#94780=CARTESIAN_POINT('Ctrl Pts',(-36.0397189421617,60.4806895737643,0.));
#94781=CARTESIAN_POINT('Ctrl Pts',(-36.0397189421617,60.4806895737643,12.));
#94782=CARTESIAN_POINT('Ctrl Pts',(-36.0547232187681,60.4947416988396,0.));
#94783=CARTESIAN_POINT('Ctrl Pts',(-36.0547232187681,60.4947416988396,12.));
#94784=CARTESIAN_POINT('Ctrl Pts',(-36.0697797118377,60.5088129911357,0.));
#94785=CARTESIAN_POINT('Ctrl Pts',(-36.0697797118377,60.5088129911357,12.));
#94786=CARTESIAN_POINT('Ctrl Pts',(-36.0848883531968,60.5229032759001,0.));
#94787=CARTESIAN_POINT('Ctrl Pts',(-36.0848883531968,60.5229032759001,12.));
#94788=CARTESIAN_POINT('Ctrl Pts',(-36.1000490738532,60.5370123768841,0.));
#94789=CARTESIAN_POINT('Ctrl Pts',(-36.1000490738532,60.5370123768841,12.));
#94790=CARTESIAN_POINT('Ctrl Pts',(-36.1152618043756,60.5511401172014,0.));
#94791=CARTESIAN_POINT('Ctrl Pts',(-36.1152618043756,60.5511401172014,12.));
#94792=CARTESIAN_POINT('Ctrl Pts',(-36.1305264752195,60.5652863200732,0.));
#94793=CARTESIAN_POINT('Ctrl Pts',(-36.1305264752195,60.5652863200732,12.));
#94794=CARTESIAN_POINT('Ctrl Pts',(-36.1458430170425,60.5794508095555,0.));
#94795=CARTESIAN_POINT('Ctrl Pts',(-36.1458430170425,60.5794508095555,12.));
#94796=CARTESIAN_POINT('Ctrl Pts',(-36.1612113610758,60.5936334114083,0.));
#94797=CARTESIAN_POINT('Ctrl Pts',(-36.1612113610758,60.5936334114083,12.));
#94798=CARTESIAN_POINT('Ctrl Pts',(-36.1766314392624,60.6078339534151,0.));
#94799=CARTESIAN_POINT('Ctrl Pts',(-36.1766314392624,60.6078339534151,12.));
#94800=CARTESIAN_POINT('Ctrl Pts',(-36.1921031840617,60.6220522649129,0.));
#94801=CARTESIAN_POINT('Ctrl Pts',(-36.1921031840617,60.6220522649129,12.));
#94802=CARTESIAN_POINT('Ctrl Pts',(-36.2076265283261,60.6362881765014,0.));
#94803=CARTESIAN_POINT('Ctrl Pts',(-36.2076265283261,60.6362881765014,12.));
#94804=CARTESIAN_POINT('Ctrl Pts',(-36.2232014051549,60.6505415197055,0.));
#94805=CARTESIAN_POINT('Ctrl Pts',(-36.2232014051549,60.6505415197055,12.));
#94806=CARTESIAN_POINT('Ctrl Pts',(-36.2388277477225,60.6648121265908,0.));
#94807=CARTESIAN_POINT('Ctrl Pts',(-36.2388277477225,60.6648121265908,12.));
#94808=CARTESIAN_POINT('Ctrl Pts',(-36.2545054892911,60.6790998297823,0.));
#94809=CARTESIAN_POINT('Ctrl Pts',(-36.2545054892911,60.6790998297823,12.));
#94810=CARTESIAN_POINT('Ctrl Pts',(-36.2702345632882,60.6934044626304,0.));
#94811=CARTESIAN_POINT('Ctrl Pts',(-36.2702345632882,60.6934044626304,12.));
#94812=CARTESIAN_POINT('Ctrl Pts',(-36.2860149033586,60.7077258593268,0.));
#94813=CARTESIAN_POINT('Ctrl Pts',(-36.2860149033586,60.7077258593268,12.));
#94814=CARTESIAN_POINT('Ctrl Pts',(-36.3018464434204,60.7220638550396,0.));
#94815=CARTESIAN_POINT('Ctrl Pts',(-36.3018464434204,60.7220638550396,12.));
#94816=CARTESIAN_POINT('Ctrl Pts',(-36.3177291177148,60.7364182860388,0.));
#94817=CARTESIAN_POINT('Ctrl Pts',(-36.3177291177148,60.7364182860388,12.));
#94818=CARTESIAN_POINT('Ctrl Pts',(-36.3336628607844,60.7507889896283,0.));
#94819=CARTESIAN_POINT('Ctrl Pts',(-36.3336628607844,60.7507889896283,12.));
#94820=CARTESIAN_POINT('Ctrl Pts',(-36.349647607448,60.7651758040791,0.));
#94821=CARTESIAN_POINT('Ctrl Pts',(-36.349647607448,60.7651758040791,12.));
#94822=CARTESIAN_POINT('Ctrl Pts',(-36.3656832927733,60.7795785685631,0.));
#94823=CARTESIAN_POINT('Ctrl Pts',(-36.3656832927733,60.7795785685631,12.));
#94824=CARTESIAN_POINT('Ctrl Pts',(-36.38176985204,60.7939971230781,0.));
#94825=CARTESIAN_POINT('Ctrl Pts',(-36.38176985204,60.7939971230781,12.));
#94826=CARTESIAN_POINT('Ctrl Pts',(-36.3979072207174,60.8084313084009,0.));
#94827=CARTESIAN_POINT('Ctrl Pts',(-36.3979072207174,60.8084313084009,12.));
#94828=CARTESIAN_POINT('Ctrl Pts',(-36.4140953344869,60.8228809661179,0.));
#94829=CARTESIAN_POINT('Ctrl Pts',(-36.4140953344869,60.8228809661179,12.));
#94830=CARTESIAN_POINT('Ctrl Pts',(-36.4303341292497,60.8373459386397,0.));
#94831=CARTESIAN_POINT('Ctrl Pts',(-36.4303341292497,60.8373459386397,12.));
#94832=CARTESIAN_POINT('Ctrl Pts',(-36.4466235411353,60.851826069218,0.));
#94833=CARTESIAN_POINT('Ctrl Pts',(-36.4466235411353,60.851826069218,12.));
#94834=CARTESIAN_POINT('Ctrl Pts',(-36.4629635065037,60.8663212019646,0.));
#94835=CARTESIAN_POINT('Ctrl Pts',(-36.4629635065037,60.8663212019646,12.));
#94836=CARTESIAN_POINT('Ctrl Pts',(-36.4793539619459,60.8808311818489,0.));
#94837=CARTESIAN_POINT('Ctrl Pts',(-36.4793539619459,60.8808311818489,12.));
#94838=CARTESIAN_POINT('Ctrl Pts',(-36.4957948442832,60.8953558546791,0.));
#94839=CARTESIAN_POINT('Ctrl Pts',(-36.4957948442832,60.8953558546791,12.));
#94840=CARTESIAN_POINT('Ctrl Pts',(-36.5122860905611,60.9098950670847,0.));
#94841=CARTESIAN_POINT('Ctrl Pts',(-36.5122860905611,60.9098950670847,12.));
#94842=CARTESIAN_POINT('Ctrl Pts',(-36.5288276380417,60.924448666499,0.));
#94843=CARTESIAN_POINT('Ctrl Pts',(-36.5288276380417,60.924448666499,12.));
#94844=CARTESIAN_POINT('Ctrl Pts',(-36.5454194241866,60.9390165011357,0.));
#94845=CARTESIAN_POINT('Ctrl Pts',(-36.5454194241866,60.9390165011357,12.));
#94846=CARTESIAN_POINT('Ctrl Pts',(-36.5620613866615,60.9535984199874,0.));
#94847=CARTESIAN_POINT('Ctrl Pts',(-36.5620613866615,60.9535984199874,12.));
#94848=CARTESIAN_POINT('Ctrl Pts',(-36.5787534633416,60.9681942728237,0.));
#94849=CARTESIAN_POINT('Ctrl Pts',(-36.5787534633416,60.9681942728237,12.));
#94850=CARTESIAN_POINT('Ctrl Pts',(-36.5954955923109,60.9828039101887,0.));
#94851=CARTESIAN_POINT('Ctrl Pts',(-36.5954955923109,60.9828039101887,12.));
#94852=CARTESIAN_POINT('Ctrl Pts',(-36.6122877118599,60.9974271833982,0.));
#94853=CARTESIAN_POINT('Ctrl Pts',(-36.6122877118599,60.9974271833982,12.));
#94854=CARTESIAN_POINT('Ctrl Pts',(-36.6291297604775,61.012063944535,0.));
#94855=CARTESIAN_POINT('Ctrl Pts',(-36.6291297604775,61.012063944535,12.));
#94856=CARTESIAN_POINT('Ctrl Pts',(-36.6460216768553,61.0267140464434,0.));
#94857=CARTESIAN_POINT('Ctrl Pts',(-36.6460216768553,61.0267140464434,12.));
#94858=CARTESIAN_POINT('Ctrl Pts',(-36.6629633998885,61.0413773427204,0.));
#94859=CARTESIAN_POINT('Ctrl Pts',(-36.6629633998885,61.0413773427204,12.));
#94860=CARTESIAN_POINT('Ctrl Pts',(-36.6799548686741,61.0560536877084,0.));
#94861=CARTESIAN_POINT('Ctrl Pts',(-36.6799548686741,61.0560536877084,12.));
#94862=CARTESIAN_POINT('Ctrl Pts',(-36.6969960225019,61.0707429364841,0.));
#94863=CARTESIAN_POINT('Ctrl Pts',(-36.6969960225019,61.0707429364841,12.));
#94864=CARTESIAN_POINT('Ctrl Pts',(-36.7140868008479,61.085444944851,0.));
#94865=CARTESIAN_POINT('Ctrl Pts',(-36.7140868008479,61.085444944851,12.));
#94866=CARTESIAN_POINT('Ctrl Pts',(-36.7312271433799,61.1001595693357,0.));
#94867=CARTESIAN_POINT('Ctrl Pts',(-36.7312271433799,61.1001595693357,12.));
#94868=CARTESIAN_POINT('Ctrl Pts',(-36.7484169899591,61.1148866671821,0.));
#94869=CARTESIAN_POINT('Ctrl Pts',(-36.7484169899591,61.1148866671821,12.));
#94870=CARTESIAN_POINT('Ctrl Pts',(-36.7656562806381,61.1296260963468,0.));
#94871=CARTESIAN_POINT('Ctrl Pts',(-36.7656562806381,61.1296260963468,12.));
#94872=CARTESIAN_POINT('Ctrl Pts',(-36.782944955654,61.1443777154926,0.));
#94873=CARTESIAN_POINT('Ctrl Pts',(-36.782944955654,61.1443777154926,12.));
#94874=CARTESIAN_POINT('Ctrl Pts',(-36.8002829554221,61.1591413839809,0.));
#94875=CARTESIAN_POINT('Ctrl Pts',(-36.8002829554221,61.1591413839809,12.));
#94876=CARTESIAN_POINT('Ctrl Pts',(-36.8176702205436,61.1739169618688,0.));
#94877=CARTESIAN_POINT('Ctrl Pts',(-36.8176702205436,61.1739169618688,12.));
#94878=CARTESIAN_POINT('Ctrl Pts',(-36.8351066918043,61.1887043099026,0.));
#94879=CARTESIAN_POINT('Ctrl Pts',(-36.8351066918043,61.1887043099026,12.));
#94880=CARTESIAN_POINT('Ctrl Pts',(-36.8525923101736,61.2035032895121,0.));
#94881=CARTESIAN_POINT('Ctrl Pts',(-36.8525923101736,61.2035032895121,12.));
#94882=CARTESIAN_POINT('Ctrl Pts',(-36.8701270167954,61.2183137628031,0.));
#94883=CARTESIAN_POINT('Ctrl Pts',(-36.8701270167954,61.2183137628031,12.));
#94884=CARTESIAN_POINT('Ctrl Pts',(-36.8877107529844,61.2331355925513,0.));
#94885=CARTESIAN_POINT('Ctrl Pts',(-36.8877107529844,61.2331355925513,12.));
#94886=CARTESIAN_POINT('Ctrl Pts',(-36.9053434602324,61.2479686421979,0.));
#94887=CARTESIAN_POINT('Ctrl Pts',(-36.9053434602324,61.2479686421979,12.));
#94888=CARTESIAN_POINT('Ctrl Pts',(-36.9230250802078,61.2628127758443,0.));
#94889=CARTESIAN_POINT('Ctrl Pts',(-36.9230250802078,61.2628127758443,12.));
#94890=CARTESIAN_POINT('Ctrl Pts',(-36.9407555547542,61.2776678582474,0.));
#94891=CARTESIAN_POINT('Ctrl Pts',(-36.9407555547542,61.2776678582474,12.));
#94892=CARTESIAN_POINT('Ctrl Pts',(-36.9585348258798,61.2925337548113,0.));
#94893=CARTESIAN_POINT('Ctrl Pts',(-36.9585348258798,61.2925337548113,12.));
#94894=CARTESIAN_POINT('Ctrl Pts',(-36.976362835757,61.3074103315834,0.));
#94895=CARTESIAN_POINT('Ctrl Pts',(-36.976362835757,61.3074103315834,12.));
#94896=CARTESIAN_POINT('Ctrl Pts',(-36.994239526729,61.3222974552519,0.));
#94897=CARTESIAN_POINT('Ctrl Pts',(-36.994239526729,61.3222974552519,12.));
#94898=CARTESIAN_POINT('Ctrl Pts',(-37.0121648413088,61.3371949931396,0.));
#94899=CARTESIAN_POINT('Ctrl Pts',(-37.0121648413088,61.3371949931396,12.));
#94900=CARTESIAN_POINT('Ctrl Pts',(-37.0301387221766,61.352102813199,0.));
#94901=CARTESIAN_POINT('Ctrl Pts',(-37.0301387221766,61.352102813199,12.));
#94902=CARTESIAN_POINT('Ctrl Pts',(-37.0481611121698,61.3670207840041,0.));
#94903=CARTESIAN_POINT('Ctrl Pts',(-37.0481611121698,61.3670207840041,12.));
#94904=CARTESIAN_POINT('Ctrl Pts',(-37.0662319542827,61.3819487747458,0.));
#94905=CARTESIAN_POINT('Ctrl Pts',(-37.0662319542827,61.3819487747458,12.));
#94906=CARTESIAN_POINT('Ctrl Pts',(-37.0843511916728,61.3968866552294,0.));
#94907=CARTESIAN_POINT('Ctrl Pts',(-37.0843511916728,61.3968866552294,12.));
#94908=CARTESIAN_POINT('Ctrl Pts',(-37.1025187676597,61.411834295869,0.));
#94909=CARTESIAN_POINT('Ctrl Pts',(-37.1025187676597,61.411834295869,12.));
#94910=CARTESIAN_POINT('Ctrl Pts',(-37.1207346257228,61.4267915676834,0.));
#94911=CARTESIAN_POINT('Ctrl Pts',(-37.1207346257228,61.4267915676834,12.));
#94912=CARTESIAN_POINT('Ctrl Pts',(-37.138998709492,61.4417583422888,0.));
#94913=CARTESIAN_POINT('Ctrl Pts',(-37.138998709492,61.4417583422888,12.));
#94914=CARTESIAN_POINT('Ctrl Pts',(-37.157310962747,61.4567344918946,0.));
#94915=CARTESIAN_POINT('Ctrl Pts',(-37.157310962747,61.4567344918946,12.));
#94916=CARTESIAN_POINT('Ctrl Pts',(-37.1756713294249,61.471719889301,0.));
#94917=CARTESIAN_POINT('Ctrl Pts',(-37.1756713294249,61.471719889301,12.));
#94918=CARTESIAN_POINT('Ctrl Pts',(-37.1940797536182,61.4867144078939,0.));
#94919=CARTESIAN_POINT('Ctrl Pts',(-37.1940797536182,61.4867144078939,12.));
#94920=CARTESIAN_POINT('Ctrl Pts',(-37.2125361795727,61.5017179216404,0.));
#94921=CARTESIAN_POINT('Ctrl Pts',(-37.2125361795727,61.5017179216404,12.));
#94922=CARTESIAN_POINT('Ctrl Pts',(-37.2310405516775,61.5167303050823,0.));
#94923=CARTESIAN_POINT('Ctrl Pts',(-37.2310405516775,61.5167303050823,12.));
#94924=CARTESIAN_POINT('Ctrl Pts',(-37.2495928144661,61.5317514333319,0.));
#94925=CARTESIAN_POINT('Ctrl Pts',(-37.2495928144661,61.5317514333319,12.));
#94926=CARTESIAN_POINT('Ctrl Pts',(-37.2681929126218,61.5467811820686,0.));
#94927=CARTESIAN_POINT('Ctrl Pts',(-37.2681929126218,61.5467811820686,12.));
#94928=CARTESIAN_POINT('Ctrl Pts',(-37.286840790977,61.5618194275349,0.));
#94929=CARTESIAN_POINT('Ctrl Pts',(-37.286840790977,61.5618194275349,12.));
#94930=CARTESIAN_POINT('Ctrl Pts',(-37.3055363945108,61.5768660465313,0.));
#94931=CARTESIAN_POINT('Ctrl Pts',(-37.3055363945108,61.5768660465313,12.));
#94932=CARTESIAN_POINT('Ctrl Pts',(-37.3242796683395,61.591920916412,0.));
#94933=CARTESIAN_POINT('Ctrl Pts',(-37.3242796683395,61.591920916412,12.));
#94934=CARTESIAN_POINT('Ctrl Pts',(-37.3430705577178,61.6069839150804,0.));
#94935=CARTESIAN_POINT('Ctrl Pts',(-37.3430705577178,61.6069839150804,12.));
#94936=CARTESIAN_POINT('Ctrl Pts',(-37.3619090080447,61.6220549209862,0.));
#94937=CARTESIAN_POINT('Ctrl Pts',(-37.3619090080447,61.6220549209862,12.));
#94938=CARTESIAN_POINT('Ctrl Pts',(-37.3807949648622,61.6371338131208,0.));
#94939=CARTESIAN_POINT('Ctrl Pts',(-37.3807949648622,61.6371338131208,12.));
#94940=CARTESIAN_POINT('Ctrl Pts',(-37.3997283738534,61.6522204710133,0.));
#94941=CARTESIAN_POINT('Ctrl Pts',(-37.3997283738534,61.6522204710133,12.));
#94942=CARTESIAN_POINT('Ctrl Pts',(-37.4187091808324,61.667314774725,0.));
#94943=CARTESIAN_POINT('Ctrl Pts',(-37.4187091808324,61.667314774725,12.));
#94944=CARTESIAN_POINT('Ctrl Pts',(-37.4377373317456,61.6824166048453,0.));
#94945=CARTESIAN_POINT('Ctrl Pts',(-37.4377373317456,61.6824166048453,12.));
#94946=CARTESIAN_POINT('Ctrl Pts',(-37.4568127726776,61.69752584249,0.));
#94947=CARTESIAN_POINT('Ctrl Pts',(-37.4568127726776,61.69752584249,12.));
#94948=CARTESIAN_POINT('Ctrl Pts',(-37.4759354498509,61.7126423692965,0.));
#94949=CARTESIAN_POINT('Ctrl Pts',(-37.4759354498509,61.7126423692965,12.));
#94950=CARTESIAN_POINT('Ctrl Pts',(-37.4951053096235,61.7277660674203,0.));
#94951=CARTESIAN_POINT('Ctrl Pts',(-37.4951053096235,61.7277660674203,12.));
#94952=CARTESIAN_POINT('Ctrl Pts',(-37.5143222984794,61.7428968195296,0.));
#94953=CARTESIAN_POINT('Ctrl Pts',(-37.5143222984794,61.7428968195296,12.));
#94954=CARTESIAN_POINT('Ctrl Pts',(-37.5335863630286,61.7580345088014,0.));
#94955=CARTESIAN_POINT('Ctrl Pts',(-37.5335863630286,61.7580345088014,12.));
#94956=CARTESIAN_POINT('Ctrl Pts',(-37.5528974500142,61.7731790189191,0.));
#94957=CARTESIAN_POINT('Ctrl Pts',(-37.5528974500142,61.7731790189191,12.));
#94958=CARTESIAN_POINT('Ctrl Pts',(-37.5722555063112,61.7883302340689,0.));
#94959=CARTESIAN_POINT('Ctrl Pts',(-37.5722555063112,61.7883302340689,12.));
#94960=CARTESIAN_POINT('Ctrl Pts',(-37.5916604789252,61.8034880389362,0.));
#94961=CARTESIAN_POINT('Ctrl Pts',(-37.5916604789252,61.8034880389362,12.));
#94962=CARTESIAN_POINT('Ctrl Pts',(-37.6111123149836,61.8186523187011,0.));
#94963=CARTESIAN_POINT('Ctrl Pts',(-37.6111123149836,61.8186523187011,12.));
#94964=CARTESIAN_POINT('Ctrl Pts',(-37.6306109617341,61.8338229590345,0.));
#94965=CARTESIAN_POINT('Ctrl Pts',(-37.6306109617341,61.8338229590345,12.));
#94966=CARTESIAN_POINT('Ctrl Pts',(-37.6501563665518,61.848999846095,0.));
#94967=CARTESIAN_POINT('Ctrl Pts',(-37.6501563665518,61.848999846095,12.));
#94968=CARTESIAN_POINT('Ctrl Pts',(-37.6697484769389,61.8641828665257,0.));
#94969=CARTESIAN_POINT('Ctrl Pts',(-37.6697484769389,61.8641828665257,12.));
#94970=CARTESIAN_POINT('Ctrl Pts',(-37.6893872405229,61.879371907451,0.));
#94971=CARTESIAN_POINT('Ctrl Pts',(-37.6893872405229,61.879371907451,12.));
#94972=CARTESIAN_POINT('Ctrl Pts',(-37.7090726050488,61.8945668564714,0.));
#94973=CARTESIAN_POINT('Ctrl Pts',(-37.7090726050488,61.8945668564714,12.));
#94974=CARTESIAN_POINT('Ctrl Pts',(-37.7288045183765,61.9097676016616,0.));
#94975=CARTESIAN_POINT('Ctrl Pts',(-37.7288045183765,61.9097676016616,12.));
#94976=CARTESIAN_POINT('Ctrl Pts',(-37.748582928488,61.9249740315664,0.));
#94977=CARTESIAN_POINT('Ctrl Pts',(-37.748582928488,61.9249740315664,12.));
#94978=CARTESIAN_POINT('Ctrl Pts',(-37.7684077834877,61.940186035198,0.));
#94979=CARTESIAN_POINT('Ctrl Pts',(-37.7684077834877,61.940186035198,12.));
#94980=CARTESIAN_POINT('Ctrl Pts',(-37.7882790316012,61.9554035020335,0.));
#94981=CARTESIAN_POINT('Ctrl Pts',(-37.7882790316012,61.9554035020335,12.));
#94982=CARTESIAN_POINT('Ctrl Pts',(-37.808196621168,61.9706263220101,0.));
#94983=CARTESIAN_POINT('Ctrl Pts',(-37.808196621168,61.9706263220101,12.));
#94984=CARTESIAN_POINT('Ctrl Pts',(-37.8281605006371,61.9858543855221,0.));
#94985=CARTESIAN_POINT('Ctrl Pts',(-37.8281605006371,61.9858543855221,12.));
#94986=CARTESIAN_POINT('Ctrl Pts',(-37.8481706185742,62.0010875834176,0.));
#94987=CARTESIAN_POINT('Ctrl Pts',(-37.8481706185742,62.0010875834176,12.));
#94988=CARTESIAN_POINT('Ctrl Pts',(-37.8682269236628,62.0163258069954,0.));
#94989=CARTESIAN_POINT('Ctrl Pts',(-37.8682269236628,62.0163258069954,12.));
#94990=CARTESIAN_POINT('Ctrl Pts',(-37.888329364703,62.0315689480022,0.));
#94991=CARTESIAN_POINT('Ctrl Pts',(-37.888329364703,62.0315689480022,12.));
#94992=CARTESIAN_POINT('Ctrl Pts',(-37.9084778906053,62.0468168986289,0.));
#94993=CARTESIAN_POINT('Ctrl Pts',(-37.9084778906053,62.0468168986289,12.));
#94994=CARTESIAN_POINT('Ctrl Pts',(-37.9286724503849,62.0620695515072,0.));
#94995=CARTESIAN_POINT('Ctrl Pts',(-37.9286724503849,62.0620695515072,12.));
#94996=CARTESIAN_POINT('Ctrl Pts',(-37.9489129931685,62.0773267997072,0.));
#94997=CARTESIAN_POINT('Ctrl Pts',(-37.9489129931685,62.0773267997072,12.));
#94998=CARTESIAN_POINT('Ctrl Pts',(-37.9691994681962,62.0925885367346,0.));
#94999=CARTESIAN_POINT('Ctrl Pts',(-37.9691994681962,62.0925885367346,12.));
#95000=CARTESIAN_POINT('Ctrl Pts',(-37.9895318248212,62.107854656528,0.));
#95001=CARTESIAN_POINT('Ctrl Pts',(-37.9895318248212,62.107854656528,12.));
#95002=CARTESIAN_POINT('Ctrl Pts',(-38.0099100125041,62.1231250534558,0.));
#95003=CARTESIAN_POINT('Ctrl Pts',(-38.0099100125041,62.1231250534558,12.));
#95004=CARTESIAN_POINT('Ctrl Pts',(-38.0303339808059,62.1383996223136,0.));
#95005=CARTESIAN_POINT('Ctrl Pts',(-38.0303339808059,62.1383996223136,12.));
#95006=CARTESIAN_POINT('Ctrl Pts',(-38.0508036793944,62.153678258321,0.));
#95007=CARTESIAN_POINT('Ctrl Pts',(-38.0508036793944,62.153678258321,12.));
#95008=CARTESIAN_POINT('Ctrl Pts',(-38.0713190580466,62.1689608571182,0.));
#95009=CARTESIAN_POINT('Ctrl Pts',(-38.0713190580466,62.1689608571182,12.));
#95010=CARTESIAN_POINT('Ctrl Pts',(-38.0918800666479,62.1842473147627,0.));
#95011=CARTESIAN_POINT('Ctrl Pts',(-38.0918800666479,62.1842473147627,12.));
#95012=CARTESIAN_POINT('Ctrl Pts',(-38.1124866551883,62.1995375277253,0.));
#95013=CARTESIAN_POINT('Ctrl Pts',(-38.1124866551883,62.1995375277253,12.));
#95014=CARTESIAN_POINT('Ctrl Pts',(-38.1331387737528,62.2148313928859,0.));
#95015=CARTESIAN_POINT('Ctrl Pts',(-38.1331387737528,62.2148313928859,12.));
#95016=CARTESIAN_POINT('Ctrl Pts',(-38.1538363725263,62.2301288075319,0.));
#95017=CARTESIAN_POINT('Ctrl Pts',(-38.1538363725263,62.2301288075319,12.));
#95018=CARTESIAN_POINT('Ctrl Pts',(-38.1745794017997,62.2454296693581,0.));
#95019=CARTESIAN_POINT('Ctrl Pts',(-38.1745794017997,62.2454296693581,12.));
#95020=CARTESIAN_POINT('Ctrl Pts',(-38.1953678119692,62.2607338764655,0.));
#95021=CARTESIAN_POINT('Ctrl Pts',(-38.1953678119692,62.2607338764655,12.));
#95022=CARTESIAN_POINT('Ctrl Pts',(-38.2162015535351,62.2760413273601,0.));
#95023=CARTESIAN_POINT('Ctrl Pts',(-38.2162015535351,62.2760413273601,12.));
#95024=CARTESIAN_POINT('Ctrl Pts',(-38.2370805770931,62.2913519209517,0.));
#95025=CARTESIAN_POINT('Ctrl Pts',(-38.2370805770931,62.2913519209517,12.));
#95026=CARTESIAN_POINT('Ctrl Pts',(-38.2580048333356,62.3066655565497,0.));
#95027=CARTESIAN_POINT('Ctrl Pts',(-38.2580048333356,62.3066655565497,12.));
#95028=CARTESIAN_POINT('Ctrl Pts',(-38.2789742730559,62.3219821338564,0.));
#95029=CARTESIAN_POINT('Ctrl Pts',(-38.2789742730559,62.3219821338564,12.));
#95030=CARTESIAN_POINT('Ctrl Pts',(-38.2999888471474,62.337301552961,0.));
#95031=CARTESIAN_POINT('Ctrl Pts',(-38.2999888471474,62.337301552961,12.));
#95032=CARTESIAN_POINT('Ctrl Pts',(-38.3210485066003,62.3526237143338,0.));
#95033=CARTESIAN_POINT('Ctrl Pts',(-38.3210485066003,62.3526237143338,12.));
#95034=CARTESIAN_POINT('Ctrl Pts',(-38.3421532024915,62.3679485188178,0.));
#95035=CARTESIAN_POINT('Ctrl Pts',(-38.3421532024915,62.3679485188178,12.));
#95036=CARTESIAN_POINT('Ctrl Pts',(-38.3633028859835,62.3832758676281,0.));
#95037=CARTESIAN_POINT('Ctrl Pts',(-38.3633028859835,62.3832758676281,12.));
#95038=CARTESIAN_POINT('Ctrl Pts',(-38.384497508335,62.3986056623587,0.));
#95039=CARTESIAN_POINT('Ctrl Pts',(-38.384497508335,62.3986056623587,12.));
#95040=CARTESIAN_POINT('Ctrl Pts',(-38.4057370209054,62.4139378049891,0.));
#95041=CARTESIAN_POINT('Ctrl Pts',(-38.4057370209054,62.4139378049891,12.));
#95042=CARTESIAN_POINT('Ctrl Pts',(-38.4270213751567,62.42927219789,0.));
#95043=CARTESIAN_POINT('Ctrl Pts',(-38.4270213751567,62.42927219789,12.));
#95044=CARTESIAN_POINT('Ctrl Pts',(-38.4483505226511,62.4446087438304,0.));
#95045=CARTESIAN_POINT('Ctrl Pts',(-38.4483505226511,62.4446087438304,12.));
#95046=CARTESIAN_POINT('Ctrl Pts',(-38.4697244150473,62.4599473459799,0.));
#95047=CARTESIAN_POINT('Ctrl Pts',(-38.4697244150473,62.4599473459799,12.));
#95048=CARTESIAN_POINT('Ctrl Pts',(-38.4911430040988,62.4752879078842,0.));
#95049=CARTESIAN_POINT('Ctrl Pts',(-38.4911430040988,62.4752879078842,12.));
#95050=CARTESIAN_POINT('Ctrl Pts',(-38.5126062416496,62.4906303334435,0.));
#95051=CARTESIAN_POINT('Ctrl Pts',(-38.5126062416496,62.4906303334435,12.));
#95052=CARTESIAN_POINT('Ctrl Pts',(-38.5341140796247,62.50597452689,0.));
#95053=CARTESIAN_POINT('Ctrl Pts',(-38.5341140796247,62.50597452689,12.));
#95054=CARTESIAN_POINT('Ctrl Pts',(-38.5556664700201,62.5213203927672,0.));
#95055=CARTESIAN_POINT('Ctrl Pts',(-38.5556664700201,62.5213203927672,12.));
#95056=CARTESIAN_POINT('Ctrl Pts',(-38.5772633648841,62.5366678359036,0.));
#95057=CARTESIAN_POINT('Ctrl Pts',(-38.5772633648841,62.5366678359036,12.));
#95058=CARTESIAN_POINT('Ctrl Pts',(-38.5989047163401,62.5520167614529,0.));
#95059=CARTESIAN_POINT('Ctrl Pts',(-38.5989047163401,62.5520167614529,12.));
#95060=CARTESIAN_POINT('Ctrl Pts',(-38.6205904766078,62.567367074937,0.));
#95061=CARTESIAN_POINT('Ctrl Pts',(-38.6205904766078,62.567367074937,12.));
#95062=CARTESIAN_POINT('Ctrl Pts',(-38.6423205980214,62.5827186822923,0.));
#95063=CARTESIAN_POINT('Ctrl Pts',(-38.6423205980214,62.5827186822923,12.));
#95064=CARTESIAN_POINT('Ctrl Pts',(-38.6640950330418,62.5980714899048,0.));
#95065=CARTESIAN_POINT('Ctrl Pts',(-38.6640950330418,62.5980714899048,12.));
#95066=CARTESIAN_POINT('Ctrl Pts',(-38.6859137342726,62.6134254046732,0.));
#95067=CARTESIAN_POINT('Ctrl Pts',(-38.6859137342726,62.6134254046732,12.));
#95068=CARTESIAN_POINT('Ctrl Pts',(-38.7077766544411,62.6287803339534,0.));
#95069=CARTESIAN_POINT('Ctrl Pts',(-38.7077766544411,62.6287803339534,12.));
#95070=CARTESIAN_POINT('Ctrl Pts',(-38.7296837463605,62.6441361854406,0.));
#95071=CARTESIAN_POINT('Ctrl Pts',(-38.7296837463605,62.6441361854406,12.));
#95072=CARTESIAN_POINT('Ctrl Pts',(-38.7516349628902,62.6594928670626,0.));
#95073=CARTESIAN_POINT('Ctrl Pts',(-38.7516349628902,62.6594928670626,12.));
#95074=CARTESIAN_POINT('Ctrl Pts',(-38.7736302568982,62.6748502868836,0.));
#95075=CARTESIAN_POINT('Ctrl Pts',(-38.7736302568982,62.6748502868836,12.));
#95076=CARTESIAN_POINT('Ctrl Pts',(-38.7956695812032,62.6902083529698,0.));
#95077=CARTESIAN_POINT('Ctrl Pts',(-38.7956695812032,62.6902083529698,12.));
#95078=CARTESIAN_POINT('Ctrl Pts',(-38.8177528885686,62.7055669733811,0.));
#95079=CARTESIAN_POINT('Ctrl Pts',(-38.8177528885686,62.7055669733811,12.));
#95080=CARTESIAN_POINT('Ctrl Pts',(-38.8398801318184,62.7209260564506,0.));
#95081=CARTESIAN_POINT('Ctrl Pts',(-38.8398801318184,62.7209260564506,12.));
#95082=CARTESIAN_POINT('Ctrl Pts',(-38.8620512639239,62.7362855110052,0.));
#95083=CARTESIAN_POINT('Ctrl Pts',(-38.8620512639239,62.7362855110052,12.));
#95084=CARTESIAN_POINT('Ctrl Pts',(-38.8842662380984,62.7516452466129,0.));
#95085=CARTESIAN_POINT('Ctrl Pts',(-38.8842662380984,62.7516452466129,12.));
#95086=CARTESIAN_POINT('Ctrl Pts',(-38.9065250078824,62.7670051738132,0.));
#95087=CARTESIAN_POINT('Ctrl Pts',(-38.9065250078824,62.7670051738132,12.));
#95088=CARTESIAN_POINT('Ctrl Pts',(-38.928827527232,62.7823652043677,0.));
#95089=CARTESIAN_POINT('Ctrl Pts',(-38.928827527232,62.7823652043677,12.));
#95090=CARTESIAN_POINT('Ctrl Pts',(-38.9511737503146,62.797725250709,0.));
#95091=CARTESIAN_POINT('Ctrl Pts',(-38.9511737503146,62.797725250709,12.));
#95092=CARTESIAN_POINT('Ctrl Pts',(-38.9735636313073,62.8130852254004,0.));
#95093=CARTESIAN_POINT('Ctrl Pts',(-38.9735636313073,62.8130852254004,12.));
#95094=CARTESIAN_POINT('Ctrl Pts',(-38.9959971241695,62.8284450405451,0.));
#95095=CARTESIAN_POINT('Ctrl Pts',(-38.9959971241695,62.8284450405451,12.));
#95096=CARTESIAN_POINT('Ctrl Pts',(-39.0184741824649,62.8438046073237,0.));
#95097=CARTESIAN_POINT('Ctrl Pts',(-39.0184741824649,62.8438046073237,12.));
#95098=CARTESIAN_POINT('Ctrl Pts',(-39.0409947590519,62.859163835209,0.));
#95099=CARTESIAN_POINT('Ctrl Pts',(-39.0409947590519,62.859163835209,12.));
#95100=CARTESIAN_POINT('Ctrl Pts',(-39.0635588063308,62.8745226326046,0.));
#95101=CARTESIAN_POINT('Ctrl Pts',(-39.0635588063308,62.8745226326046,12.));
#95102=CARTESIAN_POINT('Ctrl Pts',(-39.0861662767964,62.8898809082659,0.));
#95103=CARTESIAN_POINT('Ctrl Pts',(-39.0861662767964,62.8898809082659,12.));
#95104=CARTESIAN_POINT('Ctrl Pts',(-39.1088171235144,62.9052385725416,0.));
#95105=CARTESIAN_POINT('Ctrl Pts',(-39.1088171235144,62.9052385725416,12.));
#95106=CARTESIAN_POINT('Ctrl Pts',(-39.1315113005745,62.9205955385551,0.));
#95107=CARTESIAN_POINT('Ctrl Pts',(-39.1315113005745,62.9205955385551,12.));
#95108=CARTESIAN_POINT('Ctrl Pts',(-39.1542487636708,62.9359517237352,0.));
#95109=CARTESIAN_POINT('Ctrl Pts',(-39.1542487636708,62.9359517237352,12.));
#95110=CARTESIAN_POINT('Ctrl Pts',(-39.1770294702367,62.9513070501777,0.));
#95111=CARTESIAN_POINT('Ctrl Pts',(-39.1770294702367,62.9513070501777,12.));
#95112=CARTESIAN_POINT('Ctrl Pts',(-39.199853378159,62.9666614412627,0.));
#95113=CARTESIAN_POINT('Ctrl Pts',(-39.199853378159,62.9666614412627,12.));
#95114=CARTESIAN_POINT('Ctrl Pts',(-39.2227204447583,62.9820148189849,0.));
#95115=CARTESIAN_POINT('Ctrl Pts',(-39.2227204447583,62.9820148189849,12.));
#95116=CARTESIAN_POINT('Ctrl Pts',(-39.2456306256092,62.9973671008685,0.));
#95117=CARTESIAN_POINT('Ctrl Pts',(-39.2456306256092,62.9973671008685,12.));
#95118=CARTESIAN_POINT('Ctrl Pts',(-39.268583873541,63.0127181973702,0.));
#95119=CARTESIAN_POINT('Ctrl Pts',(-39.268583873541,63.0127181973702,12.));
#95120=CARTESIAN_POINT('Ctrl Pts',(-39.2915801372468,63.0280680082522,0.));
#95121=CARTESIAN_POINT('Ctrl Pts',(-39.2915801372468,63.0280680082522,12.));
#95122=CARTESIAN_POINT('Ctrl Pts',(-39.3146193632546,63.0434164278221,0.));
#95123=CARTESIAN_POINT('Ctrl Pts',(-39.3146193632546,63.0434164278221,12.));
#95124=CARTESIAN_POINT('Ctrl Pts',(-39.3377014983757,63.0587633513993,0.));
#95125=CARTESIAN_POINT('Ctrl Pts',(-39.3377014983757,63.0587633513993,12.));
#95126=CARTESIAN_POINT('Ctrl Pts',(-39.3608264920487,63.0741086815957,0.));
#95127=CARTESIAN_POINT('Ctrl Pts',(-39.3608264920487,63.0741086815957,12.));
#95128=CARTESIAN_POINT('Ctrl Pts',(-39.3839942985688,63.0894523341238,0.));
#95129=CARTESIAN_POINT('Ctrl Pts',(-39.3839942985688,63.0894523341238,12.));
#95130=CARTESIAN_POINT('Ctrl Pts',(-39.4072048797401,63.1047942451583,0.));
#95131=CARTESIAN_POINT('Ctrl Pts',(-39.4072048797401,63.1047942451583,12.));
#95132=CARTESIAN_POINT('Ctrl Pts',(-39.4304582059507,63.1201343730643,0.));
#95133=CARTESIAN_POINT('Ctrl Pts',(-39.4304582059507,63.1201343730643,12.));
#95134=CARTESIAN_POINT('Ctrl Pts',(-39.4537542551852,63.1354726927781,0.));
#95135=CARTESIAN_POINT('Ctrl Pts',(-39.4537542551852,63.1354726927781,12.));
#95136=CARTESIAN_POINT('Ctrl Pts',(-39.4724252610807,63.147741892189,0.));
#95137=CARTESIAN_POINT('Ctrl Pts',(-39.4724252610807,63.147741892189,12.));
#95138=CARTESIAN_POINT('Ctrl Pts',(-39.4864477303613,63.1569429707564,0.));
#95139=CARTESIAN_POINT('Ctrl Pts',(-39.4864477303613,63.1569429707564,12.));
#95140=CARTESIAN_POINT('Ctrl Pts',(-39.4958045828059,63.1630766582674,0.));
#95141=CARTESIAN_POINT('Ctrl Pts',(-39.4958045828059,63.1630766582674,12.));
#95142=CARTESIAN_POINT('Ctrl Pts',(-39.5004851439257,63.1661434108059,0.));
#95143=CARTESIAN_POINT('Ctrl Pts',(-39.5004851439257,63.1661434108059,12.));
#95144=CARTESIAN_POINT('',(-35.7368311217509,60.1903555511633,0.));
#95145=CARTESIAN_POINT('Ctrl Pts',(-35.7368311217509,60.1903555511633,0.));
#95146=CARTESIAN_POINT('Ctrl Pts',(-35.7396040203973,60.1930746580239,0.));
#95147=CARTESIAN_POINT('Ctrl Pts',(-35.7451551752456,60.1985151474406,0.));
#95148=CARTESIAN_POINT('Ctrl Pts',(-35.7534979801871,60.2066827086579,0.));
#95149=CARTESIAN_POINT('Ctrl Pts',(-35.7646538667299,60.2175864449678,0.));
#95150=CARTESIAN_POINT('Ctrl Pts',(-35.7786523045782,60.2312388621286,0.));
#95151=CARTESIAN_POINT('Ctrl Pts',(-35.7927043145164,60.2449139865206,0.));
#95152=CARTESIAN_POINT('Ctrl Pts',(-35.8068098723386,60.2586117365278,0.));
#95153=CARTESIAN_POINT('Ctrl Pts',(-35.8209689272574,60.2723319687507,0.));
#95154=CARTESIAN_POINT('Ctrl Pts',(-35.8351814020424,60.2860744798563,0.));
#95155=CARTESIAN_POINT('Ctrl Pts',(-35.8494472046783,60.2998390330173,0.));
#95156=CARTESIAN_POINT('Ctrl Pts',(-35.8637662371635,60.313625378281,0.));
#95157=CARTESIAN_POINT('Ctrl Pts',(-35.878138405151,60.3274332746782,0.));
#95158=CARTESIAN_POINT('Ctrl Pts',(-35.8925636280632,60.3412625135223,0.));
#95159=CARTESIAN_POINT('Ctrl Pts',(-35.9070418358501,60.3551129108794,0.));
#95160=CARTESIAN_POINT('Ctrl Pts',(-35.9215729642219,60.368984296546,0.));
#95161=CARTESIAN_POINT('Ctrl Pts',(-35.9361569506955,60.3828765049031,0.));
#95162=CARTESIAN_POINT('Ctrl Pts',(-35.9507937296726,60.3967893635487,0.));
#95163=CARTESIAN_POINT('Ctrl Pts',(-35.9654832299627,60.4107226875759,0.));
#95164=CARTESIAN_POINT('Ctrl Pts',(-35.9802253773534,60.4246762854961,0.));
#95165=CARTESIAN_POINT('Ctrl Pts',(-35.9950200962175,60.438649962949,0.));
#95166=CARTESIAN_POINT('Ctrl Pts',(-36.0098673113556,60.452643526964,0.));
#95167=CARTESIAN_POINT('Ctrl Pts',(-36.0247669500867,60.4666567908053,0.));
#95168=CARTESIAN_POINT('Ctrl Pts',(-36.0397189421617,60.4806895737643,0.));
#95169=CARTESIAN_POINT('Ctrl Pts',(-36.0547232187681,60.4947416988396,0.));
#95170=CARTESIAN_POINT('Ctrl Pts',(-36.0697797118377,60.5088129911357,0.));
#95171=CARTESIAN_POINT('Ctrl Pts',(-36.0848883531968,60.5229032759001,0.));
#95172=CARTESIAN_POINT('Ctrl Pts',(-36.1000490738532,60.5370123768841,0.));
#95173=CARTESIAN_POINT('Ctrl Pts',(-36.1152618043756,60.5511401172014,0.));
#95174=CARTESIAN_POINT('Ctrl Pts',(-36.1305264752195,60.5652863200732,0.));
#95175=CARTESIAN_POINT('Ctrl Pts',(-36.1458430170425,60.5794508095555,0.));
#95176=CARTESIAN_POINT('Ctrl Pts',(-36.1612113610758,60.5936334114083,0.));
#95177=CARTESIAN_POINT('Ctrl Pts',(-36.1766314392624,60.6078339534151,0.));
#95178=CARTESIAN_POINT('Ctrl Pts',(-36.1921031840617,60.6220522649129,0.));
#95179=CARTESIAN_POINT('Ctrl Pts',(-36.2076265283261,60.6362881765014,0.));
#95180=CARTESIAN_POINT('Ctrl Pts',(-36.2232014051549,60.6505415197055,0.));
#95181=CARTESIAN_POINT('Ctrl Pts',(-36.2388277477225,60.6648121265908,0.));
#95182=CARTESIAN_POINT('Ctrl Pts',(-36.2545054892911,60.6790998297823,0.));
#95183=CARTESIAN_POINT('Ctrl Pts',(-36.2702345632882,60.6934044626304,0.));
#95184=CARTESIAN_POINT('Ctrl Pts',(-36.2860149033586,60.7077258593268,0.));
#95185=CARTESIAN_POINT('Ctrl Pts',(-36.3018464434204,60.7220638550396,0.));
#95186=CARTESIAN_POINT('Ctrl Pts',(-36.3177291177148,60.7364182860388,0.));
#95187=CARTESIAN_POINT('Ctrl Pts',(-36.3336628607844,60.7507889896283,0.));
#95188=CARTESIAN_POINT('Ctrl Pts',(-36.349647607448,60.7651758040791,0.));
#95189=CARTESIAN_POINT('Ctrl Pts',(-36.3656832927733,60.7795785685631,0.));
#95190=CARTESIAN_POINT('Ctrl Pts',(-36.38176985204,60.7939971230781,0.));
#95191=CARTESIAN_POINT('Ctrl Pts',(-36.3979072207174,60.8084313084009,0.));
#95192=CARTESIAN_POINT('Ctrl Pts',(-36.4140953344869,60.8228809661179,0.));
#95193=CARTESIAN_POINT('Ctrl Pts',(-36.4303341292497,60.8373459386397,0.));
#95194=CARTESIAN_POINT('Ctrl Pts',(-36.4466235411353,60.851826069218,0.));
#95195=CARTESIAN_POINT('Ctrl Pts',(-36.4629635065037,60.8663212019646,0.));
#95196=CARTESIAN_POINT('Ctrl Pts',(-36.4793539619459,60.8808311818489,0.));
#95197=CARTESIAN_POINT('Ctrl Pts',(-36.4957948442832,60.8953558546791,0.));
#95198=CARTESIAN_POINT('Ctrl Pts',(-36.5122860905611,60.9098950670847,0.));
#95199=CARTESIAN_POINT('Ctrl Pts',(-36.5288276380417,60.924448666499,0.));
#95200=CARTESIAN_POINT('Ctrl Pts',(-36.5454194241866,60.9390165011357,0.));
#95201=CARTESIAN_POINT('Ctrl Pts',(-36.5620613866615,60.9535984199874,0.));
#95202=CARTESIAN_POINT('Ctrl Pts',(-36.5787534633416,60.9681942728237,0.));
#95203=CARTESIAN_POINT('Ctrl Pts',(-36.5954955923109,60.9828039101887,0.));
#95204=CARTESIAN_POINT('Ctrl Pts',(-36.6122877118599,60.9974271833982,0.));
#95205=CARTESIAN_POINT('Ctrl Pts',(-36.6291297604775,61.012063944535,0.));
#95206=CARTESIAN_POINT('Ctrl Pts',(-36.6460216768553,61.0267140464434,0.));
#95207=CARTESIAN_POINT('Ctrl Pts',(-36.6629633998885,61.0413773427204,0.));
#95208=CARTESIAN_POINT('Ctrl Pts',(-36.6799548686741,61.0560536877084,0.));
#95209=CARTESIAN_POINT('Ctrl Pts',(-36.6969960225019,61.0707429364841,0.));
#95210=CARTESIAN_POINT('Ctrl Pts',(-36.7140868008479,61.085444944851,0.));
#95211=CARTESIAN_POINT('Ctrl Pts',(-36.7312271433799,61.1001595693357,0.));
#95212=CARTESIAN_POINT('Ctrl Pts',(-36.7484169899591,61.1148866671821,0.));
#95213=CARTESIAN_POINT('Ctrl Pts',(-36.7656562806381,61.1296260963468,0.));
#95214=CARTESIAN_POINT('Ctrl Pts',(-36.782944955654,61.1443777154926,0.));
#95215=CARTESIAN_POINT('Ctrl Pts',(-36.8002829554221,61.1591413839809,0.));
#95216=CARTESIAN_POINT('Ctrl Pts',(-36.8176702205436,61.1739169618688,0.));
#95217=CARTESIAN_POINT('Ctrl Pts',(-36.8351066918043,61.1887043099026,0.));
#95218=CARTESIAN_POINT('Ctrl Pts',(-36.8525923101736,61.2035032895121,0.));
#95219=CARTESIAN_POINT('Ctrl Pts',(-36.8701270167954,61.2183137628031,0.));
#95220=CARTESIAN_POINT('Ctrl Pts',(-36.8877107529844,61.2331355925513,0.));
#95221=CARTESIAN_POINT('Ctrl Pts',(-36.9053434602324,61.2479686421979,0.));
#95222=CARTESIAN_POINT('Ctrl Pts',(-36.9230250802078,61.2628127758443,0.));
#95223=CARTESIAN_POINT('Ctrl Pts',(-36.9407555547542,61.2776678582474,0.));
#95224=CARTESIAN_POINT('Ctrl Pts',(-36.9585348258798,61.2925337548113,0.));
#95225=CARTESIAN_POINT('Ctrl Pts',(-36.976362835757,61.3074103315834,0.));
#95226=CARTESIAN_POINT('Ctrl Pts',(-36.994239526729,61.3222974552519,0.));
#95227=CARTESIAN_POINT('Ctrl Pts',(-37.0121648413088,61.3371949931396,0.));
#95228=CARTESIAN_POINT('Ctrl Pts',(-37.0301387221766,61.352102813199,0.));
#95229=CARTESIAN_POINT('Ctrl Pts',(-37.0481611121698,61.3670207840041,0.));
#95230=CARTESIAN_POINT('Ctrl Pts',(-37.0662319542827,61.3819487747458,0.));
#95231=CARTESIAN_POINT('Ctrl Pts',(-37.0843511916728,61.3968866552294,0.));
#95232=CARTESIAN_POINT('Ctrl Pts',(-37.1025187676597,61.411834295869,0.));
#95233=CARTESIAN_POINT('Ctrl Pts',(-37.1207346257228,61.4267915676834,0.));
#95234=CARTESIAN_POINT('Ctrl Pts',(-37.138998709492,61.4417583422888,0.));
#95235=CARTESIAN_POINT('Ctrl Pts',(-37.157310962747,61.4567344918946,0.));
#95236=CARTESIAN_POINT('Ctrl Pts',(-37.1756713294249,61.471719889301,0.));
#95237=CARTESIAN_POINT('Ctrl Pts',(-37.1940797536182,61.4867144078939,0.));
#95238=CARTESIAN_POINT('Ctrl Pts',(-37.2125361795727,61.5017179216404,0.));
#95239=CARTESIAN_POINT('Ctrl Pts',(-37.2310405516775,61.5167303050823,0.));
#95240=CARTESIAN_POINT('Ctrl Pts',(-37.2495928144661,61.5317514333319,0.));
#95241=CARTESIAN_POINT('Ctrl Pts',(-37.2681929126218,61.5467811820686,0.));
#95242=CARTESIAN_POINT('Ctrl Pts',(-37.286840790977,61.5618194275349,0.));
#95243=CARTESIAN_POINT('Ctrl Pts',(-37.3055363945108,61.5768660465313,0.));
#95244=CARTESIAN_POINT('Ctrl Pts',(-37.3242796683395,61.591920916412,0.));
#95245=CARTESIAN_POINT('Ctrl Pts',(-37.3430705577178,61.6069839150804,0.));
#95246=CARTESIAN_POINT('Ctrl Pts',(-37.3619090080447,61.6220549209862,0.));
#95247=CARTESIAN_POINT('Ctrl Pts',(-37.3807949648622,61.6371338131208,0.));
#95248=CARTESIAN_POINT('Ctrl Pts',(-37.3997283738534,61.6522204710133,0.));
#95249=CARTESIAN_POINT('Ctrl Pts',(-37.4187091808324,61.667314774725,0.));
#95250=CARTESIAN_POINT('Ctrl Pts',(-37.4377373317456,61.6824166048453,0.));
#95251=CARTESIAN_POINT('Ctrl Pts',(-37.4568127726776,61.69752584249,0.));
#95252=CARTESIAN_POINT('Ctrl Pts',(-37.4759354498509,61.7126423692965,0.));
#95253=CARTESIAN_POINT('Ctrl Pts',(-37.4951053096235,61.7277660674203,0.));
#95254=CARTESIAN_POINT('Ctrl Pts',(-37.5143222984794,61.7428968195296,0.));
#95255=CARTESIAN_POINT('Ctrl Pts',(-37.5335863630286,61.7580345088014,0.));
#95256=CARTESIAN_POINT('Ctrl Pts',(-37.5528974500142,61.7731790189191,0.));
#95257=CARTESIAN_POINT('Ctrl Pts',(-37.5722555063112,61.7883302340689,0.));
#95258=CARTESIAN_POINT('Ctrl Pts',(-37.5916604789252,61.8034880389362,0.));
#95259=CARTESIAN_POINT('Ctrl Pts',(-37.6111123149836,61.8186523187011,0.));
#95260=CARTESIAN_POINT('Ctrl Pts',(-37.6306109617341,61.8338229590345,0.));
#95261=CARTESIAN_POINT('Ctrl Pts',(-37.6501563665518,61.848999846095,0.));
#95262=CARTESIAN_POINT('Ctrl Pts',(-37.6697484769389,61.8641828665257,0.));
#95263=CARTESIAN_POINT('Ctrl Pts',(-37.6893872405229,61.879371907451,0.));
#95264=CARTESIAN_POINT('Ctrl Pts',(-37.7090726050488,61.8945668564714,0.));
#95265=CARTESIAN_POINT('Ctrl Pts',(-37.7288045183765,61.9097676016616,0.));
#95266=CARTESIAN_POINT('Ctrl Pts',(-37.748582928488,61.9249740315664,0.));
#95267=CARTESIAN_POINT('Ctrl Pts',(-37.7684077834877,61.940186035198,0.));
#95268=CARTESIAN_POINT('Ctrl Pts',(-37.7882790316012,61.9554035020335,0.));
#95269=CARTESIAN_POINT('Ctrl Pts',(-37.808196621168,61.9706263220101,0.));
#95270=CARTESIAN_POINT('Ctrl Pts',(-37.8281605006371,61.9858543855221,0.));
#95271=CARTESIAN_POINT('Ctrl Pts',(-37.8481706185742,62.0010875834176,0.));
#95272=CARTESIAN_POINT('Ctrl Pts',(-37.8682269236628,62.0163258069954,0.));
#95273=CARTESIAN_POINT('Ctrl Pts',(-37.888329364703,62.0315689480022,0.));
#95274=CARTESIAN_POINT('Ctrl Pts',(-37.9084778906053,62.0468168986289,0.));
#95275=CARTESIAN_POINT('Ctrl Pts',(-37.9286724503849,62.0620695515072,0.));
#95276=CARTESIAN_POINT('Ctrl Pts',(-37.9489129931685,62.0773267997072,0.));
#95277=CARTESIAN_POINT('Ctrl Pts',(-37.9691994681962,62.0925885367346,0.));
#95278=CARTESIAN_POINT('Ctrl Pts',(-37.9895318248212,62.107854656528,0.));
#95279=CARTESIAN_POINT('Ctrl Pts',(-38.0099100125041,62.1231250534558,0.));
#95280=CARTESIAN_POINT('Ctrl Pts',(-38.0303339808059,62.1383996223136,0.));
#95281=CARTESIAN_POINT('Ctrl Pts',(-38.0508036793944,62.153678258321,0.));
#95282=CARTESIAN_POINT('Ctrl Pts',(-38.0713190580466,62.1689608571182,0.));
#95283=CARTESIAN_POINT('Ctrl Pts',(-38.0918800666479,62.1842473147627,0.));
#95284=CARTESIAN_POINT('Ctrl Pts',(-38.1124866551883,62.1995375277253,0.));
#95285=CARTESIAN_POINT('Ctrl Pts',(-38.1331387737528,62.2148313928859,0.));
#95286=CARTESIAN_POINT('Ctrl Pts',(-38.1538363725263,62.2301288075319,0.));
#95287=CARTESIAN_POINT('Ctrl Pts',(-38.1745794017997,62.2454296693581,0.));
#95288=CARTESIAN_POINT('Ctrl Pts',(-38.1953678119692,62.2607338764655,0.));
#95289=CARTESIAN_POINT('Ctrl Pts',(-38.2162015535351,62.2760413273601,0.));
#95290=CARTESIAN_POINT('Ctrl Pts',(-38.2370805770931,62.2913519209517,0.));
#95291=CARTESIAN_POINT('Ctrl Pts',(-38.2580048333356,62.3066655565497,0.));
#95292=CARTESIAN_POINT('Ctrl Pts',(-38.2789742730559,62.3219821338564,0.));
#95293=CARTESIAN_POINT('Ctrl Pts',(-38.2999888471474,62.337301552961,0.));
#95294=CARTESIAN_POINT('Ctrl Pts',(-38.3210485066003,62.3526237143338,0.));
#95295=CARTESIAN_POINT('Ctrl Pts',(-38.3421532024915,62.3679485188178,0.));
#95296=CARTESIAN_POINT('Ctrl Pts',(-38.3633028859835,62.3832758676281,0.));
#95297=CARTESIAN_POINT('Ctrl Pts',(-38.384497508335,62.3986056623587,0.));
#95298=CARTESIAN_POINT('Ctrl Pts',(-38.4057370209054,62.4139378049891,0.));
#95299=CARTESIAN_POINT('Ctrl Pts',(-38.4270213751567,62.42927219789,0.));
#95300=CARTESIAN_POINT('Ctrl Pts',(-38.4483505226511,62.4446087438304,0.));
#95301=CARTESIAN_POINT('Ctrl Pts',(-38.4697244150473,62.4599473459799,0.));
#95302=CARTESIAN_POINT('Ctrl Pts',(-38.4911430040988,62.4752879078842,0.));
#95303=CARTESIAN_POINT('Ctrl Pts',(-38.5126062416496,62.4906303334435,0.));
#95304=CARTESIAN_POINT('Ctrl Pts',(-38.5341140796247,62.50597452689,0.));
#95305=CARTESIAN_POINT('Ctrl Pts',(-38.5556664700201,62.5213203927672,0.));
#95306=CARTESIAN_POINT('Ctrl Pts',(-38.5772633648841,62.5366678359036,0.));
#95307=CARTESIAN_POINT('Ctrl Pts',(-38.5989047163401,62.5520167614529,0.));
#95308=CARTESIAN_POINT('Ctrl Pts',(-38.6205904766078,62.567367074937,0.));
#95309=CARTESIAN_POINT('Ctrl Pts',(-38.6423205980214,62.5827186822923,0.));
#95310=CARTESIAN_POINT('Ctrl Pts',(-38.6640950330418,62.5980714899048,0.));
#95311=CARTESIAN_POINT('Ctrl Pts',(-38.6859137342726,62.6134254046732,0.));
#95312=CARTESIAN_POINT('Ctrl Pts',(-38.7077766544411,62.6287803339534,0.));
#95313=CARTESIAN_POINT('Ctrl Pts',(-38.7296837463605,62.6441361854406,0.));
#95314=CARTESIAN_POINT('Ctrl Pts',(-38.7516349628902,62.6594928670626,0.));
#95315=CARTESIAN_POINT('Ctrl Pts',(-38.7736302568982,62.6748502868836,0.));
#95316=CARTESIAN_POINT('Ctrl Pts',(-38.7956695812032,62.6902083529698,0.));
#95317=CARTESIAN_POINT('Ctrl Pts',(-38.8177528885686,62.7055669733811,0.));
#95318=CARTESIAN_POINT('Ctrl Pts',(-38.8398801318184,62.7209260564506,0.));
#95319=CARTESIAN_POINT('Ctrl Pts',(-38.8620512639239,62.7362855110052,0.));
#95320=CARTESIAN_POINT('Ctrl Pts',(-38.8842662380984,62.7516452466129,0.));
#95321=CARTESIAN_POINT('Ctrl Pts',(-38.9065250078824,62.7670051738132,0.));
#95322=CARTESIAN_POINT('Ctrl Pts',(-38.928827527232,62.7823652043677,0.));
#95323=CARTESIAN_POINT('Ctrl Pts',(-38.9511737503146,62.797725250709,0.));
#95324=CARTESIAN_POINT('Ctrl Pts',(-38.9735636313073,62.8130852254004,0.));
#95325=CARTESIAN_POINT('Ctrl Pts',(-38.9959971241695,62.8284450405451,0.));
#95326=CARTESIAN_POINT('Ctrl Pts',(-39.0184741824649,62.8438046073237,0.));
#95327=CARTESIAN_POINT('Ctrl Pts',(-39.0409947590519,62.859163835209,0.));
#95328=CARTESIAN_POINT('Ctrl Pts',(-39.0635588063308,62.8745226326046,0.));
#95329=CARTESIAN_POINT('Ctrl Pts',(-39.0861662767964,62.8898809082659,0.));
#95330=CARTESIAN_POINT('Ctrl Pts',(-39.1088171235144,62.9052385725416,0.));
#95331=CARTESIAN_POINT('Ctrl Pts',(-39.1315113005745,62.9205955385551,0.));
#95332=CARTESIAN_POINT('Ctrl Pts',(-39.1542487636708,62.9359517237352,0.));
#95333=CARTESIAN_POINT('Ctrl Pts',(-39.1770294702367,62.9513070501777,0.));
#95334=CARTESIAN_POINT('Ctrl Pts',(-39.1965939820804,62.9644687386694,0.));
#95335=CARTESIAN_POINT('Ctrl Pts',(-39.2116170128278,62.9745590018501,0.));
#95336=CARTESIAN_POINT('Ctrl Pts',(-39.2220794388575,62.9815782721131,0.));
#95337=CARTESIAN_POINT('Ctrl Pts',(-39.2279686274723,62.9855268615905,0.));
#95338=CARTESIAN_POINT('Ctrl Pts',(-39.2292784191471,62.9864049293634,0.));
#95339=CARTESIAN_POINT('',(-35.7368311217509,60.1903555511633,12.));
#95340=CARTESIAN_POINT('',(-35.7368311217509,60.1903555511633,0.));
#95341=CARTESIAN_POINT('Ctrl Pts',(-39.229278419147,62.9864049293633,12.));
#95342=CARTESIAN_POINT('Ctrl Pts',(-39.2279686274723,62.9855268615905,12.));
#95343=CARTESIAN_POINT('Ctrl Pts',(-39.2220794388575,62.9815782721131,12.));
#95344=CARTESIAN_POINT('Ctrl Pts',(-39.2116170128278,62.9745590018501,12.));
#95345=CARTESIAN_POINT('Ctrl Pts',(-39.1965939820804,62.9644687386693,12.));
#95346=CARTESIAN_POINT('Ctrl Pts',(-39.1770294702367,62.9513070501777,12.));
#95347=CARTESIAN_POINT('Ctrl Pts',(-39.1542487636708,62.9359517237352,12.));
#95348=CARTESIAN_POINT('Ctrl Pts',(-39.1315113005745,62.9205955385551,12.));
#95349=CARTESIAN_POINT('Ctrl Pts',(-39.1088171235144,62.9052385725416,12.));
#95350=CARTESIAN_POINT('Ctrl Pts',(-39.0861662767964,62.8898809082659,12.));
#95351=CARTESIAN_POINT('Ctrl Pts',(-39.0635588063308,62.8745226326046,12.));
#95352=CARTESIAN_POINT('Ctrl Pts',(-39.0409947590519,62.859163835209,12.));
#95353=CARTESIAN_POINT('Ctrl Pts',(-39.0184741824649,62.8438046073237,12.));
#95354=CARTESIAN_POINT('Ctrl Pts',(-38.9959971241695,62.8284450405451,12.));
#95355=CARTESIAN_POINT('Ctrl Pts',(-38.9735636313073,62.8130852254004,12.));
#95356=CARTESIAN_POINT('Ctrl Pts',(-38.9511737503146,62.797725250709,12.));
#95357=CARTESIAN_POINT('Ctrl Pts',(-38.928827527232,62.7823652043677,12.));
#95358=CARTESIAN_POINT('Ctrl Pts',(-38.9065250078824,62.7670051738132,12.));
#95359=CARTESIAN_POINT('Ctrl Pts',(-38.8842662380984,62.7516452466129,12.));
#95360=CARTESIAN_POINT('Ctrl Pts',(-38.8620512639239,62.7362855110052,12.));
#95361=CARTESIAN_POINT('Ctrl Pts',(-38.8398801318184,62.7209260564506,12.));
#95362=CARTESIAN_POINT('Ctrl Pts',(-38.8177528885686,62.7055669733811,12.));
#95363=CARTESIAN_POINT('Ctrl Pts',(-38.7956695812032,62.6902083529698,12.));
#95364=CARTESIAN_POINT('Ctrl Pts',(-38.7736302568982,62.6748502868836,12.));
#95365=CARTESIAN_POINT('Ctrl Pts',(-38.7516349628902,62.6594928670626,12.));
#95366=CARTESIAN_POINT('Ctrl Pts',(-38.7296837463605,62.6441361854406,12.));
#95367=CARTESIAN_POINT('Ctrl Pts',(-38.7077766544411,62.6287803339534,12.));
#95368=CARTESIAN_POINT('Ctrl Pts',(-38.6859137342726,62.6134254046732,12.));
#95369=CARTESIAN_POINT('Ctrl Pts',(-38.6640950330418,62.5980714899048,12.));
#95370=CARTESIAN_POINT('Ctrl Pts',(-38.6423205980214,62.5827186822923,12.));
#95371=CARTESIAN_POINT('Ctrl Pts',(-38.6205904766078,62.567367074937,12.));
#95372=CARTESIAN_POINT('Ctrl Pts',(-38.5989047163401,62.5520167614529,12.));
#95373=CARTESIAN_POINT('Ctrl Pts',(-38.5772633648841,62.5366678359036,12.));
#95374=CARTESIAN_POINT('Ctrl Pts',(-38.5556664700201,62.5213203927672,12.));
#95375=CARTESIAN_POINT('Ctrl Pts',(-38.5341140796247,62.50597452689,12.));
#95376=CARTESIAN_POINT('Ctrl Pts',(-38.5126062416496,62.4906303334435,12.));
#95377=CARTESIAN_POINT('Ctrl Pts',(-38.4911430040988,62.4752879078842,12.));
#95378=CARTESIAN_POINT('Ctrl Pts',(-38.4697244150473,62.4599473459799,12.));
#95379=CARTESIAN_POINT('Ctrl Pts',(-38.4483505226511,62.4446087438304,12.));
#95380=CARTESIAN_POINT('Ctrl Pts',(-38.4270213751567,62.42927219789,12.));
#95381=CARTESIAN_POINT('Ctrl Pts',(-38.4057370209054,62.4139378049891,12.));
#95382=CARTESIAN_POINT('Ctrl Pts',(-38.384497508335,62.3986056623587,12.));
#95383=CARTESIAN_POINT('Ctrl Pts',(-38.3633028859835,62.3832758676281,12.));
#95384=CARTESIAN_POINT('Ctrl Pts',(-38.3421532024915,62.3679485188178,12.));
#95385=CARTESIAN_POINT('Ctrl Pts',(-38.3210485066003,62.3526237143338,12.));
#95386=CARTESIAN_POINT('Ctrl Pts',(-38.2999888471474,62.337301552961,12.));
#95387=CARTESIAN_POINT('Ctrl Pts',(-38.2789742730559,62.3219821338564,12.));
#95388=CARTESIAN_POINT('Ctrl Pts',(-38.2580048333356,62.3066655565497,12.));
#95389=CARTESIAN_POINT('Ctrl Pts',(-38.2370805770931,62.2913519209517,12.));
#95390=CARTESIAN_POINT('Ctrl Pts',(-38.2162015535351,62.2760413273601,12.));
#95391=CARTESIAN_POINT('Ctrl Pts',(-38.1953678119692,62.2607338764655,12.));
#95392=CARTESIAN_POINT('Ctrl Pts',(-38.1745794017997,62.2454296693581,12.));
#95393=CARTESIAN_POINT('Ctrl Pts',(-38.1538363725263,62.2301288075319,12.));
#95394=CARTESIAN_POINT('Ctrl Pts',(-38.1331387737528,62.2148313928859,12.));
#95395=CARTESIAN_POINT('Ctrl Pts',(-38.1124866551883,62.1995375277253,12.));
#95396=CARTESIAN_POINT('Ctrl Pts',(-38.0918800666479,62.1842473147627,12.));
#95397=CARTESIAN_POINT('Ctrl Pts',(-38.0713190580466,62.1689608571182,12.));
#95398=CARTESIAN_POINT('Ctrl Pts',(-38.0508036793944,62.153678258321,12.));
#95399=CARTESIAN_POINT('Ctrl Pts',(-38.0303339808059,62.1383996223136,12.));
#95400=CARTESIAN_POINT('Ctrl Pts',(-38.0099100125041,62.1231250534558,12.));
#95401=CARTESIAN_POINT('Ctrl Pts',(-37.9895318248212,62.107854656528,12.));
#95402=CARTESIAN_POINT('Ctrl Pts',(-37.9691994681962,62.0925885367346,12.));
#95403=CARTESIAN_POINT('Ctrl Pts',(-37.9489129931685,62.0773267997072,12.));
#95404=CARTESIAN_POINT('Ctrl Pts',(-37.9286724503849,62.0620695515072,12.));
#95405=CARTESIAN_POINT('Ctrl Pts',(-37.9084778906053,62.0468168986289,12.));
#95406=CARTESIAN_POINT('Ctrl Pts',(-37.888329364703,62.0315689480022,12.));
#95407=CARTESIAN_POINT('Ctrl Pts',(-37.8682269236628,62.0163258069954,12.));
#95408=CARTESIAN_POINT('Ctrl Pts',(-37.8481706185742,62.0010875834176,12.));
#95409=CARTESIAN_POINT('Ctrl Pts',(-37.8281605006371,61.9858543855221,12.));
#95410=CARTESIAN_POINT('Ctrl Pts',(-37.808196621168,61.9706263220101,12.));
#95411=CARTESIAN_POINT('Ctrl Pts',(-37.7882790316012,61.9554035020335,12.));
#95412=CARTESIAN_POINT('Ctrl Pts',(-37.7684077834877,61.940186035198,12.));
#95413=CARTESIAN_POINT('Ctrl Pts',(-37.748582928488,61.9249740315664,12.));
#95414=CARTESIAN_POINT('Ctrl Pts',(-37.7288045183765,61.9097676016616,12.));
#95415=CARTESIAN_POINT('Ctrl Pts',(-37.7090726050488,61.8945668564714,12.));
#95416=CARTESIAN_POINT('Ctrl Pts',(-37.6893872405229,61.879371907451,12.));
#95417=CARTESIAN_POINT('Ctrl Pts',(-37.6697484769389,61.8641828665257,12.));
#95418=CARTESIAN_POINT('Ctrl Pts',(-37.6501563665518,61.848999846095,12.));
#95419=CARTESIAN_POINT('Ctrl Pts',(-37.6306109617341,61.8338229590345,12.));
#95420=CARTESIAN_POINT('Ctrl Pts',(-37.6111123149836,61.8186523187011,12.));
#95421=CARTESIAN_POINT('Ctrl Pts',(-37.5916604789252,61.8034880389362,12.));
#95422=CARTESIAN_POINT('Ctrl Pts',(-37.5722555063112,61.7883302340689,12.));
#95423=CARTESIAN_POINT('Ctrl Pts',(-37.5528974500142,61.7731790189191,12.));
#95424=CARTESIAN_POINT('Ctrl Pts',(-37.5335863630286,61.7580345088014,12.));
#95425=CARTESIAN_POINT('Ctrl Pts',(-37.5143222984794,61.7428968195296,12.));
#95426=CARTESIAN_POINT('Ctrl Pts',(-37.4951053096235,61.7277660674203,12.));
#95427=CARTESIAN_POINT('Ctrl Pts',(-37.4759354498509,61.7126423692965,12.));
#95428=CARTESIAN_POINT('Ctrl Pts',(-37.4568127726776,61.69752584249,12.));
#95429=CARTESIAN_POINT('Ctrl Pts',(-37.4377373317456,61.6824166048453,12.));
#95430=CARTESIAN_POINT('Ctrl Pts',(-37.4187091808324,61.667314774725,12.));
#95431=CARTESIAN_POINT('Ctrl Pts',(-37.3997283738534,61.6522204710133,12.));
#95432=CARTESIAN_POINT('Ctrl Pts',(-37.3807949648622,61.6371338131208,12.));
#95433=CARTESIAN_POINT('Ctrl Pts',(-37.3619090080447,61.6220549209862,12.));
#95434=CARTESIAN_POINT('Ctrl Pts',(-37.3430705577178,61.6069839150804,12.));
#95435=CARTESIAN_POINT('Ctrl Pts',(-37.3242796683395,61.591920916412,12.));
#95436=CARTESIAN_POINT('Ctrl Pts',(-37.3055363945108,61.5768660465313,12.));
#95437=CARTESIAN_POINT('Ctrl Pts',(-37.286840790977,61.5618194275349,12.));
#95438=CARTESIAN_POINT('Ctrl Pts',(-37.2681929126218,61.5467811820686,12.));
#95439=CARTESIAN_POINT('Ctrl Pts',(-37.2495928144661,61.5317514333319,12.));
#95440=CARTESIAN_POINT('Ctrl Pts',(-37.2310405516775,61.5167303050823,12.));
#95441=CARTESIAN_POINT('Ctrl Pts',(-37.2125361795727,61.5017179216404,12.));
#95442=CARTESIAN_POINT('Ctrl Pts',(-37.1940797536182,61.4867144078939,12.));
#95443=CARTESIAN_POINT('Ctrl Pts',(-37.1756713294249,61.471719889301,12.));
#95444=CARTESIAN_POINT('Ctrl Pts',(-37.157310962747,61.4567344918946,12.));
#95445=CARTESIAN_POINT('Ctrl Pts',(-37.138998709492,61.4417583422888,12.));
#95446=CARTESIAN_POINT('Ctrl Pts',(-37.1207346257228,61.4267915676834,12.));
#95447=CARTESIAN_POINT('Ctrl Pts',(-37.1025187676597,61.411834295869,12.));
#95448=CARTESIAN_POINT('Ctrl Pts',(-37.0843511916728,61.3968866552294,12.));
#95449=CARTESIAN_POINT('Ctrl Pts',(-37.0662319542827,61.3819487747458,12.));
#95450=CARTESIAN_POINT('Ctrl Pts',(-37.0481611121698,61.3670207840041,12.));
#95451=CARTESIAN_POINT('Ctrl Pts',(-37.0301387221766,61.352102813199,12.));
#95452=CARTESIAN_POINT('Ctrl Pts',(-37.0121648413088,61.3371949931396,12.));
#95453=CARTESIAN_POINT('Ctrl Pts',(-36.994239526729,61.3222974552519,12.));
#95454=CARTESIAN_POINT('Ctrl Pts',(-36.976362835757,61.3074103315834,12.));
#95455=CARTESIAN_POINT('Ctrl Pts',(-36.9585348258798,61.2925337548113,12.));
#95456=CARTESIAN_POINT('Ctrl Pts',(-36.9407555547542,61.2776678582474,12.));
#95457=CARTESIAN_POINT('Ctrl Pts',(-36.9230250802078,61.2628127758443,12.));
#95458=CARTESIAN_POINT('Ctrl Pts',(-36.9053434602324,61.2479686421979,12.));
#95459=CARTESIAN_POINT('Ctrl Pts',(-36.8877107529844,61.2331355925513,12.));
#95460=CARTESIAN_POINT('Ctrl Pts',(-36.8701270167954,61.2183137628031,12.));
#95461=CARTESIAN_POINT('Ctrl Pts',(-36.8525923101736,61.2035032895121,12.));
#95462=CARTESIAN_POINT('Ctrl Pts',(-36.8351066918043,61.1887043099026,12.));
#95463=CARTESIAN_POINT('Ctrl Pts',(-36.8176702205436,61.1739169618688,12.));
#95464=CARTESIAN_POINT('Ctrl Pts',(-36.8002829554221,61.1591413839809,12.));
#95465=CARTESIAN_POINT('Ctrl Pts',(-36.782944955654,61.1443777154926,12.));
#95466=CARTESIAN_POINT('Ctrl Pts',(-36.7656562806381,61.1296260963468,12.));
#95467=CARTESIAN_POINT('Ctrl Pts',(-36.7484169899591,61.1148866671821,12.));
#95468=CARTESIAN_POINT('Ctrl Pts',(-36.7312271433799,61.1001595693357,12.));
#95469=CARTESIAN_POINT('Ctrl Pts',(-36.7140868008479,61.085444944851,12.));
#95470=CARTESIAN_POINT('Ctrl Pts',(-36.6969960225019,61.0707429364841,12.));
#95471=CARTESIAN_POINT('Ctrl Pts',(-36.6799548686741,61.0560536877084,12.));
#95472=CARTESIAN_POINT('Ctrl Pts',(-36.6629633998885,61.0413773427204,12.));
#95473=CARTESIAN_POINT('Ctrl Pts',(-36.6460216768553,61.0267140464434,12.));
#95474=CARTESIAN_POINT('Ctrl Pts',(-36.6291297604775,61.012063944535,12.));
#95475=CARTESIAN_POINT('Ctrl Pts',(-36.6122877118599,60.9974271833982,12.));
#95476=CARTESIAN_POINT('Ctrl Pts',(-36.5954955923109,60.9828039101887,12.));
#95477=CARTESIAN_POINT('Ctrl Pts',(-36.5787534633416,60.9681942728237,12.));
#95478=CARTESIAN_POINT('Ctrl Pts',(-36.5620613866615,60.9535984199874,12.));
#95479=CARTESIAN_POINT('Ctrl Pts',(-36.5454194241866,60.9390165011357,12.));
#95480=CARTESIAN_POINT('Ctrl Pts',(-36.5288276380417,60.924448666499,12.));
#95481=CARTESIAN_POINT('Ctrl Pts',(-36.5122860905611,60.9098950670847,12.));
#95482=CARTESIAN_POINT('Ctrl Pts',(-36.4957948442832,60.8953558546791,12.));
#95483=CARTESIAN_POINT('Ctrl Pts',(-36.4793539619459,60.8808311818489,12.));
#95484=CARTESIAN_POINT('Ctrl Pts',(-36.4629635065037,60.8663212019646,12.));
#95485=CARTESIAN_POINT('Ctrl Pts',(-36.4466235411353,60.851826069218,12.));
#95486=CARTESIAN_POINT('Ctrl Pts',(-36.4303341292497,60.8373459386397,12.));
#95487=CARTESIAN_POINT('Ctrl Pts',(-36.4140953344869,60.8228809661179,12.));
#95488=CARTESIAN_POINT('Ctrl Pts',(-36.3979072207174,60.8084313084009,12.));
#95489=CARTESIAN_POINT('Ctrl Pts',(-36.38176985204,60.7939971230781,12.));
#95490=CARTESIAN_POINT('Ctrl Pts',(-36.3656832927733,60.7795785685631,12.));
#95491=CARTESIAN_POINT('Ctrl Pts',(-36.349647607448,60.7651758040791,12.));
#95492=CARTESIAN_POINT('Ctrl Pts',(-36.3336628607844,60.7507889896283,12.));
#95493=CARTESIAN_POINT('Ctrl Pts',(-36.3177291177148,60.7364182860388,12.));
#95494=CARTESIAN_POINT('Ctrl Pts',(-36.3018464434204,60.7220638550396,12.));
#95495=CARTESIAN_POINT('Ctrl Pts',(-36.2860149033586,60.7077258593268,12.));
#95496=CARTESIAN_POINT('Ctrl Pts',(-36.2702345632882,60.6934044626304,12.));
#95497=CARTESIAN_POINT('Ctrl Pts',(-36.2545054892911,60.6790998297823,12.));
#95498=CARTESIAN_POINT('Ctrl Pts',(-36.2388277477225,60.6648121265908,12.));
#95499=CARTESIAN_POINT('Ctrl Pts',(-36.2232014051549,60.6505415197055,12.));
#95500=CARTESIAN_POINT('Ctrl Pts',(-36.2076265283261,60.6362881765014,12.));
#95501=CARTESIAN_POINT('Ctrl Pts',(-36.1921031840617,60.6220522649129,12.));
#95502=CARTESIAN_POINT('Ctrl Pts',(-36.1766314392624,60.6078339534151,12.));
#95503=CARTESIAN_POINT('Ctrl Pts',(-36.1612113610758,60.5936334114083,12.));
#95504=CARTESIAN_POINT('Ctrl Pts',(-36.1458430170425,60.5794508095555,12.));
#95505=CARTESIAN_POINT('Ctrl Pts',(-36.1305264752195,60.5652863200732,12.));
#95506=CARTESIAN_POINT('Ctrl Pts',(-36.1152618043756,60.5511401172014,12.));
#95507=CARTESIAN_POINT('Ctrl Pts',(-36.1000490738532,60.5370123768841,12.));
#95508=CARTESIAN_POINT('Ctrl Pts',(-36.0848883531968,60.5229032759001,12.));
#95509=CARTESIAN_POINT('Ctrl Pts',(-36.0697797118377,60.5088129911357,12.));
#95510=CARTESIAN_POINT('Ctrl Pts',(-36.0547232187681,60.4947416988396,12.));
#95511=CARTESIAN_POINT('Ctrl Pts',(-36.0397189421617,60.4806895737643,12.));
#95512=CARTESIAN_POINT('Ctrl Pts',(-36.0247669500867,60.4666567908053,12.));
#95513=CARTESIAN_POINT('Ctrl Pts',(-36.0098673113556,60.452643526964,12.));
#95514=CARTESIAN_POINT('Ctrl Pts',(-35.9950200962175,60.438649962949,12.));
#95515=CARTESIAN_POINT('Ctrl Pts',(-35.9802253773534,60.4246762854961,12.));
#95516=CARTESIAN_POINT('Ctrl Pts',(-35.9654832299627,60.4107226875759,12.));
#95517=CARTESIAN_POINT('Ctrl Pts',(-35.9507937296726,60.3967893635487,12.));
#95518=CARTESIAN_POINT('Ctrl Pts',(-35.9361569506955,60.3828765049031,12.));
#95519=CARTESIAN_POINT('Ctrl Pts',(-35.9215729642219,60.368984296546,12.));
#95520=CARTESIAN_POINT('Ctrl Pts',(-35.9070418358501,60.3551129108794,12.));
#95521=CARTESIAN_POINT('Ctrl Pts',(-35.8925636280632,60.3412625135223,12.));
#95522=CARTESIAN_POINT('Ctrl Pts',(-35.878138405151,60.3274332746782,12.));
#95523=CARTESIAN_POINT('Ctrl Pts',(-35.8637662371635,60.313625378281,12.));
#95524=CARTESIAN_POINT('Ctrl Pts',(-35.8494472046783,60.2998390330173,12.));
#95525=CARTESIAN_POINT('Ctrl Pts',(-35.8351814020424,60.2860744798563,12.));
#95526=CARTESIAN_POINT('Ctrl Pts',(-35.8209689272574,60.2723319687507,12.));
#95527=CARTESIAN_POINT('Ctrl Pts',(-35.8068098723386,60.2586117365278,12.));
#95528=CARTESIAN_POINT('Ctrl Pts',(-35.7927043145164,60.2449139865206,12.));
#95529=CARTESIAN_POINT('Ctrl Pts',(-35.7786523045782,60.2312388621286,12.));
#95530=CARTESIAN_POINT('Ctrl Pts',(-35.7646538667299,60.2175864449678,12.));
#95531=CARTESIAN_POINT('Ctrl Pts',(-35.7534979801871,60.2066827086579,12.));
#95532=CARTESIAN_POINT('Ctrl Pts',(-35.7451551752456,60.1985151474406,12.));
#95533=CARTESIAN_POINT('Ctrl Pts',(-35.7396040203973,60.1930746580239,12.));
#95534=CARTESIAN_POINT('Ctrl Pts',(-35.7368311217509,60.1903555511633,12.));
#95535=CARTESIAN_POINT('Ctrl Pts',(-40.5060598100929,62.1730054756869,-5.55111512312578E-16));
#95536=CARTESIAN_POINT('Ctrl Pts',(-40.5060598100929,62.1730054756869,4.));
#95537=CARTESIAN_POINT('Ctrl Pts',(-40.5060598100929,62.1730054756869,8.));
#95538=CARTESIAN_POINT('Ctrl Pts',(-40.5060598100929,62.1730054756869,12.));
#95539=CARTESIAN_POINT('Ctrl Pts',(-40.5229411493977,62.2815834512352,-5.55111512312578E-16));
#95540=CARTESIAN_POINT('Ctrl Pts',(-40.5229411493977,62.2815834512352,4.));
#95541=CARTESIAN_POINT('Ctrl Pts',(-40.5229411493977,62.2815834512352,8.));
#95542=CARTESIAN_POINT('Ctrl Pts',(-40.5229411493977,62.2815834512352,12.));
#95543=CARTESIAN_POINT('Ctrl Pts',(-40.4873422218648,62.4810961163743,-5.55111512312578E-16));
#95544=CARTESIAN_POINT('Ctrl Pts',(-40.4873422218648,62.4810961163743,4.));
#95545=CARTESIAN_POINT('Ctrl Pts',(-40.4873422218648,62.4810961163743,7.99999999999999));
#95546=CARTESIAN_POINT('Ctrl Pts',(-40.4873422218648,62.4810961163743,12.));
#95547=CARTESIAN_POINT('Ctrl Pts',(-40.3516729626244,62.6258675056113,-5.55111512312578E-16));
#95548=CARTESIAN_POINT('Ctrl Pts',(-40.3516729626244,62.6258675056113,4.));
#95549=CARTESIAN_POINT('Ctrl Pts',(-40.3516729626244,62.6258675056113,8.00000000000001));
#95550=CARTESIAN_POINT('Ctrl Pts',(-40.3516729626244,62.6258675056113,12.));
#95551=CARTESIAN_POINT('Ctrl Pts',(-40.2823469776989,62.6704278106371,-5.55111512312578E-16));
#95552=CARTESIAN_POINT('Ctrl Pts',(-40.2823469776989,62.6704278106371,4.));
#95553=CARTESIAN_POINT('Ctrl Pts',(-40.2823469776989,62.6704278106371,8.));
#95554=CARTESIAN_POINT('Ctrl Pts',(-40.2823469776989,62.6704278106371,12.));
#95555=CARTESIAN_POINT('',(-40.5060598100929,62.1730054756869,2.77555756156289E-16));
#95556=CARTESIAN_POINT('',(-40.2823469776989,62.6704278106371,0.));
#95557=CARTESIAN_POINT('Ctrl Pts',(-40.5060598100929,62.1730054756869,-1.38777878078145E-16));
#95558=CARTESIAN_POINT('Ctrl Pts',(-40.5229411493977,62.2815834512352,-1.38777878078145E-16));
#95559=CARTESIAN_POINT('Ctrl Pts',(-40.5025989050932,62.3955906884575,-1.38777878078144E-16));
#95560=CARTESIAN_POINT('Ctrl Pts',(-40.4495806341086,62.4917232233445,-1.38777878078145E-16));
#95561=CARTESIAN_POINT('Ctrl Pts',(-40.4098169308703,62.5638226245097,-1.38777878078145E-16));
#95562=CARTESIAN_POINT('Ctrl Pts',(-40.3516729626244,62.6258675056113,-1.38777878078145E-16));
#95563=CARTESIAN_POINT('Ctrl Pts',(-40.2823469776989,62.6704278106371,-1.38777878078145E-16));
#95564=CARTESIAN_POINT('',(-40.2823469776989,62.6704278106371,12.));
#95565=CARTESIAN_POINT('Ctrl Pts',(-40.2823469776989,62.6704278106371,-5.55111512312578E-16));
#95566=CARTESIAN_POINT('Ctrl Pts',(-40.2823469776989,62.6704278106371,4.));
#95567=CARTESIAN_POINT('Ctrl Pts',(-40.2823469776989,62.6704278106371,8.));
#95568=CARTESIAN_POINT('Ctrl Pts',(-40.2823469776989,62.6704278106371,12.));
#95569=CARTESIAN_POINT('',(-40.5060598100929,62.1730054756869,12.));
#95570=CARTESIAN_POINT('Ctrl Pts',(-40.2823469776989,62.6704278106371,12.));
#95571=CARTESIAN_POINT('Ctrl Pts',(-40.3516729626244,62.6258675056113,12.));
#95572=CARTESIAN_POINT('Ctrl Pts',(-40.4098169308703,62.5638226245097,12.));
#95573=CARTESIAN_POINT('Ctrl Pts',(-40.4495806341086,62.4917232233445,12.));
#95574=CARTESIAN_POINT('Ctrl Pts',(-40.5025989050932,62.3955906884575,12.));
#95575=CARTESIAN_POINT('Ctrl Pts',(-40.5229411493977,62.2815834512352,12.));
#95576=CARTESIAN_POINT('Ctrl Pts',(-40.5060598100929,62.1730054756869,12.));
#95577=CARTESIAN_POINT('Ctrl Pts',(-40.5060598100929,62.1730054756869,12.));
#95578=CARTESIAN_POINT('Ctrl Pts',(-40.5060598100929,62.1730054756869,8.));
#95579=CARTESIAN_POINT('Ctrl Pts',(-40.5060598100929,62.1730054756869,4.));
#95580=CARTESIAN_POINT('Ctrl Pts',(-40.5060598100929,62.1730054756869,-5.55111512312578E-16));
#95581=CARTESIAN_POINT('Origin',(-2.01487121870483E-10,3.16086693261782E-10,
0.));
#95582=CARTESIAN_POINT('Origin',(-2.01487121870483E-10,3.16086693261782E-10,
12.));
#95583=CARTESIAN_POINT('Origin',(-2.01487121870483E-10,3.16086693261782E-10,
0.));
#95584=CARTESIAN_POINT('Ctrl Pts',(-34.1330090612035,66.2207497120638,0.));
#95585=CARTESIAN_POINT('Ctrl Pts',(-34.1330090612035,66.2207497120638,4.));
#95586=CARTESIAN_POINT('Ctrl Pts',(-34.1330090612036,66.2207497120638,8.));
#95587=CARTESIAN_POINT('Ctrl Pts',(-34.1330090612036,66.2207497120638,12.));
#95588=CARTESIAN_POINT('Ctrl Pts',(-34.0353379297088,66.2710935941676,0.));
#95589=CARTESIAN_POINT('Ctrl Pts',(-34.0353379297088,66.2710935941676,3.99999999999999));
#95590=CARTESIAN_POINT('Ctrl Pts',(-34.0353379297089,66.2710935941675,8.));
#95591=CARTESIAN_POINT('Ctrl Pts',(-34.0353379297089,66.2710935941675,12.));
#95592=CARTESIAN_POINT('Ctrl Pts',(-33.8348041971634,66.3003999311009,0.));
#95593=CARTESIAN_POINT('Ctrl Pts',(-33.8348041971634,66.3003999311009,4.00000000000001));
#95594=CARTESIAN_POINT('Ctrl Pts',(-33.8348041971635,66.3003999311009,7.99999999999999));
#95595=CARTESIAN_POINT('Ctrl Pts',(-33.8348041971635,66.3003999311009,12.));
#95596=CARTESIAN_POINT('Ctrl Pts',(-33.6545652280941,66.2174610329232,0.));
#95597=CARTESIAN_POINT('Ctrl Pts',(-33.6545652280941,66.2174610329232,3.99999999999999));
#95598=CARTESIAN_POINT('Ctrl Pts',(-33.6545652280943,66.2174610329232,8.00000000000001));
#95599=CARTESIAN_POINT('Ctrl Pts',(-33.6545652280943,66.2174610329232,12.));
#95600=CARTESIAN_POINT('Ctrl Pts',(-33.5903722664958,66.1657795405671,0.));
#95601=CARTESIAN_POINT('Ctrl Pts',(-33.5903722664958,66.1657795405671,4.));
#95602=CARTESIAN_POINT('Ctrl Pts',(-33.590372266496,66.1657795405672,8.));
#95603=CARTESIAN_POINT('Ctrl Pts',(-33.590372266496,66.1657795405672,12.));
#95604=CARTESIAN_POINT('',(-34.1330090612035,66.2207497120638,0.));
#95605=CARTESIAN_POINT('',(-33.5903722664959,66.1657795405671,0.));
#95606=CARTESIAN_POINT('Ctrl Pts',(-34.1330090612035,66.2207497120638,1.38777878078144E-16));
#95607=CARTESIAN_POINT('Ctrl Pts',(-34.0353379297088,66.2710935941676,1.38777878078144E-16));
#95608=CARTESIAN_POINT('Ctrl Pts',(-33.9207472253972,66.2878400724152,1.38777878078145E-16));
#95609=CARTESIAN_POINT('Ctrl Pts',(-33.8127833826287,66.2679350453204,1.38777878078144E-16));
#95610=CARTESIAN_POINT('Ctrl Pts',(-33.7318105005524,66.2530062749994,1.38777878078144E-16));
#95611=CARTESIAN_POINT('Ctrl Pts',(-33.6545652280941,66.2174610329232,1.38777878078144E-16));
#95612=CARTESIAN_POINT('Ctrl Pts',(-33.5903722664958,66.1657795405671,1.38777878078144E-16));
#95613=CARTESIAN_POINT('',(-33.590372266496,66.1657795405671,12.));
#95614=CARTESIAN_POINT('Ctrl Pts',(-33.5903722664958,66.1657795405671,0.));
#95615=CARTESIAN_POINT('Ctrl Pts',(-33.5903722664958,66.1657795405671,4.));
#95616=CARTESIAN_POINT('Ctrl Pts',(-33.590372266496,66.1657795405672,8.));
#95617=CARTESIAN_POINT('Ctrl Pts',(-33.590372266496,66.1657795405672,12.));
#95618=CARTESIAN_POINT('',(-34.1330090612036,66.2207497120638,12.));
#95619=CARTESIAN_POINT('Ctrl Pts',(-33.590372266496,66.1657795405672,12.));
#95620=CARTESIAN_POINT('Ctrl Pts',(-33.6545652280943,66.2174610329232,12.));
#95621=CARTESIAN_POINT('Ctrl Pts',(-33.7318105005525,66.2530062749993,12.));
#95622=CARTESIAN_POINT('Ctrl Pts',(-33.8127833826288,66.2679350453204,12.));
#95623=CARTESIAN_POINT('Ctrl Pts',(-33.9207472253972,66.2878400724152,12.));
#95624=CARTESIAN_POINT('Ctrl Pts',(-34.0353379297089,66.2710935941675,12.));
#95625=CARTESIAN_POINT('Ctrl Pts',(-34.1330090612036,66.2207497120638,12.));
#95626=CARTESIAN_POINT('Ctrl Pts',(-34.1330090612036,66.2207497120638,12.));
#95627=CARTESIAN_POINT('Ctrl Pts',(-34.1330090612036,66.2207497120638,8.));
#95628=CARTESIAN_POINT('Ctrl Pts',(-34.1330090612035,66.2207497120638,4.));
#95629=CARTESIAN_POINT('Ctrl Pts',(-34.1330090612035,66.2207497120638,0.));
#95630=CARTESIAN_POINT('Ctrl Pts',(-30.3549065457811,63.0759831361898,0.));
#95631=CARTESIAN_POINT('Ctrl Pts',(-30.3549065457811,63.0759831361898,12.));
#95632=CARTESIAN_POINT('Ctrl Pts',(-30.357431906933,63.078933570069,0.));
#95633=CARTESIAN_POINT('Ctrl Pts',(-30.357431906933,63.078933570069,12.));
#95634=CARTESIAN_POINT('Ctrl Pts',(-30.3624877680651,63.0848371718048,0.));
#95635=CARTESIAN_POINT('Ctrl Pts',(-30.3624877680651,63.0848371718048,12.));
#95636=CARTESIAN_POINT('Ctrl Pts',(-30.3700869762507,63.0937007763471,0.));
#95637=CARTESIAN_POINT('Ctrl Pts',(-30.3700869762507,63.0937007763471,12.));
#95638=CARTESIAN_POINT('Ctrl Pts',(-30.3802500880403,63.105535320226,0.));
#95639=CARTESIAN_POINT('Ctrl Pts',(-30.3802500880403,63.105535320226,12.));
#95640=CARTESIAN_POINT('Ctrl Pts',(-30.3930053710484,63.1203558300657,0.));
#95641=CARTESIAN_POINT('Ctrl Pts',(-30.3930053710484,63.1203558300657,12.));
#95642=CARTESIAN_POINT('Ctrl Pts',(-30.4058120432228,63.135203629844,0.));
#95643=CARTESIAN_POINT('Ctrl Pts',(-30.4058120432228,63.135203629844,12.));
#95644=CARTESIAN_POINT('Ctrl Pts',(-30.418670087563,63.1500786361459,0.));
#95645=CARTESIAN_POINT('Ctrl Pts',(-30.418670087563,63.1500786361459,12.));
#95646=CARTESIAN_POINT('Ctrl Pts',(-30.4315794659731,63.164980701691,0.));
#95647=CARTESIAN_POINT('Ctrl Pts',(-30.4315794659731,63.164980701691,12.));
#95648=CARTESIAN_POINT('Ctrl Pts',(-30.4445401192381,63.179909617189,0.));
#95649=CARTESIAN_POINT('Ctrl Pts',(-30.4445401192381,63.179909617189,12.));
#95650=CARTESIAN_POINT('Ctrl Pts',(-30.4575519763337,63.1948651386942,0.));
#95651=CARTESIAN_POINT('Ctrl Pts',(-30.4575519763337,63.1948651386942,12.));
#95652=CARTESIAN_POINT('Ctrl Pts',(-30.470614961416,63.2098470086636,0.));
#95653=CARTESIAN_POINT('Ctrl Pts',(-30.470614961416,63.2098470086636,12.));
#95654=CARTESIAN_POINT('Ctrl Pts',(-30.4837290014989,63.2248549788221,0.));
#95655=CARTESIAN_POINT('Ctrl Pts',(-30.4837290014989,63.2248549788221,12.));
#95656=CARTESIAN_POINT('Ctrl Pts',(-30.4968940344998,63.2398888342545,0.));
#95657=CARTESIAN_POINT('Ctrl Pts',(-30.4968940344998,63.2398888342545,12.));
#95658=CARTESIAN_POINT('Ctrl Pts',(-30.5101100066659,63.2549483856215,0.));
#95659=CARTESIAN_POINT('Ctrl Pts',(-30.5101100066659,63.2549483856215,12.));
#95660=CARTESIAN_POINT('Ctrl Pts',(-30.5233768687865,63.2700334577639,0.));
#95661=CARTESIAN_POINT('Ctrl Pts',(-30.5233768687865,63.2700334577639,12.));
#95662=CARTESIAN_POINT('Ctrl Pts',(-30.5366945730508,63.2851438802473,0.));
#95663=CARTESIAN_POINT('Ctrl Pts',(-30.5366945730508,63.2851438802473,12.));
#95664=CARTESIAN_POINT('Ctrl Pts',(-30.5500630691359,63.3002794756086,0.));
#95665=CARTESIAN_POINT('Ctrl Pts',(-30.5500630691359,63.3002794756086,12.));
#95666=CARTESIAN_POINT('Ctrl Pts',(-30.563482302238,63.3154400534397,0.));
#95667=CARTESIAN_POINT('Ctrl Pts',(-30.563482302238,63.3154400534397,12.));
#95668=CARTESIAN_POINT('Ctrl Pts',(-30.5769522151164,63.3306254165126,0.));
#95669=CARTESIAN_POINT('Ctrl Pts',(-30.5769522151164,63.3306254165126,12.));
#95670=CARTESIAN_POINT('Ctrl Pts',(-30.5904727493712,63.3458353646154,0.));
#95671=CARTESIAN_POINT('Ctrl Pts',(-30.5904727493712,63.3458353646154,12.));
#95672=CARTESIAN_POINT('Ctrl Pts',(-30.6040438469078,63.3610696989577,0.));
#95673=CARTESIAN_POINT('Ctrl Pts',(-30.6040438469078,63.3610696989577,12.));
#95674=CARTESIAN_POINT('Ctrl Pts',(-30.6176654515967,63.3763282271796,0.));
#95675=CARTESIAN_POINT('Ctrl Pts',(-30.6176654515967,63.3763282271796,12.));
#95676=CARTESIAN_POINT('Ctrl Pts',(-30.6313375092062,63.3916107631376,0.));
#95677=CARTESIAN_POINT('Ctrl Pts',(-30.6313375092062,63.3916107631376,12.));
#95678=CARTESIAN_POINT('Ctrl Pts',(-30.6450599666121,63.4069171245066,0.));
#95679=CARTESIAN_POINT('Ctrl Pts',(-30.6450599666121,63.4069171245066,12.));
#95680=CARTESIAN_POINT('Ctrl Pts',(-30.6588327712484,63.4222471311239,0.));
#95681=CARTESIAN_POINT('Ctrl Pts',(-30.6588327712484,63.4222471311239,12.));
#95682=CARTESIAN_POINT('Ctrl Pts',(-30.6726558704315,63.4376006029604,0.));
#95683=CARTESIAN_POINT('Ctrl Pts',(-30.6726558704315,63.4376006029604,12.));
#95684=CARTESIAN_POINT('Ctrl Pts',(-30.6865292107929,63.4529773584249,0.));
#95685=CARTESIAN_POINT('Ctrl Pts',(-30.6865292107929,63.4529773584249,12.));
#95686=CARTESIAN_POINT('Ctrl Pts',(-30.7004527385821,63.4683772152529,0.));
#95687=CARTESIAN_POINT('Ctrl Pts',(-30.7004527385821,63.4683772152529,12.));
#95688=CARTESIAN_POINT('Ctrl Pts',(-30.7144263999265,63.4837999912771,0.));
#95689=CARTESIAN_POINT('Ctrl Pts',(-30.7144263999265,63.4837999912771,12.));
#95690=CARTESIAN_POINT('Ctrl Pts',(-30.7284501410822,63.4992455051795,0.));
#95691=CARTESIAN_POINT('Ctrl Pts',(-30.7284501410822,63.4992455051795,12.));
#95692=CARTESIAN_POINT('Ctrl Pts',(-30.7425239087281,63.5147135773894,0.));
#95693=CARTESIAN_POINT('Ctrl Pts',(-30.7425239087281,63.5147135773894,12.));
#95694=CARTESIAN_POINT('Ctrl Pts',(-30.7566476500757,63.5302040304142,0.));
#95695=CARTESIAN_POINT('Ctrl Pts',(-30.7566476500757,63.5302040304142,12.));
#95696=CARTESIAN_POINT('Ctrl Pts',(-30.7708213127159,63.5457166883537,0.));
#95697=CARTESIAN_POINT('Ctrl Pts',(-30.7708213127159,63.5457166883537,12.));
#95698=CARTESIAN_POINT('Ctrl Pts',(-30.7850448445205,63.5612513766,0.));
#95699=CARTESIAN_POINT('Ctrl Pts',(-30.7850448445205,63.5612513766,12.));
#95700=CARTESIAN_POINT('Ctrl Pts',(-30.7993181935271,63.5768079214881,0.));
#95701=CARTESIAN_POINT('Ctrl Pts',(-30.7993181935271,63.5768079214881,12.));
#95702=CARTESIAN_POINT('Ctrl Pts',(-30.813641307801,63.5923861498987,0.));
#95703=CARTESIAN_POINT('Ctrl Pts',(-30.813641307801,63.5923861498987,12.));
#95704=CARTESIAN_POINT('Ctrl Pts',(-30.8280141354459,63.6079858892771,0.));
#95705=CARTESIAN_POINT('Ctrl Pts',(-30.8280141354459,63.6079858892771,12.));
#95706=CARTESIAN_POINT('Ctrl Pts',(-30.8424366246671,63.6236069678055,0.));
#95707=CARTESIAN_POINT('Ctrl Pts',(-30.8424366246671,63.6236069678055,12.));
#95708=CARTESIAN_POINT('Ctrl Pts',(-30.8569087238131,63.6392492145233,0.));
#95709=CARTESIAN_POINT('Ctrl Pts',(-30.8569087238131,63.6392492145233,12.));
#95710=CARTESIAN_POINT('Ctrl Pts',(-30.8714303814194,63.6549124594666,0.));
#95711=CARTESIAN_POINT('Ctrl Pts',(-30.8714303814194,63.6549124594666,12.));
#95712=CARTESIAN_POINT('Ctrl Pts',(-30.8860015462475,63.6705965337971,0.));
#95713=CARTESIAN_POINT('Ctrl Pts',(-30.8860015462475,63.6705965337971,12.));
#95714=CARTESIAN_POINT('Ctrl Pts',(-30.900622167269,63.6863012697328,0.));
#95715=CARTESIAN_POINT('Ctrl Pts',(-30.900622167269,63.6863012697328,12.));
#95716=CARTESIAN_POINT('Ctrl Pts',(-30.9152921936465,63.7020265004792,0.));
#95717=CARTESIAN_POINT('Ctrl Pts',(-30.9152921936465,63.7020265004792,12.));
#95718=CARTESIAN_POINT('Ctrl Pts',(-30.9300115747115,63.7177720601609,0.));
#95719=CARTESIAN_POINT('Ctrl Pts',(-30.9300115747115,63.7177720601609,12.));
#95720=CARTESIAN_POINT('Ctrl Pts',(-30.9447802599355,63.7335377837441,0.));
#95721=CARTESIAN_POINT('Ctrl Pts',(-30.9447802599355,63.7335377837441,12.));
#95722=CARTESIAN_POINT('Ctrl Pts',(-30.9595981989104,63.749323506987,0.));
#95723=CARTESIAN_POINT('Ctrl Pts',(-30.9595981989104,63.749323506987,12.));
#95724=CARTESIAN_POINT('Ctrl Pts',(-30.9744653413689,63.7651290664733,0.));
#95725=CARTESIAN_POINT('Ctrl Pts',(-30.9744653413689,63.7651290664733,12.));
#95726=CARTESIAN_POINT('Ctrl Pts',(-30.989381637191,63.7809542996264,0.));
#95727=CARTESIAN_POINT('Ctrl Pts',(-30.989381637191,63.7809542996264,12.));
#95728=CARTESIAN_POINT('Ctrl Pts',(-31.0043470364108,63.796799044728,0.));
#95729=CARTESIAN_POINT('Ctrl Pts',(-31.0043470364108,63.796799044728,12.));
#95730=CARTESIAN_POINT('Ctrl Pts',(-31.0193614892171,63.8126631409364,0.));
#95731=CARTESIAN_POINT('Ctrl Pts',(-31.0193614892171,63.8126631409364,12.));
#95732=CARTESIAN_POINT('Ctrl Pts',(-31.0344249459538,63.8285464282846,0.));
#95733=CARTESIAN_POINT('Ctrl Pts',(-31.0344249459538,63.8285464282846,12.));
#95734=CARTESIAN_POINT('Ctrl Pts',(-31.0495373571215,63.8444487476611,0.));
#95735=CARTESIAN_POINT('Ctrl Pts',(-31.0495373571215,63.8444487476611,12.));
#95736=CARTESIAN_POINT('Ctrl Pts',(-31.0646986733723,63.8603699407922,0.));
#95737=CARTESIAN_POINT('Ctrl Pts',(-31.0646986733723,63.8603699407922,12.));
#95738=CARTESIAN_POINT('Ctrl Pts',(-31.0799088455041,63.8763098502237,0.));
#95739=CARTESIAN_POINT('Ctrl Pts',(-31.0799088455041,63.8763098502237,12.));
#95740=CARTESIAN_POINT('Ctrl Pts',(-31.0951678244455,63.8922683192964,0.));
#95741=CARTESIAN_POINT('Ctrl Pts',(-31.0951678244455,63.8922683192964,12.));
#95742=CARTESIAN_POINT('Ctrl Pts',(-31.1104755612607,63.9082451921448,0.));
#95743=CARTESIAN_POINT('Ctrl Pts',(-31.1104755612607,63.9082451921448,12.));
#95744=CARTESIAN_POINT('Ctrl Pts',(-31.1258320071545,63.9242403136955,0.));
#95745=CARTESIAN_POINT('Ctrl Pts',(-31.1258320071545,63.9242403136955,12.));
#95746=CARTESIAN_POINT('Ctrl Pts',(-31.1412371134727,63.940253529665,0.));
#95747=CARTESIAN_POINT('Ctrl Pts',(-31.1412371134727,63.940253529665,12.));
#95748=CARTESIAN_POINT('Ctrl Pts',(-31.1566908316992,63.9562846865567,0.));
#95749=CARTESIAN_POINT('Ctrl Pts',(-31.1566908316992,63.9562846865567,12.));
#95750=CARTESIAN_POINT('Ctrl Pts',(-31.1721931134487,63.9723336316551,0.));
#95751=CARTESIAN_POINT('Ctrl Pts',(-31.1721931134487,63.9723336316551,12.));
#95752=CARTESIAN_POINT('Ctrl Pts',(-31.1877439104717,63.9884002130211,0.));
#95753=CARTESIAN_POINT('Ctrl Pts',(-31.1877439104717,63.9884002130211,12.));
#95754=CARTESIAN_POINT('Ctrl Pts',(-31.2033431746558,64.0044842794831,0.));
#95755=CARTESIAN_POINT('Ctrl Pts',(-31.2033431746558,64.0044842794831,12.));
#95756=CARTESIAN_POINT('Ctrl Pts',(-31.2189908580245,64.02058568063,0.));
#95757=CARTESIAN_POINT('Ctrl Pts',(-31.2189908580245,64.02058568063,12.));
#95758=CARTESIAN_POINT('Ctrl Pts',(-31.2346869127297,64.0367042667984,0.));
#95759=CARTESIAN_POINT('Ctrl Pts',(-31.2346869127297,64.0367042667984,12.));
#95760=CARTESIAN_POINT('Ctrl Pts',(-31.2504312910451,64.0528398890657,0.));
#95761=CARTESIAN_POINT('Ctrl Pts',(-31.2504312910451,64.0528398890657,12.));
#95762=CARTESIAN_POINT('Ctrl Pts',(-31.2662239453728,64.0689923992461,0.));
#95763=CARTESIAN_POINT('Ctrl Pts',(-31.2662239453728,64.0689923992461,12.));
#95764=CARTESIAN_POINT('Ctrl Pts',(-31.2820648282447,64.0851616498852,0.));
#95765=CARTESIAN_POINT('Ctrl Pts',(-31.2820648282447,64.0851616498852,12.));
#95766=CARTESIAN_POINT('Ctrl Pts',(-31.2979538923214,64.1013474942556,0.));
#95767=CARTESIAN_POINT('Ctrl Pts',(-31.2979538923214,64.1013474942556,12.));
#95768=CARTESIAN_POINT('Ctrl Pts',(-31.3138910903859,64.117549786349,0.));
#95769=CARTESIAN_POINT('Ctrl Pts',(-31.3138910903859,64.117549786349,12.));
#95770=CARTESIAN_POINT('Ctrl Pts',(-31.3298763753377,64.133768380869,0.));
#95771=CARTESIAN_POINT('Ctrl Pts',(-31.3298763753377,64.133768380869,12.));
#95772=CARTESIAN_POINT('Ctrl Pts',(-31.3459097002006,64.1500031332282,0.));
#95773=CARTESIAN_POINT('Ctrl Pts',(-31.3459097002006,64.1500031332282,12.));
#95774=CARTESIAN_POINT('Ctrl Pts',(-31.3619910181228,64.166253899542,0.));
#95775=CARTESIAN_POINT('Ctrl Pts',(-31.3619910181228,64.166253899542,12.));
#95776=CARTESIAN_POINT('Ctrl Pts',(-31.3781202823754,64.1825205366224,0.));
#95777=CARTESIAN_POINT('Ctrl Pts',(-31.3781202823754,64.1825205366224,12.));
#95778=CARTESIAN_POINT('Ctrl Pts',(-31.3942974463445,64.1988029019707,0.));
#95779=CARTESIAN_POINT('Ctrl Pts',(-31.3942974463445,64.1988029019707,12.));
#95780=CARTESIAN_POINT('Ctrl Pts',(-31.410522463528,64.2151008537697,0.));
#95781=CARTESIAN_POINT('Ctrl Pts',(-31.410522463528,64.2151008537697,12.));
#95782=CARTESIAN_POINT('Ctrl Pts',(-31.4267952875423,64.231414250881,0.));
#95783=CARTESIAN_POINT('Ctrl Pts',(-31.4267952875423,64.231414250881,12.));
#95784=CARTESIAN_POINT('Ctrl Pts',(-31.4431158721222,64.2477429528393,0.));
#95785=CARTESIAN_POINT('Ctrl Pts',(-31.4431158721222,64.2477429528393,12.));
#95786=CARTESIAN_POINT('Ctrl Pts',(-31.4594841711195,64.2640868198473,0.));
#95787=CARTESIAN_POINT('Ctrl Pts',(-31.4594841711195,64.2640868198473,12.));
#95788=CARTESIAN_POINT('Ctrl Pts',(-31.4759001384941,64.2804457127671,0.));
#95789=CARTESIAN_POINT('Ctrl Pts',(-31.4759001384941,64.2804457127671,12.));
#95790=CARTESIAN_POINT('Ctrl Pts',(-31.4923637283132,64.2968194931158,0.));
#95791=CARTESIAN_POINT('Ctrl Pts',(-31.4923637283132,64.2968194931158,12.));
#95792=CARTESIAN_POINT('Ctrl Pts',(-31.5088748947582,64.3132080230637,0.));
#95793=CARTESIAN_POINT('Ctrl Pts',(-31.5088748947582,64.3132080230637,12.));
#95794=CARTESIAN_POINT('Ctrl Pts',(-31.5254335921245,64.3296111654283,0.));
#95795=CARTESIAN_POINT('Ctrl Pts',(-31.5254335921245,64.3296111654283,12.));
#95796=CARTESIAN_POINT('Ctrl Pts',(-31.5420397748191,64.3460287836687,0.));
#95797=CARTESIAN_POINT('Ctrl Pts',(-31.5420397748191,64.3460287836687,12.));
#95798=CARTESIAN_POINT('Ctrl Pts',(-31.5586933973515,64.3624607418768,0.));
#95799=CARTESIAN_POINT('Ctrl Pts',(-31.5586933973515,64.3624607418768,12.));
#95800=CARTESIAN_POINT('Ctrl Pts',(-31.5753944143336,64.3789069047733,0.));
#95801=CARTESIAN_POINT('Ctrl Pts',(-31.5753944143336,64.3789069047733,12.));
#95802=CARTESIAN_POINT('Ctrl Pts',(-31.5921427804865,64.3953671377046,0.));
#95803=CARTESIAN_POINT('Ctrl Pts',(-31.5921427804865,64.3953671377046,12.));
#95804=CARTESIAN_POINT('Ctrl Pts',(-31.6089384506395,64.4118413066378,0.));
#95805=CARTESIAN_POINT('Ctrl Pts',(-31.6089384506395,64.4118413066378,12.));
#95806=CARTESIAN_POINT('Ctrl Pts',(-31.6257813797287,64.4283292781565,0.));
#95807=CARTESIAN_POINT('Ctrl Pts',(-31.6257813797287,64.4283292781565,12.));
#95808=CARTESIAN_POINT('Ctrl Pts',(-31.6426715227878,64.4448309194525,0.));
#95809=CARTESIAN_POINT('Ctrl Pts',(-31.6426715227878,64.4448309194525,12.));
#95810=CARTESIAN_POINT('Ctrl Pts',(-31.6596088349482,64.4613460983214,0.));
#95811=CARTESIAN_POINT('Ctrl Pts',(-31.6596088349482,64.4613460983214,12.));
#95812=CARTESIAN_POINT('Ctrl Pts',(-31.6765932714464,64.4778746831614,0.));
#95813=CARTESIAN_POINT('Ctrl Pts',(-31.6765932714464,64.4778746831614,12.));
#95814=CARTESIAN_POINT('Ctrl Pts',(-31.6936247876229,64.4944165429675,0.));
#95815=CARTESIAN_POINT('Ctrl Pts',(-31.6936247876229,64.4944165429675,12.));
#95816=CARTESIAN_POINT('Ctrl Pts',(-31.7107033389201,64.510971547327,0.));
#95817=CARTESIAN_POINT('Ctrl Pts',(-31.7107033389201,64.510971547327,12.));
#95818=CARTESIAN_POINT('Ctrl Pts',(-31.7278288808731,64.5275395664124,0.));
#95819=CARTESIAN_POINT('Ctrl Pts',(-31.7278288808731,64.5275395664124,12.));
#95820=CARTESIAN_POINT('Ctrl Pts',(-31.7450013691112,64.544120470977,0.));
#95821=CARTESIAN_POINT('Ctrl Pts',(-31.7450013691112,64.544120470977,12.));
#95822=CARTESIAN_POINT('Ctrl Pts',(-31.7622207593634,64.5607141323521,0.));
#95823=CARTESIAN_POINT('Ctrl Pts',(-31.7622207593634,64.5607141323521,12.));
#95824=CARTESIAN_POINT('Ctrl Pts',(-31.7794870074583,64.5773204224429,0.));
#95825=CARTESIAN_POINT('Ctrl Pts',(-31.7794870074583,64.5773204224429,12.));
#95826=CARTESIAN_POINT('Ctrl Pts',(-31.7968000693218,64.5939392137235,0.));
#95827=CARTESIAN_POINT('Ctrl Pts',(-31.7968000693218,64.5939392137235,12.));
#95828=CARTESIAN_POINT('Ctrl Pts',(-31.8141599009684,64.6105703792312,0.));
#95829=CARTESIAN_POINT('Ctrl Pts',(-31.8141599009684,64.6105703792312,12.));
#95830=CARTESIAN_POINT('Ctrl Pts',(-31.8315664585026,64.6272137925627,0.));
#95831=CARTESIAN_POINT('Ctrl Pts',(-31.8315664585026,64.6272137925627,12.));
#95832=CARTESIAN_POINT('Ctrl Pts',(-31.8490196981248,64.6438693278714,0.));
#95833=CARTESIAN_POINT('Ctrl Pts',(-31.8490196981248,64.6438693278714,12.));
#95834=CARTESIAN_POINT('Ctrl Pts',(-31.866519576131,64.6605368598629,0.));
#95835=CARTESIAN_POINT('Ctrl Pts',(-31.866519576131,64.6605368598629,12.));
#95836=CARTESIAN_POINT('Ctrl Pts',(-31.8840660489107,64.6772162637907,0.));
#95837=CARTESIAN_POINT('Ctrl Pts',(-31.8840660489107,64.6772162637907,12.));
#95838=CARTESIAN_POINT('Ctrl Pts',(-31.9016590729374,64.6939074154498,0.));
#95839=CARTESIAN_POINT('Ctrl Pts',(-31.9016590729374,64.6939074154498,12.));
#95840=CARTESIAN_POINT('Ctrl Pts',(-31.9192986047706,64.7106101911732,0.));
#95841=CARTESIAN_POINT('Ctrl Pts',(-31.9192986047706,64.7106101911732,12.));
#95842=CARTESIAN_POINT('Ctrl Pts',(-31.9369846010615,64.7273244678297,0.));
#95843=CARTESIAN_POINT('Ctrl Pts',(-31.9369846010615,64.7273244678297,12.));
#95844=CARTESIAN_POINT('Ctrl Pts',(-31.9547170185534,64.7440501228202,0.));
#95845=CARTESIAN_POINT('Ctrl Pts',(-31.9547170185534,64.7440501228202,12.));
#95846=CARTESIAN_POINT('Ctrl Pts',(-31.9724958140789,64.7607870340735,0.));
#95847=CARTESIAN_POINT('Ctrl Pts',(-31.9724958140789,64.7607870340735,12.));
#95848=CARTESIAN_POINT('Ctrl Pts',(-31.990320944552,64.77753508004,0.));
#95849=CARTESIAN_POINT('Ctrl Pts',(-31.990320944552,64.77753508004,12.));
#95850=CARTESIAN_POINT('Ctrl Pts',(-32.0081923669677,64.7942941396881,0.));
#95851=CARTESIAN_POINT('Ctrl Pts',(-32.0081923669677,64.7942941396881,12.));
#95852=CARTESIAN_POINT('Ctrl Pts',(-32.0261100384092,64.8110640925021,0.));
#95853=CARTESIAN_POINT('Ctrl Pts',(-32.0261100384092,64.8110640925021,12.));
#95854=CARTESIAN_POINT('Ctrl Pts',(-32.0440739160477,64.8278448184786,0.));
#95855=CARTESIAN_POINT('Ctrl Pts',(-32.0440739160477,64.8278448184786,12.));
#95856=CARTESIAN_POINT('Ctrl Pts',(-32.0620839571408,64.8446361981234,0.));
#95857=CARTESIAN_POINT('Ctrl Pts',(-32.0620839571408,64.8446361981234,12.));
#95858=CARTESIAN_POINT('Ctrl Pts',(-32.0801401190241,64.861438112445,0.));
#95859=CARTESIAN_POINT('Ctrl Pts',(-32.0801401190241,64.861438112445,12.));
#95860=CARTESIAN_POINT('Ctrl Pts',(-32.0982423591108,64.878250442952,0.));
#95861=CARTESIAN_POINT('Ctrl Pts',(-32.0982423591108,64.878250442952,12.));
#95862=CARTESIAN_POINT('Ctrl Pts',(-32.1163906348979,64.8950730716493,0.));
#95863=CARTESIAN_POINT('Ctrl Pts',(-32.1163906348979,64.8950730716493,12.));
#95864=CARTESIAN_POINT('Ctrl Pts',(-32.1345849039671,64.9119058810362,0.));
#95865=CARTESIAN_POINT('Ctrl Pts',(-32.1345849039671,64.9119058810362,12.));
#95866=CARTESIAN_POINT('Ctrl Pts',(-32.1528251239832,64.9287487541018,0.));
#95867=CARTESIAN_POINT('Ctrl Pts',(-32.1528251239832,64.9287487541018,12.));
#95868=CARTESIAN_POINT('Ctrl Pts',(-32.171111252686,64.9456015743203,0.));
#95869=CARTESIAN_POINT('Ctrl Pts',(-32.171111252686,64.9456015743203,12.));
#95870=CARTESIAN_POINT('Ctrl Pts',(-32.1894432478889,64.9624642256477,0.));
#95871=CARTESIAN_POINT('Ctrl Pts',(-32.1894432478889,64.9624642256477,12.));
#95872=CARTESIAN_POINT('Ctrl Pts',(-32.2078210674857,64.9793365925194,0.));
#95873=CARTESIAN_POINT('Ctrl Pts',(-32.2078210674857,64.9793365925194,12.));
#95874=CARTESIAN_POINT('Ctrl Pts',(-32.2262446694516,64.996218559847,0.));
#95875=CARTESIAN_POINT('Ctrl Pts',(-32.2262446694516,64.996218559847,12.));
#95876=CARTESIAN_POINT('Ctrl Pts',(-32.244714011842,65.0131100130155,0.));
#95877=CARTESIAN_POINT('Ctrl Pts',(-32.244714011842,65.0131100130155,12.));
#95878=CARTESIAN_POINT('Ctrl Pts',(-32.2632290527855,65.0300108378786,0.));
#95879=CARTESIAN_POINT('Ctrl Pts',(-32.2632290527855,65.0300108378786,12.));
#95880=CARTESIAN_POINT('Ctrl Pts',(-32.2817897504799,65.0469209207548,0.));
#95881=CARTESIAN_POINT('Ctrl Pts',(-32.2817897504799,65.0469209207548,12.));
#95882=CARTESIAN_POINT('Ctrl Pts',(-32.3003960632,65.0638401484245,0.));
#95883=CARTESIAN_POINT('Ctrl Pts',(-32.3003960632,65.0638401484245,12.));
#95884=CARTESIAN_POINT('Ctrl Pts',(-32.3190479492985,65.0807684081278,0.));
#95885=CARTESIAN_POINT('Ctrl Pts',(-32.3190479492985,65.0807684081278,12.));
#95886=CARTESIAN_POINT('Ctrl Pts',(-32.3377453672052,65.097705587561,0.));
#95887=CARTESIAN_POINT('Ctrl Pts',(-32.3377453672052,65.097705587561,12.));
#95888=CARTESIAN_POINT('Ctrl Pts',(-32.3564882754212,65.1146515748723,0.));
#95889=CARTESIAN_POINT('Ctrl Pts',(-32.3564882754212,65.1146515748723,12.));
#95890=CARTESIAN_POINT('Ctrl Pts',(-32.3752766325135,65.1316062586586,0.));
#95891=CARTESIAN_POINT('Ctrl Pts',(-32.3752766325135,65.1316062586586,12.));
#95892=CARTESIAN_POINT('Ctrl Pts',(-32.3941103971218,65.1485695279628,0.));
#95893=CARTESIAN_POINT('Ctrl Pts',(-32.3941103971218,65.1485695279628,12.));
#95894=CARTESIAN_POINT('Ctrl Pts',(-32.4129895279612,65.165541272272,0.));
#95895=CARTESIAN_POINT('Ctrl Pts',(-32.4129895279612,65.165541272272,12.));
#95896=CARTESIAN_POINT('Ctrl Pts',(-32.4319139838212,65.182521381514,0.));
#95897=CARTESIAN_POINT('Ctrl Pts',(-32.4319139838212,65.182521381514,12.));
#95898=CARTESIAN_POINT('Ctrl Pts',(-32.4508837235613,65.1995097460546,0.));
#95899=CARTESIAN_POINT('Ctrl Pts',(-32.4508837235613,65.1995097460546,12.));
#95900=CARTESIAN_POINT('Ctrl Pts',(-32.4698987061037,65.2165062566936,0.));
#95901=CARTESIAN_POINT('Ctrl Pts',(-32.4698987061037,65.2165062566936,12.));
#95902=CARTESIAN_POINT('Ctrl Pts',(-32.4889588904397,65.2335108046625,0.));
#95903=CARTESIAN_POINT('Ctrl Pts',(-32.4889588904397,65.2335108046625,12.));
#95904=CARTESIAN_POINT('Ctrl Pts',(-32.508064235633,65.2505232816215,0.));
#95905=CARTESIAN_POINT('Ctrl Pts',(-32.508064235633,65.2505232816215,12.));
#95906=CARTESIAN_POINT('Ctrl Pts',(-32.5272147008191,65.2675435796558,0.));
#95907=CARTESIAN_POINT('Ctrl Pts',(-32.5272147008191,65.2675435796558,12.));
#95908=CARTESIAN_POINT('Ctrl Pts',(-32.5464102452013,65.2845715912717,0.));
#95909=CARTESIAN_POINT('Ctrl Pts',(-32.5464102452013,65.2845715912717,12.));
#95910=CARTESIAN_POINT('Ctrl Pts',(-32.565650828042,65.3016072093907,0.));
#95911=CARTESIAN_POINT('Ctrl Pts',(-32.565650828042,65.3016072093907,12.));
#95912=CARTESIAN_POINT('Ctrl Pts',(-32.5849364086679,65.3186503273498,0.));
#95913=CARTESIAN_POINT('Ctrl Pts',(-32.5849364086679,65.3186503273498,12.));
#95914=CARTESIAN_POINT('Ctrl Pts',(-32.6042669464752,65.3357008389004,0.));
#95915=CARTESIAN_POINT('Ctrl Pts',(-32.6042669464752,65.3357008389004,12.));
#95916=CARTESIAN_POINT('Ctrl Pts',(-32.6236424009302,65.3527586382082,0.));
#95917=CARTESIAN_POINT('Ctrl Pts',(-32.6236424009302,65.3527586382082,12.));
#95918=CARTESIAN_POINT('Ctrl Pts',(-32.6430627315673,65.3698236198511,0.));
#95919=CARTESIAN_POINT('Ctrl Pts',(-32.6430627315673,65.3698236198511,12.));
#95920=CARTESIAN_POINT('Ctrl Pts',(-32.6625278979807,65.3868956788178,0.));
#95921=CARTESIAN_POINT('Ctrl Pts',(-32.6625278979807,65.3868956788178,12.));
#95922=CARTESIAN_POINT('Ctrl Pts',(-32.6820378598262,65.4039747105033,0.));
#95923=CARTESIAN_POINT('Ctrl Pts',(-32.6820378598262,65.4039747105033,12.));
#95924=CARTESIAN_POINT('Ctrl Pts',(-32.7015925768261,65.4210606107029,0.));
#95925=CARTESIAN_POINT('Ctrl Pts',(-32.7015925768261,65.4210606107029,12.));
#95926=CARTESIAN_POINT('Ctrl Pts',(-32.7211920087682,65.4381532756062,0.));
#95927=CARTESIAN_POINT('Ctrl Pts',(-32.7211920087682,65.4381532756062,12.));
#95928=CARTESIAN_POINT('Ctrl Pts',(-32.7408361155038,65.4552526017907,0.));
#95929=CARTESIAN_POINT('Ctrl Pts',(-32.7408361155038,65.4552526017907,12.));
#95930=CARTESIAN_POINT('Ctrl Pts',(-32.7605248569382,65.4723584862129,0.));
#95931=CARTESIAN_POINT('Ctrl Pts',(-32.7605248569382,65.4723584862129,12.));
#95932=CARTESIAN_POINT('Ctrl Pts',(-32.7802581930293,65.4894708262071,0.));
#95933=CARTESIAN_POINT('Ctrl Pts',(-32.7802581930293,65.4894708262071,12.));
#95934=CARTESIAN_POINT('Ctrl Pts',(-32.8000360837981,65.5065895194938,0.));
#95935=CARTESIAN_POINT('Ctrl Pts',(-32.8000360837981,65.5065895194938,12.));
#95936=CARTESIAN_POINT('Ctrl Pts',(-32.8198584893319,65.5237144641864,0.));
#95937=CARTESIAN_POINT('Ctrl Pts',(-32.8198584893319,65.5237144641864,12.));
#95938=CARTESIAN_POINT('Ctrl Pts',(-32.8397253697864,65.5408455587963,0.));
#95939=CARTESIAN_POINT('Ctrl Pts',(-32.8397253697864,65.5408455587963,12.));
#95940=CARTESIAN_POINT('Ctrl Pts',(-32.8596366853826,65.5579827022412,0.));
#95941=CARTESIAN_POINT('Ctrl Pts',(-32.8596366853826,65.5579827022412,12.));
#95942=CARTESIAN_POINT('Ctrl Pts',(-32.8795923964022,65.575125793846,0.));
#95943=CARTESIAN_POINT('Ctrl Pts',(-32.8795923964022,65.575125793846,12.));
#95944=CARTESIAN_POINT('Ctrl Pts',(-32.899592463189,65.5922747333181,0.));
#95945=CARTESIAN_POINT('Ctrl Pts',(-32.899592463189,65.5922747333181,12.));
#95946=CARTESIAN_POINT('Ctrl Pts',(-32.9196368461457,65.6094294207267,0.));
#95947=CARTESIAN_POINT('Ctrl Pts',(-32.9196368461457,65.6094294207267,12.));
#95948=CARTESIAN_POINT('Ctrl Pts',(-32.9397255057273,65.6265897564782,0.));
#95949=CARTESIAN_POINT('Ctrl Pts',(-32.9397255057273,65.6265897564782,12.));
#95950=CARTESIAN_POINT('Ctrl Pts',(-32.9598584024318,65.6437556412956,0.));
#95951=CARTESIAN_POINT('Ctrl Pts',(-32.9598584024318,65.6437556412956,12.));
#95952=CARTESIAN_POINT('Ctrl Pts',(-32.9800354967847,65.6609269761902,0.));
#95953=CARTESIAN_POINT('Ctrl Pts',(-32.9800354967847,65.6609269761902,12.));
#95954=CARTESIAN_POINT('Ctrl Pts',(-33.0002567493581,65.6781036625041,0.));
#95955=CARTESIAN_POINT('Ctrl Pts',(-33.0002567493581,65.6781036625041,12.));
#95956=CARTESIAN_POINT('Ctrl Pts',(-33.0205221207877,65.6952856019542,0.));
#95957=CARTESIAN_POINT('Ctrl Pts',(-33.0205221207877,65.6952856019542,12.));
#95958=CARTESIAN_POINT('Ctrl Pts',(-33.0408315717874,65.7124726966805,0.));
#95959=CARTESIAN_POINT('Ctrl Pts',(-33.0408315717874,65.7124726966805,12.));
#95960=CARTESIAN_POINT('Ctrl Pts',(-33.061185063158,65.729664849282,0.));
#95961=CARTESIAN_POINT('Ctrl Pts',(-33.061185063158,65.729664849282,12.));
#95962=CARTESIAN_POINT('Ctrl Pts',(-33.0815825557976,65.7468619628808,0.));
#95963=CARTESIAN_POINT('Ctrl Pts',(-33.0815825557976,65.7468619628808,12.));
#95964=CARTESIAN_POINT('Ctrl Pts',(-33.102024010688,65.7640639410653,0.));
#95965=CARTESIAN_POINT('Ctrl Pts',(-33.102024010688,65.7640639410653,12.));
#95966=CARTESIAN_POINT('Ctrl Pts',(-33.1225093888669,65.7812706877691,0.));
#95967=CARTESIAN_POINT('Ctrl Pts',(-33.1225093888669,65.7812706877691,12.));
#95968=CARTESIAN_POINT('Ctrl Pts',(-33.1430386513975,65.7984821071621,0.));
#95969=CARTESIAN_POINT('Ctrl Pts',(-33.1430386513975,65.7984821071621,12.));
#95970=CARTESIAN_POINT('Ctrl Pts',(-33.16361175934,65.8156981035504,0.));
#95971=CARTESIAN_POINT('Ctrl Pts',(-33.16361175934,65.8156981035504,12.));
#95972=CARTESIAN_POINT('Ctrl Pts',(-33.1842286737053,65.8329185812379,0.));
#95973=CARTESIAN_POINT('Ctrl Pts',(-33.1842286737053,65.8329185812379,12.));
#95974=CARTESIAN_POINT('Ctrl Pts',(-33.2048893554496,65.8501434445174,0.));
#95975=CARTESIAN_POINT('Ctrl Pts',(-33.2048893554496,65.8501434445174,12.));
#95976=CARTESIAN_POINT('Ctrl Pts',(-33.2255937655656,65.8673725979591,0.));
#95977=CARTESIAN_POINT('Ctrl Pts',(-33.2255937655656,65.8673725979591,12.));
#95978=CARTESIAN_POINT('Ctrl Pts',(-33.2463418651498,65.8846059466382,0.));
#95979=CARTESIAN_POINT('Ctrl Pts',(-33.2463418651498,65.8846059466382,12.));
#95980=CARTESIAN_POINT('Ctrl Pts',(-33.2671336154754,65.901843396389,0.));
#95981=CARTESIAN_POINT('Ctrl Pts',(-33.2671336154754,65.901843396389,12.));
#95982=CARTESIAN_POINT('Ctrl Pts',(-33.2879689780566,65.9190848540422,0.));
#95983=CARTESIAN_POINT('Ctrl Pts',(-33.2879689780566,65.9190848540422,12.));
#95984=CARTESIAN_POINT('Ctrl Pts',(-33.3088479147151,65.9363302276822,0.));
#95985=CARTESIAN_POINT('Ctrl Pts',(-33.3088479147151,65.9363302276822,12.));
#95986=CARTESIAN_POINT('Ctrl Pts',(-33.3297703874249,65.9535794260802,0.));
#95987=CARTESIAN_POINT('Ctrl Pts',(-33.3297703874249,65.9535794260802,12.));
#95988=CARTESIAN_POINT('Ctrl Pts',(-33.3507363581579,65.9708323581385,0.));
#95989=CARTESIAN_POINT('Ctrl Pts',(-33.3507363581579,65.9708323581385,12.));
#95990=CARTESIAN_POINT('Ctrl Pts',(-33.3717457887095,65.9880889322822,0.));
#95991=CARTESIAN_POINT('Ctrl Pts',(-33.3717457887095,65.9880889322822,12.));
#95992=CARTESIAN_POINT('Ctrl Pts',(-33.3927986405612,66.0053490559826,0.));
#95993=CARTESIAN_POINT('Ctrl Pts',(-33.3927986405612,66.0053490559826,12.));
#95994=CARTESIAN_POINT('Ctrl Pts',(-33.4138948746408,66.0226126349482,0.));
#95995=CARTESIAN_POINT('Ctrl Pts',(-33.4138948746408,66.0226126349482,12.));
#95996=CARTESIAN_POINT('Ctrl Pts',(-33.4350344515128,66.0398795737827,0.));
#95997=CARTESIAN_POINT('Ctrl Pts',(-33.4350344515128,66.0398795737827,12.));
#95998=CARTESIAN_POINT('Ctrl Pts',(-33.4562173318053,66.0571497774484,0.));
#95999=CARTESIAN_POINT('Ctrl Pts',(-33.4562173318053,66.0571497774484,12.));
#96000=CARTESIAN_POINT('Ctrl Pts',(-33.4774434765762,66.0744231525445,0.));
#96001=CARTESIAN_POINT('Ctrl Pts',(-33.4774434765762,66.0744231525445,12.));
#96002=CARTESIAN_POINT('Ctrl Pts',(-33.4987128476618,66.0916996085237,0.));
#96003=CARTESIAN_POINT('Ctrl Pts',(-33.4987128476618,66.0916996085237,12.));
#96004=CARTESIAN_POINT('Ctrl Pts',(-33.5200254081212,66.1089790592673,0.));
#96005=CARTESIAN_POINT('Ctrl Pts',(-33.5200254081212,66.1089790592673,12.));
#96006=CARTESIAN_POINT('Ctrl Pts',(-33.5413811223398,66.1262614234579,0.));
#96007=CARTESIAN_POINT('Ctrl Pts',(-33.5413811223398,66.1262614234579,12.));
#96008=CARTESIAN_POINT('Ctrl Pts',(-33.5627799550422,66.1435466210966,0.));
#96009=CARTESIAN_POINT('Ctrl Pts',(-33.5627799550422,66.1435466210966,12.));
#96010=CARTESIAN_POINT('Ctrl Pts',(-33.5842218705103,66.1608345707552,0.));
#96011=CARTESIAN_POINT('Ctrl Pts',(-33.5842218705103,66.1608345707552,12.));
#96012=CARTESIAN_POINT('Ctrl Pts',(-33.6057068316758,66.1781251863998,0.));
#96013=CARTESIAN_POINT('Ctrl Pts',(-33.6057068316758,66.1781251863998,12.));
#96014=CARTESIAN_POINT('Ctrl Pts',(-33.6272347993519,66.1954183747167,0.));
#96015=CARTESIAN_POINT('Ctrl Pts',(-33.6272347993519,66.1954183747167,12.));
#96016=CARTESIAN_POINT('Ctrl Pts',(-33.648805731163,66.2127140313777,0.));
#96017=CARTESIAN_POINT('Ctrl Pts',(-33.648805731163,66.2127140313777,12.));
#96018=CARTESIAN_POINT('Ctrl Pts',(-33.6704195830526,66.2300120464323,0.));
#96019=CARTESIAN_POINT('Ctrl Pts',(-33.6704195830526,66.2300120464323,12.));
#96020=CARTESIAN_POINT('Ctrl Pts',(-33.6920763111575,66.2473123109626,0.));
#96021=CARTESIAN_POINT('Ctrl Pts',(-33.6920763111575,66.2473123109626,12.));
#96022=CARTESIAN_POINT('Ctrl Pts',(-33.713775873597,66.2646147235444,0.));
#96023=CARTESIAN_POINT('Ctrl Pts',(-33.713775873597,66.2646147235444,12.));
#96024=CARTESIAN_POINT('Ctrl Pts',(-33.7355182321862,66.2819191962273,0.));
#96025=CARTESIAN_POINT('Ctrl Pts',(-33.7355182321862,66.2819191962273,12.));
#96026=CARTESIAN_POINT('Ctrl Pts',(-33.7573033544374,66.2992256621001,0.));
#96027=CARTESIAN_POINT('Ctrl Pts',(-33.7573033544374,66.2992256621001,12.));
#96028=CARTESIAN_POINT('Ctrl Pts',(-33.7791312144798,66.3165340771053,0.));
#96029=CARTESIAN_POINT('Ctrl Pts',(-33.7791312144798,66.3165340771053,12.));
#96030=CARTESIAN_POINT('Ctrl Pts',(-33.8010017925666,66.3338444143559,0.));
#96031=CARTESIAN_POINT('Ctrl Pts',(-33.8010017925666,66.3338444143559,12.));
#96032=CARTESIAN_POINT('Ctrl Pts',(-33.8185324184602,66.3476942111456,0.));
#96033=CARTESIAN_POINT('Ctrl Pts',(-33.8185324184602,66.3476942111456,12.));
#96034=CARTESIAN_POINT('Ctrl Pts',(-33.831699601175,66.3580824155565,0.));
#96035=CARTESIAN_POINT('Ctrl Pts',(-33.831699601175,66.3580824155565,12.));
#96036=CARTESIAN_POINT('Ctrl Pts',(-33.8404862618803,66.3650082659593,0.));
#96037=CARTESIAN_POINT('Ctrl Pts',(-33.8404862618803,66.3650082659593,12.));
#96038=CARTESIAN_POINT('Ctrl Pts',(-33.8448817269567,66.3684712863594,0.));
#96039=CARTESIAN_POINT('Ctrl Pts',(-33.8448817269567,66.3684712863594,12.));
#96040=CARTESIAN_POINT('',(-30.3549065457811,63.0759831361898,0.));
#96041=CARTESIAN_POINT('Ctrl Pts',(-30.3549065457811,63.0759831361898,0.));
#96042=CARTESIAN_POINT('Ctrl Pts',(-30.357431906933,63.078933570069,0.));
#96043=CARTESIAN_POINT('Ctrl Pts',(-30.3624877680651,63.0848371718048,0.));
#96044=CARTESIAN_POINT('Ctrl Pts',(-30.3700869762507,63.0937007763471,0.));
#96045=CARTESIAN_POINT('Ctrl Pts',(-30.3802500880403,63.105535320226,0.));
#96046=CARTESIAN_POINT('Ctrl Pts',(-30.3930053710484,63.1203558300657,0.));
#96047=CARTESIAN_POINT('Ctrl Pts',(-30.4058120432228,63.135203629844,0.));
#96048=CARTESIAN_POINT('Ctrl Pts',(-30.418670087563,63.1500786361459,0.));
#96049=CARTESIAN_POINT('Ctrl Pts',(-30.4315794659731,63.164980701691,0.));
#96050=CARTESIAN_POINT('Ctrl Pts',(-30.4445401192381,63.179909617189,0.));
#96051=CARTESIAN_POINT('Ctrl Pts',(-30.4575519763337,63.1948651386942,0.));
#96052=CARTESIAN_POINT('Ctrl Pts',(-30.470614961416,63.2098470086636,0.));
#96053=CARTESIAN_POINT('Ctrl Pts',(-30.4837290014989,63.2248549788221,0.));
#96054=CARTESIAN_POINT('Ctrl Pts',(-30.4968940344998,63.2398888342545,0.));
#96055=CARTESIAN_POINT('Ctrl Pts',(-30.5101100066659,63.2549483856215,0.));
#96056=CARTESIAN_POINT('Ctrl Pts',(-30.5233768687865,63.2700334577639,0.));
#96057=CARTESIAN_POINT('Ctrl Pts',(-30.5366945730508,63.2851438802473,0.));
#96058=CARTESIAN_POINT('Ctrl Pts',(-30.5500630691359,63.3002794756086,0.));
#96059=CARTESIAN_POINT('Ctrl Pts',(-30.563482302238,63.3154400534397,0.));
#96060=CARTESIAN_POINT('Ctrl Pts',(-30.5769522151164,63.3306254165126,0.));
#96061=CARTESIAN_POINT('Ctrl Pts',(-30.5904727493712,63.3458353646154,0.));
#96062=CARTESIAN_POINT('Ctrl Pts',(-30.6040438469078,63.3610696989577,0.));
#96063=CARTESIAN_POINT('Ctrl Pts',(-30.6176654515967,63.3763282271796,0.));
#96064=CARTESIAN_POINT('Ctrl Pts',(-30.6313375092062,63.3916107631376,0.));
#96065=CARTESIAN_POINT('Ctrl Pts',(-30.6450599666121,63.4069171245066,0.));
#96066=CARTESIAN_POINT('Ctrl Pts',(-30.6588327712484,63.4222471311239,0.));
#96067=CARTESIAN_POINT('Ctrl Pts',(-30.6726558704315,63.4376006029604,0.));
#96068=CARTESIAN_POINT('Ctrl Pts',(-30.6865292107929,63.4529773584249,0.));
#96069=CARTESIAN_POINT('Ctrl Pts',(-30.7004527385821,63.4683772152529,0.));
#96070=CARTESIAN_POINT('Ctrl Pts',(-30.7144263999265,63.4837999912771,0.));
#96071=CARTESIAN_POINT('Ctrl Pts',(-30.7284501410822,63.4992455051795,0.));
#96072=CARTESIAN_POINT('Ctrl Pts',(-30.7425239087281,63.5147135773894,0.));
#96073=CARTESIAN_POINT('Ctrl Pts',(-30.7566476500757,63.5302040304142,0.));
#96074=CARTESIAN_POINT('Ctrl Pts',(-30.7708213127159,63.5457166883537,0.));
#96075=CARTESIAN_POINT('Ctrl Pts',(-30.7850448445205,63.5612513766,0.));
#96076=CARTESIAN_POINT('Ctrl Pts',(-30.7993181935271,63.5768079214881,0.));
#96077=CARTESIAN_POINT('Ctrl Pts',(-30.813641307801,63.5923861498987,0.));
#96078=CARTESIAN_POINT('Ctrl Pts',(-30.8280141354459,63.6079858892771,0.));
#96079=CARTESIAN_POINT('Ctrl Pts',(-30.8424366246671,63.6236069678055,0.));
#96080=CARTESIAN_POINT('Ctrl Pts',(-30.8569087238131,63.6392492145233,0.));
#96081=CARTESIAN_POINT('Ctrl Pts',(-30.8714303814194,63.6549124594666,0.));
#96082=CARTESIAN_POINT('Ctrl Pts',(-30.8860015462475,63.6705965337971,0.));
#96083=CARTESIAN_POINT('Ctrl Pts',(-30.900622167269,63.6863012697328,0.));
#96084=CARTESIAN_POINT('Ctrl Pts',(-30.9152921936465,63.7020265004792,0.));
#96085=CARTESIAN_POINT('Ctrl Pts',(-30.9300115747115,63.7177720601609,0.));
#96086=CARTESIAN_POINT('Ctrl Pts',(-30.9447802599355,63.7335377837441,0.));
#96087=CARTESIAN_POINT('Ctrl Pts',(-30.9595981989104,63.749323506987,0.));
#96088=CARTESIAN_POINT('Ctrl Pts',(-30.9744653413689,63.7651290664733,0.));
#96089=CARTESIAN_POINT('Ctrl Pts',(-30.989381637191,63.7809542996264,0.));
#96090=CARTESIAN_POINT('Ctrl Pts',(-31.0043470364108,63.796799044728,0.));
#96091=CARTESIAN_POINT('Ctrl Pts',(-31.0193614892171,63.8126631409364,0.));
#96092=CARTESIAN_POINT('Ctrl Pts',(-31.0344249459538,63.8285464282846,0.));
#96093=CARTESIAN_POINT('Ctrl Pts',(-31.0495373571215,63.8444487476611,0.));
#96094=CARTESIAN_POINT('Ctrl Pts',(-31.0646986733723,63.8603699407922,0.));
#96095=CARTESIAN_POINT('Ctrl Pts',(-31.0799088455041,63.8763098502237,0.));
#96096=CARTESIAN_POINT('Ctrl Pts',(-31.0951678244455,63.8922683192964,0.));
#96097=CARTESIAN_POINT('Ctrl Pts',(-31.1104755612607,63.9082451921448,0.));
#96098=CARTESIAN_POINT('Ctrl Pts',(-31.1258320071545,63.9242403136955,0.));
#96099=CARTESIAN_POINT('Ctrl Pts',(-31.1412371134727,63.940253529665,0.));
#96100=CARTESIAN_POINT('Ctrl Pts',(-31.1566908316992,63.9562846865567,0.));
#96101=CARTESIAN_POINT('Ctrl Pts',(-31.1721931134487,63.9723336316551,0.));
#96102=CARTESIAN_POINT('Ctrl Pts',(-31.1877439104717,63.9884002130211,0.));
#96103=CARTESIAN_POINT('Ctrl Pts',(-31.2033431746558,64.0044842794831,0.));
#96104=CARTESIAN_POINT('Ctrl Pts',(-31.2189908580245,64.02058568063,0.));
#96105=CARTESIAN_POINT('Ctrl Pts',(-31.2346869127297,64.0367042667984,0.));
#96106=CARTESIAN_POINT('Ctrl Pts',(-31.2504312910451,64.0528398890657,0.));
#96107=CARTESIAN_POINT('Ctrl Pts',(-31.2662239453728,64.0689923992461,0.));
#96108=CARTESIAN_POINT('Ctrl Pts',(-31.2820648282447,64.0851616498852,0.));
#96109=CARTESIAN_POINT('Ctrl Pts',(-31.2979538923214,64.1013474942556,0.));
#96110=CARTESIAN_POINT('Ctrl Pts',(-31.3138910903859,64.117549786349,0.));
#96111=CARTESIAN_POINT('Ctrl Pts',(-31.3298763753377,64.133768380869,0.));
#96112=CARTESIAN_POINT('Ctrl Pts',(-31.3459097002006,64.1500031332282,0.));
#96113=CARTESIAN_POINT('Ctrl Pts',(-31.3619910181228,64.166253899542,0.));
#96114=CARTESIAN_POINT('Ctrl Pts',(-31.3781202823754,64.1825205366224,0.));
#96115=CARTESIAN_POINT('Ctrl Pts',(-31.3942974463445,64.1988029019707,0.));
#96116=CARTESIAN_POINT('Ctrl Pts',(-31.410522463528,64.2151008537697,0.));
#96117=CARTESIAN_POINT('Ctrl Pts',(-31.4267952875423,64.231414250881,0.));
#96118=CARTESIAN_POINT('Ctrl Pts',(-31.4431158721222,64.2477429528393,0.));
#96119=CARTESIAN_POINT('Ctrl Pts',(-31.4594841711195,64.2640868198473,0.));
#96120=CARTESIAN_POINT('Ctrl Pts',(-31.4759001384941,64.2804457127671,0.));
#96121=CARTESIAN_POINT('Ctrl Pts',(-31.4923637283132,64.2968194931158,0.));
#96122=CARTESIAN_POINT('Ctrl Pts',(-31.5088748947582,64.3132080230637,0.));
#96123=CARTESIAN_POINT('Ctrl Pts',(-31.5254335921245,64.3296111654283,0.));
#96124=CARTESIAN_POINT('Ctrl Pts',(-31.5420397748191,64.3460287836687,0.));
#96125=CARTESIAN_POINT('Ctrl Pts',(-31.5586933973515,64.3624607418768,0.));
#96126=CARTESIAN_POINT('Ctrl Pts',(-31.5753944143336,64.3789069047733,0.));
#96127=CARTESIAN_POINT('Ctrl Pts',(-31.5921427804865,64.3953671377046,0.));
#96128=CARTESIAN_POINT('Ctrl Pts',(-31.6089384506395,64.4118413066378,0.));
#96129=CARTESIAN_POINT('Ctrl Pts',(-31.6257813797287,64.4283292781565,0.));
#96130=CARTESIAN_POINT('Ctrl Pts',(-31.6426715227878,64.4448309194525,0.));
#96131=CARTESIAN_POINT('Ctrl Pts',(-31.6596088349482,64.4613460983214,0.));
#96132=CARTESIAN_POINT('Ctrl Pts',(-31.6765932714464,64.4778746831614,0.));
#96133=CARTESIAN_POINT('Ctrl Pts',(-31.6936247876229,64.4944165429675,0.));
#96134=CARTESIAN_POINT('Ctrl Pts',(-31.7107033389201,64.510971547327,0.));
#96135=CARTESIAN_POINT('Ctrl Pts',(-31.7278288808731,64.5275395664124,0.));
#96136=CARTESIAN_POINT('Ctrl Pts',(-31.7450013691112,64.544120470977,0.));
#96137=CARTESIAN_POINT('Ctrl Pts',(-31.7622207593634,64.5607141323521,0.));
#96138=CARTESIAN_POINT('Ctrl Pts',(-31.7794870074583,64.5773204224429,0.));
#96139=CARTESIAN_POINT('Ctrl Pts',(-31.7968000693218,64.5939392137235,0.));
#96140=CARTESIAN_POINT('Ctrl Pts',(-31.8141599009684,64.6105703792312,0.));
#96141=CARTESIAN_POINT('Ctrl Pts',(-31.8315664585026,64.6272137925627,0.));
#96142=CARTESIAN_POINT('Ctrl Pts',(-31.8490196981248,64.6438693278714,0.));
#96143=CARTESIAN_POINT('Ctrl Pts',(-31.866519576131,64.6605368598629,0.));
#96144=CARTESIAN_POINT('Ctrl Pts',(-31.8840660489107,64.6772162637907,0.));
#96145=CARTESIAN_POINT('Ctrl Pts',(-31.9016590729374,64.6939074154498,0.));
#96146=CARTESIAN_POINT('Ctrl Pts',(-31.9192986047706,64.7106101911732,0.));
#96147=CARTESIAN_POINT('Ctrl Pts',(-31.9369846010615,64.7273244678297,0.));
#96148=CARTESIAN_POINT('Ctrl Pts',(-31.9547170185534,64.7440501228202,0.));
#96149=CARTESIAN_POINT('Ctrl Pts',(-31.9724958140789,64.7607870340735,0.));
#96150=CARTESIAN_POINT('Ctrl Pts',(-31.990320944552,64.77753508004,0.));
#96151=CARTESIAN_POINT('Ctrl Pts',(-32.0081923669677,64.7942941396881,0.));
#96152=CARTESIAN_POINT('Ctrl Pts',(-32.0261100384092,64.8110640925021,0.));
#96153=CARTESIAN_POINT('Ctrl Pts',(-32.0440739160477,64.8278448184786,0.));
#96154=CARTESIAN_POINT('Ctrl Pts',(-32.0620839571408,64.8446361981234,0.));
#96155=CARTESIAN_POINT('Ctrl Pts',(-32.0801401190241,64.861438112445,0.));
#96156=CARTESIAN_POINT('Ctrl Pts',(-32.0982423591108,64.878250442952,0.));
#96157=CARTESIAN_POINT('Ctrl Pts',(-32.1163906348979,64.8950730716493,0.));
#96158=CARTESIAN_POINT('Ctrl Pts',(-32.1345849039671,64.9119058810362,0.));
#96159=CARTESIAN_POINT('Ctrl Pts',(-32.1528251239832,64.9287487541018,0.));
#96160=CARTESIAN_POINT('Ctrl Pts',(-32.171111252686,64.9456015743203,0.));
#96161=CARTESIAN_POINT('Ctrl Pts',(-32.1894432478889,64.9624642256477,0.));
#96162=CARTESIAN_POINT('Ctrl Pts',(-32.2078210674857,64.9793365925194,0.));
#96163=CARTESIAN_POINT('Ctrl Pts',(-32.2262446694516,64.996218559847,0.));
#96164=CARTESIAN_POINT('Ctrl Pts',(-32.244714011842,65.0131100130155,0.));
#96165=CARTESIAN_POINT('Ctrl Pts',(-32.2632290527855,65.0300108378786,0.));
#96166=CARTESIAN_POINT('Ctrl Pts',(-32.2817897504799,65.0469209207548,0.));
#96167=CARTESIAN_POINT('Ctrl Pts',(-32.3003960632,65.0638401484245,0.));
#96168=CARTESIAN_POINT('Ctrl Pts',(-32.3190479492985,65.0807684081278,0.));
#96169=CARTESIAN_POINT('Ctrl Pts',(-32.3377453672052,65.097705587561,0.));
#96170=CARTESIAN_POINT('Ctrl Pts',(-32.3564882754212,65.1146515748723,0.));
#96171=CARTESIAN_POINT('Ctrl Pts',(-32.3752766325135,65.1316062586586,0.));
#96172=CARTESIAN_POINT('Ctrl Pts',(-32.3941103971218,65.1485695279628,0.));
#96173=CARTESIAN_POINT('Ctrl Pts',(-32.4129895279612,65.165541272272,0.));
#96174=CARTESIAN_POINT('Ctrl Pts',(-32.4319139838212,65.182521381514,0.));
#96175=CARTESIAN_POINT('Ctrl Pts',(-32.4508837235613,65.1995097460546,0.));
#96176=CARTESIAN_POINT('Ctrl Pts',(-32.4698987061037,65.2165062566936,0.));
#96177=CARTESIAN_POINT('Ctrl Pts',(-32.4889588904397,65.2335108046625,0.));
#96178=CARTESIAN_POINT('Ctrl Pts',(-32.508064235633,65.2505232816215,0.));
#96179=CARTESIAN_POINT('Ctrl Pts',(-32.5272147008191,65.2675435796558,0.));
#96180=CARTESIAN_POINT('Ctrl Pts',(-32.5464102452013,65.2845715912717,0.));
#96181=CARTESIAN_POINT('Ctrl Pts',(-32.565650828042,65.3016072093907,0.));
#96182=CARTESIAN_POINT('Ctrl Pts',(-32.5849364086679,65.3186503273498,0.));
#96183=CARTESIAN_POINT('Ctrl Pts',(-32.6042669464752,65.3357008389004,0.));
#96184=CARTESIAN_POINT('Ctrl Pts',(-32.6236424009302,65.3527586382082,0.));
#96185=CARTESIAN_POINT('Ctrl Pts',(-32.6430627315673,65.3698236198511,0.));
#96186=CARTESIAN_POINT('Ctrl Pts',(-32.6625278979807,65.3868956788178,0.));
#96187=CARTESIAN_POINT('Ctrl Pts',(-32.6820378598262,65.4039747105033,0.));
#96188=CARTESIAN_POINT('Ctrl Pts',(-32.7015925768261,65.4210606107029,0.));
#96189=CARTESIAN_POINT('Ctrl Pts',(-32.7211920087682,65.4381532756062,0.));
#96190=CARTESIAN_POINT('Ctrl Pts',(-32.7408361155038,65.4552526017907,0.));
#96191=CARTESIAN_POINT('Ctrl Pts',(-32.7605248569382,65.4723584862129,0.));
#96192=CARTESIAN_POINT('Ctrl Pts',(-32.7802581930293,65.4894708262071,0.));
#96193=CARTESIAN_POINT('Ctrl Pts',(-32.8000360837981,65.5065895194938,0.));
#96194=CARTESIAN_POINT('Ctrl Pts',(-32.8198584893319,65.5237144641864,0.));
#96195=CARTESIAN_POINT('Ctrl Pts',(-32.8397253697864,65.5408455587963,0.));
#96196=CARTESIAN_POINT('Ctrl Pts',(-32.8596366853826,65.5579827022412,0.));
#96197=CARTESIAN_POINT('Ctrl Pts',(-32.8795923964022,65.575125793846,0.));
#96198=CARTESIAN_POINT('Ctrl Pts',(-32.899592463189,65.5922747333181,0.));
#96199=CARTESIAN_POINT('Ctrl Pts',(-32.9196368461457,65.6094294207267,0.));
#96200=CARTESIAN_POINT('Ctrl Pts',(-32.9397255057273,65.6265897564782,0.));
#96201=CARTESIAN_POINT('Ctrl Pts',(-32.9598584024318,65.6437556412956,0.));
#96202=CARTESIAN_POINT('Ctrl Pts',(-32.9800354967847,65.6609269761902,0.));
#96203=CARTESIAN_POINT('Ctrl Pts',(-33.0002567493581,65.6781036625041,0.));
#96204=CARTESIAN_POINT('Ctrl Pts',(-33.0205221207877,65.6952856019542,0.));
#96205=CARTESIAN_POINT('Ctrl Pts',(-33.0408315717874,65.7124726966805,0.));
#96206=CARTESIAN_POINT('Ctrl Pts',(-33.061185063158,65.729664849282,0.));
#96207=CARTESIAN_POINT('Ctrl Pts',(-33.0815825557976,65.7468619628808,0.));
#96208=CARTESIAN_POINT('Ctrl Pts',(-33.102024010688,65.7640639410653,0.));
#96209=CARTESIAN_POINT('Ctrl Pts',(-33.1225093888669,65.7812706877691,0.));
#96210=CARTESIAN_POINT('Ctrl Pts',(-33.1430386513975,65.7984821071621,0.));
#96211=CARTESIAN_POINT('Ctrl Pts',(-33.16361175934,65.8156981035504,0.));
#96212=CARTESIAN_POINT('Ctrl Pts',(-33.1842286737053,65.8329185812379,0.));
#96213=CARTESIAN_POINT('Ctrl Pts',(-33.2048893554496,65.8501434445174,0.));
#96214=CARTESIAN_POINT('Ctrl Pts',(-33.2255937655656,65.8673725979591,0.));
#96215=CARTESIAN_POINT('Ctrl Pts',(-33.2463418651498,65.8846059466382,0.));
#96216=CARTESIAN_POINT('Ctrl Pts',(-33.2671336154754,65.901843396389,0.));
#96217=CARTESIAN_POINT('Ctrl Pts',(-33.2879689780566,65.9190848540422,0.));
#96218=CARTESIAN_POINT('Ctrl Pts',(-33.3088479147151,65.9363302276822,0.));
#96219=CARTESIAN_POINT('Ctrl Pts',(-33.3297703874249,65.9535794260802,0.));
#96220=CARTESIAN_POINT('Ctrl Pts',(-33.3507363581579,65.9708323581385,0.));
#96221=CARTESIAN_POINT('Ctrl Pts',(-33.3717457887095,65.9880889322822,0.));
#96222=CARTESIAN_POINT('Ctrl Pts',(-33.3927986405612,66.0053490559826,0.));
#96223=CARTESIAN_POINT('Ctrl Pts',(-33.4138948746408,66.0226126349482,0.));
#96224=CARTESIAN_POINT('Ctrl Pts',(-33.4350344515128,66.0398795737827,0.));
#96225=CARTESIAN_POINT('Ctrl Pts',(-33.4562173318053,66.0571497774484,0.));
#96226=CARTESIAN_POINT('Ctrl Pts',(-33.4774434765762,66.0744231525445,0.));
#96227=CARTESIAN_POINT('Ctrl Pts',(-33.4987128476618,66.0916996085237,0.));
#96228=CARTESIAN_POINT('Ctrl Pts',(-33.5200254081212,66.1089790592673,0.));
#96229=CARTESIAN_POINT('Ctrl Pts',(-33.5413811223398,66.1262614234579,0.));
#96230=CARTESIAN_POINT('Ctrl Pts',(-33.5597240685729,66.1410781873125,0.));
#96231=CARTESIAN_POINT('Ctrl Pts',(-33.5738105077707,66.1524393973986,0.));
#96232=CARTESIAN_POINT('Ctrl Pts',(-33.5836213513974,66.1603438177306,0.));
#96233=CARTESIAN_POINT('Ctrl Pts',(-33.5891439876228,66.1647906582409,0.));
#96234=CARTESIAN_POINT('Ctrl Pts',(-33.5903722664959,66.165779540567,0.));
#96235=CARTESIAN_POINT('',(-30.3549065457811,63.0759831361898,12.));
#96236=CARTESIAN_POINT('',(-30.3549065457811,63.0759831361898,0.));
#96237=CARTESIAN_POINT('Ctrl Pts',(-33.590372266496,66.1657795405671,12.));
#96238=CARTESIAN_POINT('Ctrl Pts',(-33.5891439876229,66.164790658241,12.));
#96239=CARTESIAN_POINT('Ctrl Pts',(-33.5836213513975,66.1603438177307,12.));
#96240=CARTESIAN_POINT('Ctrl Pts',(-33.5738105077708,66.1524393973986,12.));
#96241=CARTESIAN_POINT('Ctrl Pts',(-33.5597240685729,66.1410781873125,12.));
#96242=CARTESIAN_POINT('Ctrl Pts',(-33.5413811223398,66.1262614234579,12.));
#96243=CARTESIAN_POINT('Ctrl Pts',(-33.5200254081212,66.1089790592673,12.));
#96244=CARTESIAN_POINT('Ctrl Pts',(-33.4987128476618,66.0916996085237,12.));
#96245=CARTESIAN_POINT('Ctrl Pts',(-33.4774434765762,66.0744231525445,12.));
#96246=CARTESIAN_POINT('Ctrl Pts',(-33.4562173318053,66.0571497774484,12.));
#96247=CARTESIAN_POINT('Ctrl Pts',(-33.4350344515128,66.0398795737827,12.));
#96248=CARTESIAN_POINT('Ctrl Pts',(-33.4138948746408,66.0226126349482,12.));
#96249=CARTESIAN_POINT('Ctrl Pts',(-33.3927986405612,66.0053490559826,12.));
#96250=CARTESIAN_POINT('Ctrl Pts',(-33.3717457887095,65.9880889322822,12.));
#96251=CARTESIAN_POINT('Ctrl Pts',(-33.3507363581579,65.9708323581385,12.));
#96252=CARTESIAN_POINT('Ctrl Pts',(-33.3297703874249,65.9535794260802,12.));
#96253=CARTESIAN_POINT('Ctrl Pts',(-33.3088479147151,65.9363302276822,12.));
#96254=CARTESIAN_POINT('Ctrl Pts',(-33.2879689780566,65.9190848540422,12.));
#96255=CARTESIAN_POINT('Ctrl Pts',(-33.2671336154754,65.901843396389,12.));
#96256=CARTESIAN_POINT('Ctrl Pts',(-33.2463418651498,65.8846059466382,12.));
#96257=CARTESIAN_POINT('Ctrl Pts',(-33.2255937655656,65.8673725979591,12.));
#96258=CARTESIAN_POINT('Ctrl Pts',(-33.2048893554496,65.8501434445174,12.));
#96259=CARTESIAN_POINT('Ctrl Pts',(-33.1842286737053,65.8329185812379,12.));
#96260=CARTESIAN_POINT('Ctrl Pts',(-33.16361175934,65.8156981035504,12.));
#96261=CARTESIAN_POINT('Ctrl Pts',(-33.1430386513975,65.7984821071621,12.));
#96262=CARTESIAN_POINT('Ctrl Pts',(-33.1225093888669,65.7812706877691,12.));
#96263=CARTESIAN_POINT('Ctrl Pts',(-33.102024010688,65.7640639410653,12.));
#96264=CARTESIAN_POINT('Ctrl Pts',(-33.0815825557976,65.7468619628808,12.));
#96265=CARTESIAN_POINT('Ctrl Pts',(-33.061185063158,65.729664849282,12.));
#96266=CARTESIAN_POINT('Ctrl Pts',(-33.0408315717874,65.7124726966805,12.));
#96267=CARTESIAN_POINT('Ctrl Pts',(-33.0205221207877,65.6952856019542,12.));
#96268=CARTESIAN_POINT('Ctrl Pts',(-33.0002567493581,65.6781036625041,12.));
#96269=CARTESIAN_POINT('Ctrl Pts',(-32.9800354967847,65.6609269761902,12.));
#96270=CARTESIAN_POINT('Ctrl Pts',(-32.9598584024318,65.6437556412956,12.));
#96271=CARTESIAN_POINT('Ctrl Pts',(-32.9397255057273,65.6265897564782,12.));
#96272=CARTESIAN_POINT('Ctrl Pts',(-32.9196368461457,65.6094294207267,12.));
#96273=CARTESIAN_POINT('Ctrl Pts',(-32.899592463189,65.5922747333181,12.));
#96274=CARTESIAN_POINT('Ctrl Pts',(-32.8795923964022,65.575125793846,12.));
#96275=CARTESIAN_POINT('Ctrl Pts',(-32.8596366853826,65.5579827022412,12.));
#96276=CARTESIAN_POINT('Ctrl Pts',(-32.8397253697864,65.5408455587963,12.));
#96277=CARTESIAN_POINT('Ctrl Pts',(-32.8198584893319,65.5237144641864,12.));
#96278=CARTESIAN_POINT('Ctrl Pts',(-32.8000360837981,65.5065895194938,12.));
#96279=CARTESIAN_POINT('Ctrl Pts',(-32.7802581930293,65.4894708262071,12.));
#96280=CARTESIAN_POINT('Ctrl Pts',(-32.7605248569382,65.4723584862129,12.));
#96281=CARTESIAN_POINT('Ctrl Pts',(-32.7408361155038,65.4552526017907,12.));
#96282=CARTESIAN_POINT('Ctrl Pts',(-32.7211920087682,65.4381532756062,12.));
#96283=CARTESIAN_POINT('Ctrl Pts',(-32.7015925768261,65.4210606107029,12.));
#96284=CARTESIAN_POINT('Ctrl Pts',(-32.6820378598262,65.4039747105033,12.));
#96285=CARTESIAN_POINT('Ctrl Pts',(-32.6625278979807,65.3868956788178,12.));
#96286=CARTESIAN_POINT('Ctrl Pts',(-32.6430627315673,65.3698236198511,12.));
#96287=CARTESIAN_POINT('Ctrl Pts',(-32.6236424009302,65.3527586382082,12.));
#96288=CARTESIAN_POINT('Ctrl Pts',(-32.6042669464752,65.3357008389004,12.));
#96289=CARTESIAN_POINT('Ctrl Pts',(-32.5849364086679,65.3186503273498,12.));
#96290=CARTESIAN_POINT('Ctrl Pts',(-32.565650828042,65.3016072093907,12.));
#96291=CARTESIAN_POINT('Ctrl Pts',(-32.5464102452013,65.2845715912717,12.));
#96292=CARTESIAN_POINT('Ctrl Pts',(-32.5272147008191,65.2675435796558,12.));
#96293=CARTESIAN_POINT('Ctrl Pts',(-32.508064235633,65.2505232816215,12.));
#96294=CARTESIAN_POINT('Ctrl Pts',(-32.4889588904397,65.2335108046625,12.));
#96295=CARTESIAN_POINT('Ctrl Pts',(-32.4698987061037,65.2165062566936,12.));
#96296=CARTESIAN_POINT('Ctrl Pts',(-32.4508837235613,65.1995097460546,12.));
#96297=CARTESIAN_POINT('Ctrl Pts',(-32.4319139838212,65.182521381514,12.));
#96298=CARTESIAN_POINT('Ctrl Pts',(-32.4129895279612,65.165541272272,12.));
#96299=CARTESIAN_POINT('Ctrl Pts',(-32.3941103971218,65.1485695279628,12.));
#96300=CARTESIAN_POINT('Ctrl Pts',(-32.3752766325135,65.1316062586586,12.));
#96301=CARTESIAN_POINT('Ctrl Pts',(-32.3564882754212,65.1146515748723,12.));
#96302=CARTESIAN_POINT('Ctrl Pts',(-32.3377453672052,65.097705587561,12.));
#96303=CARTESIAN_POINT('Ctrl Pts',(-32.3190479492985,65.0807684081278,12.));
#96304=CARTESIAN_POINT('Ctrl Pts',(-32.3003960632,65.0638401484245,12.));
#96305=CARTESIAN_POINT('Ctrl Pts',(-32.2817897504799,65.0469209207548,12.));
#96306=CARTESIAN_POINT('Ctrl Pts',(-32.2632290527855,65.0300108378786,12.));
#96307=CARTESIAN_POINT('Ctrl Pts',(-32.244714011842,65.0131100130155,12.));
#96308=CARTESIAN_POINT('Ctrl Pts',(-32.2262446694516,64.996218559847,12.));
#96309=CARTESIAN_POINT('Ctrl Pts',(-32.2078210674857,64.9793365925194,12.));
#96310=CARTESIAN_POINT('Ctrl Pts',(-32.1894432478889,64.9624642256477,12.));
#96311=CARTESIAN_POINT('Ctrl Pts',(-32.171111252686,64.9456015743203,12.));
#96312=CARTESIAN_POINT('Ctrl Pts',(-32.1528251239832,64.9287487541018,12.));
#96313=CARTESIAN_POINT('Ctrl Pts',(-32.1345849039671,64.9119058810362,12.));
#96314=CARTESIAN_POINT('Ctrl Pts',(-32.1163906348979,64.8950730716493,12.));
#96315=CARTESIAN_POINT('Ctrl Pts',(-32.0982423591108,64.878250442952,12.));
#96316=CARTESIAN_POINT('Ctrl Pts',(-32.0801401190241,64.861438112445,12.));
#96317=CARTESIAN_POINT('Ctrl Pts',(-32.0620839571408,64.8446361981234,12.));
#96318=CARTESIAN_POINT('Ctrl Pts',(-32.0440739160477,64.8278448184786,12.));
#96319=CARTESIAN_POINT('Ctrl Pts',(-32.0261100384092,64.8110640925021,12.));
#96320=CARTESIAN_POINT('Ctrl Pts',(-32.0081923669677,64.7942941396881,12.));
#96321=CARTESIAN_POINT('Ctrl Pts',(-31.990320944552,64.77753508004,12.));
#96322=CARTESIAN_POINT('Ctrl Pts',(-31.9724958140789,64.7607870340735,12.));
#96323=CARTESIAN_POINT('Ctrl Pts',(-31.9547170185534,64.7440501228202,12.));
#96324=CARTESIAN_POINT('Ctrl Pts',(-31.9369846010615,64.7273244678297,12.));
#96325=CARTESIAN_POINT('Ctrl Pts',(-31.9192986047706,64.7106101911732,12.));
#96326=CARTESIAN_POINT('Ctrl Pts',(-31.9016590729374,64.6939074154498,12.));
#96327=CARTESIAN_POINT('Ctrl Pts',(-31.8840660489107,64.6772162637907,12.));
#96328=CARTESIAN_POINT('Ctrl Pts',(-31.866519576131,64.6605368598629,12.));
#96329=CARTESIAN_POINT('Ctrl Pts',(-31.8490196981248,64.6438693278714,12.));
#96330=CARTESIAN_POINT('Ctrl Pts',(-31.8315664585026,64.6272137925627,12.));
#96331=CARTESIAN_POINT('Ctrl Pts',(-31.8141599009684,64.6105703792312,12.));
#96332=CARTESIAN_POINT('Ctrl Pts',(-31.7968000693218,64.5939392137235,12.));
#96333=CARTESIAN_POINT('Ctrl Pts',(-31.7794870074583,64.5773204224429,12.));
#96334=CARTESIAN_POINT('Ctrl Pts',(-31.7622207593634,64.5607141323521,12.));
#96335=CARTESIAN_POINT('Ctrl Pts',(-31.7450013691112,64.544120470977,12.));
#96336=CARTESIAN_POINT('Ctrl Pts',(-31.7278288808731,64.5275395664124,12.));
#96337=CARTESIAN_POINT('Ctrl Pts',(-31.7107033389201,64.510971547327,12.));
#96338=CARTESIAN_POINT('Ctrl Pts',(-31.6936247876229,64.4944165429675,12.));
#96339=CARTESIAN_POINT('Ctrl Pts',(-31.6765932714464,64.4778746831614,12.));
#96340=CARTESIAN_POINT('Ctrl Pts',(-31.6596088349482,64.4613460983214,12.));
#96341=CARTESIAN_POINT('Ctrl Pts',(-31.6426715227878,64.4448309194525,12.));
#96342=CARTESIAN_POINT('Ctrl Pts',(-31.6257813797287,64.4283292781565,12.));
#96343=CARTESIAN_POINT('Ctrl Pts',(-31.6089384506395,64.4118413066378,12.));
#96344=CARTESIAN_POINT('Ctrl Pts',(-31.5921427804865,64.3953671377046,12.));
#96345=CARTESIAN_POINT('Ctrl Pts',(-31.5753944143336,64.3789069047733,12.));
#96346=CARTESIAN_POINT('Ctrl Pts',(-31.5586933973515,64.3624607418768,12.));
#96347=CARTESIAN_POINT('Ctrl Pts',(-31.5420397748191,64.3460287836687,12.));
#96348=CARTESIAN_POINT('Ctrl Pts',(-31.5254335921245,64.3296111654283,12.));
#96349=CARTESIAN_POINT('Ctrl Pts',(-31.5088748947582,64.3132080230637,12.));
#96350=CARTESIAN_POINT('Ctrl Pts',(-31.4923637283132,64.2968194931158,12.));
#96351=CARTESIAN_POINT('Ctrl Pts',(-31.4759001384941,64.2804457127671,12.));
#96352=CARTESIAN_POINT('Ctrl Pts',(-31.4594841711195,64.2640868198473,12.));
#96353=CARTESIAN_POINT('Ctrl Pts',(-31.4431158721222,64.2477429528393,12.));
#96354=CARTESIAN_POINT('Ctrl Pts',(-31.4267952875423,64.231414250881,12.));
#96355=CARTESIAN_POINT('Ctrl Pts',(-31.410522463528,64.2151008537697,12.));
#96356=CARTESIAN_POINT('Ctrl Pts',(-31.3942974463445,64.1988029019707,12.));
#96357=CARTESIAN_POINT('Ctrl Pts',(-31.3781202823754,64.1825205366224,12.));
#96358=CARTESIAN_POINT('Ctrl Pts',(-31.3619910181228,64.166253899542,12.));
#96359=CARTESIAN_POINT('Ctrl Pts',(-31.3459097002006,64.1500031332282,12.));
#96360=CARTESIAN_POINT('Ctrl Pts',(-31.3298763753377,64.133768380869,12.));
#96361=CARTESIAN_POINT('Ctrl Pts',(-31.3138910903859,64.117549786349,12.));
#96362=CARTESIAN_POINT('Ctrl Pts',(-31.2979538923214,64.1013474942556,12.));
#96363=CARTESIAN_POINT('Ctrl Pts',(-31.2820648282447,64.0851616498852,12.));
#96364=CARTESIAN_POINT('Ctrl Pts',(-31.2662239453728,64.0689923992461,12.));
#96365=CARTESIAN_POINT('Ctrl Pts',(-31.2504312910451,64.0528398890657,12.));
#96366=CARTESIAN_POINT('Ctrl Pts',(-31.2346869127297,64.0367042667984,12.));
#96367=CARTESIAN_POINT('Ctrl Pts',(-31.2189908580245,64.02058568063,12.));
#96368=CARTESIAN_POINT('Ctrl Pts',(-31.2033431746558,64.0044842794831,12.));
#96369=CARTESIAN_POINT('Ctrl Pts',(-31.1877439104717,63.9884002130211,12.));
#96370=CARTESIAN_POINT('Ctrl Pts',(-31.1721931134487,63.9723336316551,12.));
#96371=CARTESIAN_POINT('Ctrl Pts',(-31.1566908316992,63.9562846865567,12.));
#96372=CARTESIAN_POINT('Ctrl Pts',(-31.1412371134727,63.940253529665,12.));
#96373=CARTESIAN_POINT('Ctrl Pts',(-31.1258320071545,63.9242403136955,12.));
#96374=CARTESIAN_POINT('Ctrl Pts',(-31.1104755612607,63.9082451921448,12.));
#96375=CARTESIAN_POINT('Ctrl Pts',(-31.0951678244455,63.8922683192964,12.));
#96376=CARTESIAN_POINT('Ctrl Pts',(-31.0799088455041,63.8763098502237,12.));
#96377=CARTESIAN_POINT('Ctrl Pts',(-31.0646986733723,63.8603699407922,12.));
#96378=CARTESIAN_POINT('Ctrl Pts',(-31.0495373571215,63.8444487476611,12.));
#96379=CARTESIAN_POINT('Ctrl Pts',(-31.0344249459538,63.8285464282846,12.));
#96380=CARTESIAN_POINT('Ctrl Pts',(-31.0193614892171,63.8126631409364,12.));
#96381=CARTESIAN_POINT('Ctrl Pts',(-31.0043470364108,63.796799044728,12.));
#96382=CARTESIAN_POINT('Ctrl Pts',(-30.989381637191,63.7809542996264,12.));
#96383=CARTESIAN_POINT('Ctrl Pts',(-30.9744653413689,63.7651290664733,12.));
#96384=CARTESIAN_POINT('Ctrl Pts',(-30.9595981989104,63.749323506987,12.));
#96385=CARTESIAN_POINT('Ctrl Pts',(-30.9447802599355,63.7335377837441,12.));
#96386=CARTESIAN_POINT('Ctrl Pts',(-30.9300115747115,63.7177720601609,12.));
#96387=CARTESIAN_POINT('Ctrl Pts',(-30.9152921936465,63.7020265004792,12.));
#96388=CARTESIAN_POINT('Ctrl Pts',(-30.900622167269,63.6863012697328,12.));
#96389=CARTESIAN_POINT('Ctrl Pts',(-30.8860015462475,63.6705965337971,12.));
#96390=CARTESIAN_POINT('Ctrl Pts',(-30.8714303814194,63.6549124594666,12.));
#96391=CARTESIAN_POINT('Ctrl Pts',(-30.8569087238131,63.6392492145233,12.));
#96392=CARTESIAN_POINT('Ctrl Pts',(-30.8424366246671,63.6236069678055,12.));
#96393=CARTESIAN_POINT('Ctrl Pts',(-30.8280141354459,63.6079858892771,12.));
#96394=CARTESIAN_POINT('Ctrl Pts',(-30.813641307801,63.5923861498987,12.));
#96395=CARTESIAN_POINT('Ctrl Pts',(-30.7993181935271,63.5768079214881,12.));
#96396=CARTESIAN_POINT('Ctrl Pts',(-30.7850448445205,63.5612513766,12.));
#96397=CARTESIAN_POINT('Ctrl Pts',(-30.7708213127159,63.5457166883537,12.));
#96398=CARTESIAN_POINT('Ctrl Pts',(-30.7566476500757,63.5302040304142,12.));
#96399=CARTESIAN_POINT('Ctrl Pts',(-30.7425239087281,63.5147135773894,12.));
#96400=CARTESIAN_POINT('Ctrl Pts',(-30.7284501410822,63.4992455051795,12.));
#96401=CARTESIAN_POINT('Ctrl Pts',(-30.7144263999265,63.4837999912771,12.));
#96402=CARTESIAN_POINT('Ctrl Pts',(-30.7004527385821,63.4683772152529,12.));
#96403=CARTESIAN_POINT('Ctrl Pts',(-30.6865292107929,63.4529773584249,12.));
#96404=CARTESIAN_POINT('Ctrl Pts',(-30.6726558704315,63.4376006029604,12.));
#96405=CARTESIAN_POINT('Ctrl Pts',(-30.6588327712484,63.4222471311239,12.));
#96406=CARTESIAN_POINT('Ctrl Pts',(-30.6450599666121,63.4069171245066,12.));
#96407=CARTESIAN_POINT('Ctrl Pts',(-30.6313375092062,63.3916107631376,12.));
#96408=CARTESIAN_POINT('Ctrl Pts',(-30.6176654515967,63.3763282271796,12.));
#96409=CARTESIAN_POINT('Ctrl Pts',(-30.6040438469078,63.3610696989577,12.));
#96410=CARTESIAN_POINT('Ctrl Pts',(-30.5904727493712,63.3458353646154,12.));
#96411=CARTESIAN_POINT('Ctrl Pts',(-30.5769522151164,63.3306254165126,12.));
#96412=CARTESIAN_POINT('Ctrl Pts',(-30.563482302238,63.3154400534397,12.));
#96413=CARTESIAN_POINT('Ctrl Pts',(-30.5500630691359,63.3002794756086,12.));
#96414=CARTESIAN_POINT('Ctrl Pts',(-30.5366945730508,63.2851438802473,12.));
#96415=CARTESIAN_POINT('Ctrl Pts',(-30.5233768687865,63.2700334577639,12.));
#96416=CARTESIAN_POINT('Ctrl Pts',(-30.5101100066659,63.2549483856215,12.));
#96417=CARTESIAN_POINT('Ctrl Pts',(-30.4968940344998,63.2398888342545,12.));
#96418=CARTESIAN_POINT('Ctrl Pts',(-30.4837290014989,63.2248549788221,12.));
#96419=CARTESIAN_POINT('Ctrl Pts',(-30.470614961416,63.2098470086636,12.));
#96420=CARTESIAN_POINT('Ctrl Pts',(-30.4575519763337,63.1948651386942,12.));
#96421=CARTESIAN_POINT('Ctrl Pts',(-30.4445401192381,63.179909617189,12.));
#96422=CARTESIAN_POINT('Ctrl Pts',(-30.4315794659731,63.164980701691,12.));
#96423=CARTESIAN_POINT('Ctrl Pts',(-30.418670087563,63.1500786361459,12.));
#96424=CARTESIAN_POINT('Ctrl Pts',(-30.4058120432228,63.135203629844,12.));
#96425=CARTESIAN_POINT('Ctrl Pts',(-30.3930053710484,63.1203558300657,12.));
#96426=CARTESIAN_POINT('Ctrl Pts',(-30.3802500880403,63.105535320226,12.));
#96427=CARTESIAN_POINT('Ctrl Pts',(-30.3700869762507,63.0937007763471,12.));
#96428=CARTESIAN_POINT('Ctrl Pts',(-30.3624877680651,63.0848371718048,12.));
#96429=CARTESIAN_POINT('Ctrl Pts',(-30.357431906933,63.078933570069,12.));
#96430=CARTESIAN_POINT('Ctrl Pts',(-30.3549065457811,63.0759831361898,12.));
#96431=CARTESIAN_POINT('Ctrl Pts',(-34.933187552314,65.4667541478384,-5.55111512312578E-16));
#96432=CARTESIAN_POINT('Ctrl Pts',(-34.933187552314,65.4667541478384,4.));
#96433=CARTESIAN_POINT('Ctrl Pts',(-34.933187552314,65.4667541478384,8.));
#96434=CARTESIAN_POINT('Ctrl Pts',(-34.933187552314,65.4667541478384,12.));
#96435=CARTESIAN_POINT('Ctrl Pts',(-34.940541458921,65.5763902570748,-5.55111512312578E-16));
#96436=CARTESIAN_POINT('Ctrl Pts',(-34.940541458921,65.5763902570748,4.));
#96437=CARTESIAN_POINT('Ctrl Pts',(-34.940541458921,65.5763902570748,8.));
#96438=CARTESIAN_POINT('Ctrl Pts',(-34.940541458921,65.5763902570748,12.));
#96439=CARTESIAN_POINT('Ctrl Pts',(-34.8876896346299,65.7720412680587,-5.55111512312578E-16));
#96440=CARTESIAN_POINT('Ctrl Pts',(-34.8876896346299,65.7720412680587,4.00000000000001));
#96441=CARTESIAN_POINT('Ctrl Pts',(-34.8876896346299,65.7720412680587,7.99999999999999));
#96442=CARTESIAN_POINT('Ctrl Pts',(-34.8876896346299,65.7720412680587,12.));
#96443=CARTESIAN_POINT('Ctrl Pts',(-34.7399186668304,65.9044372006541,-5.55111512312578E-16));
#96444=CARTESIAN_POINT('Ctrl Pts',(-34.7399186668304,65.9044372006541,4.));
#96445=CARTESIAN_POINT('Ctrl Pts',(-34.7399186668304,65.9044372006541,8.00000000000001));
#96446=CARTESIAN_POINT('Ctrl Pts',(-34.7399186668304,65.9044372006541,12.));
#96447=CARTESIAN_POINT('Ctrl Pts',(-34.6669728017261,65.9427857825583,-5.55111512312578E-16));
#96448=CARTESIAN_POINT('Ctrl Pts',(-34.6669728017261,65.9427857825583,4.));
#96449=CARTESIAN_POINT('Ctrl Pts',(-34.6669728017261,65.9427857825583,8.));
#96450=CARTESIAN_POINT('Ctrl Pts',(-34.6669728017261,65.9427857825583,12.));
#96451=CARTESIAN_POINT('',(-34.933187552314,65.4667541478384,0.));
#96452=CARTESIAN_POINT('',(-34.6669728017262,65.9427857825584,2.77555756156289E-16));
#96453=CARTESIAN_POINT('Ctrl Pts',(-34.933187552314,65.4667541478384,4.16333634234434E-16));
#96454=CARTESIAN_POINT('Ctrl Pts',(-34.940541458921,65.5763902570748,4.16333634234433E-16));
#96455=CARTESIAN_POINT('Ctrl Pts',(-34.910340416469,65.6881908347799,4.16333634234434E-16));
#96456=CARTESIAN_POINT('Ctrl Pts',(-34.8491453679733,65.7793366930112,4.16333634234434E-16));
#96457=CARTESIAN_POINT('Ctrl Pts',(-34.8032490816016,65.8476960866847,4.16333634234434E-16));
#96458=CARTESIAN_POINT('Ctrl Pts',(-34.7399186668304,65.9044372006541,4.16333634234433E-16));
#96459=CARTESIAN_POINT('Ctrl Pts',(-34.6669728017261,65.9427857825583,4.16333634234434E-16));
#96460=CARTESIAN_POINT('',(-34.6669728017262,65.9427857825584,12.));
#96461=CARTESIAN_POINT('Ctrl Pts',(-34.6669728017261,65.9427857825583,-5.55111512312578E-16));
#96462=CARTESIAN_POINT('Ctrl Pts',(-34.6669728017261,65.9427857825583,4.));
#96463=CARTESIAN_POINT('Ctrl Pts',(-34.6669728017261,65.9427857825583,8.));
#96464=CARTESIAN_POINT('Ctrl Pts',(-34.6669728017261,65.9427857825583,12.));
#96465=CARTESIAN_POINT('',(-34.933187552314,65.4667541478384,12.));
#96466=CARTESIAN_POINT('Ctrl Pts',(-34.6669728017261,65.9427857825583,12.));
#96467=CARTESIAN_POINT('Ctrl Pts',(-34.7399186668304,65.9044372006541,12.));
#96468=CARTESIAN_POINT('Ctrl Pts',(-34.8032490816016,65.8476960866846,12.));
#96469=CARTESIAN_POINT('Ctrl Pts',(-34.8491453679733,65.7793366930112,12.));
#96470=CARTESIAN_POINT('Ctrl Pts',(-34.910340416469,65.6881908347799,12.));
#96471=CARTESIAN_POINT('Ctrl Pts',(-34.940541458921,65.5763902570748,12.));
#96472=CARTESIAN_POINT('Ctrl Pts',(-34.933187552314,65.4667541478384,12.));
#96473=CARTESIAN_POINT('Ctrl Pts',(-34.933187552314,65.4667541478384,12.));
#96474=CARTESIAN_POINT('Ctrl Pts',(-34.933187552314,65.4667541478384,8.));
#96475=CARTESIAN_POINT('Ctrl Pts',(-34.933187552314,65.4667541478384,4.));
#96476=CARTESIAN_POINT('Ctrl Pts',(-34.933187552314,65.4667541478384,-5.55111512312578E-16));
#96477=CARTESIAN_POINT('Origin',(-1.73171632017259E-10,3.32444647725448E-10,
0.));
#96478=CARTESIAN_POINT('Origin',(-1.73171632017259E-10,3.32444647725448E-10,
12.));
#96479=CARTESIAN_POINT('Origin',(-1.73171632017259E-10,3.32444647725448E-10,
0.));
#96480=CARTESIAN_POINT('Ctrl Pts',(-28.2316040302268,68.9436475237602,-5.55111512312578E-16));
#96481=CARTESIAN_POINT('Ctrl Pts',(-28.2316040302268,68.9436475237602,4.));
#96482=CARTESIAN_POINT('Ctrl Pts',(-28.2316040302269,68.9436475237602,8.));
#96483=CARTESIAN_POINT('Ctrl Pts',(-28.2316040302269,68.9436475237602,12.));
#96484=CARTESIAN_POINT('Ctrl Pts',(-28.1299168084378,68.9852872321828,-5.55111512312578E-16));
#96485=CARTESIAN_POINT('Ctrl Pts',(-28.1299168084378,68.9852872321828,4.));
#96486=CARTESIAN_POINT('Ctrl Pts',(-28.1299168084378,68.9852872321828,8.00000000000001));
#96487=CARTESIAN_POINT('Ctrl Pts',(-28.1299168084378,68.9852872321828,12.));
#96488=CARTESIAN_POINT('Ctrl Pts',(-27.9275918177432,68.9970049015576,-5.55111512312578E-16));
#96489=CARTESIAN_POINT('Ctrl Pts',(-27.9275918177432,68.9970049015576,4.));
#96490=CARTESIAN_POINT('Ctrl Pts',(-27.9275918177433,68.9970049015576,7.99999999999999));
#96491=CARTESIAN_POINT('Ctrl Pts',(-27.9275918177433,68.9970049015576,12.));
#96492=CARTESIAN_POINT('Ctrl Pts',(-27.7552674476222,68.8986722313991,-5.55111512312578E-16));
#96493=CARTESIAN_POINT('Ctrl Pts',(-27.7552674476222,68.8986722313991,4.));
#96494=CARTESIAN_POINT('Ctrl Pts',(-27.7552674476223,68.8986722313991,8.00000000000001));
#96495=CARTESIAN_POINT('Ctrl Pts',(-27.7552674476223,68.8986722313991,12.));
#96496=CARTESIAN_POINT('Ctrl Pts',(-27.6958230984758,68.8415926174774,-5.55111512312578E-16));
#96497=CARTESIAN_POINT('Ctrl Pts',(-27.6958230984758,68.8415926174774,4.));
#96498=CARTESIAN_POINT('Ctrl Pts',(-27.6958230984758,68.8415926174774,8.));
#96499=CARTESIAN_POINT('Ctrl Pts',(-27.6958230984758,68.8415926174774,12.));
#96500=CARTESIAN_POINT('',(-28.2316040302268,68.9436475237602,0.));
#96501=CARTESIAN_POINT('',(-27.6958230984757,68.8415926174774,2.77555756156289E-16));
#96502=CARTESIAN_POINT('Ctrl Pts',(-28.2316040302268,68.9436475237602,-5.55111512312578E-16));
#96503=CARTESIAN_POINT('Ctrl Pts',(-28.1299168084378,68.9852872321828,-5.55111512312578E-16));
#96504=CARTESIAN_POINT('Ctrl Pts',(-28.0143025280409,68.9919830432541,-5.55111512312578E-16));
#96505=CARTESIAN_POINT('Ctrl Pts',(-27.9084843686476,68.9627440495799,-5.55111512312578E-16));
#96506=CARTESIAN_POINT('Ctrl Pts',(-27.8291207491026,68.9408148043242,-5.55111512312578E-16));
#96507=CARTESIAN_POINT('Ctrl Pts',(-27.7552674476222,68.8986722313991,-5.55111512312578E-16));
#96508=CARTESIAN_POINT('Ctrl Pts',(-27.6958230984758,68.8415926174774,-5.55111512312578E-16));
#96509=CARTESIAN_POINT('',(-27.6958230984758,68.8415926174774,12.));
#96510=CARTESIAN_POINT('Ctrl Pts',(-27.6958230984758,68.8415926174774,-5.55111512312578E-16));
#96511=CARTESIAN_POINT('Ctrl Pts',(-27.6958230984758,68.8415926174774,4.));
#96512=CARTESIAN_POINT('Ctrl Pts',(-27.6958230984758,68.8415926174774,8.));
#96513=CARTESIAN_POINT('Ctrl Pts',(-27.6958230984758,68.8415926174774,12.));
#96514=CARTESIAN_POINT('',(-28.2316040302269,68.9436475237602,12.));
#96515=CARTESIAN_POINT('Ctrl Pts',(-27.6958230984758,68.8415926174774,12.));
#96516=CARTESIAN_POINT('Ctrl Pts',(-27.7552674476223,68.8986722313991,12.));
#96517=CARTESIAN_POINT('Ctrl Pts',(-27.8291207491027,68.9408148043242,12.));
#96518=CARTESIAN_POINT('Ctrl Pts',(-27.9084843686477,68.9627440495799,12.));
#96519=CARTESIAN_POINT('Ctrl Pts',(-28.0143025280409,68.9919830432541,12.));
#96520=CARTESIAN_POINT('Ctrl Pts',(-28.1299168084378,68.9852872321828,12.));
#96521=CARTESIAN_POINT('Ctrl Pts',(-28.2316040302269,68.9436475237602,12.));
#96522=CARTESIAN_POINT('Ctrl Pts',(-28.2316040302269,68.9436475237602,12.));
#96523=CARTESIAN_POINT('Ctrl Pts',(-28.2316040302269,68.9436475237602,8.));
#96524=CARTESIAN_POINT('Ctrl Pts',(-28.2316040302268,68.9436475237602,4.));
#96525=CARTESIAN_POINT('Ctrl Pts',(-28.2316040302268,68.9436475237602,-5.55111512312578E-16));
#96526=CARTESIAN_POINT('Ctrl Pts',(-24.7419628022042,65.4815644032299,0.));
#96527=CARTESIAN_POINT('Ctrl Pts',(-24.7419628022042,65.4815644032299,12.));
#96528=CARTESIAN_POINT('Ctrl Pts',(-24.7442214063382,65.4847237095443,0.));
#96529=CARTESIAN_POINT('Ctrl Pts',(-24.7442214063382,65.4847237095443,12.));
#96530=CARTESIAN_POINT('Ctrl Pts',(-24.7487434955982,65.4910454936254,0.));
#96531=CARTESIAN_POINT('Ctrl Pts',(-24.7487434955982,65.4910454936254,12.));
#96532=CARTESIAN_POINT('Ctrl Pts',(-24.7555412724651,65.5005376841101,0.));
#96533=CARTESIAN_POINT('Ctrl Pts',(-24.7555412724651,65.5005376841101,12.));
#96534=CARTESIAN_POINT('Ctrl Pts',(-24.7646342620841,65.5132129675333,0.));
#96535=CARTESIAN_POINT('Ctrl Pts',(-24.7646342620841,65.5132129675333,12.));
#96536=CARTESIAN_POINT('Ctrl Pts',(-24.7760493148465,65.5290887770232,0.));
#96537=CARTESIAN_POINT('Ctrl Pts',(-24.7760493148465,65.5290887770232,12.));
#96538=CARTESIAN_POINT('Ctrl Pts',(-24.7875131827491,65.5449962514661,0.));
#96539=CARTESIAN_POINT('Ctrl Pts',(-24.7875131827491,65.5449962514661,12.));
#96540=CARTESIAN_POINT('Ctrl Pts',(-24.799025856126,65.5609353062829,0.));
#96541=CARTESIAN_POINT('Ctrl Pts',(-24.799025856126,65.5609353062829,12.));
#96542=CARTESIAN_POINT('Ctrl Pts',(-24.8105873098626,65.5769057914333,0.));
#96543=CARTESIAN_POINT('Ctrl Pts',(-24.8105873098626,65.5769057914333,12.));
#96544=CARTESIAN_POINT('Ctrl Pts',(-24.8221975032104,65.5929074932624,0.));
#96545=CARTESIAN_POINT('Ctrl Pts',(-24.8221975032104,65.5929074932624,12.));
#96546=CARTESIAN_POINT('Ctrl Pts',(-24.8338563866764,65.6089401625628,0.));
#96547=CARTESIAN_POINT('Ctrl Pts',(-24.8338563866764,65.6089401625628,12.));
#96548=CARTESIAN_POINT('Ctrl Pts',(-24.8455639071517,65.6250035361612,0.));
#96549=CARTESIAN_POINT('Ctrl Pts',(-24.8455639071517,65.6250035361612,12.));
#96550=CARTESIAN_POINT('Ctrl Pts',(-24.8573200135666,65.6410973603661,0.));
#96551=CARTESIAN_POINT('Ctrl Pts',(-24.8573200135666,65.6410973603661,12.));
#96552=CARTESIAN_POINT('Ctrl Pts',(-24.8691246628057,65.6572214156692,0.));
#96553=CARTESIAN_POINT('Ctrl Pts',(-24.8691246628057,65.6572214156692,12.));
#96554=CARTESIAN_POINT('Ctrl Pts',(-24.8809778178229,65.6733755087669,0.));
#96555=CARTESIAN_POINT('Ctrl Pts',(-24.8809778178229,65.6733755087669,12.));
#96556=CARTESIAN_POINT('Ctrl Pts',(-24.8928794448607,65.6895594608775,0.));
#96557=CARTESIAN_POINT('Ctrl Pts',(-24.8928794448607,65.6895594608775,12.));
#96558=CARTESIAN_POINT('Ctrl Pts',(-24.9048295111448,65.7057730980483,0.));
#96559=CARTESIAN_POINT('Ctrl Pts',(-24.9048295111448,65.7057730980483,12.));
#96560=CARTESIAN_POINT('Ctrl Pts',(-24.9168279820106,65.7220162391053,0.));
#96561=CARTESIAN_POINT('Ctrl Pts',(-24.9168279820106,65.7220162391053,12.));
#96562=CARTESIAN_POINT('Ctrl Pts',(-24.928874819458,65.7382886895888,0.));
#96563=CARTESIAN_POINT('Ctrl Pts',(-24.928874819458,65.7382886895888,12.));
#96564=CARTESIAN_POINT('Ctrl Pts',(-24.9409699836537,65.7545902480323,0.));
#96565=CARTESIAN_POINT('Ctrl Pts',(-24.9409699836537,65.7545902480323,12.));
#96566=CARTESIAN_POINT('Ctrl Pts',(-24.9531134338696,65.7709207098959,0.));
#96567=CARTESIAN_POINT('Ctrl Pts',(-24.9531134338696,65.7709207098959,12.));
#96568=CARTESIAN_POINT('Ctrl Pts',(-24.9653051295581,65.7872798720823,0.));
#96569=CARTESIAN_POINT('Ctrl Pts',(-24.9653051295581,65.7872798720823,12.));
#96570=CARTESIAN_POINT('Ctrl Pts',(-24.9775450315683,65.8036675380718,0.));
#96571=CARTESIAN_POINT('Ctrl Pts',(-24.9775450315683,65.8036675380718,12.));
#96572=CARTESIAN_POINT('Ctrl Pts',(-24.9898331020983,65.8200835177024,0.));
#96573=CARTESIAN_POINT('Ctrl Pts',(-24.9898331020983,65.8200835177024,12.));
#96574=CARTESIAN_POINT('Ctrl Pts',(-25.002169304117,65.8365276247128,0.));
#96575=CARTESIAN_POINT('Ctrl Pts',(-25.002169304117,65.8365276247128,12.));
#96576=CARTESIAN_POINT('Ctrl Pts',(-25.0145536009604,65.8529996750445,0.));
#96577=CARTESIAN_POINT('Ctrl Pts',(-25.0145536009604,65.8529996750445,12.));
#96578=CARTESIAN_POINT('Ctrl Pts',(-25.0269859558363,65.8694994847616,0.));
#96579=CARTESIAN_POINT('Ctrl Pts',(-25.0269859558363,65.8694994847616,12.));
#96580=CARTESIAN_POINT('Ctrl Pts',(-25.0394663314055,65.8860268683128,0.));
#96581=CARTESIAN_POINT('Ctrl Pts',(-25.0394663314055,65.8860268683128,12.));
#96582=CARTESIAN_POINT('Ctrl Pts',(-25.0519946900078,65.9025816394424,0.));
#96583=CARTESIAN_POINT('Ctrl Pts',(-25.0519946900078,65.9025816394424,12.));
#96584=CARTESIAN_POINT('Ctrl Pts',(-25.0645709938524,65.919163611981,0.));
#96585=CARTESIAN_POINT('Ctrl Pts',(-25.0645709938524,65.919163611981,12.));
#96586=CARTESIAN_POINT('Ctrl Pts',(-25.0771952052028,65.9357726006163,0.));
#96587=CARTESIAN_POINT('Ctrl Pts',(-25.0771952052028,65.9357726006163,12.));
#96588=CARTESIAN_POINT('Ctrl Pts',(-25.0898672865915,65.9524084218139,0.));
#96589=CARTESIAN_POINT('Ctrl Pts',(-25.0898672865915,65.9524084218139,12.));
#96590=CARTESIAN_POINT('Ctrl Pts',(-25.1025872009004,65.9690708941558,0.));
#96591=CARTESIAN_POINT('Ctrl Pts',(-25.1025872009004,65.9690708941558,12.));
#96592=CARTESIAN_POINT('Ctrl Pts',(-25.1153549112503,65.9857598378433,0.));
#96593=CARTESIAN_POINT('Ctrl Pts',(-25.1153549112503,65.9857598378433,12.));
#96594=CARTESIAN_POINT('Ctrl Pts',(-25.1281703809297,66.0024750743897,0.));
#96595=CARTESIAN_POINT('Ctrl Pts',(-25.1281703809297,66.0024750743897,12.));
#96596=CARTESIAN_POINT('Ctrl Pts',(-25.1410335733099,66.0192164262621,0.));
#96597=CARTESIAN_POINT('Ctrl Pts',(-25.1410335733099,66.0192164262621,12.));
#96598=CARTESIAN_POINT('Ctrl Pts',(-25.1539444517419,66.0359837164734,0.));
#96599=CARTESIAN_POINT('Ctrl Pts',(-25.1539444517419,66.0359837164734,12.));
#96600=CARTESIAN_POINT('Ctrl Pts',(-25.1669029795661,66.0527767686025,0.));
#96601=CARTESIAN_POINT('Ctrl Pts',(-25.1669029795661,66.0527767686025,12.));
#96602=CARTESIAN_POINT('Ctrl Pts',(-25.1799091201599,66.0695954069713,0.));
#96603=CARTESIAN_POINT('Ctrl Pts',(-25.1799091201599,66.0695954069713,12.));
#96604=CARTESIAN_POINT('Ctrl Pts',(-25.1929628369685,66.086439456768,0.));
#96605=CARTESIAN_POINT('Ctrl Pts',(-25.1929628369685,66.086439456768,12.));
#96606=CARTESIAN_POINT('Ctrl Pts',(-25.2060640935365,66.10330874419,0.));
#96607=CARTESIAN_POINT('Ctrl Pts',(-25.2060640935365,66.10330874419,12.));
#96608=CARTESIAN_POINT('Ctrl Pts',(-25.2192128535357,66.1202030965758,0.));
#96609=CARTESIAN_POINT('Ctrl Pts',(-25.2192128535357,66.1202030965758,12.));
#96610=CARTESIAN_POINT('Ctrl Pts',(-25.232409080755,66.1371223423345,0.));
#96611=CARTESIAN_POINT('Ctrl Pts',(-25.232409080755,66.1371223423345,12.));
#96612=CARTESIAN_POINT('Ctrl Pts',(-25.2456527390875,66.1540663108754,0.));
#96613=CARTESIAN_POINT('Ctrl Pts',(-25.2456527390875,66.1540663108754,12.));
#96614=CARTESIAN_POINT('Ctrl Pts',(-25.2589437925147,66.1710348325384,0.));
#96615=CARTESIAN_POINT('Ctrl Pts',(-25.2589437925147,66.1710348325384,12.));
#96616=CARTESIAN_POINT('Ctrl Pts',(-25.2722822050837,66.1880277385136,0.));
#96617=CARTESIAN_POINT('Ctrl Pts',(-25.2722822050837,66.1880277385136,12.));
#96618=CARTESIAN_POINT('Ctrl Pts',(-25.285667940893,66.2050448607911,0.));
#96619=CARTESIAN_POINT('Ctrl Pts',(-25.285667940893,66.2050448607911,12.));
#96620=CARTESIAN_POINT('Ctrl Pts',(-25.2991009641094,66.2220860321952,0.));
#96621=CARTESIAN_POINT('Ctrl Pts',(-25.2991009641094,66.2220860321952,12.));
#96622=CARTESIAN_POINT('Ctrl Pts',(-25.312581238973,66.2391510863998,0.));
#96623=CARTESIAN_POINT('Ctrl Pts',(-25.312581238973,66.2391510863998,12.));
#96624=CARTESIAN_POINT('Ctrl Pts',(-25.3261087298026,66.2562398579471,0.));
#96625=CARTESIAN_POINT('Ctrl Pts',(-25.3261087298026,66.2562398579471,12.));
#96626=CARTESIAN_POINT('Ctrl Pts',(-25.3396834009949,66.2733521822662,0.));
#96627=CARTESIAN_POINT('Ctrl Pts',(-25.3396834009949,66.2733521822662,12.));
#96628=CARTESIAN_POINT('Ctrl Pts',(-25.3533052170249,66.290487895671,0.));
#96629=CARTESIAN_POINT('Ctrl Pts',(-25.3533052170249,66.290487895671,12.));
#96630=CARTESIAN_POINT('Ctrl Pts',(-25.3669741424488,66.3076468353412,0.));
#96631=CARTESIAN_POINT('Ctrl Pts',(-25.3669741424488,66.3076468353412,12.));
#96632=CARTESIAN_POINT('Ctrl Pts',(-25.3806901419012,66.3248288393046,0.));
#96633=CARTESIAN_POINT('Ctrl Pts',(-25.3806901419012,66.3248288393046,12.));
#96634=CARTESIAN_POINT('Ctrl Pts',(-25.3944531800901,66.3420337464178,0.));
#96635=CARTESIAN_POINT('Ctrl Pts',(-25.3944531800901,66.3420337464178,12.));
#96636=CARTESIAN_POINT('Ctrl Pts',(-25.4082632217847,66.359261396341,0.));
#96637=CARTESIAN_POINT('Ctrl Pts',(-25.4082632217847,66.359261396341,12.));
#96638=CARTESIAN_POINT('Ctrl Pts',(-25.4221202318199,66.3765116295364,0.));
#96639=CARTESIAN_POINT('Ctrl Pts',(-25.4221202318199,66.3765116295364,12.));
#96640=CARTESIAN_POINT('Ctrl Pts',(-25.4360241751018,66.3937842872685,0.));
#96641=CARTESIAN_POINT('Ctrl Pts',(-25.4360241751018,66.3937842872685,12.));
#96642=CARTESIAN_POINT('Ctrl Pts',(-25.4499750166079,66.4110792116,0.));
#96643=CARTESIAN_POINT('Ctrl Pts',(-25.4499750166079,66.4110792116,12.));
#96644=CARTESIAN_POINT('Ctrl Pts',(-25.4639727213849,66.4283962453899,0.));
#96645=CARTESIAN_POINT('Ctrl Pts',(-25.4639727213849,66.4283962453899,12.));
#96646=CARTESIAN_POINT('Ctrl Pts',(-25.4780172545417,66.4457352322871,0.));
#96647=CARTESIAN_POINT('Ctrl Pts',(-25.4780172545417,66.4457352322871,12.));
#96648=CARTESIAN_POINT('Ctrl Pts',(-25.4921085812548,66.4630960167252,0.));
#96649=CARTESIAN_POINT('Ctrl Pts',(-25.4921085812548,66.4630960167252,12.));
#96650=CARTESIAN_POINT('Ctrl Pts',(-25.5062466667702,66.4804784439148,0.));
#96651=CARTESIAN_POINT('Ctrl Pts',(-25.5062466667702,66.4804784439148,12.));
#96652=CARTESIAN_POINT('Ctrl Pts',(-25.5204314764033,66.4978823598354,0.));
#96653=CARTESIAN_POINT('Ctrl Pts',(-25.5204314764033,66.4978823598354,12.));
#96654=CARTESIAN_POINT('Ctrl Pts',(-25.534662975532,66.5153076112231,0.));
#96655=CARTESIAN_POINT('Ctrl Pts',(-25.534662975532,66.5153076112231,12.));
#96656=CARTESIAN_POINT('Ctrl Pts',(-25.5489411295912,66.5327540455624,0.));
#96657=CARTESIAN_POINT('Ctrl Pts',(-25.5489411295912,66.5327540455624,12.));
#96658=CARTESIAN_POINT('Ctrl Pts',(-25.5632659040792,66.5502215110829,0.));
#96659=CARTESIAN_POINT('Ctrl Pts',(-25.5632659040792,66.5502215110829,12.));
#96660=CARTESIAN_POINT('Ctrl Pts',(-25.5776372645601,66.5677098567542,0.));
#96661=CARTESIAN_POINT('Ctrl Pts',(-25.5776372645601,66.5677098567542,12.));
#96662=CARTESIAN_POINT('Ctrl Pts',(-25.5920551766629,66.5852189322813,0.));
#96663=CARTESIAN_POINT('Ctrl Pts',(-25.5920551766629,66.5852189322813,12.));
#96664=CARTESIAN_POINT('Ctrl Pts',(-25.6065196060756,66.6027485880963,0.));
#96665=CARTESIAN_POINT('Ctrl Pts',(-25.6065196060756,66.6027485880963,12.));
#96666=CARTESIAN_POINT('Ctrl Pts',(-25.6210305185403,66.6202986753506,0.));
#96667=CARTESIAN_POINT('Ctrl Pts',(-25.6210305185403,66.6202986753506,12.));
#96668=CARTESIAN_POINT('Ctrl Pts',(-25.6355878798614,66.6378690459129,0.));
#96669=CARTESIAN_POINT('Ctrl Pts',(-25.6355878798614,66.6378690459129,12.));
#96670=CARTESIAN_POINT('Ctrl Pts',(-25.6501916559055,66.6554595523624,0.));
#96671=CARTESIAN_POINT('Ctrl Pts',(-25.6501916559055,66.6554595523624,12.));
#96672=CARTESIAN_POINT('Ctrl Pts',(-25.6648418126013,66.6730700479837,0.));
#96673=CARTESIAN_POINT('Ctrl Pts',(-25.6648418126013,66.6730700479837,12.));
#96674=CARTESIAN_POINT('Ctrl Pts',(-25.6795383159319,66.6907003867572,0.));
#96675=CARTESIAN_POINT('Ctrl Pts',(-25.6795383159319,66.6907003867572,12.));
#96676=CARTESIAN_POINT('Ctrl Pts',(-25.6942811319322,66.7083504233529,0.));
#96677=CARTESIAN_POINT('Ctrl Pts',(-25.6942811319322,66.7083504233529,12.));
#96678=CARTESIAN_POINT('Ctrl Pts',(-25.7090702266963,66.7260200131266,0.));
#96679=CARTESIAN_POINT('Ctrl Pts',(-25.7090702266963,66.7260200131266,12.));
#96680=CARTESIAN_POINT('Ctrl Pts',(-25.7239055663772,66.7437090121153,0.));
#96681=CARTESIAN_POINT('Ctrl Pts',(-25.7239055663772,66.7437090121153,12.));
#96682=CARTESIAN_POINT('Ctrl Pts',(-25.7387871171866,66.7614172770316,0.));
#96683=CARTESIAN_POINT('Ctrl Pts',(-25.7387871171866,66.7614172770316,12.));
#96684=CARTESIAN_POINT('Ctrl Pts',(-25.7537148453864,66.7791446652545,0.));
#96685=CARTESIAN_POINT('Ctrl Pts',(-25.7537148453864,66.7791446652545,12.));
#96686=CARTESIAN_POINT('Ctrl Pts',(-25.7686887172878,66.7968910348245,0.));
#96687=CARTESIAN_POINT('Ctrl Pts',(-25.7686887172878,66.7968910348245,12.));
#96688=CARTESIAN_POINT('Ctrl Pts',(-25.7837086992595,66.8146562444433,0.));
#96689=CARTESIAN_POINT('Ctrl Pts',(-25.7837086992595,66.8146562444433,12.));
#96690=CARTESIAN_POINT('Ctrl Pts',(-25.7987747577269,66.8324401534668,0.));
#96691=CARTESIAN_POINT('Ctrl Pts',(-25.7987747577269,66.8324401534668,12.));
#96692=CARTESIAN_POINT('Ctrl Pts',(-25.8138868591709,66.8502426219001,0.));
#96693=CARTESIAN_POINT('Ctrl Pts',(-25.8138868591709,66.8502426219001,12.));
#96694=CARTESIAN_POINT('Ctrl Pts',(-25.8290449701193,66.8680635103876,0.));
#96695=CARTESIAN_POINT('Ctrl Pts',(-25.8290449701193,66.8680635103876,12.));
#96696=CARTESIAN_POINT('Ctrl Pts',(-25.844249057147,66.8859026802088,0.));
#96697=CARTESIAN_POINT('Ctrl Pts',(-25.844249057147,66.8859026802088,12.));
#96698=CARTESIAN_POINT('Ctrl Pts',(-25.8594990868833,66.9037599932761,0.));
#96699=CARTESIAN_POINT('Ctrl Pts',(-25.8594990868833,66.9037599932761,12.));
#96700=CARTESIAN_POINT('Ctrl Pts',(-25.8747950260111,66.92163531213,0.));
#96701=CARTESIAN_POINT('Ctrl Pts',(-25.8747950260111,66.92163531213,12.));
#96702=CARTESIAN_POINT('Ctrl Pts',(-25.890136841266,66.939528499934,0.));
#96703=CARTESIAN_POINT('Ctrl Pts',(-25.890136841266,66.939528499934,12.));
#96704=CARTESIAN_POINT('Ctrl Pts',(-25.9055244994277,66.9574394204663,0.));
#96705=CARTESIAN_POINT('Ctrl Pts',(-25.9055244994277,66.9574394204663,12.));
#96706=CARTESIAN_POINT('Ctrl Pts',(-25.9209579673209,66.975367938115,0.));
#96707=CARTESIAN_POINT('Ctrl Pts',(-25.9209579673209,66.975367938115,12.));
#96708=CARTESIAN_POINT('Ctrl Pts',(-25.9364372118222,66.9933139178778,0.));
#96709=CARTESIAN_POINT('Ctrl Pts',(-25.9364372118222,66.9933139178778,12.));
#96710=CARTESIAN_POINT('Ctrl Pts',(-25.9519621998598,67.0112772253556,0.));
#96711=CARTESIAN_POINT('Ctrl Pts',(-25.9519621998598,67.0112772253556,12.));
#96712=CARTESIAN_POINT('Ctrl Pts',(-25.9675328984121,67.0292577267489,0.));
#96713=CARTESIAN_POINT('Ctrl Pts',(-25.9675328984121,67.0292577267489,12.));
#96714=CARTESIAN_POINT('Ctrl Pts',(-25.9831492744984,67.0472552888485,0.));
#96715=CARTESIAN_POINT('Ctrl Pts',(-25.9831492744984,67.0472552888485,12.));
#96716=CARTESIAN_POINT('Ctrl Pts',(-25.9988112951814,67.0652697790325,0.));
#96717=CARTESIAN_POINT('Ctrl Pts',(-25.9988112951814,67.0652697790325,12.));
#96718=CARTESIAN_POINT('Ctrl Pts',(-26.014518927573,67.0833010652634,0.));
#96719=CARTESIAN_POINT('Ctrl Pts',(-26.014518927573,67.0833010652634,12.));
#96720=CARTESIAN_POINT('Ctrl Pts',(-26.030272138834,67.101349016084,0.));
#96721=CARTESIAN_POINT('Ctrl Pts',(-26.030272138834,67.101349016084,12.));
#96722=CARTESIAN_POINT('Ctrl Pts',(-26.0460708961725,67.1194135006124,0.));
#96723=CARTESIAN_POINT('Ctrl Pts',(-26.0460708961725,67.1194135006124,12.));
#96724=CARTESIAN_POINT('Ctrl Pts',(-26.061915166836,67.1374943885354,0.));
#96725=CARTESIAN_POINT('Ctrl Pts',(-26.061915166836,67.1374943885354,12.));
#96726=CARTESIAN_POINT('Ctrl Pts',(-26.0778049181128,67.1555915501049,0.));
#96727=CARTESIAN_POINT('Ctrl Pts',(-26.0778049181128,67.1555915501049,12.));
#96728=CARTESIAN_POINT('Ctrl Pts',(-26.0937401173383,67.173704856136,0.));
#96729=CARTESIAN_POINT('Ctrl Pts',(-26.0937401173383,67.173704856136,12.));
#96730=CARTESIAN_POINT('Ctrl Pts',(-26.1097207318949,67.1918341780018,0.));
#96731=CARTESIAN_POINT('Ctrl Pts',(-26.1097207318949,67.1918341780018,12.));
#96732=CARTESIAN_POINT('Ctrl Pts',(-26.1257467292102,67.2099793876297,0.));
#96733=CARTESIAN_POINT('Ctrl Pts',(-26.1257467292102,67.2099793876297,12.));
#96734=CARTESIAN_POINT('Ctrl Pts',(-26.1418180767489,67.2281403574938,0.));
#96735=CARTESIAN_POINT('Ctrl Pts',(-26.1418180767489,67.2281403574938,12.));
#96736=CARTESIAN_POINT('Ctrl Pts',(-26.1579347420138,67.2463169606115,0.));
#96737=CARTESIAN_POINT('Ctrl Pts',(-26.1579347420138,67.2463169606115,12.));
#96738=CARTESIAN_POINT('Ctrl Pts',(-26.1740966925529,67.2645090705421,0.));
#96739=CARTESIAN_POINT('Ctrl Pts',(-26.1740966925529,67.2645090705421,12.));
#96740=CARTESIAN_POINT('Ctrl Pts',(-26.1903038959589,67.282716561383,0.));
#96741=CARTESIAN_POINT('Ctrl Pts',(-26.1903038959589,67.282716561383,12.));
#96742=CARTESIAN_POINT('Ctrl Pts',(-26.2065563198683,67.3009393077651,0.));
#96743=CARTESIAN_POINT('Ctrl Pts',(-26.2065563198683,67.3009393077651,12.));
#96744=CARTESIAN_POINT('Ctrl Pts',(-26.2228539319526,67.3191771848463,0.));
#96745=CARTESIAN_POINT('Ctrl Pts',(-26.2228539319526,67.3191771848463,12.));
#96746=CARTESIAN_POINT('Ctrl Pts',(-26.2391966999191,67.3374300683073,0.));
#96747=CARTESIAN_POINT('Ctrl Pts',(-26.2391966999191,67.3374300683073,12.));
#96748=CARTESIAN_POINT('Ctrl Pts',(-26.255584591518,67.3556978343507,0.));
#96749=CARTESIAN_POINT('Ctrl Pts',(-26.255584591518,67.3556978343507,12.));
#96750=CARTESIAN_POINT('Ctrl Pts',(-26.2720175745423,67.3739803596969,0.));
#96751=CARTESIAN_POINT('Ctrl Pts',(-26.2720175745423,67.3739803596969,12.));
#96752=CARTESIAN_POINT('Ctrl Pts',(-26.288495616827,67.392277521581,0.));
#96753=CARTESIAN_POINT('Ctrl Pts',(-26.288495616827,67.392277521581,12.));
#96754=CARTESIAN_POINT('Ctrl Pts',(-26.3050186862407,67.4105891977461,0.));
#96755=CARTESIAN_POINT('Ctrl Pts',(-26.3050186862407,67.4105891977461,12.));
#96756=CARTESIAN_POINT('Ctrl Pts',(-26.321586750686,67.4289152664398,0.));
#96757=CARTESIAN_POINT('Ctrl Pts',(-26.321586750686,67.4289152664398,12.));
#96758=CARTESIAN_POINT('Ctrl Pts',(-26.3381997781055,67.4472556064119,0.));
#96759=CARTESIAN_POINT('Ctrl Pts',(-26.3381997781055,67.4472556064119,12.));
#96760=CARTESIAN_POINT('Ctrl Pts',(-26.3548577364833,67.4656100969116,0.));
#96761=CARTESIAN_POINT('Ctrl Pts',(-26.3548577364833,67.4656100969116,12.));
#96762=CARTESIAN_POINT('Ctrl Pts',(-26.3715605938433,67.4839786176836,0.));
#96763=CARTESIAN_POINT('Ctrl Pts',(-26.3715605938433,67.4839786176836,12.));
#96764=CARTESIAN_POINT('Ctrl Pts',(-26.3883083182421,67.5023610489622,0.));
#96765=CARTESIAN_POINT('Ctrl Pts',(-26.3883083182421,67.5023610489622,12.));
#96766=CARTESIAN_POINT('Ctrl Pts',(-26.4051008777675,67.5207572714683,0.));
#96767=CARTESIAN_POINT('Ctrl Pts',(-26.4051008777675,67.5207572714683,12.));
#96768=CARTESIAN_POINT('Ctrl Pts',(-26.4219382405458,67.5391671664072,0.));
#96769=CARTESIAN_POINT('Ctrl Pts',(-26.4219382405458,67.5391671664072,12.));
#96770=CARTESIAN_POINT('Ctrl Pts',(-26.4388203747425,67.5575906154657,0.));
#96771=CARTESIAN_POINT('Ctrl Pts',(-26.4388203747425,67.5575906154657,12.));
#96772=CARTESIAN_POINT('Ctrl Pts',(-26.4557472485621,67.5760275008093,0.));
#96773=CARTESIAN_POINT('Ctrl Pts',(-26.4557472485621,67.5760275008093,12.));
#96774=CARTESIAN_POINT('Ctrl Pts',(-26.4727188302409,67.5944777050768,0.));
#96775=CARTESIAN_POINT('Ctrl Pts',(-26.4727188302409,67.5944777050768,12.));
#96776=CARTESIAN_POINT('Ctrl Pts',(-26.489735088044,67.6129411113757,0.));
#96777=CARTESIAN_POINT('Ctrl Pts',(-26.489735088044,67.6129411113757,12.));
#96778=CARTESIAN_POINT('Ctrl Pts',(-26.5067959902725,67.6314176032811,0.));
#96779=CARTESIAN_POINT('Ctrl Pts',(-26.5067959902725,67.6314176032811,12.));
#96780=CARTESIAN_POINT('Ctrl Pts',(-26.5239015052654,67.649907064832,0.));
#96781=CARTESIAN_POINT('Ctrl Pts',(-26.5239015052654,67.649907064832,12.));
#96782=CARTESIAN_POINT('Ctrl Pts',(-26.5410516013985,67.6684093805291,0.));
#96783=CARTESIAN_POINT('Ctrl Pts',(-26.5410516013985,67.6684093805291,12.));
#96784=CARTESIAN_POINT('Ctrl Pts',(-26.5582462470794,67.6869244353294,0.));
#96785=CARTESIAN_POINT('Ctrl Pts',(-26.5582462470794,67.6869244353294,12.));
#96786=CARTESIAN_POINT('Ctrl Pts',(-26.5754854107421,67.7054521146424,0.));
#96787=CARTESIAN_POINT('Ctrl Pts',(-26.5754854107421,67.7054521146424,12.));
#96788=CARTESIAN_POINT('Ctrl Pts',(-26.5927690608544,67.7239923043288,0.));
#96789=CARTESIAN_POINT('Ctrl Pts',(-26.5927690608544,67.7239923043288,12.));
#96790=CARTESIAN_POINT('Ctrl Pts',(-26.6100971659202,67.7425448906977,0.));
#96791=CARTESIAN_POINT('Ctrl Pts',(-26.6100971659202,67.7425448906977,12.));
#96792=CARTESIAN_POINT('Ctrl Pts',(-26.6274696944793,67.7611097605042,0.));
#96793=CARTESIAN_POINT('Ctrl Pts',(-26.6274696944793,67.7611097605042,12.));
#96794=CARTESIAN_POINT('Ctrl Pts',(-26.6448866151029,67.7796868009455,0.));
#96795=CARTESIAN_POINT('Ctrl Pts',(-26.6448866151029,67.7796868009455,12.));
#96796=CARTESIAN_POINT('Ctrl Pts',(-26.6623478963871,67.798275899657,0.));
#96797=CARTESIAN_POINT('Ctrl Pts',(-26.6623478963871,67.798275899657,12.));
#96798=CARTESIAN_POINT('Ctrl Pts',(-26.6798535069589,67.8168769447098,0.));
#96799=CARTESIAN_POINT('Ctrl Pts',(-26.6798535069589,67.8168769447098,12.));
#96800=CARTESIAN_POINT('Ctrl Pts',(-26.6974034154804,67.8354898246086,0.));
#96801=CARTESIAN_POINT('Ctrl Pts',(-26.6974034154804,67.8354898246086,12.));
#96802=CARTESIAN_POINT('Ctrl Pts',(-26.7149975906478,67.8541144282875,0.));
#96803=CARTESIAN_POINT('Ctrl Pts',(-26.7149975906478,67.8541144282875,12.));
#96804=CARTESIAN_POINT('Ctrl Pts',(-26.7326360011885,67.8727506451063,0.));
#96805=CARTESIAN_POINT('Ctrl Pts',(-26.7326360011885,67.8727506451063,12.));
#96806=CARTESIAN_POINT('Ctrl Pts',(-26.7503186158522,67.8913983648436,0.));
#96807=CARTESIAN_POINT('Ctrl Pts',(-26.7503186158522,67.8913983648436,12.));
#96808=CARTESIAN_POINT('Ctrl Pts',(-26.7680454034169,67.9100574776972,0.));
#96809=CARTESIAN_POINT('Ctrl Pts',(-26.7680454034169,67.9100574776972,12.));
#96810=CARTESIAN_POINT('Ctrl Pts',(-26.7858163326934,67.928727874284,0.));
#96811=CARTESIAN_POINT('Ctrl Pts',(-26.7858163326934,67.928727874284,12.));
#96812=CARTESIAN_POINT('Ctrl Pts',(-26.8036313725262,67.9474094456396,0.));
#96813=CARTESIAN_POINT('Ctrl Pts',(-26.8036313725262,67.9474094456396,12.));
#96814=CARTESIAN_POINT('Ctrl Pts',(-26.821490491792,67.9661020832164,0.));
#96815=CARTESIAN_POINT('Ctrl Pts',(-26.821490491792,67.9661020832164,12.));
#96816=CARTESIAN_POINT('Ctrl Pts',(-26.8393936593911,67.9848056788809,0.));
#96817=CARTESIAN_POINT('Ctrl Pts',(-26.8393936593911,67.9848056788809,12.));
#96818=CARTESIAN_POINT('Ctrl Pts',(-26.8573408442496,68.0035201249102,0.));
#96819=CARTESIAN_POINT('Ctrl Pts',(-26.8573408442496,68.0035201249102,12.));
#96820=CARTESIAN_POINT('Ctrl Pts',(-26.8753320153252,68.0222453139856,0.));
#96821=CARTESIAN_POINT('Ctrl Pts',(-26.8753320153252,68.0222453139856,12.));
#96822=CARTESIAN_POINT('Ctrl Pts',(-26.8933671416063,68.0409811391869,0.));
#96823=CARTESIAN_POINT('Ctrl Pts',(-26.8933671416063,68.0409811391869,12.));
#96824=CARTESIAN_POINT('Ctrl Pts',(-26.911446192111,68.0597274939859,0.));
#96825=CARTESIAN_POINT('Ctrl Pts',(-26.911446192111,68.0597274939859,12.));
#96826=CARTESIAN_POINT('Ctrl Pts',(-26.9295691358779,68.0784842722369,0.));
#96827=CARTESIAN_POINT('Ctrl Pts',(-26.9295691358779,68.0784842722369,12.));
#96828=CARTESIAN_POINT('Ctrl Pts',(-26.9477359419652,68.0972513681751,0.));
#96829=CARTESIAN_POINT('Ctrl Pts',(-26.9477359419652,68.0972513681751,12.));
#96830=CARTESIAN_POINT('Ctrl Pts',(-26.9659465794601,68.1160286764255,0.));
#96831=CARTESIAN_POINT('Ctrl Pts',(-26.9659465794601,68.1160286764255,12.));
#96832=CARTESIAN_POINT('Ctrl Pts',(-26.9842010174822,68.1348160920106,0.));
#96833=CARTESIAN_POINT('Ctrl Pts',(-26.9842010174822,68.1348160920106,12.));
#96834=CARTESIAN_POINT('Ctrl Pts',(-27.0024992251838,68.1536135103557,0.));
#96835=CARTESIAN_POINT('Ctrl Pts',(-27.0024992251838,68.1536135103557,12.));
#96836=CARTESIAN_POINT('Ctrl Pts',(-27.0208411717472,68.1724208272958,0.));
#96837=CARTESIAN_POINT('Ctrl Pts',(-27.0208411717472,68.1724208272958,12.));
#96838=CARTESIAN_POINT('Ctrl Pts',(-27.0392268263798,68.1912379390773,0.));
#96839=CARTESIAN_POINT('Ctrl Pts',(-27.0392268263798,68.1912379390773,12.));
#96840=CARTESIAN_POINT('Ctrl Pts',(-27.0576561583172,68.2100647423332,0.));
#96841=CARTESIAN_POINT('Ctrl Pts',(-27.0576561583172,68.2100647423332,12.));
#96842=CARTESIAN_POINT('Ctrl Pts',(-27.0761291368226,68.2289011340615,0.));
#96843=CARTESIAN_POINT('Ctrl Pts',(-27.0761291368226,68.2289011340615,12.));
#96844=CARTESIAN_POINT('Ctrl Pts',(-27.0946457311813,68.2477470116012,0.));
#96845=CARTESIAN_POINT('Ctrl Pts',(-27.0946457311813,68.2477470116012,12.));
#96846=CARTESIAN_POINT('Ctrl Pts',(-27.1132059106943,68.2666022726104,0.));
#96847=CARTESIAN_POINT('Ctrl Pts',(-27.1132059106943,68.2666022726104,12.));
#96848=CARTESIAN_POINT('Ctrl Pts',(-27.1318096446649,68.2854668150364,0.));
#96849=CARTESIAN_POINT('Ctrl Pts',(-27.1318096446649,68.2854668150364,12.));
#96850=CARTESIAN_POINT('Ctrl Pts',(-27.1504569024136,68.3043405371603,0.));
#96851=CARTESIAN_POINT('Ctrl Pts',(-27.1504569024136,68.3043405371603,12.));
#96852=CARTESIAN_POINT('Ctrl Pts',(-27.1691476532921,68.3232233376425,0.));
#96853=CARTESIAN_POINT('Ctrl Pts',(-27.1691476532921,68.3232233376425,12.));
#96854=CARTESIAN_POINT('Ctrl Pts',(-27.1878818666926,68.3421151155711,0.));
#96855=CARTESIAN_POINT('Ctrl Pts',(-27.1878818666926,68.3421151155711,12.));
#96856=CARTESIAN_POINT('Ctrl Pts',(-27.2066595120542,68.3610157704994,0.));
#96857=CARTESIAN_POINT('Ctrl Pts',(-27.2066595120542,68.3610157704994,12.));
#96858=CARTESIAN_POINT('Ctrl Pts',(-27.2254805588673,68.3799252025102,0.));
#96859=CARTESIAN_POINT('Ctrl Pts',(-27.2254805588673,68.3799252025102,12.));
#96860=CARTESIAN_POINT('Ctrl Pts',(-27.244344976665,68.3988433121581,0.));
#96861=CARTESIAN_POINT('Ctrl Pts',(-27.244344976665,68.3988433121581,12.));
#96862=CARTESIAN_POINT('Ctrl Pts',(-27.263252735006,68.4177700003465,0.));
#96863=CARTESIAN_POINT('Ctrl Pts',(-27.263252735006,68.4177700003465,12.));
#96864=CARTESIAN_POINT('Ctrl Pts',(-27.2822038034538,68.4367051682164,0.));
#96865=CARTESIAN_POINT('Ctrl Pts',(-27.2822038034538,68.4367051682164,12.));
#96866=CARTESIAN_POINT('Ctrl Pts',(-27.301198151557,68.4556487170441,0.));
#96867=CARTESIAN_POINT('Ctrl Pts',(-27.301198151557,68.4556487170441,12.));
#96868=CARTESIAN_POINT('Ctrl Pts',(-27.3202357488154,68.4746005480997,0.));
#96869=CARTESIAN_POINT('Ctrl Pts',(-27.3202357488154,68.4746005480997,12.));
#96870=CARTESIAN_POINT('Ctrl Pts',(-27.3393165646752,68.4935605626372,0.));
#96871=CARTESIAN_POINT('Ctrl Pts',(-27.3393165646752,68.4935605626372,12.));
#96872=CARTESIAN_POINT('Ctrl Pts',(-27.3584405685947,68.5125286621902,0.));
#96873=CARTESIAN_POINT('Ctrl Pts',(-27.3584405685947,68.5125286621902,12.));
#96874=CARTESIAN_POINT('Ctrl Pts',(-27.3776077300918,68.5315047488046,0.));
#96875=CARTESIAN_POINT('Ctrl Pts',(-27.3776077300918,68.5315047488046,12.));
#96876=CARTESIAN_POINT('Ctrl Pts',(-27.3968180187941,68.5504887252976,0.));
#96877=CARTESIAN_POINT('Ctrl Pts',(-27.3968180187941,68.5504887252976,12.));
#96878=CARTESIAN_POINT('Ctrl Pts',(-27.4160714044825,68.5694804955002,0.));
#96879=CARTESIAN_POINT('Ctrl Pts',(-27.4160714044825,68.5694804955002,12.));
#96880=CARTESIAN_POINT('Ctrl Pts',(-27.4353678571349,68.5884799645193,0.));
#96881=CARTESIAN_POINT('Ctrl Pts',(-27.4353678571349,68.5884799645193,12.));
#96882=CARTESIAN_POINT('Ctrl Pts',(-27.4547073468213,68.6074870381588,0.));
#96883=CARTESIAN_POINT('Ctrl Pts',(-27.4547073468213,68.6074870381588,12.));
#96884=CARTESIAN_POINT('Ctrl Pts',(-27.4740898435977,68.6265016223536,0.));
#96885=CARTESIAN_POINT('Ctrl Pts',(-27.4740898435977,68.6265016223536,12.));
#96886=CARTESIAN_POINT('Ctrl Pts',(-27.4935153173863,68.6455236225471,0.));
#96887=CARTESIAN_POINT('Ctrl Pts',(-27.4935153173863,68.6455236225471,12.));
#96888=CARTESIAN_POINT('Ctrl Pts',(-27.5129837378798,68.6645529432059,0.));
#96889=CARTESIAN_POINT('Ctrl Pts',(-27.5129837378798,68.6645529432059,12.));
#96890=CARTESIAN_POINT('Ctrl Pts',(-27.5324950743723,68.683589486992,0.));
#96891=CARTESIAN_POINT('Ctrl Pts',(-27.5324950743723,68.683589486992,12.));
#96892=CARTESIAN_POINT('Ctrl Pts',(-27.552049295893,68.7026331554348,0.));
#96893=CARTESIAN_POINT('Ctrl Pts',(-27.552049295893,68.7026331554348,12.));
#96894=CARTESIAN_POINT('Ctrl Pts',(-27.5716463715027,68.721683850427,0.));
#96895=CARTESIAN_POINT('Ctrl Pts',(-27.5716463715027,68.721683850427,12.));
#96896=CARTESIAN_POINT('Ctrl Pts',(-27.5912862705482,68.7407414755291,0.));
#96897=CARTESIAN_POINT('Ctrl Pts',(-27.5912862705482,68.7407414755291,12.));
#96898=CARTESIAN_POINT('Ctrl Pts',(-27.6109689629025,68.7598059372121,0.));
#96899=CARTESIAN_POINT('Ctrl Pts',(-27.6109689629025,68.7598059372121,12.));
#96900=CARTESIAN_POINT('Ctrl Pts',(-27.6306944192711,68.7788771464655,0.));
#96901=CARTESIAN_POINT('Ctrl Pts',(-27.6306944192711,68.7788771464655,12.));
#96902=CARTESIAN_POINT('Ctrl Pts',(-27.6504626112621,68.7979550191773,0.));
#96903=CARTESIAN_POINT('Ctrl Pts',(-27.6504626112621,68.7979550191773,12.));
#96904=CARTESIAN_POINT('Ctrl Pts',(-27.670273510707,68.8170394725786,0.));
#96905=CARTESIAN_POINT('Ctrl Pts',(-27.670273510707,68.8170394725786,12.));
#96906=CARTESIAN_POINT('Ctrl Pts',(-27.6901270891201,68.8361304224378,0.));
#96907=CARTESIAN_POINT('Ctrl Pts',(-27.6901270891201,68.8361304224378,12.));
#96908=CARTESIAN_POINT('Ctrl Pts',(-27.7100233170728,68.855227779818,0.));
#96909=CARTESIAN_POINT('Ctrl Pts',(-27.7100233170728,68.855227779818,12.));
#96910=CARTESIAN_POINT('Ctrl Pts',(-27.7299621636602,68.8743314483451,0.));
#96911=CARTESIAN_POINT('Ctrl Pts',(-27.7299621636602,68.8743314483451,12.));
#96912=CARTESIAN_POINT('Ctrl Pts',(-27.7499435957608,68.8934413203945,0.));
#96913=CARTESIAN_POINT('Ctrl Pts',(-27.7499435957608,68.8934413203945,12.));
#96914=CARTESIAN_POINT('Ctrl Pts',(-27.7699675790683,68.9125572825946,0.));
#96915=CARTESIAN_POINT('Ctrl Pts',(-27.7699675790683,68.9125572825946,12.));
#96916=CARTESIAN_POINT('Ctrl Pts',(-27.7900340793796,68.9316792226187,0.));
#96917=CARTESIAN_POINT('Ctrl Pts',(-27.7900340793796,68.9316792226187,12.));
#96918=CARTESIAN_POINT('Ctrl Pts',(-27.8101430638128,68.9508070357786,0.));
#96919=CARTESIAN_POINT('Ctrl Pts',(-27.8101430638128,68.9508070357786,12.));
#96920=CARTESIAN_POINT('Ctrl Pts',(-27.8302945019939,68.9699406311305,0.));
#96921=CARTESIAN_POINT('Ctrl Pts',(-27.8302945019939,68.9699406311305,12.));
#96922=CARTESIAN_POINT('Ctrl Pts',(-27.8504883673903,68.9890799391863,0.));
#96923=CARTESIAN_POINT('Ctrl Pts',(-27.8504883673903,68.9890799391863,12.));
#96924=CARTESIAN_POINT('Ctrl Pts',(-27.8707246380697,69.0082249138015,0.));
#96925=CARTESIAN_POINT('Ctrl Pts',(-27.8707246380697,69.0082249138015,12.));
#96926=CARTESIAN_POINT('Ctrl Pts',(-27.8910032967037,69.0273755264702,0.));
#96927=CARTESIAN_POINT('Ctrl Pts',(-27.8910032967037,69.0273755264702,12.));
#96928=CARTESIAN_POINT('Ctrl Pts',(-27.9072601239469,69.0427005153223,0.));
#96929=CARTESIAN_POINT('Ctrl Pts',(-27.9072601239469,69.0427005153223,12.));
#96930=CARTESIAN_POINT('Ctrl Pts',(-27.9194718098851,69.0541967850685,0.));
#96931=CARTESIAN_POINT('Ctrl Pts',(-27.9194718098851,69.0541967850685,12.));
#96932=CARTESIAN_POINT('Ctrl Pts',(-27.9276214070576,69.0618620884596,0.));
#96933=CARTESIAN_POINT('Ctrl Pts',(-27.9276214070576,69.0618620884596,12.));
#96934=CARTESIAN_POINT('Ctrl Pts',(-27.9316983239472,69.065695021045,0.));
#96935=CARTESIAN_POINT('Ctrl Pts',(-27.9316983239472,69.065695021045,12.));
#96936=CARTESIAN_POINT('',(-24.7419628022042,65.4815644032299,0.));
#96937=CARTESIAN_POINT('Ctrl Pts',(-24.7419628022042,65.4815644032299,0.));
#96938=CARTESIAN_POINT('Ctrl Pts',(-24.7442214063382,65.4847237095443,0.));
#96939=CARTESIAN_POINT('Ctrl Pts',(-24.7487434955982,65.4910454936254,0.));
#96940=CARTESIAN_POINT('Ctrl Pts',(-24.7555412724651,65.5005376841101,0.));
#96941=CARTESIAN_POINT('Ctrl Pts',(-24.7646342620841,65.5132129675333,0.));
#96942=CARTESIAN_POINT('Ctrl Pts',(-24.7760493148465,65.5290887770232,0.));
#96943=CARTESIAN_POINT('Ctrl Pts',(-24.7875131827491,65.5449962514661,0.));
#96944=CARTESIAN_POINT('Ctrl Pts',(-24.799025856126,65.5609353062829,0.));
#96945=CARTESIAN_POINT('Ctrl Pts',(-24.8105873098626,65.5769057914333,0.));
#96946=CARTESIAN_POINT('Ctrl Pts',(-24.8221975032104,65.5929074932624,0.));
#96947=CARTESIAN_POINT('Ctrl Pts',(-24.8338563866764,65.6089401625628,0.));
#96948=CARTESIAN_POINT('Ctrl Pts',(-24.8455639071517,65.6250035361612,0.));
#96949=CARTESIAN_POINT('Ctrl Pts',(-24.8573200135666,65.6410973603661,0.));
#96950=CARTESIAN_POINT('Ctrl Pts',(-24.8691246628057,65.6572214156692,0.));
#96951=CARTESIAN_POINT('Ctrl Pts',(-24.8809778178229,65.6733755087669,0.));
#96952=CARTESIAN_POINT('Ctrl Pts',(-24.8928794448607,65.6895594608775,0.));
#96953=CARTESIAN_POINT('Ctrl Pts',(-24.9048295111448,65.7057730980483,0.));
#96954=CARTESIAN_POINT('Ctrl Pts',(-24.9168279820106,65.7220162391053,0.));
#96955=CARTESIAN_POINT('Ctrl Pts',(-24.928874819458,65.7382886895888,0.));
#96956=CARTESIAN_POINT('Ctrl Pts',(-24.9409699836537,65.7545902480323,0.));
#96957=CARTESIAN_POINT('Ctrl Pts',(-24.9531134338696,65.7709207098959,0.));
#96958=CARTESIAN_POINT('Ctrl Pts',(-24.9653051295581,65.7872798720823,0.));
#96959=CARTESIAN_POINT('Ctrl Pts',(-24.9775450315683,65.8036675380718,0.));
#96960=CARTESIAN_POINT('Ctrl Pts',(-24.9898331020983,65.8200835177024,0.));
#96961=CARTESIAN_POINT('Ctrl Pts',(-25.002169304117,65.8365276247128,0.));
#96962=CARTESIAN_POINT('Ctrl Pts',(-25.0145536009604,65.8529996750445,0.));
#96963=CARTESIAN_POINT('Ctrl Pts',(-25.0269859558363,65.8694994847616,0.));
#96964=CARTESIAN_POINT('Ctrl Pts',(-25.0394663314055,65.8860268683128,0.));
#96965=CARTESIAN_POINT('Ctrl Pts',(-25.0519946900078,65.9025816394424,0.));
#96966=CARTESIAN_POINT('Ctrl Pts',(-25.0645709938524,65.919163611981,0.));
#96967=CARTESIAN_POINT('Ctrl Pts',(-25.0771952052028,65.9357726006163,0.));
#96968=CARTESIAN_POINT('Ctrl Pts',(-25.0898672865915,65.9524084218139,0.));
#96969=CARTESIAN_POINT('Ctrl Pts',(-25.1025872009004,65.9690708941558,0.));
#96970=CARTESIAN_POINT('Ctrl Pts',(-25.1153549112503,65.9857598378433,0.));
#96971=CARTESIAN_POINT('Ctrl Pts',(-25.1281703809297,66.0024750743897,0.));
#96972=CARTESIAN_POINT('Ctrl Pts',(-25.1410335733099,66.0192164262621,0.));
#96973=CARTESIAN_POINT('Ctrl Pts',(-25.1539444517419,66.0359837164734,0.));
#96974=CARTESIAN_POINT('Ctrl Pts',(-25.1669029795661,66.0527767686025,0.));
#96975=CARTESIAN_POINT('Ctrl Pts',(-25.1799091201599,66.0695954069713,0.));
#96976=CARTESIAN_POINT('Ctrl Pts',(-25.1929628369685,66.086439456768,0.));
#96977=CARTESIAN_POINT('Ctrl Pts',(-25.2060640935365,66.10330874419,0.));
#96978=CARTESIAN_POINT('Ctrl Pts',(-25.2192128535357,66.1202030965758,0.));
#96979=CARTESIAN_POINT('Ctrl Pts',(-25.232409080755,66.1371223423345,0.));
#96980=CARTESIAN_POINT('Ctrl Pts',(-25.2456527390875,66.1540663108754,0.));
#96981=CARTESIAN_POINT('Ctrl Pts',(-25.2589437925147,66.1710348325384,0.));
#96982=CARTESIAN_POINT('Ctrl Pts',(-25.2722822050837,66.1880277385136,0.));
#96983=CARTESIAN_POINT('Ctrl Pts',(-25.285667940893,66.2050448607911,0.));
#96984=CARTESIAN_POINT('Ctrl Pts',(-25.2991009641094,66.2220860321952,0.));
#96985=CARTESIAN_POINT('Ctrl Pts',(-25.312581238973,66.2391510863998,0.));
#96986=CARTESIAN_POINT('Ctrl Pts',(-25.3261087298026,66.2562398579471,0.));
#96987=CARTESIAN_POINT('Ctrl Pts',(-25.3396834009949,66.2733521822662,0.));
#96988=CARTESIAN_POINT('Ctrl Pts',(-25.3533052170249,66.290487895671,0.));
#96989=CARTESIAN_POINT('Ctrl Pts',(-25.3669741424488,66.3076468353412,0.));
#96990=CARTESIAN_POINT('Ctrl Pts',(-25.3806901419012,66.3248288393046,0.));
#96991=CARTESIAN_POINT('Ctrl Pts',(-25.3944531800901,66.3420337464178,0.));
#96992=CARTESIAN_POINT('Ctrl Pts',(-25.4082632217847,66.359261396341,0.));
#96993=CARTESIAN_POINT('Ctrl Pts',(-25.4221202318199,66.3765116295364,0.));
#96994=CARTESIAN_POINT('Ctrl Pts',(-25.4360241751018,66.3937842872685,0.));
#96995=CARTESIAN_POINT('Ctrl Pts',(-25.4499750166079,66.4110792116,0.));
#96996=CARTESIAN_POINT('Ctrl Pts',(-25.4639727213849,66.4283962453899,0.));
#96997=CARTESIAN_POINT('Ctrl Pts',(-25.4780172545417,66.4457352322871,0.));
#96998=CARTESIAN_POINT('Ctrl Pts',(-25.4921085812548,66.4630960167252,0.));
#96999=CARTESIAN_POINT('Ctrl Pts',(-25.5062466667702,66.4804784439148,0.));
#97000=CARTESIAN_POINT('Ctrl Pts',(-25.5204314764033,66.4978823598354,0.));
#97001=CARTESIAN_POINT('Ctrl Pts',(-25.534662975532,66.5153076112231,0.));
#97002=CARTESIAN_POINT('Ctrl Pts',(-25.5489411295912,66.5327540455624,0.));
#97003=CARTESIAN_POINT('Ctrl Pts',(-25.5632659040792,66.5502215110829,0.));
#97004=CARTESIAN_POINT('Ctrl Pts',(-25.5776372645601,66.5677098567542,0.));
#97005=CARTESIAN_POINT('Ctrl Pts',(-25.5920551766629,66.5852189322813,0.));
#97006=CARTESIAN_POINT('Ctrl Pts',(-25.6065196060756,66.6027485880963,0.));
#97007=CARTESIAN_POINT('Ctrl Pts',(-25.6210305185403,66.6202986753506,0.));
#97008=CARTESIAN_POINT('Ctrl Pts',(-25.6355878798614,66.6378690459129,0.));
#97009=CARTESIAN_POINT('Ctrl Pts',(-25.6501916559055,66.6554595523624,0.));
#97010=CARTESIAN_POINT('Ctrl Pts',(-25.6648418126013,66.6730700479837,0.));
#97011=CARTESIAN_POINT('Ctrl Pts',(-25.6795383159319,66.6907003867572,0.));
#97012=CARTESIAN_POINT('Ctrl Pts',(-25.6942811319322,66.7083504233529,0.));
#97013=CARTESIAN_POINT('Ctrl Pts',(-25.7090702266963,66.7260200131266,0.));
#97014=CARTESIAN_POINT('Ctrl Pts',(-25.7239055663772,66.7437090121153,0.));
#97015=CARTESIAN_POINT('Ctrl Pts',(-25.7387871171866,66.7614172770316,0.));
#97016=CARTESIAN_POINT('Ctrl Pts',(-25.7537148453864,66.7791446652545,0.));
#97017=CARTESIAN_POINT('Ctrl Pts',(-25.7686887172878,66.7968910348245,0.));
#97018=CARTESIAN_POINT('Ctrl Pts',(-25.7837086992595,66.8146562444433,0.));
#97019=CARTESIAN_POINT('Ctrl Pts',(-25.7987747577269,66.8324401534668,0.));
#97020=CARTESIAN_POINT('Ctrl Pts',(-25.8138868591709,66.8502426219001,0.));
#97021=CARTESIAN_POINT('Ctrl Pts',(-25.8290449701193,66.8680635103876,0.));
#97022=CARTESIAN_POINT('Ctrl Pts',(-25.844249057147,66.8859026802088,0.));
#97023=CARTESIAN_POINT('Ctrl Pts',(-25.8594990868833,66.9037599932761,0.));
#97024=CARTESIAN_POINT('Ctrl Pts',(-25.8747950260111,66.92163531213,0.));
#97025=CARTESIAN_POINT('Ctrl Pts',(-25.890136841266,66.939528499934,0.));
#97026=CARTESIAN_POINT('Ctrl Pts',(-25.9055244994277,66.9574394204663,0.));
#97027=CARTESIAN_POINT('Ctrl Pts',(-25.9209579673209,66.975367938115,0.));
#97028=CARTESIAN_POINT('Ctrl Pts',(-25.9364372118222,66.9933139178778,0.));
#97029=CARTESIAN_POINT('Ctrl Pts',(-25.9519621998598,67.0112772253556,0.));
#97030=CARTESIAN_POINT('Ctrl Pts',(-25.9675328984121,67.0292577267489,0.));
#97031=CARTESIAN_POINT('Ctrl Pts',(-25.9831492744984,67.0472552888485,0.));
#97032=CARTESIAN_POINT('Ctrl Pts',(-25.9988112951814,67.0652697790325,0.));
#97033=CARTESIAN_POINT('Ctrl Pts',(-26.014518927573,67.0833010652634,0.));
#97034=CARTESIAN_POINT('Ctrl Pts',(-26.030272138834,67.101349016084,0.));
#97035=CARTESIAN_POINT('Ctrl Pts',(-26.0460708961725,67.1194135006124,0.));
#97036=CARTESIAN_POINT('Ctrl Pts',(-26.061915166836,67.1374943885354,0.));
#97037=CARTESIAN_POINT('Ctrl Pts',(-26.0778049181128,67.1555915501049,0.));
#97038=CARTESIAN_POINT('Ctrl Pts',(-26.0937401173383,67.173704856136,0.));
#97039=CARTESIAN_POINT('Ctrl Pts',(-26.1097207318949,67.1918341780018,0.));
#97040=CARTESIAN_POINT('Ctrl Pts',(-26.1257467292102,67.2099793876297,0.));
#97041=CARTESIAN_POINT('Ctrl Pts',(-26.1418180767489,67.2281403574938,0.));
#97042=CARTESIAN_POINT('Ctrl Pts',(-26.1579347420138,67.2463169606115,0.));
#97043=CARTESIAN_POINT('Ctrl Pts',(-26.1740966925529,67.2645090705421,0.));
#97044=CARTESIAN_POINT('Ctrl Pts',(-26.1903038959589,67.282716561383,0.));
#97045=CARTESIAN_POINT('Ctrl Pts',(-26.2065563198683,67.3009393077651,0.));
#97046=CARTESIAN_POINT('Ctrl Pts',(-26.2228539319526,67.3191771848463,0.));
#97047=CARTESIAN_POINT('Ctrl Pts',(-26.2391966999191,67.3374300683073,0.));
#97048=CARTESIAN_POINT('Ctrl Pts',(-26.255584591518,67.3556978343507,0.));
#97049=CARTESIAN_POINT('Ctrl Pts',(-26.2720175745423,67.3739803596969,0.));
#97050=CARTESIAN_POINT('Ctrl Pts',(-26.288495616827,67.392277521581,0.));
#97051=CARTESIAN_POINT('Ctrl Pts',(-26.3050186862407,67.4105891977461,0.));
#97052=CARTESIAN_POINT('Ctrl Pts',(-26.321586750686,67.4289152664398,0.));
#97053=CARTESIAN_POINT('Ctrl Pts',(-26.3381997781055,67.4472556064119,0.));
#97054=CARTESIAN_POINT('Ctrl Pts',(-26.3548577364833,67.4656100969116,0.));
#97055=CARTESIAN_POINT('Ctrl Pts',(-26.3715605938433,67.4839786176836,0.));
#97056=CARTESIAN_POINT('Ctrl Pts',(-26.3883083182421,67.5023610489622,0.));
#97057=CARTESIAN_POINT('Ctrl Pts',(-26.4051008777675,67.5207572714683,0.));
#97058=CARTESIAN_POINT('Ctrl Pts',(-26.4219382405458,67.5391671664072,0.));
#97059=CARTESIAN_POINT('Ctrl Pts',(-26.4388203747425,67.5575906154657,0.));
#97060=CARTESIAN_POINT('Ctrl Pts',(-26.4557472485621,67.5760275008093,0.));
#97061=CARTESIAN_POINT('Ctrl Pts',(-26.4727188302409,67.5944777050768,0.));
#97062=CARTESIAN_POINT('Ctrl Pts',(-26.489735088044,67.6129411113757,0.));
#97063=CARTESIAN_POINT('Ctrl Pts',(-26.5067959902725,67.6314176032811,0.));
#97064=CARTESIAN_POINT('Ctrl Pts',(-26.5239015052654,67.649907064832,0.));
#97065=CARTESIAN_POINT('Ctrl Pts',(-26.5410516013985,67.6684093805291,0.));
#97066=CARTESIAN_POINT('Ctrl Pts',(-26.5582462470794,67.6869244353294,0.));
#97067=CARTESIAN_POINT('Ctrl Pts',(-26.5754854107421,67.7054521146424,0.));
#97068=CARTESIAN_POINT('Ctrl Pts',(-26.5927690608544,67.7239923043288,0.));
#97069=CARTESIAN_POINT('Ctrl Pts',(-26.6100971659202,67.7425448906977,0.));
#97070=CARTESIAN_POINT('Ctrl Pts',(-26.6274696944793,67.7611097605042,0.));
#97071=CARTESIAN_POINT('Ctrl Pts',(-26.6448866151029,67.7796868009455,0.));
#97072=CARTESIAN_POINT('Ctrl Pts',(-26.6623478963871,67.798275899657,0.));
#97073=CARTESIAN_POINT('Ctrl Pts',(-26.6798535069589,67.8168769447098,0.));
#97074=CARTESIAN_POINT('Ctrl Pts',(-26.6974034154804,67.8354898246086,0.));
#97075=CARTESIAN_POINT('Ctrl Pts',(-26.7149975906478,67.8541144282875,0.));
#97076=CARTESIAN_POINT('Ctrl Pts',(-26.7326360011885,67.8727506451063,0.));
#97077=CARTESIAN_POINT('Ctrl Pts',(-26.7503186158522,67.8913983648436,0.));
#97078=CARTESIAN_POINT('Ctrl Pts',(-26.7680454034169,67.9100574776972,0.));
#97079=CARTESIAN_POINT('Ctrl Pts',(-26.7858163326934,67.928727874284,0.));
#97080=CARTESIAN_POINT('Ctrl Pts',(-26.8036313725262,67.9474094456396,0.));
#97081=CARTESIAN_POINT('Ctrl Pts',(-26.821490491792,67.9661020832164,0.));
#97082=CARTESIAN_POINT('Ctrl Pts',(-26.8393936593911,67.9848056788809,0.));
#97083=CARTESIAN_POINT('Ctrl Pts',(-26.8573408442496,68.0035201249102,0.));
#97084=CARTESIAN_POINT('Ctrl Pts',(-26.8753320153252,68.0222453139856,0.));
#97085=CARTESIAN_POINT('Ctrl Pts',(-26.8933671416063,68.0409811391869,0.));
#97086=CARTESIAN_POINT('Ctrl Pts',(-26.911446192111,68.0597274939859,0.));
#97087=CARTESIAN_POINT('Ctrl Pts',(-26.9295691358779,68.0784842722369,0.));
#97088=CARTESIAN_POINT('Ctrl Pts',(-26.9477359419652,68.0972513681751,0.));
#97089=CARTESIAN_POINT('Ctrl Pts',(-26.9659465794601,68.1160286764255,0.));
#97090=CARTESIAN_POINT('Ctrl Pts',(-26.9842010174822,68.1348160920106,0.));
#97091=CARTESIAN_POINT('Ctrl Pts',(-27.0024992251838,68.1536135103557,0.));
#97092=CARTESIAN_POINT('Ctrl Pts',(-27.0208411717472,68.1724208272958,0.));
#97093=CARTESIAN_POINT('Ctrl Pts',(-27.0392268263798,68.1912379390773,0.));
#97094=CARTESIAN_POINT('Ctrl Pts',(-27.0576561583172,68.2100647423332,0.));
#97095=CARTESIAN_POINT('Ctrl Pts',(-27.0761291368226,68.2289011340615,0.));
#97096=CARTESIAN_POINT('Ctrl Pts',(-27.0946457311813,68.2477470116012,0.));
#97097=CARTESIAN_POINT('Ctrl Pts',(-27.1132059106943,68.2666022726104,0.));
#97098=CARTESIAN_POINT('Ctrl Pts',(-27.1318096446649,68.2854668150364,0.));
#97099=CARTESIAN_POINT('Ctrl Pts',(-27.1504569024136,68.3043405371603,0.));
#97100=CARTESIAN_POINT('Ctrl Pts',(-27.1691476532921,68.3232233376425,0.));
#97101=CARTESIAN_POINT('Ctrl Pts',(-27.1878818666926,68.3421151155711,0.));
#97102=CARTESIAN_POINT('Ctrl Pts',(-27.2066595120542,68.3610157704994,0.));
#97103=CARTESIAN_POINT('Ctrl Pts',(-27.2254805588673,68.3799252025102,0.));
#97104=CARTESIAN_POINT('Ctrl Pts',(-27.244344976665,68.3988433121581,0.));
#97105=CARTESIAN_POINT('Ctrl Pts',(-27.263252735006,68.4177700003465,0.));
#97106=CARTESIAN_POINT('Ctrl Pts',(-27.2822038034538,68.4367051682164,0.));
#97107=CARTESIAN_POINT('Ctrl Pts',(-27.301198151557,68.4556487170441,0.));
#97108=CARTESIAN_POINT('Ctrl Pts',(-27.3202357488154,68.4746005480997,0.));
#97109=CARTESIAN_POINT('Ctrl Pts',(-27.3393165646752,68.4935605626372,0.));
#97110=CARTESIAN_POINT('Ctrl Pts',(-27.3584405685947,68.5125286621902,0.));
#97111=CARTESIAN_POINT('Ctrl Pts',(-27.3776077300918,68.5315047488046,0.));
#97112=CARTESIAN_POINT('Ctrl Pts',(-27.3968180187941,68.5504887252976,0.));
#97113=CARTESIAN_POINT('Ctrl Pts',(-27.4160714044825,68.5694804955002,0.));
#97114=CARTESIAN_POINT('Ctrl Pts',(-27.4353678571349,68.5884799645193,0.));
#97115=CARTESIAN_POINT('Ctrl Pts',(-27.4547073468213,68.6074870381588,0.));
#97116=CARTESIAN_POINT('Ctrl Pts',(-27.4740898435977,68.6265016223536,0.));
#97117=CARTESIAN_POINT('Ctrl Pts',(-27.4935153173863,68.6455236225471,0.));
#97118=CARTESIAN_POINT('Ctrl Pts',(-27.5129837378798,68.6645529432059,0.));
#97119=CARTESIAN_POINT('Ctrl Pts',(-27.5324950743723,68.683589486992,0.));
#97120=CARTESIAN_POINT('Ctrl Pts',(-27.552049295893,68.7026331554348,0.));
#97121=CARTESIAN_POINT('Ctrl Pts',(-27.5716463715027,68.721683850427,0.));
#97122=CARTESIAN_POINT('Ctrl Pts',(-27.5912862705482,68.7407414755291,0.));
#97123=CARTESIAN_POINT('Ctrl Pts',(-27.6109689629025,68.7598059372121,0.));
#97124=CARTESIAN_POINT('Ctrl Pts',(-27.6306944192711,68.7788771464655,0.));
#97125=CARTESIAN_POINT('Ctrl Pts',(-27.6504626112621,68.7979550191773,0.));
#97126=CARTESIAN_POINT('Ctrl Pts',(-27.6674443909882,68.8143140938753,0.));
#97127=CARTESIAN_POINT('Ctrl Pts',(-27.6804870323286,68.826859785198,0.));
#97128=CARTESIAN_POINT('Ctrl Pts',(-27.6895716271084,68.8355891981877,0.));
#97129=CARTESIAN_POINT('Ctrl Pts',(-27.6946856803482,68.8405004465895,0.));
#97130=CARTESIAN_POINT('Ctrl Pts',(-27.6958230984757,68.8415926174774,0.));
#97131=CARTESIAN_POINT('',(-24.7419628022042,65.4815644032299,12.));
#97132=CARTESIAN_POINT('',(-24.7419628022042,65.4815644032299,0.));
#97133=CARTESIAN_POINT('Ctrl Pts',(-27.6958230984758,68.8415926174774,12.));
#97134=CARTESIAN_POINT('Ctrl Pts',(-27.6946856803482,68.8405004465895,12.));
#97135=CARTESIAN_POINT('Ctrl Pts',(-27.6895716271084,68.8355891981877,12.));
#97136=CARTESIAN_POINT('Ctrl Pts',(-27.6804870323286,68.826859785198,12.));
#97137=CARTESIAN_POINT('Ctrl Pts',(-27.6674443909882,68.8143140938753,12.));
#97138=CARTESIAN_POINT('Ctrl Pts',(-27.6504626112621,68.7979550191773,12.));
#97139=CARTESIAN_POINT('Ctrl Pts',(-27.6306944192711,68.7788771464655,12.));
#97140=CARTESIAN_POINT('Ctrl Pts',(-27.6109689629025,68.7598059372121,12.));
#97141=CARTESIAN_POINT('Ctrl Pts',(-27.5912862705482,68.7407414755291,12.));
#97142=CARTESIAN_POINT('Ctrl Pts',(-27.5716463715027,68.721683850427,12.));
#97143=CARTESIAN_POINT('Ctrl Pts',(-27.552049295893,68.7026331554348,12.));
#97144=CARTESIAN_POINT('Ctrl Pts',(-27.5324950743723,68.683589486992,12.));
#97145=CARTESIAN_POINT('Ctrl Pts',(-27.5129837378798,68.6645529432059,12.));
#97146=CARTESIAN_POINT('Ctrl Pts',(-27.4935153173863,68.6455236225471,12.));
#97147=CARTESIAN_POINT('Ctrl Pts',(-27.4740898435977,68.6265016223536,12.));
#97148=CARTESIAN_POINT('Ctrl Pts',(-27.4547073468213,68.6074870381588,12.));
#97149=CARTESIAN_POINT('Ctrl Pts',(-27.4353678571349,68.5884799645193,12.));
#97150=CARTESIAN_POINT('Ctrl Pts',(-27.4160714044825,68.5694804955002,12.));
#97151=CARTESIAN_POINT('Ctrl Pts',(-27.3968180187941,68.5504887252976,12.));
#97152=CARTESIAN_POINT('Ctrl Pts',(-27.3776077300918,68.5315047488046,12.));
#97153=CARTESIAN_POINT('Ctrl Pts',(-27.3584405685947,68.5125286621902,12.));
#97154=CARTESIAN_POINT('Ctrl Pts',(-27.3393165646752,68.4935605626372,12.));
#97155=CARTESIAN_POINT('Ctrl Pts',(-27.3202357488154,68.4746005480997,12.));
#97156=CARTESIAN_POINT('Ctrl Pts',(-27.301198151557,68.4556487170441,12.));
#97157=CARTESIAN_POINT('Ctrl Pts',(-27.2822038034538,68.4367051682164,12.));
#97158=CARTESIAN_POINT('Ctrl Pts',(-27.263252735006,68.4177700003465,12.));
#97159=CARTESIAN_POINT('Ctrl Pts',(-27.244344976665,68.3988433121581,12.));
#97160=CARTESIAN_POINT('Ctrl Pts',(-27.2254805588673,68.3799252025102,12.));
#97161=CARTESIAN_POINT('Ctrl Pts',(-27.2066595120542,68.3610157704994,12.));
#97162=CARTESIAN_POINT('Ctrl Pts',(-27.1878818666926,68.3421151155711,12.));
#97163=CARTESIAN_POINT('Ctrl Pts',(-27.1691476532921,68.3232233376425,12.));
#97164=CARTESIAN_POINT('Ctrl Pts',(-27.1504569024136,68.3043405371603,12.));
#97165=CARTESIAN_POINT('Ctrl Pts',(-27.1318096446649,68.2854668150364,12.));
#97166=CARTESIAN_POINT('Ctrl Pts',(-27.1132059106943,68.2666022726104,12.));
#97167=CARTESIAN_POINT('Ctrl Pts',(-27.0946457311813,68.2477470116012,12.));
#97168=CARTESIAN_POINT('Ctrl Pts',(-27.0761291368226,68.2289011340615,12.));
#97169=CARTESIAN_POINT('Ctrl Pts',(-27.0576561583172,68.2100647423332,12.));
#97170=CARTESIAN_POINT('Ctrl Pts',(-27.0392268263798,68.1912379390773,12.));
#97171=CARTESIAN_POINT('Ctrl Pts',(-27.0208411717472,68.1724208272958,12.));
#97172=CARTESIAN_POINT('Ctrl Pts',(-27.0024992251838,68.1536135103557,12.));
#97173=CARTESIAN_POINT('Ctrl Pts',(-26.9842010174822,68.1348160920106,12.));
#97174=CARTESIAN_POINT('Ctrl Pts',(-26.9659465794601,68.1160286764255,12.));
#97175=CARTESIAN_POINT('Ctrl Pts',(-26.9477359419652,68.0972513681751,12.));
#97176=CARTESIAN_POINT('Ctrl Pts',(-26.9295691358779,68.0784842722369,12.));
#97177=CARTESIAN_POINT('Ctrl Pts',(-26.911446192111,68.0597274939859,12.));
#97178=CARTESIAN_POINT('Ctrl Pts',(-26.8933671416063,68.0409811391869,12.));
#97179=CARTESIAN_POINT('Ctrl Pts',(-26.8753320153252,68.0222453139856,12.));
#97180=CARTESIAN_POINT('Ctrl Pts',(-26.8573408442496,68.0035201249102,12.));
#97181=CARTESIAN_POINT('Ctrl Pts',(-26.8393936593911,67.9848056788809,12.));
#97182=CARTESIAN_POINT('Ctrl Pts',(-26.821490491792,67.9661020832164,12.));
#97183=CARTESIAN_POINT('Ctrl Pts',(-26.8036313725262,67.9474094456396,12.));
#97184=CARTESIAN_POINT('Ctrl Pts',(-26.7858163326934,67.928727874284,12.));
#97185=CARTESIAN_POINT('Ctrl Pts',(-26.7680454034169,67.9100574776972,12.));
#97186=CARTESIAN_POINT('Ctrl Pts',(-26.7503186158522,67.8913983648436,12.));
#97187=CARTESIAN_POINT('Ctrl Pts',(-26.7326360011885,67.8727506451063,12.));
#97188=CARTESIAN_POINT('Ctrl Pts',(-26.7149975906478,67.8541144282875,12.));
#97189=CARTESIAN_POINT('Ctrl Pts',(-26.6974034154804,67.8354898246086,12.));
#97190=CARTESIAN_POINT('Ctrl Pts',(-26.6798535069589,67.8168769447098,12.));
#97191=CARTESIAN_POINT('Ctrl Pts',(-26.6623478963871,67.798275899657,12.));
#97192=CARTESIAN_POINT('Ctrl Pts',(-26.6448866151029,67.7796868009455,12.));
#97193=CARTESIAN_POINT('Ctrl Pts',(-26.6274696944793,67.7611097605042,12.));
#97194=CARTESIAN_POINT('Ctrl Pts',(-26.6100971659202,67.7425448906977,12.));
#97195=CARTESIAN_POINT('Ctrl Pts',(-26.5927690608544,67.7239923043288,12.));
#97196=CARTESIAN_POINT('Ctrl Pts',(-26.5754854107421,67.7054521146424,12.));
#97197=CARTESIAN_POINT('Ctrl Pts',(-26.5582462470794,67.6869244353294,12.));
#97198=CARTESIAN_POINT('Ctrl Pts',(-26.5410516013985,67.6684093805291,12.));
#97199=CARTESIAN_POINT('Ctrl Pts',(-26.5239015052654,67.649907064832,12.));
#97200=CARTESIAN_POINT('Ctrl Pts',(-26.5067959902725,67.6314176032811,12.));
#97201=CARTESIAN_POINT('Ctrl Pts',(-26.489735088044,67.6129411113757,12.));
#97202=CARTESIAN_POINT('Ctrl Pts',(-26.4727188302409,67.5944777050768,12.));
#97203=CARTESIAN_POINT('Ctrl Pts',(-26.4557472485621,67.5760275008093,12.));
#97204=CARTESIAN_POINT('Ctrl Pts',(-26.4388203747425,67.5575906154657,12.));
#97205=CARTESIAN_POINT('Ctrl Pts',(-26.4219382405458,67.5391671664072,12.));
#97206=CARTESIAN_POINT('Ctrl Pts',(-26.4051008777675,67.5207572714683,12.));
#97207=CARTESIAN_POINT('Ctrl Pts',(-26.3883083182421,67.5023610489622,12.));
#97208=CARTESIAN_POINT('Ctrl Pts',(-26.3715605938433,67.4839786176836,12.));
#97209=CARTESIAN_POINT('Ctrl Pts',(-26.3548577364833,67.4656100969116,12.));
#97210=CARTESIAN_POINT('Ctrl Pts',(-26.3381997781055,67.4472556064119,12.));
#97211=CARTESIAN_POINT('Ctrl Pts',(-26.321586750686,67.4289152664398,12.));
#97212=CARTESIAN_POINT('Ctrl Pts',(-26.3050186862407,67.4105891977461,12.));
#97213=CARTESIAN_POINT('Ctrl Pts',(-26.288495616827,67.392277521581,12.));
#97214=CARTESIAN_POINT('Ctrl Pts',(-26.2720175745423,67.3739803596969,12.));
#97215=CARTESIAN_POINT('Ctrl Pts',(-26.255584591518,67.3556978343507,12.));
#97216=CARTESIAN_POINT('Ctrl Pts',(-26.2391966999191,67.3374300683073,12.));
#97217=CARTESIAN_POINT('Ctrl Pts',(-26.2228539319526,67.3191771848463,12.));
#97218=CARTESIAN_POINT('Ctrl Pts',(-26.2065563198683,67.3009393077651,12.));
#97219=CARTESIAN_POINT('Ctrl Pts',(-26.1903038959589,67.282716561383,12.));
#97220=CARTESIAN_POINT('Ctrl Pts',(-26.1740966925529,67.2645090705421,12.));
#97221=CARTESIAN_POINT('Ctrl Pts',(-26.1579347420138,67.2463169606115,12.));
#97222=CARTESIAN_POINT('Ctrl Pts',(-26.1418180767489,67.2281403574938,12.));
#97223=CARTESIAN_POINT('Ctrl Pts',(-26.1257467292102,67.2099793876297,12.));
#97224=CARTESIAN_POINT('Ctrl Pts',(-26.1097207318949,67.1918341780018,12.));
#97225=CARTESIAN_POINT('Ctrl Pts',(-26.0937401173383,67.173704856136,12.));
#97226=CARTESIAN_POINT('Ctrl Pts',(-26.0778049181128,67.1555915501049,12.));
#97227=CARTESIAN_POINT('Ctrl Pts',(-26.061915166836,67.1374943885354,12.));
#97228=CARTESIAN_POINT('Ctrl Pts',(-26.0460708961725,67.1194135006124,12.));
#97229=CARTESIAN_POINT('Ctrl Pts',(-26.030272138834,67.101349016084,12.));
#97230=CARTESIAN_POINT('Ctrl Pts',(-26.014518927573,67.0833010652634,12.));
#97231=CARTESIAN_POINT('Ctrl Pts',(-25.9988112951814,67.0652697790325,12.));
#97232=CARTESIAN_POINT('Ctrl Pts',(-25.9831492744984,67.0472552888485,12.));
#97233=CARTESIAN_POINT('Ctrl Pts',(-25.9675328984121,67.0292577267489,12.));
#97234=CARTESIAN_POINT('Ctrl Pts',(-25.9519621998598,67.0112772253556,12.));
#97235=CARTESIAN_POINT('Ctrl Pts',(-25.9364372118222,66.9933139178778,12.));
#97236=CARTESIAN_POINT('Ctrl Pts',(-25.9209579673209,66.975367938115,12.));
#97237=CARTESIAN_POINT('Ctrl Pts',(-25.9055244994277,66.9574394204663,12.));
#97238=CARTESIAN_POINT('Ctrl Pts',(-25.890136841266,66.939528499934,12.));
#97239=CARTESIAN_POINT('Ctrl Pts',(-25.8747950260111,66.92163531213,12.));
#97240=CARTESIAN_POINT('Ctrl Pts',(-25.8594990868833,66.9037599932761,12.));
#97241=CARTESIAN_POINT('Ctrl Pts',(-25.844249057147,66.8859026802088,12.));
#97242=CARTESIAN_POINT('Ctrl Pts',(-25.8290449701193,66.8680635103876,12.));
#97243=CARTESIAN_POINT('Ctrl Pts',(-25.8138868591709,66.8502426219001,12.));
#97244=CARTESIAN_POINT('Ctrl Pts',(-25.7987747577269,66.8324401534668,12.));
#97245=CARTESIAN_POINT('Ctrl Pts',(-25.7837086992595,66.8146562444433,12.));
#97246=CARTESIAN_POINT('Ctrl Pts',(-25.7686887172878,66.7968910348245,12.));
#97247=CARTESIAN_POINT('Ctrl Pts',(-25.7537148453864,66.7791446652545,12.));
#97248=CARTESIAN_POINT('Ctrl Pts',(-25.7387871171866,66.7614172770316,12.));
#97249=CARTESIAN_POINT('Ctrl Pts',(-25.7239055663772,66.7437090121153,12.));
#97250=CARTESIAN_POINT('Ctrl Pts',(-25.7090702266963,66.7260200131266,12.));
#97251=CARTESIAN_POINT('Ctrl Pts',(-25.6942811319322,66.7083504233529,12.));
#97252=CARTESIAN_POINT('Ctrl Pts',(-25.6795383159319,66.6907003867572,12.));
#97253=CARTESIAN_POINT('Ctrl Pts',(-25.6648418126013,66.6730700479837,12.));
#97254=CARTESIAN_POINT('Ctrl Pts',(-25.6501916559055,66.6554595523624,12.));
#97255=CARTESIAN_POINT('Ctrl Pts',(-25.6355878798614,66.6378690459129,12.));
#97256=CARTESIAN_POINT('Ctrl Pts',(-25.6210305185403,66.6202986753506,12.));
#97257=CARTESIAN_POINT('Ctrl Pts',(-25.6065196060756,66.6027485880963,12.));
#97258=CARTESIAN_POINT('Ctrl Pts',(-25.5920551766629,66.5852189322813,12.));
#97259=CARTESIAN_POINT('Ctrl Pts',(-25.5776372645601,66.5677098567542,12.));
#97260=CARTESIAN_POINT('Ctrl Pts',(-25.5632659040792,66.5502215110829,12.));
#97261=CARTESIAN_POINT('Ctrl Pts',(-25.5489411295912,66.5327540455624,12.));
#97262=CARTESIAN_POINT('Ctrl Pts',(-25.534662975532,66.5153076112231,12.));
#97263=CARTESIAN_POINT('Ctrl Pts',(-25.5204314764033,66.4978823598354,12.));
#97264=CARTESIAN_POINT('Ctrl Pts',(-25.5062466667702,66.4804784439148,12.));
#97265=CARTESIAN_POINT('Ctrl Pts',(-25.4921085812548,66.4630960167252,12.));
#97266=CARTESIAN_POINT('Ctrl Pts',(-25.4780172545417,66.4457352322871,12.));
#97267=CARTESIAN_POINT('Ctrl Pts',(-25.4639727213849,66.4283962453899,12.));
#97268=CARTESIAN_POINT('Ctrl Pts',(-25.4499750166079,66.4110792116,12.));
#97269=CARTESIAN_POINT('Ctrl Pts',(-25.4360241751018,66.3937842872685,12.));
#97270=CARTESIAN_POINT('Ctrl Pts',(-25.4221202318199,66.3765116295364,12.));
#97271=CARTESIAN_POINT('Ctrl Pts',(-25.4082632217847,66.359261396341,12.));
#97272=CARTESIAN_POINT('Ctrl Pts',(-25.3944531800901,66.3420337464178,12.));
#97273=CARTESIAN_POINT('Ctrl Pts',(-25.3806901419012,66.3248288393046,12.));
#97274=CARTESIAN_POINT('Ctrl Pts',(-25.3669741424488,66.3076468353412,12.));
#97275=CARTESIAN_POINT('Ctrl Pts',(-25.3533052170249,66.290487895671,12.));
#97276=CARTESIAN_POINT('Ctrl Pts',(-25.3396834009949,66.2733521822662,12.));
#97277=CARTESIAN_POINT('Ctrl Pts',(-25.3261087298026,66.2562398579471,12.));
#97278=CARTESIAN_POINT('Ctrl Pts',(-25.312581238973,66.2391510863998,12.));
#97279=CARTESIAN_POINT('Ctrl Pts',(-25.2991009641094,66.2220860321952,12.));
#97280=CARTESIAN_POINT('Ctrl Pts',(-25.285667940893,66.2050448607911,12.));
#97281=CARTESIAN_POINT('Ctrl Pts',(-25.2722822050837,66.1880277385136,12.));
#97282=CARTESIAN_POINT('Ctrl Pts',(-25.2589437925147,66.1710348325384,12.));
#97283=CARTESIAN_POINT('Ctrl Pts',(-25.2456527390875,66.1540663108754,12.));
#97284=CARTESIAN_POINT('Ctrl Pts',(-25.232409080755,66.1371223423345,12.));
#97285=CARTESIAN_POINT('Ctrl Pts',(-25.2192128535357,66.1202030965758,12.));
#97286=CARTESIAN_POINT('Ctrl Pts',(-25.2060640935365,66.10330874419,12.));
#97287=CARTESIAN_POINT('Ctrl Pts',(-25.1929628369685,66.086439456768,12.));
#97288=CARTESIAN_POINT('Ctrl Pts',(-25.1799091201599,66.0695954069713,12.));
#97289=CARTESIAN_POINT('Ctrl Pts',(-25.1669029795661,66.0527767686025,12.));
#97290=CARTESIAN_POINT('Ctrl Pts',(-25.1539444517419,66.0359837164734,12.));
#97291=CARTESIAN_POINT('Ctrl Pts',(-25.1410335733099,66.0192164262621,12.));
#97292=CARTESIAN_POINT('Ctrl Pts',(-25.1281703809297,66.0024750743897,12.));
#97293=CARTESIAN_POINT('Ctrl Pts',(-25.1153549112503,65.9857598378433,12.));
#97294=CARTESIAN_POINT('Ctrl Pts',(-25.1025872009004,65.9690708941558,12.));
#97295=CARTESIAN_POINT('Ctrl Pts',(-25.0898672865915,65.9524084218139,12.));
#97296=CARTESIAN_POINT('Ctrl Pts',(-25.0771952052028,65.9357726006163,12.));
#97297=CARTESIAN_POINT('Ctrl Pts',(-25.0645709938524,65.919163611981,12.));
#97298=CARTESIAN_POINT('Ctrl Pts',(-25.0519946900078,65.9025816394424,12.));
#97299=CARTESIAN_POINT('Ctrl Pts',(-25.0394663314055,65.8860268683128,12.));
#97300=CARTESIAN_POINT('Ctrl Pts',(-25.0269859558363,65.8694994847616,12.));
#97301=CARTESIAN_POINT('Ctrl Pts',(-25.0145536009604,65.8529996750445,12.));
#97302=CARTESIAN_POINT('Ctrl Pts',(-25.002169304117,65.8365276247128,12.));
#97303=CARTESIAN_POINT('Ctrl Pts',(-24.9898331020983,65.8200835177024,12.));
#97304=CARTESIAN_POINT('Ctrl Pts',(-24.9775450315683,65.8036675380718,12.));
#97305=CARTESIAN_POINT('Ctrl Pts',(-24.9653051295581,65.7872798720823,12.));
#97306=CARTESIAN_POINT('Ctrl Pts',(-24.9531134338696,65.7709207098959,12.));
#97307=CARTESIAN_POINT('Ctrl Pts',(-24.9409699836537,65.7545902480323,12.));
#97308=CARTESIAN_POINT('Ctrl Pts',(-24.928874819458,65.7382886895888,12.));
#97309=CARTESIAN_POINT('Ctrl Pts',(-24.9168279820106,65.7220162391053,12.));
#97310=CARTESIAN_POINT('Ctrl Pts',(-24.9048295111448,65.7057730980483,12.));
#97311=CARTESIAN_POINT('Ctrl Pts',(-24.8928794448607,65.6895594608775,12.));
#97312=CARTESIAN_POINT('Ctrl Pts',(-24.8809778178229,65.6733755087669,12.));
#97313=CARTESIAN_POINT('Ctrl Pts',(-24.8691246628057,65.6572214156692,12.));
#97314=CARTESIAN_POINT('Ctrl Pts',(-24.8573200135666,65.6410973603661,12.));
#97315=CARTESIAN_POINT('Ctrl Pts',(-24.8455639071517,65.6250035361612,12.));
#97316=CARTESIAN_POINT('Ctrl Pts',(-24.8338563866764,65.6089401625628,12.));
#97317=CARTESIAN_POINT('Ctrl Pts',(-24.8221975032104,65.5929074932624,12.));
#97318=CARTESIAN_POINT('Ctrl Pts',(-24.8105873098626,65.5769057914333,12.));
#97319=CARTESIAN_POINT('Ctrl Pts',(-24.799025856126,65.5609353062829,12.));
#97320=CARTESIAN_POINT('Ctrl Pts',(-24.7875131827491,65.5449962514661,12.));
#97321=CARTESIAN_POINT('Ctrl Pts',(-24.7760493148465,65.5290887770232,12.));
#97322=CARTESIAN_POINT('Ctrl Pts',(-24.7646342620841,65.5132129675333,12.));
#97323=CARTESIAN_POINT('Ctrl Pts',(-24.7555412724651,65.5005376841101,12.));
#97324=CARTESIAN_POINT('Ctrl Pts',(-24.7487434955982,65.4910454936254,12.));
#97325=CARTESIAN_POINT('Ctrl Pts',(-24.7442214063382,65.4847237095443,12.));
#97326=CARTESIAN_POINT('Ctrl Pts',(-24.7419628022042,65.4815644032299,12.));
#97327=CARTESIAN_POINT('Ctrl Pts',(-29.0944526440266,68.2622612910177,0.));
#97328=CARTESIAN_POINT('Ctrl Pts',(-29.0944526440266,68.2622612910177,4.));
#97329=CARTESIAN_POINT('Ctrl Pts',(-29.0944526440266,68.2622612910177,8.));
#97330=CARTESIAN_POINT('Ctrl Pts',(-29.0944526440266,68.2622612910177,12.));
#97331=CARTESIAN_POINT('Ctrl Pts',(-29.0922231502663,68.3721211369508,0.));
#97332=CARTESIAN_POINT('Ctrl Pts',(-29.0922231502663,68.3721211369508,4.));
#97333=CARTESIAN_POINT('Ctrl Pts',(-29.0922231502664,68.3721211369509,8.00000000000001));
#97334=CARTESIAN_POINT('Ctrl Pts',(-29.0922231502664,68.3721211369509,12.));
#97335=CARTESIAN_POINT('Ctrl Pts',(-29.0225207419381,68.5624216146675,0.));
#97336=CARTESIAN_POINT('Ctrl Pts',(-29.0225207419381,68.5624216146675,4.00000000000001));
#97337=CARTESIAN_POINT('Ctrl Pts',(-29.0225207419382,68.5624216146676,7.99999999999999));
#97338=CARTESIAN_POINT('Ctrl Pts',(-29.0225207419382,68.5624216146676,12.));
#97339=CARTESIAN_POINT('Ctrl Pts',(-28.8637726134455,68.6814343344131,0.));
#97340=CARTESIAN_POINT('Ctrl Pts',(-28.8637726134455,68.6814343344131,3.99999999999999));
#97341=CARTESIAN_POINT('Ctrl Pts',(-28.8637726134455,68.6814343344132,8.00000000000001));
#97342=CARTESIAN_POINT('Ctrl Pts',(-28.8637726134455,68.6814343344132,12.));
#97343=CARTESIAN_POINT('Ctrl Pts',(-28.7877620302417,68.7132793373318,0.));
#97344=CARTESIAN_POINT('Ctrl Pts',(-28.7877620302417,68.7132793373318,4.));
#97345=CARTESIAN_POINT('Ctrl Pts',(-28.7877620302417,68.7132793373319,8.));
#97346=CARTESIAN_POINT('Ctrl Pts',(-28.7877620302417,68.7132793373319,12.));
#97347=CARTESIAN_POINT('',(-29.0944526440266,68.2622612910177,0.));
#97348=CARTESIAN_POINT('',(-28.7877620302417,68.7132793373317,0.));
#97349=CARTESIAN_POINT('Ctrl Pts',(-29.0944526440266,68.2622612910177,0.));
#97350=CARTESIAN_POINT('Ctrl Pts',(-29.0922231502663,68.3721211369508,0.));
#97351=CARTESIAN_POINT('Ctrl Pts',(-29.0523932026502,68.4808642670747,0.));
#97352=CARTESIAN_POINT('Ctrl Pts',(-28.983487101511,68.5663297619426,0.));
#97353=CARTESIAN_POINT('Ctrl Pts',(-28.9318075256566,68.6304288830936,0.));
#97354=CARTESIAN_POINT('Ctrl Pts',(-28.8637726134455,68.6814343344131,0.));
#97355=CARTESIAN_POINT('Ctrl Pts',(-28.7877620302417,68.7132793373318,0.));
#97356=CARTESIAN_POINT('',(-28.7877620302417,68.7132793373317,12.));
#97357=CARTESIAN_POINT('Ctrl Pts',(-28.7877620302417,68.7132793373318,0.));
#97358=CARTESIAN_POINT('Ctrl Pts',(-28.7877620302417,68.7132793373318,4.));
#97359=CARTESIAN_POINT('Ctrl Pts',(-28.7877620302417,68.7132793373319,8.));
#97360=CARTESIAN_POINT('Ctrl Pts',(-28.7877620302417,68.7132793373319,12.));
#97361=CARTESIAN_POINT('',(-29.0944526440266,68.2622612910177,12.));
#97362=CARTESIAN_POINT('Ctrl Pts',(-28.7877620302417,68.7132793373319,12.));
#97363=CARTESIAN_POINT('Ctrl Pts',(-28.8637726134455,68.6814343344132,12.));
#97364=CARTESIAN_POINT('Ctrl Pts',(-28.9318075256567,68.6304288830936,12.));
#97365=CARTESIAN_POINT('Ctrl Pts',(-28.9834871015111,68.5663297619426,12.));
#97366=CARTESIAN_POINT('Ctrl Pts',(-29.0523932026503,68.4808642670747,12.));
#97367=CARTESIAN_POINT('Ctrl Pts',(-29.0922231502664,68.3721211369509,12.));
#97368=CARTESIAN_POINT('Ctrl Pts',(-29.0944526440266,68.2622612910177,12.));
#97369=CARTESIAN_POINT('Ctrl Pts',(-29.0944526440266,68.2622612910177,12.));
#97370=CARTESIAN_POINT('Ctrl Pts',(-29.0944526440266,68.2622612910177,8.));
#97371=CARTESIAN_POINT('Ctrl Pts',(-29.0944526440266,68.2622612910177,4.));
#97372=CARTESIAN_POINT('Ctrl Pts',(-29.0944526440266,68.2622612910177,0.));
#97373=CARTESIAN_POINT('Origin',(-1.43538201480493E-10,3.46272497684358E-10,
0.));
#97374=CARTESIAN_POINT('Origin',(-1.43538201480493E-10,3.46272497684358E-10,
12.));
#97375=CARTESIAN_POINT('Origin',(-1.43538201480493E-10,3.46272497684358E-10,
0.));
#97376=CARTESIAN_POINT('Ctrl Pts',(-22.1153394458717,71.1418425484881,0.));
#97377=CARTESIAN_POINT('Ctrl Pts',(-22.1153394458717,71.1418425484881,4.));
#97378=CARTESIAN_POINT('Ctrl Pts',(-22.1153394458717,71.1418425484881,8.));
#97379=CARTESIAN_POINT('Ctrl Pts',(-22.1153394458717,71.1418425484881,12.));
#97380=CARTESIAN_POINT('Ctrl Pts',(-22.0104100349463,71.1744611799059,0.));
#97381=CARTESIAN_POINT('Ctrl Pts',(-22.0104100349463,71.1744611799059,4.));
#97382=CARTESIAN_POINT('Ctrl Pts',(-22.0104100349463,71.1744611799059,8.));
#97383=CARTESIAN_POINT('Ctrl Pts',(-22.0104100349463,71.1744611799059,12.));
#97384=CARTESIAN_POINT('Ctrl Pts',(-21.8078334561031,71.1685011351939,0.));
#97385=CARTESIAN_POINT('Ctrl Pts',(-21.8078334561031,71.1685011351939,4.00000000000001));
#97386=CARTESIAN_POINT('Ctrl Pts',(-21.8078334561031,71.1685011351939,8.));
#97387=CARTESIAN_POINT('Ctrl Pts',(-21.8078334561031,71.1685011351939,12.));
#97388=CARTESIAN_POINT('Ctrl Pts',(-21.6447353227844,71.0555229320374,0.));
#97389=CARTESIAN_POINT('Ctrl Pts',(-21.6447353227844,71.0555229320374,4.));
#97390=CARTESIAN_POINT('Ctrl Pts',(-21.6447353227845,71.0555229320374,8.00000000000001));
#97391=CARTESIAN_POINT('Ctrl Pts',(-21.6447353227845,71.0555229320374,12.));
#97392=CARTESIAN_POINT('Ctrl Pts',(-21.5904919934804,70.9934796068773,0.));
#97393=CARTESIAN_POINT('Ctrl Pts',(-21.5904919934804,70.9934796068773,4.));
#97394=CARTESIAN_POINT('Ctrl Pts',(-21.5904919934805,70.9934796068772,8.));
#97395=CARTESIAN_POINT('Ctrl Pts',(-21.5904919934805,70.9934796068772,12.));
#97396=CARTESIAN_POINT('',(-22.1153394458717,71.1418425484881,0.));
#97397=CARTESIAN_POINT('',(-21.59049199348,70.9934796068777,0.));
#97398=CARTESIAN_POINT('Ctrl Pts',(-22.1153394458717,71.1418425484881,1.38777878078145E-16));
#97399=CARTESIAN_POINT('Ctrl Pts',(-22.0104100349463,71.1744611799059,1.38777878078144E-16));
#97400=CARTESIAN_POINT('Ctrl Pts',(-21.894651989893,71.1710554400705,1.38777878078145E-16));
#97401=CARTESIAN_POINT('Ctrl Pts',(-21.7917848658274,71.1327049954369,1.38777878078145E-16));
#97402=CARTESIAN_POINT('Ctrl Pts',(-21.7146345227781,71.1039421619616,1.38777878078145E-16));
#97403=CARTESIAN_POINT('Ctrl Pts',(-21.6447353227844,71.0555229320374,1.38777878078144E-16));
#97404=CARTESIAN_POINT('Ctrl Pts',(-21.5904919934804,70.9934796068773,1.38777878078145E-16));
#97405=CARTESIAN_POINT('',(-21.59049199348,70.9934796068777,12.));
#97406=CARTESIAN_POINT('Ctrl Pts',(-21.5904919934804,70.9934796068773,0.));
#97407=CARTESIAN_POINT('Ctrl Pts',(-21.5904919934804,70.9934796068773,4.));
#97408=CARTESIAN_POINT('Ctrl Pts',(-21.5904919934805,70.9934796068772,8.));
#97409=CARTESIAN_POINT('Ctrl Pts',(-21.5904919934805,70.9934796068772,12.));
#97410=CARTESIAN_POINT('',(-22.1153394458717,71.1418425484881,12.));
#97411=CARTESIAN_POINT('Ctrl Pts',(-21.5904919934805,70.9934796068772,12.));
#97412=CARTESIAN_POINT('Ctrl Pts',(-21.6447353227845,71.0555229320374,12.));
#97413=CARTESIAN_POINT('Ctrl Pts',(-21.7146345227782,71.1039421619616,12.));
#97414=CARTESIAN_POINT('Ctrl Pts',(-21.7917848658274,71.1327049954368,12.));
#97415=CARTESIAN_POINT('Ctrl Pts',(-21.894651989893,71.1710554400705,12.));
#97416=CARTESIAN_POINT('Ctrl Pts',(-22.0104100349463,71.1744611799059,12.));
#97417=CARTESIAN_POINT('Ctrl Pts',(-22.1153394458717,71.1418425484881,12.));
#97418=CARTESIAN_POINT('Ctrl Pts',(-22.1153394458717,71.1418425484881,12.));
#97419=CARTESIAN_POINT('Ctrl Pts',(-22.1153394458717,71.1418425484881,8.));
#97420=CARTESIAN_POINT('Ctrl Pts',(-22.1153394458717,71.1418425484881,4.));
#97421=CARTESIAN_POINT('Ctrl Pts',(-22.1153394458717,71.1418425484881,0.));
#97422=CARTESIAN_POINT('Ctrl Pts',(-18.9407177820969,67.3887914263118,0.));
#97423=CARTESIAN_POINT('Ctrl Pts',(-18.9407177820969,67.3887914263118,12.));
#97424=CARTESIAN_POINT('Ctrl Pts',(-18.9426924398719,67.3921355608328,0.));
#97425=CARTESIAN_POINT('Ctrl Pts',(-18.9426924398719,67.3921355608328,12.));
#97426=CARTESIAN_POINT('Ctrl Pts',(-18.9466463414299,67.3988274146651,0.));
#97427=CARTESIAN_POINT('Ctrl Pts',(-18.9466463414299,67.3988274146651,12.));
#97428=CARTESIAN_POINT('Ctrl Pts',(-18.9525909517915,67.4088759497911,0.));
#97429=CARTESIAN_POINT('Ctrl Pts',(-18.9525909517915,67.4088759497911,12.));
#97430=CARTESIAN_POINT('Ctrl Pts',(-18.9605446160985,67.4222955061981,0.));
#97431=CARTESIAN_POINT('Ctrl Pts',(-18.9605446160985,67.4222955061981,12.));
#97432=CARTESIAN_POINT('Ctrl Pts',(-18.9705325631711,67.4391057908418,0.));
#97433=CARTESIAN_POINT('Ctrl Pts',(-18.9705325631711,67.4391057908418,12.));
#97434=CARTESIAN_POINT('Ctrl Pts',(-18.9805663798448,67.4559518744638,0.));
#97435=CARTESIAN_POINT('Ctrl Pts',(-18.9805663798448,67.4559518744638,12.));
#97436=CARTESIAN_POINT('Ctrl Pts',(-18.9906460638625,67.472833671964,0.));
#97437=CARTESIAN_POINT('Ctrl Pts',(-18.9906460638625,67.472833671964,12.));
#97438=CARTESIAN_POINT('Ctrl Pts',(-19.0007716032819,67.4897510316844,0.));
#97439=CARTESIAN_POINT('Ctrl Pts',(-19.0007716032819,67.4897510316844,12.));
#97440=CARTESIAN_POINT('Ctrl Pts',(-19.0109429761306,67.5067037372317,0.));
#97441=CARTESIAN_POINT('Ctrl Pts',(-19.0109429761306,67.5067037372317,12.));
#97442=CARTESIAN_POINT('Ctrl Pts',(-19.021160154824,67.5236915360331,0.));
#97443=CARTESIAN_POINT('Ctrl Pts',(-19.021160154824,67.5236915360331,12.));
#97444=CARTESIAN_POINT('Ctrl Pts',(-19.0314231093923,67.540714161288,0.));
#97445=CARTESIAN_POINT('Ctrl Pts',(-19.0314231093923,67.540714161288,12.));
#97446=CARTESIAN_POINT('Ctrl Pts',(-19.0417318110708,67.5577713558194,0.));
#97447=CARTESIAN_POINT('Ctrl Pts',(-19.0417318110708,67.5577713558194,12.));
#97448=CARTESIAN_POINT('Ctrl Pts',(-19.0520862360396,67.5748628971964,0.));
#97449=CARTESIAN_POINT('Ctrl Pts',(-19.0520862360396,67.5748628971964,12.));
#97450=CARTESIAN_POINT('Ctrl Pts',(-19.062486364241,67.5919885896222,0.));
#97451=CARTESIAN_POINT('Ctrl Pts',(-19.062486364241,67.5919885896222,12.));
#97452=CARTESIAN_POINT('Ctrl Pts',(-19.072932177628,67.6091482520534,0.));
#97453=CARTESIAN_POINT('Ctrl Pts',(-19.072932177628,67.6091482520534,12.));
#97454=CARTESIAN_POINT('Ctrl Pts',(-19.0834236587118,67.6263417083426,0.));
#97455=CARTESIAN_POINT('Ctrl Pts',(-19.0834236587118,67.6263417083426,12.));
#97456=CARTESIAN_POINT('Ctrl Pts',(-19.0939607887501,67.6435687749841,0.));
#97457=CARTESIAN_POINT('Ctrl Pts',(-19.0939607887501,67.6435687749841,12.));
#97458=CARTESIAN_POINT('Ctrl Pts',(-19.1045435468358,67.6608292549462,0.));
#97459=CARTESIAN_POINT('Ctrl Pts',(-19.1045435468358,67.6608292549462,12.));
#97460=CARTESIAN_POINT('Ctrl Pts',(-19.115171910846,67.6781229440573,0.));
#97461=CARTESIAN_POINT('Ctrl Pts',(-19.115171910846,67.6781229440573,12.));
#97462=CARTESIAN_POINT('Ctrl Pts',(-19.1258458580345,67.6954496350063,0.));
#97463=CARTESIAN_POINT('Ctrl Pts',(-19.1258458580345,67.6954496350063,12.));
#97464=CARTESIAN_POINT('Ctrl Pts',(-19.136565365709,67.7128091219348,0.));
#97465=CARTESIAN_POINT('Ctrl Pts',(-19.136565365709,67.7128091219348,12.));
#97466=CARTESIAN_POINT('Ctrl Pts',(-19.1473304119955,67.7302012056584,0.));
#97467=CARTESIAN_POINT('Ctrl Pts',(-19.1473304119955,67.7302012056584,12.));
#97468=CARTESIAN_POINT('Ctrl Pts',(-19.1581409758097,67.7476256934444,0.));
#97469=CARTESIAN_POINT('Ctrl Pts',(-19.1581409758097,67.7476256934444,12.));
#97470=CARTESIAN_POINT('Ctrl Pts',(-19.168997036495,67.7650823965127,0.));
#97471=CARTESIAN_POINT('Ctrl Pts',(-19.168997036495,67.7650823965127,12.));
#97472=CARTESIAN_POINT('Ctrl Pts',(-19.1798985735688,67.7825711283096,0.));
#97473=CARTESIAN_POINT('Ctrl Pts',(-19.1798985735688,67.7825711283096,12.));
#97474=CARTESIAN_POINT('Ctrl Pts',(-19.1908455664098,67.8000917023926,0.));
#97475=CARTESIAN_POINT('Ctrl Pts',(-19.1908455664098,67.8000917023926,12.));
#97476=CARTESIAN_POINT('Ctrl Pts',(-19.201837993993,67.8176439306621,0.));
#97477=CARTESIAN_POINT('Ctrl Pts',(-19.201837993993,67.8176439306621,12.));
#97478=CARTESIAN_POINT('Ctrl Pts',(-19.2128758350346,67.835227624289,0.));
#97479=CARTESIAN_POINT('Ctrl Pts',(-19.2128758350346,67.835227624289,12.));
#97480=CARTESIAN_POINT('Ctrl Pts',(-19.2239590681133,67.8528425945184,0.));
#97481=CARTESIAN_POINT('Ctrl Pts',(-19.2239590681133,67.8528425945184,12.));
#97482=CARTESIAN_POINT('Ctrl Pts',(-19.2350876717874,67.8704886534544,0.));
#97483=CARTESIAN_POINT('Ctrl Pts',(-19.2350876717874,67.8704886534544,12.));
#97484=CARTESIAN_POINT('Ctrl Pts',(-19.2462616247279,67.8881656149955,0.));
#97485=CARTESIAN_POINT('Ctrl Pts',(-19.2462616247279,67.8881656149955,12.));
#97486=CARTESIAN_POINT('Ctrl Pts',(-19.2574809057696,67.9058732951788,0.));
#97487=CARTESIAN_POINT('Ctrl Pts',(-19.2574809057696,67.9058732951788,12.));
#97488=CARTESIAN_POINT('Ctrl Pts',(-19.2687454938442,67.9236115116758,0.));
#97489=CARTESIAN_POINT('Ctrl Pts',(-19.2687454938442,67.9236115116758,12.));
#97490=CARTESIAN_POINT('Ctrl Pts',(-19.280055367936,67.9413800834793,0.));
#97491=CARTESIAN_POINT('Ctrl Pts',(-19.280055367936,67.9413800834793,12.));
#97492=CARTESIAN_POINT('Ctrl Pts',(-19.2914105070286,67.9591788305394,0.));
#97493=CARTESIAN_POINT('Ctrl Pts',(-19.2914105070286,67.9591788305394,12.));
#97494=CARTESIAN_POINT('Ctrl Pts',(-19.302810890038,67.9770075733485,0.));
#97495=CARTESIAN_POINT('Ctrl Pts',(-19.302810890038,67.9770075733485,12.));
#97496=CARTESIAN_POINT('Ctrl Pts',(-19.3142564958203,67.9948661329617,0.));
#97497=CARTESIAN_POINT('Ctrl Pts',(-19.3142564958203,67.9948661329617,12.));
#97498=CARTESIAN_POINT('Ctrl Pts',(-19.3257473032034,68.0127543311776,0.));
#97499=CARTESIAN_POINT('Ctrl Pts',(-19.3257473032034,68.0127543311776,12.));
#97500=CARTESIAN_POINT('Ctrl Pts',(-19.3372832910076,68.0306719906636,0.));
#97501=CARTESIAN_POINT('Ctrl Pts',(-19.3372832910076,68.0306719906636,12.));
#97502=CARTESIAN_POINT('Ctrl Pts',(-19.3488644380641,68.0486189351011,0.));
#97503=CARTESIAN_POINT('Ctrl Pts',(-19.3488644380641,68.0486189351011,12.));
#97504=CARTESIAN_POINT('Ctrl Pts',(-19.3604907232314,68.0665949893195,0.));
#97505=CARTESIAN_POINT('Ctrl Pts',(-19.3604907232314,68.0665949893195,12.));
#97506=CARTESIAN_POINT('Ctrl Pts',(-19.3721621253912,68.0845999792247,0.));
#97507=CARTESIAN_POINT('Ctrl Pts',(-19.3721621253912,68.0845999792247,12.));
#97508=CARTESIAN_POINT('Ctrl Pts',(-19.3838786234421,68.1026337317285,0.));
#97509=CARTESIAN_POINT('Ctrl Pts',(-19.3838786234421,68.1026337317285,12.));
#97510=CARTESIAN_POINT('Ctrl Pts',(-19.3956401962895,68.1206960746769,0.));
#97511=CARTESIAN_POINT('Ctrl Pts',(-19.3956401962895,68.1206960746769,12.));
#97512=CARTESIAN_POINT('Ctrl Pts',(-19.40744682283,68.1387868367691,0.));
#97513=CARTESIAN_POINT('Ctrl Pts',(-19.40744682283,68.1387868367691,12.));
#97514=CARTESIAN_POINT('Ctrl Pts',(-19.4192984819418,68.1569058475054,0.));
#97515=CARTESIAN_POINT('Ctrl Pts',(-19.4192984819418,68.1569058475054,12.));
#97516=CARTESIAN_POINT('Ctrl Pts',(-19.4311951524983,68.1750529372232,0.));
#97517=CARTESIAN_POINT('Ctrl Pts',(-19.4311951524983,68.1750529372232,12.));
#97518=CARTESIAN_POINT('Ctrl Pts',(-19.4431368133719,68.1932279371127,0.));
#97519=CARTESIAN_POINT('Ctrl Pts',(-19.4431368133719,68.1932279371127,12.));
#97520=CARTESIAN_POINT('Ctrl Pts',(-19.455123443438,68.2114306792358,0.));
#97521=CARTESIAN_POINT('Ctrl Pts',(-19.455123443438,68.2114306792358,12.));
#97522=CARTESIAN_POINT('Ctrl Pts',(-19.467155021572,68.2296609965448,0.));
#97523=CARTESIAN_POINT('Ctrl Pts',(-19.467155021572,68.2296609965448,12.));
#97524=CARTESIAN_POINT('Ctrl Pts',(-19.4792315266501,68.2479187228803,0.));
#97525=CARTESIAN_POINT('Ctrl Pts',(-19.4792315266501,68.2479187228803,12.));
#97526=CARTESIAN_POINT('Ctrl Pts',(-19.4913529375543,68.2662036929526,0.));
#97527=CARTESIAN_POINT('Ctrl Pts',(-19.4913529375543,68.2662036929526,12.));
#97528=CARTESIAN_POINT('Ctrl Pts',(-19.5035192331705,68.2845157423233,0.));
#97529=CARTESIAN_POINT('Ctrl Pts',(-19.5035192331705,68.2845157423233,12.));
#97530=CARTESIAN_POINT('Ctrl Pts',(-19.5157303923856,68.3028547073864,0.));
#97531=CARTESIAN_POINT('Ctrl Pts',(-19.5157303923856,68.3028547073864,12.));
#97532=CARTESIAN_POINT('Ctrl Pts',(-19.5279863940773,68.3212204253417,0.));
#97533=CARTESIAN_POINT('Ctrl Pts',(-19.5279863940773,68.3212204253417,12.));
#97534=CARTESIAN_POINT('Ctrl Pts',(-19.5402872171191,68.3396127341938,0.));
#97535=CARTESIAN_POINT('Ctrl Pts',(-19.5402872171191,68.3396127341938,12.));
#97536=CARTESIAN_POINT('Ctrl Pts',(-19.5526328403852,68.3580314727523,0.));
#97537=CARTESIAN_POINT('Ctrl Pts',(-19.5526328403852,68.3580314727523,12.));
#97538=CARTESIAN_POINT('Ctrl Pts',(-19.5650232427516,68.3764764806287,0.));
#97539=CARTESIAN_POINT('Ctrl Pts',(-19.5650232427516,68.3764764806287,12.));
#97540=CARTESIAN_POINT('Ctrl Pts',(-19.5774584030938,68.3949475982335,0.));
#97541=CARTESIAN_POINT('Ctrl Pts',(-19.5774584030938,68.3949475982335,12.));
#97542=CARTESIAN_POINT('Ctrl Pts',(-19.5899383002802,68.4134446667696,0.));
#97543=CARTESIAN_POINT('Ctrl Pts',(-19.5899383002802,68.4134446667696,12.));
#97544=CARTESIAN_POINT('Ctrl Pts',(-19.6024629131785,68.4319675282275,0.));
#97545=CARTESIAN_POINT('Ctrl Pts',(-19.6024629131785,68.4319675282275,12.));
#97546=CARTESIAN_POINT('Ctrl Pts',(-19.6150322206577,68.4505160253778,0.));
#97547=CARTESIAN_POINT('Ctrl Pts',(-19.6150322206577,68.4505160253778,12.));
#97548=CARTESIAN_POINT('Ctrl Pts',(-19.6276462015888,68.4690900017632,0.));
#97549=CARTESIAN_POINT('Ctrl Pts',(-19.6276462015888,68.4690900017632,12.));
#97550=CARTESIAN_POINT('Ctrl Pts',(-19.6403048348395,68.4876893016856,0.));
#97551=CARTESIAN_POINT('Ctrl Pts',(-19.6403048348395,68.4876893016856,12.));
#97552=CARTESIAN_POINT('Ctrl Pts',(-19.6530080992686,68.5063137701971,0.));
#97553=CARTESIAN_POINT('Ctrl Pts',(-19.6530080992686,68.5063137701971,12.));
#97554=CARTESIAN_POINT('Ctrl Pts',(-19.6657559737336,68.5249632530979,0.));
#97555=CARTESIAN_POINT('Ctrl Pts',(-19.6657559737336,68.5249632530979,12.));
#97556=CARTESIAN_POINT('Ctrl Pts',(-19.6785484370927,68.5436375969311,0.));
#97557=CARTESIAN_POINT('Ctrl Pts',(-19.6785484370927,68.5436375969311,12.));
#97558=CARTESIAN_POINT('Ctrl Pts',(-19.6913854682046,68.5623366489779,0.));
#97559=CARTESIAN_POINT('Ctrl Pts',(-19.6913854682046,68.5623366489779,12.));
#97560=CARTESIAN_POINT('Ctrl Pts',(-19.7042670459237,68.581060257249,0.));
#97561=CARTESIAN_POINT('Ctrl Pts',(-19.7042670459237,68.581060257249,12.));
#97562=CARTESIAN_POINT('Ctrl Pts',(-19.7171931490956,68.5998082704766,0.));
#97563=CARTESIAN_POINT('Ctrl Pts',(-19.7171931490956,68.5998082704766,12.));
#97564=CARTESIAN_POINT('Ctrl Pts',(-19.7301637565652,68.6185805381126,0.));
#97565=CARTESIAN_POINT('Ctrl Pts',(-19.7301637565652,68.6185805381126,12.));
#97566=CARTESIAN_POINT('Ctrl Pts',(-19.7431788471776,68.6373769103224,0.));
#97567=CARTESIAN_POINT('Ctrl Pts',(-19.7431788471776,68.6373769103224,12.));
#97568=CARTESIAN_POINT('Ctrl Pts',(-19.7562383997781,68.6561972379793,0.));
#97569=CARTESIAN_POINT('Ctrl Pts',(-19.7562383997781,68.6561972379793,12.));
#97570=CARTESIAN_POINT('Ctrl Pts',(-19.7693423932058,68.6750413726547,0.));
#97571=CARTESIAN_POINT('Ctrl Pts',(-19.7693423932058,68.6750413726547,12.));
#97572=CARTESIAN_POINT('Ctrl Pts',(-19.7824908062913,68.6939091666111,0.));
#97573=CARTESIAN_POINT('Ctrl Pts',(-19.7824908062913,68.6939091666111,12.));
#97574=CARTESIAN_POINT('Ctrl Pts',(-19.795683617864,68.7128004727998,0.));
#97575=CARTESIAN_POINT('Ctrl Pts',(-19.795683617864,68.7128004727998,12.));
#97576=CARTESIAN_POINT('Ctrl Pts',(-19.8089208067532,68.7317151448557,0.));
#97577=CARTESIAN_POINT('Ctrl Pts',(-19.8089208067532,68.7317151448557,12.));
#97578=CARTESIAN_POINT('Ctrl Pts',(-19.8222023517874,68.7506530370918,0.));
#97579=CARTESIAN_POINT('Ctrl Pts',(-19.8222023517874,68.7506530370918,12.));
#97580=CARTESIAN_POINT('Ctrl Pts',(-19.835528231787,68.7696140044892,0.));
#97581=CARTESIAN_POINT('Ctrl Pts',(-19.835528231787,68.7696140044892,12.));
#97582=CARTESIAN_POINT('Ctrl Pts',(-19.8488984255641,68.7885979026927,0.));
#97583=CARTESIAN_POINT('Ctrl Pts',(-19.8488984255641,68.7885979026927,12.));
#97584=CARTESIAN_POINT('Ctrl Pts',(-19.8623129119304,68.8076045880102,0.));
#97585=CARTESIAN_POINT('Ctrl Pts',(-19.8623129119304,68.8076045880102,12.));
#97586=CARTESIAN_POINT('Ctrl Pts',(-19.8757716696969,68.8266339174068,0.));
#97587=CARTESIAN_POINT('Ctrl Pts',(-19.8757716696969,68.8266339174068,12.));
#97588=CARTESIAN_POINT('Ctrl Pts',(-19.8892746776734,68.8456857484988,0.));
#97589=CARTESIAN_POINT('Ctrl Pts',(-19.8892746776734,68.8456857484988,12.));
#97590=CARTESIAN_POINT('Ctrl Pts',(-19.9028219146607,68.8647599395437,0.));
#97591=CARTESIAN_POINT('Ctrl Pts',(-19.9028219146607,68.8647599395437,12.));
#97592=CARTESIAN_POINT('Ctrl Pts',(-19.9164133594513,68.8838563494356,0.));
#97593=CARTESIAN_POINT('Ctrl Pts',(-19.9164133594513,68.8838563494356,12.));
#97594=CARTESIAN_POINT('Ctrl Pts',(-19.9300489908364,68.902974837704,0.));
#97595=CARTESIAN_POINT('Ctrl Pts',(-19.9300489908364,68.902974837704,12.));
#97596=CARTESIAN_POINT('Ctrl Pts',(-19.9437287876063,68.9221152645086,0.));
#97597=CARTESIAN_POINT('Ctrl Pts',(-19.9437287876063,68.9221152645086,12.));
#97598=CARTESIAN_POINT('Ctrl Pts',(-19.9574527285492,68.9412774906346,0.));
#97599=CARTESIAN_POINT('Ctrl Pts',(-19.9574527285492,68.9412774906346,12.));
#97600=CARTESIAN_POINT('Ctrl Pts',(-19.9712207924437,68.960461377483,0.));
#97601=CARTESIAN_POINT('Ctrl Pts',(-19.9712207924437,68.960461377483,12.));
#97602=CARTESIAN_POINT('Ctrl Pts',(-19.98503295806,68.9796667870667,0.));
#97603=CARTESIAN_POINT('Ctrl Pts',(-19.98503295806,68.9796667870667,12.));
#97604=CARTESIAN_POINT('Ctrl Pts',(-19.9988892041671,68.9988935820101,0.));
#97605=CARTESIAN_POINT('Ctrl Pts',(-19.9988892041671,68.9988935820101,12.));
#97606=CARTESIAN_POINT('Ctrl Pts',(-20.0127895095327,69.0181416255433,0.));
#97607=CARTESIAN_POINT('Ctrl Pts',(-20.0127895095327,69.0181416255433,12.));
#97608=CARTESIAN_POINT('Ctrl Pts',(-20.0267338529221,69.0374107814977,0.));
#97609=CARTESIAN_POINT('Ctrl Pts',(-20.0267338529221,69.0374107814977,12.));
#97610=CARTESIAN_POINT('Ctrl Pts',(-20.0407222130902,69.0567009142968,0.));
#97611=CARTESIAN_POINT('Ctrl Pts',(-20.0407222130902,69.0567009142968,12.));
#97612=CARTESIAN_POINT('Ctrl Pts',(-20.0547545687839,69.0760118889525,0.));
#97613=CARTESIAN_POINT('Ctrl Pts',(-20.0547545687839,69.0760118889525,12.));
#97614=CARTESIAN_POINT('Ctrl Pts',(-20.0688308987478,69.0953435710634,0.));
#97615=CARTESIAN_POINT('Ctrl Pts',(-20.0688308987478,69.0953435710634,12.));
#97616=CARTESIAN_POINT('Ctrl Pts',(-20.082951181725,69.1146958268104,0.));
#97617=CARTESIAN_POINT('Ctrl Pts',(-20.082951181725,69.1146958268104,12.));
#97618=CARTESIAN_POINT('Ctrl Pts',(-20.0971153964557,69.1340685229516,0.));
#97619=CARTESIAN_POINT('Ctrl Pts',(-20.0971153964557,69.1340685229516,12.));
#97620=CARTESIAN_POINT('Ctrl Pts',(-20.1113235216694,69.1534615268153,0.));
#97621=CARTESIAN_POINT('Ctrl Pts',(-20.1113235216694,69.1534615268153,12.));
#97622=CARTESIAN_POINT('Ctrl Pts',(-20.1255755360871,69.172874706296,0.));
#97623=CARTESIAN_POINT('Ctrl Pts',(-20.1255755360871,69.172874706296,12.));
#97624=CARTESIAN_POINT('Ctrl Pts',(-20.1398714184278,69.1923079298534,0.));
#97625=CARTESIAN_POINT('Ctrl Pts',(-20.1398714184278,69.1923079298534,12.));
#97626=CARTESIAN_POINT('Ctrl Pts',(-20.1542111474086,69.2117610665073,0.));
#97627=CARTESIAN_POINT('Ctrl Pts',(-20.1542111474086,69.2117610665073,12.));
#97628=CARTESIAN_POINT('Ctrl Pts',(-20.1685947017433,69.2312339858337,0.));
#97629=CARTESIAN_POINT('Ctrl Pts',(-20.1685947017433,69.2312339858337,12.));
#97630=CARTESIAN_POINT('Ctrl Pts',(-20.183022060135,69.2507265579562,0.));
#97631=CARTESIAN_POINT('Ctrl Pts',(-20.183022060135,69.2507265579562,12.));
#97632=CARTESIAN_POINT('Ctrl Pts',(-20.1974932012775,69.2702386535432,0.));
#97633=CARTESIAN_POINT('Ctrl Pts',(-20.1974932012775,69.2702386535432,12.));
#97634=CARTESIAN_POINT('Ctrl Pts',(-20.2120081038622,69.2897701438066,0.));
#97635=CARTESIAN_POINT('Ctrl Pts',(-20.2120081038622,69.2897701438066,12.));
#97636=CARTESIAN_POINT('Ctrl Pts',(-20.2265667465784,69.3093209004986,0.));
#97637=CARTESIAN_POINT('Ctrl Pts',(-20.2265667465784,69.3093209004986,12.));
#97638=CARTESIAN_POINT('Ctrl Pts',(-20.2411691081122,69.3288907959065,0.));
#97639=CARTESIAN_POINT('Ctrl Pts',(-20.2411691081122,69.3288907959065,12.));
#97640=CARTESIAN_POINT('Ctrl Pts',(-20.255815167139,69.3484797028454,0.));
#97641=CARTESIAN_POINT('Ctrl Pts',(-20.255815167139,69.3484797028454,12.));
#97642=CARTESIAN_POINT('Ctrl Pts',(-20.2705049023241,69.3680874946548,0.));
#97643=CARTESIAN_POINT('Ctrl Pts',(-20.2705049023241,69.3680874946548,12.));
#97644=CARTESIAN_POINT('Ctrl Pts',(-20.2852382923299,69.3877140451975,0.));
#97645=CARTESIAN_POINT('Ctrl Pts',(-20.2852382923299,69.3877140451975,12.));
#97646=CARTESIAN_POINT('Ctrl Pts',(-20.3000153158167,69.4073592288562,0.));
#97647=CARTESIAN_POINT('Ctrl Pts',(-20.3000153158167,69.4073592288562,12.));
#97648=CARTESIAN_POINT('Ctrl Pts',(-20.3148359514414,69.4270229205296,0.));
#97649=CARTESIAN_POINT('Ctrl Pts',(-20.3148359514414,69.4270229205296,12.));
#97650=CARTESIAN_POINT('Ctrl Pts',(-20.3297001778505,69.4467049956257,0.));
#97651=CARTESIAN_POINT('Ctrl Pts',(-20.3297001778505,69.4467049956257,12.));
#97652=CARTESIAN_POINT('Ctrl Pts',(-20.3446079736799,69.4664053300579,0.));
#97653=CARTESIAN_POINT('Ctrl Pts',(-20.3446079736799,69.4664053300579,12.));
#97654=CARTESIAN_POINT('Ctrl Pts',(-20.3595593175619,69.4861238002433,0.));
#97655=CARTESIAN_POINT('Ctrl Pts',(-20.3595593175619,69.4861238002433,12.));
#97656=CARTESIAN_POINT('Ctrl Pts',(-20.3745541881266,69.5058602831004,0.));
#97657=CARTESIAN_POINT('Ctrl Pts',(-20.3745541881266,69.5058602831004,12.));
#97658=CARTESIAN_POINT('Ctrl Pts',(-20.3895925640006,69.5256146560444,0.));
#97659=CARTESIAN_POINT('Ctrl Pts',(-20.3895925640006,69.5256146560444,12.));
#97660=CARTESIAN_POINT('Ctrl Pts',(-20.4046744238002,69.5453867969815,0.));
#97661=CARTESIAN_POINT('Ctrl Pts',(-20.4046744238002,69.5453867969815,12.));
#97662=CARTESIAN_POINT('Ctrl Pts',(-20.4197997461305,69.565176584305,0.));
#97663=CARTESIAN_POINT('Ctrl Pts',(-20.4197997461305,69.565176584305,12.));
#97664=CARTESIAN_POINT('Ctrl Pts',(-20.4349685095928,69.5849838968944,0.));
#97665=CARTESIAN_POINT('Ctrl Pts',(-20.4349685095928,69.5849838968944,12.));
#97666=CARTESIAN_POINT('Ctrl Pts',(-20.4501806927854,69.6048086141122,0.));
#97667=CARTESIAN_POINT('Ctrl Pts',(-20.4501806927854,69.6048086141122,12.));
#97668=CARTESIAN_POINT('Ctrl Pts',(-20.4654362743036,69.6246506158009,0.));
#97669=CARTESIAN_POINT('Ctrl Pts',(-20.4654362743036,69.6246506158009,12.));
#97670=CARTESIAN_POINT('Ctrl Pts',(-20.4807352327335,69.6445097822778,0.));
#97671=CARTESIAN_POINT('Ctrl Pts',(-20.4807352327335,69.6445097822778,12.));
#97672=CARTESIAN_POINT('Ctrl Pts',(-20.4960775466487,69.6643859943291,0.));
#97673=CARTESIAN_POINT('Ctrl Pts',(-20.4960775466487,69.6643859943291,12.));
#97674=CARTESIAN_POINT('Ctrl Pts',(-20.511463194618,69.6842791332102,0.));
#97675=CARTESIAN_POINT('Ctrl Pts',(-20.511463194618,69.6842791332102,12.));
#97676=CARTESIAN_POINT('Ctrl Pts',(-20.5268921552075,69.7041890806421,0.));
#97677=CARTESIAN_POINT('Ctrl Pts',(-20.5268921552075,69.7041890806421,12.));
#97678=CARTESIAN_POINT('Ctrl Pts',(-20.54236440698,69.7241157188086,0.));
#97679=CARTESIAN_POINT('Ctrl Pts',(-20.54236440698,69.7241157188086,12.));
#97680=CARTESIAN_POINT('Ctrl Pts',(-20.5578799284898,69.7440589303511,0.));
#97681=CARTESIAN_POINT('Ctrl Pts',(-20.5578799284898,69.7440589303511,12.));
#97682=CARTESIAN_POINT('Ctrl Pts',(-20.5734386982781,69.7640185983641,0.));
#97683=CARTESIAN_POINT('Ctrl Pts',(-20.5734386982781,69.7640185983641,12.));
#97684=CARTESIAN_POINT('Ctrl Pts',(-20.5890406948809,69.7839946063942,0.));
#97685=CARTESIAN_POINT('Ctrl Pts',(-20.5890406948809,69.7839946063942,12.));
#97686=CARTESIAN_POINT('Ctrl Pts',(-20.6046858968305,69.8039868384382,0.));
#97687=CARTESIAN_POINT('Ctrl Pts',(-20.6046858968305,69.8039868384382,12.));
#97688=CARTESIAN_POINT('Ctrl Pts',(-20.6203742826566,69.8239951789402,0.));
#97689=CARTESIAN_POINT('Ctrl Pts',(-20.6203742826566,69.8239951789402,12.));
#97690=CARTESIAN_POINT('Ctrl Pts',(-20.6361058308812,69.8440195127874,0.));
#97691=CARTESIAN_POINT('Ctrl Pts',(-20.6361058308812,69.8440195127874,12.));
#97692=CARTESIAN_POINT('Ctrl Pts',(-20.6518805200132,69.8640597253058,0.));
#97693=CARTESIAN_POINT('Ctrl Pts',(-20.6518805200132,69.8640597253058,12.));
#97694=CARTESIAN_POINT('Ctrl Pts',(-20.6676983285542,69.884115702258,0.));
#97695=CARTESIAN_POINT('Ctrl Pts',(-20.6676983285542,69.884115702258,12.));
#97696=CARTESIAN_POINT('Ctrl Pts',(-20.6835592350031,69.9041873298416,0.));
#97697=CARTESIAN_POINT('Ctrl Pts',(-20.6835592350031,69.9041873298416,12.));
#97698=CARTESIAN_POINT('Ctrl Pts',(-20.6994632178551,69.9242744946854,0.));
#97699=CARTESIAN_POINT('Ctrl Pts',(-20.6994632178551,69.9242744946854,12.));
#97700=CARTESIAN_POINT('Ctrl Pts',(-20.7154102555996,69.9443770838444,0.));
#97701=CARTESIAN_POINT('Ctrl Pts',(-20.7154102555996,69.9443770838444,12.));
#97702=CARTESIAN_POINT('Ctrl Pts',(-20.7314003267118,69.9644949847929,0.));
#97703=CARTESIAN_POINT('Ctrl Pts',(-20.7314003267118,69.9644949847929,12.));
#97704=CARTESIAN_POINT('Ctrl Pts',(-20.7474334096581,69.9846280854254,0.));
#97705=CARTESIAN_POINT('Ctrl Pts',(-20.7474334096581,69.9846280854254,12.));
#97706=CARTESIAN_POINT('Ctrl Pts',(-20.7635094829016,70.0047762740569,0.));
#97707=CARTESIAN_POINT('Ctrl Pts',(-20.7635094829016,70.0047762740569,12.));
#97708=CARTESIAN_POINT('Ctrl Pts',(-20.7796285249023,70.0249394394221,0.));
#97709=CARTESIAN_POINT('Ctrl Pts',(-20.7796285249023,70.0249394394221,12.));
#97710=CARTESIAN_POINT('Ctrl Pts',(-20.7957905141155,70.0451174706739,0.));
#97711=CARTESIAN_POINT('Ctrl Pts',(-20.7957905141155,70.0451174706739,12.));
#97712=CARTESIAN_POINT('Ctrl Pts',(-20.8119954289845,70.0653102573798,0.));
#97713=CARTESIAN_POINT('Ctrl Pts',(-20.8119954289845,70.0653102573798,12.));
#97714=CARTESIAN_POINT('Ctrl Pts',(-20.8282432479425,70.0855176895185,0.));
#97715=CARTESIAN_POINT('Ctrl Pts',(-20.8282432479425,70.0855176895185,12.));
#97716=CARTESIAN_POINT('Ctrl Pts',(-20.8445339494184,70.1057396574741,0.));
#97717=CARTESIAN_POINT('Ctrl Pts',(-20.8445339494184,70.1057396574741,12.));
#97718=CARTESIAN_POINT('Ctrl Pts',(-20.8608675118377,70.1259760520306,0.));
#97719=CARTESIAN_POINT('Ctrl Pts',(-20.8608675118377,70.1259760520306,12.));
#97720=CARTESIAN_POINT('Ctrl Pts',(-20.8772439136207,70.1462267643649,0.));
#97721=CARTESIAN_POINT('Ctrl Pts',(-20.8772439136207,70.1462267643649,12.));
#97722=CARTESIAN_POINT('Ctrl Pts',(-20.8936631331751,70.1664916860366,0.));
#97723=CARTESIAN_POINT('Ctrl Pts',(-20.8936631331751,70.1664916860366,12.));
#97724=CARTESIAN_POINT('Ctrl Pts',(-20.9101251488948,70.1867707089866,0.));
#97725=CARTESIAN_POINT('Ctrl Pts',(-20.9101251488948,70.1867707089866,12.));
#97726=CARTESIAN_POINT('Ctrl Pts',(-20.9266299391688,70.2070637255469,0.));
#97727=CARTESIAN_POINT('Ctrl Pts',(-20.9266299391688,70.2070637255469,12.));
#97728=CARTESIAN_POINT('Ctrl Pts',(-20.9431774823833,70.2273706284479,0.));
#97729=CARTESIAN_POINT('Ctrl Pts',(-20.9431774823833,70.2273706284479,12.));
#97730=CARTESIAN_POINT('Ctrl Pts',(-20.9597677569227,70.2476913108242,0.));
#97731=CARTESIAN_POINT('Ctrl Pts',(-20.9597677569227,70.2476913108242,12.));
#97732=CARTESIAN_POINT('Ctrl Pts',(-20.9764007411648,70.2680256662215,0.));
#97733=CARTESIAN_POINT('Ctrl Pts',(-20.9764007411648,70.2680256662215,12.));
#97734=CARTESIAN_POINT('Ctrl Pts',(-20.993076413477,70.288373588597,0.));
#97735=CARTESIAN_POINT('Ctrl Pts',(-20.993076413477,70.288373588597,12.));
#97736=CARTESIAN_POINT('Ctrl Pts',(-21.0097947522212,70.3087349722959,0.));
#97737=CARTESIAN_POINT('Ctrl Pts',(-21.0097947522212,70.3087349722959,12.));
#97738=CARTESIAN_POINT('Ctrl Pts',(-21.0265557357544,70.3291097120293,0.));
#97739=CARTESIAN_POINT('Ctrl Pts',(-21.0265557357544,70.3291097120293,12.));
#97740=CARTESIAN_POINT('Ctrl Pts',(-21.0433593424266,70.3494977028497,0.));
#97741=CARTESIAN_POINT('Ctrl Pts',(-21.0433593424266,70.3494977028497,12.));
#97742=CARTESIAN_POINT('Ctrl Pts',(-21.0602055505751,70.3698988401291,0.));
#97743=CARTESIAN_POINT('Ctrl Pts',(-21.0602055505751,70.3698988401291,12.));
#97744=CARTESIAN_POINT('Ctrl Pts',(-21.0770943385146,70.3903130195279,0.));
#97745=CARTESIAN_POINT('Ctrl Pts',(-21.0770943385146,70.3903130195279,12.));
#97746=CARTESIAN_POINT('Ctrl Pts',(-21.0940256845477,70.4107401370403,0.));
#97747=CARTESIAN_POINT('Ctrl Pts',(-21.0940256845477,70.4107401370403,12.));
#97748=CARTESIAN_POINT('Ctrl Pts',(-21.110999566975,70.4311800890411,0.));
#97749=CARTESIAN_POINT('Ctrl Pts',(-21.110999566975,70.4311800890411,12.));
#97750=CARTESIAN_POINT('Ctrl Pts',(-21.1280159641003,70.4516327723349,0.));
#97751=CARTESIAN_POINT('Ctrl Pts',(-21.1280159641003,70.4516327723349,12.));
#97752=CARTESIAN_POINT('Ctrl Pts',(-21.1450748542335,70.4720980841934,0.));
#97753=CARTESIAN_POINT('Ctrl Pts',(-21.1450748542335,70.4720980841934,12.));
#97754=CARTESIAN_POINT('Ctrl Pts',(-21.1621762156894,70.4925759224208,0.));
#97755=CARTESIAN_POINT('Ctrl Pts',(-21.1621762156894,70.4925759224208,12.));
#97756=CARTESIAN_POINT('Ctrl Pts',(-21.1793200267843,70.5130661852946,0.));
#97757=CARTESIAN_POINT('Ctrl Pts',(-21.1793200267843,70.5130661852946,12.));
#97758=CARTESIAN_POINT('Ctrl Pts',(-21.1965062658296,70.5335687714422,0.));
#97759=CARTESIAN_POINT('Ctrl Pts',(-21.1965062658296,70.5335687714422,12.));
#97760=CARTESIAN_POINT('Ctrl Pts',(-21.2137349111207,70.5540835797281,0.));
#97761=CARTESIAN_POINT('Ctrl Pts',(-21.2137349111207,70.5540835797281,12.));
#97762=CARTESIAN_POINT('Ctrl Pts',(-21.2310059409265,70.5746105091503,0.));
#97763=CARTESIAN_POINT('Ctrl Pts',(-21.2310059409265,70.5746105091503,12.));
#97764=CARTESIAN_POINT('Ctrl Pts',(-21.2483193334676,70.5951494586961,0.));
#97765=CARTESIAN_POINT('Ctrl Pts',(-21.2483193334676,70.5951494586961,12.));
#97766=CARTESIAN_POINT('Ctrl Pts',(-21.2656750669129,70.6157003273326,0.));
#97767=CARTESIAN_POINT('Ctrl Pts',(-21.2656750669129,70.6157003273326,12.));
#97768=CARTESIAN_POINT('Ctrl Pts',(-21.2830731194187,70.6362630143062,0.));
#97769=CARTESIAN_POINT('Ctrl Pts',(-21.2830731194187,70.6362630143062,12.));
#97770=CARTESIAN_POINT('Ctrl Pts',(-21.3005134691563,70.6568374193786,0.));
#97771=CARTESIAN_POINT('Ctrl Pts',(-21.3005134691563,70.6568374193786,12.));
#97772=CARTESIAN_POINT('Ctrl Pts',(-21.3179960943388,70.6774234430899,0.));
#97773=CARTESIAN_POINT('Ctrl Pts',(-21.3179960943388,70.6774234430899,12.));
#97774=CARTESIAN_POINT('Ctrl Pts',(-21.3355209732438,70.6980209870032,0.));
#97775=CARTESIAN_POINT('Ctrl Pts',(-21.3355209732438,70.6980209870032,12.));
#97776=CARTESIAN_POINT('Ctrl Pts',(-21.353088084234,70.7186299539698,0.));
#97777=CARTESIAN_POINT('Ctrl Pts',(-21.353088084234,70.7186299539698,12.));
#97778=CARTESIAN_POINT('Ctrl Pts',(-21.3706974057028,70.7392502475438,0.));
#97779=CARTESIAN_POINT('Ctrl Pts',(-21.3706974057028,70.7392502475438,12.));
#97780=CARTESIAN_POINT('Ctrl Pts',(-21.3883489160187,70.7598817714078,0.));
#97781=CARTESIAN_POINT('Ctrl Pts',(-21.3883489160187,70.7598817714078,12.));
#97782=CARTESIAN_POINT('Ctrl Pts',(-21.4060425934595,70.780524428744,0.));
#97783=CARTESIAN_POINT('Ctrl Pts',(-21.4060425934595,70.780524428744,12.));
#97784=CARTESIAN_POINT('Ctrl Pts',(-21.4237784161592,70.8011781217409,0.));
#97785=CARTESIAN_POINT('Ctrl Pts',(-21.4237784161592,70.8011781217409,12.));
#97786=CARTESIAN_POINT('Ctrl Pts',(-21.4415563620127,70.8218427507545,0.));
#97787=CARTESIAN_POINT('Ctrl Pts',(-21.4415563620127,70.8218427507545,12.));
#97788=CARTESIAN_POINT('Ctrl Pts',(-21.4593764087492,70.84251821499,0.));
#97789=CARTESIAN_POINT('Ctrl Pts',(-21.4593764087492,70.84251821499,12.));
#97790=CARTESIAN_POINT('Ctrl Pts',(-21.4772385340978,70.8632044140166,0.));
#97791=CARTESIAN_POINT('Ctrl Pts',(-21.4772385340978,70.8632044140166,12.));
#97792=CARTESIAN_POINT('Ctrl Pts',(-21.4951427159272,70.8839012490903,0.));
#97793=CARTESIAN_POINT('Ctrl Pts',(-21.4951427159272,70.8839012490903,12.));
#97794=CARTESIAN_POINT('Ctrl Pts',(-21.5130889323767,70.9046086244123,0.));
#97795=CARTESIAN_POINT('Ctrl Pts',(-21.5130889323767,70.9046086244123,12.));
#97796=CARTESIAN_POINT('Ctrl Pts',(-21.5310771620209,70.9253264487576,0.));
#97797=CARTESIAN_POINT('Ctrl Pts',(-21.5310771620209,70.9253264487576,12.));
#97798=CARTESIAN_POINT('Ctrl Pts',(-21.549107383907,70.9460546358597,0.));
#97799=CARTESIAN_POINT('Ctrl Pts',(-21.549107383907,70.9460546358597,12.));
#97800=CARTESIAN_POINT('Ctrl Pts',(-21.5671795771873,70.9667931008097,0.));
#97801=CARTESIAN_POINT('Ctrl Pts',(-21.5671795771873,70.9667931008097,12.));
#97802=CARTESIAN_POINT('Ctrl Pts',(-21.5852937208258,70.9875417572138,0.));
#97803=CARTESIAN_POINT('Ctrl Pts',(-21.5852937208258,70.9875417572138,12.));
#97804=CARTESIAN_POINT('Ctrl Pts',(-21.6034497932573,71.0083005139086,0.));
#97805=CARTESIAN_POINT('Ctrl Pts',(-21.6034497932573,71.0083005139086,12.));
#97806=CARTESIAN_POINT('Ctrl Pts',(-21.6216477720941,71.0290692721932,0.));
#97807=CARTESIAN_POINT('Ctrl Pts',(-21.6216477720941,71.0290692721932,12.));
#97808=CARTESIAN_POINT('Ctrl Pts',(-21.6398876337207,71.0498479219659,0.));
#97809=CARTESIAN_POINT('Ctrl Pts',(-21.6398876337207,71.0498479219659,12.));
#97810=CARTESIAN_POINT('Ctrl Pts',(-21.6581693538424,71.0706363472965,0.));
#97811=CARTESIAN_POINT('Ctrl Pts',(-21.6581693538424,71.0706363472965,12.));
#97812=CARTESIAN_POINT('Ctrl Pts',(-21.6764929081762,71.0914344333048,0.));
#97813=CARTESIAN_POINT('Ctrl Pts',(-21.6764929081762,71.0914344333048,12.));
#97814=CARTESIAN_POINT('Ctrl Pts',(-21.6948582730895,71.1122420728349,0.));
#97815=CARTESIAN_POINT('Ctrl Pts',(-21.6948582730895,71.1122420728349,12.));
#97816=CARTESIAN_POINT('Ctrl Pts',(-21.7132654262501,71.133059172642,0.));
#97817=CARTESIAN_POINT('Ctrl Pts',(-21.7132654262501,71.133059172642,12.));
#97818=CARTESIAN_POINT('Ctrl Pts',(-21.7317143472827,71.1538856611899,0.));
#97819=CARTESIAN_POINT('Ctrl Pts',(-21.7317143472827,71.1538856611899,12.));
#97820=CARTESIAN_POINT('Ctrl Pts',(-21.7502050183602,71.1747214905981,0.));
#97821=CARTESIAN_POINT('Ctrl Pts',(-21.7502050183602,71.1747214905981,12.));
#97822=CARTESIAN_POINT('Ctrl Pts',(-21.7687374247045,71.1955666309591,0.));
#97823=CARTESIAN_POINT('Ctrl Pts',(-21.7687374247045,71.1955666309591,12.));
#97824=CARTESIAN_POINT('Ctrl Pts',(-21.7835967290261,71.212250179455,0.));
#97825=CARTESIAN_POINT('Ctrl Pts',(-21.7835967290261,71.212250179455,12.));
#97826=CARTESIAN_POINT('Ctrl Pts',(-21.7947599798839,71.2247670209821,0.));
#97827=CARTESIAN_POINT('Ctrl Pts',(-21.7947599798839,71.2247670209821,12.));
#97828=CARTESIAN_POINT('Ctrl Pts',(-21.8022104901682,71.2331134397743,0.));
#97829=CARTESIAN_POINT('Ctrl Pts',(-21.8022104901682,71.2331134397743,12.));
#97830=CARTESIAN_POINT('Ctrl Pts',(-21.8059378310719,71.2372871136137,0.));
#97831=CARTESIAN_POINT('Ctrl Pts',(-21.8059378310719,71.2372871136137,12.));
#97832=CARTESIAN_POINT('',(-18.9407177820969,67.3887914263118,0.));
#97833=CARTESIAN_POINT('Ctrl Pts',(-18.9407177820969,67.3887914263118,0.));
#97834=CARTESIAN_POINT('Ctrl Pts',(-18.9426924398719,67.3921355608328,0.));
#97835=CARTESIAN_POINT('Ctrl Pts',(-18.9466463414299,67.3988274146651,0.));
#97836=CARTESIAN_POINT('Ctrl Pts',(-18.9525909517915,67.4088759497911,0.));
#97837=CARTESIAN_POINT('Ctrl Pts',(-18.9605446160985,67.4222955061981,0.));
#97838=CARTESIAN_POINT('Ctrl Pts',(-18.9705325631711,67.4391057908418,0.));
#97839=CARTESIAN_POINT('Ctrl Pts',(-18.9805663798448,67.4559518744638,0.));
#97840=CARTESIAN_POINT('Ctrl Pts',(-18.9906460638625,67.472833671964,0.));
#97841=CARTESIAN_POINT('Ctrl Pts',(-19.0007716032819,67.4897510316844,0.));
#97842=CARTESIAN_POINT('Ctrl Pts',(-19.0109429761306,67.5067037372317,0.));
#97843=CARTESIAN_POINT('Ctrl Pts',(-19.021160154824,67.5236915360331,0.));
#97844=CARTESIAN_POINT('Ctrl Pts',(-19.0314231093923,67.540714161288,0.));
#97845=CARTESIAN_POINT('Ctrl Pts',(-19.0417318110708,67.5577713558194,0.));
#97846=CARTESIAN_POINT('Ctrl Pts',(-19.0520862360396,67.5748628971964,0.));
#97847=CARTESIAN_POINT('Ctrl Pts',(-19.062486364241,67.5919885896222,0.));
#97848=CARTESIAN_POINT('Ctrl Pts',(-19.072932177628,67.6091482520534,0.));
#97849=CARTESIAN_POINT('Ctrl Pts',(-19.0834236587118,67.6263417083426,0.));
#97850=CARTESIAN_POINT('Ctrl Pts',(-19.0939607887501,67.6435687749841,0.));
#97851=CARTESIAN_POINT('Ctrl Pts',(-19.1045435468358,67.6608292549462,0.));
#97852=CARTESIAN_POINT('Ctrl Pts',(-19.115171910846,67.6781229440573,0.));
#97853=CARTESIAN_POINT('Ctrl Pts',(-19.1258458580345,67.6954496350063,0.));
#97854=CARTESIAN_POINT('Ctrl Pts',(-19.136565365709,67.7128091219348,0.));
#97855=CARTESIAN_POINT('Ctrl Pts',(-19.1473304119955,67.7302012056584,0.));
#97856=CARTESIAN_POINT('Ctrl Pts',(-19.1581409758097,67.7476256934444,0.));
#97857=CARTESIAN_POINT('Ctrl Pts',(-19.168997036495,67.7650823965127,0.));
#97858=CARTESIAN_POINT('Ctrl Pts',(-19.1798985735688,67.7825711283096,0.));
#97859=CARTESIAN_POINT('Ctrl Pts',(-19.1908455664098,67.8000917023926,0.));
#97860=CARTESIAN_POINT('Ctrl Pts',(-19.201837993993,67.8176439306621,0.));
#97861=CARTESIAN_POINT('Ctrl Pts',(-19.2128758350346,67.835227624289,0.));
#97862=CARTESIAN_POINT('Ctrl Pts',(-19.2239590681133,67.8528425945184,0.));
#97863=CARTESIAN_POINT('Ctrl Pts',(-19.2350876717874,67.8704886534544,0.));
#97864=CARTESIAN_POINT('Ctrl Pts',(-19.2462616247279,67.8881656149955,0.));
#97865=CARTESIAN_POINT('Ctrl Pts',(-19.2574809057696,67.9058732951788,0.));
#97866=CARTESIAN_POINT('Ctrl Pts',(-19.2687454938442,67.9236115116758,0.));
#97867=CARTESIAN_POINT('Ctrl Pts',(-19.280055367936,67.9413800834793,0.));
#97868=CARTESIAN_POINT('Ctrl Pts',(-19.2914105070286,67.9591788305394,0.));
#97869=CARTESIAN_POINT('Ctrl Pts',(-19.302810890038,67.9770075733485,0.));
#97870=CARTESIAN_POINT('Ctrl Pts',(-19.3142564958203,67.9948661329617,0.));
#97871=CARTESIAN_POINT('Ctrl Pts',(-19.3257473032034,68.0127543311776,0.));
#97872=CARTESIAN_POINT('Ctrl Pts',(-19.3372832910076,68.0306719906636,0.));
#97873=CARTESIAN_POINT('Ctrl Pts',(-19.3488644380641,68.0486189351011,0.));
#97874=CARTESIAN_POINT('Ctrl Pts',(-19.3604907232314,68.0665949893195,0.));
#97875=CARTESIAN_POINT('Ctrl Pts',(-19.3721621253912,68.0845999792247,0.));
#97876=CARTESIAN_POINT('Ctrl Pts',(-19.3838786234421,68.1026337317285,0.));
#97877=CARTESIAN_POINT('Ctrl Pts',(-19.3956401962895,68.1206960746769,0.));
#97878=CARTESIAN_POINT('Ctrl Pts',(-19.40744682283,68.1387868367691,0.));
#97879=CARTESIAN_POINT('Ctrl Pts',(-19.4192984819418,68.1569058475054,0.));
#97880=CARTESIAN_POINT('Ctrl Pts',(-19.4311951524983,68.1750529372232,0.));
#97881=CARTESIAN_POINT('Ctrl Pts',(-19.4431368133719,68.1932279371127,0.));
#97882=CARTESIAN_POINT('Ctrl Pts',(-19.455123443438,68.2114306792358,0.));
#97883=CARTESIAN_POINT('Ctrl Pts',(-19.467155021572,68.2296609965448,0.));
#97884=CARTESIAN_POINT('Ctrl Pts',(-19.4792315266501,68.2479187228803,0.));
#97885=CARTESIAN_POINT('Ctrl Pts',(-19.4913529375543,68.2662036929526,0.));
#97886=CARTESIAN_POINT('Ctrl Pts',(-19.5035192331705,68.2845157423233,0.));
#97887=CARTESIAN_POINT('Ctrl Pts',(-19.5157303923856,68.3028547073864,0.));
#97888=CARTESIAN_POINT('Ctrl Pts',(-19.5279863940773,68.3212204253417,0.));
#97889=CARTESIAN_POINT('Ctrl Pts',(-19.5402872171191,68.3396127341938,0.));
#97890=CARTESIAN_POINT('Ctrl Pts',(-19.5526328403852,68.3580314727523,0.));
#97891=CARTESIAN_POINT('Ctrl Pts',(-19.5650232427516,68.3764764806287,0.));
#97892=CARTESIAN_POINT('Ctrl Pts',(-19.5774584030938,68.3949475982335,0.));
#97893=CARTESIAN_POINT('Ctrl Pts',(-19.5899383002802,68.4134446667696,0.));
#97894=CARTESIAN_POINT('Ctrl Pts',(-19.6024629131785,68.4319675282275,0.));
#97895=CARTESIAN_POINT('Ctrl Pts',(-19.6150322206577,68.4505160253778,0.));
#97896=CARTESIAN_POINT('Ctrl Pts',(-19.6276462015888,68.4690900017632,0.));
#97897=CARTESIAN_POINT('Ctrl Pts',(-19.6403048348395,68.4876893016856,0.));
#97898=CARTESIAN_POINT('Ctrl Pts',(-19.6530080992686,68.5063137701971,0.));
#97899=CARTESIAN_POINT('Ctrl Pts',(-19.6657559737336,68.5249632530979,0.));
#97900=CARTESIAN_POINT('Ctrl Pts',(-19.6785484370927,68.5436375969311,0.));
#97901=CARTESIAN_POINT('Ctrl Pts',(-19.6913854682046,68.5623366489779,0.));
#97902=CARTESIAN_POINT('Ctrl Pts',(-19.7042670459237,68.581060257249,0.));
#97903=CARTESIAN_POINT('Ctrl Pts',(-19.7171931490956,68.5998082704766,0.));
#97904=CARTESIAN_POINT('Ctrl Pts',(-19.7301637565652,68.6185805381126,0.));
#97905=CARTESIAN_POINT('Ctrl Pts',(-19.7431788471776,68.6373769103224,0.));
#97906=CARTESIAN_POINT('Ctrl Pts',(-19.7562383997781,68.6561972379793,0.));
#97907=CARTESIAN_POINT('Ctrl Pts',(-19.7693423932058,68.6750413726547,0.));
#97908=CARTESIAN_POINT('Ctrl Pts',(-19.7824908062913,68.6939091666111,0.));
#97909=CARTESIAN_POINT('Ctrl Pts',(-19.795683617864,68.7128004727998,0.));
#97910=CARTESIAN_POINT('Ctrl Pts',(-19.8089208067532,68.7317151448557,0.));
#97911=CARTESIAN_POINT('Ctrl Pts',(-19.8222023517874,68.7506530370918,0.));
#97912=CARTESIAN_POINT('Ctrl Pts',(-19.835528231787,68.7696140044892,0.));
#97913=CARTESIAN_POINT('Ctrl Pts',(-19.8488984255641,68.7885979026927,0.));
#97914=CARTESIAN_POINT('Ctrl Pts',(-19.8623129119304,68.8076045880102,0.));
#97915=CARTESIAN_POINT('Ctrl Pts',(-19.8757716696969,68.8266339174068,0.));
#97916=CARTESIAN_POINT('Ctrl Pts',(-19.8892746776734,68.8456857484988,0.));
#97917=CARTESIAN_POINT('Ctrl Pts',(-19.9028219146607,68.8647599395437,0.));
#97918=CARTESIAN_POINT('Ctrl Pts',(-19.9164133594513,68.8838563494356,0.));
#97919=CARTESIAN_POINT('Ctrl Pts',(-19.9300489908364,68.902974837704,0.));
#97920=CARTESIAN_POINT('Ctrl Pts',(-19.9437287876063,68.9221152645086,0.));
#97921=CARTESIAN_POINT('Ctrl Pts',(-19.9574527285492,68.9412774906346,0.));
#97922=CARTESIAN_POINT('Ctrl Pts',(-19.9712207924437,68.960461377483,0.));
#97923=CARTESIAN_POINT('Ctrl Pts',(-19.98503295806,68.9796667870667,0.));
#97924=CARTESIAN_POINT('Ctrl Pts',(-19.9988892041671,68.9988935820101,0.));
#97925=CARTESIAN_POINT('Ctrl Pts',(-20.0127895095327,69.0181416255433,0.));
#97926=CARTESIAN_POINT('Ctrl Pts',(-20.0267338529221,69.0374107814977,0.));
#97927=CARTESIAN_POINT('Ctrl Pts',(-20.0407222130902,69.0567009142968,0.));
#97928=CARTESIAN_POINT('Ctrl Pts',(-20.0547545687839,69.0760118889525,0.));
#97929=CARTESIAN_POINT('Ctrl Pts',(-20.0688308987478,69.0953435710634,0.));
#97930=CARTESIAN_POINT('Ctrl Pts',(-20.082951181725,69.1146958268104,0.));
#97931=CARTESIAN_POINT('Ctrl Pts',(-20.0971153964557,69.1340685229516,0.));
#97932=CARTESIAN_POINT('Ctrl Pts',(-20.1113235216694,69.1534615268153,0.));
#97933=CARTESIAN_POINT('Ctrl Pts',(-20.1255755360871,69.172874706296,0.));
#97934=CARTESIAN_POINT('Ctrl Pts',(-20.1398714184278,69.1923079298534,0.));
#97935=CARTESIAN_POINT('Ctrl Pts',(-20.1542111474086,69.2117610665073,0.));
#97936=CARTESIAN_POINT('Ctrl Pts',(-20.1685947017433,69.2312339858337,0.));
#97937=CARTESIAN_POINT('Ctrl Pts',(-20.183022060135,69.2507265579562,0.));
#97938=CARTESIAN_POINT('Ctrl Pts',(-20.1974932012775,69.2702386535432,0.));
#97939=CARTESIAN_POINT('Ctrl Pts',(-20.2120081038622,69.2897701438066,0.));
#97940=CARTESIAN_POINT('Ctrl Pts',(-20.2265667465784,69.3093209004986,0.));
#97941=CARTESIAN_POINT('Ctrl Pts',(-20.2411691081122,69.3288907959065,0.));
#97942=CARTESIAN_POINT('Ctrl Pts',(-20.255815167139,69.3484797028454,0.));
#97943=CARTESIAN_POINT('Ctrl Pts',(-20.2705049023241,69.3680874946548,0.));
#97944=CARTESIAN_POINT('Ctrl Pts',(-20.2852382923299,69.3877140451975,0.));
#97945=CARTESIAN_POINT('Ctrl Pts',(-20.3000153158167,69.4073592288562,0.));
#97946=CARTESIAN_POINT('Ctrl Pts',(-20.3148359514414,69.4270229205296,0.));
#97947=CARTESIAN_POINT('Ctrl Pts',(-20.3297001778505,69.4467049956257,0.));
#97948=CARTESIAN_POINT('Ctrl Pts',(-20.3446079736799,69.4664053300579,0.));
#97949=CARTESIAN_POINT('Ctrl Pts',(-20.3595593175619,69.4861238002433,0.));
#97950=CARTESIAN_POINT('Ctrl Pts',(-20.3745541881266,69.5058602831004,0.));
#97951=CARTESIAN_POINT('Ctrl Pts',(-20.3895925640006,69.5256146560444,0.));
#97952=CARTESIAN_POINT('Ctrl Pts',(-20.4046744238002,69.5453867969815,0.));
#97953=CARTESIAN_POINT('Ctrl Pts',(-20.4197997461305,69.565176584305,0.));
#97954=CARTESIAN_POINT('Ctrl Pts',(-20.4349685095928,69.5849838968944,0.));
#97955=CARTESIAN_POINT('Ctrl Pts',(-20.4501806927854,69.6048086141122,0.));
#97956=CARTESIAN_POINT('Ctrl Pts',(-20.4654362743036,69.6246506158009,0.));
#97957=CARTESIAN_POINT('Ctrl Pts',(-20.4807352327335,69.6445097822778,0.));
#97958=CARTESIAN_POINT('Ctrl Pts',(-20.4960775466487,69.6643859943291,0.));
#97959=CARTESIAN_POINT('Ctrl Pts',(-20.511463194618,69.6842791332102,0.));
#97960=CARTESIAN_POINT('Ctrl Pts',(-20.5268921552075,69.7041890806421,0.));
#97961=CARTESIAN_POINT('Ctrl Pts',(-20.54236440698,69.7241157188086,0.));
#97962=CARTESIAN_POINT('Ctrl Pts',(-20.5578799284898,69.7440589303511,0.));
#97963=CARTESIAN_POINT('Ctrl Pts',(-20.5734386982781,69.7640185983641,0.));
#97964=CARTESIAN_POINT('Ctrl Pts',(-20.5890406948809,69.7839946063942,0.));
#97965=CARTESIAN_POINT('Ctrl Pts',(-20.6046858968305,69.8039868384382,0.));
#97966=CARTESIAN_POINT('Ctrl Pts',(-20.6203742826566,69.8239951789402,0.));
#97967=CARTESIAN_POINT('Ctrl Pts',(-20.6361058308812,69.8440195127874,0.));
#97968=CARTESIAN_POINT('Ctrl Pts',(-20.6518805200132,69.8640597253058,0.));
#97969=CARTESIAN_POINT('Ctrl Pts',(-20.6676983285542,69.884115702258,0.));
#97970=CARTESIAN_POINT('Ctrl Pts',(-20.6835592350031,69.9041873298416,0.));
#97971=CARTESIAN_POINT('Ctrl Pts',(-20.6994632178551,69.9242744946854,0.));
#97972=CARTESIAN_POINT('Ctrl Pts',(-20.7154102555996,69.9443770838444,0.));
#97973=CARTESIAN_POINT('Ctrl Pts',(-20.7314003267118,69.9644949847929,0.));
#97974=CARTESIAN_POINT('Ctrl Pts',(-20.7474334096581,69.9846280854254,0.));
#97975=CARTESIAN_POINT('Ctrl Pts',(-20.7635094829016,70.0047762740569,0.));
#97976=CARTESIAN_POINT('Ctrl Pts',(-20.7796285249023,70.0249394394221,0.));
#97977=CARTESIAN_POINT('Ctrl Pts',(-20.7957905141155,70.0451174706739,0.));
#97978=CARTESIAN_POINT('Ctrl Pts',(-20.8119954289845,70.0653102573798,0.));
#97979=CARTESIAN_POINT('Ctrl Pts',(-20.8282432479425,70.0855176895185,0.));
#97980=CARTESIAN_POINT('Ctrl Pts',(-20.8445339494184,70.1057396574741,0.));
#97981=CARTESIAN_POINT('Ctrl Pts',(-20.8608675118377,70.1259760520306,0.));
#97982=CARTESIAN_POINT('Ctrl Pts',(-20.8772439136207,70.1462267643649,0.));
#97983=CARTESIAN_POINT('Ctrl Pts',(-20.8936631331751,70.1664916860366,0.));
#97984=CARTESIAN_POINT('Ctrl Pts',(-20.9101251488948,70.1867707089866,0.));
#97985=CARTESIAN_POINT('Ctrl Pts',(-20.9266299391688,70.2070637255469,0.));
#97986=CARTESIAN_POINT('Ctrl Pts',(-20.9431774823833,70.2273706284479,0.));
#97987=CARTESIAN_POINT('Ctrl Pts',(-20.9597677569227,70.2476913108242,0.));
#97988=CARTESIAN_POINT('Ctrl Pts',(-20.9764007411648,70.2680256662215,0.));
#97989=CARTESIAN_POINT('Ctrl Pts',(-20.993076413477,70.288373588597,0.));
#97990=CARTESIAN_POINT('Ctrl Pts',(-21.0097947522212,70.3087349722959,0.));
#97991=CARTESIAN_POINT('Ctrl Pts',(-21.0265557357544,70.3291097120293,0.));
#97992=CARTESIAN_POINT('Ctrl Pts',(-21.0433593424266,70.3494977028497,0.));
#97993=CARTESIAN_POINT('Ctrl Pts',(-21.0602055505751,70.3698988401291,0.));
#97994=CARTESIAN_POINT('Ctrl Pts',(-21.0770943385146,70.3903130195279,0.));
#97995=CARTESIAN_POINT('Ctrl Pts',(-21.0940256845477,70.4107401370403,0.));
#97996=CARTESIAN_POINT('Ctrl Pts',(-21.110999566975,70.4311800890411,0.));
#97997=CARTESIAN_POINT('Ctrl Pts',(-21.1280159641003,70.4516327723349,0.));
#97998=CARTESIAN_POINT('Ctrl Pts',(-21.1450748542335,70.4720980841934,0.));
#97999=CARTESIAN_POINT('Ctrl Pts',(-21.1621762156894,70.4925759224208,0.));
#98000=CARTESIAN_POINT('Ctrl Pts',(-21.1793200267843,70.5130661852946,0.));
#98001=CARTESIAN_POINT('Ctrl Pts',(-21.1965062658296,70.5335687714422,0.));
#98002=CARTESIAN_POINT('Ctrl Pts',(-21.2137349111207,70.5540835797281,0.));
#98003=CARTESIAN_POINT('Ctrl Pts',(-21.2310059409265,70.5746105091503,0.));
#98004=CARTESIAN_POINT('Ctrl Pts',(-21.2483193334676,70.5951494586961,0.));
#98005=CARTESIAN_POINT('Ctrl Pts',(-21.2656750669129,70.6157003273326,0.));
#98006=CARTESIAN_POINT('Ctrl Pts',(-21.2830731194187,70.6362630143062,0.));
#98007=CARTESIAN_POINT('Ctrl Pts',(-21.3005134691563,70.6568374193786,0.));
#98008=CARTESIAN_POINT('Ctrl Pts',(-21.3179960943388,70.6774234430899,0.));
#98009=CARTESIAN_POINT('Ctrl Pts',(-21.3355209732438,70.6980209870032,0.));
#98010=CARTESIAN_POINT('Ctrl Pts',(-21.353088084234,70.7186299539698,0.));
#98011=CARTESIAN_POINT('Ctrl Pts',(-21.3706974057028,70.7392502475438,0.));
#98012=CARTESIAN_POINT('Ctrl Pts',(-21.3883489160187,70.7598817714078,0.));
#98013=CARTESIAN_POINT('Ctrl Pts',(-21.4060425934595,70.780524428744,0.));
#98014=CARTESIAN_POINT('Ctrl Pts',(-21.4237784161592,70.8011781217409,0.));
#98015=CARTESIAN_POINT('Ctrl Pts',(-21.4415563620127,70.8218427507545,0.));
#98016=CARTESIAN_POINT('Ctrl Pts',(-21.4593764087492,70.84251821499,0.));
#98017=CARTESIAN_POINT('Ctrl Pts',(-21.4772385340978,70.8632044140166,0.));
#98018=CARTESIAN_POINT('Ctrl Pts',(-21.4951427159272,70.8839012490903,0.));
#98019=CARTESIAN_POINT('Ctrl Pts',(-21.5130889323767,70.9046086244123,0.));
#98020=CARTESIAN_POINT('Ctrl Pts',(-21.5310771620209,70.9253264487576,0.));
#98021=CARTESIAN_POINT('Ctrl Pts',(-21.549107383907,70.9460546358597,0.));
#98022=CARTESIAN_POINT('Ctrl Pts',(-21.5645987555282,70.9638315189646,0.));
#98023=CARTESIAN_POINT('Ctrl Pts',(-21.576498336635,70.9774662112375,0.));
#98024=CARTESIAN_POINT('Ctrl Pts',(-21.5847875433159,70.9869541807807,0.));
#98025=CARTESIAN_POINT('Ctrl Pts',(-21.5894540925368,70.9922924595081,0.));
#98026=CARTESIAN_POINT('Ctrl Pts',(-21.59049199348,70.9934796068777,0.));
#98027=CARTESIAN_POINT('',(-18.9407177820969,67.3887914263118,12.));
#98028=CARTESIAN_POINT('',(-18.9407177820969,67.3887914263118,0.));
#98029=CARTESIAN_POINT('Ctrl Pts',(-21.59049199348,70.9934796068777,12.));
#98030=CARTESIAN_POINT('Ctrl Pts',(-21.5894540925368,70.9922924595081,12.));
#98031=CARTESIAN_POINT('Ctrl Pts',(-21.5847875433159,70.9869541807807,12.));
#98032=CARTESIAN_POINT('Ctrl Pts',(-21.576498336635,70.9774662112375,12.));
#98033=CARTESIAN_POINT('Ctrl Pts',(-21.5645987555282,70.9638315189647,12.));
#98034=CARTESIAN_POINT('Ctrl Pts',(-21.549107383907,70.9460546358597,12.));
#98035=CARTESIAN_POINT('Ctrl Pts',(-21.5310771620209,70.9253264487576,12.));
#98036=CARTESIAN_POINT('Ctrl Pts',(-21.5130889323767,70.9046086244123,12.));
#98037=CARTESIAN_POINT('Ctrl Pts',(-21.4951427159272,70.8839012490903,12.));
#98038=CARTESIAN_POINT('Ctrl Pts',(-21.4772385340978,70.8632044140166,12.));
#98039=CARTESIAN_POINT('Ctrl Pts',(-21.4593764087492,70.84251821499,12.));
#98040=CARTESIAN_POINT('Ctrl Pts',(-21.4415563620127,70.8218427507545,12.));
#98041=CARTESIAN_POINT('Ctrl Pts',(-21.4237784161592,70.8011781217409,12.));
#98042=CARTESIAN_POINT('Ctrl Pts',(-21.4060425934595,70.780524428744,12.));
#98043=CARTESIAN_POINT('Ctrl Pts',(-21.3883489160187,70.7598817714078,12.));
#98044=CARTESIAN_POINT('Ctrl Pts',(-21.3706974057028,70.7392502475438,12.));
#98045=CARTESIAN_POINT('Ctrl Pts',(-21.353088084234,70.7186299539698,12.));
#98046=CARTESIAN_POINT('Ctrl Pts',(-21.3355209732438,70.6980209870032,12.));
#98047=CARTESIAN_POINT('Ctrl Pts',(-21.3179960943388,70.6774234430899,12.));
#98048=CARTESIAN_POINT('Ctrl Pts',(-21.3005134691563,70.6568374193786,12.));
#98049=CARTESIAN_POINT('Ctrl Pts',(-21.2830731194187,70.6362630143062,12.));
#98050=CARTESIAN_POINT('Ctrl Pts',(-21.2656750669129,70.6157003273326,12.));
#98051=CARTESIAN_POINT('Ctrl Pts',(-21.2483193334676,70.5951494586961,12.));
#98052=CARTESIAN_POINT('Ctrl Pts',(-21.2310059409265,70.5746105091503,12.));
#98053=CARTESIAN_POINT('Ctrl Pts',(-21.2137349111207,70.5540835797281,12.));
#98054=CARTESIAN_POINT('Ctrl Pts',(-21.1965062658296,70.5335687714422,12.));
#98055=CARTESIAN_POINT('Ctrl Pts',(-21.1793200267843,70.5130661852946,12.));
#98056=CARTESIAN_POINT('Ctrl Pts',(-21.1621762156894,70.4925759224208,12.));
#98057=CARTESIAN_POINT('Ctrl Pts',(-21.1450748542335,70.4720980841934,12.));
#98058=CARTESIAN_POINT('Ctrl Pts',(-21.1280159641003,70.4516327723349,12.));
#98059=CARTESIAN_POINT('Ctrl Pts',(-21.110999566975,70.4311800890411,12.));
#98060=CARTESIAN_POINT('Ctrl Pts',(-21.0940256845477,70.4107401370403,12.));
#98061=CARTESIAN_POINT('Ctrl Pts',(-21.0770943385146,70.3903130195279,12.));
#98062=CARTESIAN_POINT('Ctrl Pts',(-21.0602055505751,70.3698988401291,12.));
#98063=CARTESIAN_POINT('Ctrl Pts',(-21.0433593424266,70.3494977028497,12.));
#98064=CARTESIAN_POINT('Ctrl Pts',(-21.0265557357544,70.3291097120293,12.));
#98065=CARTESIAN_POINT('Ctrl Pts',(-21.0097947522212,70.3087349722959,12.));
#98066=CARTESIAN_POINT('Ctrl Pts',(-20.993076413477,70.288373588597,12.));
#98067=CARTESIAN_POINT('Ctrl Pts',(-20.9764007411648,70.2680256662215,12.));
#98068=CARTESIAN_POINT('Ctrl Pts',(-20.9597677569227,70.2476913108242,12.));
#98069=CARTESIAN_POINT('Ctrl Pts',(-20.9431774823833,70.2273706284479,12.));
#98070=CARTESIAN_POINT('Ctrl Pts',(-20.9266299391688,70.2070637255469,12.));
#98071=CARTESIAN_POINT('Ctrl Pts',(-20.9101251488948,70.1867707089866,12.));
#98072=CARTESIAN_POINT('Ctrl Pts',(-20.8936631331751,70.1664916860366,12.));
#98073=CARTESIAN_POINT('Ctrl Pts',(-20.8772439136207,70.1462267643649,12.));
#98074=CARTESIAN_POINT('Ctrl Pts',(-20.8608675118377,70.1259760520306,12.));
#98075=CARTESIAN_POINT('Ctrl Pts',(-20.8445339494184,70.1057396574741,12.));
#98076=CARTESIAN_POINT('Ctrl Pts',(-20.8282432479425,70.0855176895185,12.));
#98077=CARTESIAN_POINT('Ctrl Pts',(-20.8119954289845,70.0653102573798,12.));
#98078=CARTESIAN_POINT('Ctrl Pts',(-20.7957905141155,70.0451174706739,12.));
#98079=CARTESIAN_POINT('Ctrl Pts',(-20.7796285249023,70.0249394394221,12.));
#98080=CARTESIAN_POINT('Ctrl Pts',(-20.7635094829016,70.0047762740569,12.));
#98081=CARTESIAN_POINT('Ctrl Pts',(-20.7474334096581,69.9846280854254,12.));
#98082=CARTESIAN_POINT('Ctrl Pts',(-20.7314003267118,69.9644949847929,12.));
#98083=CARTESIAN_POINT('Ctrl Pts',(-20.7154102555996,69.9443770838444,12.));
#98084=CARTESIAN_POINT('Ctrl Pts',(-20.6994632178551,69.9242744946854,12.));
#98085=CARTESIAN_POINT('Ctrl Pts',(-20.6835592350031,69.9041873298416,12.));
#98086=CARTESIAN_POINT('Ctrl Pts',(-20.6676983285542,69.884115702258,12.));
#98087=CARTESIAN_POINT('Ctrl Pts',(-20.6518805200132,69.8640597253058,12.));
#98088=CARTESIAN_POINT('Ctrl Pts',(-20.6361058308812,69.8440195127874,12.));
#98089=CARTESIAN_POINT('Ctrl Pts',(-20.6203742826566,69.8239951789402,12.));
#98090=CARTESIAN_POINT('Ctrl Pts',(-20.6046858968305,69.8039868384382,12.));
#98091=CARTESIAN_POINT('Ctrl Pts',(-20.5890406948809,69.7839946063942,12.));
#98092=CARTESIAN_POINT('Ctrl Pts',(-20.5734386982781,69.7640185983641,12.));
#98093=CARTESIAN_POINT('Ctrl Pts',(-20.5578799284898,69.7440589303511,12.));
#98094=CARTESIAN_POINT('Ctrl Pts',(-20.54236440698,69.7241157188086,12.));
#98095=CARTESIAN_POINT('Ctrl Pts',(-20.5268921552075,69.7041890806421,12.));
#98096=CARTESIAN_POINT('Ctrl Pts',(-20.511463194618,69.6842791332102,12.));
#98097=CARTESIAN_POINT('Ctrl Pts',(-20.4960775466487,69.6643859943291,12.));
#98098=CARTESIAN_POINT('Ctrl Pts',(-20.4807352327335,69.6445097822778,12.));
#98099=CARTESIAN_POINT('Ctrl Pts',(-20.4654362743036,69.6246506158009,12.));
#98100=CARTESIAN_POINT('Ctrl Pts',(-20.4501806927854,69.6048086141122,12.));
#98101=CARTESIAN_POINT('Ctrl Pts',(-20.4349685095928,69.5849838968944,12.));
#98102=CARTESIAN_POINT('Ctrl Pts',(-20.4197997461305,69.565176584305,12.));
#98103=CARTESIAN_POINT('Ctrl Pts',(-20.4046744238002,69.5453867969815,12.));
#98104=CARTESIAN_POINT('Ctrl Pts',(-20.3895925640006,69.5256146560444,12.));
#98105=CARTESIAN_POINT('Ctrl Pts',(-20.3745541881266,69.5058602831004,12.));
#98106=CARTESIAN_POINT('Ctrl Pts',(-20.3595593175619,69.4861238002433,12.));
#98107=CARTESIAN_POINT('Ctrl Pts',(-20.3446079736799,69.4664053300579,12.));
#98108=CARTESIAN_POINT('Ctrl Pts',(-20.3297001778505,69.4467049956257,12.));
#98109=CARTESIAN_POINT('Ctrl Pts',(-20.3148359514414,69.4270229205296,12.));
#98110=CARTESIAN_POINT('Ctrl Pts',(-20.3000153158167,69.4073592288562,12.));
#98111=CARTESIAN_POINT('Ctrl Pts',(-20.2852382923299,69.3877140451975,12.));
#98112=CARTESIAN_POINT('Ctrl Pts',(-20.2705049023241,69.3680874946548,12.));
#98113=CARTESIAN_POINT('Ctrl Pts',(-20.255815167139,69.3484797028454,12.));
#98114=CARTESIAN_POINT('Ctrl Pts',(-20.2411691081122,69.3288907959065,12.));
#98115=CARTESIAN_POINT('Ctrl Pts',(-20.2265667465784,69.3093209004986,12.));
#98116=CARTESIAN_POINT('Ctrl Pts',(-20.2120081038622,69.2897701438066,12.));
#98117=CARTESIAN_POINT('Ctrl Pts',(-20.1974932012775,69.2702386535432,12.));
#98118=CARTESIAN_POINT('Ctrl Pts',(-20.183022060135,69.2507265579562,12.));
#98119=CARTESIAN_POINT('Ctrl Pts',(-20.1685947017433,69.2312339858337,12.));
#98120=CARTESIAN_POINT('Ctrl Pts',(-20.1542111474086,69.2117610665073,12.));
#98121=CARTESIAN_POINT('Ctrl Pts',(-20.1398714184278,69.1923079298534,12.));
#98122=CARTESIAN_POINT('Ctrl Pts',(-20.1255755360871,69.172874706296,12.));
#98123=CARTESIAN_POINT('Ctrl Pts',(-20.1113235216694,69.1534615268153,12.));
#98124=CARTESIAN_POINT('Ctrl Pts',(-20.0971153964557,69.1340685229516,12.));
#98125=CARTESIAN_POINT('Ctrl Pts',(-20.082951181725,69.1146958268104,12.));
#98126=CARTESIAN_POINT('Ctrl Pts',(-20.0688308987478,69.0953435710634,12.));
#98127=CARTESIAN_POINT('Ctrl Pts',(-20.0547545687839,69.0760118889525,12.));
#98128=CARTESIAN_POINT('Ctrl Pts',(-20.0407222130902,69.0567009142968,12.));
#98129=CARTESIAN_POINT('Ctrl Pts',(-20.0267338529221,69.0374107814977,12.));
#98130=CARTESIAN_POINT('Ctrl Pts',(-20.0127895095327,69.0181416255433,12.));
#98131=CARTESIAN_POINT('Ctrl Pts',(-19.9988892041671,68.9988935820101,12.));
#98132=CARTESIAN_POINT('Ctrl Pts',(-19.98503295806,68.9796667870667,12.));
#98133=CARTESIAN_POINT('Ctrl Pts',(-19.9712207924437,68.960461377483,12.));
#98134=CARTESIAN_POINT('Ctrl Pts',(-19.9574527285492,68.9412774906346,12.));
#98135=CARTESIAN_POINT('Ctrl Pts',(-19.9437287876063,68.9221152645086,12.));
#98136=CARTESIAN_POINT('Ctrl Pts',(-19.9300489908364,68.902974837704,12.));
#98137=CARTESIAN_POINT('Ctrl Pts',(-19.9164133594513,68.8838563494356,12.));
#98138=CARTESIAN_POINT('Ctrl Pts',(-19.9028219146607,68.8647599395437,12.));
#98139=CARTESIAN_POINT('Ctrl Pts',(-19.8892746776734,68.8456857484988,12.));
#98140=CARTESIAN_POINT('Ctrl Pts',(-19.8757716696969,68.8266339174068,12.));
#98141=CARTESIAN_POINT('Ctrl Pts',(-19.8623129119304,68.8076045880102,12.));
#98142=CARTESIAN_POINT('Ctrl Pts',(-19.8488984255641,68.7885979026927,12.));
#98143=CARTESIAN_POINT('Ctrl Pts',(-19.835528231787,68.7696140044892,12.));
#98144=CARTESIAN_POINT('Ctrl Pts',(-19.8222023517874,68.7506530370918,12.));
#98145=CARTESIAN_POINT('Ctrl Pts',(-19.8089208067532,68.7317151448557,12.));
#98146=CARTESIAN_POINT('Ctrl Pts',(-19.795683617864,68.7128004727998,12.));
#98147=CARTESIAN_POINT('Ctrl Pts',(-19.7824908062913,68.6939091666111,12.));
#98148=CARTESIAN_POINT('Ctrl Pts',(-19.7693423932058,68.6750413726547,12.));
#98149=CARTESIAN_POINT('Ctrl Pts',(-19.7562383997781,68.6561972379793,12.));
#98150=CARTESIAN_POINT('Ctrl Pts',(-19.7431788471776,68.6373769103224,12.));
#98151=CARTESIAN_POINT('Ctrl Pts',(-19.7301637565652,68.6185805381126,12.));
#98152=CARTESIAN_POINT('Ctrl Pts',(-19.7171931490956,68.5998082704766,12.));
#98153=CARTESIAN_POINT('Ctrl Pts',(-19.7042670459237,68.581060257249,12.));
#98154=CARTESIAN_POINT('Ctrl Pts',(-19.6913854682046,68.5623366489779,12.));
#98155=CARTESIAN_POINT('Ctrl Pts',(-19.6785484370927,68.5436375969311,12.));
#98156=CARTESIAN_POINT('Ctrl Pts',(-19.6657559737336,68.5249632530979,12.));
#98157=CARTESIAN_POINT('Ctrl Pts',(-19.6530080992686,68.5063137701971,12.));
#98158=CARTESIAN_POINT('Ctrl Pts',(-19.6403048348395,68.4876893016856,12.));
#98159=CARTESIAN_POINT('Ctrl Pts',(-19.6276462015888,68.4690900017632,12.));
#98160=CARTESIAN_POINT('Ctrl Pts',(-19.6150322206577,68.4505160253778,12.));
#98161=CARTESIAN_POINT('Ctrl Pts',(-19.6024629131785,68.4319675282275,12.));
#98162=CARTESIAN_POINT('Ctrl Pts',(-19.5899383002802,68.4134446667696,12.));
#98163=CARTESIAN_POINT('Ctrl Pts',(-19.5774584030938,68.3949475982335,12.));
#98164=CARTESIAN_POINT('Ctrl Pts',(-19.5650232427516,68.3764764806287,12.));
#98165=CARTESIAN_POINT('Ctrl Pts',(-19.5526328403852,68.3580314727523,12.));
#98166=CARTESIAN_POINT('Ctrl Pts',(-19.5402872171191,68.3396127341938,12.));
#98167=CARTESIAN_POINT('Ctrl Pts',(-19.5279863940773,68.3212204253417,12.));
#98168=CARTESIAN_POINT('Ctrl Pts',(-19.5157303923856,68.3028547073864,12.));
#98169=CARTESIAN_POINT('Ctrl Pts',(-19.5035192331705,68.2845157423233,12.));
#98170=CARTESIAN_POINT('Ctrl Pts',(-19.4913529375543,68.2662036929526,12.));
#98171=CARTESIAN_POINT('Ctrl Pts',(-19.4792315266501,68.2479187228803,12.));
#98172=CARTESIAN_POINT('Ctrl Pts',(-19.467155021572,68.2296609965448,12.));
#98173=CARTESIAN_POINT('Ctrl Pts',(-19.455123443438,68.2114306792358,12.));
#98174=CARTESIAN_POINT('Ctrl Pts',(-19.4431368133719,68.1932279371127,12.));
#98175=CARTESIAN_POINT('Ctrl Pts',(-19.4311951524983,68.1750529372232,12.));
#98176=CARTESIAN_POINT('Ctrl Pts',(-19.4192984819418,68.1569058475054,12.));
#98177=CARTESIAN_POINT('Ctrl Pts',(-19.40744682283,68.1387868367691,12.));
#98178=CARTESIAN_POINT('Ctrl Pts',(-19.3956401962895,68.1206960746769,12.));
#98179=CARTESIAN_POINT('Ctrl Pts',(-19.3838786234421,68.1026337317285,12.));
#98180=CARTESIAN_POINT('Ctrl Pts',(-19.3721621253912,68.0845999792247,12.));
#98181=CARTESIAN_POINT('Ctrl Pts',(-19.3604907232314,68.0665949893195,12.));
#98182=CARTESIAN_POINT('Ctrl Pts',(-19.3488644380641,68.0486189351011,12.));
#98183=CARTESIAN_POINT('Ctrl Pts',(-19.3372832910076,68.0306719906636,12.));
#98184=CARTESIAN_POINT('Ctrl Pts',(-19.3257473032034,68.0127543311776,12.));
#98185=CARTESIAN_POINT('Ctrl Pts',(-19.3142564958203,67.9948661329617,12.));
#98186=CARTESIAN_POINT('Ctrl Pts',(-19.302810890038,67.9770075733485,12.));
#98187=CARTESIAN_POINT('Ctrl Pts',(-19.2914105070286,67.9591788305394,12.));
#98188=CARTESIAN_POINT('Ctrl Pts',(-19.280055367936,67.9413800834793,12.));
#98189=CARTESIAN_POINT('Ctrl Pts',(-19.2687454938442,67.9236115116758,12.));
#98190=CARTESIAN_POINT('Ctrl Pts',(-19.2574809057696,67.9058732951788,12.));
#98191=CARTESIAN_POINT('Ctrl Pts',(-19.2462616247279,67.8881656149955,12.));
#98192=CARTESIAN_POINT('Ctrl Pts',(-19.2350876717874,67.8704886534544,12.));
#98193=CARTESIAN_POINT('Ctrl Pts',(-19.2239590681133,67.8528425945184,12.));
#98194=CARTESIAN_POINT('Ctrl Pts',(-19.2128758350346,67.835227624289,12.));
#98195=CARTESIAN_POINT('Ctrl Pts',(-19.201837993993,67.8176439306621,12.));
#98196=CARTESIAN_POINT('Ctrl Pts',(-19.1908455664098,67.8000917023926,12.));
#98197=CARTESIAN_POINT('Ctrl Pts',(-19.1798985735688,67.7825711283096,12.));
#98198=CARTESIAN_POINT('Ctrl Pts',(-19.168997036495,67.7650823965127,12.));
#98199=CARTESIAN_POINT('Ctrl Pts',(-19.1581409758097,67.7476256934444,12.));
#98200=CARTESIAN_POINT('Ctrl Pts',(-19.1473304119955,67.7302012056584,12.));
#98201=CARTESIAN_POINT('Ctrl Pts',(-19.136565365709,67.7128091219348,12.));
#98202=CARTESIAN_POINT('Ctrl Pts',(-19.1258458580345,67.6954496350063,12.));
#98203=CARTESIAN_POINT('Ctrl Pts',(-19.115171910846,67.6781229440573,12.));
#98204=CARTESIAN_POINT('Ctrl Pts',(-19.1045435468358,67.6608292549462,12.));
#98205=CARTESIAN_POINT('Ctrl Pts',(-19.0939607887501,67.6435687749841,12.));
#98206=CARTESIAN_POINT('Ctrl Pts',(-19.0834236587118,67.6263417083426,12.));
#98207=CARTESIAN_POINT('Ctrl Pts',(-19.072932177628,67.6091482520534,12.));
#98208=CARTESIAN_POINT('Ctrl Pts',(-19.062486364241,67.5919885896222,12.));
#98209=CARTESIAN_POINT('Ctrl Pts',(-19.0520862360396,67.5748628971964,12.));
#98210=CARTESIAN_POINT('Ctrl Pts',(-19.0417318110708,67.5577713558194,12.));
#98211=CARTESIAN_POINT('Ctrl Pts',(-19.0314231093923,67.540714161288,12.));
#98212=CARTESIAN_POINT('Ctrl Pts',(-19.021160154824,67.5236915360331,12.));
#98213=CARTESIAN_POINT('Ctrl Pts',(-19.0109429761306,67.5067037372317,12.));
#98214=CARTESIAN_POINT('Ctrl Pts',(-19.0007716032819,67.4897510316844,12.));
#98215=CARTESIAN_POINT('Ctrl Pts',(-18.9906460638625,67.472833671964,12.));
#98216=CARTESIAN_POINT('Ctrl Pts',(-18.9805663798448,67.4559518744638,12.));
#98217=CARTESIAN_POINT('Ctrl Pts',(-18.9705325631711,67.4391057908418,12.));
#98218=CARTESIAN_POINT('Ctrl Pts',(-18.9605446160985,67.4222955061981,12.));
#98219=CARTESIAN_POINT('Ctrl Pts',(-18.9525909517915,67.4088759497911,12.));
#98220=CARTESIAN_POINT('Ctrl Pts',(-18.9466463414299,67.3988274146651,12.));
#98221=CARTESIAN_POINT('Ctrl Pts',(-18.9426924398719,67.3921355608328,12.));
#98222=CARTESIAN_POINT('Ctrl Pts',(-18.9407177820969,67.3887914263118,12.));
#98223=CARTESIAN_POINT('Ctrl Pts',(-23.0342913834073,70.5382514078919,-5.55111512312578E-16));
#98224=CARTESIAN_POINT('Ctrl Pts',(-23.0342913834073,70.5382514078919,4.));
#98225=CARTESIAN_POINT('Ctrl Pts',(-23.0342913834073,70.5382514078919,8.));
#98226=CARTESIAN_POINT('Ctrl Pts',(-23.0342913834073,70.5382514078919,12.));
#98227=CARTESIAN_POINT('Ctrl Pts',(-23.0224954570735,70.6474988907591,-5.55111512312578E-16));
#98228=CARTESIAN_POINT('Ctrl Pts',(-23.0224954570735,70.6474988907591,4.));
#98229=CARTESIAN_POINT('Ctrl Pts',(-23.0224954570735,70.647498890759,8.));
#98230=CARTESIAN_POINT('Ctrl Pts',(-23.0224954570735,70.647498890759,12.));
#98231=CARTESIAN_POINT('Ctrl Pts',(-22.9364730048791,70.8310007146901,-5.55111512312578E-16));
#98232=CARTESIAN_POINT('Ctrl Pts',(-22.9364730048791,70.8310007146901,4.));
#98233=CARTESIAN_POINT('Ctrl Pts',(-22.9364730048791,70.83100071469,7.99999999999999));
#98234=CARTESIAN_POINT('Ctrl Pts',(-22.9364730048791,70.83100071469,12.));
#98235=CARTESIAN_POINT('Ctrl Pts',(-22.7679558220499,70.9357242819031,-5.55111512312578E-16));
#98236=CARTESIAN_POINT('Ctrl Pts',(-22.7679558220499,70.9357242819031,4.));
#98237=CARTESIAN_POINT('Ctrl Pts',(-22.7679558220499,70.9357242819031,8.00000000000001));
#98238=CARTESIAN_POINT('Ctrl Pts',(-22.7679558220499,70.9357242819031,12.));
#98239=CARTESIAN_POINT('Ctrl Pts',(-22.6894590071812,70.9608233461356,-5.55111512312578E-16));
#98240=CARTESIAN_POINT('Ctrl Pts',(-22.6894590071812,70.9608233461356,4.));
#98241=CARTESIAN_POINT('Ctrl Pts',(-22.6894590071812,70.9608233461356,8.));
#98242=CARTESIAN_POINT('Ctrl Pts',(-22.6894590071812,70.9608233461356,12.));
#98243=CARTESIAN_POINT('',(-23.0342913834073,70.5382514078919,0.));
#98244=CARTESIAN_POINT('',(-22.6894590071812,70.9608233461355,2.77555756156289E-16));
#98245=CARTESIAN_POINT('Ctrl Pts',(-23.0342913834073,70.5382514078919,-1.38777878078145E-16));
#98246=CARTESIAN_POINT('Ctrl Pts',(-23.0224954570735,70.6474988907591,-1.38777878078145E-16));
#98247=CARTESIAN_POINT('Ctrl Pts',(-22.9733397701052,70.7523570758625,-1.38777878078145E-16));
#98248=CARTESIAN_POINT('Ctrl Pts',(-22.8972470282358,70.8314917485682,-1.38777878078145E-16));
#98249=CARTESIAN_POINT('Ctrl Pts',(-22.8401774718338,70.8908427530975,-1.38777878078145E-16));
#98250=CARTESIAN_POINT('Ctrl Pts',(-22.7679558220499,70.9357242819031,-1.38777878078145E-16));
#98251=CARTESIAN_POINT('Ctrl Pts',(-22.6894590071812,70.9608233461356,-1.38777878078145E-16));
#98252=CARTESIAN_POINT('',(-22.6894590071812,70.9608233461355,12.));
#98253=CARTESIAN_POINT('Ctrl Pts',(-22.6894590071812,70.9608233461356,-5.55111512312578E-16));
#98254=CARTESIAN_POINT('Ctrl Pts',(-22.6894590071812,70.9608233461356,4.));
#98255=CARTESIAN_POINT('Ctrl Pts',(-22.6894590071812,70.9608233461356,8.));
#98256=CARTESIAN_POINT('Ctrl Pts',(-22.6894590071812,70.9608233461356,12.));
#98257=CARTESIAN_POINT('',(-23.0342913834073,70.5382514078919,12.));
#98258=CARTESIAN_POINT('Ctrl Pts',(-22.6894590071812,70.9608233461356,12.));
#98259=CARTESIAN_POINT('Ctrl Pts',(-22.7679558220499,70.9357242819031,12.));
#98260=CARTESIAN_POINT('Ctrl Pts',(-22.8401774718338,70.8908427530975,12.));
#98261=CARTESIAN_POINT('Ctrl Pts',(-22.8972470282358,70.8314917485682,12.));
#98262=CARTESIAN_POINT('Ctrl Pts',(-22.9733397701052,70.7523570758625,12.));
#98263=CARTESIAN_POINT('Ctrl Pts',(-23.0224954570735,70.647498890759,12.));
#98264=CARTESIAN_POINT('Ctrl Pts',(-23.0342913834073,70.5382514078919,12.));
#98265=CARTESIAN_POINT('Ctrl Pts',(-23.0342913834073,70.5382514078919,12.));
#98266=CARTESIAN_POINT('Ctrl Pts',(-23.0342913834073,70.5382514078919,8.));
#98267=CARTESIAN_POINT('Ctrl Pts',(-23.0342913834073,70.5382514078919,4.));
#98268=CARTESIAN_POINT('Ctrl Pts',(-23.0342913834073,70.5382514078919,-5.55111512312578E-16));
#98269=CARTESIAN_POINT('Origin',(-1.12812358559725E-10,3.57465004850839E-10,
0.));
#98270=CARTESIAN_POINT('Origin',(-1.12812358559725E-10,3.57465004850839E-10,
12.));
#98271=CARTESIAN_POINT('Origin',(-1.12812358559725E-10,3.57465004850839E-10,
0.));
#98272=CARTESIAN_POINT('Ctrl Pts',(-15.8307637747257,72.7986051948032,0.));
#98273=CARTESIAN_POINT('Ctrl Pts',(-15.8307637747257,72.7986051948032,4.));
#98274=CARTESIAN_POINT('Ctrl Pts',(-15.8307637747257,72.7986051948032,8.));
#98275=CARTESIAN_POINT('Ctrl Pts',(-15.8307637747257,72.7986051948032,12.));
#98276=CARTESIAN_POINT('Ctrl Pts',(-15.7233907508393,72.8219545017354,0.));
#98277=CARTESIAN_POINT('Ctrl Pts',(-15.7233907508393,72.8219545017354,4.));
#98278=CARTESIAN_POINT('Ctrl Pts',(-15.7233907508393,72.8219545017354,8.));
#98279=CARTESIAN_POINT('Ctrl Pts',(-15.7233907508393,72.8219545017354,12.));
#98280=CARTESIAN_POINT('Ctrl Pts',(-15.5221041200717,72.7983622347337,0.));
#98281=CARTESIAN_POINT('Ctrl Pts',(-15.5221041200717,72.7983622347337,4.00000000000001));
#98282=CARTESIAN_POINT('Ctrl Pts',(-15.5221041200718,72.7983622347338,7.99999999999999));
#98283=CARTESIAN_POINT('Ctrl Pts',(-15.5221041200718,72.7983622347338,12.));
#98284=CARTESIAN_POINT('Ctrl Pts',(-15.3694736926913,72.6715981986664,0.));
#98285=CARTESIAN_POINT('Ctrl Pts',(-15.3694736926913,72.6715981986664,4.));
#98286=CARTESIAN_POINT('Ctrl Pts',(-15.3694736926914,72.6715981986665,8.00000000000001));
#98287=CARTESIAN_POINT('Ctrl Pts',(-15.3694736926914,72.6715981986665,12.));
#98288=CARTESIAN_POINT('Ctrl Pts',(-15.3208442077185,72.6050633494354,0.));
#98289=CARTESIAN_POINT('Ctrl Pts',(-15.3208442077185,72.6050633494354,4.));
#98290=CARTESIAN_POINT('Ctrl Pts',(-15.3208442077186,72.6050633494355,8.));
#98291=CARTESIAN_POINT('Ctrl Pts',(-15.3208442077186,72.6050633494355,12.));
#98292=CARTESIAN_POINT('',(-15.8307637747257,72.7986051948032,0.));
#98293=CARTESIAN_POINT('',(-15.3208442077189,72.6050633494351,0.));
#98294=CARTESIAN_POINT('Ctrl Pts',(-15.8307637747257,72.7986051948032,0.));
#98295=CARTESIAN_POINT('Ctrl Pts',(-15.7233907508393,72.8219545017354,0.));
#98296=CARTESIAN_POINT('Ctrl Pts',(-15.6083698189721,72.8084732063059,0.));
#98297=CARTESIAN_POINT('Ctrl Pts',(-15.5092366269864,72.7613031699569,0.));
#98298=CARTESIAN_POINT('Ctrl Pts',(-15.4348867329972,72.7259256426953,0.));
#98299=CARTESIAN_POINT('Ctrl Pts',(-15.3694736926913,72.6715981986664,0.));
#98300=CARTESIAN_POINT('Ctrl Pts',(-15.3208442077185,72.6050633494354,0.));
#98301=CARTESIAN_POINT('',(-15.320844207719,72.6050633494352,12.));
#98302=CARTESIAN_POINT('Ctrl Pts',(-15.3208442077185,72.6050633494354,0.));
#98303=CARTESIAN_POINT('Ctrl Pts',(-15.3208442077185,72.6050633494354,4.));
#98304=CARTESIAN_POINT('Ctrl Pts',(-15.3208442077186,72.6050633494355,8.));
#98305=CARTESIAN_POINT('Ctrl Pts',(-15.3208442077186,72.6050633494355,12.));
#98306=CARTESIAN_POINT('',(-15.8307637747257,72.7986051948032,12.));
#98307=CARTESIAN_POINT('Ctrl Pts',(-15.3208442077186,72.6050633494355,12.));
#98308=CARTESIAN_POINT('Ctrl Pts',(-15.3694736926914,72.6715981986665,12.));
#98309=CARTESIAN_POINT('Ctrl Pts',(-15.4348867329973,72.7259256426953,12.));
#98310=CARTESIAN_POINT('Ctrl Pts',(-15.5092366269865,72.761303169957,12.));
#98311=CARTESIAN_POINT('Ctrl Pts',(-15.6083698189722,72.8084732063059,12.));
#98312=CARTESIAN_POINT('Ctrl Pts',(-15.7233907508393,72.8219545017354,12.));
#98313=CARTESIAN_POINT('Ctrl Pts',(-15.8307637747257,72.7986051948032,12.));
#98314=CARTESIAN_POINT('Ctrl Pts',(-15.8307637747257,72.7986051948032,12.));
#98315=CARTESIAN_POINT('Ctrl Pts',(-15.8307637747257,72.7986051948032,8.));
#98316=CARTESIAN_POINT('Ctrl Pts',(-15.8307637747257,72.7986051948032,4.));
#98317=CARTESIAN_POINT('Ctrl Pts',(-15.8307637747257,72.7986051948032,0.));
#98318=CARTESIAN_POINT('Ctrl Pts',(-12.9953224629497,68.7831490561748,0.));
#98319=CARTESIAN_POINT('Ctrl Pts',(-12.9953224629497,68.7831490561748,12.));
#98320=CARTESIAN_POINT('Ctrl Pts',(-12.9969981460277,68.7866525680193,0.));
#98321=CARTESIAN_POINT('Ctrl Pts',(-12.9969981460277,68.7866525680193,12.));
#98322=CARTESIAN_POINT('Ctrl Pts',(-13.0003537683055,68.7936635625545,0.));
#98323=CARTESIAN_POINT('Ctrl Pts',(-13.0003537683055,68.7936635625545,12.));
#98324=CARTESIAN_POINT('Ctrl Pts',(-13.0053999700875,68.804191966902,0.));
#98325=CARTESIAN_POINT('Ctrl Pts',(-13.0053999700875,68.804191966902,12.));
#98326=CARTESIAN_POINT('Ctrl Pts',(-13.0121537768946,68.8182536653656,0.));
#98327=CARTESIAN_POINT('Ctrl Pts',(-13.0121537768946,68.8182536653656,12.));
#98328=CARTESIAN_POINT('Ctrl Pts',(-13.0206386039691,68.8358704887468,0.));
#98329=CARTESIAN_POINT('Ctrl Pts',(-13.0206386039691,68.8358704887468,12.));
#98330=CARTESIAN_POINT('Ctrl Pts',(-13.0291660060107,68.8535269726794,0.));
#98331=CARTESIAN_POINT('Ctrl Pts',(-13.0291660060107,68.8535269726794,12.));
#98332=CARTESIAN_POINT('Ctrl Pts',(-13.0377359881875,68.8712230321906,0.));
#98333=CARTESIAN_POINT('Ctrl Pts',(-13.0377359881875,68.8712230321906,12.));
#98334=CARTESIAN_POINT('Ctrl Pts',(-13.0463485518207,68.8889585151585,0.));
#98335=CARTESIAN_POINT('Ctrl Pts',(-13.0463485518207,68.8889585151585,12.));
#98336=CARTESIAN_POINT('Ctrl Pts',(-13.0550036938813,68.9067332040985,0.));
#98337=CARTESIAN_POINT('Ctrl Pts',(-13.0550036938813,68.9067332040985,12.));
#98338=CARTESIAN_POINT('Ctrl Pts',(-13.0637014089029,68.9245468449945,0.));
#98339=CARTESIAN_POINT('Ctrl Pts',(-13.0637014089029,68.9245468449945,12.));
#98340=CARTESIAN_POINT('Ctrl Pts',(-13.072441690283,68.9423991694492,0.));
#98341=CARTESIAN_POINT('Ctrl Pts',(-13.072441690283,68.9423991694492,12.));
#98342=CARTESIAN_POINT('Ctrl Pts',(-13.0812245317808,68.9602899187573,0.));
#98343=CARTESIAN_POINT('Ctrl Pts',(-13.0812245317808,68.9602899187573,12.));
#98344=CARTESIAN_POINT('Ctrl Pts',(-13.090049929053,68.9782188692581,0.));
#98345=CARTESIAN_POINT('Ctrl Pts',(-13.090049929053,68.9782188692581,12.));
#98346=CARTESIAN_POINT('Ctrl Pts',(-13.0989178791834,68.9961858241519,0.));
#98347=CARTESIAN_POINT('Ctrl Pts',(-13.0989178791834,68.9961858241519,12.));
#98348=CARTESIAN_POINT('Ctrl Pts',(-13.1078283799722,69.0141906015113,0.));
#98349=CARTESIAN_POINT('Ctrl Pts',(-13.1078283799722,69.0141906015113,12.));
#98350=CARTESIAN_POINT('Ctrl Pts',(-13.1167814293497,69.0322330243348,0.));
#98351=CARTESIAN_POINT('Ctrl Pts',(-13.1167814293497,69.0322330243348,12.));
#98352=CARTESIAN_POINT('Ctrl Pts',(-13.1257770246385,69.0503129081817,0.));
#98353=CARTESIAN_POINT('Ctrl Pts',(-13.1257770246385,69.0503129081817,12.));
#98354=CARTESIAN_POINT('Ctrl Pts',(-13.1348151621834,69.0684300549477,0.));
#98355=CARTESIAN_POINT('Ctrl Pts',(-13.1348151621834,69.0684300549477,12.));
#98356=CARTESIAN_POINT('Ctrl Pts',(-13.1438958377404,69.0865842593102,0.));
#98357=CARTESIAN_POINT('Ctrl Pts',(-13.1438958377404,69.0865842593102,12.));
#98358=CARTESIAN_POINT('Ctrl Pts',(-13.1530190467183,69.1047753127643,0.));
#98359=CARTESIAN_POINT('Ctrl Pts',(-13.1530190467183,69.1047753127643,12.));
#98360=CARTESIAN_POINT('Ctrl Pts',(-13.1621847844528,69.1230030082573,0.));
#98361=CARTESIAN_POINT('Ctrl Pts',(-13.1621847844528,69.1230030082573,12.));
#98362=CARTESIAN_POINT('Ctrl Pts',(-13.1713930465133,69.1412671454564,0.));
#98363=CARTESIAN_POINT('Ctrl Pts',(-13.1713930465133,69.1412671454564,12.));
#98364=CARTESIAN_POINT('Ctrl Pts',(-13.1806438286934,69.1595675305245,0.));
#98365=CARTESIAN_POINT('Ctrl Pts',(-13.1806438286934,69.1595675305245,12.));
#98366=CARTESIAN_POINT('Ctrl Pts',(-13.1899371268683,69.1779039735996,0.));
#98367=CARTESIAN_POINT('Ctrl Pts',(-13.1899371268683,69.1779039735996,12.));
#98368=CARTESIAN_POINT('Ctrl Pts',(-13.1992729368928,69.1962762870527,0.));
#98369=CARTESIAN_POINT('Ctrl Pts',(-13.1992729368928,69.1962762870527,12.));
#98370=CARTESIAN_POINT('Ctrl Pts',(-13.2086512544735,69.2146842833537,0.));
#98371=CARTESIAN_POINT('Ctrl Pts',(-13.2086512544735,69.2146842833537,12.));
#98372=CARTESIAN_POINT('Ctrl Pts',(-13.2180720750594,69.2331277732861,0.));
#98373=CARTESIAN_POINT('Ctrl Pts',(-13.2180720750594,69.2331277732861,12.));
#98374=CARTESIAN_POINT('Ctrl Pts',(-13.2275353939051,69.2516065668844,0.));
#98375=CARTESIAN_POINT('Ctrl Pts',(-13.2275353939051,69.2516065668844,12.));
#98376=CARTESIAN_POINT('Ctrl Pts',(-13.237041206122,69.270120474245,0.));
#98377=CARTESIAN_POINT('Ctrl Pts',(-13.237041206122,69.270120474245,12.));
#98378=CARTESIAN_POINT('Ctrl Pts',(-13.2465895067262,69.2886693063182,0.));
#98379=CARTESIAN_POINT('Ctrl Pts',(-13.2465895067262,69.2886693063182,12.));
#98380=CARTESIAN_POINT('Ctrl Pts',(-13.2561802906896,69.3072528758518,0.));
#98381=CARTESIAN_POINT('Ctrl Pts',(-13.2561802906896,69.3072528758518,12.));
#98382=CARTESIAN_POINT('Ctrl Pts',(-13.265813552961,69.3258709977382,0.));
#98383=CARTESIAN_POINT('Ctrl Pts',(-13.265813552961,69.3258709977382,12.));
#98384=CARTESIAN_POINT('Ctrl Pts',(-13.2754892884433,69.3445234885065,0.));
#98385=CARTESIAN_POINT('Ctrl Pts',(-13.2754892884433,69.3445234885065,12.));
#98386=CARTESIAN_POINT('Ctrl Pts',(-13.2852074919766,69.3632101660066,0.));
#98387=CARTESIAN_POINT('Ctrl Pts',(-13.2852074919766,69.3632101660066,12.));
#98388=CARTESIAN_POINT('Ctrl Pts',(-13.2949681583167,69.3819308490422,0.));
#98389=CARTESIAN_POINT('Ctrl Pts',(-13.2949681583167,69.3819308490422,12.));
#98390=CARTESIAN_POINT('Ctrl Pts',(-13.3047712821051,69.4006853569511,0.));
#98391=CARTESIAN_POINT('Ctrl Pts',(-13.3047712821051,69.4006853569511,12.));
#98392=CARTESIAN_POINT('Ctrl Pts',(-13.3146168578743,69.4194735096265,0.));
#98393=CARTESIAN_POINT('Ctrl Pts',(-13.3146168578743,69.4194735096265,12.));
#98394=CARTESIAN_POINT('Ctrl Pts',(-13.3245048800643,69.4382951276998,0.));
#98395=CARTESIAN_POINT('Ctrl Pts',(-13.3245048800643,69.4382951276998,12.));
#98396=CARTESIAN_POINT('Ctrl Pts',(-13.3344353430313,69.4571500326673,0.));
#98397=CARTESIAN_POINT('Ctrl Pts',(-13.3344353430313,69.4571500326673,12.));
#98398=CARTESIAN_POINT('Ctrl Pts',(-13.3444082410543,69.4760380470365,0.));
#98399=CARTESIAN_POINT('Ctrl Pts',(-13.3444082410543,69.4760380470365,12.));
#98400=CARTESIAN_POINT('Ctrl Pts',(-13.3544235683394,69.4949589944606,0.));
#98401=CARTESIAN_POINT('Ctrl Pts',(-13.3544235683394,69.4949589944606,12.));
#98402=CARTESIAN_POINT('Ctrl Pts',(-13.3644813190219,69.5139126996675,0.));
#98403=CARTESIAN_POINT('Ctrl Pts',(-13.3644813190219,69.5139126996675,12.));
#98404=CARTESIAN_POINT('Ctrl Pts',(-13.3745814871665,69.5328989883885,0.));
#98405=CARTESIAN_POINT('Ctrl Pts',(-13.3745814871665,69.5328989883885,12.));
#98406=CARTESIAN_POINT('Ctrl Pts',(-13.3847240667628,69.5519176872862,0.));
#98407=CARTESIAN_POINT('Ctrl Pts',(-13.3847240667628,69.5519176872862,12.));
#98408=CARTESIAN_POINT('Ctrl Pts',(-13.3949090517177,69.5709686238724,0.));
#98409=CARTESIAN_POINT('Ctrl Pts',(-13.3949090517177,69.5709686238724,12.));
#98410=CARTESIAN_POINT('Ctrl Pts',(-13.40513643585,69.5900516264553,0.));
#98411=CARTESIAN_POINT('Ctrl Pts',(-13.40513643585,69.5900516264553,12.));
#98412=CARTESIAN_POINT('Ctrl Pts',(-13.4154062129002,69.6091665241765,0.));
#98413=CARTESIAN_POINT('Ctrl Pts',(-13.4154062129002,69.6091665241765,12.));
#98414=CARTESIAN_POINT('Ctrl Pts',(-13.4257183765341,69.6283131470273,0.));
#98415=CARTESIAN_POINT('Ctrl Pts',(-13.4257183765341,69.6283131470273,12.));
#98416=CARTESIAN_POINT('Ctrl Pts',(-13.4360729203442,69.6474913258675,0.));
#98417=CARTESIAN_POINT('Ctrl Pts',(-13.4360729203442,69.6474913258675,12.));
#98418=CARTESIAN_POINT('Ctrl Pts',(-13.4464698378453,69.666700892444,0.));
#98419=CARTESIAN_POINT('Ctrl Pts',(-13.4464698378453,69.666700892444,12.));
#98420=CARTESIAN_POINT('Ctrl Pts',(-13.456909122476,69.6859416793885,0.));
#98421=CARTESIAN_POINT('Ctrl Pts',(-13.456909122476,69.6859416793885,12.));
#98422=CARTESIAN_POINT('Ctrl Pts',(-13.4673907676044,69.7052135201998,0.));
#98423=CARTESIAN_POINT('Ctrl Pts',(-13.4673907676044,69.7052135201998,12.));
#98424=CARTESIAN_POINT('Ctrl Pts',(-13.4779147665285,69.724516249225,0.));
#98425=CARTESIAN_POINT('Ctrl Pts',(-13.4779147665285,69.724516249225,12.));
#98426=CARTESIAN_POINT('Ctrl Pts',(-13.4884811124748,69.7438497016406,0.));
#98427=CARTESIAN_POINT('Ctrl Pts',(-13.4884811124748,69.7438497016406,12.));
#98428=CARTESIAN_POINT('Ctrl Pts',(-13.4990897985905,69.7632137134249,0.));
#98429=CARTESIAN_POINT('Ctrl Pts',(-13.4990897985905,69.7632137134249,12.));
#98430=CARTESIAN_POINT('Ctrl Pts',(-13.5097408179479,69.7826081213576,0.));
#98431=CARTESIAN_POINT('Ctrl Pts',(-13.5097408179479,69.7826081213576,12.));
#98432=CARTESIAN_POINT('Ctrl Pts',(-13.5204341635507,69.8020327630205,0.));
#98433=CARTESIAN_POINT('Ctrl Pts',(-13.5204341635507,69.8020327630205,12.));
#98434=CARTESIAN_POINT('Ctrl Pts',(-13.5311698283339,69.8214874767944,0.));
#98435=CARTESIAN_POINT('Ctrl Pts',(-13.5311698283339,69.8214874767944,12.));
#98436=CARTESIAN_POINT('Ctrl Pts',(-13.5419478051625,69.840972101856,0.));
#98437=CARTESIAN_POINT('Ctrl Pts',(-13.5419478051625,69.840972101856,12.));
#98438=CARTESIAN_POINT('Ctrl Pts',(-13.5527680868255,69.8604864781706,0.));
#98439=CARTESIAN_POINT('Ctrl Pts',(-13.5527680868255,69.8604864781706,12.));
#98440=CARTESIAN_POINT('Ctrl Pts',(-13.5636306660422,69.8800304464882,0.));
#98441=CARTESIAN_POINT('Ctrl Pts',(-13.5636306660422,69.8800304464882,12.));
#98442=CARTESIAN_POINT('Ctrl Pts',(-13.5745355354657,69.8996038483361,0.));
#98443=CARTESIAN_POINT('Ctrl Pts',(-13.5745355354657,69.8996038483361,12.));
#98444=CARTESIAN_POINT('Ctrl Pts',(-13.5854826876835,69.9192065260108,0.));
#98445=CARTESIAN_POINT('Ctrl Pts',(-13.5854826876835,69.9192065260108,12.));
#98446=CARTESIAN_POINT('Ctrl Pts',(-13.5964721152135,69.9388383225648,0.));
#98447=CARTESIAN_POINT('Ctrl Pts',(-13.5964721152135,69.9388383225648,12.));
#98448=CARTESIAN_POINT('Ctrl Pts',(-13.6075038104999,69.9584990817974,0.));
#98449=CARTESIAN_POINT('Ctrl Pts',(-13.6075038104999,69.9584990817974,12.));
#98450=CARTESIAN_POINT('Ctrl Pts',(-13.6185777659198,69.9781886482528,0.));
#98451=CARTESIAN_POINT('Ctrl Pts',(-13.6185777659198,69.9781886482528,12.));
#98452=CARTESIAN_POINT('Ctrl Pts',(-13.6296939737865,69.9979068672153,0.));
#98453=CARTESIAN_POINT('Ctrl Pts',(-13.6296939737865,69.9979068672153,12.));
#98454=CARTESIAN_POINT('Ctrl Pts',(-13.6408524263496,70.0176535847049,0.));
#98455=CARTESIAN_POINT('Ctrl Pts',(-13.6408524263496,70.0176535847049,12.));
#98456=CARTESIAN_POINT('Ctrl Pts',(-13.6520531157907,70.0374286474677,0.));
#98457=CARTESIAN_POINT('Ctrl Pts',(-13.6520531157907,70.0374286474677,12.));
#98458=CARTESIAN_POINT('Ctrl Pts',(-13.6632960342196,70.0572319029676,0.));
#98459=CARTESIAN_POINT('Ctrl Pts',(-13.6632960342196,70.0572319029676,12.));
#98460=CARTESIAN_POINT('Ctrl Pts',(-13.674581173683,70.0770631993856,0.));
#98461=CARTESIAN_POINT('Ctrl Pts',(-13.674581173683,70.0770631993856,12.));
#98462=CARTESIAN_POINT('Ctrl Pts',(-13.6859085261653,70.0969223856136,0.));
#98463=CARTESIAN_POINT('Ctrl Pts',(-13.6859085261653,70.0969223856136,12.));
#98464=CARTESIAN_POINT('Ctrl Pts',(-13.6972780835897,70.1168093112486,0.));
#98465=CARTESIAN_POINT('Ctrl Pts',(-13.6972780835897,70.1168093112486,12.));
#98466=CARTESIAN_POINT('Ctrl Pts',(-13.7086898378122,70.1367238265825,0.));
#98467=CARTESIAN_POINT('Ctrl Pts',(-13.7086898378122,70.1367238265825,12.));
#98468=CARTESIAN_POINT('Ctrl Pts',(-13.7201437806199,70.156665782595,0.));
#98469=CARTESIAN_POINT('Ctrl Pts',(-13.7201437806199,70.156665782595,12.));
#98470=CARTESIAN_POINT('Ctrl Pts',(-13.7316399037393,70.1766350309518,0.));
#98471=CARTESIAN_POINT('Ctrl Pts',(-13.7316399037393,70.1766350309518,12.));
#98472=CARTESIAN_POINT('Ctrl Pts',(-13.7431781988365,70.1966314239995,0.));
#98473=CARTESIAN_POINT('Ctrl Pts',(-13.7431781988365,70.1966314239995,12.));
#98474=CARTESIAN_POINT('Ctrl Pts',(-13.7547586575181,70.2166548147604,0.));
#98475=CARTESIAN_POINT('Ctrl Pts',(-13.7547586575181,70.2166548147604,12.));
#98476=CARTESIAN_POINT('Ctrl Pts',(-13.7663812713243,70.2367050569216,0.));
#98477=CARTESIAN_POINT('Ctrl Pts',(-13.7663812713243,70.2367050569216,12.));
#98478=CARTESIAN_POINT('Ctrl Pts',(-13.7780460317294,70.2567820048303,0.));
#98479=CARTESIAN_POINT('Ctrl Pts',(-13.7780460317294,70.2567820048303,12.));
#98480=CARTESIAN_POINT('Ctrl Pts',(-13.7897529301491,70.2768855134947,0.));
#98481=CARTESIAN_POINT('Ctrl Pts',(-13.7897529301491,70.2768855134947,12.));
#98482=CARTESIAN_POINT('Ctrl Pts',(-13.8015019579414,70.2970154385774,0.));
#98483=CARTESIAN_POINT('Ctrl Pts',(-13.8015019579414,70.2970154385774,12.));
#98484=CARTESIAN_POINT('Ctrl Pts',(-13.8132931064064,70.3171716363897,0.));
#98485=CARTESIAN_POINT('Ctrl Pts',(-13.8132931064064,70.3171716363897,12.));
#98486=CARTESIAN_POINT('Ctrl Pts',(-13.8251263667791,70.3373539638809,0.));
#98487=CARTESIAN_POINT('Ctrl Pts',(-13.8251263667791,70.3373539638809,12.));
#98488=CARTESIAN_POINT('Ctrl Pts',(-13.8370017302309,70.3575622786335,0.));
#98489=CARTESIAN_POINT('Ctrl Pts',(-13.8370017302309,70.3575622786335,12.));
#98490=CARTESIAN_POINT('Ctrl Pts',(-13.8489191878767,70.3777964388632,0.));
#98491=CARTESIAN_POINT('Ctrl Pts',(-13.8489191878767,70.3777964388632,12.));
#98492=CARTESIAN_POINT('Ctrl Pts',(-13.8608787307752,70.3980563034133,0.));
#98493=CARTESIAN_POINT('Ctrl Pts',(-13.8608787307752,70.3980563034133,12.));
#98494=CARTESIAN_POINT('Ctrl Pts',(-13.8728803499287,70.41834173175,0.));
#98495=CARTESIAN_POINT('Ctrl Pts',(-13.8728803499287,70.41834173175,12.));
#98496=CARTESIAN_POINT('Ctrl Pts',(-13.8849240362763,70.4386525839521,0.));
#98497=CARTESIAN_POINT('Ctrl Pts',(-13.8849240362763,70.4386525839521,12.));
#98498=CARTESIAN_POINT('Ctrl Pts',(-13.8970097806954,70.4589887207073,0.));
#98499=CARTESIAN_POINT('Ctrl Pts',(-13.8970097806954,70.4589887207073,12.));
#98500=CARTESIAN_POINT('Ctrl Pts',(-13.9091375740088,70.4793500033124,0.));
#98501=CARTESIAN_POINT('Ctrl Pts',(-13.9091375740088,70.4793500033124,12.));
#98502=CARTESIAN_POINT('Ctrl Pts',(-13.9213074069853,70.4997362936673,0.));
#98503=CARTESIAN_POINT('Ctrl Pts',(-13.9213074069853,70.4997362936673,12.));
#98504=CARTESIAN_POINT('Ctrl Pts',(-13.9335192703388,70.520147454271,0.));
#98505=CARTESIAN_POINT('Ctrl Pts',(-13.9335192703388,70.520147454271,12.));
#98506=CARTESIAN_POINT('Ctrl Pts',(-13.9457731547215,70.5405833482112,0.));
#98507=CARTESIAN_POINT('Ctrl Pts',(-13.9457731547215,70.5405833482112,12.));
#98508=CARTESIAN_POINT('Ctrl Pts',(-13.958069050726,70.5610438391612,0.));
#98509=CARTESIAN_POINT('Ctrl Pts',(-13.958069050726,70.5610438391612,12.));
#98510=CARTESIAN_POINT('Ctrl Pts',(-13.9704069488917,70.5815287913784,0.));
#98511=CARTESIAN_POINT('Ctrl Pts',(-13.9704069488917,70.5815287913784,12.));
#98512=CARTESIAN_POINT('Ctrl Pts',(-13.9827868397057,70.6020380697005,0.));
#98513=CARTESIAN_POINT('Ctrl Pts',(-13.9827868397057,70.6020380697005,12.));
#98514=CARTESIAN_POINT('Ctrl Pts',(-13.9952087136018,70.6225715395394,0.));
#98515=CARTESIAN_POINT('Ctrl Pts',(-13.9952087136018,70.6225715395394,12.));
#98516=CARTESIAN_POINT('Ctrl Pts',(-14.0076725609537,70.6431290668745,0.));
#98517=CARTESIAN_POINT('Ctrl Pts',(-14.0076725609537,70.6431290668745,12.));
#98518=CARTESIAN_POINT('Ctrl Pts',(-14.020178372077,70.6637105182484,0.));
#98519=CARTESIAN_POINT('Ctrl Pts',(-14.020178372077,70.6637105182484,12.));
#98520=CARTESIAN_POINT('Ctrl Pts',(-14.0327261372362,70.6843157607668,0.));
#98521=CARTESIAN_POINT('Ctrl Pts',(-14.0327261372362,70.6843157607668,12.));
#98522=CARTESIAN_POINT('Ctrl Pts',(-14.0453158466451,70.7049446620928,0.));
#98523=CARTESIAN_POINT('Ctrl Pts',(-14.0453158466451,70.7049446620928,12.));
#98524=CARTESIAN_POINT('Ctrl Pts',(-14.0579474904657,70.7255970904436,0.));
#98525=CARTESIAN_POINT('Ctrl Pts',(-14.0579474904657,70.7255970904436,12.));
#98526=CARTESIAN_POINT('Ctrl Pts',(-14.0706210588016,70.7462729145807,0.));
#98527=CARTESIAN_POINT('Ctrl Pts',(-14.0706210588016,70.7462729145807,12.));
#98528=CARTESIAN_POINT('Ctrl Pts',(-14.0833365416996,70.7669720038077,0.));
#98529=CARTESIAN_POINT('Ctrl Pts',(-14.0833365416996,70.7669720038077,12.));
#98530=CARTESIAN_POINT('Ctrl Pts',(-14.0960939291569,70.7876942279697,0.));
#98531=CARTESIAN_POINT('Ctrl Pts',(-14.0960939291569,70.7876942279697,12.));
#98532=CARTESIAN_POINT('Ctrl Pts',(-14.1088932111214,70.8084394574493,0.));
#98533=CARTESIAN_POINT('Ctrl Pts',(-14.1088932111214,70.8084394574493,12.));
#98534=CARTESIAN_POINT('Ctrl Pts',(-14.1217343774913,70.8292075631621,0.));
#98535=CARTESIAN_POINT('Ctrl Pts',(-14.1217343774913,70.8292075631621,12.));
#98536=CARTESIAN_POINT('Ctrl Pts',(-14.1346174181079,70.8499984165489,0.));
#98537=CARTESIAN_POINT('Ctrl Pts',(-14.1346174181079,70.8499984165489,12.));
#98538=CARTESIAN_POINT('Ctrl Pts',(-14.1475423227568,70.8708118895715,0.));
#98539=CARTESIAN_POINT('Ctrl Pts',(-14.1475423227568,70.8708118895715,12.));
#98540=CARTESIAN_POINT('Ctrl Pts',(-14.1605090811754,70.8916478547132,0.));
#98541=CARTESIAN_POINT('Ctrl Pts',(-14.1605090811754,70.8916478547132,12.));
#98542=CARTESIAN_POINT('Ctrl Pts',(-14.1735176830533,70.9125061849745,0.));
#98543=CARTESIAN_POINT('Ctrl Pts',(-14.1735176830533,70.9125061849745,12.));
#98544=CARTESIAN_POINT('Ctrl Pts',(-14.1865681180321,70.9333867538704,0.));
#98545=CARTESIAN_POINT('Ctrl Pts',(-14.1865681180321,70.9333867538704,12.));
#98546=CARTESIAN_POINT('Ctrl Pts',(-14.1996603756982,70.9542894354216,0.));
#98547=CARTESIAN_POINT('Ctrl Pts',(-14.1996603756982,70.9542894354216,12.));
#98548=CARTESIAN_POINT('Ctrl Pts',(-14.2127944455839,70.9752141041518,0.));
#98549=CARTESIAN_POINT('Ctrl Pts',(-14.2127944455839,70.9752141041518,12.));
#98550=CARTESIAN_POINT('Ctrl Pts',(-14.2259703171737,70.9961606350861,0.));
#98551=CARTESIAN_POINT('Ctrl Pts',(-14.2259703171737,70.9961606350861,12.));
#98552=CARTESIAN_POINT('Ctrl Pts',(-14.2391879799062,71.0171289037488,0.));
#98553=CARTESIAN_POINT('Ctrl Pts',(-14.2391879799062,71.0171289037488,12.));
#98554=CARTESIAN_POINT('Ctrl Pts',(-14.2524474231733,71.0381187861588,0.));
#98555=CARTESIAN_POINT('Ctrl Pts',(-14.2524474231733,71.0381187861588,12.));
#98556=CARTESIAN_POINT('Ctrl Pts',(-14.2657486363139,71.0591301588231,0.));
#98557=CARTESIAN_POINT('Ctrl Pts',(-14.2657486363139,71.0591301588231,12.));
#98558=CARTESIAN_POINT('Ctrl Pts',(-14.2790916086133,71.0801628987332,0.));
#98559=CARTESIAN_POINT('Ctrl Pts',(-14.2790916086133,71.0801628987332,12.));
#98560=CARTESIAN_POINT('Ctrl Pts',(-14.2924763293105,71.1012168833643,0.));
#98561=CARTESIAN_POINT('Ctrl Pts',(-14.2924763293105,71.1012168833643,12.));
#98562=CARTESIAN_POINT('Ctrl Pts',(-14.3059027875994,71.1222919906727,0.));
#98563=CARTESIAN_POINT('Ctrl Pts',(-14.3059027875994,71.1222919906727,12.));
#98564=CARTESIAN_POINT('Ctrl Pts',(-14.3193709726294,71.1433880990929,0.));
#98565=CARTESIAN_POINT('Ctrl Pts',(-14.3193709726294,71.1433880990929,12.));
#98566=CARTESIAN_POINT('Ctrl Pts',(-14.332880873499,71.1645050875308,0.));
#98567=CARTESIAN_POINT('Ctrl Pts',(-14.332880873499,71.1645050875308,12.));
#98568=CARTESIAN_POINT('Ctrl Pts',(-14.3464324792534,71.1856428353593,0.));
#98569=CARTESIAN_POINT('Ctrl Pts',(-14.3464324792534,71.1856428353593,12.));
#98570=CARTESIAN_POINT('Ctrl Pts',(-14.3600257788924,71.2068012224174,0.));
#98571=CARTESIAN_POINT('Ctrl Pts',(-14.3600257788924,71.2068012224174,12.));
#98572=CARTESIAN_POINT('Ctrl Pts',(-14.3736607613722,71.2279801290084,0.));
#98573=CARTESIAN_POINT('Ctrl Pts',(-14.3736607613722,71.2279801290084,12.));
#98574=CARTESIAN_POINT('Ctrl Pts',(-14.3873374156056,71.2491794358958,0.));
#98575=CARTESIAN_POINT('Ctrl Pts',(-14.3873374156056,71.2491794358958,12.));
#98576=CARTESIAN_POINT('Ctrl Pts',(-14.401055730457,71.2703990242988,0.));
#98577=CARTESIAN_POINT('Ctrl Pts',(-14.401055730457,71.2703990242988,12.));
#98578=CARTESIAN_POINT('Ctrl Pts',(-14.4148156947384,71.2916387758861,0.));
#98579=CARTESIAN_POINT('Ctrl Pts',(-14.4148156947384,71.2916387758861,12.));
#98580=CARTESIAN_POINT('Ctrl Pts',(-14.4286172972167,71.312898572777,0.));
#98581=CARTESIAN_POINT('Ctrl Pts',(-14.4286172972167,71.312898572777,12.));
#98582=CARTESIAN_POINT('Ctrl Pts',(-14.4424605266165,71.3341782975386,0.));
#98583=CARTESIAN_POINT('Ctrl Pts',(-14.4424605266165,71.3341782975386,12.));
#98584=CARTESIAN_POINT('Ctrl Pts',(-14.4563453716204,71.3554778331835,0.));
#98585=CARTESIAN_POINT('Ctrl Pts',(-14.4563453716204,71.3554778331835,12.));
#98586=CARTESIAN_POINT('Ctrl Pts',(-14.4702718208651,71.376797063165,0.));
#98587=CARTESIAN_POINT('Ctrl Pts',(-14.4702718208651,71.376797063165,12.));
#98588=CARTESIAN_POINT('Ctrl Pts',(-14.4842398629355,71.3981358713723,0.));
#98589=CARTESIAN_POINT('Ctrl Pts',(-14.4842398629355,71.3981358713723,12.));
#98590=CARTESIAN_POINT('Ctrl Pts',(-14.4982494863718,71.4194941421292,0.));
#98591=CARTESIAN_POINT('Ctrl Pts',(-14.4982494863718,71.4194941421292,12.));
#98592=CARTESIAN_POINT('Ctrl Pts',(-14.5123006796728,71.4408717601923,0.));
#98593=CARTESIAN_POINT('Ctrl Pts',(-14.5123006796728,71.4408717601923,12.));
#98594=CARTESIAN_POINT('Ctrl Pts',(-14.5263934312969,71.4622686107475,0.));
#98595=CARTESIAN_POINT('Ctrl Pts',(-14.5263934312969,71.4622686107475,12.));
#98596=CARTESIAN_POINT('Ctrl Pts',(-14.540527729659,71.4836845794048,0.));
#98597=CARTESIAN_POINT('Ctrl Pts',(-14.540527729659,71.4836845794048,12.));
#98598=CARTESIAN_POINT('Ctrl Pts',(-14.5547035631234,71.5051195521909,0.));
#98599=CARTESIAN_POINT('Ctrl Pts',(-14.5547035631234,71.5051195521909,12.));
#98600=CARTESIAN_POINT('Ctrl Pts',(-14.5689209200091,71.5265734155498,0.));
#98601=CARTESIAN_POINT('Ctrl Pts',(-14.5689209200091,71.5265734155498,12.));
#98602=CARTESIAN_POINT('Ctrl Pts',(-14.5831797885952,71.5480460563447,0.));
#98603=CARTESIAN_POINT('Ctrl Pts',(-14.5831797885952,71.5480460563447,12.));
#98604=CARTESIAN_POINT('Ctrl Pts',(-14.597480157121,71.5695373618562,0.));
#98605=CARTESIAN_POINT('Ctrl Pts',(-14.597480157121,71.5695373618562,12.));
#98606=CARTESIAN_POINT('Ctrl Pts',(-14.6118220137849,71.5910472197813,0.));
#98607=CARTESIAN_POINT('Ctrl Pts',(-14.6118220137849,71.5910472197813,12.));
#98608=CARTESIAN_POINT('Ctrl Pts',(-14.626205346737,71.612575518229,0.));
#98609=CARTESIAN_POINT('Ctrl Pts',(-14.626205346737,71.612575518229,12.));
#98610=CARTESIAN_POINT('Ctrl Pts',(-14.6406301440814,71.6341221457169,0.));
#98611=CARTESIAN_POINT('Ctrl Pts',(-14.6406301440814,71.6341221457169,12.));
#98612=CARTESIAN_POINT('Ctrl Pts',(-14.6550963938829,71.6556869911662,0.));
#98613=CARTESIAN_POINT('Ctrl Pts',(-14.6550963938829,71.6556869911662,12.));
#98614=CARTESIAN_POINT('Ctrl Pts',(-14.6696040841678,71.6772699438963,0.));
#98615=CARTESIAN_POINT('Ctrl Pts',(-14.6696040841678,71.6772699438963,12.));
#98616=CARTESIAN_POINT('Ctrl Pts',(-14.6841532029232,71.6988708936172,0.));
#98617=CARTESIAN_POINT('Ctrl Pts',(-14.6841532029232,71.6988708936172,12.));
#98618=CARTESIAN_POINT('Ctrl Pts',(-14.6987437380901,71.7204897304194,0.));
#98619=CARTESIAN_POINT('Ctrl Pts',(-14.6987437380901,71.7204897304194,12.));
#98620=CARTESIAN_POINT('Ctrl Pts',(-14.7133756775626,71.7421263447719,0.));
#98621=CARTESIAN_POINT('Ctrl Pts',(-14.7133756775626,71.7421263447719,12.));
#98622=CARTESIAN_POINT('Ctrl Pts',(-14.7280490091957,71.7637806275328,0.));
#98623=CARTESIAN_POINT('Ctrl Pts',(-14.7280490091957,71.7637806275328,12.));
#98624=CARTESIAN_POINT('Ctrl Pts',(-14.7427637208073,71.7854524699569,0.));
#98625=CARTESIAN_POINT('Ctrl Pts',(-14.7427637208073,71.7854524699569,12.));
#98626=CARTESIAN_POINT('Ctrl Pts',(-14.7575198001776,71.8071417637017,0.));
#98627=CARTESIAN_POINT('Ctrl Pts',(-14.7575198001776,71.8071417637017,12.));
#98628=CARTESIAN_POINT('Ctrl Pts',(-14.7723172350451,71.8288484008333,0.));
#98629=CARTESIAN_POINT('Ctrl Pts',(-14.7723172350451,71.8288484008333,12.));
#98630=CARTESIAN_POINT('Ctrl Pts',(-14.7871560131017,71.8505722738272,0.));
#98631=CARTESIAN_POINT('Ctrl Pts',(-14.7871560131017,71.8505722738272,12.));
#98632=CARTESIAN_POINT('Ctrl Pts',(-14.8020361219998,71.8723132755446,0.));
#98633=CARTESIAN_POINT('Ctrl Pts',(-14.8020361219998,71.8723132755446,12.));
#98634=CARTESIAN_POINT('Ctrl Pts',(-14.8169575493557,71.8940712992109,0.));
#98635=CARTESIAN_POINT('Ctrl Pts',(-14.8169575493557,71.8940712992109,12.));
#98636=CARTESIAN_POINT('Ctrl Pts',(-14.8319202827482,71.9158462383914,0.));
#98637=CARTESIAN_POINT('Ctrl Pts',(-14.8319202827482,71.9158462383914,12.));
#98638=CARTESIAN_POINT('Ctrl Pts',(-14.8469243097163,71.9376379869678,0.));
#98639=CARTESIAN_POINT('Ctrl Pts',(-14.8469243097163,71.9376379869678,12.));
#98640=CARTESIAN_POINT('Ctrl Pts',(-14.8619696177506,71.9594464391078,0.));
#98641=CARTESIAN_POINT('Ctrl Pts',(-14.8619696177506,71.9594464391078,12.));
#98642=CARTESIAN_POINT('Ctrl Pts',(-14.8770561943014,71.9812714893102,0.));
#98643=CARTESIAN_POINT('Ctrl Pts',(-14.8770561943014,71.9812714893102,12.));
#98644=CARTESIAN_POINT('Ctrl Pts',(-14.8921840267832,72.0031130324529,0.));
#98645=CARTESIAN_POINT('Ctrl Pts',(-14.8921840267832,72.0031130324529,12.));
#98646=CARTESIAN_POINT('Ctrl Pts',(-14.9073531025764,72.0249709638422,0.));
#98647=CARTESIAN_POINT('Ctrl Pts',(-14.9073531025764,72.0249709638422,12.));
#98648=CARTESIAN_POINT('Ctrl Pts',(-14.9225634090268,72.0468451792505,0.));
#98649=CARTESIAN_POINT('Ctrl Pts',(-14.9225634090268,72.0468451792505,12.));
#98650=CARTESIAN_POINT('Ctrl Pts',(-14.9378149334388,72.0687355749807,0.));
#98651=CARTESIAN_POINT('Ctrl Pts',(-14.9378149334388,72.0687355749807,12.));
#98652=CARTESIAN_POINT('Ctrl Pts',(-14.9531076630768,72.0906420478076,0.));
#98653=CARTESIAN_POINT('Ctrl Pts',(-14.9531076630768,72.0906420478076,12.));
#98654=CARTESIAN_POINT('Ctrl Pts',(-14.9684415851698,72.112564494854,0.));
#98655=CARTESIAN_POINT('Ctrl Pts',(-14.9684415851698,72.112564494854,12.));
#98656=CARTESIAN_POINT('Ctrl Pts',(-14.9838166869107,72.1345028134777,0.));
#98657=CARTESIAN_POINT('Ctrl Pts',(-14.9838166869107,72.1345028134777,12.));
#98658=CARTESIAN_POINT('Ctrl Pts',(-14.9992329554537,72.1564569011669,0.));
#98659=CARTESIAN_POINT('Ctrl Pts',(-14.9992329554537,72.1564569011669,12.));
#98660=CARTESIAN_POINT('Ctrl Pts',(-15.0146903779062,72.1784266553953,0.));
#98661=CARTESIAN_POINT('Ctrl Pts',(-15.0146903779062,72.1784266553953,12.));
#98662=CARTESIAN_POINT('Ctrl Pts',(-15.0301889413257,72.2004119736115,0.));
#98663=CARTESIAN_POINT('Ctrl Pts',(-15.0301889413257,72.2004119736115,12.));
#98664=CARTESIAN_POINT('Ctrl Pts',(-15.0457286327331,72.2224127535415,0.));
#98665=CARTESIAN_POINT('Ctrl Pts',(-15.0457286327331,72.2224127535415,12.));
#98666=CARTESIAN_POINT('Ctrl Pts',(-15.0613094391189,72.2444288934262,0.));
#98667=CARTESIAN_POINT('Ctrl Pts',(-15.0613094391189,72.2444288934262,12.));
#98668=CARTESIAN_POINT('Ctrl Pts',(-15.0769313474477,72.2664602922852,0.));
#98669=CARTESIAN_POINT('Ctrl Pts',(-15.0769313474477,72.2664602922852,12.));
#98670=CARTESIAN_POINT('Ctrl Pts',(-15.092594344659,72.2885068501628,0.));
#98671=CARTESIAN_POINT('Ctrl Pts',(-15.092594344659,72.2885068501628,12.));
#98672=CARTESIAN_POINT('Ctrl Pts',(-15.1082984176649,72.3105684683944,0.));
#98673=CARTESIAN_POINT('Ctrl Pts',(-15.1082984176649,72.3105684683944,12.));
#98674=CARTESIAN_POINT('Ctrl Pts',(-15.124043553347,72.3326450490177,0.));
#98675=CARTESIAN_POINT('Ctrl Pts',(-15.124043553347,72.3326450490177,12.));
#98676=CARTESIAN_POINT('Ctrl Pts',(-15.1398297385506,72.3547364941969,0.));
#98677=CARTESIAN_POINT('Ctrl Pts',(-15.1398297385506,72.3547364941969,12.));
#98678=CARTESIAN_POINT('Ctrl Pts',(-15.1556569600745,72.376842705589,0.));
#98679=CARTESIAN_POINT('Ctrl Pts',(-15.1556569600745,72.376842705589,12.));
#98680=CARTESIAN_POINT('Ctrl Pts',(-15.1715252046606,72.3989635838492,0.));
#98681=CARTESIAN_POINT('Ctrl Pts',(-15.1715252046606,72.3989635838492,12.));
#98682=CARTESIAN_POINT('Ctrl Pts',(-15.1874344589726,72.421099027786,0.));
#98683=CARTESIAN_POINT('Ctrl Pts',(-15.1874344589726,72.421099027786,12.));
#98684=CARTESIAN_POINT('Ctrl Pts',(-15.2033847096091,72.4432489350471,0.));
#98685=CARTESIAN_POINT('Ctrl Pts',(-15.2033847096091,72.4432489350471,12.));
#98686=CARTESIAN_POINT('Ctrl Pts',(-15.2193759431373,72.4654132036428,0.));
#98687=CARTESIAN_POINT('Ctrl Pts',(-15.2193759431373,72.4654132036428,12.));
#98688=CARTESIAN_POINT('Ctrl Pts',(-15.235408146116,72.4875917332762,0.));
#98689=CARTESIAN_POINT('Ctrl Pts',(-15.235408146116,72.4875917332762,12.));
#98690=CARTESIAN_POINT('Ctrl Pts',(-15.2514813051172,72.5097844266075,0.));
#98691=CARTESIAN_POINT('Ctrl Pts',(-15.2514813051172,72.5097844266075,12.));
#98692=CARTESIAN_POINT('Ctrl Pts',(-15.2675954067479,72.5319911908917,0.));
#98693=CARTESIAN_POINT('Ctrl Pts',(-15.2675954067479,72.5319911908917,12.));
#98694=CARTESIAN_POINT('Ctrl Pts',(-15.2837504376536,72.5542119383642,0.));
#98695=CARTESIAN_POINT('Ctrl Pts',(-15.2837504376536,72.5542119383642,12.));
#98696=CARTESIAN_POINT('Ctrl Pts',(-15.2999463844661,72.5764465826224,0.));
#98697=CARTESIAN_POINT('Ctrl Pts',(-15.2999463844661,72.5764465826224,12.));
#98698=CARTESIAN_POINT('Ctrl Pts',(-15.3161832337594,72.5986950357677,0.));
#98699=CARTESIAN_POINT('Ctrl Pts',(-15.3161832337594,72.5986950357677,12.));
#98700=CARTESIAN_POINT('Ctrl Pts',(-15.3324609719956,72.6209572051042,0.));
#98701=CARTESIAN_POINT('Ctrl Pts',(-15.3324609719956,72.6209572051042,12.));
#98702=CARTESIAN_POINT('Ctrl Pts',(-15.3487795854745,72.6432329903553,0.));
#98703=CARTESIAN_POINT('Ctrl Pts',(-15.3487795854745,72.6432329903553,12.));
#98704=CARTESIAN_POINT('Ctrl Pts',(-15.3651390602666,72.6655222797801,0.));
#98705=CARTESIAN_POINT('Ctrl Pts',(-15.3651390602666,72.6655222797801,12.));
#98706=CARTESIAN_POINT('Ctrl Pts',(-15.3815393822736,72.687824955772,0.));
#98707=CARTESIAN_POINT('Ctrl Pts',(-15.3815393822736,72.687824955772,12.));
#98708=CARTESIAN_POINT('Ctrl Pts',(-15.3979805373174,72.7101409017716,0.));
#98709=CARTESIAN_POINT('Ctrl Pts',(-15.3979805373174,72.7101409017716,12.));
#98710=CARTESIAN_POINT('Ctrl Pts',(-15.4144625111944,72.7324700089712,0.));
#98711=CARTESIAN_POINT('Ctrl Pts',(-15.4144625111944,72.7324700089712,12.));
#98712=CARTESIAN_POINT('Ctrl Pts',(-15.4309852897844,72.7548121825342,0.));
#98713=CARTESIAN_POINT('Ctrl Pts',(-15.4309852897844,72.7548121825342,12.));
#98714=CARTESIAN_POINT('Ctrl Pts',(-15.4475488590244,72.777167349421,0.));
#98715=CARTESIAN_POINT('Ctrl Pts',(-15.4475488590244,72.777167349421,12.));
#98716=CARTESIAN_POINT('Ctrl Pts',(-15.4641532053281,72.7995354603795,0.));
#98717=CARTESIAN_POINT('Ctrl Pts',(-15.4641532053281,72.7995354603795,12.));
#98718=CARTESIAN_POINT('Ctrl Pts',(-15.4807983165804,72.8219164843279,0.));
#98719=CARTESIAN_POINT('Ctrl Pts',(-15.4807983165804,72.8219164843279,12.));
#98720=CARTESIAN_POINT('Ctrl Pts',(-15.494147009702,72.8398316205897,0.));
#98721=CARTESIAN_POINT('Ctrl Pts',(-15.494147009702,72.8398316205897,12.));
#98722=CARTESIAN_POINT('Ctrl Pts',(-15.5041768663999,72.8532737731759,0.));
#98723=CARTESIAN_POINT('Ctrl Pts',(-15.5041768663999,72.8532737731759,12.));
#98724=CARTESIAN_POINT('Ctrl Pts',(-15.5108715869141,72.8622377860824,0.));
#98725=CARTESIAN_POINT('Ctrl Pts',(-15.5108715869141,72.8622377860824,12.));
#98726=CARTESIAN_POINT('Ctrl Pts',(-15.5142209845168,72.8667204369977,0.));
#98727=CARTESIAN_POINT('Ctrl Pts',(-15.5142209845168,72.8667204369977,12.));
#98728=CARTESIAN_POINT('',(-12.9953224629497,68.7831490561748,0.));
#98729=CARTESIAN_POINT('Ctrl Pts',(-12.9953224629497,68.7831490561748,0.));
#98730=CARTESIAN_POINT('Ctrl Pts',(-12.9969981460277,68.7866525680193,0.));
#98731=CARTESIAN_POINT('Ctrl Pts',(-13.0003537683055,68.7936635625545,0.));
#98732=CARTESIAN_POINT('Ctrl Pts',(-13.0053999700875,68.804191966902,0.));
#98733=CARTESIAN_POINT('Ctrl Pts',(-13.0121537768946,68.8182536653656,0.));
#98734=CARTESIAN_POINT('Ctrl Pts',(-13.0206386039691,68.8358704887468,0.));
#98735=CARTESIAN_POINT('Ctrl Pts',(-13.0291660060107,68.8535269726794,0.));
#98736=CARTESIAN_POINT('Ctrl Pts',(-13.0377359881875,68.8712230321906,0.));
#98737=CARTESIAN_POINT('Ctrl Pts',(-13.0463485518207,68.8889585151585,0.));
#98738=CARTESIAN_POINT('Ctrl Pts',(-13.0550036938813,68.9067332040985,0.));
#98739=CARTESIAN_POINT('Ctrl Pts',(-13.0637014089029,68.9245468449945,0.));
#98740=CARTESIAN_POINT('Ctrl Pts',(-13.072441690283,68.9423991694492,0.));
#98741=CARTESIAN_POINT('Ctrl Pts',(-13.0812245317808,68.9602899187573,0.));
#98742=CARTESIAN_POINT('Ctrl Pts',(-13.090049929053,68.9782188692581,0.));
#98743=CARTESIAN_POINT('Ctrl Pts',(-13.0989178791834,68.9961858241519,0.));
#98744=CARTESIAN_POINT('Ctrl Pts',(-13.1078283799722,69.0141906015113,0.));
#98745=CARTESIAN_POINT('Ctrl Pts',(-13.1167814293497,69.0322330243348,0.));
#98746=CARTESIAN_POINT('Ctrl Pts',(-13.1257770246385,69.0503129081817,0.));
#98747=CARTESIAN_POINT('Ctrl Pts',(-13.1348151621834,69.0684300549477,0.));
#98748=CARTESIAN_POINT('Ctrl Pts',(-13.1438958377404,69.0865842593102,0.));
#98749=CARTESIAN_POINT('Ctrl Pts',(-13.1530190467183,69.1047753127643,0.));
#98750=CARTESIAN_POINT('Ctrl Pts',(-13.1621847844528,69.1230030082573,0.));
#98751=CARTESIAN_POINT('Ctrl Pts',(-13.1713930465133,69.1412671454564,0.));
#98752=CARTESIAN_POINT('Ctrl Pts',(-13.1806438286934,69.1595675305245,0.));
#98753=CARTESIAN_POINT('Ctrl Pts',(-13.1899371268683,69.1779039735996,0.));
#98754=CARTESIAN_POINT('Ctrl Pts',(-13.1992729368928,69.1962762870527,0.));
#98755=CARTESIAN_POINT('Ctrl Pts',(-13.2086512544735,69.2146842833537,0.));
#98756=CARTESIAN_POINT('Ctrl Pts',(-13.2180720750594,69.2331277732861,0.));
#98757=CARTESIAN_POINT('Ctrl Pts',(-13.2275353939051,69.2516065668844,0.));
#98758=CARTESIAN_POINT('Ctrl Pts',(-13.237041206122,69.270120474245,0.));
#98759=CARTESIAN_POINT('Ctrl Pts',(-13.2465895067262,69.2886693063182,0.));
#98760=CARTESIAN_POINT('Ctrl Pts',(-13.2561802906896,69.3072528758518,0.));
#98761=CARTESIAN_POINT('Ctrl Pts',(-13.265813552961,69.3258709977382,0.));
#98762=CARTESIAN_POINT('Ctrl Pts',(-13.2754892884433,69.3445234885065,0.));
#98763=CARTESIAN_POINT('Ctrl Pts',(-13.2852074919766,69.3632101660066,0.));
#98764=CARTESIAN_POINT('Ctrl Pts',(-13.2949681583167,69.3819308490422,0.));
#98765=CARTESIAN_POINT('Ctrl Pts',(-13.3047712821051,69.4006853569511,0.));
#98766=CARTESIAN_POINT('Ctrl Pts',(-13.3146168578743,69.4194735096265,0.));
#98767=CARTESIAN_POINT('Ctrl Pts',(-13.3245048800643,69.4382951276998,0.));
#98768=CARTESIAN_POINT('Ctrl Pts',(-13.3344353430313,69.4571500326673,0.));
#98769=CARTESIAN_POINT('Ctrl Pts',(-13.3444082410543,69.4760380470365,0.));
#98770=CARTESIAN_POINT('Ctrl Pts',(-13.3544235683394,69.4949589944606,0.));
#98771=CARTESIAN_POINT('Ctrl Pts',(-13.3644813190219,69.5139126996675,0.));
#98772=CARTESIAN_POINT('Ctrl Pts',(-13.3745814871665,69.5328989883885,0.));
#98773=CARTESIAN_POINT('Ctrl Pts',(-13.3847240667628,69.5519176872862,0.));
#98774=CARTESIAN_POINT('Ctrl Pts',(-13.3949090517177,69.5709686238724,0.));
#98775=CARTESIAN_POINT('Ctrl Pts',(-13.40513643585,69.5900516264553,0.));
#98776=CARTESIAN_POINT('Ctrl Pts',(-13.4154062129002,69.6091665241765,0.));
#98777=CARTESIAN_POINT('Ctrl Pts',(-13.4257183765341,69.6283131470273,0.));
#98778=CARTESIAN_POINT('Ctrl Pts',(-13.4360729203442,69.6474913258675,0.));
#98779=CARTESIAN_POINT('Ctrl Pts',(-13.4464698378453,69.666700892444,0.));
#98780=CARTESIAN_POINT('Ctrl Pts',(-13.456909122476,69.6859416793885,0.));
#98781=CARTESIAN_POINT('Ctrl Pts',(-13.4673907676044,69.7052135201998,0.));
#98782=CARTESIAN_POINT('Ctrl Pts',(-13.4779147665285,69.724516249225,0.));
#98783=CARTESIAN_POINT('Ctrl Pts',(-13.4884811124748,69.7438497016406,0.));
#98784=CARTESIAN_POINT('Ctrl Pts',(-13.4990897985905,69.7632137134249,0.));
#98785=CARTESIAN_POINT('Ctrl Pts',(-13.5097408179479,69.7826081213576,0.));
#98786=CARTESIAN_POINT('Ctrl Pts',(-13.5204341635507,69.8020327630205,0.));
#98787=CARTESIAN_POINT('Ctrl Pts',(-13.5311698283339,69.8214874767944,0.));
#98788=CARTESIAN_POINT('Ctrl Pts',(-13.5419478051625,69.840972101856,0.));
#98789=CARTESIAN_POINT('Ctrl Pts',(-13.5527680868255,69.8604864781706,0.));
#98790=CARTESIAN_POINT('Ctrl Pts',(-13.5636306660422,69.8800304464882,0.));
#98791=CARTESIAN_POINT('Ctrl Pts',(-13.5745355354657,69.8996038483361,0.));
#98792=CARTESIAN_POINT('Ctrl Pts',(-13.5854826876835,69.9192065260108,0.));
#98793=CARTESIAN_POINT('Ctrl Pts',(-13.5964721152135,69.9388383225648,0.));
#98794=CARTESIAN_POINT('Ctrl Pts',(-13.6075038104999,69.9584990817974,0.));
#98795=CARTESIAN_POINT('Ctrl Pts',(-13.6185777659198,69.9781886482528,0.));
#98796=CARTESIAN_POINT('Ctrl Pts',(-13.6296939737865,69.9979068672153,0.));
#98797=CARTESIAN_POINT('Ctrl Pts',(-13.6408524263496,70.0176535847049,0.));
#98798=CARTESIAN_POINT('Ctrl Pts',(-13.6520531157907,70.0374286474677,0.));
#98799=CARTESIAN_POINT('Ctrl Pts',(-13.6632960342196,70.0572319029676,0.));
#98800=CARTESIAN_POINT('Ctrl Pts',(-13.674581173683,70.0770631993856,0.));
#98801=CARTESIAN_POINT('Ctrl Pts',(-13.6859085261653,70.0969223856136,0.));
#98802=CARTESIAN_POINT('Ctrl Pts',(-13.6972780835897,70.1168093112486,0.));
#98803=CARTESIAN_POINT('Ctrl Pts',(-13.7086898378122,70.1367238265825,0.));
#98804=CARTESIAN_POINT('Ctrl Pts',(-13.7201437806199,70.156665782595,0.));
#98805=CARTESIAN_POINT('Ctrl Pts',(-13.7316399037393,70.1766350309518,0.));
#98806=CARTESIAN_POINT('Ctrl Pts',(-13.7431781988365,70.1966314239995,0.));
#98807=CARTESIAN_POINT('Ctrl Pts',(-13.7547586575181,70.2166548147604,0.));
#98808=CARTESIAN_POINT('Ctrl Pts',(-13.7663812713243,70.2367050569216,0.));
#98809=CARTESIAN_POINT('Ctrl Pts',(-13.7780460317294,70.2567820048303,0.));
#98810=CARTESIAN_POINT('Ctrl Pts',(-13.7897529301491,70.2768855134947,0.));
#98811=CARTESIAN_POINT('Ctrl Pts',(-13.8015019579414,70.2970154385774,0.));
#98812=CARTESIAN_POINT('Ctrl Pts',(-13.8132931064064,70.3171716363897,0.));
#98813=CARTESIAN_POINT('Ctrl Pts',(-13.8251263667791,70.3373539638809,0.));
#98814=CARTESIAN_POINT('Ctrl Pts',(-13.8370017302309,70.3575622786335,0.));
#98815=CARTESIAN_POINT('Ctrl Pts',(-13.8489191878767,70.3777964388632,0.));
#98816=CARTESIAN_POINT('Ctrl Pts',(-13.8608787307752,70.3980563034133,0.));
#98817=CARTESIAN_POINT('Ctrl Pts',(-13.8728803499287,70.41834173175,0.));
#98818=CARTESIAN_POINT('Ctrl Pts',(-13.8849240362763,70.4386525839521,0.));
#98819=CARTESIAN_POINT('Ctrl Pts',(-13.8970097806954,70.4589887207073,0.));
#98820=CARTESIAN_POINT('Ctrl Pts',(-13.9091375740088,70.4793500033124,0.));
#98821=CARTESIAN_POINT('Ctrl Pts',(-13.9213074069853,70.4997362936673,0.));
#98822=CARTESIAN_POINT('Ctrl Pts',(-13.9335192703388,70.520147454271,0.));
#98823=CARTESIAN_POINT('Ctrl Pts',(-13.9457731547215,70.5405833482112,0.));
#98824=CARTESIAN_POINT('Ctrl Pts',(-13.958069050726,70.5610438391612,0.));
#98825=CARTESIAN_POINT('Ctrl Pts',(-13.9704069488917,70.5815287913784,0.));
#98826=CARTESIAN_POINT('Ctrl Pts',(-13.9827868397057,70.6020380697005,0.));
#98827=CARTESIAN_POINT('Ctrl Pts',(-13.9952087136018,70.6225715395394,0.));
#98828=CARTESIAN_POINT('Ctrl Pts',(-14.0076725609537,70.6431290668745,0.));
#98829=CARTESIAN_POINT('Ctrl Pts',(-14.020178372077,70.6637105182484,0.));
#98830=CARTESIAN_POINT('Ctrl Pts',(-14.0327261372362,70.6843157607668,0.));
#98831=CARTESIAN_POINT('Ctrl Pts',(-14.0453158466451,70.7049446620928,0.));
#98832=CARTESIAN_POINT('Ctrl Pts',(-14.0579474904657,70.7255970904436,0.));
#98833=CARTESIAN_POINT('Ctrl Pts',(-14.0706210588016,70.7462729145807,0.));
#98834=CARTESIAN_POINT('Ctrl Pts',(-14.0833365416996,70.7669720038077,0.));
#98835=CARTESIAN_POINT('Ctrl Pts',(-14.0960939291569,70.7876942279697,0.));
#98836=CARTESIAN_POINT('Ctrl Pts',(-14.1088932111214,70.8084394574493,0.));
#98837=CARTESIAN_POINT('Ctrl Pts',(-14.1217343774913,70.8292075631621,0.));
#98838=CARTESIAN_POINT('Ctrl Pts',(-14.1346174181079,70.8499984165489,0.));
#98839=CARTESIAN_POINT('Ctrl Pts',(-14.1475423227568,70.8708118895715,0.));
#98840=CARTESIAN_POINT('Ctrl Pts',(-14.1605090811754,70.8916478547132,0.));
#98841=CARTESIAN_POINT('Ctrl Pts',(-14.1735176830533,70.9125061849745,0.));
#98842=CARTESIAN_POINT('Ctrl Pts',(-14.1865681180321,70.9333867538704,0.));
#98843=CARTESIAN_POINT('Ctrl Pts',(-14.1996603756982,70.9542894354216,0.));
#98844=CARTESIAN_POINT('Ctrl Pts',(-14.2127944455839,70.9752141041518,0.));
#98845=CARTESIAN_POINT('Ctrl Pts',(-14.2259703171737,70.9961606350861,0.));
#98846=CARTESIAN_POINT('Ctrl Pts',(-14.2391879799062,71.0171289037488,0.));
#98847=CARTESIAN_POINT('Ctrl Pts',(-14.2524474231733,71.0381187861588,0.));
#98848=CARTESIAN_POINT('Ctrl Pts',(-14.2657486363139,71.0591301588231,0.));
#98849=CARTESIAN_POINT('Ctrl Pts',(-14.2790916086133,71.0801628987332,0.));
#98850=CARTESIAN_POINT('Ctrl Pts',(-14.2924763293105,71.1012168833643,0.));
#98851=CARTESIAN_POINT('Ctrl Pts',(-14.3059027875994,71.1222919906727,0.));
#98852=CARTESIAN_POINT('Ctrl Pts',(-14.3193709726294,71.1433880990929,0.));
#98853=CARTESIAN_POINT('Ctrl Pts',(-14.332880873499,71.1645050875308,0.));
#98854=CARTESIAN_POINT('Ctrl Pts',(-14.3464324792534,71.1856428353593,0.));
#98855=CARTESIAN_POINT('Ctrl Pts',(-14.3600257788924,71.2068012224174,0.));
#98856=CARTESIAN_POINT('Ctrl Pts',(-14.3736607613722,71.2279801290084,0.));
#98857=CARTESIAN_POINT('Ctrl Pts',(-14.3873374156056,71.2491794358958,0.));
#98858=CARTESIAN_POINT('Ctrl Pts',(-14.401055730457,71.2703990242988,0.));
#98859=CARTESIAN_POINT('Ctrl Pts',(-14.4148156947384,71.2916387758861,0.));
#98860=CARTESIAN_POINT('Ctrl Pts',(-14.4286172972167,71.312898572777,0.));
#98861=CARTESIAN_POINT('Ctrl Pts',(-14.4424605266165,71.3341782975386,0.));
#98862=CARTESIAN_POINT('Ctrl Pts',(-14.4563453716204,71.3554778331835,0.));
#98863=CARTESIAN_POINT('Ctrl Pts',(-14.4702718208651,71.376797063165,0.));
#98864=CARTESIAN_POINT('Ctrl Pts',(-14.4842398629355,71.3981358713723,0.));
#98865=CARTESIAN_POINT('Ctrl Pts',(-14.4982494863718,71.4194941421292,0.));
#98866=CARTESIAN_POINT('Ctrl Pts',(-14.5123006796728,71.4408717601923,0.));
#98867=CARTESIAN_POINT('Ctrl Pts',(-14.5263934312969,71.4622686107475,0.));
#98868=CARTESIAN_POINT('Ctrl Pts',(-14.540527729659,71.4836845794048,0.));
#98869=CARTESIAN_POINT('Ctrl Pts',(-14.5547035631234,71.5051195521909,0.));
#98870=CARTESIAN_POINT('Ctrl Pts',(-14.5689209200091,71.5265734155498,0.));
#98871=CARTESIAN_POINT('Ctrl Pts',(-14.5831797885952,71.5480460563447,0.));
#98872=CARTESIAN_POINT('Ctrl Pts',(-14.597480157121,71.5695373618562,0.));
#98873=CARTESIAN_POINT('Ctrl Pts',(-14.6118220137849,71.5910472197813,0.));
#98874=CARTESIAN_POINT('Ctrl Pts',(-14.626205346737,71.612575518229,0.));
#98875=CARTESIAN_POINT('Ctrl Pts',(-14.6406301440814,71.6341221457169,0.));
#98876=CARTESIAN_POINT('Ctrl Pts',(-14.6550963938829,71.6556869911662,0.));
#98877=CARTESIAN_POINT('Ctrl Pts',(-14.6696040841678,71.6772699438963,0.));
#98878=CARTESIAN_POINT('Ctrl Pts',(-14.6841532029232,71.6988708936172,0.));
#98879=CARTESIAN_POINT('Ctrl Pts',(-14.6987437380901,71.7204897304194,0.));
#98880=CARTESIAN_POINT('Ctrl Pts',(-14.7133756775626,71.7421263447719,0.));
#98881=CARTESIAN_POINT('Ctrl Pts',(-14.7280490091957,71.7637806275328,0.));
#98882=CARTESIAN_POINT('Ctrl Pts',(-14.7427637208073,71.7854524699569,0.));
#98883=CARTESIAN_POINT('Ctrl Pts',(-14.7575198001776,71.8071417637017,0.));
#98884=CARTESIAN_POINT('Ctrl Pts',(-14.7723172350451,71.8288484008333,0.));
#98885=CARTESIAN_POINT('Ctrl Pts',(-14.7871560131017,71.8505722738272,0.));
#98886=CARTESIAN_POINT('Ctrl Pts',(-14.8020361219998,71.8723132755446,0.));
#98887=CARTESIAN_POINT('Ctrl Pts',(-14.8169575493557,71.8940712992109,0.));
#98888=CARTESIAN_POINT('Ctrl Pts',(-14.8319202827482,71.9158462383914,0.));
#98889=CARTESIAN_POINT('Ctrl Pts',(-14.8469243097163,71.9376379869678,0.));
#98890=CARTESIAN_POINT('Ctrl Pts',(-14.8619696177506,71.9594464391078,0.));
#98891=CARTESIAN_POINT('Ctrl Pts',(-14.8770561943014,71.9812714893102,0.));
#98892=CARTESIAN_POINT('Ctrl Pts',(-14.8921840267832,72.0031130324529,0.));
#98893=CARTESIAN_POINT('Ctrl Pts',(-14.9073531025764,72.0249709638422,0.));
#98894=CARTESIAN_POINT('Ctrl Pts',(-14.9225634090268,72.0468451792505,0.));
#98895=CARTESIAN_POINT('Ctrl Pts',(-14.9378149334388,72.0687355749807,0.));
#98896=CARTESIAN_POINT('Ctrl Pts',(-14.9531076630768,72.0906420478076,0.));
#98897=CARTESIAN_POINT('Ctrl Pts',(-14.9684415851698,72.112564494854,0.));
#98898=CARTESIAN_POINT('Ctrl Pts',(-14.9838166869107,72.1345028134777,0.));
#98899=CARTESIAN_POINT('Ctrl Pts',(-14.9992329554537,72.1564569011669,0.));
#98900=CARTESIAN_POINT('Ctrl Pts',(-15.0146903779062,72.1784266553953,0.));
#98901=CARTESIAN_POINT('Ctrl Pts',(-15.0301889413257,72.2004119736115,0.));
#98902=CARTESIAN_POINT('Ctrl Pts',(-15.0457286327331,72.2224127535415,0.));
#98903=CARTESIAN_POINT('Ctrl Pts',(-15.0613094391189,72.2444288934262,0.));
#98904=CARTESIAN_POINT('Ctrl Pts',(-15.0769313474477,72.2664602922852,0.));
#98905=CARTESIAN_POINT('Ctrl Pts',(-15.092594344659,72.2885068501628,0.));
#98906=CARTESIAN_POINT('Ctrl Pts',(-15.1082984176649,72.3105684683944,0.));
#98907=CARTESIAN_POINT('Ctrl Pts',(-15.124043553347,72.3326450490177,0.));
#98908=CARTESIAN_POINT('Ctrl Pts',(-15.1398297385506,72.3547364941969,0.));
#98909=CARTESIAN_POINT('Ctrl Pts',(-15.1556569600745,72.376842705589,0.));
#98910=CARTESIAN_POINT('Ctrl Pts',(-15.1715252046606,72.3989635838492,0.));
#98911=CARTESIAN_POINT('Ctrl Pts',(-15.1874344589726,72.421099027786,0.));
#98912=CARTESIAN_POINT('Ctrl Pts',(-15.2033847096091,72.4432489350471,0.));
#98913=CARTESIAN_POINT('Ctrl Pts',(-15.2193759431373,72.4654132036428,0.));
#98914=CARTESIAN_POINT('Ctrl Pts',(-15.235408146116,72.4875917332762,0.));
#98915=CARTESIAN_POINT('Ctrl Pts',(-15.2514813051172,72.5097844266075,0.));
#98916=CARTESIAN_POINT('Ctrl Pts',(-15.2675954067479,72.5319911908917,0.));
#98917=CARTESIAN_POINT('Ctrl Pts',(-15.2837504376536,72.5542119383642,0.));
#98918=CARTESIAN_POINT('Ctrl Pts',(-15.297633502478,72.5732713370618,0.));
#98919=CARTESIAN_POINT('Ctrl Pts',(-15.3082994603539,72.5878912620439,0.));
#98920=CARTESIAN_POINT('Ctrl Pts',(-15.3157301930682,72.5980655789635,0.));
#98921=CARTESIAN_POINT('Ctrl Pts',(-15.3199137230129,72.6037902604921,0.));
#98922=CARTESIAN_POINT('Ctrl Pts',(-15.3208442077189,72.6050633494351,0.));
#98923=CARTESIAN_POINT('',(-12.9953224629497,68.7831490561748,12.));
#98924=CARTESIAN_POINT('',(-12.9953224629497,68.7831490561748,0.));
#98925=CARTESIAN_POINT('Ctrl Pts',(-15.320844207719,72.6050633494352,12.));
#98926=CARTESIAN_POINT('Ctrl Pts',(-15.319913723013,72.6037902604922,12.));
#98927=CARTESIAN_POINT('Ctrl Pts',(-15.3157301930682,72.5980655789636,12.));
#98928=CARTESIAN_POINT('Ctrl Pts',(-15.308299460354,72.5878912620439,12.));
#98929=CARTESIAN_POINT('Ctrl Pts',(-15.297633502478,72.5732713370618,12.));
#98930=CARTESIAN_POINT('Ctrl Pts',(-15.2837504376536,72.5542119383642,12.));
#98931=CARTESIAN_POINT('Ctrl Pts',(-15.2675954067479,72.5319911908917,12.));
#98932=CARTESIAN_POINT('Ctrl Pts',(-15.2514813051172,72.5097844266075,12.));
#98933=CARTESIAN_POINT('Ctrl Pts',(-15.235408146116,72.4875917332762,12.));
#98934=CARTESIAN_POINT('Ctrl Pts',(-15.2193759431373,72.4654132036428,12.));
#98935=CARTESIAN_POINT('Ctrl Pts',(-15.2033847096091,72.4432489350471,12.));
#98936=CARTESIAN_POINT('Ctrl Pts',(-15.1874344589726,72.421099027786,12.));
#98937=CARTESIAN_POINT('Ctrl Pts',(-15.1715252046606,72.3989635838492,12.));
#98938=CARTESIAN_POINT('Ctrl Pts',(-15.1556569600745,72.376842705589,12.));
#98939=CARTESIAN_POINT('Ctrl Pts',(-15.1398297385506,72.3547364941969,12.));
#98940=CARTESIAN_POINT('Ctrl Pts',(-15.124043553347,72.3326450490177,12.));
#98941=CARTESIAN_POINT('Ctrl Pts',(-15.1082984176649,72.3105684683944,12.));
#98942=CARTESIAN_POINT('Ctrl Pts',(-15.092594344659,72.2885068501628,12.));
#98943=CARTESIAN_POINT('Ctrl Pts',(-15.0769313474477,72.2664602922852,12.));
#98944=CARTESIAN_POINT('Ctrl Pts',(-15.0613094391189,72.2444288934262,12.));
#98945=CARTESIAN_POINT('Ctrl Pts',(-15.0457286327331,72.2224127535415,12.));
#98946=CARTESIAN_POINT('Ctrl Pts',(-15.0301889413257,72.2004119736115,12.));
#98947=CARTESIAN_POINT('Ctrl Pts',(-15.0146903779062,72.1784266553953,12.));
#98948=CARTESIAN_POINT('Ctrl Pts',(-14.9992329554537,72.1564569011669,12.));
#98949=CARTESIAN_POINT('Ctrl Pts',(-14.9838166869107,72.1345028134777,12.));
#98950=CARTESIAN_POINT('Ctrl Pts',(-14.9684415851698,72.112564494854,12.));
#98951=CARTESIAN_POINT('Ctrl Pts',(-14.9531076630768,72.0906420478076,12.));
#98952=CARTESIAN_POINT('Ctrl Pts',(-14.9378149334388,72.0687355749807,12.));
#98953=CARTESIAN_POINT('Ctrl Pts',(-14.9225634090268,72.0468451792505,12.));
#98954=CARTESIAN_POINT('Ctrl Pts',(-14.9073531025764,72.0249709638422,12.));
#98955=CARTESIAN_POINT('Ctrl Pts',(-14.8921840267832,72.0031130324529,12.));
#98956=CARTESIAN_POINT('Ctrl Pts',(-14.8770561943014,71.9812714893102,12.));
#98957=CARTESIAN_POINT('Ctrl Pts',(-14.8619696177506,71.9594464391078,12.));
#98958=CARTESIAN_POINT('Ctrl Pts',(-14.8469243097163,71.9376379869678,12.));
#98959=CARTESIAN_POINT('Ctrl Pts',(-14.8319202827482,71.9158462383914,12.));
#98960=CARTESIAN_POINT('Ctrl Pts',(-14.8169575493557,71.8940712992109,12.));
#98961=CARTESIAN_POINT('Ctrl Pts',(-14.8020361219998,71.8723132755446,12.));
#98962=CARTESIAN_POINT('Ctrl Pts',(-14.7871560131017,71.8505722738272,12.));
#98963=CARTESIAN_POINT('Ctrl Pts',(-14.7723172350451,71.8288484008333,12.));
#98964=CARTESIAN_POINT('Ctrl Pts',(-14.7575198001776,71.8071417637017,12.));
#98965=CARTESIAN_POINT('Ctrl Pts',(-14.7427637208073,71.7854524699569,12.));
#98966=CARTESIAN_POINT('Ctrl Pts',(-14.7280490091957,71.7637806275328,12.));
#98967=CARTESIAN_POINT('Ctrl Pts',(-14.7133756775626,71.7421263447719,12.));
#98968=CARTESIAN_POINT('Ctrl Pts',(-14.6987437380901,71.7204897304194,12.));
#98969=CARTESIAN_POINT('Ctrl Pts',(-14.6841532029232,71.6988708936172,12.));
#98970=CARTESIAN_POINT('Ctrl Pts',(-14.6696040841678,71.6772699438963,12.));
#98971=CARTESIAN_POINT('Ctrl Pts',(-14.6550963938829,71.6556869911662,12.));
#98972=CARTESIAN_POINT('Ctrl Pts',(-14.6406301440814,71.6341221457169,12.));
#98973=CARTESIAN_POINT('Ctrl Pts',(-14.626205346737,71.612575518229,12.));
#98974=CARTESIAN_POINT('Ctrl Pts',(-14.6118220137849,71.5910472197813,12.));
#98975=CARTESIAN_POINT('Ctrl Pts',(-14.597480157121,71.5695373618562,12.));
#98976=CARTESIAN_POINT('Ctrl Pts',(-14.5831797885952,71.5480460563447,12.));
#98977=CARTESIAN_POINT('Ctrl Pts',(-14.5689209200091,71.5265734155498,12.));
#98978=CARTESIAN_POINT('Ctrl Pts',(-14.5547035631234,71.5051195521909,12.));
#98979=CARTESIAN_POINT('Ctrl Pts',(-14.540527729659,71.4836845794048,12.));
#98980=CARTESIAN_POINT('Ctrl Pts',(-14.5263934312969,71.4622686107475,12.));
#98981=CARTESIAN_POINT('Ctrl Pts',(-14.5123006796728,71.4408717601923,12.));
#98982=CARTESIAN_POINT('Ctrl Pts',(-14.4982494863718,71.4194941421292,12.));
#98983=CARTESIAN_POINT('Ctrl Pts',(-14.4842398629355,71.3981358713723,12.));
#98984=CARTESIAN_POINT('Ctrl Pts',(-14.4702718208651,71.376797063165,12.));
#98985=CARTESIAN_POINT('Ctrl Pts',(-14.4563453716204,71.3554778331835,12.));
#98986=CARTESIAN_POINT('Ctrl Pts',(-14.4424605266165,71.3341782975386,12.));
#98987=CARTESIAN_POINT('Ctrl Pts',(-14.4286172972167,71.312898572777,12.));
#98988=CARTESIAN_POINT('Ctrl Pts',(-14.4148156947384,71.2916387758861,12.));
#98989=CARTESIAN_POINT('Ctrl Pts',(-14.401055730457,71.2703990242988,12.));
#98990=CARTESIAN_POINT('Ctrl Pts',(-14.3873374156056,71.2491794358958,12.));
#98991=CARTESIAN_POINT('Ctrl Pts',(-14.3736607613722,71.2279801290084,12.));
#98992=CARTESIAN_POINT('Ctrl Pts',(-14.3600257788924,71.2068012224174,12.));
#98993=CARTESIAN_POINT('Ctrl Pts',(-14.3464324792534,71.1856428353593,12.));
#98994=CARTESIAN_POINT('Ctrl Pts',(-14.332880873499,71.1645050875308,12.));
#98995=CARTESIAN_POINT('Ctrl Pts',(-14.3193709726294,71.1433880990929,12.));
#98996=CARTESIAN_POINT('Ctrl Pts',(-14.3059027875994,71.1222919906727,12.));
#98997=CARTESIAN_POINT('Ctrl Pts',(-14.2924763293105,71.1012168833643,12.));
#98998=CARTESIAN_POINT('Ctrl Pts',(-14.2790916086133,71.0801628987332,12.));
#98999=CARTESIAN_POINT('Ctrl Pts',(-14.2657486363139,71.0591301588231,12.));
#99000=CARTESIAN_POINT('Ctrl Pts',(-14.2524474231733,71.0381187861588,12.));
#99001=CARTESIAN_POINT('Ctrl Pts',(-14.2391879799062,71.0171289037488,12.));
#99002=CARTESIAN_POINT('Ctrl Pts',(-14.2259703171737,70.9961606350861,12.));
#99003=CARTESIAN_POINT('Ctrl Pts',(-14.2127944455839,70.9752141041518,12.));
#99004=CARTESIAN_POINT('Ctrl Pts',(-14.1996603756982,70.9542894354216,12.));
#99005=CARTESIAN_POINT('Ctrl Pts',(-14.1865681180321,70.9333867538704,12.));
#99006=CARTESIAN_POINT('Ctrl Pts',(-14.1735176830533,70.9125061849745,12.));
#99007=CARTESIAN_POINT('Ctrl Pts',(-14.1605090811754,70.8916478547132,12.));
#99008=CARTESIAN_POINT('Ctrl Pts',(-14.1475423227568,70.8708118895715,12.));
#99009=CARTESIAN_POINT('Ctrl Pts',(-14.1346174181079,70.8499984165489,12.));
#99010=CARTESIAN_POINT('Ctrl Pts',(-14.1217343774913,70.8292075631621,12.));
#99011=CARTESIAN_POINT('Ctrl Pts',(-14.1088932111214,70.8084394574493,12.));
#99012=CARTESIAN_POINT('Ctrl Pts',(-14.0960939291569,70.7876942279697,12.));
#99013=CARTESIAN_POINT('Ctrl Pts',(-14.0833365416996,70.7669720038077,12.));
#99014=CARTESIAN_POINT('Ctrl Pts',(-14.0706210588016,70.7462729145807,12.));
#99015=CARTESIAN_POINT('Ctrl Pts',(-14.0579474904657,70.7255970904436,12.));
#99016=CARTESIAN_POINT('Ctrl Pts',(-14.0453158466451,70.7049446620928,12.));
#99017=CARTESIAN_POINT('Ctrl Pts',(-14.0327261372362,70.6843157607668,12.));
#99018=CARTESIAN_POINT('Ctrl Pts',(-14.020178372077,70.6637105182484,12.));
#99019=CARTESIAN_POINT('Ctrl Pts',(-14.0076725609537,70.6431290668745,12.));
#99020=CARTESIAN_POINT('Ctrl Pts',(-13.9952087136018,70.6225715395394,12.));
#99021=CARTESIAN_POINT('Ctrl Pts',(-13.9827868397057,70.6020380697005,12.));
#99022=CARTESIAN_POINT('Ctrl Pts',(-13.9704069488917,70.5815287913784,12.));
#99023=CARTESIAN_POINT('Ctrl Pts',(-13.958069050726,70.5610438391612,12.));
#99024=CARTESIAN_POINT('Ctrl Pts',(-13.9457731547215,70.5405833482112,12.));
#99025=CARTESIAN_POINT('Ctrl Pts',(-13.9335192703388,70.520147454271,12.));
#99026=CARTESIAN_POINT('Ctrl Pts',(-13.9213074069853,70.4997362936673,12.));
#99027=CARTESIAN_POINT('Ctrl Pts',(-13.9091375740088,70.4793500033124,12.));
#99028=CARTESIAN_POINT('Ctrl Pts',(-13.8970097806954,70.4589887207073,12.));
#99029=CARTESIAN_POINT('Ctrl Pts',(-13.8849240362763,70.4386525839521,12.));
#99030=CARTESIAN_POINT('Ctrl Pts',(-13.8728803499287,70.41834173175,12.));
#99031=CARTESIAN_POINT('Ctrl Pts',(-13.8608787307752,70.3980563034133,12.));
#99032=CARTESIAN_POINT('Ctrl Pts',(-13.8489191878767,70.3777964388632,12.));
#99033=CARTESIAN_POINT('Ctrl Pts',(-13.8370017302309,70.3575622786335,12.));
#99034=CARTESIAN_POINT('Ctrl Pts',(-13.8251263667791,70.3373539638809,12.));
#99035=CARTESIAN_POINT('Ctrl Pts',(-13.8132931064064,70.3171716363897,12.));
#99036=CARTESIAN_POINT('Ctrl Pts',(-13.8015019579414,70.2970154385774,12.));
#99037=CARTESIAN_POINT('Ctrl Pts',(-13.7897529301491,70.2768855134947,12.));
#99038=CARTESIAN_POINT('Ctrl Pts',(-13.7780460317294,70.2567820048303,12.));
#99039=CARTESIAN_POINT('Ctrl Pts',(-13.7663812713243,70.2367050569216,12.));
#99040=CARTESIAN_POINT('Ctrl Pts',(-13.7547586575181,70.2166548147604,12.));
#99041=CARTESIAN_POINT('Ctrl Pts',(-13.7431781988365,70.1966314239995,12.));
#99042=CARTESIAN_POINT('Ctrl Pts',(-13.7316399037393,70.1766350309518,12.));
#99043=CARTESIAN_POINT('Ctrl Pts',(-13.7201437806199,70.156665782595,12.));
#99044=CARTESIAN_POINT('Ctrl Pts',(-13.7086898378122,70.1367238265825,12.));
#99045=CARTESIAN_POINT('Ctrl Pts',(-13.6972780835897,70.1168093112486,12.));
#99046=CARTESIAN_POINT('Ctrl Pts',(-13.6859085261653,70.0969223856136,12.));
#99047=CARTESIAN_POINT('Ctrl Pts',(-13.674581173683,70.0770631993856,12.));
#99048=CARTESIAN_POINT('Ctrl Pts',(-13.6632960342196,70.0572319029676,12.));
#99049=CARTESIAN_POINT('Ctrl Pts',(-13.6520531157907,70.0374286474677,12.));
#99050=CARTESIAN_POINT('Ctrl Pts',(-13.6408524263496,70.0176535847049,12.));
#99051=CARTESIAN_POINT('Ctrl Pts',(-13.6296939737865,69.9979068672153,12.));
#99052=CARTESIAN_POINT('Ctrl Pts',(-13.6185777659198,69.9781886482528,12.));
#99053=CARTESIAN_POINT('Ctrl Pts',(-13.6075038104999,69.9584990817974,12.));
#99054=CARTESIAN_POINT('Ctrl Pts',(-13.5964721152135,69.9388383225648,12.));
#99055=CARTESIAN_POINT('Ctrl Pts',(-13.5854826876835,69.9192065260108,12.));
#99056=CARTESIAN_POINT('Ctrl Pts',(-13.5745355354657,69.8996038483361,12.));
#99057=CARTESIAN_POINT('Ctrl Pts',(-13.5636306660422,69.8800304464882,12.));
#99058=CARTESIAN_POINT('Ctrl Pts',(-13.5527680868255,69.8604864781706,12.));
#99059=CARTESIAN_POINT('Ctrl Pts',(-13.5419478051625,69.840972101856,12.));
#99060=CARTESIAN_POINT('Ctrl Pts',(-13.5311698283339,69.8214874767944,12.));
#99061=CARTESIAN_POINT('Ctrl Pts',(-13.5204341635507,69.8020327630205,12.));
#99062=CARTESIAN_POINT('Ctrl Pts',(-13.5097408179479,69.7826081213576,12.));
#99063=CARTESIAN_POINT('Ctrl Pts',(-13.4990897985905,69.7632137134249,12.));
#99064=CARTESIAN_POINT('Ctrl Pts',(-13.4884811124748,69.7438497016406,12.));
#99065=CARTESIAN_POINT('Ctrl Pts',(-13.4779147665285,69.724516249225,12.));
#99066=CARTESIAN_POINT('Ctrl Pts',(-13.4673907676044,69.7052135201998,12.));
#99067=CARTESIAN_POINT('Ctrl Pts',(-13.456909122476,69.6859416793885,12.));
#99068=CARTESIAN_POINT('Ctrl Pts',(-13.4464698378453,69.666700892444,12.));
#99069=CARTESIAN_POINT('Ctrl Pts',(-13.4360729203442,69.6474913258675,12.));
#99070=CARTESIAN_POINT('Ctrl Pts',(-13.4257183765341,69.6283131470273,12.));
#99071=CARTESIAN_POINT('Ctrl Pts',(-13.4154062129002,69.6091665241765,12.));
#99072=CARTESIAN_POINT('Ctrl Pts',(-13.40513643585,69.5900516264553,12.));
#99073=CARTESIAN_POINT('Ctrl Pts',(-13.3949090517177,69.5709686238724,12.));
#99074=CARTESIAN_POINT('Ctrl Pts',(-13.3847240667628,69.5519176872862,12.));
#99075=CARTESIAN_POINT('Ctrl Pts',(-13.3745814871665,69.5328989883885,12.));
#99076=CARTESIAN_POINT('Ctrl Pts',(-13.3644813190219,69.5139126996675,12.));
#99077=CARTESIAN_POINT('Ctrl Pts',(-13.3544235683394,69.4949589944606,12.));
#99078=CARTESIAN_POINT('Ctrl Pts',(-13.3444082410543,69.4760380470365,12.));
#99079=CARTESIAN_POINT('Ctrl Pts',(-13.3344353430313,69.4571500326673,12.));
#99080=CARTESIAN_POINT('Ctrl Pts',(-13.3245048800643,69.4382951276998,12.));
#99081=CARTESIAN_POINT('Ctrl Pts',(-13.3146168578743,69.4194735096265,12.));
#99082=CARTESIAN_POINT('Ctrl Pts',(-13.3047712821051,69.4006853569511,12.));
#99083=CARTESIAN_POINT('Ctrl Pts',(-13.2949681583167,69.3819308490422,12.));
#99084=CARTESIAN_POINT('Ctrl Pts',(-13.2852074919766,69.3632101660066,12.));
#99085=CARTESIAN_POINT('Ctrl Pts',(-13.2754892884433,69.3445234885065,12.));
#99086=CARTESIAN_POINT('Ctrl Pts',(-13.265813552961,69.3258709977382,12.));
#99087=CARTESIAN_POINT('Ctrl Pts',(-13.2561802906896,69.3072528758518,12.));
#99088=CARTESIAN_POINT('Ctrl Pts',(-13.2465895067262,69.2886693063182,12.));
#99089=CARTESIAN_POINT('Ctrl Pts',(-13.237041206122,69.270120474245,12.));
#99090=CARTESIAN_POINT('Ctrl Pts',(-13.2275353939051,69.2516065668844,12.));
#99091=CARTESIAN_POINT('Ctrl Pts',(-13.2180720750594,69.2331277732861,12.));
#99092=CARTESIAN_POINT('Ctrl Pts',(-13.2086512544735,69.2146842833537,12.));
#99093=CARTESIAN_POINT('Ctrl Pts',(-13.1992729368928,69.1962762870527,12.));
#99094=CARTESIAN_POINT('Ctrl Pts',(-13.1899371268683,69.1779039735996,12.));
#99095=CARTESIAN_POINT('Ctrl Pts',(-13.1806438286934,69.1595675305245,12.));
#99096=CARTESIAN_POINT('Ctrl Pts',(-13.1713930465133,69.1412671454564,12.));
#99097=CARTESIAN_POINT('Ctrl Pts',(-13.1621847844528,69.1230030082573,12.));
#99098=CARTESIAN_POINT('Ctrl Pts',(-13.1530190467183,69.1047753127643,12.));
#99099=CARTESIAN_POINT('Ctrl Pts',(-13.1438958377404,69.0865842593102,12.));
#99100=CARTESIAN_POINT('Ctrl Pts',(-13.1348151621834,69.0684300549477,12.));
#99101=CARTESIAN_POINT('Ctrl Pts',(-13.1257770246385,69.0503129081817,12.));
#99102=CARTESIAN_POINT('Ctrl Pts',(-13.1167814293497,69.0322330243348,12.));
#99103=CARTESIAN_POINT('Ctrl Pts',(-13.1078283799722,69.0141906015113,12.));
#99104=CARTESIAN_POINT('Ctrl Pts',(-13.0989178791834,68.9961858241519,12.));
#99105=CARTESIAN_POINT('Ctrl Pts',(-13.090049929053,68.9782188692581,12.));
#99106=CARTESIAN_POINT('Ctrl Pts',(-13.0812245317808,68.9602899187573,12.));
#99107=CARTESIAN_POINT('Ctrl Pts',(-13.072441690283,68.9423991694492,12.));
#99108=CARTESIAN_POINT('Ctrl Pts',(-13.0637014089029,68.9245468449945,12.));
#99109=CARTESIAN_POINT('Ctrl Pts',(-13.0550036938813,68.9067332040985,12.));
#99110=CARTESIAN_POINT('Ctrl Pts',(-13.0463485518207,68.8889585151585,12.));
#99111=CARTESIAN_POINT('Ctrl Pts',(-13.0377359881875,68.8712230321906,12.));
#99112=CARTESIAN_POINT('Ctrl Pts',(-13.0291660060107,68.8535269726794,12.));
#99113=CARTESIAN_POINT('Ctrl Pts',(-13.0206386039691,68.8358704887468,12.));
#99114=CARTESIAN_POINT('Ctrl Pts',(-13.0121537768946,68.8182536653656,12.));
#99115=CARTESIAN_POINT('Ctrl Pts',(-13.0053999700875,68.804191966902,12.));
#99116=CARTESIAN_POINT('Ctrl Pts',(-13.0003537683055,68.7936635625545,12.));
#99117=CARTESIAN_POINT('Ctrl Pts',(-12.9969981460277,68.7866525680193,12.));
#99118=CARTESIAN_POINT('Ctrl Pts',(-12.9953224629497,68.7831490561748,12.));
#99119=CARTESIAN_POINT('Ctrl Pts',(-16.7988252568748,72.2774028393914,0.));
#99120=CARTESIAN_POINT('Ctrl Pts',(-16.7988252568748,72.2774028393914,4.));
#99121=CARTESIAN_POINT('Ctrl Pts',(-16.7988252568748,72.2774028393914,8.));
#99122=CARTESIAN_POINT('Ctrl Pts',(-16.7988252568748,72.2774028393914,12.));
#99123=CARTESIAN_POINT('Ctrl Pts',(-16.7775526720894,72.3852065198825,0.));
#99124=CARTESIAN_POINT('Ctrl Pts',(-16.7775526720894,72.3852065198825,4.));
#99125=CARTESIAN_POINT('Ctrl Pts',(-16.7775526720894,72.3852065198825,8.));
#99126=CARTESIAN_POINT('Ctrl Pts',(-16.7775526720894,72.3852065198825,12.));
#99127=CARTESIAN_POINT('Ctrl Pts',(-16.6758649025559,72.5605133546289,0.));
#99128=CARTESIAN_POINT('Ctrl Pts',(-16.6758649025559,72.5605133546289,4.00000000000001));
#99129=CARTESIAN_POINT('Ctrl Pts',(-16.6758649025559,72.5605133546289,7.99999999999999));
#99130=CARTESIAN_POINT('Ctrl Pts',(-16.6758649025559,72.5605133546289,12.));
#99131=CARTESIAN_POINT('Ctrl Pts',(-16.4988611391808,72.6501505354462,0.));
#99132=CARTESIAN_POINT('Ctrl Pts',(-16.4988611391808,72.6501505354462,3.99999999999999));
#99133=CARTESIAN_POINT('Ctrl Pts',(-16.4988611391808,72.6501505354462,8.00000000000001));
#99134=CARTESIAN_POINT('Ctrl Pts',(-16.4988611391808,72.6501505354462,12.));
#99135=CARTESIAN_POINT('Ctrl Pts',(-16.4184755008061,72.6683126419585,0.));
#99136=CARTESIAN_POINT('Ctrl Pts',(-16.4184755008061,72.6683126419585,4.));
#99137=CARTESIAN_POINT('Ctrl Pts',(-16.4184755008061,72.6683126419585,8.));
#99138=CARTESIAN_POINT('Ctrl Pts',(-16.4184755008061,72.6683126419585,12.));
#99139=CARTESIAN_POINT('',(-16.7988252568748,72.2774028393914,0.));
#99140=CARTESIAN_POINT('',(-16.4184755008061,72.6683126419586,0.));
#99141=CARTESIAN_POINT('Ctrl Pts',(-16.7988252568748,72.2774028393914,2.03133674691991E-34));
#99142=CARTESIAN_POINT('Ctrl Pts',(-16.7775526720894,72.3852065198825,2.03133674691991E-34));
#99143=CARTESIAN_POINT('Ctrl Pts',(-16.7194453752131,72.4853818540233,2.03133674691991E-34));
#99144=CARTESIAN_POINT('Ctrl Pts',(-16.6367451007559,72.5575834236158,2.03133674691991E-34));
#99145=CARTESIAN_POINT('Ctrl Pts',(-16.574719894913,72.6117346008102,2.03133674691991E-34));
#99146=CARTESIAN_POINT('Ctrl Pts',(-16.4988611391808,72.6501505354462,2.03133674691991E-34));
#99147=CARTESIAN_POINT('Ctrl Pts',(-16.4184755008061,72.6683126419585,2.03133674691991E-34));
#99148=CARTESIAN_POINT('',(-16.4184755008061,72.6683126419586,12.));
#99149=CARTESIAN_POINT('Ctrl Pts',(-16.4184755008061,72.6683126419585,0.));
#99150=CARTESIAN_POINT('Ctrl Pts',(-16.4184755008061,72.6683126419585,4.));
#99151=CARTESIAN_POINT('Ctrl Pts',(-16.4184755008061,72.6683126419585,8.));
#99152=CARTESIAN_POINT('Ctrl Pts',(-16.4184755008061,72.6683126419585,12.));
#99153=CARTESIAN_POINT('',(-16.7988252568748,72.2774028393914,12.));
#99154=CARTESIAN_POINT('Ctrl Pts',(-16.4184755008061,72.6683126419585,12.));
#99155=CARTESIAN_POINT('Ctrl Pts',(-16.4988611391808,72.6501505354462,12.));
#99156=CARTESIAN_POINT('Ctrl Pts',(-16.574719894913,72.6117346008102,12.));
#99157=CARTESIAN_POINT('Ctrl Pts',(-16.6367451007559,72.5575834236158,12.));
#99158=CARTESIAN_POINT('Ctrl Pts',(-16.7194453752131,72.4853818540233,12.));
#99159=CARTESIAN_POINT('Ctrl Pts',(-16.7775526720894,72.3852065198825,12.));
#99160=CARTESIAN_POINT('Ctrl Pts',(-16.7988252568748,72.2774028393914,12.));
#99161=CARTESIAN_POINT('Ctrl Pts',(-16.7988252568748,72.2774028393914,12.));
#99162=CARTESIAN_POINT('Ctrl Pts',(-16.7988252568748,72.2774028393914,8.));
#99163=CARTESIAN_POINT('Ctrl Pts',(-16.7988252568748,72.2774028393914,4.));
#99164=CARTESIAN_POINT('Ctrl Pts',(-16.7988252568748,72.2774028393914,0.));
#99165=CARTESIAN_POINT('Origin',(-8.12279454723526E-11,3.65936987487134E-10,
0.));
#99166=CARTESIAN_POINT('Origin',(-8.12279454723526E-11,3.65936987487134E-10,
12.));
#99167=CARTESIAN_POINT('Origin',(-8.12279454723526E-11,3.65936987487134E-10,
0.));
#99168=CARTESIAN_POINT('Ctrl Pts',(-9.42570643237823,73.9013264985861,5.55111512312578E-16));
#99169=CARTESIAN_POINT('Ctrl Pts',(-9.42570643237823,73.9013264985861,4.));
#99170=CARTESIAN_POINT('Ctrl Pts',(-9.42570643237823,73.9013264985861,8.));
#99171=CARTESIAN_POINT('Ctrl Pts',(-9.42570643237823,73.9013264985861,12.));
#99172=CARTESIAN_POINT('Ctrl Pts',(-9.31670696907609,73.9152287787081,5.55111512312578E-16));
#99173=CARTESIAN_POINT('Ctrl Pts',(-9.31670696907609,73.9152287787081,4.));
#99174=CARTESIAN_POINT('Ctrl Pts',(-9.31670696907609,73.9152287787081,8.00000000000001));
#99175=CARTESIAN_POINT('Ctrl Pts',(-9.31670696907609,73.9152287787081,12.));
#99176=CARTESIAN_POINT('Ctrl Pts',(-9.11824194722539,73.8741839722667,4.82031436765098E-16));
#99177=CARTESIAN_POINT('Ctrl Pts',(-9.11824194722539,73.8741839722667,4.00000000000001));
#99178=CARTESIAN_POINT('Ctrl Pts',(-9.11824194722539,73.8741839722667,7.99999999999999));
#99179=CARTESIAN_POINT('Ctrl Pts',(-9.11824194722539,73.8741839722667,12.));
#99180=CARTESIAN_POINT('Ctrl Pts',(-8.9772410874556,73.7345987226918,3.08500332079893E-16));
#99181=CARTESIAN_POINT('Ctrl Pts',(-8.9772410874556,73.7345987226918,4.));
#99182=CARTESIAN_POINT('Ctrl Pts',(-8.9772410874556,73.7345987226918,8.00000000000001));
#99183=CARTESIAN_POINT('Ctrl Pts',(-8.9772410874556,73.7345987226918,12.));
#99184=CARTESIAN_POINT('Ctrl Pts',(-8.93459554655819,73.6640787197672,2.24846351842411E-16));
#99185=CARTESIAN_POINT('Ctrl Pts',(-8.93459554655819,73.6640787197672,4.));
#99186=CARTESIAN_POINT('Ctrl Pts',(-8.93459554655819,73.6640787197672,8.));
#99187=CARTESIAN_POINT('Ctrl Pts',(-8.93459554655819,73.6640787197672,12.));
#99188=CARTESIAN_POINT('',(-9.42570643237823,73.9013264985861,2.77555756156289E-16));
#99189=CARTESIAN_POINT('',(-8.93459554655823,73.6640787197672,0.));
#99190=CARTESIAN_POINT('Ctrl Pts',(-9.42570643237823,73.9013264985861,5.82554064063016E-16));
#99191=CARTESIAN_POINT('Ctrl Pts',(-9.31670696907609,73.9152287787081,5.82554064063016E-16));
#99192=CARTESIAN_POINT('Ctrl Pts',(-9.20329838516141,73.8917746035987,5.40794020893028E-16));
#99193=CARTESIAN_POINT('Ctrl Pts',(-9.10865360927314,73.8361439572621,4.66233641678068E-16));
#99194=CARTESIAN_POINT('Ctrl Pts',(-9.03767002735694,73.7944209725096,4.10313357266848E-16));
#99195=CARTESIAN_POINT('Ctrl Pts',(-8.9772410874556,73.7345987226918,3.35942883830331E-16));
#99196=CARTESIAN_POINT('Ctrl Pts',(-8.93459554655819,73.6640787197672,2.5228890359285E-16));
#99197=CARTESIAN_POINT('',(-8.93459554655823,73.6640787197672,12.));
#99198=CARTESIAN_POINT('Ctrl Pts',(-8.93459554655819,73.6640787197672,2.24846351842411E-16));
#99199=CARTESIAN_POINT('Ctrl Pts',(-8.93459554655819,73.6640787197672,4.));
#99200=CARTESIAN_POINT('Ctrl Pts',(-8.93459554655819,73.6640787197672,8.));
#99201=CARTESIAN_POINT('Ctrl Pts',(-8.93459554655819,73.6640787197672,12.));
#99202=CARTESIAN_POINT('',(-9.42570643237823,73.9013264985861,12.));
#99203=CARTESIAN_POINT('Ctrl Pts',(-8.93459554655819,73.6640787197672,12.));
#99204=CARTESIAN_POINT('Ctrl Pts',(-8.9772410874556,73.7345987226918,12.));
#99205=CARTESIAN_POINT('Ctrl Pts',(-9.03767002735694,73.7944209725096,12.));
#99206=CARTESIAN_POINT('Ctrl Pts',(-9.10865360927314,73.8361439572621,12.));
#99207=CARTESIAN_POINT('Ctrl Pts',(-9.20329838516141,73.8917746035987,12.));
#99208=CARTESIAN_POINT('Ctrl Pts',(-9.31670696907609,73.9152287787081,12.));
#99209=CARTESIAN_POINT('Ctrl Pts',(-9.42570643237823,73.9013264985861,12.));
#99210=CARTESIAN_POINT('Ctrl Pts',(-9.42570643237823,73.9013264985861,12.));
#99211=CARTESIAN_POINT('Ctrl Pts',(-9.42570643237823,73.9013264985861,8.));
#99212=CARTESIAN_POINT('Ctrl Pts',(-9.42570643237823,73.9013264985861,4.));
#99213=CARTESIAN_POINT('Ctrl Pts',(-9.42570643237823,73.9013264985861,5.55111512312578E-16));
#99214=CARTESIAN_POINT('Ctrl Pts',(-6.95102489306926,69.6540253893192,0.));
#99215=CARTESIAN_POINT('Ctrl Pts',(-6.95102489306926,69.6540253893192,12.));
#99216=CARTESIAN_POINT('Ctrl Pts',(-6.95238884849025,69.6576616146467,0.));
#99217=CARTESIAN_POINT('Ctrl Pts',(-6.95238884849025,69.6576616146467,12.));
#99218=CARTESIAN_POINT('Ctrl Pts',(-6.955120653176,69.664938391983,0.));
#99219=CARTESIAN_POINT('Ctrl Pts',(-6.955120653176,69.664938391983,12.));
#99220=CARTESIAN_POINT('Ctrl Pts',(-6.95923004173591,69.6758665380378,0.));
#99221=CARTESIAN_POINT('Ctrl Pts',(-6.95923004173591,69.6758665380378,12.));
#99222=CARTESIAN_POINT('Ctrl Pts',(-6.96473259049513,69.6904633605421,0.));
#99223=CARTESIAN_POINT('Ctrl Pts',(-6.96473259049513,69.6904633605421,12.));
#99224=CARTESIAN_POINT('Ctrl Pts',(-6.9716497229144,69.7087526479973,0.));
#99225=CARTESIAN_POINT('Ctrl Pts',(-6.9716497229144,69.7087526479973,12.));
#99226=CARTESIAN_POINT('Ctrl Pts',(-6.97860581164527,69.7270851557366,0.));
#99227=CARTESIAN_POINT('Ctrl Pts',(-6.97860581164527,69.7270851557366,12.));
#99228=CARTESIAN_POINT('Ctrl Pts',(-6.98560086924214,69.7454607995607,0.));
#99229=CARTESIAN_POINT('Ctrl Pts',(-6.98560086924214,69.7454607995607,12.));
#99230=CARTESIAN_POINT('Ctrl Pts',(-6.9926349102794,69.7638794280419,0.));
#99231=CARTESIAN_POINT('Ctrl Pts',(-6.9926349102794,69.7638794280419,12.));
#99232=CARTESIAN_POINT('Ctrl Pts',(-6.99970795069476,69.782340824259,0.));
#99233=CARTESIAN_POINT('Ctrl Pts',(-6.99970795069476,69.782340824259,12.));
#99234=CARTESIAN_POINT('Ctrl Pts',(-7.00682000718151,69.8008447346863,0.));
#99235=CARTESIAN_POINT('Ctrl Pts',(-7.00682000718151,69.8008447346863,12.));
#99236=CARTESIAN_POINT('Ctrl Pts',(-7.01397109655455,69.8193908913722,0.));
#99237=CARTESIAN_POINT('Ctrl Pts',(-7.01397109655455,69.8193908913722,12.));
#99238=CARTESIAN_POINT('Ctrl Pts',(-7.02116123514452,69.8379790360518,0.));
#99239=CARTESIAN_POINT('Ctrl Pts',(-7.02116123514452,69.8379790360518,12.));
#99240=CARTESIAN_POINT('Ctrl Pts',(-7.02839043811812,69.8566089455375,0.));
#99241=CARTESIAN_POINT('Ctrl Pts',(-7.02839043811812,69.8566089455375,12.));
#99242=CARTESIAN_POINT('Ctrl Pts',(-7.03565871972221,69.8752804235238,0.));
#99243=CARTESIAN_POINT('Ctrl Pts',(-7.03565871972221,69.8752804235238,12.));
#99244=CARTESIAN_POINT('Ctrl Pts',(-7.04296609362166,69.8939932885841,0.));
#99245=CARTESIAN_POINT('Ctrl Pts',(-7.04296609362166,69.8939932885841,12.));
#99246=CARTESIAN_POINT('Ctrl Pts',(-7.05031257318115,69.9127473642099,0.));
#99247=CARTESIAN_POINT('Ctrl Pts',(-7.05031257318115,69.9127473642099,12.));
#99248=CARTESIAN_POINT('Ctrl Pts',(-7.05769817180857,69.9315424664291,0.));
#99249=CARTESIAN_POINT('Ctrl Pts',(-7.05769817180857,69.9315424664291,12.));
#99250=CARTESIAN_POINT('Ctrl Pts',(-7.0651229031285,69.9503783975727,0.));
#99251=CARTESIAN_POINT('Ctrl Pts',(-7.0651229031285,69.9503783975727,12.));
#99252=CARTESIAN_POINT('Ctrl Pts',(-7.07258678080831,69.9692549527296,0.));
#99253=CARTESIAN_POINT('Ctrl Pts',(-7.07258678080831,69.9692549527296,12.));
#99254=CARTESIAN_POINT('Ctrl Pts',(-7.08008981844652,69.988171923788,0.));
#99255=CARTESIAN_POINT('Ctrl Pts',(-7.08008981844652,69.988171923788,12.));
#99256=CARTESIAN_POINT('Ctrl Pts',(-7.08763202944246,70.0071291040766,0.));
#99257=CARTESIAN_POINT('Ctrl Pts',(-7.08763202944246,70.0071291040766,12.));
#99258=CARTESIAN_POINT('Ctrl Pts',(-7.09521342684249,70.0261262936388,0.));
#99259=CARTESIAN_POINT('Ctrl Pts',(-7.09521342684249,70.0261262936388,12.));
#99260=CARTESIAN_POINT('Ctrl Pts',(-7.10283402335034,70.0451632990086,0.));
#99261=CARTESIAN_POINT('Ctrl Pts',(-7.10283402335034,70.0451632990086,12.));
#99262=CARTESIAN_POINT('Ctrl Pts',(-7.11049383140446,70.0642399306869,0.));
#99263=CARTESIAN_POINT('Ctrl Pts',(-7.11049383140446,70.0642399306869,12.));
#99264=CARTESIAN_POINT('Ctrl Pts',(-7.11819286322826,70.0833560013975,0.));
#99265=CARTESIAN_POINT('Ctrl Pts',(-7.11819286322826,70.0833560013975,12.));
#99266=CARTESIAN_POINT('Ctrl Pts',(-7.12593113088904,70.1025113239495,0.));
#99267=CARTESIAN_POINT('Ctrl Pts',(-7.12593113088904,70.1025113239495,12.));
#99268=CARTESIAN_POINT('Ctrl Pts',(-7.13370864634442,70.1217057094499,0.));
#99269=CARTESIAN_POINT('Ctrl Pts',(-7.13370864634442,70.1217057094499,12.));
#99270=CARTESIAN_POINT('Ctrl Pts',(-7.14152542142374,70.1409389682424,0.));
#99271=CARTESIAN_POINT('Ctrl Pts',(-7.14152542142374,70.1409389682424,12.));
#99272=CARTESIAN_POINT('Ctrl Pts',(-7.14938146780813,70.1602109107202,0.));
#99273=CARTESIAN_POINT('Ctrl Pts',(-7.14938146780813,70.1602109107202,12.));
#99274=CARTESIAN_POINT('Ctrl Pts',(-7.15727679700933,70.1795213481185,0.));
#99275=CARTESIAN_POINT('Ctrl Pts',(-7.15727679700933,70.1795213481185,12.));
#99276=CARTESIAN_POINT('Ctrl Pts',(-7.16521142033864,70.1988700934593,0.));
#99277=CARTESIAN_POINT('Ctrl Pts',(-7.16521142033864,70.1988700934593,12.));
#99278=CARTESIAN_POINT('Ctrl Pts',(-7.17318534889716,70.2182569618994,0.));
#99279=CARTESIAN_POINT('Ctrl Pts',(-7.17318534889716,70.2182569618994,12.));
#99280=CARTESIAN_POINT('Ctrl Pts',(-7.18119859359778,70.2376817702215,0.));
#99281=CARTESIAN_POINT('Ctrl Pts',(-7.18119859359778,70.2376817702215,12.));
#99282=CARTESIAN_POINT('Ctrl Pts',(-7.18925116517555,70.2571443365192,0.));
#99283=CARTESIAN_POINT('Ctrl Pts',(-7.18925116517555,70.2571443365192,12.));
#99284=CARTESIAN_POINT('Ctrl Pts',(-7.19734307419873,70.2766444798285,0.));
#99285=CARTESIAN_POINT('Ctrl Pts',(-7.19734307419873,70.2766444798285,12.));
#99286=CARTESIAN_POINT('Ctrl Pts',(-7.20547433107483,70.2961820197077,0.));
#99287=CARTESIAN_POINT('Ctrl Pts',(-7.20547433107483,70.2961820197077,12.));
#99288=CARTESIAN_POINT('Ctrl Pts',(-7.2136449460545,70.3157567762588,0.));
#99289=CARTESIAN_POINT('Ctrl Pts',(-7.2136449460545,70.3157567762588,12.));
#99290=CARTESIAN_POINT('Ctrl Pts',(-7.22185492923191,70.3353685703112,0.));
#99291=CARTESIAN_POINT('Ctrl Pts',(-7.22185492923191,70.3353685703112,12.));
#99292=CARTESIAN_POINT('Ctrl Pts',(-7.23010429054229,70.3550172235486,0.));
#99293=CARTESIAN_POINT('Ctrl Pts',(-7.23010429054229,70.3550172235486,12.));
#99294=CARTESIAN_POINT('Ctrl Pts',(-7.23839303975607,70.3747025586552,0.));
#99295=CARTESIAN_POINT('Ctrl Pts',(-7.23839303975607,70.3747025586552,12.));
#99296=CARTESIAN_POINT('Ctrl Pts',(-7.24672118647085,70.3944243994504,0.));
#99297=CARTESIAN_POINT('Ctrl Pts',(-7.24672118647085,70.3944243994504,12.));
#99298=CARTESIAN_POINT('Ctrl Pts',(-7.25508874012043,70.4141825708178,0.));
#99299=CARTESIAN_POINT('Ctrl Pts',(-7.25508874012043,70.4141825708178,12.));
#99300=CARTESIAN_POINT('Ctrl Pts',(-7.26349570998033,70.4339768986346,0.));
#99301=CARTESIAN_POINT('Ctrl Pts',(-7.26349570998033,70.4339768986346,12.));
#99302=CARTESIAN_POINT('Ctrl Pts',(-7.27194210517063,70.4538072096992,0.));
#99303=CARTESIAN_POINT('Ctrl Pts',(-7.27194210517063,70.4538072096992,12.));
#99304=CARTESIAN_POINT('Ctrl Pts',(-7.28042793465471,70.4736733316487,0.));
#99305=CARTESIAN_POINT('Ctrl Pts',(-7.28042793465471,70.4736733316487,12.));
#99306=CARTESIAN_POINT('Ctrl Pts',(-7.28895320723862,70.4935750929058,0.));
#99307=CARTESIAN_POINT('Ctrl Pts',(-7.28895320723862,70.4935750929058,12.));
#99308=CARTESIAN_POINT('Ctrl Pts',(-7.29751793157823,70.5135123227169,0.));
#99309=CARTESIAN_POINT('Ctrl Pts',(-7.29751793157823,70.5135123227169,12.));
#99310=CARTESIAN_POINT('Ctrl Pts',(-7.30612211618053,70.5334848511681,0.));
#99311=CARTESIAN_POINT('Ctrl Pts',(-7.30612211618053,70.5334848511681,12.));
#99312=CARTESIAN_POINT('Ctrl Pts',(-7.31476576940392,70.5534925092043,0.));
#99313=CARTESIAN_POINT('Ctrl Pts',(-7.31476576940392,70.5534925092043,12.));
#99314=CARTESIAN_POINT('Ctrl Pts',(-7.3234488994522,70.5735351286476,0.));
#99315=CARTESIAN_POINT('Ctrl Pts',(-7.3234488994522,70.5735351286476,12.));
#99316=CARTESIAN_POINT('Ctrl Pts',(-7.3321715143759,70.5936125421946,0.));
#99317=CARTESIAN_POINT('Ctrl Pts',(-7.3321715143759,70.5936125421946,12.));
#99318=CARTESIAN_POINT('Ctrl Pts',(-7.34093362208008,70.6137245833996,0.));
#99319=CARTESIAN_POINT('Ctrl Pts',(-7.34093362208008,70.6137245833996,12.));
#99320=CARTESIAN_POINT('Ctrl Pts',(-7.34973523032577,70.6338710866562,0.));
#99321=CARTESIAN_POINT('Ctrl Pts',(-7.34973523032577,70.6338710866562,12.));
#99322=CARTESIAN_POINT('Ctrl Pts',(-7.35857634673055,70.6540518871775,0.));
#99323=CARTESIAN_POINT('Ctrl Pts',(-7.35857634673055,70.6540518871775,12.));
#99324=CARTESIAN_POINT('Ctrl Pts',(-7.36745697876301,70.6742668209687,0.));
#99325=CARTESIAN_POINT('Ctrl Pts',(-7.36745697876301,70.6742668209687,12.));
#99326=CARTESIAN_POINT('Ctrl Pts',(-7.37637713374768,70.694515724827,0.));
#99327=CARTESIAN_POINT('Ctrl Pts',(-7.37637713374768,70.694515724827,12.));
#99328=CARTESIAN_POINT('Ctrl Pts',(-7.38533681887033,70.7147984363424,0.));
#99329=CARTESIAN_POINT('Ctrl Pts',(-7.38533681887033,70.7147984363424,12.));
#99330=CARTESIAN_POINT('Ctrl Pts',(-7.39433604117891,70.735114793895,0.));
#99331=CARTESIAN_POINT('Ctrl Pts',(-7.39433604117891,70.735114793895,12.));
#99332=CARTESIAN_POINT('Ctrl Pts',(-7.4033748075823,70.7554646366514,0.));
#99333=CARTESIAN_POINT('Ctrl Pts',(-7.4033748075823,70.7554646366514,12.));
#99334=CARTESIAN_POINT('Ctrl Pts',(-7.41245312484487,70.7758478045576,0.));
#99335=CARTESIAN_POINT('Ctrl Pts',(-7.41245312484487,70.7758478045576,12.));
#99336=CARTESIAN_POINT('Ctrl Pts',(-7.42157099959316,70.7962641383351,0.));
#99337=CARTESIAN_POINT('Ctrl Pts',(-7.42157099959316,70.7962641383351,12.));
#99338=CARTESIAN_POINT('Ctrl Pts',(-7.43072843832008,70.8167134794738,0.));
#99339=CARTESIAN_POINT('Ctrl Pts',(-7.43072843832008,70.8167134794738,12.));
#99340=CARTESIAN_POINT('Ctrl Pts',(-7.43992544738607,70.8371956702242,0.));
#99341=CARTESIAN_POINT('Ctrl Pts',(-7.43992544738607,70.8371956702242,12.));
#99342=CARTESIAN_POINT('Ctrl Pts',(-7.44916203301645,70.8577105535841,0.));
#99343=CARTESIAN_POINT('Ctrl Pts',(-7.44916203301645,70.8577105535841,12.));
#99344=CARTESIAN_POINT('Ctrl Pts',(-7.45843820129776,70.8782579732885,0.));
#99345=CARTESIAN_POINT('Ctrl Pts',(-7.45843820129776,70.8782579732885,12.));
#99346=CARTESIAN_POINT('Ctrl Pts',(-7.46775395818519,70.8988377738088,0.));
#99347=CARTESIAN_POINT('Ctrl Pts',(-7.46775395818519,70.8988377738088,12.));
#99348=CARTESIAN_POINT('Ctrl Pts',(-7.47710930950554,70.9194498003483,0.));
#99349=CARTESIAN_POINT('Ctrl Pts',(-7.47710930950554,70.9194498003483,12.));
#99350=CARTESIAN_POINT('Ctrl Pts',(-7.48650426095823,70.9400938988373,0.));
#99351=CARTESIAN_POINT('Ctrl Pts',(-7.48650426095823,70.9400938988373,12.));
#99352=CARTESIAN_POINT('Ctrl Pts',(-7.49593881811141,70.9607699159234,0.));
#99353=CARTESIAN_POINT('Ctrl Pts',(-7.49593881811141,70.9607699159234,12.));
#99354=CARTESIAN_POINT('Ctrl Pts',(-7.50541298639948,70.9814776989637,0.));
#99355=CARTESIAN_POINT('Ctrl Pts',(-7.50541298639948,70.9814776989637,12.));
#99356=CARTESIAN_POINT('Ctrl Pts',(-7.51492677113112,71.0022170960235,0.));
#99357=CARTESIAN_POINT('Ctrl Pts',(-7.51492677113112,71.0022170960235,12.));
#99358=CARTESIAN_POINT('Ctrl Pts',(-7.52448017749136,71.0229879558713,0.));
#99359=CARTESIAN_POINT('Ctrl Pts',(-7.52448017749136,71.0229879558713,12.));
#99360=CARTESIAN_POINT('Ctrl Pts',(-7.53407321054254,71.0437901279722,0.));
#99361=CARTESIAN_POINT('Ctrl Pts',(-7.53407321054254,71.0437901279722,12.));
#99362=CARTESIAN_POINT('Ctrl Pts',(-7.54370587521948,71.0646234624783,0.));
#99363=CARTESIAN_POINT('Ctrl Pts',(-7.54370587521948,71.0646234624783,12.));
#99364=CARTESIAN_POINT('Ctrl Pts',(-7.55337817632873,71.0854878102203,0.));
#99365=CARTESIAN_POINT('Ctrl Pts',(-7.55337817632873,71.0854878102203,12.));
#99366=CARTESIAN_POINT('Ctrl Pts',(-7.56309011855617,71.1063830227074,0.));
#99367=CARTESIAN_POINT('Ctrl Pts',(-7.56309011855617,71.1063830227074,12.));
#99368=CARTESIAN_POINT('Ctrl Pts',(-7.57284170646866,71.1273089521218,0.));
#99369=CARTESIAN_POINT('Ctrl Pts',(-7.57284170646866,71.1273089521218,12.));
#99370=CARTESIAN_POINT('Ctrl Pts',(-7.58263294451465,71.1482654513133,0.));
#99371=CARTESIAN_POINT('Ctrl Pts',(-7.58263294451465,71.1482654513133,12.));
#99372=CARTESIAN_POINT('Ctrl Pts',(-7.5924638370186,71.1692523737887,0.));
#99373=CARTESIAN_POINT('Ctrl Pts',(-7.5924638370186,71.1692523737887,12.));
#99374=CARTESIAN_POINT('Ctrl Pts',(-7.60233438818156,71.1902695737063,0.));
#99375=CARTESIAN_POINT('Ctrl Pts',(-7.60233438818156,71.1902695737063,12.));
#99376=CARTESIAN_POINT('Ctrl Pts',(-7.61224460208887,71.2113169058778,0.));
#99377=CARTESIAN_POINT('Ctrl Pts',(-7.61224460208887,71.2113169058778,12.));
#99378=CARTESIAN_POINT('Ctrl Pts',(-7.62219448271125,71.232394225762,0.));
#99379=CARTESIAN_POINT('Ctrl Pts',(-7.62219448271125,71.232394225762,12.));
#99380=CARTESIAN_POINT('Ctrl Pts',(-7.63218403390515,71.2535013894587,0.));
#99381=CARTESIAN_POINT('Ctrl Pts',(-7.63218403390515,71.2535013894587,12.));
#99382=CARTESIAN_POINT('Ctrl Pts',(-7.64221325940672,71.2746382536974,0.));
#99383=CARTESIAN_POINT('Ctrl Pts',(-7.64221325940672,71.2746382536974,12.));
#99384=CARTESIAN_POINT('Ctrl Pts',(-7.65228216283343,71.2958046758334,0.));
#99385=CARTESIAN_POINT('Ctrl Pts',(-7.65228216283343,71.2958046758334,12.));
#99386=CARTESIAN_POINT('Ctrl Pts',(-7.66239074769119,71.3170005138474,0.));
#99387=CARTESIAN_POINT('Ctrl Pts',(-7.66239074769119,71.3170005138474,12.));
#99388=CARTESIAN_POINT('Ctrl Pts',(-7.67253901737539,71.3382256263405,0.));
#99389=CARTESIAN_POINT('Ctrl Pts',(-7.67253901737539,71.3382256263405,12.));
#99390=CARTESIAN_POINT('Ctrl Pts',(-7.68272697517103,71.3594798725294,0.));
#99391=CARTESIAN_POINT('Ctrl Pts',(-7.68272697517103,71.3594798725294,12.));
#99392=CARTESIAN_POINT('Ctrl Pts',(-7.69295462424647,71.380763112236,0.));
#99393=CARTESIAN_POINT('Ctrl Pts',(-7.69295462424647,71.380763112236,12.));
#99394=CARTESIAN_POINT('Ctrl Pts',(-7.70322196765573,71.4020752058827,0.));
#99395=CARTESIAN_POINT('Ctrl Pts',(-7.70322196765573,71.4020752058827,12.));
#99396=CARTESIAN_POINT('Ctrl Pts',(-7.71352900834538,71.4234160144943,0.));
#99397=CARTESIAN_POINT('Ctrl Pts',(-7.71352900834538,71.4234160144943,12.));
#99398=CARTESIAN_POINT('Ctrl Pts',(-7.72387574915544,71.4447853996919,0.));
#99399=CARTESIAN_POINT('Ctrl Pts',(-7.72387574915544,71.4447853996919,12.));
#99400=CARTESIAN_POINT('Ctrl Pts',(-7.73426219281932,71.4661832236881,0.));
#99401=CARTESIAN_POINT('Ctrl Pts',(-7.73426219281932,71.4661832236881,12.));
#99402=CARTESIAN_POINT('Ctrl Pts',(-7.74468834195734,71.487609349277,0.));
#99403=CARTESIAN_POINT('Ctrl Pts',(-7.74468834195734,71.487609349277,12.));
#99404=CARTESIAN_POINT('Ctrl Pts',(-7.75515419907955,71.5090636398307,0.));
#99405=CARTESIAN_POINT('Ctrl Pts',(-7.75515419907955,71.5090636398307,12.));
#99406=CARTESIAN_POINT('Ctrl Pts',(-7.76565976659218,71.5305459592987,0.));
#99407=CARTESIAN_POINT('Ctrl Pts',(-7.76565976659218,71.5305459592987,12.));
#99408=CARTESIAN_POINT('Ctrl Pts',(-7.77620504679868,71.5520561722039,0.));
#99409=CARTESIAN_POINT('Ctrl Pts',(-7.77620504679868,71.5520561722039,12.));
#99410=CARTESIAN_POINT('Ctrl Pts',(-7.78679004189935,71.5735941436366,0.));
#99411=CARTESIAN_POINT('Ctrl Pts',(-7.78679004189935,71.5735941436366,12.));
#99412=CARTESIAN_POINT('Ctrl Pts',(-7.79741475398512,71.5951597392471,0.));
#99413=CARTESIAN_POINT('Ctrl Pts',(-7.79741475398512,71.5951597392471,12.));
#99414=CARTESIAN_POINT('Ctrl Pts',(-7.80807918504017,71.616752825242,0.));
#99415=CARTESIAN_POINT('Ctrl Pts',(-7.80807918504017,71.616752825242,12.));
#99416=CARTESIAN_POINT('Ctrl Pts',(-7.81878333694856,71.638373268384,0.));
#99417=CARTESIAN_POINT('Ctrl Pts',(-7.81878333694856,71.638373268384,12.));
#99418=CARTESIAN_POINT('Ctrl Pts',(-7.82952721149504,71.6600209359869,0.));
#99419=CARTESIAN_POINT('Ctrl Pts',(-7.82952721149504,71.6600209359869,12.));
#99420=CARTESIAN_POINT('Ctrl Pts',(-7.84031081036489,71.681695695912,0.));
#99421=CARTESIAN_POINT('Ctrl Pts',(-7.84031081036489,71.681695695912,12.));
#99422=CARTESIAN_POINT('Ctrl Pts',(-7.85113413513739,71.7033974165576,0.));
#99423=CARTESIAN_POINT('Ctrl Pts',(-7.85113413513739,71.7033974165576,12.));
#99424=CARTESIAN_POINT('Ctrl Pts',(-7.8619971872883,71.7251259668573,0.));
#99425=CARTESIAN_POINT('Ctrl Pts',(-7.8619971872883,71.7251259668573,12.));
#99426=CARTESIAN_POINT('Ctrl Pts',(-7.87289996819654,71.7468812162795,0.));
#99427=CARTESIAN_POINT('Ctrl Pts',(-7.87289996819654,71.7468812162795,12.));
#99428=CARTESIAN_POINT('Ctrl Pts',(-7.88384247914522,71.768663034824,0.));
#99429=CARTESIAN_POINT('Ctrl Pts',(-7.88384247914522,71.768663034824,12.));
#99430=CARTESIAN_POINT('Ctrl Pts',(-7.89482472132135,71.7904712930172,0.));
#99431=CARTESIAN_POINT('Ctrl Pts',(-7.89482472132135,71.7904712930172,12.));
#99432=CARTESIAN_POINT('Ctrl Pts',(-7.90584669580955,71.8123058619038,0.));
#99433=CARTESIAN_POINT('Ctrl Pts',(-7.90584669580955,71.8123058619038,12.));
#99434=CARTESIAN_POINT('Ctrl Pts',(-7.91690840359371,71.8341666130424,0.));
#99435=CARTESIAN_POINT('Ctrl Pts',(-7.91690840359371,71.8341666130424,12.));
#99436=CARTESIAN_POINT('Ctrl Pts',(-7.928009845564,71.8560534185071,0.));
#99437=CARTESIAN_POINT('Ctrl Pts',(-7.928009845564,71.8560534185071,12.));
#99438=CARTESIAN_POINT('Ctrl Pts',(-7.93915102251796,71.8779661508833,0.));
#99439=CARTESIAN_POINT('Ctrl Pts',(-7.93915102251796,71.8779661508833,12.));
#99440=CARTESIAN_POINT('Ctrl Pts',(-7.95033193516046,71.8999046832642,0.));
#99441=CARTESIAN_POINT('Ctrl Pts',(-7.95033193516046,71.8999046832642,12.));
#99442=CARTESIAN_POINT('Ctrl Pts',(-7.96155258409752,71.9218688892426,0.));
#99443=CARTESIAN_POINT('Ctrl Pts',(-7.96155258409752,71.9218688892426,12.));
#99444=CARTESIAN_POINT('Ctrl Pts',(-7.97281296983702,71.9438586429072,0.));
#99445=CARTESIAN_POINT('Ctrl Pts',(-7.97281296983702,71.9438586429072,12.));
#99446=CARTESIAN_POINT('Ctrl Pts',(-7.98411309279598,71.9658738188421,0.));
#99447=CARTESIAN_POINT('Ctrl Pts',(-7.98411309279598,71.9658738188421,12.));
#99448=CARTESIAN_POINT('Ctrl Pts',(-7.99545295330182,71.9879142921248,0.));
#99449=CARTESIAN_POINT('Ctrl Pts',(-7.99545295330182,71.9879142921248,12.));
#99450=CARTESIAN_POINT('Ctrl Pts',(-8.0068325515925,72.0099799383216,0.));
#99451=CARTESIAN_POINT('Ctrl Pts',(-8.0068325515925,72.0099799383216,12.));
#99452=CARTESIAN_POINT('Ctrl Pts',(-8.0182518878107,72.0320706334802,0.));
#99453=CARTESIAN_POINT('Ctrl Pts',(-8.0182518878107,72.0320706334802,12.));
#99454=CARTESIAN_POINT('Ctrl Pts',(-8.02971096200329,72.0541862541262,0.));
#99455=CARTESIAN_POINT('Ctrl Pts',(-8.02971096200329,72.0541862541262,12.));
#99456=CARTESIAN_POINT('Ctrl Pts',(-8.04120977412891,72.0763266772632,0.));
#99457=CARTESIAN_POINT('Ctrl Pts',(-8.04120977412891,72.0763266772632,12.));
#99458=CARTESIAN_POINT('Ctrl Pts',(-8.05274832405957,72.0984917803702,0.));
#99459=CARTESIAN_POINT('Ctrl Pts',(-8.05274832405957,72.0984917803702,12.));
#99460=CARTESIAN_POINT('Ctrl Pts',(-8.06432661158089,72.1206814413985,0.));
#99461=CARTESIAN_POINT('Ctrl Pts',(-8.06432661158089,72.1206814413985,12.));
#99462=CARTESIAN_POINT('Ctrl Pts',(-8.07594463638699,72.1428955387648,0.));
#99463=CARTESIAN_POINT('Ctrl Pts',(-8.07594463638699,72.1428955387648,12.));
#99464=CARTESIAN_POINT('Ctrl Pts',(-8.08760239807815,72.165133951346,0.));
#99465=CARTESIAN_POINT('Ctrl Pts',(-8.08760239807815,72.165133951346,12.));
#99466=CARTESIAN_POINT('Ctrl Pts',(-8.09929989616874,72.18739655848,0.));
#99467=CARTESIAN_POINT('Ctrl Pts',(-8.09929989616874,72.18739655848,12.));
#99468=CARTESIAN_POINT('Ctrl Pts',(-8.11103713008922,72.2096832399626,0.));
#99469=CARTESIAN_POINT('Ctrl Pts',(-8.11103713008922,72.2096832399626,12.));
#99470=CARTESIAN_POINT('Ctrl Pts',(-8.12281409918662,72.2319938760451,0.));
#99471=CARTESIAN_POINT('Ctrl Pts',(-8.12281409918662,72.2319938760451,12.));
#99472=CARTESIAN_POINT('Ctrl Pts',(-8.13463080272029,72.2543283474279,0.));
#99473=CARTESIAN_POINT('Ctrl Pts',(-8.13463080272029,72.2543283474279,12.));
#99474=CARTESIAN_POINT('Ctrl Pts',(-8.14648723985793,72.2766865352552,0.));
#99475=CARTESIAN_POINT('Ctrl Pts',(-8.14648723985793,72.2766865352552,12.));
#99476=CARTESIAN_POINT('Ctrl Pts',(-8.15838340968328,72.2990683211155,0.));
#99477=CARTESIAN_POINT('Ctrl Pts',(-8.15838340968328,72.2990683211155,12.));
#99478=CARTESIAN_POINT('Ctrl Pts',(-8.17031931119882,72.3214735870402,0.));
#99479=CARTESIAN_POINT('Ctrl Pts',(-8.17031931119882,72.3214735870402,12.));
#99480=CARTESIAN_POINT('Ctrl Pts',(-8.18229494332622,72.3439022155007,0.));
#99481=CARTESIAN_POINT('Ctrl Pts',(-8.18229494332622,72.3439022155007,12.));
#99482=CARTESIAN_POINT('Ctrl Pts',(-8.19431030490319,72.3663540894034,0.));
#99483=CARTESIAN_POINT('Ctrl Pts',(-8.19431030490319,72.3663540894034,12.));
#99484=CARTESIAN_POINT('Ctrl Pts',(-8.20636539467782,72.3888290920845,0.));
#99485=CARTESIAN_POINT('Ctrl Pts',(-8.20636539467782,72.3888290920845,12.));
#99486=CARTESIAN_POINT('Ctrl Pts',(-8.21846021131564,72.4113271073091,0.));
#99487=CARTESIAN_POINT('Ctrl Pts',(-8.21846021131564,72.4113271073091,12.));
#99488=CARTESIAN_POINT('Ctrl Pts',(-8.23059475340354,72.4338480192701,0.));
#99489=CARTESIAN_POINT('Ctrl Pts',(-8.23059475340354,72.4338480192701,12.));
#99490=CARTESIAN_POINT('Ctrl Pts',(-8.24276901945037,72.4563917125842,0.));
#99491=CARTESIAN_POINT('Ctrl Pts',(-8.24276901945037,72.4563917125842,12.));
#99492=CARTESIAN_POINT('Ctrl Pts',(-8.25498300788493,72.4789580722871,0.));
#99493=CARTESIAN_POINT('Ctrl Pts',(-8.25498300788493,72.4789580722871,12.));
#99494=CARTESIAN_POINT('Ctrl Pts',(-8.26723671704924,72.501546983825,0.));
#99495=CARTESIAN_POINT('Ctrl Pts',(-8.26723671704924,72.501546983825,12.));
#99496=CARTESIAN_POINT('Ctrl Pts',(-8.27953014520385,72.524158333056,0.));
#99497=CARTESIAN_POINT('Ctrl Pts',(-8.27953014520385,72.524158333056,12.));
#99498=CARTESIAN_POINT('Ctrl Pts',(-8.29186329053289,72.5467920062522,0.));
#99499=CARTESIAN_POINT('Ctrl Pts',(-8.29186329053289,72.5467920062522,12.));
#99500=CARTESIAN_POINT('Ctrl Pts',(-8.30423615114455,72.5694478900983,0.));
#99501=CARTESIAN_POINT('Ctrl Pts',(-8.30423615114455,72.5694478900983,12.));
#99502=CARTESIAN_POINT('Ctrl Pts',(-8.31664872507008,72.5921258716899,0.));
#99503=CARTESIAN_POINT('Ctrl Pts',(-8.31664872507008,72.5921258716899,12.));
#99504=CARTESIAN_POINT('Ctrl Pts',(-8.32910101025653,72.614825838529,0.));
#99505=CARTESIAN_POINT('Ctrl Pts',(-8.32910101025653,72.614825838529,12.));
#99506=CARTESIAN_POINT('Ctrl Pts',(-8.34159300456965,72.6375476785208,0.));
#99507=CARTESIAN_POINT('Ctrl Pts',(-8.34159300456965,72.6375476785208,12.));
#99508=CARTESIAN_POINT('Ctrl Pts',(-8.35412470580083,72.6602912799689,0.));
#99509=CARTESIAN_POINT('Ctrl Pts',(-8.35412470580083,72.6602912799689,12.));
#99510=CARTESIAN_POINT('Ctrl Pts',(-8.36669611166834,72.68305653157,0.));
#99511=CARTESIAN_POINT('Ctrl Pts',(-8.36669611166834,72.68305653157,12.));
#99512=CARTESIAN_POINT('Ctrl Pts',(-8.37930721981735,72.7058433224072,0.));
#99513=CARTESIAN_POINT('Ctrl Pts',(-8.37930721981735,72.7058433224072,12.));
#99514=CARTESIAN_POINT('Ctrl Pts',(-8.39195802781407,72.728651541938,0.));
#99515=CARTESIAN_POINT('Ctrl Pts',(-8.39195802781407,72.728651541938,12.));
#99516=CARTESIAN_POINT('Ctrl Pts',(-8.40464853314493,72.7514810799932,0.));
#99517=CARTESIAN_POINT('Ctrl Pts',(-8.40464853314493,72.7514810799932,12.));
#99518=CARTESIAN_POINT('Ctrl Pts',(-8.41737873322353,72.7743318267876,0.));
#99519=CARTESIAN_POINT('Ctrl Pts',(-8.41737873322353,72.7743318267876,12.));
#99520=CARTESIAN_POINT('Ctrl Pts',(-8.43014862539171,72.7972036729283,0.));
#99521=CARTESIAN_POINT('Ctrl Pts',(-8.43014862539171,72.7972036729283,12.));
#99522=CARTESIAN_POINT('Ctrl Pts',(-8.44295820691907,72.8200965094197,0.));
#99523=CARTESIAN_POINT('Ctrl Pts',(-8.44295820691907,72.8200965094197,12.));
#99524=CARTESIAN_POINT('Ctrl Pts',(-8.45580747499771,72.8430102276703,0.));
#99525=CARTESIAN_POINT('Ctrl Pts',(-8.45580747499771,72.8430102276703,12.));
#99526=CARTESIAN_POINT('Ctrl Pts',(-8.46869642673763,72.8659447194918,0.));
#99527=CARTESIAN_POINT('Ctrl Pts',(-8.46869642673763,72.8659447194918,12.));
#99528=CARTESIAN_POINT('Ctrl Pts',(-8.48162505917628,72.888899877077,0.));
#99529=CARTESIAN_POINT('Ctrl Pts',(-8.48162505917628,72.888899877077,12.));
#99530=CARTESIAN_POINT('Ctrl Pts',(-8.49459336928276,72.9118755929785,0.));
#99531=CARTESIAN_POINT('Ctrl Pts',(-8.49459336928276,72.9118755929785,12.));
#99532=CARTESIAN_POINT('Ctrl Pts',(-8.50760135395979,72.9348717600837,0.));
#99533=CARTESIAN_POINT('Ctrl Pts',(-8.50760135395979,72.9348717600837,12.));
#99534=CARTESIAN_POINT('Ctrl Pts',(-8.52064901004244,72.9578882715923,0.));
#99535=CARTESIAN_POINT('Ctrl Pts',(-8.52064901004244,72.9578882715923,12.));
#99536=CARTESIAN_POINT('Ctrl Pts',(-8.53373633429303,72.9809250209843,0.));
#99537=CARTESIAN_POINT('Ctrl Pts',(-8.53373633429303,72.9809250209843,12.));
#99538=CARTESIAN_POINT('Ctrl Pts',(-8.54686332340439,73.0039819020663,0.));
#99539=CARTESIAN_POINT('Ctrl Pts',(-8.54686332340439,73.0039819020663,12.));
#99540=CARTESIAN_POINT('Ctrl Pts',(-8.56002997400096,73.0270588090193,0.));
#99541=CARTESIAN_POINT('Ctrl Pts',(-8.56002997400096,73.0270588090193,12.));
#99542=CARTESIAN_POINT('Ctrl Pts',(-8.57323628263595,73.0501556364482,0.));
#99543=CARTESIAN_POINT('Ctrl Pts',(-8.57323628263595,73.0501556364482,12.));
#99544=CARTESIAN_POINT('Ctrl Pts',(-8.58648224578723,73.073272279419,0.));
#99545=CARTESIAN_POINT('Ctrl Pts',(-8.58648224578723,73.073272279419,12.));
#99546=CARTESIAN_POINT('Ctrl Pts',(-8.59976785984539,73.0964086335226,0.));
#99547=CARTESIAN_POINT('Ctrl Pts',(-8.59976785984539,73.0964086335226,12.));
#99548=CARTESIAN_POINT('Ctrl Pts',(-8.61309312111989,73.1195645948169,0.));
#99549=CARTESIAN_POINT('Ctrl Pts',(-8.61309312111989,73.1195645948169,12.));
#99550=CARTESIAN_POINT('Ctrl Pts',(-8.62645802585475,73.142740059703,0.));
#99551=CARTESIAN_POINT('Ctrl Pts',(-8.62645802585475,73.142740059703,12.));
#99552=CARTESIAN_POINT('Ctrl Pts',(-8.63986257023735,73.165934924813,0.));
#99553=CARTESIAN_POINT('Ctrl Pts',(-8.63986257023735,73.165934924813,12.));
#99554=CARTESIAN_POINT('Ctrl Pts',(-8.65330675040535,73.1891490869057,0.));
#99555=CARTESIAN_POINT('Ctrl Pts',(-8.65330675040535,73.1891490869057,12.));
#99556=CARTESIAN_POINT('Ctrl Pts',(-8.66679056245095,73.2123824427212,0.));
#99557=CARTESIAN_POINT('Ctrl Pts',(-8.66679056245095,73.2123824427212,12.));
#99558=CARTESIAN_POINT('Ctrl Pts',(-8.68031400241884,73.2356348889704,0.));
#99559=CARTESIAN_POINT('Ctrl Pts',(-8.68031400241884,73.2356348889704,12.));
#99560=CARTESIAN_POINT('Ctrl Pts',(-8.69387706629304,73.2589063226373,0.));
#99561=CARTESIAN_POINT('Ctrl Pts',(-8.69387706629304,73.2589063226373,12.));
#99562=CARTESIAN_POINT('Ctrl Pts',(-8.70747974998245,73.282196641216,0.));
#99563=CARTESIAN_POINT('Ctrl Pts',(-8.70747974998245,73.282196641216,12.));
#99564=CARTESIAN_POINT('Ctrl Pts',(-8.72112204930232,73.3055057429744,0.));
#99565=CARTESIAN_POINT('Ctrl Pts',(-8.72112204930232,73.3055057429744,12.));
#99566=CARTESIAN_POINT('Ctrl Pts',(-8.7348039599536,73.3288335271989,0.));
#99567=CARTESIAN_POINT('Ctrl Pts',(-8.7348039599536,73.3288335271989,12.));
#99568=CARTESIAN_POINT('Ctrl Pts',(-8.74852547749736,73.3521798944595,0.));
#99569=CARTESIAN_POINT('Ctrl Pts',(-8.74852547749736,73.3521798944595,12.));
#99570=CARTESIAN_POINT('Ctrl Pts',(-8.76228659740305,73.3755447460235,0.));
#99571=CARTESIAN_POINT('Ctrl Pts',(-8.76228659740305,73.3755447460235,12.));
#99572=CARTESIAN_POINT('Ctrl Pts',(-8.77608731509304,73.3989279832808,0.));
#99573=CARTESIAN_POINT('Ctrl Pts',(-8.77608731509304,73.3989279832808,12.));
#99574=CARTESIAN_POINT('Ctrl Pts',(-8.78992762598738,73.422329507112,0.));
#99575=CARTESIAN_POINT('Ctrl Pts',(-8.78992762598738,73.422329507112,12.));
#99576=CARTESIAN_POINT('Ctrl Pts',(-8.80380752553714,73.4457492173949,0.));
#99577=CARTESIAN_POINT('Ctrl Pts',(-8.80380752553714,73.4457492173949,12.));
#99578=CARTESIAN_POINT('Ctrl Pts',(-8.81772700927593,73.4691870121608,0.));
#99579=CARTESIAN_POINT('Ctrl Pts',(-8.81772700927593,73.4691870121608,12.));
#99580=CARTESIAN_POINT('Ctrl Pts',(-8.83168607277415,73.4926427882787,0.));
#99581=CARTESIAN_POINT('Ctrl Pts',(-8.83168607277415,73.4926427882787,12.));
#99582=CARTESIAN_POINT('Ctrl Pts',(-8.84568471153894,73.5161164429765,0.));
#99583=CARTESIAN_POINT('Ctrl Pts',(-8.84568471153894,73.5161164429765,12.));
#99584=CARTESIAN_POINT('Ctrl Pts',(-8.85972292092183,73.5396078751672,0.));
#99585=CARTESIAN_POINT('Ctrl Pts',(-8.85972292092183,73.5396078751672,12.));
#99586=CARTESIAN_POINT('Ctrl Pts',(-8.87380069602955,73.5631169867113,0.));
#99587=CARTESIAN_POINT('Ctrl Pts',(-8.87380069602955,73.5631169867113,12.));
#99588=CARTESIAN_POINT('Ctrl Pts',(-8.88791803160341,73.5866436840493,0.));
#99589=CARTESIAN_POINT('Ctrl Pts',(-8.88791803160341,73.5866436840493,12.));
#99590=CARTESIAN_POINT('Ctrl Pts',(-8.90207492198871,73.6101878785868,0.));
#99591=CARTESIAN_POINT('Ctrl Pts',(-8.90207492198871,73.6101878785868,12.));
#99592=CARTESIAN_POINT('Ctrl Pts',(-8.91627136139887,73.6337494830846,0.));
#99593=CARTESIAN_POINT('Ctrl Pts',(-8.91627136139887,73.6337494830846,12.));
#99594=CARTESIAN_POINT('Ctrl Pts',(-8.93050734411971,73.6573284088088,0.));
#99595=CARTESIAN_POINT('Ctrl Pts',(-8.93050734411971,73.6573284088088,12.));
#99596=CARTESIAN_POINT('Ctrl Pts',(-8.94478286474383,73.6809245622361,0.));
#99597=CARTESIAN_POINT('Ctrl Pts',(-8.94478286474383,73.6809245622361,12.));
#99598=CARTESIAN_POINT('Ctrl Pts',(-8.9590979183629,73.7045378422775,0.));
#99599=CARTESIAN_POINT('Ctrl Pts',(-8.9590979183629,73.7045378422775,12.));
#99600=CARTESIAN_POINT('Ctrl Pts',(-8.97345250083918,73.7281681364031,0.));
#99601=CARTESIAN_POINT('Ctrl Pts',(-8.97345250083918,73.7281681364031,12.));
#99602=CARTESIAN_POINT('Ctrl Pts',(-8.98784660837828,73.7518153262253,0.));
#99603=CARTESIAN_POINT('Ctrl Pts',(-8.98784660837828,73.7518153262253,12.));
#99604=CARTESIAN_POINT('Ctrl Pts',(-9.00228023701466,73.7754792943925,0.));
#99605=CARTESIAN_POINT('Ctrl Pts',(-9.00228023701466,73.7754792943925,12.));
#99606=CARTESIAN_POINT('Ctrl Pts',(-9.01675338208222,73.7991599312731,0.));
#99607=CARTESIAN_POINT('Ctrl Pts',(-9.01675338208222,73.7991599312731,12.));
#99608=CARTESIAN_POINT('Ctrl Pts',(-9.03126603777981,73.8228571411607,0.));
#99609=CARTESIAN_POINT('Ctrl Pts',(-9.03126603777981,73.8228571411607,12.));
#99610=CARTESIAN_POINT('Ctrl Pts',(-9.04581819646385,73.8465708500679,0.));
#99611=CARTESIAN_POINT('Ctrl Pts',(-9.04581819646385,73.8465708500679,12.));
#99612=CARTESIAN_POINT('Ctrl Pts',(-9.0604098488925,73.870301007746,0.));
#99613=CARTESIAN_POINT('Ctrl Pts',(-9.0604098488925,73.870301007746,12.));
#99614=CARTESIAN_POINT('Ctrl Pts',(-9.07504098570547,73.8940475821756,0.));
#99615=CARTESIAN_POINT('Ctrl Pts',(-9.07504098570547,73.8940475821756,12.));
#99616=CARTESIAN_POINT('Ctrl Pts',(-9.08677747601238,73.9130579611989,0.));
#99617=CARTESIAN_POINT('Ctrl Pts',(-9.08677747601238,73.9130579611989,12.));
#99618=CARTESIAN_POINT('Ctrl Pts',(-9.09559760528458,73.9273231219464,0.));
#99619=CARTESIAN_POINT('Ctrl Pts',(-9.09559760528458,73.9273231219464,12.));
#99620=CARTESIAN_POINT('Ctrl Pts',(-9.10148558516324,73.9368365074164,0.));
#99621=CARTESIAN_POINT('Ctrl Pts',(-9.10148558516324,73.9368365074164,12.));
#99622=CARTESIAN_POINT('Ctrl Pts',(-9.10443154852687,73.9415940197274,0.));
#99623=CARTESIAN_POINT('Ctrl Pts',(-9.10443154852687,73.9415940197274,12.));
#99624=CARTESIAN_POINT('',(-6.95102489306926,69.6540253893192,0.));
#99625=CARTESIAN_POINT('Ctrl Pts',(-6.95102489306926,69.6540253893192,0.));
#99626=CARTESIAN_POINT('Ctrl Pts',(-6.95238884849025,69.6576616146467,0.));
#99627=CARTESIAN_POINT('Ctrl Pts',(-6.955120653176,69.664938391983,0.));
#99628=CARTESIAN_POINT('Ctrl Pts',(-6.95923004173591,69.6758665380378,0.));
#99629=CARTESIAN_POINT('Ctrl Pts',(-6.96473259049513,69.6904633605421,0.));
#99630=CARTESIAN_POINT('Ctrl Pts',(-6.9716497229144,69.7087526479973,0.));
#99631=CARTESIAN_POINT('Ctrl Pts',(-6.97860581164527,69.7270851557366,0.));
#99632=CARTESIAN_POINT('Ctrl Pts',(-6.98560086924214,69.7454607995607,0.));
#99633=CARTESIAN_POINT('Ctrl Pts',(-6.9926349102794,69.7638794280419,0.));
#99634=CARTESIAN_POINT('Ctrl Pts',(-6.99970795069476,69.782340824259,0.));
#99635=CARTESIAN_POINT('Ctrl Pts',(-7.00682000718151,69.8008447346863,0.));
#99636=CARTESIAN_POINT('Ctrl Pts',(-7.01397109655455,69.8193908913722,0.));
#99637=CARTESIAN_POINT('Ctrl Pts',(-7.02116123514452,69.8379790360518,0.));
#99638=CARTESIAN_POINT('Ctrl Pts',(-7.02839043811812,69.8566089455375,0.));
#99639=CARTESIAN_POINT('Ctrl Pts',(-7.03565871972221,69.8752804235238,0.));
#99640=CARTESIAN_POINT('Ctrl Pts',(-7.04296609362166,69.8939932885841,0.));
#99641=CARTESIAN_POINT('Ctrl Pts',(-7.05031257318115,69.9127473642099,0.));
#99642=CARTESIAN_POINT('Ctrl Pts',(-7.05769817180857,69.9315424664291,0.));
#99643=CARTESIAN_POINT('Ctrl Pts',(-7.0651229031285,69.9503783975727,0.));
#99644=CARTESIAN_POINT('Ctrl Pts',(-7.07258678080831,69.9692549527296,0.));
#99645=CARTESIAN_POINT('Ctrl Pts',(-7.08008981844652,69.988171923788,0.));
#99646=CARTESIAN_POINT('Ctrl Pts',(-7.08763202944246,70.0071291040766,0.));
#99647=CARTESIAN_POINT('Ctrl Pts',(-7.09521342684249,70.0261262936388,0.));
#99648=CARTESIAN_POINT('Ctrl Pts',(-7.10283402335034,70.0451632990086,0.));
#99649=CARTESIAN_POINT('Ctrl Pts',(-7.11049383140446,70.0642399306869,0.));
#99650=CARTESIAN_POINT('Ctrl Pts',(-7.11819286322826,70.0833560013975,0.));
#99651=CARTESIAN_POINT('Ctrl Pts',(-7.12593113088904,70.1025113239495,0.));
#99652=CARTESIAN_POINT('Ctrl Pts',(-7.13370864634442,70.1217057094499,0.));
#99653=CARTESIAN_POINT('Ctrl Pts',(-7.14152542142374,70.1409389682424,0.));
#99654=CARTESIAN_POINT('Ctrl Pts',(-7.14938146780813,70.1602109107202,0.));
#99655=CARTESIAN_POINT('Ctrl Pts',(-7.15727679700933,70.1795213481185,0.));
#99656=CARTESIAN_POINT('Ctrl Pts',(-7.16521142033864,70.1988700934593,0.));
#99657=CARTESIAN_POINT('Ctrl Pts',(-7.17318534889716,70.2182569618994,0.));
#99658=CARTESIAN_POINT('Ctrl Pts',(-7.18119859359778,70.2376817702215,0.));
#99659=CARTESIAN_POINT('Ctrl Pts',(-7.18925116517555,70.2571443365192,0.));
#99660=CARTESIAN_POINT('Ctrl Pts',(-7.19734307419873,70.2766444798285,0.));
#99661=CARTESIAN_POINT('Ctrl Pts',(-7.20547433107483,70.2961820197077,0.));
#99662=CARTESIAN_POINT('Ctrl Pts',(-7.2136449460545,70.3157567762588,0.));
#99663=CARTESIAN_POINT('Ctrl Pts',(-7.22185492923191,70.3353685703112,0.));
#99664=CARTESIAN_POINT('Ctrl Pts',(-7.23010429054229,70.3550172235486,0.));
#99665=CARTESIAN_POINT('Ctrl Pts',(-7.23839303975607,70.3747025586552,0.));
#99666=CARTESIAN_POINT('Ctrl Pts',(-7.24672118647085,70.3944243994504,0.));
#99667=CARTESIAN_POINT('Ctrl Pts',(-7.25508874012043,70.4141825708178,0.));
#99668=CARTESIAN_POINT('Ctrl Pts',(-7.26349570998033,70.4339768986346,0.));
#99669=CARTESIAN_POINT('Ctrl Pts',(-7.27194210517063,70.4538072096992,0.));
#99670=CARTESIAN_POINT('Ctrl Pts',(-7.28042793465471,70.4736733316487,0.));
#99671=CARTESIAN_POINT('Ctrl Pts',(-7.28895320723862,70.4935750929058,0.));
#99672=CARTESIAN_POINT('Ctrl Pts',(-7.29751793157823,70.5135123227169,0.));
#99673=CARTESIAN_POINT('Ctrl Pts',(-7.30612211618053,70.5334848511681,0.));
#99674=CARTESIAN_POINT('Ctrl Pts',(-7.31476576940392,70.5534925092043,0.));
#99675=CARTESIAN_POINT('Ctrl Pts',(-7.3234488994522,70.5735351286476,0.));
#99676=CARTESIAN_POINT('Ctrl Pts',(-7.3321715143759,70.5936125421946,0.));
#99677=CARTESIAN_POINT('Ctrl Pts',(-7.34093362208008,70.6137245833996,0.));
#99678=CARTESIAN_POINT('Ctrl Pts',(-7.34973523032577,70.6338710866562,0.));
#99679=CARTESIAN_POINT('Ctrl Pts',(-7.35857634673055,70.6540518871775,0.));
#99680=CARTESIAN_POINT('Ctrl Pts',(-7.36745697876301,70.6742668209687,0.));
#99681=CARTESIAN_POINT('Ctrl Pts',(-7.37637713374768,70.694515724827,0.));
#99682=CARTESIAN_POINT('Ctrl Pts',(-7.38533681887033,70.7147984363424,0.));
#99683=CARTESIAN_POINT('Ctrl Pts',(-7.39433604117891,70.735114793895,0.));
#99684=CARTESIAN_POINT('Ctrl Pts',(-7.4033748075823,70.7554646366514,0.));
#99685=CARTESIAN_POINT('Ctrl Pts',(-7.41245312484487,70.7758478045576,0.));
#99686=CARTESIAN_POINT('Ctrl Pts',(-7.42157099959316,70.7962641383351,0.));
#99687=CARTESIAN_POINT('Ctrl Pts',(-7.43072843832008,70.8167134794738,0.));
#99688=CARTESIAN_POINT('Ctrl Pts',(-7.43992544738607,70.8371956702242,0.));
#99689=CARTESIAN_POINT('Ctrl Pts',(-7.44916203301645,70.8577105535841,0.));
#99690=CARTESIAN_POINT('Ctrl Pts',(-7.45843820129776,70.8782579732885,0.));
#99691=CARTESIAN_POINT('Ctrl Pts',(-7.46775395818519,70.8988377738088,0.));
#99692=CARTESIAN_POINT('Ctrl Pts',(-7.47710930950554,70.9194498003483,0.));
#99693=CARTESIAN_POINT('Ctrl Pts',(-7.48650426095823,70.9400938988373,0.));
#99694=CARTESIAN_POINT('Ctrl Pts',(-7.49593881811141,70.9607699159234,0.));
#99695=CARTESIAN_POINT('Ctrl Pts',(-7.50541298639948,70.9814776989637,0.));
#99696=CARTESIAN_POINT('Ctrl Pts',(-7.51492677113112,71.0022170960235,0.));
#99697=CARTESIAN_POINT('Ctrl Pts',(-7.52448017749136,71.0229879558713,0.));
#99698=CARTESIAN_POINT('Ctrl Pts',(-7.53407321054254,71.0437901279722,0.));
#99699=CARTESIAN_POINT('Ctrl Pts',(-7.54370587521948,71.0646234624783,0.));
#99700=CARTESIAN_POINT('Ctrl Pts',(-7.55337817632873,71.0854878102203,0.));
#99701=CARTESIAN_POINT('Ctrl Pts',(-7.56309011855617,71.1063830227074,0.));
#99702=CARTESIAN_POINT('Ctrl Pts',(-7.57284170646866,71.1273089521218,0.));
#99703=CARTESIAN_POINT('Ctrl Pts',(-7.58263294451465,71.1482654513133,0.));
#99704=CARTESIAN_POINT('Ctrl Pts',(-7.5924638370186,71.1692523737887,0.));
#99705=CARTESIAN_POINT('Ctrl Pts',(-7.60233438818156,71.1902695737063,0.));
#99706=CARTESIAN_POINT('Ctrl Pts',(-7.61224460208887,71.2113169058778,0.));
#99707=CARTESIAN_POINT('Ctrl Pts',(-7.62219448271125,71.232394225762,0.));
#99708=CARTESIAN_POINT('Ctrl Pts',(-7.63218403390515,71.2535013894587,0.));
#99709=CARTESIAN_POINT('Ctrl Pts',(-7.64221325940672,71.2746382536974,0.));
#99710=CARTESIAN_POINT('Ctrl Pts',(-7.65228216283343,71.2958046758334,0.));
#99711=CARTESIAN_POINT('Ctrl Pts',(-7.66239074769119,71.3170005138474,0.));
#99712=CARTESIAN_POINT('Ctrl Pts',(-7.67253901737539,71.3382256263405,0.));
#99713=CARTESIAN_POINT('Ctrl Pts',(-7.68272697517103,71.3594798725294,0.));
#99714=CARTESIAN_POINT('Ctrl Pts',(-7.69295462424647,71.380763112236,0.));
#99715=CARTESIAN_POINT('Ctrl Pts',(-7.70322196765573,71.4020752058827,0.));
#99716=CARTESIAN_POINT('Ctrl Pts',(-7.71352900834538,71.4234160144943,0.));
#99717=CARTESIAN_POINT('Ctrl Pts',(-7.72387574915544,71.4447853996919,0.));
#99718=CARTESIAN_POINT('Ctrl Pts',(-7.73426219281932,71.4661832236881,0.));
#99719=CARTESIAN_POINT('Ctrl Pts',(-7.74468834195734,71.487609349277,0.));
#99720=CARTESIAN_POINT('Ctrl Pts',(-7.75515419907955,71.5090636398307,0.));
#99721=CARTESIAN_POINT('Ctrl Pts',(-7.76565976659218,71.5305459592987,0.));
#99722=CARTESIAN_POINT('Ctrl Pts',(-7.77620504679868,71.5520561722039,0.));
#99723=CARTESIAN_POINT('Ctrl Pts',(-7.78679004189935,71.5735941436366,0.));
#99724=CARTESIAN_POINT('Ctrl Pts',(-7.79741475398512,71.5951597392471,0.));
#99725=CARTESIAN_POINT('Ctrl Pts',(-7.80807918504017,71.616752825242,0.));
#99726=CARTESIAN_POINT('Ctrl Pts',(-7.81878333694856,71.638373268384,0.));
#99727=CARTESIAN_POINT('Ctrl Pts',(-7.82952721149504,71.6600209359869,0.));
#99728=CARTESIAN_POINT('Ctrl Pts',(-7.84031081036489,71.681695695912,0.));
#99729=CARTESIAN_POINT('Ctrl Pts',(-7.85113413513739,71.7033974165576,0.));
#99730=CARTESIAN_POINT('Ctrl Pts',(-7.8619971872883,71.7251259668573,0.));
#99731=CARTESIAN_POINT('Ctrl Pts',(-7.87289996819654,71.7468812162795,0.));
#99732=CARTESIAN_POINT('Ctrl Pts',(-7.88384247914522,71.768663034824,0.));
#99733=CARTESIAN_POINT('Ctrl Pts',(-7.89482472132135,71.7904712930172,0.));
#99734=CARTESIAN_POINT('Ctrl Pts',(-7.90584669580955,71.8123058619038,0.));
#99735=CARTESIAN_POINT('Ctrl Pts',(-7.91690840359371,71.8341666130424,0.));
#99736=CARTESIAN_POINT('Ctrl Pts',(-7.928009845564,71.8560534185071,0.));
#99737=CARTESIAN_POINT('Ctrl Pts',(-7.93915102251796,71.8779661508833,0.));
#99738=CARTESIAN_POINT('Ctrl Pts',(-7.95033193516046,71.8999046832642,0.));
#99739=CARTESIAN_POINT('Ctrl Pts',(-7.96155258409752,71.9218688892426,0.));
#99740=CARTESIAN_POINT('Ctrl Pts',(-7.97281296983702,71.9438586429072,0.));
#99741=CARTESIAN_POINT('Ctrl Pts',(-7.98411309279598,71.9658738188421,0.));
#99742=CARTESIAN_POINT('Ctrl Pts',(-7.99545295330182,71.9879142921248,0.));
#99743=CARTESIAN_POINT('Ctrl Pts',(-8.0068325515925,72.0099799383216,0.));
#99744=CARTESIAN_POINT('Ctrl Pts',(-8.0182518878107,72.0320706334802,0.));
#99745=CARTESIAN_POINT('Ctrl Pts',(-8.02971096200329,72.0541862541262,0.));
#99746=CARTESIAN_POINT('Ctrl Pts',(-8.04120977412891,72.0763266772632,0.));
#99747=CARTESIAN_POINT('Ctrl Pts',(-8.05274832405957,72.0984917803702,0.));
#99748=CARTESIAN_POINT('Ctrl Pts',(-8.06432661158089,72.1206814413985,0.));
#99749=CARTESIAN_POINT('Ctrl Pts',(-8.07594463638699,72.1428955387648,0.));
#99750=CARTESIAN_POINT('Ctrl Pts',(-8.08760239807815,72.165133951346,0.));
#99751=CARTESIAN_POINT('Ctrl Pts',(-8.09929989616874,72.18739655848,0.));
#99752=CARTESIAN_POINT('Ctrl Pts',(-8.11103713008922,72.2096832399626,0.));
#99753=CARTESIAN_POINT('Ctrl Pts',(-8.12281409918662,72.2319938760451,0.));
#99754=CARTESIAN_POINT('Ctrl Pts',(-8.13463080272029,72.2543283474279,0.));
#99755=CARTESIAN_POINT('Ctrl Pts',(-8.14648723985793,72.2766865352552,0.));
#99756=CARTESIAN_POINT('Ctrl Pts',(-8.15838340968328,72.2990683211155,0.));
#99757=CARTESIAN_POINT('Ctrl Pts',(-8.17031931119882,72.3214735870402,0.));
#99758=CARTESIAN_POINT('Ctrl Pts',(-8.18229494332622,72.3439022155007,0.));
#99759=CARTESIAN_POINT('Ctrl Pts',(-8.19431030490319,72.3663540894034,0.));
#99760=CARTESIAN_POINT('Ctrl Pts',(-8.20636539467782,72.3888290920845,0.));
#99761=CARTESIAN_POINT('Ctrl Pts',(-8.21846021131564,72.4113271073091,0.));
#99762=CARTESIAN_POINT('Ctrl Pts',(-8.23059475340354,72.4338480192701,0.));
#99763=CARTESIAN_POINT('Ctrl Pts',(-8.24276901945037,72.4563917125842,0.));
#99764=CARTESIAN_POINT('Ctrl Pts',(-8.25498300788493,72.4789580722871,0.));
#99765=CARTESIAN_POINT('Ctrl Pts',(-8.26723671704924,72.501546983825,0.));
#99766=CARTESIAN_POINT('Ctrl Pts',(-8.27953014520385,72.524158333056,0.));
#99767=CARTESIAN_POINT('Ctrl Pts',(-8.29186329053289,72.5467920062522,0.));
#99768=CARTESIAN_POINT('Ctrl Pts',(-8.30423615114455,72.5694478900983,0.));
#99769=CARTESIAN_POINT('Ctrl Pts',(-8.31664872507008,72.5921258716899,0.));
#99770=CARTESIAN_POINT('Ctrl Pts',(-8.32910101025653,72.614825838529,0.));
#99771=CARTESIAN_POINT('Ctrl Pts',(-8.34159300456965,72.6375476785208,0.));
#99772=CARTESIAN_POINT('Ctrl Pts',(-8.35412470580083,72.6602912799689,0.));
#99773=CARTESIAN_POINT('Ctrl Pts',(-8.36669611166834,72.68305653157,0.));
#99774=CARTESIAN_POINT('Ctrl Pts',(-8.37930721981735,72.7058433224072,0.));
#99775=CARTESIAN_POINT('Ctrl Pts',(-8.39195802781407,72.728651541938,0.));
#99776=CARTESIAN_POINT('Ctrl Pts',(-8.40464853314493,72.7514810799932,0.));
#99777=CARTESIAN_POINT('Ctrl Pts',(-8.41737873322353,72.7743318267876,0.));
#99778=CARTESIAN_POINT('Ctrl Pts',(-8.43014862539171,72.7972036729283,0.));
#99779=CARTESIAN_POINT('Ctrl Pts',(-8.44295820691907,72.8200965094197,0.));
#99780=CARTESIAN_POINT('Ctrl Pts',(-8.45580747499771,72.8430102276703,0.));
#99781=CARTESIAN_POINT('Ctrl Pts',(-8.46869642673763,72.8659447194918,0.));
#99782=CARTESIAN_POINT('Ctrl Pts',(-8.48162505917628,72.888899877077,0.));
#99783=CARTESIAN_POINT('Ctrl Pts',(-8.49459336928276,72.9118755929785,0.));
#99784=CARTESIAN_POINT('Ctrl Pts',(-8.50760135395979,72.9348717600837,0.));
#99785=CARTESIAN_POINT('Ctrl Pts',(-8.52064901004244,72.9578882715923,0.));
#99786=CARTESIAN_POINT('Ctrl Pts',(-8.53373633429303,72.9809250209843,0.));
#99787=CARTESIAN_POINT('Ctrl Pts',(-8.54686332340439,73.0039819020663,0.));
#99788=CARTESIAN_POINT('Ctrl Pts',(-8.56002997400096,73.0270588090193,0.));
#99789=CARTESIAN_POINT('Ctrl Pts',(-8.57323628263595,73.0501556364482,0.));
#99790=CARTESIAN_POINT('Ctrl Pts',(-8.58648224578723,73.073272279419,0.));
#99791=CARTESIAN_POINT('Ctrl Pts',(-8.59976785984539,73.0964086335226,0.));
#99792=CARTESIAN_POINT('Ctrl Pts',(-8.61309312111989,73.1195645948169,0.));
#99793=CARTESIAN_POINT('Ctrl Pts',(-8.62645802585475,73.142740059703,0.));
#99794=CARTESIAN_POINT('Ctrl Pts',(-8.63986257023735,73.165934924813,0.));
#99795=CARTESIAN_POINT('Ctrl Pts',(-8.65330675040535,73.1891490869057,0.));
#99796=CARTESIAN_POINT('Ctrl Pts',(-8.66679056245095,73.2123824427212,0.));
#99797=CARTESIAN_POINT('Ctrl Pts',(-8.68031400241884,73.2356348889704,0.));
#99798=CARTESIAN_POINT('Ctrl Pts',(-8.69387706629304,73.2589063226373,0.));
#99799=CARTESIAN_POINT('Ctrl Pts',(-8.70747974998245,73.282196641216,0.));
#99800=CARTESIAN_POINT('Ctrl Pts',(-8.72112204930232,73.3055057429744,0.));
#99801=CARTESIAN_POINT('Ctrl Pts',(-8.7348039599536,73.3288335271989,0.));
#99802=CARTESIAN_POINT('Ctrl Pts',(-8.74852547749736,73.3521798944595,0.));
#99803=CARTESIAN_POINT('Ctrl Pts',(-8.76228659740305,73.3755447460235,0.));
#99804=CARTESIAN_POINT('Ctrl Pts',(-8.77608731509304,73.3989279832808,0.));
#99805=CARTESIAN_POINT('Ctrl Pts',(-8.78992762598738,73.422329507112,0.));
#99806=CARTESIAN_POINT('Ctrl Pts',(-8.80380752553714,73.4457492173949,0.));
#99807=CARTESIAN_POINT('Ctrl Pts',(-8.81772700927593,73.4691870121608,0.));
#99808=CARTESIAN_POINT('Ctrl Pts',(-8.83168607277415,73.4926427882787,0.));
#99809=CARTESIAN_POINT('Ctrl Pts',(-8.84568471153894,73.5161164429765,0.));
#99810=CARTESIAN_POINT('Ctrl Pts',(-8.85972292092183,73.5396078751672,0.));
#99811=CARTESIAN_POINT('Ctrl Pts',(-8.87380069602955,73.5631169867113,0.));
#99812=CARTESIAN_POINT('Ctrl Pts',(-8.88791803160341,73.5866436840493,0.));
#99813=CARTESIAN_POINT('Ctrl Pts',(-8.90207492198871,73.6101878785868,0.));
#99814=CARTESIAN_POINT('Ctrl Pts',(-8.91424402151025,73.6303847393445,0.));
#99815=CARTESIAN_POINT('Ctrl Pts',(-8.92359518177556,73.6458786305789,0.));
#99816=CARTESIAN_POINT('Ctrl Pts',(-8.93011088816032,73.6566618621798,0.));
#99817=CARTESIAN_POINT('Ctrl Pts',(-8.93377955963992,73.6627293782263,0.));
#99818=CARTESIAN_POINT('Ctrl Pts',(-8.93459554655822,73.6640787197672,0.));
#99819=CARTESIAN_POINT('',(-6.95102489306926,69.6540253893192,12.));
#99820=CARTESIAN_POINT('',(-6.95102489306926,69.6540253893192,0.));
#99821=CARTESIAN_POINT('Ctrl Pts',(-8.93459554655822,73.6640787197672,12.));
#99822=CARTESIAN_POINT('Ctrl Pts',(-8.93377955963992,73.6627293782263,12.));
#99823=CARTESIAN_POINT('Ctrl Pts',(-8.93011088816032,73.6566618621798,12.));
#99824=CARTESIAN_POINT('Ctrl Pts',(-8.92359518177556,73.6458786305789,12.));
#99825=CARTESIAN_POINT('Ctrl Pts',(-8.91424402151025,73.6303847393445,12.));
#99826=CARTESIAN_POINT('Ctrl Pts',(-8.90207492198871,73.6101878785868,12.));
#99827=CARTESIAN_POINT('Ctrl Pts',(-8.88791803160341,73.5866436840493,12.));
#99828=CARTESIAN_POINT('Ctrl Pts',(-8.87380069602955,73.5631169867113,12.));
#99829=CARTESIAN_POINT('Ctrl Pts',(-8.85972292092183,73.5396078751672,12.));
#99830=CARTESIAN_POINT('Ctrl Pts',(-8.84568471153894,73.5161164429765,12.));
#99831=CARTESIAN_POINT('Ctrl Pts',(-8.83168607277415,73.4926427882787,12.));
#99832=CARTESIAN_POINT('Ctrl Pts',(-8.81772700927593,73.4691870121608,12.));
#99833=CARTESIAN_POINT('Ctrl Pts',(-8.80380752553714,73.4457492173949,12.));
#99834=CARTESIAN_POINT('Ctrl Pts',(-8.78992762598738,73.422329507112,12.));
#99835=CARTESIAN_POINT('Ctrl Pts',(-8.77608731509304,73.3989279832808,12.));
#99836=CARTESIAN_POINT('Ctrl Pts',(-8.76228659740305,73.3755447460235,12.));
#99837=CARTESIAN_POINT('Ctrl Pts',(-8.74852547749736,73.3521798944595,12.));
#99838=CARTESIAN_POINT('Ctrl Pts',(-8.7348039599536,73.3288335271989,12.));
#99839=CARTESIAN_POINT('Ctrl Pts',(-8.72112204930232,73.3055057429744,12.));
#99840=CARTESIAN_POINT('Ctrl Pts',(-8.70747974998245,73.282196641216,12.));
#99841=CARTESIAN_POINT('Ctrl Pts',(-8.69387706629304,73.2589063226373,12.));
#99842=CARTESIAN_POINT('Ctrl Pts',(-8.68031400241884,73.2356348889704,12.));
#99843=CARTESIAN_POINT('Ctrl Pts',(-8.66679056245095,73.2123824427212,12.));
#99844=CARTESIAN_POINT('Ctrl Pts',(-8.65330675040535,73.1891490869057,12.));
#99845=CARTESIAN_POINT('Ctrl Pts',(-8.63986257023735,73.165934924813,12.));
#99846=CARTESIAN_POINT('Ctrl Pts',(-8.62645802585475,73.142740059703,12.));
#99847=CARTESIAN_POINT('Ctrl Pts',(-8.61309312111989,73.1195645948169,12.));
#99848=CARTESIAN_POINT('Ctrl Pts',(-8.59976785984539,73.0964086335226,12.));
#99849=CARTESIAN_POINT('Ctrl Pts',(-8.58648224578723,73.073272279419,12.));
#99850=CARTESIAN_POINT('Ctrl Pts',(-8.57323628263595,73.0501556364482,12.));
#99851=CARTESIAN_POINT('Ctrl Pts',(-8.56002997400096,73.0270588090193,12.));
#99852=CARTESIAN_POINT('Ctrl Pts',(-8.54686332340439,73.0039819020663,12.));
#99853=CARTESIAN_POINT('Ctrl Pts',(-8.53373633429303,72.9809250209843,12.));
#99854=CARTESIAN_POINT('Ctrl Pts',(-8.52064901004244,72.9578882715923,12.));
#99855=CARTESIAN_POINT('Ctrl Pts',(-8.50760135395979,72.9348717600837,12.));
#99856=CARTESIAN_POINT('Ctrl Pts',(-8.49459336928276,72.9118755929785,12.));
#99857=CARTESIAN_POINT('Ctrl Pts',(-8.48162505917628,72.888899877077,12.));
#99858=CARTESIAN_POINT('Ctrl Pts',(-8.46869642673763,72.8659447194918,12.));
#99859=CARTESIAN_POINT('Ctrl Pts',(-8.45580747499771,72.8430102276703,12.));
#99860=CARTESIAN_POINT('Ctrl Pts',(-8.44295820691907,72.8200965094197,12.));
#99861=CARTESIAN_POINT('Ctrl Pts',(-8.43014862539171,72.7972036729283,12.));
#99862=CARTESIAN_POINT('Ctrl Pts',(-8.41737873322353,72.7743318267876,12.));
#99863=CARTESIAN_POINT('Ctrl Pts',(-8.40464853314493,72.7514810799932,12.));
#99864=CARTESIAN_POINT('Ctrl Pts',(-8.39195802781407,72.728651541938,12.));
#99865=CARTESIAN_POINT('Ctrl Pts',(-8.37930721981735,72.7058433224072,12.));
#99866=CARTESIAN_POINT('Ctrl Pts',(-8.36669611166834,72.68305653157,12.));
#99867=CARTESIAN_POINT('Ctrl Pts',(-8.35412470580083,72.6602912799689,12.));
#99868=CARTESIAN_POINT('Ctrl Pts',(-8.34159300456965,72.6375476785208,12.));
#99869=CARTESIAN_POINT('Ctrl Pts',(-8.32910101025653,72.614825838529,12.));
#99870=CARTESIAN_POINT('Ctrl Pts',(-8.31664872507008,72.5921258716899,12.));
#99871=CARTESIAN_POINT('Ctrl Pts',(-8.30423615114455,72.5694478900983,12.));
#99872=CARTESIAN_POINT('Ctrl Pts',(-8.29186329053289,72.5467920062522,12.));
#99873=CARTESIAN_POINT('Ctrl Pts',(-8.27953014520385,72.524158333056,12.));
#99874=CARTESIAN_POINT('Ctrl Pts',(-8.26723671704924,72.501546983825,12.));
#99875=CARTESIAN_POINT('Ctrl Pts',(-8.25498300788493,72.4789580722871,12.));
#99876=CARTESIAN_POINT('Ctrl Pts',(-8.24276901945037,72.4563917125842,12.));
#99877=CARTESIAN_POINT('Ctrl Pts',(-8.23059475340354,72.4338480192701,12.));
#99878=CARTESIAN_POINT('Ctrl Pts',(-8.21846021131564,72.4113271073091,12.));
#99879=CARTESIAN_POINT('Ctrl Pts',(-8.20636539467782,72.3888290920845,12.));
#99880=CARTESIAN_POINT('Ctrl Pts',(-8.19431030490319,72.3663540894034,12.));
#99881=CARTESIAN_POINT('Ctrl Pts',(-8.18229494332622,72.3439022155007,12.));
#99882=CARTESIAN_POINT('Ctrl Pts',(-8.17031931119882,72.3214735870402,12.));
#99883=CARTESIAN_POINT('Ctrl Pts',(-8.15838340968328,72.2990683211155,12.));
#99884=CARTESIAN_POINT('Ctrl Pts',(-8.14648723985793,72.2766865352552,12.));
#99885=CARTESIAN_POINT('Ctrl Pts',(-8.13463080272029,72.2543283474279,12.));
#99886=CARTESIAN_POINT('Ctrl Pts',(-8.12281409918662,72.2319938760451,12.));
#99887=CARTESIAN_POINT('Ctrl Pts',(-8.11103713008922,72.2096832399626,12.));
#99888=CARTESIAN_POINT('Ctrl Pts',(-8.09929989616874,72.18739655848,12.));
#99889=CARTESIAN_POINT('Ctrl Pts',(-8.08760239807815,72.165133951346,12.));
#99890=CARTESIAN_POINT('Ctrl Pts',(-8.07594463638699,72.1428955387648,12.));
#99891=CARTESIAN_POINT('Ctrl Pts',(-8.06432661158089,72.1206814413985,12.));
#99892=CARTESIAN_POINT('Ctrl Pts',(-8.05274832405957,72.0984917803702,12.));
#99893=CARTESIAN_POINT('Ctrl Pts',(-8.04120977412891,72.0763266772632,12.));
#99894=CARTESIAN_POINT('Ctrl Pts',(-8.02971096200329,72.0541862541262,12.));
#99895=CARTESIAN_POINT('Ctrl Pts',(-8.0182518878107,72.0320706334802,12.));
#99896=CARTESIAN_POINT('Ctrl Pts',(-8.0068325515925,72.0099799383216,12.));
#99897=CARTESIAN_POINT('Ctrl Pts',(-7.99545295330182,71.9879142921248,12.));
#99898=CARTESIAN_POINT('Ctrl Pts',(-7.98411309279598,71.9658738188421,12.));
#99899=CARTESIAN_POINT('Ctrl Pts',(-7.97281296983702,71.9438586429072,12.));
#99900=CARTESIAN_POINT('Ctrl Pts',(-7.96155258409752,71.9218688892426,12.));
#99901=CARTESIAN_POINT('Ctrl Pts',(-7.95033193516046,71.8999046832642,12.));
#99902=CARTESIAN_POINT('Ctrl Pts',(-7.93915102251796,71.8779661508833,12.));
#99903=CARTESIAN_POINT('Ctrl Pts',(-7.928009845564,71.8560534185071,12.));
#99904=CARTESIAN_POINT('Ctrl Pts',(-7.91690840359371,71.8341666130424,12.));
#99905=CARTESIAN_POINT('Ctrl Pts',(-7.90584669580955,71.8123058619038,12.));
#99906=CARTESIAN_POINT('Ctrl Pts',(-7.89482472132135,71.7904712930172,12.));
#99907=CARTESIAN_POINT('Ctrl Pts',(-7.88384247914522,71.768663034824,12.));
#99908=CARTESIAN_POINT('Ctrl Pts',(-7.87289996819654,71.7468812162795,12.));
#99909=CARTESIAN_POINT('Ctrl Pts',(-7.8619971872883,71.7251259668573,12.));
#99910=CARTESIAN_POINT('Ctrl Pts',(-7.85113413513739,71.7033974165576,12.));
#99911=CARTESIAN_POINT('Ctrl Pts',(-7.84031081036489,71.681695695912,12.));
#99912=CARTESIAN_POINT('Ctrl Pts',(-7.82952721149504,71.6600209359869,12.));
#99913=CARTESIAN_POINT('Ctrl Pts',(-7.81878333694856,71.638373268384,12.));
#99914=CARTESIAN_POINT('Ctrl Pts',(-7.80807918504017,71.616752825242,12.));
#99915=CARTESIAN_POINT('Ctrl Pts',(-7.79741475398512,71.5951597392471,12.));
#99916=CARTESIAN_POINT('Ctrl Pts',(-7.78679004189935,71.5735941436366,12.));
#99917=CARTESIAN_POINT('Ctrl Pts',(-7.77620504679868,71.5520561722039,12.));
#99918=CARTESIAN_POINT('Ctrl Pts',(-7.76565976659218,71.5305459592987,12.));
#99919=CARTESIAN_POINT('Ctrl Pts',(-7.75515419907955,71.5090636398307,12.));
#99920=CARTESIAN_POINT('Ctrl Pts',(-7.74468834195734,71.487609349277,12.));
#99921=CARTESIAN_POINT('Ctrl Pts',(-7.73426219281932,71.4661832236881,12.));
#99922=CARTESIAN_POINT('Ctrl Pts',(-7.72387574915544,71.4447853996919,12.));
#99923=CARTESIAN_POINT('Ctrl Pts',(-7.71352900834538,71.4234160144943,12.));
#99924=CARTESIAN_POINT('Ctrl Pts',(-7.70322196765573,71.4020752058827,12.));
#99925=CARTESIAN_POINT('Ctrl Pts',(-7.69295462424647,71.380763112236,12.));
#99926=CARTESIAN_POINT('Ctrl Pts',(-7.68272697517103,71.3594798725294,12.));
#99927=CARTESIAN_POINT('Ctrl Pts',(-7.67253901737539,71.3382256263405,12.));
#99928=CARTESIAN_POINT('Ctrl Pts',(-7.66239074769119,71.3170005138474,12.));
#99929=CARTESIAN_POINT('Ctrl Pts',(-7.65228216283343,71.2958046758334,12.));
#99930=CARTESIAN_POINT('Ctrl Pts',(-7.64221325940672,71.2746382536974,12.));
#99931=CARTESIAN_POINT('Ctrl Pts',(-7.63218403390515,71.2535013894587,12.));
#99932=CARTESIAN_POINT('Ctrl Pts',(-7.62219448271125,71.232394225762,12.));
#99933=CARTESIAN_POINT('Ctrl Pts',(-7.61224460208887,71.2113169058778,12.));
#99934=CARTESIAN_POINT('Ctrl Pts',(-7.60233438818156,71.1902695737063,12.));
#99935=CARTESIAN_POINT('Ctrl Pts',(-7.5924638370186,71.1692523737887,12.));
#99936=CARTESIAN_POINT('Ctrl Pts',(-7.58263294451465,71.1482654513133,12.));
#99937=CARTESIAN_POINT('Ctrl Pts',(-7.57284170646866,71.1273089521218,12.));
#99938=CARTESIAN_POINT('Ctrl Pts',(-7.56309011855617,71.1063830227074,12.));
#99939=CARTESIAN_POINT('Ctrl Pts',(-7.55337817632873,71.0854878102203,12.));
#99940=CARTESIAN_POINT('Ctrl Pts',(-7.54370587521948,71.0646234624783,12.));
#99941=CARTESIAN_POINT('Ctrl Pts',(-7.53407321054254,71.0437901279722,12.));
#99942=CARTESIAN_POINT('Ctrl Pts',(-7.52448017749136,71.0229879558713,12.));
#99943=CARTESIAN_POINT('Ctrl Pts',(-7.51492677113112,71.0022170960235,12.));
#99944=CARTESIAN_POINT('Ctrl Pts',(-7.50541298639948,70.9814776989637,12.));
#99945=CARTESIAN_POINT('Ctrl Pts',(-7.49593881811141,70.9607699159234,12.));
#99946=CARTESIAN_POINT('Ctrl Pts',(-7.48650426095823,70.9400938988373,12.));
#99947=CARTESIAN_POINT('Ctrl Pts',(-7.47710930950554,70.9194498003483,12.));
#99948=CARTESIAN_POINT('Ctrl Pts',(-7.46775395818519,70.8988377738088,12.));
#99949=CARTESIAN_POINT('Ctrl Pts',(-7.45843820129776,70.8782579732885,12.));
#99950=CARTESIAN_POINT('Ctrl Pts',(-7.44916203301645,70.8577105535841,12.));
#99951=CARTESIAN_POINT('Ctrl Pts',(-7.43992544738607,70.8371956702242,12.));
#99952=CARTESIAN_POINT('Ctrl Pts',(-7.43072843832008,70.8167134794738,12.));
#99953=CARTESIAN_POINT('Ctrl Pts',(-7.42157099959316,70.7962641383351,12.));
#99954=CARTESIAN_POINT('Ctrl Pts',(-7.41245312484487,70.7758478045576,12.));
#99955=CARTESIAN_POINT('Ctrl Pts',(-7.4033748075823,70.7554646366514,12.));
#99956=CARTESIAN_POINT('Ctrl Pts',(-7.39433604117891,70.735114793895,12.));
#99957=CARTESIAN_POINT('Ctrl Pts',(-7.38533681887033,70.7147984363424,12.));
#99958=CARTESIAN_POINT('Ctrl Pts',(-7.37637713374768,70.694515724827,12.));
#99959=CARTESIAN_POINT('Ctrl Pts',(-7.36745697876301,70.6742668209687,12.));
#99960=CARTESIAN_POINT('Ctrl Pts',(-7.35857634673055,70.6540518871775,12.));
#99961=CARTESIAN_POINT('Ctrl Pts',(-7.34973523032577,70.6338710866562,12.));
#99962=CARTESIAN_POINT('Ctrl Pts',(-7.34093362208008,70.6137245833996,12.));
#99963=CARTESIAN_POINT('Ctrl Pts',(-7.3321715143759,70.5936125421946,12.));
#99964=CARTESIAN_POINT('Ctrl Pts',(-7.3234488994522,70.5735351286476,12.));
#99965=CARTESIAN_POINT('Ctrl Pts',(-7.31476576940392,70.5534925092043,12.));
#99966=CARTESIAN_POINT('Ctrl Pts',(-7.30612211618053,70.5334848511681,12.));
#99967=CARTESIAN_POINT('Ctrl Pts',(-7.29751793157823,70.5135123227169,12.));
#99968=CARTESIAN_POINT('Ctrl Pts',(-7.28895320723862,70.4935750929058,12.));
#99969=CARTESIAN_POINT('Ctrl Pts',(-7.28042793465471,70.4736733316487,12.));
#99970=CARTESIAN_POINT('Ctrl Pts',(-7.27194210517063,70.4538072096992,12.));
#99971=CARTESIAN_POINT('Ctrl Pts',(-7.26349570998033,70.4339768986346,12.));
#99972=CARTESIAN_POINT('Ctrl Pts',(-7.25508874012043,70.4141825708178,12.));
#99973=CARTESIAN_POINT('Ctrl Pts',(-7.24672118647085,70.3944243994504,12.));
#99974=CARTESIAN_POINT('Ctrl Pts',(-7.23839303975607,70.3747025586552,12.));
#99975=CARTESIAN_POINT('Ctrl Pts',(-7.23010429054229,70.3550172235486,12.));
#99976=CARTESIAN_POINT('Ctrl Pts',(-7.22185492923191,70.3353685703112,12.));
#99977=CARTESIAN_POINT('Ctrl Pts',(-7.2136449460545,70.3157567762588,12.));
#99978=CARTESIAN_POINT('Ctrl Pts',(-7.20547433107483,70.2961820197077,12.));
#99979=CARTESIAN_POINT('Ctrl Pts',(-7.19734307419873,70.2766444798285,12.));
#99980=CARTESIAN_POINT('Ctrl Pts',(-7.18925116517555,70.2571443365192,12.));
#99981=CARTESIAN_POINT('Ctrl Pts',(-7.18119859359778,70.2376817702215,12.));
#99982=CARTESIAN_POINT('Ctrl Pts',(-7.17318534889716,70.2182569618994,12.));
#99983=CARTESIAN_POINT('Ctrl Pts',(-7.16521142033864,70.1988700934593,12.));
#99984=CARTESIAN_POINT('Ctrl Pts',(-7.15727679700933,70.1795213481185,12.));
#99985=CARTESIAN_POINT('Ctrl Pts',(-7.14938146780813,70.1602109107202,12.));
#99986=CARTESIAN_POINT('Ctrl Pts',(-7.14152542142374,70.1409389682424,12.));
#99987=CARTESIAN_POINT('Ctrl Pts',(-7.13370864634442,70.1217057094499,12.));
#99988=CARTESIAN_POINT('Ctrl Pts',(-7.12593113088904,70.1025113239495,12.));
#99989=CARTESIAN_POINT('Ctrl Pts',(-7.11819286322826,70.0833560013975,12.));
#99990=CARTESIAN_POINT('Ctrl Pts',(-7.11049383140446,70.0642399306869,12.));
#99991=CARTESIAN_POINT('Ctrl Pts',(-7.10283402335034,70.0451632990086,12.));
#99992=CARTESIAN_POINT('Ctrl Pts',(-7.09521342684249,70.0261262936388,12.));
#99993=CARTESIAN_POINT('Ctrl Pts',(-7.08763202944246,70.0071291040766,12.));
#99994=CARTESIAN_POINT('Ctrl Pts',(-7.08008981844652,69.988171923788,12.));
#99995=CARTESIAN_POINT('Ctrl Pts',(-7.07258678080831,69.9692549527296,12.));
#99996=CARTESIAN_POINT('Ctrl Pts',(-7.0651229031285,69.9503783975727,12.));
#99997=CARTESIAN_POINT('Ctrl Pts',(-7.05769817180857,69.9315424664291,12.));
#99998=CARTESIAN_POINT('Ctrl Pts',(-7.05031257318115,69.9127473642099,12.));
#99999=CARTESIAN_POINT('Ctrl Pts',(-7.04296609362166,69.8939932885841,12.));
#100000=CARTESIAN_POINT('Ctrl Pts',(-7.03565871972221,69.8752804235238,
12.));
#100001=CARTESIAN_POINT('Ctrl Pts',(-7.02839043811812,69.8566089455375,
12.));
#100002=CARTESIAN_POINT('Ctrl Pts',(-7.02116123514452,69.8379790360518,
12.));
#100003=CARTESIAN_POINT('Ctrl Pts',(-7.01397109655455,69.8193908913722,
12.));
#100004=CARTESIAN_POINT('Ctrl Pts',(-7.00682000718151,69.8008447346863,
12.));
#100005=CARTESIAN_POINT('Ctrl Pts',(-6.99970795069476,69.782340824259,12.));
#100006=CARTESIAN_POINT('Ctrl Pts',(-6.9926349102794,69.7638794280419,12.));
#100007=CARTESIAN_POINT('Ctrl Pts',(-6.98560086924214,69.7454607995607,
12.));
#100008=CARTESIAN_POINT('Ctrl Pts',(-6.97860581164527,69.7270851557366,
12.));
#100009=CARTESIAN_POINT('Ctrl Pts',(-6.9716497229144,69.7087526479973,12.));
#100010=CARTESIAN_POINT('Ctrl Pts',(-6.96473259049513,69.6904633605421,
12.));
#100011=CARTESIAN_POINT('Ctrl Pts',(-6.95923004173591,69.6758665380378,
12.));
#100012=CARTESIAN_POINT('Ctrl Pts',(-6.955120653176,69.664938391983,12.));
#100013=CARTESIAN_POINT('Ctrl Pts',(-6.95238884849025,69.6576616146467,
12.));
#100014=CARTESIAN_POINT('Ctrl Pts',(-6.95102489306926,69.6540253893192,
12.));
#100015=CARTESIAN_POINT('Ctrl Pts',(-10.4355099267296,73.4664795929939,
-5.55111512312578E-16));
#100016=CARTESIAN_POINT('Ctrl Pts',(-10.4355099267296,73.4664795929939,
4.));
#100017=CARTESIAN_POINT('Ctrl Pts',(-10.4355099267296,73.4664795929939,
8.));
#100018=CARTESIAN_POINT('Ctrl Pts',(-10.4355099267296,73.4664795929939,
12.));
#100019=CARTESIAN_POINT('Ctrl Pts',(-10.4049225807075,73.5720190200068,
-5.55111512312578E-16));
#100020=CARTESIAN_POINT('Ctrl Pts',(-10.4049225807075,73.5720190200068,
4.));
#100021=CARTESIAN_POINT('Ctrl Pts',(-10.4049225807075,73.5720190200068,
8.));
#100022=CARTESIAN_POINT('Ctrl Pts',(-10.4049225807075,73.5720190200068,
12.));
#100023=CARTESIAN_POINT('Ctrl Pts',(-10.2883434191783,73.7377969500799,
-5.55111512312578E-16));
#100024=CARTESIAN_POINT('Ctrl Pts',(-10.2883434191783,73.7377969500799,
4.00000000000001));
#100025=CARTESIAN_POINT('Ctrl Pts',(-10.2883434191783,73.7377969500799,
7.99999999999999));
#100026=CARTESIAN_POINT('Ctrl Pts',(-10.2883434191783,73.7377969500799,
12.));
#100027=CARTESIAN_POINT('Ctrl Pts',(-10.1042001607579,73.8116652760546,
-5.55111512312578E-16));
#100028=CARTESIAN_POINT('Ctrl Pts',(-10.1042001607579,73.8116652760546,
4.));
#100029=CARTESIAN_POINT('Ctrl Pts',(-10.1042001607579,73.8116652760546,
8.00000000000001));
#100030=CARTESIAN_POINT('Ctrl Pts',(-10.1042001607579,73.8116652760546,
12.));
#100031=CARTESIAN_POINT('Ctrl Pts',(-10.0225374821233,73.8227522002495,
-5.55111512312578E-16));
#100032=CARTESIAN_POINT('Ctrl Pts',(-10.0225374821233,73.8227522002495,
4.));
#100033=CARTESIAN_POINT('Ctrl Pts',(-10.0225374821233,73.8227522002495,
8.));
#100034=CARTESIAN_POINT('Ctrl Pts',(-10.0225374821233,73.8227522002495,
12.));
#100035=CARTESIAN_POINT('',(-10.4355099267296,73.4664795929939,0.));
#100036=CARTESIAN_POINT('',(-10.0225374821233,73.8227522002494,2.77555756156289E-16));
#100037=CARTESIAN_POINT('Ctrl Pts',(-10.4355099267296,73.4664795929939,
4.16333634234434E-16));
#100038=CARTESIAN_POINT('Ctrl Pts',(-10.4049225807075,73.5720190200068,
4.16333634234433E-16));
#100039=CARTESIAN_POINT('Ctrl Pts',(-10.3383059169765,73.6667492657628,
4.16333634234434E-16));
#100040=CARTESIAN_POINT('Ctrl Pts',(-10.2496275073219,73.7314682122214,
4.16333634234434E-16));
#100041=CARTESIAN_POINT('Ctrl Pts',(-10.1831187000809,73.7800074220654,
4.16333634234434E-16));
#100042=CARTESIAN_POINT('Ctrl Pts',(-10.1042001607579,73.8116652760546,
4.16333634234433E-16));
#100043=CARTESIAN_POINT('Ctrl Pts',(-10.0225374821233,73.8227522002495,
4.16333634234434E-16));
#100044=CARTESIAN_POINT('',(-10.0225374821233,73.8227522002494,12.));
#100045=CARTESIAN_POINT('Ctrl Pts',(-10.0225374821233,73.8227522002495,
-5.55111512312578E-16));
#100046=CARTESIAN_POINT('Ctrl Pts',(-10.0225374821233,73.8227522002495,
4.));
#100047=CARTESIAN_POINT('Ctrl Pts',(-10.0225374821233,73.8227522002495,
8.));
#100048=CARTESIAN_POINT('Ctrl Pts',(-10.0225374821233,73.8227522002495,
12.));
#100049=CARTESIAN_POINT('',(-10.4355099267296,73.4664795929939,12.));
#100050=CARTESIAN_POINT('Ctrl Pts',(-10.0225374821233,73.8227522002495,
12.));
#100051=CARTESIAN_POINT('Ctrl Pts',(-10.1042001607579,73.8116652760546,
12.));
#100052=CARTESIAN_POINT('Ctrl Pts',(-10.1831187000809,73.7800074220654,
12.));
#100053=CARTESIAN_POINT('Ctrl Pts',(-10.2496275073219,73.7314682122214,
12.));
#100054=CARTESIAN_POINT('Ctrl Pts',(-10.3383059169765,73.6667492657628,
12.));
#100055=CARTESIAN_POINT('Ctrl Pts',(-10.4049225807075,73.5720190200068,
12.));
#100056=CARTESIAN_POINT('Ctrl Pts',(-10.4355099267296,73.4664795929939,
12.));
#100057=CARTESIAN_POINT('Ctrl Pts',(-10.4355099267296,73.4664795929939,
12.));
#100058=CARTESIAN_POINT('Ctrl Pts',(-10.4355099267296,73.4664795929939,
8.));
#100059=CARTESIAN_POINT('Ctrl Pts',(-10.4355099267296,73.4664795929939,
4.));
#100060=CARTESIAN_POINT('Ctrl Pts',(-10.4355099267296,73.4664795929939,
-5.55111512312578E-16));
#100061=CARTESIAN_POINT('Origin',(-4.90253386731614E-11,3.71623968689858E-10,
0.));
#100062=CARTESIAN_POINT('Origin',(-4.90253386731614E-11,3.71623968689858E-10,
12.));
#100063=CARTESIAN_POINT('Origin',(-4.90253386731614E-11,3.71623968689858E-10,
0.));
#100064=CARTESIAN_POINT('Ctrl Pts',(-2.94891377268295,74.4416140848738,
0.));
#100065=CARTESIAN_POINT('Ctrl Pts',(-2.94891377268295,74.4416140848738,
4.));
#100066=CARTESIAN_POINT('Ctrl Pts',(-2.94891377268296,74.4416140848738,
8.));
#100067=CARTESIAN_POINT('Ctrl Pts',(-2.94891377268296,74.4416140848738,
12.));
#100068=CARTESIAN_POINT('Ctrl Pts',(-2.83911742169671,74.4459635334396,
0.));
#100069=CARTESIAN_POINT('Ctrl Pts',(-2.83911742169671,74.4459635334396,
4.));
#100070=CARTESIAN_POINT('Ctrl Pts',(-2.83911742169673,74.4459635334396,
8.00000000000001));
#100071=CARTESIAN_POINT('Ctrl Pts',(-2.83911742169673,74.4459635334396,
12.));
#100072=CARTESIAN_POINT('Ctrl Pts',(-2.64498412359367,74.3877786926473,
0.));
#100073=CARTESIAN_POINT('Ctrl Pts',(-2.64498412359367,74.3877786926473,
4.));
#100074=CARTESIAN_POINT('Ctrl Pts',(-2.6449841235937,74.3877786926473,7.99999999999999));
#100075=CARTESIAN_POINT('Ctrl Pts',(-2.6449841235937,74.3877786926473,12.));
#100076=CARTESIAN_POINT('Ctrl Pts',(-2.51668625693817,74.2364344282704,
0.));
#100077=CARTESIAN_POINT('Ctrl Pts',(-2.51668625693817,74.2364344282704,
4.));
#100078=CARTESIAN_POINT('Ctrl Pts',(-2.51668625693821,74.2364344282705,
8.00000000000001));
#100079=CARTESIAN_POINT('Ctrl Pts',(-2.51668625693821,74.2364344282705,
12.));
#100080=CARTESIAN_POINT('Ctrl Pts',(-2.48034921843231,74.1624659714559,
0.));
#100081=CARTESIAN_POINT('Ctrl Pts',(-2.48034921843231,74.1624659714559,
4.));
#100082=CARTESIAN_POINT('Ctrl Pts',(-2.48034921843235,74.1624659714559,
8.));
#100083=CARTESIAN_POINT('Ctrl Pts',(-2.48034921843235,74.1624659714559,
12.));
#100084=CARTESIAN_POINT('',(-2.94891377268295,74.4416140848738,0.));
#100085=CARTESIAN_POINT('',(-2.48034921843244,74.1624659714558,0.));
#100086=CARTESIAN_POINT('Ctrl Pts',(-2.94891377268295,74.4416140848738,
1.38777878078145E-16));
#100087=CARTESIAN_POINT('Ctrl Pts',(-2.83911742169671,74.4459635334396,
1.38777878078145E-16));
#100088=CARTESIAN_POINT('Ctrl Pts',(-2.72818410849497,74.4127150529868,
1.38777878078145E-16));
#100089=CARTESIAN_POINT('Ctrl Pts',(-2.63874807903121,74.3490471689147,
1.38777878078145E-16));
#100090=CARTESIAN_POINT('Ctrl Pts',(-2.57167105693338,74.3012962558605,
1.38777878078145E-16));
#100091=CARTESIAN_POINT('Ctrl Pts',(-2.51668625693817,74.2364344282704,
1.38777878078144E-16));
#100092=CARTESIAN_POINT('Ctrl Pts',(-2.48034921843231,74.1624659714559,
1.38777878078145E-16));
#100093=CARTESIAN_POINT('',(-2.48034921843246,74.1624659714559,12.));
#100094=CARTESIAN_POINT('Ctrl Pts',(-2.48034921843231,74.1624659714559,
0.));
#100095=CARTESIAN_POINT('Ctrl Pts',(-2.48034921843231,74.1624659714559,
4.));
#100096=CARTESIAN_POINT('Ctrl Pts',(-2.48034921843235,74.1624659714559,
8.));
#100097=CARTESIAN_POINT('Ctrl Pts',(-2.48034921843235,74.1624659714559,
12.));
#100098=CARTESIAN_POINT('',(-2.94891377268296,74.4416140848738,12.));
#100099=CARTESIAN_POINT('Ctrl Pts',(-2.48034921843235,74.1624659714559,
12.));
#100100=CARTESIAN_POINT('Ctrl Pts',(-2.51668625693821,74.2364344282705,
12.));
#100101=CARTESIAN_POINT('Ctrl Pts',(-2.57167105693342,74.3012962558605,
12.));
#100102=CARTESIAN_POINT('Ctrl Pts',(-2.63874807903124,74.3490471689147,
12.));
#100103=CARTESIAN_POINT('Ctrl Pts',(-2.728184108495,74.4127150529868,12.));
#100104=CARTESIAN_POINT('Ctrl Pts',(-2.83911742169673,74.4459635334396,
12.));
#100105=CARTESIAN_POINT('Ctrl Pts',(-2.94891377268296,74.4416140848738,
12.));
#100106=CARTESIAN_POINT('Ctrl Pts',(-2.94891377268296,74.4416140848738,
12.));
#100107=CARTESIAN_POINT('Ctrl Pts',(-2.94891377268296,74.4416140848738,
8.));
#100108=CARTESIAN_POINT('Ctrl Pts',(-2.94891377268295,74.4416140848738,
4.));
#100109=CARTESIAN_POINT('Ctrl Pts',(-2.94891377268295,74.4416140848738,
0.));
#100110=CARTESIAN_POINT('Ctrl Pts',(-0.853825826608985,69.9947925310006,
0.));
#100111=CARTESIAN_POINT('Ctrl Pts',(-0.853825826608985,69.9947925310006,
12.));
#100112=CARTESIAN_POINT('Ctrl Pts',(-0.854867673848596,69.9985337959407,
0.));
#100113=CARTESIAN_POINT('Ctrl Pts',(-0.854867673848596,69.9985337959407,
12.));
#100114=CARTESIAN_POINT('Ctrl Pts',(-0.856954870259207,70.0060209754087,
0.));
#100115=CARTESIAN_POINT('Ctrl Pts',(-0.856954870259207,70.0060209754087,
12.));
#100116=CARTESIAN_POINT('Ctrl Pts',(-0.860096170668736,70.0172656933806,
0.));
#100117=CARTESIAN_POINT('Ctrl Pts',(-0.860096170668736,70.0172656933806,
12.));
#100118=CARTESIAN_POINT('Ctrl Pts',(-0.864305583661547,70.0322865492925,
0.));
#100119=CARTESIAN_POINT('Ctrl Pts',(-0.864305583661547,70.0322865492925,
12.));
#100120=CARTESIAN_POINT('Ctrl Pts',(-0.869602377871126,70.051109108301,
0.));
#100121=CARTESIAN_POINT('Ctrl Pts',(-0.869602377871126,70.051109108301,
12.));
#100122=CARTESIAN_POINT('Ctrl Pts',(-0.874934213255839,70.0699781183935,
0.));
#100123=CARTESIAN_POINT('Ctrl Pts',(-0.874934213255839,70.0699781183935,
12.));
#100124=CARTESIAN_POINT('Ctrl Pts',(-0.880301109660729,70.0888934967855,
0.));
#100125=CARTESIAN_POINT('Ctrl Pts',(-0.880301109660729,70.0888934967855,
12.));
#100126=CARTESIAN_POINT('Ctrl Pts',(-0.885703094802537,70.1078550938958,
0.));
#100127=CARTESIAN_POINT('Ctrl Pts',(-0.885703094802537,70.1078550938958,
12.));
#100128=CARTESIAN_POINT('Ctrl Pts',(-0.891140203464243,70.1268626950175,
0.));
#100129=CARTESIAN_POINT('Ctrl Pts',(-0.891140203464243,70.1268626950175,
12.));
#100130=CARTESIAN_POINT('Ctrl Pts',(-0.896612474371846,70.1459160490446,
0.));
#100131=CARTESIAN_POINT('Ctrl Pts',(-0.896612474371846,70.1459160490446,
12.));
#100132=CARTESIAN_POINT('Ctrl Pts',(-0.902119947629773,70.1650148905109,
0.));
#100133=CARTESIAN_POINT('Ctrl Pts',(-0.902119947629773,70.1650148905109,
12.));
#100134=CARTESIAN_POINT('Ctrl Pts',(-0.907662662015787,70.1841589635574,
0.));
#100135=CARTESIAN_POINT('Ctrl Pts',(-0.907662662015787,70.1841589635574,
12.));
#100136=CARTESIAN_POINT('Ctrl Pts',(-0.913240652090982,70.2033480471676,
0.));
#100137=CARTESIAN_POINT('Ctrl Pts',(-0.913240652090982,70.2033480471676,
12.));
#100138=CARTESIAN_POINT('Ctrl Pts',(-0.91885394915712,70.2225819470248,
0.));
#100139=CARTESIAN_POINT('Ctrl Pts',(-0.91885394915712,70.2225819470248,
12.));
#100140=CARTESIAN_POINT('Ctrl Pts',(-0.924502582639457,70.2418604835837,
0.));
#100141=CARTESIAN_POINT('Ctrl Pts',(-0.924502582639457,70.2418604835837,
12.));
#100142=CARTESIAN_POINT('Ctrl Pts',(-0.930186581235549,70.2611834821724,
0.));
#100143=CARTESIAN_POINT('Ctrl Pts',(-0.930186581235549,70.2611834821724,
12.));
#100144=CARTESIAN_POINT('Ctrl Pts',(-0.935905974336482,70.2805507606872,
0.));
#100145=CARTESIAN_POINT('Ctrl Pts',(-0.935905974336482,70.2805507606872,
12.));
#100146=CARTESIAN_POINT('Ctrl Pts',(-0.941660792742981,70.299962123399,
0.));
#100147=CARTESIAN_POINT('Ctrl Pts',(-0.941660792742981,70.299962123399,
12.));
#100148=CARTESIAN_POINT('Ctrl Pts',(-0.947451067929606,70.3194173673674,
0.));
#100149=CARTESIAN_POINT('Ctrl Pts',(-0.947451067929606,70.3194173673674,
12.));
#100150=CARTESIAN_POINT('Ctrl Pts',(-0.953276831581243,70.338916286458,
0.));
#100151=CARTESIAN_POINT('Ctrl Pts',(-0.953276831581243,70.338916286458,
12.));
#100152=CARTESIAN_POINT('Ctrl Pts',(-0.959138115058833,70.3584586759536,
0.));
#100153=CARTESIAN_POINT('Ctrl Pts',(-0.959138115058833,70.3584586759536,
12.));
#100154=CARTESIAN_POINT('Ctrl Pts',(-0.965034948786451,70.3780443377956,
0.));
#100155=CARTESIAN_POINT('Ctrl Pts',(-0.965034948786451,70.3780443377956,
12.));
#100156=CARTESIAN_POINT('Ctrl Pts',(-0.970967362281175,70.3976730803614,
0.));
#100157=CARTESIAN_POINT('Ctrl Pts',(-0.970967362281175,70.3976730803614,
12.));
#100158=CARTESIAN_POINT('Ctrl Pts',(-0.976935384450043,70.417344715957,
0.));
#100159=CARTESIAN_POINT('Ctrl Pts',(-0.976935384450043,70.417344715957,
12.));
#100160=CARTESIAN_POINT('Ctrl Pts',(-0.982939043792157,70.4370590590842,
0.));
#100161=CARTESIAN_POINT('Ctrl Pts',(-0.982939043792157,70.4370590590842,
12.));
#100162=CARTESIAN_POINT('Ctrl Pts',(-0.98897836864365,70.4568159243163,
0.));
#100163=CARTESIAN_POINT('Ctrl Pts',(-0.98897836864365,70.4568159243163,
12.));
#100164=CARTESIAN_POINT('Ctrl Pts',(-0.995053387379757,70.4766151245212,
0.));
#100165=CARTESIAN_POINT('Ctrl Pts',(-0.995053387379757,70.4766151245212,
12.));
#100166=CARTESIAN_POINT('Ctrl Pts',(-1.00116412831442,70.4964564717953,
0.));
#100167=CARTESIAN_POINT('Ctrl Pts',(-1.00116412831442,70.4964564717953,
12.));
#100168=CARTESIAN_POINT('Ctrl Pts',(-1.00731061960968,70.5163397782713,
0.));
#100169=CARTESIAN_POINT('Ctrl Pts',(-1.00731061960968,70.5163397782713,
12.));
#100170=CARTESIAN_POINT('Ctrl Pts',(-1.01349288918537,70.5362648569061,
0.));
#100171=CARTESIAN_POINT('Ctrl Pts',(-1.01349288918537,70.5362648569061,
12.));
#100172=CARTESIAN_POINT('Ctrl Pts',(-1.01971096460597,70.556231522419,0.));
#100173=CARTESIAN_POINT('Ctrl Pts',(-1.01971096460597,70.556231522419,12.));
#100174=CARTESIAN_POINT('Ctrl Pts',(-1.02596487304049,70.5762395916377,
0.));
#100175=CARTESIAN_POINT('Ctrl Pts',(-1.02596487304049,70.5762395916377,
12.));
#100176=CARTESIAN_POINT('Ctrl Pts',(-1.0322546413287,70.5962888829934,0.));
#100177=CARTESIAN_POINT('Ctrl Pts',(-1.0322546413287,70.5962888829934,12.));
#100178=CARTESIAN_POINT('Ctrl Pts',(-1.03858029601904,70.6163792162073,
0.));
#100179=CARTESIAN_POINT('Ctrl Pts',(-1.03858029601904,70.6163792162073,
12.));
#100180=CARTESIAN_POINT('Ctrl Pts',(-1.04494186341156,70.6365104119252,
0.));
#100181=CARTESIAN_POINT('Ctrl Pts',(-1.04494186341156,70.6365104119252,
12.));
#100182=CARTESIAN_POINT('Ctrl Pts',(-1.05133936960072,70.6566822912991,
0.));
#100183=CARTESIAN_POINT('Ctrl Pts',(-1.05133936960072,70.6566822912991,
12.));
#100184=CARTESIAN_POINT('Ctrl Pts',(-1.0577728404773,70.676894676009,0.));
#100185=CARTESIAN_POINT('Ctrl Pts',(-1.0577728404773,70.676894676009,12.));
#100186=CARTESIAN_POINT('Ctrl Pts',(-1.06424230171281,70.6971473884459,
0.));
#100187=CARTESIAN_POINT('Ctrl Pts',(-1.06424230171281,70.6971473884459,
12.));
#100188=CARTESIAN_POINT('Ctrl Pts',(-1.07074777874596,70.7174402518378,
0.));
#100189=CARTESIAN_POINT('Ctrl Pts',(-1.07074777874596,70.7174402518378,
12.));
#100190=CARTESIAN_POINT('Ctrl Pts',(-1.07728929676408,70.7377730903953,
0.));
#100191=CARTESIAN_POINT('Ctrl Pts',(-1.07728929676408,70.7377730903953,
12.));
#100192=CARTESIAN_POINT('Ctrl Pts',(-1.08386688068342,70.7581457294447,
0.));
#100193=CARTESIAN_POINT('Ctrl Pts',(-1.08386688068342,70.7581457294447,
12.));
#100194=CARTESIAN_POINT('Ctrl Pts',(-1.09048055516427,70.7785579953583,
0.));
#100195=CARTESIAN_POINT('Ctrl Pts',(-1.09048055516427,70.7785579953583,
12.));
#100196=CARTESIAN_POINT('Ctrl Pts',(-1.09713034462265,70.799009715484,0.));
#100197=CARTESIAN_POINT('Ctrl Pts',(-1.09713034462265,70.799009715484,12.));
#100198=CARTESIAN_POINT('Ctrl Pts',(-1.10381627323947,70.8195007180745,
0.));
#100199=CARTESIAN_POINT('Ctrl Pts',(-1.10381627323947,70.8195007180745,
12.));
#100200=CARTESIAN_POINT('Ctrl Pts',(-1.1105383649664,70.8400308322037,0.));
#100201=CARTESIAN_POINT('Ctrl Pts',(-1.1105383649664,70.8400308322037,12.));
#100202=CARTESIAN_POINT('Ctrl Pts',(-1.11729664352993,70.8605998877149,
0.));
#100203=CARTESIAN_POINT('Ctrl Pts',(-1.11729664352993,70.8605998877149,
12.));
#100204=CARTESIAN_POINT('Ctrl Pts',(-1.12409113243514,70.8812077152586,
0.));
#100205=CARTESIAN_POINT('Ctrl Pts',(-1.12409113243514,70.8812077152586,
12.));
#100206=CARTESIAN_POINT('Ctrl Pts',(-1.13092185496565,70.9018541463089,
0.));
#100207=CARTESIAN_POINT('Ctrl Pts',(-1.13092185496565,70.9018541463089,
12.));
#100208=CARTESIAN_POINT('Ctrl Pts',(-1.13778883418214,70.9225390131826,
0.));
#100209=CARTESIAN_POINT('Ctrl Pts',(-1.13778883418214,70.9225390131826,
12.));
#100210=CARTESIAN_POINT('Ctrl Pts',(-1.14469209291489,70.9432621490566,
0.));
#100211=CARTESIAN_POINT('Ctrl Pts',(-1.14469209291489,70.9432621490566,
12.));
#100212=CARTESIAN_POINT('Ctrl Pts',(-1.15163165376524,70.9640233879659,
0.));
#100213=CARTESIAN_POINT('Ctrl Pts',(-1.15163165376524,70.9640233879659,
12.));
#100214=CARTESIAN_POINT('Ctrl Pts',(-1.15860753911485,70.9848225647871,
0.));
#100215=CARTESIAN_POINT('Ctrl Pts',(-1.15860753911485,70.9848225647871,
12.));
#100216=CARTESIAN_POINT('Ctrl Pts',(-1.1656197711288,71.0056595152204,0.));
#100217=CARTESIAN_POINT('Ctrl Pts',(-1.1656197711288,71.0056595152204,12.));
#100218=CARTESIAN_POINT('Ctrl Pts',(-1.17266837175777,71.0265340757699,
0.));
#100219=CARTESIAN_POINT('Ctrl Pts',(-1.17266837175777,71.0265340757699,
12.));
#100220=CARTESIAN_POINT('Ctrl Pts',(-1.17975336273504,71.0474460837159,
0.));
#100221=CARTESIAN_POINT('Ctrl Pts',(-1.17975336273504,71.0474460837159,
12.));
#100222=CARTESIAN_POINT('Ctrl Pts',(-1.18687476558133,71.0683953771149,
0.));
#100223=CARTESIAN_POINT('Ctrl Pts',(-1.18687476558133,71.0683953771149,
12.));
#100224=CARTESIAN_POINT('Ctrl Pts',(-1.19403260161002,71.089381794801,0.));
#100225=CARTESIAN_POINT('Ctrl Pts',(-1.19403260161002,71.089381794801,12.));
#100226=CARTESIAN_POINT('Ctrl Pts',(-1.20122689192836,71.1104051763839,
0.));
#100227=CARTESIAN_POINT('Ctrl Pts',(-1.20122689192836,71.1104051763839,
12.));
#100228=CARTESIAN_POINT('Ctrl Pts',(-1.20845765743648,71.1314653622442,
0.));
#100229=CARTESIAN_POINT('Ctrl Pts',(-1.20845765743648,71.1314653622442,
12.));
#100230=CARTESIAN_POINT('Ctrl Pts',(-1.21572491882263,71.1525621935267,
0.));
#100231=CARTESIAN_POINT('Ctrl Pts',(-1.21572491882263,71.1525621935267,
12.));
#100232=CARTESIAN_POINT('Ctrl Pts',(-1.22302869657018,71.1736955121362,
0.));
#100233=CARTESIAN_POINT('Ctrl Pts',(-1.22302869657018,71.1736955121362,
12.));
#100234=CARTESIAN_POINT('Ctrl Pts',(-1.23036901096239,71.194865160732,0.));
#100235=CARTESIAN_POINT('Ctrl Pts',(-1.23036901096239,71.194865160732,12.));
#100236=CARTESIAN_POINT('Ctrl Pts',(-1.23774588208427,71.2160709827191,
0.));
#100237=CARTESIAN_POINT('Ctrl Pts',(-1.23774588208427,71.2160709827191,
12.));
#100238=CARTESIAN_POINT('Ctrl Pts',(-1.24515932982113,71.2373128222352,
0.));
#100239=CARTESIAN_POINT('Ctrl Pts',(-1.24515932982113,71.2373128222352,
12.));
#100240=CARTESIAN_POINT('Ctrl Pts',(-1.25260937385569,71.2585905241406,
0.));
#100241=CARTESIAN_POINT('Ctrl Pts',(-1.25260937385569,71.2585905241406,
12.));
#100242=CARTESIAN_POINT('Ctrl Pts',(-1.26009603367571,71.2799039340175,
0.));
#100243=CARTESIAN_POINT('Ctrl Pts',(-1.26009603367571,71.2799039340175,
12.));
#100244=CARTESIAN_POINT('Ctrl Pts',(-1.26761932857724,71.3012528981661,
0.));
#100245=CARTESIAN_POINT('Ctrl Pts',(-1.26761932857724,71.3012528981661,
12.));
#100246=CARTESIAN_POINT('Ctrl Pts',(-1.27517927766608,71.3226372635996,
0.));
#100247=CARTESIAN_POINT('Ctrl Pts',(-1.27517927766608,71.3226372635996,
12.));
#100248=CARTESIAN_POINT('Ctrl Pts',(-1.28277589985472,71.3440568780347,
0.));
#100249=CARTESIAN_POINT('Ctrl Pts',(-1.28277589985472,71.3440568780347,
12.));
#100250=CARTESIAN_POINT('Ctrl Pts',(-1.29040921386059,71.3655115898827,
0.));
#100251=CARTESIAN_POINT('Ctrl Pts',(-1.29040921386059,71.3655115898827,
12.));
#100252=CARTESIAN_POINT('Ctrl Pts',(-1.29807923821414,71.3870012482499,
0.));
#100253=CARTESIAN_POINT('Ctrl Pts',(-1.29807923821414,71.3870012482499,
12.));
#100254=CARTESIAN_POINT('Ctrl Pts',(-1.3057859912614,71.4085257029322,0.));
#100255=CARTESIAN_POINT('Ctrl Pts',(-1.3057859912614,71.4085257029322,12.));
#100256=CARTESIAN_POINT('Ctrl Pts',(-1.31352949116537,71.4300848044087,
0.));
#100257=CARTESIAN_POINT('Ctrl Pts',(-1.31352949116537,71.4300848044087,
12.));
#100258=CARTESIAN_POINT('Ctrl Pts',(-1.32130975590226,71.4516784038317,
0.));
#100259=CARTESIAN_POINT('Ctrl Pts',(-1.32130975590226,71.4516784038317,
12.));
#100260=CARTESIAN_POINT('Ctrl Pts',(-1.32912680326124,71.4733063530187,
0.));
#100261=CARTESIAN_POINT('Ctrl Pts',(-1.32912680326124,71.4733063530187,
12.));
#100262=CARTESIAN_POINT('Ctrl Pts',(-1.3369806508522,71.4949685044522,0.));
#100263=CARTESIAN_POINT('Ctrl Pts',(-1.3369806508522,71.4949685044522,12.));
#100264=CARTESIAN_POINT('Ctrl Pts',(-1.34487131610781,71.516664711275,0.));
#100265=CARTESIAN_POINT('Ctrl Pts',(-1.34487131610781,71.516664711275,12.));
#100266=CARTESIAN_POINT('Ctrl Pts',(-1.35279881628455,71.5383948272845,
0.));
#100267=CARTESIAN_POINT('Ctrl Pts',(-1.35279881628455,71.5383948272845,
12.));
#100268=CARTESIAN_POINT('Ctrl Pts',(-1.36076316845816,71.5601587069217,
0.));
#100269=CARTESIAN_POINT('Ctrl Pts',(-1.36076316845816,71.5601587069217,
12.));
#100270=CARTESIAN_POINT('Ctrl Pts',(-1.36876438952466,71.5819562052663,
0.));
#100271=CARTESIAN_POINT('Ctrl Pts',(-1.36876438952466,71.5819562052663,
12.));
#100272=CARTESIAN_POINT('Ctrl Pts',(-1.3768024962078,71.6037871780385,0.));
#100273=CARTESIAN_POINT('Ctrl Pts',(-1.3768024962078,71.6037871780385,12.));
#100274=CARTESIAN_POINT('Ctrl Pts',(-1.38487750506082,71.625651481593,0.));
#100275=CARTESIAN_POINT('Ctrl Pts',(-1.38487750506082,71.625651481593,12.));
#100276=CARTESIAN_POINT('Ctrl Pts',(-1.39298943246722,71.6475489729134,
0.));
#100277=CARTESIAN_POINT('Ctrl Pts',(-1.39298943246722,71.6475489729134,
12.));
#100278=CARTESIAN_POINT('Ctrl Pts',(-1.40113829463577,71.6694795096001,
0.));
#100279=CARTESIAN_POINT('Ctrl Pts',(-1.40113829463577,71.6694795096001,
12.));
#100280=CARTESIAN_POINT('Ctrl Pts',(-1.40932410760248,71.6914429498663,
0.));
#100281=CARTESIAN_POINT('Ctrl Pts',(-1.40932410760248,71.6914429498663,
12.));
#100282=CARTESIAN_POINT('Ctrl Pts',(-1.41754688723773,71.7134391525389,
0.));
#100283=CARTESIAN_POINT('Ctrl Pts',(-1.41754688723773,71.7134391525389,
12.));
#100284=CARTESIAN_POINT('Ctrl Pts',(-1.4258066492477,71.7354679770528,0.));
#100285=CARTESIAN_POINT('Ctrl Pts',(-1.4258066492477,71.7354679770528,12.));
#100286=CARTESIAN_POINT('Ctrl Pts',(-1.43410340917496,71.7575292834469,
0.));
#100287=CARTESIAN_POINT('Ctrl Pts',(-1.43410340917496,71.7575292834469,
12.));
#100288=CARTESIAN_POINT('Ctrl Pts',(-1.44243718239315,71.7796229323526,
0.));
#100289=CARTESIAN_POINT('Ctrl Pts',(-1.44243718239315,71.7796229323526,
12.));
#100290=CARTESIAN_POINT('Ctrl Pts',(-1.45080798410965,71.8017487849895,
0.));
#100291=CARTESIAN_POINT('Ctrl Pts',(-1.45080798410965,71.8017487849895,
12.));
#100292=CARTESIAN_POINT('Ctrl Pts',(-1.45921582937232,71.8239067031683,
0.));
#100293=CARTESIAN_POINT('Ctrl Pts',(-1.45921582937232,71.8239067031683,
12.));
#100294=CARTESIAN_POINT('Ctrl Pts',(-1.46766073307088,71.8460965492839,
0.));
#100295=CARTESIAN_POINT('Ctrl Pts',(-1.46766073307088,71.8460965492839,
12.));
#100296=CARTESIAN_POINT('Ctrl Pts',(-1.47614270993729,71.8683181863116,
0.));
#100297=CARTESIAN_POINT('Ctrl Pts',(-1.47614270993729,71.8683181863116,
12.));
#100298=CARTESIAN_POINT('Ctrl Pts',(-1.4846617745402,71.8905714777961,0.));
#100299=CARTESIAN_POINT('Ctrl Pts',(-1.4846617745402,71.8905714777961,12.));
#100300=CARTESIAN_POINT('Ctrl Pts',(-1.49321794128799,71.912856287848,0.));
#100301=CARTESIAN_POINT('Ctrl Pts',(-1.49321794128799,71.912856287848,12.));
#100302=CARTESIAN_POINT('Ctrl Pts',(-1.50181122443534,71.9351724811443,
0.));
#100303=CARTESIAN_POINT('Ctrl Pts',(-1.50181122443534,71.9351724811443,
12.));
#100304=CARTESIAN_POINT('Ctrl Pts',(-1.51044163808454,71.9575199229241,
0.));
#100305=CARTESIAN_POINT('Ctrl Pts',(-1.51044163808454,71.9575199229241,
12.));
#100306=CARTESIAN_POINT('Ctrl Pts',(-1.51910919618566,71.979898478983,0.));
#100307=CARTESIAN_POINT('Ctrl Pts',(-1.51910919618566,71.979898478983,12.));
#100308=CARTESIAN_POINT('Ctrl Pts',(-1.52781391253102,72.0023080156647,
0.));
#100309=CARTESIAN_POINT('Ctrl Pts',(-1.52781391253102,72.0023080156647,
12.));
#100310=CARTESIAN_POINT('Ctrl Pts',(-1.53655580075813,72.0247483998578,
0.));
#100311=CARTESIAN_POINT('Ctrl Pts',(-1.53655580075813,72.0247483998578,
12.));
#100312=CARTESIAN_POINT('Ctrl Pts',(-1.54533487435626,72.0472194989963,
0.));
#100313=CARTESIAN_POINT('Ctrl Pts',(-1.54533487435626,72.0472194989963,
12.));
#100314=CARTESIAN_POINT('Ctrl Pts',(-1.55415114666774,72.0697211810545,
0.));
#100315=CARTESIAN_POINT('Ctrl Pts',(-1.55415114666774,72.0697211810545,
12.));
#100316=CARTESIAN_POINT('Ctrl Pts',(-1.56300463088809,72.0922533145433,
0.));
#100317=CARTESIAN_POINT('Ctrl Pts',(-1.56300463088809,72.0922533145433,
12.));
#100318=CARTESIAN_POINT('Ctrl Pts',(-1.5718953400604,72.1148157684995,0.));
#100319=CARTESIAN_POINT('Ctrl Pts',(-1.5718953400604,72.1148157684995,12.));
#100320=CARTESIAN_POINT('Ctrl Pts',(-1.58082328707803,72.1374084124839,
0.));
#100321=CARTESIAN_POINT('Ctrl Pts',(-1.58082328707803,72.1374084124839,
12.));
#100322=CARTESIAN_POINT('Ctrl Pts',(-1.58978848469123,72.1600311165821,
0.));
#100323=CARTESIAN_POINT('Ctrl Pts',(-1.58978848469123,72.1600311165821,
12.));
#100324=CARTESIAN_POINT('Ctrl Pts',(-1.59879094550847,72.1826837514001,
0.));
#100325=CARTESIAN_POINT('Ctrl Pts',(-1.59879094550847,72.1826837514001,
12.));
#100326=CARTESIAN_POINT('Ctrl Pts',(-1.60783068199663,72.2053661880608,
0.));
#100327=CARTESIAN_POINT('Ctrl Pts',(-1.60783068199663,72.2053661880608,
12.));
#100328=CARTESIAN_POINT('Ctrl Pts',(-1.6169077064754,72.2280782981937,0.));
#100329=CARTESIAN_POINT('Ctrl Pts',(-1.6169077064754,72.2280782981937,12.));
#100330=CARTESIAN_POINT('Ctrl Pts',(-1.6260220311193,72.2508199539323,0.));
#100331=CARTESIAN_POINT('Ctrl Pts',(-1.6260220311193,72.2508199539323,12.));
#100332=CARTESIAN_POINT('Ctrl Pts',(-1.63517366796463,72.2735910279149,
0.));
#100333=CARTESIAN_POINT('Ctrl Pts',(-1.63517366796463,72.2735910279149,
12.));
#100334=CARTESIAN_POINT('Ctrl Pts',(-1.64436262891079,72.2963913932813,
0.));
#100335=CARTESIAN_POINT('Ctrl Pts',(-1.64436262891079,72.2963913932813,
12.));
#100336=CARTESIAN_POINT('Ctrl Pts',(-1.65358892572063,72.319220923669,0.));
#100337=CARTESIAN_POINT('Ctrl Pts',(-1.65358892572063,72.319220923669,12.));
#100338=CARTESIAN_POINT('Ctrl Pts',(-1.66285257001496,72.3420794932047,
0.));
#100339=CARTESIAN_POINT('Ctrl Pts',(-1.66285257001496,72.3420794932047,
12.));
#100340=CARTESIAN_POINT('Ctrl Pts',(-1.67215357327365,72.3649669765004,
0.));
#100341=CARTESIAN_POINT('Ctrl Pts',(-1.67215357327365,72.3649669765004,
12.));
#100342=CARTESIAN_POINT('Ctrl Pts',(-1.68149194684282,72.387883248654,0.));
#100343=CARTESIAN_POINT('Ctrl Pts',(-1.68149194684282,72.387883248654,12.));
#100344=CARTESIAN_POINT('Ctrl Pts',(-1.69086770193637,72.4108281852467,
0.));
#100345=CARTESIAN_POINT('Ctrl Pts',(-1.69086770193637,72.4108281852467,
12.));
#100346=CARTESIAN_POINT('Ctrl Pts',(-1.70028084963647,72.4338016623391,
0.));
#100347=CARTESIAN_POINT('Ctrl Pts',(-1.70028084963647,72.4338016623391,
12.));
#100348=CARTESIAN_POINT('Ctrl Pts',(-1.70973140088842,72.456803556463,0.));
#100349=CARTESIAN_POINT('Ctrl Pts',(-1.70973140088842,72.456803556463,12.));
#100350=CARTESIAN_POINT('Ctrl Pts',(-1.71921936650038,72.479833744618,0.));
#100351=CARTESIAN_POINT('Ctrl Pts',(-1.71921936650038,72.479833744618,12.));
#100352=CARTESIAN_POINT('Ctrl Pts',(-1.72874475715103,72.5028921042721,
0.));
#100353=CARTESIAN_POINT('Ctrl Pts',(-1.72874475715103,72.5028921042721,
12.));
#100354=CARTESIAN_POINT('Ctrl Pts',(-1.73830758339125,72.5259785133595,
0.));
#100355=CARTESIAN_POINT('Ctrl Pts',(-1.73830758339125,72.5259785133595,
12.));
#100356=CARTESIAN_POINT('Ctrl Pts',(-1.74790785564474,72.5490928502769,
0.));
#100357=CARTESIAN_POINT('Ctrl Pts',(-1.74790785564474,72.5490928502769,
12.));
#100358=CARTESIAN_POINT('Ctrl Pts',(-1.75754558420344,72.5722349938774,
0.));
#100359=CARTESIAN_POINT('Ctrl Pts',(-1.75754558420344,72.5722349938774,
12.));
#100360=CARTESIAN_POINT('Ctrl Pts',(-1.76722077922574,72.5954048234638,
0.));
#100361=CARTESIAN_POINT('Ctrl Pts',(-1.76722077922574,72.5954048234638,
12.));
#100362=CARTESIAN_POINT('Ctrl Pts',(-1.77693345074427,72.6186022187907,
0.));
#100363=CARTESIAN_POINT('Ctrl Pts',(-1.77693345074427,72.6186022187907,
12.));
#100364=CARTESIAN_POINT('Ctrl Pts',(-1.78668360866811,72.6418270600619,
0.));
#100365=CARTESIAN_POINT('Ctrl Pts',(-1.78668360866811,72.6418270600619,
12.));
#100366=CARTESIAN_POINT('Ctrl Pts',(-1.79647126278359,72.6650792279274,
0.));
#100367=CARTESIAN_POINT('Ctrl Pts',(-1.79647126278359,72.6650792279274,
12.));
#100368=CARTESIAN_POINT('Ctrl Pts',(-1.80629642275051,72.6883586034769,
0.));
#100369=CARTESIAN_POINT('Ctrl Pts',(-1.80629642275051,72.6883586034769,
12.));
#100370=CARTESIAN_POINT('Ctrl Pts',(-1.81615909809871,72.7116650682344,
0.));
#100371=CARTESIAN_POINT('Ctrl Pts',(-1.81615909809871,72.7116650682344,
12.));
#100372=CARTESIAN_POINT('Ctrl Pts',(-1.82605929823564,72.7349985041592,
0.));
#100373=CARTESIAN_POINT('Ctrl Pts',(-1.82605929823564,72.7349985041592,
12.));
#100374=CARTESIAN_POINT('Ctrl Pts',(-1.83599703244924,72.7583587936447,
0.));
#100375=CARTESIAN_POINT('Ctrl Pts',(-1.83599703244924,72.7583587936447,
12.));
#100376=CARTESIAN_POINT('Ctrl Pts',(-1.84597230990857,72.7817458195155,
0.));
#100377=CARTESIAN_POINT('Ctrl Pts',(-1.84597230990857,72.7817458195155,
12.));
#100378=CARTESIAN_POINT('Ctrl Pts',(-1.85598513966114,72.8051594650222,
0.));
#100379=CARTESIAN_POINT('Ctrl Pts',(-1.85598513966114,72.8051594650222,
12.));
#100380=CARTESIAN_POINT('Ctrl Pts',(-1.86603553062771,72.8285996138359,
0.));
#100381=CARTESIAN_POINT('Ctrl Pts',(-1.86603553062771,72.8285996138359,
12.));
#100382=CARTESIAN_POINT('Ctrl Pts',(-1.87612349160945,72.8520661500477,
0.));
#100383=CARTESIAN_POINT('Ctrl Pts',(-1.87612349160945,72.8520661500477,
12.));
#100384=CARTESIAN_POINT('Ctrl Pts',(-1.88624903129188,72.875558958168,0.));
#100385=CARTESIAN_POINT('Ctrl Pts',(-1.88624903129188,72.875558958168,12.));
#100386=CARTESIAN_POINT('Ctrl Pts',(-1.89641215824582,72.8990779231226,
0.));
#100387=CARTESIAN_POINT('Ctrl Pts',(-1.89641215824582,72.8990779231226,
12.));
#100388=CARTESIAN_POINT('Ctrl Pts',(-1.90661288092587,72.9226229302478,
0.));
#100389=CARTESIAN_POINT('Ctrl Pts',(-1.90661288092587,72.9226229302478,
12.));
#100390=CARTESIAN_POINT('Ctrl Pts',(-1.91685120766437,72.9461938652811,
0.));
#100391=CARTESIAN_POINT('Ctrl Pts',(-1.91685120766437,72.9461938652811,
12.));
#100392=CARTESIAN_POINT('Ctrl Pts',(-1.9271271466766,72.9697906143636,0.));
#100393=CARTESIAN_POINT('Ctrl Pts',(-1.9271271466766,72.9697906143636,12.));
#100394=CARTESIAN_POINT('Ctrl Pts',(-1.93744070606566,72.9934130640415,
0.));
#100395=CARTESIAN_POINT('Ctrl Pts',(-1.93744070606566,72.9934130640415,
12.));
#100396=CARTESIAN_POINT('Ctrl Pts',(-1.94779189382302,73.0170611012661,
0.));
#100397=CARTESIAN_POINT('Ctrl Pts',(-1.94779189382302,73.0170611012661,
12.));
#100398=CARTESIAN_POINT('Ctrl Pts',(-1.95818071782767,73.040734613391,0.));
#100399=CARTESIAN_POINT('Ctrl Pts',(-1.95818071782767,73.040734613391,12.));
#100400=CARTESIAN_POINT('Ctrl Pts',(-1.96860718583932,73.0644334881673,
0.));
#100401=CARTESIAN_POINT('Ctrl Pts',(-1.96860718583932,73.0644334881673,
12.));
#100402=CARTESIAN_POINT('Ctrl Pts',(-1.97907130550158,73.0881576137407,
0.));
#100403=CARTESIAN_POINT('Ctrl Pts',(-1.97907130550158,73.0881576137407,
12.));
#100404=CARTESIAN_POINT('Ctrl Pts',(-1.98957308434918,73.1119068786475,
0.));
#100405=CARTESIAN_POINT('Ctrl Pts',(-1.98957308434918,73.1119068786475,
12.));
#100406=CARTESIAN_POINT('Ctrl Pts',(-2.00011252980982,73.1356811718091,
0.));
#100407=CARTESIAN_POINT('Ctrl Pts',(-2.00011252980982,73.1356811718091,
12.));
#100408=CARTESIAN_POINT('Ctrl Pts',(-2.01068964920467,73.1594803825252,
0.));
#100409=CARTESIAN_POINT('Ctrl Pts',(-2.01068964920467,73.1594803825252,
12.));
#100410=CARTESIAN_POINT('Ctrl Pts',(-2.02130444974362,73.183304400462,0.));
#100411=CARTESIAN_POINT('Ctrl Pts',(-2.02130444974362,73.183304400462,12.));
#100412=CARTESIAN_POINT('Ctrl Pts',(-2.03195693852455,73.2071531156504,
0.));
#100413=CARTESIAN_POINT('Ctrl Pts',(-2.03195693852455,73.2071531156504,
12.));
#100414=CARTESIAN_POINT('Ctrl Pts',(-2.04264712253929,73.2310264184976,
0.));
#100415=CARTESIAN_POINT('Ctrl Pts',(-2.04264712253929,73.2310264184976,
12.));
#100416=CARTESIAN_POINT('Ctrl Pts',(-2.05337500867403,73.2549241997953,
0.));
#100417=CARTESIAN_POINT('Ctrl Pts',(-2.05337500867403,73.2549241997953,
12.));
#100418=CARTESIAN_POINT('Ctrl Pts',(-2.06414060370835,73.2788463507246,
0.));
#100419=CARTESIAN_POINT('Ctrl Pts',(-2.06414060370835,73.2788463507246,
12.));
#100420=CARTESIAN_POINT('Ctrl Pts',(-2.07494391430941,73.3027927628626,
0.));
#100421=CARTESIAN_POINT('Ctrl Pts',(-2.07494391430941,73.3027927628626,
12.));
#100422=CARTESIAN_POINT('Ctrl Pts',(-2.08578494702744,73.3267633281807,
0.));
#100423=CARTESIAN_POINT('Ctrl Pts',(-2.08578494702744,73.3267633281807,
12.));
#100424=CARTESIAN_POINT('Ctrl Pts',(-2.09666370830716,73.3507579390239,
0.));
#100425=CARTESIAN_POINT('Ctrl Pts',(-2.09666370830716,73.3507579390239,
12.));
#100426=CARTESIAN_POINT('Ctrl Pts',(-2.1075802044939,73.3747764880893,0.));
#100427=CARTESIAN_POINT('Ctrl Pts',(-2.1075802044939,73.3747764880893,12.));
#100428=CARTESIAN_POINT('Ctrl Pts',(-2.11853444183762,73.3988188684021,
0.));
#100429=CARTESIAN_POINT('Ctrl Pts',(-2.11853444183762,73.3988188684021,
12.));
#100430=CARTESIAN_POINT('Ctrl Pts',(-2.12952642649368,73.4228849732925,
0.));
#100431=CARTESIAN_POINT('Ctrl Pts',(-2.12952642649368,73.4228849732925,
12.));
#100432=CARTESIAN_POINT('Ctrl Pts',(-2.14055616452058,73.4469746963637,
0.));
#100433=CARTESIAN_POINT('Ctrl Pts',(-2.14055616452058,73.4469746963637,
12.));
#100434=CARTESIAN_POINT('Ctrl Pts',(-2.15162366187907,73.4710879315382,
0.));
#100435=CARTESIAN_POINT('Ctrl Pts',(-2.15162366187907,73.4710879315382,
12.));
#100436=CARTESIAN_POINT('Ctrl Pts',(-2.1627289244292,73.4952245731054,0.));
#100437=CARTESIAN_POINT('Ctrl Pts',(-2.1627289244292,73.4952245731054,12.));
#100438=CARTESIAN_POINT('Ctrl Pts',(-2.17387195792306,73.5193845157708,
0.));
#100439=CARTESIAN_POINT('Ctrl Pts',(-2.17387195792306,73.5193845157708,
12.));
#100440=CARTESIAN_POINT('Ctrl Pts',(-2.18505276799753,73.5435676546929,
0.));
#100441=CARTESIAN_POINT('Ctrl Pts',(-2.18505276799753,73.5435676546929,
12.));
#100442=CARTESIAN_POINT('Ctrl Pts',(-2.19627136015678,73.5677738855452,
0.));
#100443=CARTESIAN_POINT('Ctrl Pts',(-2.19627136015678,73.5677738855452,
12.));
#100444=CARTESIAN_POINT('Ctrl Pts',(-2.20752773978349,73.5920031044595,
0.));
#100445=CARTESIAN_POINT('Ctrl Pts',(-2.20752773978349,73.5920031044595,
12.));
#100446=CARTESIAN_POINT('Ctrl Pts',(-2.21882191216518,73.6162552079038,
0.));
#100447=CARTESIAN_POINT('Ctrl Pts',(-2.21882191216518,73.6162552079038,
12.));
#100448=CARTESIAN_POINT('Ctrl Pts',(-2.23015388251288,73.6405300925712,
0.));
#100449=CARTESIAN_POINT('Ctrl Pts',(-2.23015388251288,73.6405300925712,
12.));
#100450=CARTESIAN_POINT('Ctrl Pts',(-2.24152365597698,73.6648276552767,
0.));
#100451=CARTESIAN_POINT('Ctrl Pts',(-2.24152365597698,73.6648276552767,
12.));
#100452=CARTESIAN_POINT('Ctrl Pts',(-2.25293123766425,73.6891477928129,
0.));
#100453=CARTESIAN_POINT('Ctrl Pts',(-2.25293123766425,73.6891477928129,
12.));
#100454=CARTESIAN_POINT('Ctrl Pts',(-2.26437663263667,73.7134904019389,
0.));
#100455=CARTESIAN_POINT('Ctrl Pts',(-2.26437663263667,73.7134904019389,
12.));
#100456=CARTESIAN_POINT('Ctrl Pts',(-2.27585984587199,73.7378553796807,
0.));
#100457=CARTESIAN_POINT('Ctrl Pts',(-2.27585984587199,73.7378553796807,
12.));
#100458=CARTESIAN_POINT('Ctrl Pts',(-2.28738088222864,73.762242623566,0.));
#100459=CARTESIAN_POINT('Ctrl Pts',(-2.28738088222864,73.762242623566,12.));
#100460=CARTESIAN_POINT('Ctrl Pts',(-2.29893974640434,73.786652031885,0.));
#100461=CARTESIAN_POINT('Ctrl Pts',(-2.29893974640434,73.786652031885,12.));
#100462=CARTESIAN_POINT('Ctrl Pts',(-2.31053644289417,73.8110835039327,
0.));
#100463=CARTESIAN_POINT('Ctrl Pts',(-2.31053644289417,73.8110835039327,
12.));
#100464=CARTESIAN_POINT('Ctrl Pts',(-2.32217097594198,73.8355369402706,
0.));
#100465=CARTESIAN_POINT('Ctrl Pts',(-2.32217097594198,73.8355369402706,
12.));
#100466=CARTESIAN_POINT('Ctrl Pts',(-2.33384334963958,73.8600122421468,
0.));
#100467=CARTESIAN_POINT('Ctrl Pts',(-2.33384334963958,73.8600122421468,
12.));
#100468=CARTESIAN_POINT('Ctrl Pts',(-2.34555356802121,73.8845093109274,
0.));
#100469=CARTESIAN_POINT('Ctrl Pts',(-2.34555356802121,73.8845093109274,
12.));
#100470=CARTESIAN_POINT('Ctrl Pts',(-2.35730163516316,73.9090280474712,
0.));
#100471=CARTESIAN_POINT('Ctrl Pts',(-2.35730163516316,73.9090280474712,
12.));
#100472=CARTESIAN_POINT('Ctrl Pts',(-2.36908755526003,73.9335683516404,
0.));
#100473=CARTESIAN_POINT('Ctrl Pts',(-2.36908755526003,73.9335683516404,
12.));
#100474=CARTESIAN_POINT('Ctrl Pts',(-2.38091133274961,73.958130121465,0.));
#100475=CARTESIAN_POINT('Ctrl Pts',(-2.38091133274961,73.958130121465,12.));
#100476=CARTESIAN_POINT('Ctrl Pts',(-2.39277297220757,73.9827132538206,
0.));
#100477=CARTESIAN_POINT('Ctrl Pts',(-2.39277297220757,73.9827132538206,
12.));
#100478=CARTESIAN_POINT('Ctrl Pts',(-2.40467247811536,74.0073176459344,
0.));
#100479=CARTESIAN_POINT('Ctrl Pts',(-2.40467247811536,74.0073176459344,
12.));
#100480=CARTESIAN_POINT('Ctrl Pts',(-2.41660985465252,74.0319431966989,
0.));
#100481=CARTESIAN_POINT('Ctrl Pts',(-2.41660985465252,74.0319431966989,
12.));
#100482=CARTESIAN_POINT('Ctrl Pts',(-2.42858510549779,74.0565898079218,
0.));
#100483=CARTESIAN_POINT('Ctrl Pts',(-2.42858510549779,74.0565898079218,
12.));
#100484=CARTESIAN_POINT('Ctrl Pts',(-2.44059823356676,74.0812573859411,
0.));
#100485=CARTESIAN_POINT('Ctrl Pts',(-2.44059823356676,74.0812573859411,
12.));
#100486=CARTESIAN_POINT('Ctrl Pts',(-2.45264924094775,74.1059458420067,
0.));
#100487=CARTESIAN_POINT('Ctrl Pts',(-2.45264924094775,74.1059458420067,
12.));
#100488=CARTESIAN_POINT('Ctrl Pts',(-2.4647381294796,74.1306550887071,0.));
#100489=CARTESIAN_POINT('Ctrl Pts',(-2.4647381294796,74.1306550887071,12.));
#100490=CARTESIAN_POINT('Ctrl Pts',(-2.47686490120354,74.155385037148,0.));
#100491=CARTESIAN_POINT('Ctrl Pts',(-2.47686490120354,74.155385037148,12.));
#100492=CARTESIAN_POINT('Ctrl Pts',(-2.48902955888385,74.1801355936907,
0.));
#100493=CARTESIAN_POINT('Ctrl Pts',(-2.48902955888385,74.1801355936907,
12.));
#100494=CARTESIAN_POINT('Ctrl Pts',(-2.50123210644135,74.2049066572031,
0.));
#100495=CARTESIAN_POINT('Ctrl Pts',(-2.50123210644135,74.2049066572031,
12.));
#100496=CARTESIAN_POINT('Ctrl Pts',(-2.51347254956167,74.229698115223,0.));
#100497=CARTESIAN_POINT('Ctrl Pts',(-2.51347254956167,74.229698115223,12.));
#100498=CARTESIAN_POINT('Ctrl Pts',(-2.52575089478304,74.2545098494824,
0.));
#100499=CARTESIAN_POINT('Ctrl Pts',(-2.52575089478304,74.2545098494824,
12.));
#100500=CARTESIAN_POINT('Ctrl Pts',(-2.53806714838286,74.2793417427308,
0.));
#100501=CARTESIAN_POINT('Ctrl Pts',(-2.53806714838286,74.2793417427308,
12.));
#100502=CARTESIAN_POINT('Ctrl Pts',(-2.55042131526781,74.3041936853468,
0.));
#100503=CARTESIAN_POINT('Ctrl Pts',(-2.55042131526781,74.3041936853468,
12.));
#100504=CARTESIAN_POINT('Ctrl Pts',(-2.56281339800018,74.3290655814831,
0.));
#100505=CARTESIAN_POINT('Ctrl Pts',(-2.56281339800018,74.3290655814831,
12.));
#100506=CARTESIAN_POINT('Ctrl Pts',(-2.5752433954139,74.3539573567672,0.));
#100507=CARTESIAN_POINT('Ctrl Pts',(-2.5752433954139,74.3539573567672,12.));
#100508=CARTESIAN_POINT('Ctrl Pts',(-2.58771130268176,74.3788689603363,
0.));
#100509=CARTESIAN_POINT('Ctrl Pts',(-2.58771130268176,74.3788689603363,
12.));
#100510=CARTESIAN_POINT('Ctrl Pts',(-2.60021711326977,74.4038003594771,
0.));
#100511=CARTESIAN_POINT('Ctrl Pts',(-2.60021711326977,74.4038003594771,
12.));
#100512=CARTESIAN_POINT('Ctrl Pts',(-2.61025207898403,74.4237613007988,
0.));
#100513=CARTESIAN_POINT('Ctrl Pts',(-2.61025207898403,74.4237613007988,
12.));
#100514=CARTESIAN_POINT('Ctrl Pts',(-2.61779535432112,74.4387409032207,
0.));
#100515=CARTESIAN_POINT('Ctrl Pts',(-2.61779535432112,74.4387409032207,
12.));
#100516=CARTESIAN_POINT('Ctrl Pts',(-2.62283178248203,74.4487312586464,
0.));
#100517=CARTESIAN_POINT('Ctrl Pts',(-2.62283178248203,74.4487312586464,
12.));
#100518=CARTESIAN_POINT('Ctrl Pts',(-2.62535189104655,74.4537274248118,
0.));
#100519=CARTESIAN_POINT('Ctrl Pts',(-2.62535189104655,74.4537274248118,
12.));
#100520=CARTESIAN_POINT('',(-0.853825826608985,69.9947925310006,0.));
#100521=CARTESIAN_POINT('Ctrl Pts',(-0.853825826608985,69.9947925310006,
0.));
#100522=CARTESIAN_POINT('Ctrl Pts',(-0.854867673848596,69.9985337959407,
0.));
#100523=CARTESIAN_POINT('Ctrl Pts',(-0.856954870259207,70.0060209754087,
0.));
#100524=CARTESIAN_POINT('Ctrl Pts',(-0.860096170668736,70.0172656933806,
0.));
#100525=CARTESIAN_POINT('Ctrl Pts',(-0.864305583661547,70.0322865492925,
0.));
#100526=CARTESIAN_POINT('Ctrl Pts',(-0.869602377871126,70.051109108301,
0.));
#100527=CARTESIAN_POINT('Ctrl Pts',(-0.874934213255839,70.0699781183935,
0.));
#100528=CARTESIAN_POINT('Ctrl Pts',(-0.880301109660729,70.0888934967855,
0.));
#100529=CARTESIAN_POINT('Ctrl Pts',(-0.885703094802537,70.1078550938958,
0.));
#100530=CARTESIAN_POINT('Ctrl Pts',(-0.891140203464243,70.1268626950175,
0.));
#100531=CARTESIAN_POINT('Ctrl Pts',(-0.896612474371846,70.1459160490446,
0.));
#100532=CARTESIAN_POINT('Ctrl Pts',(-0.902119947629773,70.1650148905109,
0.));
#100533=CARTESIAN_POINT('Ctrl Pts',(-0.907662662015787,70.1841589635574,
0.));
#100534=CARTESIAN_POINT('Ctrl Pts',(-0.913240652090982,70.2033480471676,
0.));
#100535=CARTESIAN_POINT('Ctrl Pts',(-0.91885394915712,70.2225819470248,
0.));
#100536=CARTESIAN_POINT('Ctrl Pts',(-0.924502582639457,70.2418604835837,
0.));
#100537=CARTESIAN_POINT('Ctrl Pts',(-0.930186581235549,70.2611834821724,
0.));
#100538=CARTESIAN_POINT('Ctrl Pts',(-0.935905974336482,70.2805507606872,
0.));
#100539=CARTESIAN_POINT('Ctrl Pts',(-0.941660792742981,70.299962123399,
0.));
#100540=CARTESIAN_POINT('Ctrl Pts',(-0.947451067929606,70.3194173673674,
0.));
#100541=CARTESIAN_POINT('Ctrl Pts',(-0.953276831581243,70.338916286458,
0.));
#100542=CARTESIAN_POINT('Ctrl Pts',(-0.959138115058833,70.3584586759536,
0.));
#100543=CARTESIAN_POINT('Ctrl Pts',(-0.965034948786451,70.3780443377956,
0.));
#100544=CARTESIAN_POINT('Ctrl Pts',(-0.970967362281175,70.3976730803614,
0.));
#100545=CARTESIAN_POINT('Ctrl Pts',(-0.976935384450043,70.417344715957,
0.));
#100546=CARTESIAN_POINT('Ctrl Pts',(-0.982939043792157,70.4370590590842,
0.));
#100547=CARTESIAN_POINT('Ctrl Pts',(-0.98897836864365,70.4568159243163,
0.));
#100548=CARTESIAN_POINT('Ctrl Pts',(-0.995053387379757,70.4766151245212,
0.));
#100549=CARTESIAN_POINT('Ctrl Pts',(-1.00116412831442,70.4964564717953,
0.));
#100550=CARTESIAN_POINT('Ctrl Pts',(-1.00731061960968,70.5163397782713,
0.));
#100551=CARTESIAN_POINT('Ctrl Pts',(-1.01349288918537,70.5362648569061,
0.));
#100552=CARTESIAN_POINT('Ctrl Pts',(-1.01971096460597,70.556231522419,0.));
#100553=CARTESIAN_POINT('Ctrl Pts',(-1.02596487304049,70.5762395916377,
0.));
#100554=CARTESIAN_POINT('Ctrl Pts',(-1.0322546413287,70.5962888829934,0.));
#100555=CARTESIAN_POINT('Ctrl Pts',(-1.03858029601904,70.6163792162073,
0.));
#100556=CARTESIAN_POINT('Ctrl Pts',(-1.04494186341156,70.6365104119252,
0.));
#100557=CARTESIAN_POINT('Ctrl Pts',(-1.05133936960072,70.6566822912991,
0.));
#100558=CARTESIAN_POINT('Ctrl Pts',(-1.0577728404773,70.676894676009,0.));
#100559=CARTESIAN_POINT('Ctrl Pts',(-1.06424230171281,70.6971473884459,
0.));
#100560=CARTESIAN_POINT('Ctrl Pts',(-1.07074777874596,70.7174402518378,
0.));
#100561=CARTESIAN_POINT('Ctrl Pts',(-1.07728929676408,70.7377730903953,
0.));
#100562=CARTESIAN_POINT('Ctrl Pts',(-1.08386688068342,70.7581457294447,
0.));
#100563=CARTESIAN_POINT('Ctrl Pts',(-1.09048055516427,70.7785579953583,
0.));
#100564=CARTESIAN_POINT('Ctrl Pts',(-1.09713034462265,70.799009715484,0.));
#100565=CARTESIAN_POINT('Ctrl Pts',(-1.10381627323947,70.8195007180745,
0.));
#100566=CARTESIAN_POINT('Ctrl Pts',(-1.1105383649664,70.8400308322037,0.));
#100567=CARTESIAN_POINT('Ctrl Pts',(-1.11729664352993,70.8605998877149,
0.));
#100568=CARTESIAN_POINT('Ctrl Pts',(-1.12409113243514,70.8812077152586,
0.));
#100569=CARTESIAN_POINT('Ctrl Pts',(-1.13092185496565,70.9018541463089,
0.));
#100570=CARTESIAN_POINT('Ctrl Pts',(-1.13778883418214,70.9225390131826,
0.));
#100571=CARTESIAN_POINT('Ctrl Pts',(-1.14469209291489,70.9432621490566,
0.));
#100572=CARTESIAN_POINT('Ctrl Pts',(-1.15163165376524,70.9640233879659,
0.));
#100573=CARTESIAN_POINT('Ctrl Pts',(-1.15860753911485,70.9848225647871,
0.));
#100574=CARTESIAN_POINT('Ctrl Pts',(-1.1656197711288,71.0056595152204,0.));
#100575=CARTESIAN_POINT('Ctrl Pts',(-1.17266837175777,71.0265340757699,
0.));
#100576=CARTESIAN_POINT('Ctrl Pts',(-1.17975336273504,71.0474460837159,
0.));
#100577=CARTESIAN_POINT('Ctrl Pts',(-1.18687476558133,71.0683953771149,
0.));
#100578=CARTESIAN_POINT('Ctrl Pts',(-1.19403260161002,71.089381794801,0.));
#100579=CARTESIAN_POINT('Ctrl Pts',(-1.20122689192836,71.1104051763839,
0.));
#100580=CARTESIAN_POINT('Ctrl Pts',(-1.20845765743648,71.1314653622442,
0.));
#100581=CARTESIAN_POINT('Ctrl Pts',(-1.21572491882263,71.1525621935267,
0.));
#100582=CARTESIAN_POINT('Ctrl Pts',(-1.22302869657018,71.1736955121362,
0.));
#100583=CARTESIAN_POINT('Ctrl Pts',(-1.23036901096239,71.194865160732,0.));
#100584=CARTESIAN_POINT('Ctrl Pts',(-1.23774588208427,71.2160709827191,
0.));
#100585=CARTESIAN_POINT('Ctrl Pts',(-1.24515932982113,71.2373128222352,
0.));
#100586=CARTESIAN_POINT('Ctrl Pts',(-1.25260937385569,71.2585905241406,
0.));
#100587=CARTESIAN_POINT('Ctrl Pts',(-1.26009603367571,71.2799039340175,
0.));
#100588=CARTESIAN_POINT('Ctrl Pts',(-1.26761932857724,71.3012528981661,
0.));
#100589=CARTESIAN_POINT('Ctrl Pts',(-1.27517927766608,71.3226372635996,
0.));
#100590=CARTESIAN_POINT('Ctrl Pts',(-1.28277589985472,71.3440568780347,
0.));
#100591=CARTESIAN_POINT('Ctrl Pts',(-1.29040921386059,71.3655115898827,
0.));
#100592=CARTESIAN_POINT('Ctrl Pts',(-1.29807923821414,71.3870012482499,
0.));
#100593=CARTESIAN_POINT('Ctrl Pts',(-1.3057859912614,71.4085257029322,0.));
#100594=CARTESIAN_POINT('Ctrl Pts',(-1.31352949116537,71.4300848044087,
0.));
#100595=CARTESIAN_POINT('Ctrl Pts',(-1.32130975590226,71.4516784038317,
0.));
#100596=CARTESIAN_POINT('Ctrl Pts',(-1.32912680326124,71.4733063530187,
0.));
#100597=CARTESIAN_POINT('Ctrl Pts',(-1.3369806508522,71.4949685044522,0.));
#100598=CARTESIAN_POINT('Ctrl Pts',(-1.34487131610781,71.516664711275,0.));
#100599=CARTESIAN_POINT('Ctrl Pts',(-1.35279881628455,71.5383948272845,
0.));
#100600=CARTESIAN_POINT('Ctrl Pts',(-1.36076316845816,71.5601587069217,
0.));
#100601=CARTESIAN_POINT('Ctrl Pts',(-1.36876438952466,71.5819562052663,
0.));
#100602=CARTESIAN_POINT('Ctrl Pts',(-1.3768024962078,71.6037871780385,0.));
#100603=CARTESIAN_POINT('Ctrl Pts',(-1.38487750506082,71.625651481593,0.));
#100604=CARTESIAN_POINT('Ctrl Pts',(-1.39298943246722,71.6475489729134,
0.));
#100605=CARTESIAN_POINT('Ctrl Pts',(-1.40113829463577,71.6694795096001,
0.));
#100606=CARTESIAN_POINT('Ctrl Pts',(-1.40932410760248,71.6914429498663,
0.));
#100607=CARTESIAN_POINT('Ctrl Pts',(-1.41754688723773,71.7134391525389,
0.));
#100608=CARTESIAN_POINT('Ctrl Pts',(-1.4258066492477,71.7354679770528,0.));
#100609=CARTESIAN_POINT('Ctrl Pts',(-1.43410340917496,71.7575292834469,
0.));
#100610=CARTESIAN_POINT('Ctrl Pts',(-1.44243718239315,71.7796229323526,
0.));
#100611=CARTESIAN_POINT('Ctrl Pts',(-1.45080798410965,71.8017487849895,
0.));
#100612=CARTESIAN_POINT('Ctrl Pts',(-1.45921582937232,71.8239067031683,
0.));
#100613=CARTESIAN_POINT('Ctrl Pts',(-1.46766073307088,71.8460965492839,
0.));
#100614=CARTESIAN_POINT('Ctrl Pts',(-1.47614270993729,71.8683181863116,
0.));
#100615=CARTESIAN_POINT('Ctrl Pts',(-1.4846617745402,71.8905714777961,0.));
#100616=CARTESIAN_POINT('Ctrl Pts',(-1.49321794128799,71.912856287848,0.));
#100617=CARTESIAN_POINT('Ctrl Pts',(-1.50181122443534,71.9351724811443,
0.));
#100618=CARTESIAN_POINT('Ctrl Pts',(-1.51044163808454,71.9575199229241,
0.));
#100619=CARTESIAN_POINT('Ctrl Pts',(-1.51910919618566,71.979898478983,0.));
#100620=CARTESIAN_POINT('Ctrl Pts',(-1.52781391253102,72.0023080156647,
0.));
#100621=CARTESIAN_POINT('Ctrl Pts',(-1.53655580075813,72.0247483998578,
0.));
#100622=CARTESIAN_POINT('Ctrl Pts',(-1.54533487435626,72.0472194989963,
0.));
#100623=CARTESIAN_POINT('Ctrl Pts',(-1.55415114666774,72.0697211810545,
0.));
#100624=CARTESIAN_POINT('Ctrl Pts',(-1.56300463088809,72.0922533145433,
0.));
#100625=CARTESIAN_POINT('Ctrl Pts',(-1.5718953400604,72.1148157684995,0.));
#100626=CARTESIAN_POINT('Ctrl Pts',(-1.58082328707803,72.1374084124839,
0.));
#100627=CARTESIAN_POINT('Ctrl Pts',(-1.58978848469123,72.1600311165821,
0.));
#100628=CARTESIAN_POINT('Ctrl Pts',(-1.59879094550847,72.1826837514001,
0.));
#100629=CARTESIAN_POINT('Ctrl Pts',(-1.60783068199663,72.2053661880608,
0.));
#100630=CARTESIAN_POINT('Ctrl Pts',(-1.6169077064754,72.2280782981937,0.));
#100631=CARTESIAN_POINT('Ctrl Pts',(-1.6260220311193,72.2508199539323,0.));
#100632=CARTESIAN_POINT('Ctrl Pts',(-1.63517366796463,72.2735910279149,
0.));
#100633=CARTESIAN_POINT('Ctrl Pts',(-1.64436262891079,72.2963913932813,
0.));
#100634=CARTESIAN_POINT('Ctrl Pts',(-1.65358892572063,72.319220923669,0.));
#100635=CARTESIAN_POINT('Ctrl Pts',(-1.66285257001496,72.3420794932047,
0.));
#100636=CARTESIAN_POINT('Ctrl Pts',(-1.67215357327365,72.3649669765004,
0.));
#100637=CARTESIAN_POINT('Ctrl Pts',(-1.68149194684282,72.387883248654,0.));
#100638=CARTESIAN_POINT('Ctrl Pts',(-1.69086770193637,72.4108281852467,
0.));
#100639=CARTESIAN_POINT('Ctrl Pts',(-1.70028084963647,72.4338016623391,
0.));
#100640=CARTESIAN_POINT('Ctrl Pts',(-1.70973140088842,72.456803556463,0.));
#100641=CARTESIAN_POINT('Ctrl Pts',(-1.71921936650038,72.479833744618,0.));
#100642=CARTESIAN_POINT('Ctrl Pts',(-1.72874475715103,72.5028921042721,
0.));
#100643=CARTESIAN_POINT('Ctrl Pts',(-1.73830758339125,72.5259785133595,
0.));
#100644=CARTESIAN_POINT('Ctrl Pts',(-1.74790785564474,72.5490928502769,
0.));
#100645=CARTESIAN_POINT('Ctrl Pts',(-1.75754558420344,72.5722349938774,
0.));
#100646=CARTESIAN_POINT('Ctrl Pts',(-1.76722077922574,72.5954048234638,
0.));
#100647=CARTESIAN_POINT('Ctrl Pts',(-1.77693345074427,72.6186022187907,
0.));
#100648=CARTESIAN_POINT('Ctrl Pts',(-1.78668360866811,72.6418270600619,
0.));
#100649=CARTESIAN_POINT('Ctrl Pts',(-1.79647126278359,72.6650792279274,
0.));
#100650=CARTESIAN_POINT('Ctrl Pts',(-1.80629642275051,72.6883586034769,
0.));
#100651=CARTESIAN_POINT('Ctrl Pts',(-1.81615909809871,72.7116650682344,
0.));
#100652=CARTESIAN_POINT('Ctrl Pts',(-1.82605929823564,72.7349985041592,
0.));
#100653=CARTESIAN_POINT('Ctrl Pts',(-1.83599703244924,72.7583587936447,
0.));
#100654=CARTESIAN_POINT('Ctrl Pts',(-1.84597230990857,72.7817458195155,
0.));
#100655=CARTESIAN_POINT('Ctrl Pts',(-1.85598513966114,72.8051594650222,
0.));
#100656=CARTESIAN_POINT('Ctrl Pts',(-1.86603553062771,72.8285996138359,
0.));
#100657=CARTESIAN_POINT('Ctrl Pts',(-1.87612349160945,72.8520661500477,
0.));
#100658=CARTESIAN_POINT('Ctrl Pts',(-1.88624903129188,72.875558958168,0.));
#100659=CARTESIAN_POINT('Ctrl Pts',(-1.89641215824582,72.8990779231226,
0.));
#100660=CARTESIAN_POINT('Ctrl Pts',(-1.90661288092587,72.9226229302478,
0.));
#100661=CARTESIAN_POINT('Ctrl Pts',(-1.91685120766437,72.9461938652811,
0.));
#100662=CARTESIAN_POINT('Ctrl Pts',(-1.9271271466766,72.9697906143636,0.));
#100663=CARTESIAN_POINT('Ctrl Pts',(-1.93744070606566,72.9934130640415,
0.));
#100664=CARTESIAN_POINT('Ctrl Pts',(-1.94779189382302,73.0170611012661,
0.));
#100665=CARTESIAN_POINT('Ctrl Pts',(-1.95818071782767,73.040734613391,0.));
#100666=CARTESIAN_POINT('Ctrl Pts',(-1.96860718583932,73.0644334881673,
0.));
#100667=CARTESIAN_POINT('Ctrl Pts',(-1.97907130550158,73.0881576137407,
0.));
#100668=CARTESIAN_POINT('Ctrl Pts',(-1.98957308434918,73.1119068786475,
0.));
#100669=CARTESIAN_POINT('Ctrl Pts',(-2.00011252980982,73.1356811718091,
0.));
#100670=CARTESIAN_POINT('Ctrl Pts',(-2.01068964920467,73.1594803825252,
0.));
#100671=CARTESIAN_POINT('Ctrl Pts',(-2.02130444974362,73.183304400462,0.));
#100672=CARTESIAN_POINT('Ctrl Pts',(-2.03195693852455,73.2071531156504,
0.));
#100673=CARTESIAN_POINT('Ctrl Pts',(-2.04264712253929,73.2310264184976,
0.));
#100674=CARTESIAN_POINT('Ctrl Pts',(-2.05337500867403,73.2549241997953,
0.));
#100675=CARTESIAN_POINT('Ctrl Pts',(-2.06414060370835,73.2788463507246,
0.));
#100676=CARTESIAN_POINT('Ctrl Pts',(-2.07494391430941,73.3027927628626,
0.));
#100677=CARTESIAN_POINT('Ctrl Pts',(-2.08578494702744,73.3267633281807,
0.));
#100678=CARTESIAN_POINT('Ctrl Pts',(-2.09666370830716,73.3507579390239,
0.));
#100679=CARTESIAN_POINT('Ctrl Pts',(-2.1075802044939,73.3747764880893,0.));
#100680=CARTESIAN_POINT('Ctrl Pts',(-2.11853444183762,73.3988188684021,
0.));
#100681=CARTESIAN_POINT('Ctrl Pts',(-2.12952642649368,73.4228849732925,
0.));
#100682=CARTESIAN_POINT('Ctrl Pts',(-2.14055616452058,73.4469746963637,
0.));
#100683=CARTESIAN_POINT('Ctrl Pts',(-2.15162366187907,73.4710879315382,
0.));
#100684=CARTESIAN_POINT('Ctrl Pts',(-2.1627289244292,73.4952245731054,0.));
#100685=CARTESIAN_POINT('Ctrl Pts',(-2.17387195792306,73.5193845157708,
0.));
#100686=CARTESIAN_POINT('Ctrl Pts',(-2.18505276799753,73.5435676546929,
0.));
#100687=CARTESIAN_POINT('Ctrl Pts',(-2.19627136015678,73.5677738855452,
0.));
#100688=CARTESIAN_POINT('Ctrl Pts',(-2.20752773978349,73.5920031044595,
0.));
#100689=CARTESIAN_POINT('Ctrl Pts',(-2.21882191216518,73.6162552079038,
0.));
#100690=CARTESIAN_POINT('Ctrl Pts',(-2.23015388251288,73.6405300925712,
0.));
#100691=CARTESIAN_POINT('Ctrl Pts',(-2.24152365597698,73.6648276552767,
0.));
#100692=CARTESIAN_POINT('Ctrl Pts',(-2.25293123766425,73.6891477928129,
0.));
#100693=CARTESIAN_POINT('Ctrl Pts',(-2.26437663263667,73.7134904019389,
0.));
#100694=CARTESIAN_POINT('Ctrl Pts',(-2.27585984587199,73.7378553796807,
0.));
#100695=CARTESIAN_POINT('Ctrl Pts',(-2.28738088222864,73.762242623566,0.));
#100696=CARTESIAN_POINT('Ctrl Pts',(-2.29893974640434,73.786652031885,0.));
#100697=CARTESIAN_POINT('Ctrl Pts',(-2.31053644289417,73.8110835039327,
0.));
#100698=CARTESIAN_POINT('Ctrl Pts',(-2.32217097594198,73.8355369402706,
0.));
#100699=CARTESIAN_POINT('Ctrl Pts',(-2.33384334963958,73.8600122421468,
0.));
#100700=CARTESIAN_POINT('Ctrl Pts',(-2.34555356802121,73.8845093109274,
0.));
#100701=CARTESIAN_POINT('Ctrl Pts',(-2.35730163516316,73.9090280474712,
0.));
#100702=CARTESIAN_POINT('Ctrl Pts',(-2.36908755526003,73.9335683516404,
0.));
#100703=CARTESIAN_POINT('Ctrl Pts',(-2.38091133274961,73.958130121465,0.));
#100704=CARTESIAN_POINT('Ctrl Pts',(-2.39277297220757,73.9827132538206,
0.));
#100705=CARTESIAN_POINT('Ctrl Pts',(-2.40467247811536,74.0073176459344,
0.));
#100706=CARTESIAN_POINT('Ctrl Pts',(-2.41660985465252,74.0319431966989,
0.));
#100707=CARTESIAN_POINT('Ctrl Pts',(-2.42858510549779,74.0565898079218,
0.));
#100708=CARTESIAN_POINT('Ctrl Pts',(-2.44059823356676,74.0812573859411,
0.));
#100709=CARTESIAN_POINT('Ctrl Pts',(-2.45264924094775,74.1059458420067,
0.));
#100710=CARTESIAN_POINT('Ctrl Pts',(-2.46301176097121,74.127126454519,0.));
#100711=CARTESIAN_POINT('Ctrl Pts',(-2.47097695564999,74.1433763941381,
0.));
#100712=CARTESIAN_POINT('Ctrl Pts',(-2.47652804724547,74.1546864735168,
0.));
#100713=CARTESIAN_POINT('Ctrl Pts',(-2.47965393945487,74.1610506466209,
0.));
#100714=CARTESIAN_POINT('Ctrl Pts',(-2.48034921843244,74.1624659714558,
0.));
#100715=CARTESIAN_POINT('',(-0.853825826608985,69.9947925310006,12.));
#100716=CARTESIAN_POINT('',(-0.853825826608985,69.9947925310006,0.));
#100717=CARTESIAN_POINT('Ctrl Pts',(-2.48034921843246,74.1624659714558,
12.));
#100718=CARTESIAN_POINT('Ctrl Pts',(-2.47965393945489,74.1610506466209,
12.));
#100719=CARTESIAN_POINT('Ctrl Pts',(-2.47652804724548,74.1546864735169,
12.));
#100720=CARTESIAN_POINT('Ctrl Pts',(-2.47097695565,74.1433763941382,12.));
#100721=CARTESIAN_POINT('Ctrl Pts',(-2.46301176097121,74.127126454519,12.));
#100722=CARTESIAN_POINT('Ctrl Pts',(-2.45264924094775,74.1059458420067,
12.));
#100723=CARTESIAN_POINT('Ctrl Pts',(-2.44059823356676,74.0812573859411,
12.));
#100724=CARTESIAN_POINT('Ctrl Pts',(-2.42858510549779,74.0565898079218,
12.));
#100725=CARTESIAN_POINT('Ctrl Pts',(-2.41660985465252,74.0319431966989,
12.));
#100726=CARTESIAN_POINT('Ctrl Pts',(-2.40467247811536,74.0073176459344,
12.));
#100727=CARTESIAN_POINT('Ctrl Pts',(-2.39277297220757,73.9827132538206,
12.));
#100728=CARTESIAN_POINT('Ctrl Pts',(-2.38091133274961,73.958130121465,12.));
#100729=CARTESIAN_POINT('Ctrl Pts',(-2.36908755526003,73.9335683516404,
12.));
#100730=CARTESIAN_POINT('Ctrl Pts',(-2.35730163516316,73.9090280474712,
12.));
#100731=CARTESIAN_POINT('Ctrl Pts',(-2.34555356802121,73.8845093109274,
12.));
#100732=CARTESIAN_POINT('Ctrl Pts',(-2.33384334963958,73.8600122421468,
12.));
#100733=CARTESIAN_POINT('Ctrl Pts',(-2.32217097594198,73.8355369402706,
12.));
#100734=CARTESIAN_POINT('Ctrl Pts',(-2.31053644289417,73.8110835039327,
12.));
#100735=CARTESIAN_POINT('Ctrl Pts',(-2.29893974640434,73.786652031885,12.));
#100736=CARTESIAN_POINT('Ctrl Pts',(-2.28738088222864,73.762242623566,12.));
#100737=CARTESIAN_POINT('Ctrl Pts',(-2.27585984587199,73.7378553796807,
12.));
#100738=CARTESIAN_POINT('Ctrl Pts',(-2.26437663263667,73.7134904019389,
12.));
#100739=CARTESIAN_POINT('Ctrl Pts',(-2.25293123766425,73.6891477928129,
12.));
#100740=CARTESIAN_POINT('Ctrl Pts',(-2.24152365597698,73.6648276552767,
12.));
#100741=CARTESIAN_POINT('Ctrl Pts',(-2.23015388251288,73.6405300925712,
12.));
#100742=CARTESIAN_POINT('Ctrl Pts',(-2.21882191216518,73.6162552079038,
12.));
#100743=CARTESIAN_POINT('Ctrl Pts',(-2.20752773978349,73.5920031044595,
12.));
#100744=CARTESIAN_POINT('Ctrl Pts',(-2.19627136015678,73.5677738855452,
12.));
#100745=CARTESIAN_POINT('Ctrl Pts',(-2.18505276799753,73.5435676546929,
12.));
#100746=CARTESIAN_POINT('Ctrl Pts',(-2.17387195792306,73.5193845157708,
12.));
#100747=CARTESIAN_POINT('Ctrl Pts',(-2.1627289244292,73.4952245731054,12.));
#100748=CARTESIAN_POINT('Ctrl Pts',(-2.15162366187907,73.4710879315382,
12.));
#100749=CARTESIAN_POINT('Ctrl Pts',(-2.14055616452058,73.4469746963637,
12.));
#100750=CARTESIAN_POINT('Ctrl Pts',(-2.12952642649368,73.4228849732925,
12.));
#100751=CARTESIAN_POINT('Ctrl Pts',(-2.11853444183762,73.3988188684021,
12.));
#100752=CARTESIAN_POINT('Ctrl Pts',(-2.1075802044939,73.3747764880893,12.));
#100753=CARTESIAN_POINT('Ctrl Pts',(-2.09666370830716,73.3507579390239,
12.));
#100754=CARTESIAN_POINT('Ctrl Pts',(-2.08578494702744,73.3267633281807,
12.));
#100755=CARTESIAN_POINT('Ctrl Pts',(-2.07494391430941,73.3027927628626,
12.));
#100756=CARTESIAN_POINT('Ctrl Pts',(-2.06414060370835,73.2788463507246,
12.));
#100757=CARTESIAN_POINT('Ctrl Pts',(-2.05337500867403,73.2549241997953,
12.));
#100758=CARTESIAN_POINT('Ctrl Pts',(-2.04264712253929,73.2310264184976,
12.));
#100759=CARTESIAN_POINT('Ctrl Pts',(-2.03195693852455,73.2071531156504,
12.));
#100760=CARTESIAN_POINT('Ctrl Pts',(-2.02130444974362,73.183304400462,12.));
#100761=CARTESIAN_POINT('Ctrl Pts',(-2.01068964920467,73.1594803825252,
12.));
#100762=CARTESIAN_POINT('Ctrl Pts',(-2.00011252980982,73.1356811718091,
12.));
#100763=CARTESIAN_POINT('Ctrl Pts',(-1.98957308434918,73.1119068786475,
12.));
#100764=CARTESIAN_POINT('Ctrl Pts',(-1.97907130550158,73.0881576137407,
12.));
#100765=CARTESIAN_POINT('Ctrl Pts',(-1.96860718583932,73.0644334881673,
12.));
#100766=CARTESIAN_POINT('Ctrl Pts',(-1.95818071782767,73.040734613391,12.));
#100767=CARTESIAN_POINT('Ctrl Pts',(-1.94779189382302,73.0170611012661,
12.));
#100768=CARTESIAN_POINT('Ctrl Pts',(-1.93744070606566,72.9934130640415,
12.));
#100769=CARTESIAN_POINT('Ctrl Pts',(-1.9271271466766,72.9697906143636,12.));
#100770=CARTESIAN_POINT('Ctrl Pts',(-1.91685120766437,72.9461938652811,
12.));
#100771=CARTESIAN_POINT('Ctrl Pts',(-1.90661288092587,72.9226229302478,
12.));
#100772=CARTESIAN_POINT('Ctrl Pts',(-1.89641215824582,72.8990779231226,
12.));
#100773=CARTESIAN_POINT('Ctrl Pts',(-1.88624903129188,72.875558958168,12.));
#100774=CARTESIAN_POINT('Ctrl Pts',(-1.87612349160945,72.8520661500477,
12.));
#100775=CARTESIAN_POINT('Ctrl Pts',(-1.86603553062771,72.8285996138359,
12.));
#100776=CARTESIAN_POINT('Ctrl Pts',(-1.85598513966114,72.8051594650222,
12.));
#100777=CARTESIAN_POINT('Ctrl Pts',(-1.84597230990857,72.7817458195155,
12.));
#100778=CARTESIAN_POINT('Ctrl Pts',(-1.83599703244924,72.7583587936447,
12.));
#100779=CARTESIAN_POINT('Ctrl Pts',(-1.82605929823564,72.7349985041592,
12.));
#100780=CARTESIAN_POINT('Ctrl Pts',(-1.81615909809871,72.7116650682344,
12.));
#100781=CARTESIAN_POINT('Ctrl Pts',(-1.80629642275051,72.6883586034769,
12.));
#100782=CARTESIAN_POINT('Ctrl Pts',(-1.79647126278359,72.6650792279274,
12.));
#100783=CARTESIAN_POINT('Ctrl Pts',(-1.78668360866811,72.6418270600619,
12.));
#100784=CARTESIAN_POINT('Ctrl Pts',(-1.77693345074427,72.6186022187907,
12.));
#100785=CARTESIAN_POINT('Ctrl Pts',(-1.76722077922574,72.5954048234638,
12.));
#100786=CARTESIAN_POINT('Ctrl Pts',(-1.75754558420344,72.5722349938774,
12.));
#100787=CARTESIAN_POINT('Ctrl Pts',(-1.74790785564474,72.5490928502769,
12.));
#100788=CARTESIAN_POINT('Ctrl Pts',(-1.73830758339125,72.5259785133595,
12.));
#100789=CARTESIAN_POINT('Ctrl Pts',(-1.72874475715103,72.5028921042721,
12.));
#100790=CARTESIAN_POINT('Ctrl Pts',(-1.71921936650038,72.479833744618,12.));
#100791=CARTESIAN_POINT('Ctrl Pts',(-1.70973140088842,72.456803556463,12.));
#100792=CARTESIAN_POINT('Ctrl Pts',(-1.70028084963647,72.4338016623391,
12.));
#100793=CARTESIAN_POINT('Ctrl Pts',(-1.69086770193637,72.4108281852467,
12.));
#100794=CARTESIAN_POINT('Ctrl Pts',(-1.68149194684282,72.387883248654,12.));
#100795=CARTESIAN_POINT('Ctrl Pts',(-1.67215357327365,72.3649669765004,
12.));
#100796=CARTESIAN_POINT('Ctrl Pts',(-1.66285257001496,72.3420794932047,
12.));
#100797=CARTESIAN_POINT('Ctrl Pts',(-1.65358892572063,72.319220923669,12.));
#100798=CARTESIAN_POINT('Ctrl Pts',(-1.64436262891079,72.2963913932813,
12.));
#100799=CARTESIAN_POINT('Ctrl Pts',(-1.63517366796463,72.2735910279149,
12.));
#100800=CARTESIAN_POINT('Ctrl Pts',(-1.6260220311193,72.2508199539323,12.));
#100801=CARTESIAN_POINT('Ctrl Pts',(-1.6169077064754,72.2280782981937,12.));
#100802=CARTESIAN_POINT('Ctrl Pts',(-1.60783068199663,72.2053661880608,
12.));
#100803=CARTESIAN_POINT('Ctrl Pts',(-1.59879094550847,72.1826837514001,
12.));
#100804=CARTESIAN_POINT('Ctrl Pts',(-1.58978848469123,72.1600311165821,
12.));
#100805=CARTESIAN_POINT('Ctrl Pts',(-1.58082328707803,72.1374084124839,
12.));
#100806=CARTESIAN_POINT('Ctrl Pts',(-1.5718953400604,72.1148157684995,12.));
#100807=CARTESIAN_POINT('Ctrl Pts',(-1.56300463088809,72.0922533145433,
12.));
#100808=CARTESIAN_POINT('Ctrl Pts',(-1.55415114666774,72.0697211810545,
12.));
#100809=CARTESIAN_POINT('Ctrl Pts',(-1.54533487435626,72.0472194989963,
12.));
#100810=CARTESIAN_POINT('Ctrl Pts',(-1.53655580075813,72.0247483998578,
12.));
#100811=CARTESIAN_POINT('Ctrl Pts',(-1.52781391253102,72.0023080156647,
12.));
#100812=CARTESIAN_POINT('Ctrl Pts',(-1.51910919618566,71.979898478983,12.));
#100813=CARTESIAN_POINT('Ctrl Pts',(-1.51044163808454,71.9575199229241,
12.));
#100814=CARTESIAN_POINT('Ctrl Pts',(-1.50181122443534,71.9351724811443,
12.));
#100815=CARTESIAN_POINT('Ctrl Pts',(-1.49321794128799,71.912856287848,12.));
#100816=CARTESIAN_POINT('Ctrl Pts',(-1.4846617745402,71.8905714777961,12.));
#100817=CARTESIAN_POINT('Ctrl Pts',(-1.47614270993729,71.8683181863116,
12.));
#100818=CARTESIAN_POINT('Ctrl Pts',(-1.46766073307088,71.8460965492839,
12.));
#100819=CARTESIAN_POINT('Ctrl Pts',(-1.45921582937232,71.8239067031683,
12.));
#100820=CARTESIAN_POINT('Ctrl Pts',(-1.45080798410965,71.8017487849895,
12.));
#100821=CARTESIAN_POINT('Ctrl Pts',(-1.44243718239315,71.7796229323526,
12.));
#100822=CARTESIAN_POINT('Ctrl Pts',(-1.43410340917496,71.7575292834469,
12.));
#100823=CARTESIAN_POINT('Ctrl Pts',(-1.4258066492477,71.7354679770528,12.));
#100824=CARTESIAN_POINT('Ctrl Pts',(-1.41754688723773,71.7134391525389,
12.));
#100825=CARTESIAN_POINT('Ctrl Pts',(-1.40932410760248,71.6914429498663,
12.));
#100826=CARTESIAN_POINT('Ctrl Pts',(-1.40113829463577,71.6694795096001,
12.));
#100827=CARTESIAN_POINT('Ctrl Pts',(-1.39298943246722,71.6475489729134,
12.));
#100828=CARTESIAN_POINT('Ctrl Pts',(-1.38487750506082,71.625651481593,12.));
#100829=CARTESIAN_POINT('Ctrl Pts',(-1.3768024962078,71.6037871780385,12.));
#100830=CARTESIAN_POINT('Ctrl Pts',(-1.36876438952466,71.5819562052663,
12.));
#100831=CARTESIAN_POINT('Ctrl Pts',(-1.36076316845816,71.5601587069217,
12.));
#100832=CARTESIAN_POINT('Ctrl Pts',(-1.35279881628455,71.5383948272845,
12.));
#100833=CARTESIAN_POINT('Ctrl Pts',(-1.34487131610781,71.516664711275,12.));
#100834=CARTESIAN_POINT('Ctrl Pts',(-1.3369806508522,71.4949685044522,12.));
#100835=CARTESIAN_POINT('Ctrl Pts',(-1.32912680326124,71.4733063530187,
12.));
#100836=CARTESIAN_POINT('Ctrl Pts',(-1.32130975590226,71.4516784038317,
12.));
#100837=CARTESIAN_POINT('Ctrl Pts',(-1.31352949116537,71.4300848044087,
12.));
#100838=CARTESIAN_POINT('Ctrl Pts',(-1.3057859912614,71.4085257029322,12.));
#100839=CARTESIAN_POINT('Ctrl Pts',(-1.29807923821414,71.3870012482499,
12.));
#100840=CARTESIAN_POINT('Ctrl Pts',(-1.29040921386059,71.3655115898827,
12.));
#100841=CARTESIAN_POINT('Ctrl Pts',(-1.28277589985472,71.3440568780347,
12.));
#100842=CARTESIAN_POINT('Ctrl Pts',(-1.27517927766608,71.3226372635996,
12.));
#100843=CARTESIAN_POINT('Ctrl Pts',(-1.26761932857724,71.3012528981661,
12.));
#100844=CARTESIAN_POINT('Ctrl Pts',(-1.26009603367571,71.2799039340175,
12.));
#100845=CARTESIAN_POINT('Ctrl Pts',(-1.25260937385569,71.2585905241406,
12.));
#100846=CARTESIAN_POINT('Ctrl Pts',(-1.24515932982113,71.2373128222352,
12.));
#100847=CARTESIAN_POINT('Ctrl Pts',(-1.23774588208427,71.2160709827191,
12.));
#100848=CARTESIAN_POINT('Ctrl Pts',(-1.23036901096239,71.194865160732,12.));
#100849=CARTESIAN_POINT('Ctrl Pts',(-1.22302869657018,71.1736955121362,
12.));
#100850=CARTESIAN_POINT('Ctrl Pts',(-1.21572491882263,71.1525621935267,
12.));
#100851=CARTESIAN_POINT('Ctrl Pts',(-1.20845765743648,71.1314653622442,
12.));
#100852=CARTESIAN_POINT('Ctrl Pts',(-1.20122689192836,71.1104051763839,
12.));
#100853=CARTESIAN_POINT('Ctrl Pts',(-1.19403260161002,71.089381794801,12.));
#100854=CARTESIAN_POINT('Ctrl Pts',(-1.18687476558133,71.0683953771149,
12.));
#100855=CARTESIAN_POINT('Ctrl Pts',(-1.17975336273504,71.0474460837159,
12.));
#100856=CARTESIAN_POINT('Ctrl Pts',(-1.17266837175777,71.0265340757699,
12.));
#100857=CARTESIAN_POINT('Ctrl Pts',(-1.1656197711288,71.0056595152204,12.));
#100858=CARTESIAN_POINT('Ctrl Pts',(-1.15860753911485,70.9848225647871,
12.));
#100859=CARTESIAN_POINT('Ctrl Pts',(-1.15163165376524,70.9640233879659,
12.));
#100860=CARTESIAN_POINT('Ctrl Pts',(-1.14469209291489,70.9432621490566,
12.));
#100861=CARTESIAN_POINT('Ctrl Pts',(-1.13778883418214,70.9225390131826,
12.));
#100862=CARTESIAN_POINT('Ctrl Pts',(-1.13092185496565,70.9018541463089,
12.));
#100863=CARTESIAN_POINT('Ctrl Pts',(-1.12409113243514,70.8812077152586,
12.));
#100864=CARTESIAN_POINT('Ctrl Pts',(-1.11729664352993,70.8605998877149,
12.));
#100865=CARTESIAN_POINT('Ctrl Pts',(-1.1105383649664,70.8400308322037,12.));
#100866=CARTESIAN_POINT('Ctrl Pts',(-1.10381627323947,70.8195007180745,
12.));
#100867=CARTESIAN_POINT('Ctrl Pts',(-1.09713034462265,70.799009715484,12.));
#100868=CARTESIAN_POINT('Ctrl Pts',(-1.09048055516427,70.7785579953583,
12.));
#100869=CARTESIAN_POINT('Ctrl Pts',(-1.08386688068342,70.7581457294447,
12.));
#100870=CARTESIAN_POINT('Ctrl Pts',(-1.07728929676408,70.7377730903953,
12.));
#100871=CARTESIAN_POINT('Ctrl Pts',(-1.07074777874596,70.7174402518378,
12.));
#100872=CARTESIAN_POINT('Ctrl Pts',(-1.06424230171281,70.6971473884459,
12.));
#100873=CARTESIAN_POINT('Ctrl Pts',(-1.0577728404773,70.676894676009,12.));
#100874=CARTESIAN_POINT('Ctrl Pts',(-1.05133936960072,70.6566822912991,
12.));
#100875=CARTESIAN_POINT('Ctrl Pts',(-1.04494186341156,70.6365104119252,
12.));
#100876=CARTESIAN_POINT('Ctrl Pts',(-1.03858029601904,70.6163792162073,
12.));
#100877=CARTESIAN_POINT('Ctrl Pts',(-1.0322546413287,70.5962888829934,12.));
#100878=CARTESIAN_POINT('Ctrl Pts',(-1.02596487304049,70.5762395916377,
12.));
#100879=CARTESIAN_POINT('Ctrl Pts',(-1.01971096460597,70.556231522419,12.));
#100880=CARTESIAN_POINT('Ctrl Pts',(-1.01349288918537,70.5362648569061,
12.));
#100881=CARTESIAN_POINT('Ctrl Pts',(-1.00731061960968,70.5163397782713,
12.));
#100882=CARTESIAN_POINT('Ctrl Pts',(-1.00116412831442,70.4964564717953,
12.));
#100883=CARTESIAN_POINT('Ctrl Pts',(-0.995053387379757,70.4766151245212,
12.));
#100884=CARTESIAN_POINT('Ctrl Pts',(-0.98897836864365,70.4568159243163,
12.));
#100885=CARTESIAN_POINT('Ctrl Pts',(-0.982939043792157,70.4370590590842,
12.));
#100886=CARTESIAN_POINT('Ctrl Pts',(-0.976935384450043,70.417344715957,
12.));
#100887=CARTESIAN_POINT('Ctrl Pts',(-0.970967362281175,70.3976730803614,
12.));
#100888=CARTESIAN_POINT('Ctrl Pts',(-0.965034948786451,70.3780443377956,
12.));
#100889=CARTESIAN_POINT('Ctrl Pts',(-0.959138115058833,70.3584586759536,
12.));
#100890=CARTESIAN_POINT('Ctrl Pts',(-0.953276831581243,70.338916286458,
12.));
#100891=CARTESIAN_POINT('Ctrl Pts',(-0.947451067929606,70.3194173673674,
12.));
#100892=CARTESIAN_POINT('Ctrl Pts',(-0.941660792742981,70.299962123399,
12.));
#100893=CARTESIAN_POINT('Ctrl Pts',(-0.935905974336482,70.2805507606872,
12.));
#100894=CARTESIAN_POINT('Ctrl Pts',(-0.930186581235549,70.2611834821724,
12.));
#100895=CARTESIAN_POINT('Ctrl Pts',(-0.924502582639457,70.2418604835837,
12.));
#100896=CARTESIAN_POINT('Ctrl Pts',(-0.91885394915712,70.2225819470248,
12.));
#100897=CARTESIAN_POINT('Ctrl Pts',(-0.913240652090982,70.2033480471676,
12.));
#100898=CARTESIAN_POINT('Ctrl Pts',(-0.907662662015787,70.1841589635574,
12.));
#100899=CARTESIAN_POINT('Ctrl Pts',(-0.902119947629773,70.1650148905109,
12.));
#100900=CARTESIAN_POINT('Ctrl Pts',(-0.896612474371846,70.1459160490446,
12.));
#100901=CARTESIAN_POINT('Ctrl Pts',(-0.891140203464243,70.1268626950175,
12.));
#100902=CARTESIAN_POINT('Ctrl Pts',(-0.885703094802537,70.1078550938958,
12.));
#100903=CARTESIAN_POINT('Ctrl Pts',(-0.880301109660729,70.0888934967855,
12.));
#100904=CARTESIAN_POINT('Ctrl Pts',(-0.874934213255839,70.0699781183935,
12.));
#100905=CARTESIAN_POINT('Ctrl Pts',(-0.869602377871126,70.051109108301,
12.));
#100906=CARTESIAN_POINT('Ctrl Pts',(-0.864305583661547,70.0322865492925,
12.));
#100907=CARTESIAN_POINT('Ctrl Pts',(-0.860096170668736,70.0172656933806,
12.));
#100908=CARTESIAN_POINT('Ctrl Pts',(-0.856954870259207,70.0060209754087,
12.));
#100909=CARTESIAN_POINT('Ctrl Pts',(-0.854867673848596,69.9985337959407,
12.));
#100910=CARTESIAN_POINT('Ctrl Pts',(-0.853825826608985,69.9947925310006,
12.));
#100911=CARTESIAN_POINT('Ctrl Pts',(-3.99277406490868,74.0964320766208,
0.));
#100912=CARTESIAN_POINT('Ctrl Pts',(-3.99277406490868,74.0964320766208,
4.));
#100913=CARTESIAN_POINT('Ctrl Pts',(-3.99277406490873,74.0964320766207,
8.));
#100914=CARTESIAN_POINT('Ctrl Pts',(-3.99277406490873,74.0964320766207,
12.));
#100915=CARTESIAN_POINT('Ctrl Pts',(-3.95310474582227,74.1989040313893,
0.));
#100916=CARTESIAN_POINT('Ctrl Pts',(-3.95310474582227,74.1989040313893,
4.));
#100917=CARTESIAN_POINT('Ctrl Pts',(-3.95310474582232,74.1989040313892,
8.00000000000001));
#100918=CARTESIAN_POINT('Ctrl Pts',(-3.95310474582232,74.1989040313892,
12.));
#100919=CARTESIAN_POINT('Ctrl Pts',(-3.8225214201853,74.3538917248566,0.));
#100920=CARTESIAN_POINT('Ctrl Pts',(-3.8225214201853,74.3538917248566,4.));
#100921=CARTESIAN_POINT('Ctrl Pts',(-3.82252142018534,74.3538917248565,
7.99999999999999));
#100922=CARTESIAN_POINT('Ctrl Pts',(-3.82252142018534,74.3538917248565,
12.));
#100923=CARTESIAN_POINT('Ctrl Pts',(-3.63264011802871,74.4114286752098,
0.));
#100924=CARTESIAN_POINT('Ctrl Pts',(-3.63264011802871,74.4114286752098,
4.));
#100925=CARTESIAN_POINT('Ctrl Pts',(-3.63264011802875,74.4114286752097,
8.00000000000001));
#100926=CARTESIAN_POINT('Ctrl Pts',(-3.63264011802875,74.4114286752097,
12.));
#100927=CARTESIAN_POINT('Ctrl Pts',(-3.55032190142806,74.4153560388998,
0.));
#100928=CARTESIAN_POINT('Ctrl Pts',(-3.55032190142806,74.4153560388998,
4.));
#100929=CARTESIAN_POINT('Ctrl Pts',(-3.55032190142811,74.4153560388997,
8.));
#100930=CARTESIAN_POINT('Ctrl Pts',(-3.55032190142811,74.4153560388997,
12.));
#100931=CARTESIAN_POINT('',(-3.99277406490868,74.0964320766208,0.));
#100932=CARTESIAN_POINT('',(-3.55032190142807,74.4153560388999,0.));
#100933=CARTESIAN_POINT('Ctrl Pts',(-3.99277406490868,74.0964320766208,
2.77555756156289E-16));
#100934=CARTESIAN_POINT('Ctrl Pts',(-3.95310474582227,74.1989040313893,
2.77555756156289E-16));
#100935=CARTESIAN_POINT('Ctrl Pts',(-3.87848570260114,74.2874684276564,
2.77555756156289E-16));
#100936=CARTESIAN_POINT('Ctrl Pts',(-3.78450405480218,74.3442121731106,
2.77555756156289E-16));
#100937=CARTESIAN_POINT('Ctrl Pts',(-3.71401781895296,74.3867699822013,
2.77555756156289E-16));
#100938=CARTESIAN_POINT('Ctrl Pts',(-3.63264011802871,74.4114286752098,
2.77555756156289E-16));
#100939=CARTESIAN_POINT('Ctrl Pts',(-3.55032190142806,74.4153560388998,
2.77555756156289E-16));
#100940=CARTESIAN_POINT('',(-3.55032190142812,74.4153560388999,12.));
#100941=CARTESIAN_POINT('Ctrl Pts',(-3.55032190142806,74.4153560388998,
0.));
#100942=CARTESIAN_POINT('Ctrl Pts',(-3.55032190142806,74.4153560388998,
4.));
#100943=CARTESIAN_POINT('Ctrl Pts',(-3.55032190142811,74.4153560388997,
8.));
#100944=CARTESIAN_POINT('Ctrl Pts',(-3.55032190142811,74.4153560388997,
12.));
#100945=CARTESIAN_POINT('',(-3.99277406490873,74.0964320766207,12.));
#100946=CARTESIAN_POINT('Ctrl Pts',(-3.55032190142811,74.4153560388997,
12.));
#100947=CARTESIAN_POINT('Ctrl Pts',(-3.63264011802875,74.4114286752097,
12.));
#100948=CARTESIAN_POINT('Ctrl Pts',(-3.714017818953,74.3867699822012,12.));
#100949=CARTESIAN_POINT('Ctrl Pts',(-3.78450405480223,74.3442121731105,
12.));
#100950=CARTESIAN_POINT('Ctrl Pts',(-3.87848570260119,74.2874684276563,
12.));
#100951=CARTESIAN_POINT('Ctrl Pts',(-3.95310474582232,74.1989040313892,
12.));
#100952=CARTESIAN_POINT('Ctrl Pts',(-3.99277406490873,74.0964320766207,
12.));
#100953=CARTESIAN_POINT('Ctrl Pts',(-3.99277406490873,74.0964320766207,
12.));
#100954=CARTESIAN_POINT('Ctrl Pts',(-3.99277406490873,74.0964320766207,
8.));
#100955=CARTESIAN_POINT('Ctrl Pts',(-3.99277406490868,74.0964320766208,
4.));
#100956=CARTESIAN_POINT('Ctrl Pts',(-3.99277406490868,74.0964320766208,
0.));
#100957=CARTESIAN_POINT('Origin',(-1.64496194443586E-11,3.74482667098164E-10,
0.));
#100958=CARTESIAN_POINT('Origin',(-1.64496194443586E-11,3.74482667098164E-10,
12.));
#100959=CARTESIAN_POINT('Origin',(-1.64496194443586E-11,3.74482667098164E-10,
0.));
#100960=CARTESIAN_POINT('Ctrl Pts',(3.55032190142515,74.4153560389001,-5.55111512312578E-16));
#100961=CARTESIAN_POINT('Ctrl Pts',(3.55032190142515,74.4153560389001,4.));
#100962=CARTESIAN_POINT('Ctrl Pts',(3.55032190142515,74.4153560389001,8.));
#100963=CARTESIAN_POINT('Ctrl Pts',(3.55032190142515,74.4153560389001,12.));
#100964=CARTESIAN_POINT('Ctrl Pts',(3.66007952356777,74.4101195539797,-5.55111512312578E-16));
#100965=CARTESIAN_POINT('Ctrl Pts',(3.66007952356777,74.4101195539797,4.));
#100966=CARTESIAN_POINT('Ctrl Pts',(3.66007952356776,74.4101195539797,8.00000000000001));
#100967=CARTESIAN_POINT('Ctrl Pts',(3.66007952356776,74.4101195539797,12.));
#100968=CARTESIAN_POINT('Ctrl Pts',(3.8484028241923,74.3352361483148,-5.55111512312578E-16));
#100969=CARTESIAN_POINT('Ctrl Pts',(3.8484028241923,74.3352361483148,4.));
#100970=CARTESIAN_POINT('Ctrl Pts',(3.84840282419229,74.3352361483148,7.99999999999999));
#100971=CARTESIAN_POINT('Ctrl Pts',(3.84840282419229,74.3352361483148,12.));
#100972=CARTESIAN_POINT('Ctrl Pts',(3.96302207561147,74.1732860426647,-5.55111512312578E-16));
#100973=CARTESIAN_POINT('Ctrl Pts',(3.96302207561147,74.1732860426647,4.));
#100974=CARTESIAN_POINT('Ctrl Pts',(3.96302207561146,74.1732860426647,8.00000000000001));
#100975=CARTESIAN_POINT('Ctrl Pts',(3.96302207561146,74.1732860426647,12.));
#100976=CARTESIAN_POINT('Ctrl Pts',(3.99277406492175,74.0964320765798,-5.55111512312578E-16));
#100977=CARTESIAN_POINT('Ctrl Pts',(3.99277406492175,74.0964320765798,4.));
#100978=CARTESIAN_POINT('Ctrl Pts',(3.99277406492174,74.0964320765798,8.));
#100979=CARTESIAN_POINT('Ctrl Pts',(3.99277406492174,74.0964320765798,12.));
#100980=CARTESIAN_POINT('',(3.55032190142515,74.4153560389001,0.));
#100981=CARTESIAN_POINT('',(3.99277406492179,74.0964320765798,0.));
#100982=CARTESIAN_POINT('Ctrl Pts',(3.55032190142515,74.4153560389001,0.));
#100983=CARTESIAN_POINT('Ctrl Pts',(3.66007952356777,74.4101195539797,-1.54074395550979E-31));
#100984=CARTESIAN_POINT('Ctrl Pts',(3.76769283821036,74.3673290364569,1.54074395550979E-31));
#100985=CARTESIAN_POINT('Ctrl Pts',(3.85123952454099,74.2961085760818,7.70371977754893E-32));
#100986=CARTESIAN_POINT('Ctrl Pts',(3.91389953928897,74.2426932308005,-7.70371977754894E-32));
#100987=CARTESIAN_POINT('Ctrl Pts',(3.96302207561147,74.1732860426647,-5.39260384428426E-31));
#100988=CARTESIAN_POINT('Ctrl Pts',(3.99277406492175,74.0964320765798,-7.70371977754895E-32));
#100989=CARTESIAN_POINT('',(3.99277406492179,74.0964320765798,12.));
#100990=CARTESIAN_POINT('Ctrl Pts',(3.99277406492175,74.0964320765798,-5.55111512312578E-16));
#100991=CARTESIAN_POINT('Ctrl Pts',(3.99277406492175,74.0964320765798,4.));
#100992=CARTESIAN_POINT('Ctrl Pts',(3.99277406492174,74.0964320765798,8.));
#100993=CARTESIAN_POINT('Ctrl Pts',(3.99277406492174,74.0964320765798,12.));
#100994=CARTESIAN_POINT('',(3.55032190142515,74.4153560389001,12.));
#100995=CARTESIAN_POINT('Ctrl Pts',(3.99277406492174,74.0964320765798,12.));
#100996=CARTESIAN_POINT('Ctrl Pts',(3.96302207561146,74.1732860426647,12.));
#100997=CARTESIAN_POINT('Ctrl Pts',(3.91389953928896,74.2426932308005,12.));
#100998=CARTESIAN_POINT('Ctrl Pts',(3.85123952454098,74.2961085760818,12.));
#100999=CARTESIAN_POINT('Ctrl Pts',(3.76769283821035,74.3673290364569,12.));
#101000=CARTESIAN_POINT('Ctrl Pts',(3.66007952356776,74.4101195539797,12.));
#101001=CARTESIAN_POINT('Ctrl Pts',(3.55032190142515,74.4153560389001,12.));
#101002=CARTESIAN_POINT('Ctrl Pts',(3.55032190142515,74.4153560389001,12.));
#101003=CARTESIAN_POINT('Ctrl Pts',(3.55032190142515,74.4153560389001,8.));
#101004=CARTESIAN_POINT('Ctrl Pts',(3.55032190142515,74.4153560389001,4.));
#101005=CARTESIAN_POINT('Ctrl Pts',(3.55032190142515,74.4153560389001,-5.55111512312578E-16));
#101006=CARTESIAN_POINT('Ctrl Pts',(5.24987136994593,69.8028570375097,0.));
#101007=CARTESIAN_POINT('Ctrl Pts',(5.24987136994593,69.8028570375097,12.));
#101008=CARTESIAN_POINT('Ctrl Pts',(5.24915955997427,69.8066748687772,0.));
#101009=CARTESIAN_POINT('Ctrl Pts',(5.24915955997427,69.8066748687772,12.));
#101010=CARTESIAN_POINT('Ctrl Pts',(5.24773285666377,69.8143154684204,0.));
#101011=CARTESIAN_POINT('Ctrl Pts',(5.24773285666377,69.8143154684204,12.));
#101012=CARTESIAN_POINT('Ctrl Pts',(5.24558355159751,69.8257911792159,0.));
#101013=CARTESIAN_POINT('Ctrl Pts',(5.24558355159751,69.8257911792159,12.));
#101014=CARTESIAN_POINT('Ctrl Pts',(5.2426993105457,69.841121750752,0.));
#101015=CARTESIAN_POINT('Ctrl Pts',(5.2426993105457,69.841121750752,12.));
#101016=CARTESIAN_POINT('Ctrl Pts',(5.23906316634803,69.8603343302743,0.));
#101017=CARTESIAN_POINT('Ctrl Pts',(5.23906316634803,69.8603343302743,12.));
#101018=CARTESIAN_POINT('Ctrl Pts',(5.23539616279621,69.8795962381599,0.));
#101019=CARTESIAN_POINT('Ctrl Pts',(5.23539616279621,69.8795962381599,12.));
#101020=CARTESIAN_POINT('Ctrl Pts',(5.23169827290556,69.8989073936688,0.));
#101021=CARTESIAN_POINT('Ctrl Pts',(5.23169827290556,69.8989073936688,12.));
#101022=CARTESIAN_POINT('Ctrl Pts',(5.22796945602795,69.9182676502048,0.));
#101023=CARTESIAN_POINT('Ctrl Pts',(5.22796945602795,69.9182676502048,12.));
#101024=CARTESIAN_POINT('Ctrl Pts',(5.22420965879982,69.9376767969095,0.));
#101025=CARTESIAN_POINT('Ctrl Pts',(5.22420965879982,69.9376767969095,12.));
#101026=CARTESIAN_POINT('Ctrl Pts',(5.22041882075722,69.9571345870076,0.));
#101027=CARTESIAN_POINT('Ctrl Pts',(5.22041882075722,69.9571345870076,12.));
#101028=CARTESIAN_POINT('Ctrl Pts',(5.2165968788114,69.9766407595385,0.));
#101029=CARTESIAN_POINT('Ctrl Pts',(5.2165968788114,69.9766407595385,12.));
#101030=CARTESIAN_POINT('Ctrl Pts',(5.2127437720326,69.9961950629965,0.));
#101031=CARTESIAN_POINT('Ctrl Pts',(5.2127437720326,69.9961950629965,12.));
#101032=CARTESIAN_POINT('Ctrl Pts',(5.20885944672837,70.0157972802182,0.));
#101033=CARTESIAN_POINT('Ctrl Pts',(5.20885944672837,70.0157972802182,12.));
#101034=CARTESIAN_POINT('Ctrl Pts',(5.20494385478026,70.0354472203546,0.));
#101035=CARTESIAN_POINT('Ctrl Pts',(5.20494385478026,70.0354472203546,12.));
#101036=CARTESIAN_POINT('Ctrl Pts',(5.20099695122657,70.0551447071082,0.));
#101037=CARTESIAN_POINT('Ctrl Pts',(5.20099695122657,70.0551447071082,12.));
#101038=CARTESIAN_POINT('Ctrl Pts',(5.19701869225529,70.0748895689729,0.));
#101039=CARTESIAN_POINT('Ctrl Pts',(5.19701869225529,70.0748895689729,12.));
#101040=CARTESIAN_POINT('Ctrl Pts',(5.19300903271581,70.0946816270997,0.));
#101041=CARTESIAN_POINT('Ctrl Pts',(5.19300903271581,70.0946816270997,12.));
#101042=CARTESIAN_POINT('Ctrl Pts',(5.18896792486566,70.1145206891885,0.));
#101043=CARTESIAN_POINT('Ctrl Pts',(5.18896792486566,70.1145206891885,12.));
#101044=CARTESIAN_POINT('Ctrl Pts',(5.18489531966266,70.1344065558145,0.));
#101045=CARTESIAN_POINT('Ctrl Pts',(5.18489531966266,70.1344065558145,12.));
#101046=CARTESIAN_POINT('Ctrl Pts',(5.18079116757667,70.1543390243892,0.));
#101047=CARTESIAN_POINT('Ctrl Pts',(5.18079116757667,70.1543390243892,12.));
#101048=CARTESIAN_POINT('Ctrl Pts',(5.17665541952384,70.1743178937077,0.));
#101049=CARTESIAN_POINT('Ctrl Pts',(5.17665541952384,70.1743178937077,12.));
#101050=CARTESIAN_POINT('Ctrl Pts',(5.1724880279339,70.1943429691167,0.));
#101051=CARTESIAN_POINT('Ctrl Pts',(5.1724880279339,70.1943429691167,12.));
#101052=CARTESIAN_POINT('Ctrl Pts',(5.16828894670109,70.2144140622953,0.));
#101053=CARTESIAN_POINT('Ctrl Pts',(5.16828894670109,70.2144140622953,12.));
#101054=CARTESIAN_POINT('Ctrl Pts',(5.16405813066977,70.2345309887833,0.));
#101055=CARTESIAN_POINT('Ctrl Pts',(5.16405813066977,70.2345309887833,12.));
#101056=CARTESIAN_POINT('Ctrl Pts',(5.15979553528204,70.2546935662722,0.));
#101057=CARTESIAN_POINT('Ctrl Pts',(5.15979553528204,70.2546935662722,12.));
#101058=CARTESIAN_POINT('Ctrl Pts',(5.1555011161486,70.2749016125105,0.));
#101059=CARTESIAN_POINT('Ctrl Pts',(5.1555011161486,70.2749016125105,12.));
#101060=CARTESIAN_POINT('Ctrl Pts',(5.15117482869255,70.2951549435512,0.));
#101061=CARTESIAN_POINT('Ctrl Pts',(5.15117482869255,70.2951549435512,12.));
#101062=CARTESIAN_POINT('Ctrl Pts',(5.14681662833081,70.3154533746736,0.));
#101063=CARTESIAN_POINT('Ctrl Pts',(5.14681662833081,70.3154533746736,12.));
#101064=CARTESIAN_POINT('Ctrl Pts',(5.1424264706348,70.3357967211796,0.));
#101065=CARTESIAN_POINT('Ctrl Pts',(5.1424264706348,70.3357967211796,12.));
#101066=CARTESIAN_POINT('Ctrl Pts',(5.13800431148904,70.3561847991714,0.));
#101067=CARTESIAN_POINT('Ctrl Pts',(5.13800431148904,70.3561847991714,12.));
#101068=CARTESIAN_POINT('Ctrl Pts',(5.13355010728568,70.3766174264757,0.));
#101069=CARTESIAN_POINT('Ctrl Pts',(5.13355010728568,70.3766174264757,12.));
#101070=CARTESIAN_POINT('Ctrl Pts',(5.12906381499457,70.3970944229851,0.));
#101071=CARTESIAN_POINT('Ctrl Pts',(5.12906381499457,70.3970944229851,12.));
#101072=CARTESIAN_POINT('Ctrl Pts',(5.12454539205329,70.417615610161,0.));
#101073=CARTESIAN_POINT('Ctrl Pts',(5.12454539205329,70.417615610161,12.));
#101074=CARTESIAN_POINT('Ctrl Pts',(5.11999479630212,70.4381808107245,0.));
#101075=CARTESIAN_POINT('Ctrl Pts',(5.11999479630212,70.4381808107245,12.));
#101076=CARTESIAN_POINT('Ctrl Pts',(5.11541198590933,70.458789848296,0.));
#101077=CARTESIAN_POINT('Ctrl Pts',(5.11541198590933,70.458789848296,12.));
#101078=CARTESIAN_POINT('Ctrl Pts',(5.11079691929214,70.4794425469825,0.));
#101079=CARTESIAN_POINT('Ctrl Pts',(5.11079691929214,70.4794425469825,12.));
#101080=CARTESIAN_POINT('Ctrl Pts',(5.10614955511665,70.500138731399,0.));
#101081=CARTESIAN_POINT('Ctrl Pts',(5.10614955511665,70.500138731399,12.));
#101082=CARTESIAN_POINT('Ctrl Pts',(5.10146985232942,70.5208782268497,0.));
#101083=CARTESIAN_POINT('Ctrl Pts',(5.10146985232942,70.5208782268497,12.));
#101084=CARTESIAN_POINT('Ctrl Pts',(5.09675777018184,70.5416608594526,0.));
#101085=CARTESIAN_POINT('Ctrl Pts',(5.09675777018184,70.5416608594526,12.));
#101086=CARTESIAN_POINT('Ctrl Pts',(5.09201326826135,70.5624864562824,0.));
#101087=CARTESIAN_POINT('Ctrl Pts',(5.09201326826135,70.5624864562824,12.));
#101088=CARTESIAN_POINT('Ctrl Pts',(5.08723630652274,70.5833548455014,0.));
#101089=CARTESIAN_POINT('Ctrl Pts',(5.08723630652274,70.5833548455014,12.));
#101090=CARTESIAN_POINT('Ctrl Pts',(5.08242684526687,70.6042658562923,0.));
#101091=CARTESIAN_POINT('Ctrl Pts',(5.08242684526687,70.6042658562923,12.));
#101092=CARTESIAN_POINT('Ctrl Pts',(5.07758484512303,70.6252193187878,0.));
#101093=CARTESIAN_POINT('Ctrl Pts',(5.07758484512303,70.6252193187878,12.));
#101094=CARTESIAN_POINT('Ctrl Pts',(5.07271026703356,70.6462150640015,0.));
#101095=CARTESIAN_POINT('Ctrl Pts',(5.07271026703356,70.6462150640015,12.));
#101096=CARTESIAN_POINT('Ctrl Pts',(5.06780307224073,70.6672529237455,0.));
#101097=CARTESIAN_POINT('Ctrl Pts',(5.06780307224073,70.6672529237455,12.));
#101098=CARTESIAN_POINT('Ctrl Pts',(5.06286322227821,70.6883327305784,0.));
#101099=CARTESIAN_POINT('Ctrl Pts',(5.06286322227821,70.6883327305784,12.));
#101100=CARTESIAN_POINT('Ctrl Pts',(5.05789067897058,70.7094543178438,0.));
#101101=CARTESIAN_POINT('Ctrl Pts',(5.05789067897058,70.7094543178438,12.));
#101102=CARTESIAN_POINT('Ctrl Pts',(5.05288540443483,70.7306175196863,0.));
#101103=CARTESIAN_POINT('Ctrl Pts',(5.05288540443483,70.7306175196863,12.));
#101104=CARTESIAN_POINT('Ctrl Pts',(5.04784736108347,70.7518221710706,0.));
#101105=CARTESIAN_POINT('Ctrl Pts',(5.04784736108347,70.7518221710706,12.));
#101106=CARTESIAN_POINT('Ctrl Pts',(5.0427765116335,70.7730681077983,0.));
#101107=CARTESIAN_POINT('Ctrl Pts',(5.0427765116335,70.7730681077983,12.));
#101108=CARTESIAN_POINT('Ctrl Pts',(5.0376728191048,70.7943551665059,0.));
#101109=CARTESIAN_POINT('Ctrl Pts',(5.0376728191048,70.7943551665059,12.));
#101110=CARTESIAN_POINT('Ctrl Pts',(5.03253624680942,70.8156831846488,0.));
#101111=CARTESIAN_POINT('Ctrl Pts',(5.03253624680942,70.8156831846488,12.));
#101112=CARTESIAN_POINT('Ctrl Pts',(5.02736675834694,70.8370520004843,0.));
#101113=CARTESIAN_POINT('Ctrl Pts',(5.02736675834694,70.8370520004843,12.));
#101114=CARTESIAN_POINT('Ctrl Pts',(5.02216431760061,70.8584614530519,0.));
#101115=CARTESIAN_POINT('Ctrl Pts',(5.02216431760061,70.8584614530519,12.));
#101116=CARTESIAN_POINT('Ctrl Pts',(5.01692888873791,70.8799113821452,0.));
#101117=CARTESIAN_POINT('Ctrl Pts',(5.01692888873791,70.8799113821452,12.));
#101118=CARTESIAN_POINT('Ctrl Pts',(5.01166043620568,70.9014016283124,0.));
#101119=CARTESIAN_POINT('Ctrl Pts',(5.01166043620568,70.9014016283124,12.));
#101120=CARTESIAN_POINT('Ctrl Pts',(5.00635892472514,70.9229320328589,0.));
#101121=CARTESIAN_POINT('Ctrl Pts',(5.00635892472514,70.9229320328589,12.));
#101122=CARTESIAN_POINT('Ctrl Pts',(5.0010243192904,70.9445024378439,0.));
#101123=CARTESIAN_POINT('Ctrl Pts',(5.0010243192904,70.9445024378439,12.));
#101124=CARTESIAN_POINT('Ctrl Pts',(4.99565658516914,70.9661126860773,0.));
#101125=CARTESIAN_POINT('Ctrl Pts',(4.99565658516914,70.9661126860773,12.));
#101126=CARTESIAN_POINT('Ctrl Pts',(4.99025568790665,70.9877626211113,0.));
#101127=CARTESIAN_POINT('Ctrl Pts',(4.99025568790665,70.9877626211113,12.));
#101128=CARTESIAN_POINT('Ctrl Pts',(4.98482159331864,71.0094520872377,0.));
#101129=CARTESIAN_POINT('Ctrl Pts',(4.98482159331864,71.0094520872377,12.));
#101130=CARTESIAN_POINT('Ctrl Pts',(4.97935426748585,71.0311809294821,0.));
#101131=CARTESIAN_POINT('Ctrl Pts',(4.97935426748585,71.0311809294821,12.));
#101132=CARTESIAN_POINT('Ctrl Pts',(4.97385367675159,71.0529489935961,0.));
#101133=CARTESIAN_POINT('Ctrl Pts',(4.97385367675159,71.0529489935961,12.));
#101134=CARTESIAN_POINT('Ctrl Pts',(4.96831978772191,71.0747561260436,0.));
#101135=CARTESIAN_POINT('Ctrl Pts',(4.96831978772191,71.0747561260436,12.));
#101136=CARTESIAN_POINT('Ctrl Pts',(4.96275256726767,71.0966021739907,0.));
#101137=CARTESIAN_POINT('Ctrl Pts',(4.96275256726767,71.0966021739907,12.));
#101138=CARTESIAN_POINT('Ctrl Pts',(4.95715198251685,71.1184869853056,0.));
#101139=CARTESIAN_POINT('Ctrl Pts',(4.95715198251685,71.1184869853056,12.));
#101140=CARTESIAN_POINT('Ctrl Pts',(4.95151800085102,71.1404104085552,0.));
#101141=CARTESIAN_POINT('Ctrl Pts',(4.95151800085102,71.1404104085552,12.));
#101142=CARTESIAN_POINT('Ctrl Pts',(4.94585058990342,71.1623722930001,0.));
#101143=CARTESIAN_POINT('Ctrl Pts',(4.94585058990342,71.1623722930001,12.));
#101144=CARTESIAN_POINT('Ctrl Pts',(4.94014971756115,71.1843724885847,0.));
#101145=CARTESIAN_POINT('Ctrl Pts',(4.94014971756115,71.1843724885847,12.));
#101146=CARTESIAN_POINT('Ctrl Pts',(4.93441535196618,71.2064108459286,0.));
#101147=CARTESIAN_POINT('Ctrl Pts',(4.93441535196618,71.2064108459286,12.));
#101148=CARTESIAN_POINT('Ctrl Pts',(4.92864746150733,71.2284872163273,0.));
#101149=CARTESIAN_POINT('Ctrl Pts',(4.92864746150733,71.2284872163273,12.));
#101150=CARTESIAN_POINT('Ctrl Pts',(4.92284601481722,71.250601451747,0.));
#101151=CARTESIAN_POINT('Ctrl Pts',(4.92284601481722,71.250601451747,12.));
#101152=CARTESIAN_POINT('Ctrl Pts',(4.91701098077037,71.2727534048192,0.));
#101153=CARTESIAN_POINT('Ctrl Pts',(4.91701098077037,71.2727534048192,12.));
#101154=CARTESIAN_POINT('Ctrl Pts',(4.91114232848604,71.294942928829,0.));
#101155=CARTESIAN_POINT('Ctrl Pts',(4.91114232848604,71.294942928829,12.));
#101156=CARTESIAN_POINT('Ctrl Pts',(4.9052400273278,71.3171698777084,0.));
#101157=CARTESIAN_POINT('Ctrl Pts',(4.9052400273278,71.3171698777084,12.));
#101158=CARTESIAN_POINT('Ctrl Pts',(4.89930404689576,71.3394341060359,0.));
#101159=CARTESIAN_POINT('Ctrl Pts',(4.89930404689576,71.3394341060359,12.));
#101160=CARTESIAN_POINT('Ctrl Pts',(4.89333435702414,71.3617354690325,0.));
#101161=CARTESIAN_POINT('Ctrl Pts',(4.89333435702414,71.3617354690325,12.));
#101162=CARTESIAN_POINT('Ctrl Pts',(4.88733092777976,71.3840738225562,0.));
#101163=CARTESIAN_POINT('Ctrl Pts',(4.88733092777976,71.3840738225562,12.));
#101164=CARTESIAN_POINT('Ctrl Pts',(4.88129372946552,71.4064490230899,0.));
#101165=CARTESIAN_POINT('Ctrl Pts',(4.88129372946552,71.4064490230899,12.));
#101166=CARTESIAN_POINT('Ctrl Pts',(4.87522273261908,71.4288609277374,0.));
#101167=CARTESIAN_POINT('Ctrl Pts',(4.87522273261908,71.4288609277374,12.));
#101168=CARTESIAN_POINT('Ctrl Pts',(4.86911790800551,71.4513093942255,0.));
#101169=CARTESIAN_POINT('Ctrl Pts',(4.86911790800551,71.4513093942255,12.));
#101170=CARTESIAN_POINT('Ctrl Pts',(4.86297922661503,71.4737942808982,0.));
#101171=CARTESIAN_POINT('Ctrl Pts',(4.86297922661503,71.4737942808982,12.));
#101172=CARTESIAN_POINT('Ctrl Pts',(4.85680665966181,71.4963154467113,0.));
#101173=CARTESIAN_POINT('Ctrl Pts',(4.85680665966181,71.4963154467113,12.));
#101174=CARTESIAN_POINT('Ctrl Pts',(4.85060017858781,71.5188727512197,0.));
#101175=CARTESIAN_POINT('Ctrl Pts',(4.85060017858781,71.5188727512197,12.));
#101176=CARTESIAN_POINT('Ctrl Pts',(4.84435975506049,71.5414660545739,0.));
#101177=CARTESIAN_POINT('Ctrl Pts',(4.84435975506049,71.5414660545739,12.));
#101178=CARTESIAN_POINT('Ctrl Pts',(4.83808536096584,71.564095217521,0.));
#101179=CARTESIAN_POINT('Ctrl Pts',(4.83808536096584,71.564095217521,12.));
#101180=CARTESIAN_POINT('Ctrl Pts',(4.83177696840638,71.5867601014,0.));
#101181=CARTESIAN_POINT('Ctrl Pts',(4.83177696840638,71.5867601014,12.));
#101182=CARTESIAN_POINT('Ctrl Pts',(4.82543454970027,71.6094605681366,0.));
#101183=CARTESIAN_POINT('Ctrl Pts',(4.82543454970027,71.6094605681366,12.));
#101184=CARTESIAN_POINT('Ctrl Pts',(4.81905807738558,71.6321964802326,0.));
#101185=CARTESIAN_POINT('Ctrl Pts',(4.81905807738558,71.6321964802326,12.));
#101186=CARTESIAN_POINT('Ctrl Pts',(4.81264752421732,71.6549677007613,0.));
#101187=CARTESIAN_POINT('Ctrl Pts',(4.81264752421732,71.6549677007613,12.));
#101188=CARTESIAN_POINT('Ctrl Pts',(4.80620286316089,71.6777740933705,0.));
#101189=CARTESIAN_POINT('Ctrl Pts',(4.80620286316089,71.6777740933705,12.));
#101190=CARTESIAN_POINT('Ctrl Pts',(4.79972406739015,71.7006155222766,0.));
#101191=CARTESIAN_POINT('Ctrl Pts',(4.79972406739015,71.7006155222766,12.));
#101192=CARTESIAN_POINT('Ctrl Pts',(4.79321111028673,71.7234918522604,0.));
#101193=CARTESIAN_POINT('Ctrl Pts',(4.79321111028673,71.7234918522604,12.));
#101194=CARTESIAN_POINT('Ctrl Pts',(4.78666396544451,71.7464029486552,0.));
#101195=CARTESIAN_POINT('Ctrl Pts',(4.78666396544451,71.7464029486552,12.));
#101196=CARTESIAN_POINT('Ctrl Pts',(4.78008260666643,71.7693486773449,0.));
#101197=CARTESIAN_POINT('Ctrl Pts',(4.78008260666643,71.7693486773449,12.));
#101198=CARTESIAN_POINT('Ctrl Pts',(4.77346700795788,71.7923289047636,0.));
#101199=CARTESIAN_POINT('Ctrl Pts',(4.77346700795788,71.7923289047636,12.));
#101200=CARTESIAN_POINT('Ctrl Pts',(4.76681714352504,71.8153434978924,0.));
#101201=CARTESIAN_POINT('Ctrl Pts',(4.76681714352504,71.8153434978924,12.));
#101202=CARTESIAN_POINT('Ctrl Pts',(4.76013298777423,71.8383923242533,0.));
#101203=CARTESIAN_POINT('Ctrl Pts',(4.76013298777423,71.8383923242533,12.));
#101204=CARTESIAN_POINT('Ctrl Pts',(4.75341451531672,71.8614752519008,0.));
#101205=CARTESIAN_POINT('Ctrl Pts',(4.75341451531672,71.8614752519008,12.));
#101206=CARTESIAN_POINT('Ctrl Pts',(4.74666170096546,71.8845921494186,0.));
#101207=CARTESIAN_POINT('Ctrl Pts',(4.74666170096546,71.8845921494186,12.));
#101208=CARTESIAN_POINT('Ctrl Pts',(4.73987451972861,71.9077428859207,0.));
#101209=CARTESIAN_POINT('Ctrl Pts',(4.73987451972861,71.9077428859207,12.));
#101210=CARTESIAN_POINT('Ctrl Pts',(4.73305294680784,71.9309273310469,0.));
#101211=CARTESIAN_POINT('Ctrl Pts',(4.73305294680784,71.9309273310469,12.));
#101212=CARTESIAN_POINT('Ctrl Pts',(4.72619695759779,71.9541453549582,0.));
#101213=CARTESIAN_POINT('Ctrl Pts',(4.72619695759779,71.9541453549582,12.));
#101214=CARTESIAN_POINT('Ctrl Pts',(4.71930652769081,71.9773968283267,0.));
#101215=CARTESIAN_POINT('Ctrl Pts',(4.71930652769081,71.9773968283267,12.));
#101216=CARTESIAN_POINT('Ctrl Pts',(4.71238163287411,72.0006816223335,0.));
#101217=CARTESIAN_POINT('Ctrl Pts',(4.71238163287411,72.0006816223335,12.));
#101218=CARTESIAN_POINT('Ctrl Pts',(4.70542224912313,72.0239996086694,0.));
#101219=CARTESIAN_POINT('Ctrl Pts',(4.70542224912313,72.0239996086694,12.));
#101220=CARTESIAN_POINT('Ctrl Pts',(4.69842835259998,72.047350659532,0.));
#101221=CARTESIAN_POINT('Ctrl Pts',(4.69842835259998,72.047350659532,12.));
#101222=CARTESIAN_POINT('Ctrl Pts',(4.69139991965281,72.070734647621,0.));
#101223=CARTESIAN_POINT('Ctrl Pts',(4.69139991965281,72.070734647621,12.));
#101224=CARTESIAN_POINT('Ctrl Pts',(4.68433692682061,72.0941514461283,0.));
#101225=CARTESIAN_POINT('Ctrl Pts',(4.68433692682061,72.0941514461283,12.));
#101226=CARTESIAN_POINT('Ctrl Pts',(4.67723935083088,72.1176009287349,0.));
#101227=CARTESIAN_POINT('Ctrl Pts',(4.67723935083088,72.1176009287349,12.));
#101228=CARTESIAN_POINT('Ctrl Pts',(4.67010716859282,72.1410829696129,0.));
#101229=CARTESIAN_POINT('Ctrl Pts',(4.67010716859282,72.1410829696129,12.));
#101230=CARTESIAN_POINT('Ctrl Pts',(4.66294035719571,72.1645974434218,0.));
#101231=CARTESIAN_POINT('Ctrl Pts',(4.66294035719571,72.1645974434218,12.));
#101232=CARTESIAN_POINT('Ctrl Pts',(4.65573889390825,72.1881442253052,0.));
#101233=CARTESIAN_POINT('Ctrl Pts',(4.65573889390825,72.1881442253052,12.));
#101234=CARTESIAN_POINT('Ctrl Pts',(4.64850275618326,72.2117231908816,0.));
#101235=CARTESIAN_POINT('Ctrl Pts',(4.64850275618326,72.2117231908816,12.));
#101236=CARTESIAN_POINT('Ctrl Pts',(4.64123192165628,72.2353342162408,0.));
#101237=CARTESIAN_POINT('Ctrl Pts',(4.64123192165628,72.2353342162408,12.));
#101238=CARTESIAN_POINT('Ctrl Pts',(4.63392636813843,72.2589771779447,0.));
#101239=CARTESIAN_POINT('Ctrl Pts',(4.63392636813843,72.2589771779447,12.));
#101240=CARTESIAN_POINT('Ctrl Pts',(4.62658607361466,72.2826519530254,0.));
#101241=CARTESIAN_POINT('Ctrl Pts',(4.62658607361466,72.2826519530254,12.));
#101242=CARTESIAN_POINT('Ctrl Pts',(4.61921101624295,72.306358418981,0.));
#101243=CARTESIAN_POINT('Ctrl Pts',(4.61921101624295,72.306358418981,12.));
#101244=CARTESIAN_POINT('Ctrl Pts',(4.61180117435869,72.330096453767,0.));
#101245=CARTESIAN_POINT('Ctrl Pts',(4.61180117435869,72.330096453767,12.));
#101246=CARTESIAN_POINT('Ctrl Pts',(4.60435652647464,72.3538659357932,0.));
#101247=CARTESIAN_POINT('Ctrl Pts',(4.60435652647464,72.3538659357932,12.));
#101248=CARTESIAN_POINT('Ctrl Pts',(4.59687705127341,72.3776667439244,0.));
#101249=CARTESIAN_POINT('Ctrl Pts',(4.59687705127341,72.3776667439244,12.));
#101250=CARTESIAN_POINT('Ctrl Pts',(4.58936272760551,72.4014987574789,0.));
#101251=CARTESIAN_POINT('Ctrl Pts',(4.58936272760551,72.4014987574789,12.));
#101252=CARTESIAN_POINT('Ctrl Pts',(4.58181353448852,72.4253618562249,0.));
#101253=CARTESIAN_POINT('Ctrl Pts',(4.58181353448852,72.4253618562249,12.));
#101254=CARTESIAN_POINT('Ctrl Pts',(4.57422945111095,72.449255920373,0.));
#101255=CARTESIAN_POINT('Ctrl Pts',(4.57422945111095,72.449255920373,12.));
#101256=CARTESIAN_POINT('Ctrl Pts',(4.56661045683367,72.473180830571,0.));
#101257=CARTESIAN_POINT('Ctrl Pts',(4.56661045683367,72.473180830571,12.));
#101258=CARTESIAN_POINT('Ctrl Pts',(4.55895653118214,72.4971364679055,0.));
#101259=CARTESIAN_POINT('Ctrl Pts',(4.55895653118214,72.4971364679055,12.));
#101260=CARTESIAN_POINT('Ctrl Pts',(4.55126765384403,72.5211227138997,0.));
#101261=CARTESIAN_POINT('Ctrl Pts',(4.55126765384403,72.5211227138997,12.));
#101262=CARTESIAN_POINT('Ctrl Pts',(4.54354380466826,72.5451394505106,0.));
#101263=CARTESIAN_POINT('Ctrl Pts',(4.54354380466826,72.5451394505106,12.));
#101264=CARTESIAN_POINT('Ctrl Pts',(4.53578496366802,72.5691865601225,0.));
#101265=CARTESIAN_POINT('Ctrl Pts',(4.53578496366802,72.5691865601225,12.));
#101266=CARTESIAN_POINT('Ctrl Pts',(4.52799111102391,72.5932639255406,0.));
#101267=CARTESIAN_POINT('Ctrl Pts',(4.52799111102391,72.5932639255406,12.));
#101268=CARTESIAN_POINT('Ctrl Pts',(4.52016222707633,72.6173714299935,0.));
#101269=CARTESIAN_POINT('Ctrl Pts',(4.52016222707633,72.6173714299935,12.));
#101270=CARTESIAN_POINT('Ctrl Pts',(4.5122982923226,72.6415089571314,0.));
#101271=CARTESIAN_POINT('Ctrl Pts',(4.5122982923226,72.6415089571314,12.));
#101272=CARTESIAN_POINT('Ctrl Pts',(4.50439928741605,72.6656763910241,0.));
#101273=CARTESIAN_POINT('Ctrl Pts',(4.50439928741605,72.6656763910241,12.));
#101274=CARTESIAN_POINT('Ctrl Pts',(4.49646519316822,72.689873616155,0.));
#101275=CARTESIAN_POINT('Ctrl Pts',(4.49646519316822,72.689873616155,12.));
#101276=CARTESIAN_POINT('Ctrl Pts',(4.48849599055354,72.7141005174153,0.));
#101277=CARTESIAN_POINT('Ctrl Pts',(4.48849599055354,72.7141005174153,12.));
#101278=CARTESIAN_POINT('Ctrl Pts',(4.48049166070224,72.7383569801042,0.));
#101279=CARTESIAN_POINT('Ctrl Pts',(4.48049166070224,72.7383569801042,12.));
#101280=CARTESIAN_POINT('Ctrl Pts',(4.47245218489623,72.7626428899287,0.));
#101281=CARTESIAN_POINT('Ctrl Pts',(4.47245218489623,72.7626428899287,12.));
#101282=CARTESIAN_POINT('Ctrl Pts',(4.46437754456796,72.7869581329994,0.));
#101283=CARTESIAN_POINT('Ctrl Pts',(4.46437754456796,72.7869581329994,12.));
#101284=CARTESIAN_POINT('Ctrl Pts',(4.45626772130139,72.8113025958258,0.));
#101285=CARTESIAN_POINT('Ctrl Pts',(4.45626772130139,72.8113025958258,12.));
#101286=CARTESIAN_POINT('Ctrl Pts',(4.44812269683725,72.8356761653064,0.));
#101287=CARTESIAN_POINT('Ctrl Pts',(4.44812269683725,72.8356761653064,12.));
#101288=CARTESIAN_POINT('Ctrl Pts',(4.43994245306805,72.8600787287316,0.));
#101289=CARTESIAN_POINT('Ctrl Pts',(4.43994245306805,72.8600787287316,12.));
#101290=CARTESIAN_POINT('Ctrl Pts',(4.43172697203342,72.8845101737856,0.));
#101291=CARTESIAN_POINT('Ctrl Pts',(4.43172697203342,72.8845101737856,12.));
#101292=CARTESIAN_POINT('Ctrl Pts',(4.42347623591942,72.9089703885464,0.));
#101293=CARTESIAN_POINT('Ctrl Pts',(4.42347623591942,72.9089703885464,12.));
#101294=CARTESIAN_POINT('Ctrl Pts',(4.41519022705927,72.9334592614828,0.));
#101295=CARTESIAN_POINT('Ctrl Pts',(4.41519022705927,72.9334592614828,12.));
#101296=CARTESIAN_POINT('Ctrl Pts',(4.40686892793966,72.9579766814495,0.));
#101297=CARTESIAN_POINT('Ctrl Pts',(4.40686892793966,72.9579766814495,12.));
#101298=CARTESIAN_POINT('Ctrl Pts',(4.39851232119731,72.9825225376839,0.));
#101299=CARTESIAN_POINT('Ctrl Pts',(4.39851232119731,72.9825225376839,12.));
#101300=CARTESIAN_POINT('Ctrl Pts',(4.39012038961145,73.0070967198033,0.));
#101301=CARTESIAN_POINT('Ctrl Pts',(4.39012038961145,73.0070967198033,12.));
#101302=CARTESIAN_POINT('Ctrl Pts',(4.38169311610154,73.031699117799,0.));
#101303=CARTESIAN_POINT('Ctrl Pts',(4.38169311610154,73.031699117799,12.));
#101304=CARTESIAN_POINT('Ctrl Pts',(4.37323048372607,73.0563296220301,0.));
#101305=CARTESIAN_POINT('Ctrl Pts',(4.37323048372607,73.0563296220301,12.));
#101306=CARTESIAN_POINT('Ctrl Pts',(4.36473247568639,73.0809881232111,0.));
#101307=CARTESIAN_POINT('Ctrl Pts',(4.36473247568639,73.0809881232111,12.));
#101308=CARTESIAN_POINT('Ctrl Pts',(4.35619907532716,73.1056745124099,0.));
#101309=CARTESIAN_POINT('Ctrl Pts',(4.35619907532716,73.1056745124099,12.));
#101310=CARTESIAN_POINT('Ctrl Pts',(4.34763026613155,73.1303886810602,0.));
#101311=CARTESIAN_POINT('Ctrl Pts',(4.34763026613155,73.1303886810602,12.));
#101312=CARTESIAN_POINT('Ctrl Pts',(4.3390260317214,73.1551305209692,0.));
#101313=CARTESIAN_POINT('Ctrl Pts',(4.3390260317214,73.1551305209692,12.));
#101314=CARTESIAN_POINT('Ctrl Pts',(4.33038635585878,73.1798999243234,0.));
#101315=CARTESIAN_POINT('Ctrl Pts',(4.33038635585878,73.1798999243234,12.));
#101316=CARTESIAN_POINT('Ctrl Pts',(4.32171122245219,73.204696783693,0.));
#101317=CARTESIAN_POINT('Ctrl Pts',(4.32171122245219,73.204696783693,12.));
#101318=CARTESIAN_POINT('Ctrl Pts',(4.31300061556103,73.2295209920319,0.));
#101319=CARTESIAN_POINT('Ctrl Pts',(4.31300061556103,73.2295209920319,12.));
#101320=CARTESIAN_POINT('Ctrl Pts',(4.30425451938235,73.2543724426562,0.));
#101321=CARTESIAN_POINT('Ctrl Pts',(4.30425451938235,73.2543724426562,12.));
#101322=CARTESIAN_POINT('Ctrl Pts',(4.29547291824289,73.2792510292243,0.));
#101323=CARTESIAN_POINT('Ctrl Pts',(4.29547291824289,73.2792510292243,12.));
#101324=CARTESIAN_POINT('Ctrl Pts',(4.28665579659303,73.3041566457134,0.));
#101325=CARTESIAN_POINT('Ctrl Pts',(4.28665579659303,73.3041566457134,12.));
#101326=CARTESIAN_POINT('Ctrl Pts',(4.27780313900392,73.3290891863959,0.));
#101327=CARTESIAN_POINT('Ctrl Pts',(4.27780313900392,73.3290891863959,12.));
#101328=CARTESIAN_POINT('Ctrl Pts',(4.26891493016704,73.354048545808,0.));
#101329=CARTESIAN_POINT('Ctrl Pts',(4.26891493016704,73.354048545808,12.));
#101330=CARTESIAN_POINT('Ctrl Pts',(4.25999115489905,73.3790346187953,0.));
#101331=CARTESIAN_POINT('Ctrl Pts',(4.25999115489905,73.3790346187953,12.));
#101332=CARTESIAN_POINT('Ctrl Pts',(4.25103179814892,73.4040473005603,0.));
#101333=CARTESIAN_POINT('Ctrl Pts',(4.25103179814892,73.4040473005603,12.));
#101334=CARTESIAN_POINT('Ctrl Pts',(4.24203684500942,73.4290864867103,0.));
#101335=CARTESIAN_POINT('Ctrl Pts',(4.24203684500942,73.4290864867103,12.));
#101336=CARTESIAN_POINT('Ctrl Pts',(4.23300628072758,73.4541520732943,0.));
#101337=CARTESIAN_POINT('Ctrl Pts',(4.23300628072758,73.4541520732943,12.));
#101338=CARTESIAN_POINT('Ctrl Pts',(4.22394009072754,73.4792439568624,0.));
#101339=CARTESIAN_POINT('Ctrl Pts',(4.22394009072754,73.4792439568624,12.));
#101340=CARTESIAN_POINT('Ctrl Pts',(4.21483826059437,73.5043620344107,0.));
#101341=CARTESIAN_POINT('Ctrl Pts',(4.21483826059437,73.5043620344107,12.));
#101342=CARTESIAN_POINT('Ctrl Pts',(4.20570077603728,73.5295062032621,0.));
#101343=CARTESIAN_POINT('Ctrl Pts',(4.20570077603728,73.5295062032621,12.));
#101344=CARTESIAN_POINT('Ctrl Pts',(4.19652762286127,73.554676360957,0.));
#101345=CARTESIAN_POINT('Ctrl Pts',(4.19652762286127,73.554676360957,12.));
#101346=CARTESIAN_POINT('Ctrl Pts',(4.18731878694239,73.5798724051519,0.));
#101347=CARTESIAN_POINT('Ctrl Pts',(4.18731878694239,73.5798724051519,12.));
#101348=CARTESIAN_POINT('Ctrl Pts',(4.17807425419817,73.6050942334773,0.));
#101349=CARTESIAN_POINT('Ctrl Pts',(4.17807425419817,73.6050942334773,12.));
#101350=CARTESIAN_POINT('Ctrl Pts',(4.16879401058787,73.6303417435262,0.));
#101351=CARTESIAN_POINT('Ctrl Pts',(4.16879401058787,73.6303417435262,12.));
#101352=CARTESIAN_POINT('Ctrl Pts',(4.15947804217791,73.6556148331504,0.));
#101353=CARTESIAN_POINT('Ctrl Pts',(4.15947804217791,73.6556148331504,12.));
#101354=CARTESIAN_POINT('Ctrl Pts',(4.15012633519729,73.6809134006909,0.));
#101355=CARTESIAN_POINT('Ctrl Pts',(4.15012633519729,73.6809134006909,12.));
#101356=CARTESIAN_POINT('Ctrl Pts',(4.14073887610155,73.7062373452344,0.));
#101357=CARTESIAN_POINT('Ctrl Pts',(4.14073887610155,73.7062373452344,12.));
#101358=CARTESIAN_POINT('Ctrl Pts',(4.13131565163575,73.7315865668508,0.));
#101359=CARTESIAN_POINT('Ctrl Pts',(4.13131565163575,73.7315865668508,12.));
#101360=CARTESIAN_POINT('Ctrl Pts',(4.12185664890552,73.7569609668501,0.));
#101361=CARTESIAN_POINT('Ctrl Pts',(4.12185664890552,73.7569609668501,12.));
#101362=CARTESIAN_POINT('Ctrl Pts',(4.11236185522781,73.7823604472126,0.));
#101363=CARTESIAN_POINT('Ctrl Pts',(4.11236185522781,73.7823604472126,12.));
#101364=CARTESIAN_POINT('Ctrl Pts',(4.10283125798725,73.8077849100314,0.));
#101365=CARTESIAN_POINT('Ctrl Pts',(4.10283125798725,73.8077849100314,12.));
#101366=CARTESIAN_POINT('Ctrl Pts',(4.09326484448232,73.8332342568978,0.));
#101367=CARTESIAN_POINT('Ctrl Pts',(4.09326484448232,73.8332342568978,12.));
#101368=CARTESIAN_POINT('Ctrl Pts',(4.0836626018068,73.8587083884208,0.));
#101369=CARTESIAN_POINT('Ctrl Pts',(4.0836626018068,73.8587083884208,12.));
#101370=CARTESIAN_POINT('Ctrl Pts',(4.07402451665254,73.884207203405,0.));
#101371=CARTESIAN_POINT('Ctrl Pts',(4.07402451665254,73.884207203405,12.));
#101372=CARTESIAN_POINT('Ctrl Pts',(4.06435057547335,73.9097305995173,0.));
#101373=CARTESIAN_POINT('Ctrl Pts',(4.06435057547335,73.9097305995173,12.));
#101374=CARTESIAN_POINT('Ctrl Pts',(4.05464076484762,73.9352784747665,0.));
#101375=CARTESIAN_POINT('Ctrl Pts',(4.05464076484762,73.9352784747665,12.));
#101376=CARTESIAN_POINT('Ctrl Pts',(4.04489507179964,73.9608507287943,0.));
#101377=CARTESIAN_POINT('Ctrl Pts',(4.04489507179964,73.9608507287943,12.));
#101378=CARTESIAN_POINT('Ctrl Pts',(4.03511348410661,73.9864472641025,0.));
#101379=CARTESIAN_POINT('Ctrl Pts',(4.03511348410661,73.9864472641025,12.));
#101380=CARTESIAN_POINT('Ctrl Pts',(4.02529599070086,74.0120679876396,0.));
#101381=CARTESIAN_POINT('Ctrl Pts',(4.02529599070086,74.0120679876396,12.));
#101382=CARTESIAN_POINT('Ctrl Pts',(4.01544258176694,74.0377128111754,0.));
#101383=CARTESIAN_POINT('Ctrl Pts',(4.01544258176694,74.0377128111754,12.));
#101384=CARTESIAN_POINT('Ctrl Pts',(4.0055532478546,74.0633816477912,0.));
#101385=CARTESIAN_POINT('Ctrl Pts',(4.0055532478546,74.0633816477912,12.));
#101386=CARTESIAN_POINT('Ctrl Pts',(3.99562797918272,74.0890744091088,0.));
#101387=CARTESIAN_POINT('Ctrl Pts',(3.99562797918272,74.0890744091088,12.));
#101388=CARTESIAN_POINT('Ctrl Pts',(3.98566676483639,74.1147910020869,0.));
#101389=CARTESIAN_POINT('Ctrl Pts',(3.98566676483639,74.1147910020869,12.));
#101390=CARTESIAN_POINT('Ctrl Pts',(3.97566959209547,74.1405313263198,0.));
#101391=CARTESIAN_POINT('Ctrl Pts',(3.97566959209547,74.1405313263198,12.));
#101392=CARTESIAN_POINT('Ctrl Pts',(3.96563644549423,74.1662952702689,0.));
#101393=CARTESIAN_POINT('Ctrl Pts',(3.96563644549423,74.1662952702689,12.));
#101394=CARTESIAN_POINT('Ctrl Pts',(3.95556730821161,74.1920827166861,0.));
#101395=CARTESIAN_POINT('Ctrl Pts',(3.95556730821161,74.1920827166861,12.));
#101396=CARTESIAN_POINT('Ctrl Pts',(3.94546216377499,74.217893549314,0.));
#101397=CARTESIAN_POINT('Ctrl Pts',(3.94546216377499,74.217893549314,12.));
#101398=CARTESIAN_POINT('Ctrl Pts',(3.9353209977423,74.2437276593763,0.));
#101399=CARTESIAN_POINT('Ctrl Pts',(3.9353209977423,74.2437276593763,12.));
#101400=CARTESIAN_POINT('Ctrl Pts',(3.92514379920729,74.2695849516134,0.));
#101401=CARTESIAN_POINT('Ctrl Pts',(3.92514379920729,74.2695849516134,12.));
#101402=CARTESIAN_POINT('Ctrl Pts',(3.91493056284965,74.2954653518346,0.));
#101403=CARTESIAN_POINT('Ctrl Pts',(3.91493056284965,74.2954653518346,12.));
#101404=CARTESIAN_POINT('Ctrl Pts',(3.90468128904521,74.3213688089495,0.));
#101405=CARTESIAN_POINT('Ctrl Pts',(3.90468128904521,74.3213688089495,12.));
#101406=CARTESIAN_POINT('Ctrl Pts',(3.89439598145194,74.3472952898,0.));
#101407=CARTESIAN_POINT('Ctrl Pts',(3.89439598145194,74.3472952898,12.));
#101408=CARTESIAN_POINT('Ctrl Pts',(3.8861389124787,74.3680548786039,0.));
#101409=CARTESIAN_POINT('Ctrl Pts',(3.8861389124787,74.3680548786039,12.));
#101410=CARTESIAN_POINT('Ctrl Pts',(3.87992989995679,74.3836349188809,0.));
#101411=CARTESIAN_POINT('Ctrl Pts',(3.87992989995679,74.3836349188809,12.));
#101412=CARTESIAN_POINT('Ctrl Pts',(3.87578335377302,74.3940262116251,0.));
#101413=CARTESIAN_POINT('Ctrl Pts',(3.87578335377302,74.3940262116251,12.));
#101414=CARTESIAN_POINT('Ctrl Pts',(3.87370827955545,74.3992230078037,0.));
#101415=CARTESIAN_POINT('Ctrl Pts',(3.87370827955545,74.3992230078037,12.));
#101416=CARTESIAN_POINT('',(5.24987136994593,69.8028570375097,0.));
#101417=CARTESIAN_POINT('Ctrl Pts',(5.24987136994593,69.8028570375097,0.));
#101418=CARTESIAN_POINT('Ctrl Pts',(5.24915955997427,69.8066748687772,0.));
#101419=CARTESIAN_POINT('Ctrl Pts',(5.24773285666377,69.8143154684204,0.));
#101420=CARTESIAN_POINT('Ctrl Pts',(5.24558355159751,69.8257911792159,0.));
#101421=CARTESIAN_POINT('Ctrl Pts',(5.2426993105457,69.841121750752,0.));
#101422=CARTESIAN_POINT('Ctrl Pts',(5.23906316634803,69.8603343302743,0.));
#101423=CARTESIAN_POINT('Ctrl Pts',(5.23539616279621,69.8795962381599,0.));
#101424=CARTESIAN_POINT('Ctrl Pts',(5.23169827290556,69.8989073936688,0.));
#101425=CARTESIAN_POINT('Ctrl Pts',(5.22796945602795,69.9182676502048,0.));
#101426=CARTESIAN_POINT('Ctrl Pts',(5.22420965879982,69.9376767969095,0.));
#101427=CARTESIAN_POINT('Ctrl Pts',(5.22041882075722,69.9571345870076,0.));
#101428=CARTESIAN_POINT('Ctrl Pts',(5.2165968788114,69.9766407595385,0.));
#101429=CARTESIAN_POINT('Ctrl Pts',(5.2127437720326,69.9961950629965,0.));
#101430=CARTESIAN_POINT('Ctrl Pts',(5.20885944672837,70.0157972802182,0.));
#101431=CARTESIAN_POINT('Ctrl Pts',(5.20494385478026,70.0354472203546,0.));
#101432=CARTESIAN_POINT('Ctrl Pts',(5.20099695122657,70.0551447071082,0.));
#101433=CARTESIAN_POINT('Ctrl Pts',(5.19701869225529,70.0748895689729,0.));
#101434=CARTESIAN_POINT('Ctrl Pts',(5.19300903271581,70.0946816270997,0.));
#101435=CARTESIAN_POINT('Ctrl Pts',(5.18896792486566,70.1145206891885,0.));
#101436=CARTESIAN_POINT('Ctrl Pts',(5.18489531966266,70.1344065558145,0.));
#101437=CARTESIAN_POINT('Ctrl Pts',(5.18079116757667,70.1543390243892,0.));
#101438=CARTESIAN_POINT('Ctrl Pts',(5.17665541952384,70.1743178937077,0.));
#101439=CARTESIAN_POINT('Ctrl Pts',(5.1724880279339,70.1943429691167,0.));
#101440=CARTESIAN_POINT('Ctrl Pts',(5.16828894670109,70.2144140622953,0.));
#101441=CARTESIAN_POINT('Ctrl Pts',(5.16405813066977,70.2345309887833,0.));
#101442=CARTESIAN_POINT('Ctrl Pts',(5.15979553528204,70.2546935662722,0.));
#101443=CARTESIAN_POINT('Ctrl Pts',(5.1555011161486,70.2749016125105,0.));
#101444=CARTESIAN_POINT('Ctrl Pts',(5.15117482869255,70.2951549435512,0.));
#101445=CARTESIAN_POINT('Ctrl Pts',(5.14681662833081,70.3154533746736,0.));
#101446=CARTESIAN_POINT('Ctrl Pts',(5.1424264706348,70.3357967211796,0.));
#101447=CARTESIAN_POINT('Ctrl Pts',(5.13800431148904,70.3561847991714,0.));
#101448=CARTESIAN_POINT('Ctrl Pts',(5.13355010728568,70.3766174264757,0.));
#101449=CARTESIAN_POINT('Ctrl Pts',(5.12906381499457,70.3970944229851,0.));
#101450=CARTESIAN_POINT('Ctrl Pts',(5.12454539205329,70.417615610161,0.));
#101451=CARTESIAN_POINT('Ctrl Pts',(5.11999479630212,70.4381808107245,0.));
#101452=CARTESIAN_POINT('Ctrl Pts',(5.11541198590933,70.458789848296,0.));
#101453=CARTESIAN_POINT('Ctrl Pts',(5.11079691929214,70.4794425469825,0.));
#101454=CARTESIAN_POINT('Ctrl Pts',(5.10614955511665,70.500138731399,0.));
#101455=CARTESIAN_POINT('Ctrl Pts',(5.10146985232942,70.5208782268497,0.));
#101456=CARTESIAN_POINT('Ctrl Pts',(5.09675777018184,70.5416608594526,0.));
#101457=CARTESIAN_POINT('Ctrl Pts',(5.09201326826135,70.5624864562824,0.));
#101458=CARTESIAN_POINT('Ctrl Pts',(5.08723630652274,70.5833548455014,0.));
#101459=CARTESIAN_POINT('Ctrl Pts',(5.08242684526687,70.6042658562923,0.));
#101460=CARTESIAN_POINT('Ctrl Pts',(5.07758484512303,70.6252193187878,0.));
#101461=CARTESIAN_POINT('Ctrl Pts',(5.07271026703356,70.6462150640015,0.));
#101462=CARTESIAN_POINT('Ctrl Pts',(5.06780307224073,70.6672529237455,0.));
#101463=CARTESIAN_POINT('Ctrl Pts',(5.06286322227821,70.6883327305784,0.));
#101464=CARTESIAN_POINT('Ctrl Pts',(5.05789067897058,70.7094543178438,0.));
#101465=CARTESIAN_POINT('Ctrl Pts',(5.05288540443483,70.7306175196863,0.));
#101466=CARTESIAN_POINT('Ctrl Pts',(5.04784736108347,70.7518221710706,0.));
#101467=CARTESIAN_POINT('Ctrl Pts',(5.0427765116335,70.7730681077983,0.));
#101468=CARTESIAN_POINT('Ctrl Pts',(5.0376728191048,70.7943551665059,0.));
#101469=CARTESIAN_POINT('Ctrl Pts',(5.03253624680942,70.8156831846488,0.));
#101470=CARTESIAN_POINT('Ctrl Pts',(5.02736675834694,70.8370520004843,0.));
#101471=CARTESIAN_POINT('Ctrl Pts',(5.02216431760061,70.8584614530519,0.));
#101472=CARTESIAN_POINT('Ctrl Pts',(5.01692888873791,70.8799113821452,0.));
#101473=CARTESIAN_POINT('Ctrl Pts',(5.01166043620568,70.9014016283124,0.));
#101474=CARTESIAN_POINT('Ctrl Pts',(5.00635892472514,70.9229320328589,0.));
#101475=CARTESIAN_POINT('Ctrl Pts',(5.0010243192904,70.9445024378439,0.));
#101476=CARTESIAN_POINT('Ctrl Pts',(4.99565658516914,70.9661126860773,0.));
#101477=CARTESIAN_POINT('Ctrl Pts',(4.99025568790665,70.9877626211113,0.));
#101478=CARTESIAN_POINT('Ctrl Pts',(4.98482159331864,71.0094520872377,0.));
#101479=CARTESIAN_POINT('Ctrl Pts',(4.97935426748585,71.0311809294821,0.));
#101480=CARTESIAN_POINT('Ctrl Pts',(4.97385367675159,71.0529489935961,0.));
#101481=CARTESIAN_POINT('Ctrl Pts',(4.96831978772191,71.0747561260436,0.));
#101482=CARTESIAN_POINT('Ctrl Pts',(4.96275256726767,71.0966021739907,0.));
#101483=CARTESIAN_POINT('Ctrl Pts',(4.95715198251685,71.1184869853056,0.));
#101484=CARTESIAN_POINT('Ctrl Pts',(4.95151800085102,71.1404104085552,0.));
#101485=CARTESIAN_POINT('Ctrl Pts',(4.94585058990342,71.1623722930001,0.));
#101486=CARTESIAN_POINT('Ctrl Pts',(4.94014971756115,71.1843724885847,0.));
#101487=CARTESIAN_POINT('Ctrl Pts',(4.93441535196618,71.2064108459286,0.));
#101488=CARTESIAN_POINT('Ctrl Pts',(4.92864746150733,71.2284872163273,0.));
#101489=CARTESIAN_POINT('Ctrl Pts',(4.92284601481722,71.250601451747,0.));
#101490=CARTESIAN_POINT('Ctrl Pts',(4.91701098077037,71.2727534048192,0.));
#101491=CARTESIAN_POINT('Ctrl Pts',(4.91114232848604,71.294942928829,0.));
#101492=CARTESIAN_POINT('Ctrl Pts',(4.9052400273278,71.3171698777084,0.));
#101493=CARTESIAN_POINT('Ctrl Pts',(4.89930404689576,71.3394341060359,0.));
#101494=CARTESIAN_POINT('Ctrl Pts',(4.89333435702414,71.3617354690325,0.));
#101495=CARTESIAN_POINT('Ctrl Pts',(4.88733092777976,71.3840738225562,0.));
#101496=CARTESIAN_POINT('Ctrl Pts',(4.88129372946552,71.4064490230899,0.));
#101497=CARTESIAN_POINT('Ctrl Pts',(4.87522273261908,71.4288609277374,0.));
#101498=CARTESIAN_POINT('Ctrl Pts',(4.86911790800551,71.4513093942255,0.));
#101499=CARTESIAN_POINT('Ctrl Pts',(4.86297922661503,71.4737942808982,0.));
#101500=CARTESIAN_POINT('Ctrl Pts',(4.85680665966181,71.4963154467113,0.));
#101501=CARTESIAN_POINT('Ctrl Pts',(4.85060017858781,71.5188727512197,0.));
#101502=CARTESIAN_POINT('Ctrl Pts',(4.84435975506049,71.5414660545739,0.));
#101503=CARTESIAN_POINT('Ctrl Pts',(4.83808536096584,71.564095217521,0.));
#101504=CARTESIAN_POINT('Ctrl Pts',(4.83177696840638,71.5867601014,0.));
#101505=CARTESIAN_POINT('Ctrl Pts',(4.82543454970027,71.6094605681366,0.));
#101506=CARTESIAN_POINT('Ctrl Pts',(4.81905807738558,71.6321964802326,0.));
#101507=CARTESIAN_POINT('Ctrl Pts',(4.81264752421732,71.6549677007613,0.));
#101508=CARTESIAN_POINT('Ctrl Pts',(4.80620286316089,71.6777740933705,0.));
#101509=CARTESIAN_POINT('Ctrl Pts',(4.79972406739015,71.7006155222766,0.));
#101510=CARTESIAN_POINT('Ctrl Pts',(4.79321111028673,71.7234918522604,0.));
#101511=CARTESIAN_POINT('Ctrl Pts',(4.78666396544451,71.7464029486552,0.));
#101512=CARTESIAN_POINT('Ctrl Pts',(4.78008260666643,71.7693486773449,0.));
#101513=CARTESIAN_POINT('Ctrl Pts',(4.77346700795788,71.7923289047636,0.));
#101514=CARTESIAN_POINT('Ctrl Pts',(4.76681714352504,71.8153434978924,0.));
#101515=CARTESIAN_POINT('Ctrl Pts',(4.76013298777423,71.8383923242533,0.));
#101516=CARTESIAN_POINT('Ctrl Pts',(4.75341451531672,71.8614752519008,0.));
#101517=CARTESIAN_POINT('Ctrl Pts',(4.74666170096546,71.8845921494186,0.));
#101518=CARTESIAN_POINT('Ctrl Pts',(4.73987451972861,71.9077428859207,0.));
#101519=CARTESIAN_POINT('Ctrl Pts',(4.73305294680784,71.9309273310469,0.));
#101520=CARTESIAN_POINT('Ctrl Pts',(4.72619695759779,71.9541453549582,0.));
#101521=CARTESIAN_POINT('Ctrl Pts',(4.71930652769081,71.9773968283267,0.));
#101522=CARTESIAN_POINT('Ctrl Pts',(4.71238163287411,72.0006816223335,0.));
#101523=CARTESIAN_POINT('Ctrl Pts',(4.70542224912313,72.0239996086694,0.));
#101524=CARTESIAN_POINT('Ctrl Pts',(4.69842835259998,72.047350659532,0.));
#101525=CARTESIAN_POINT('Ctrl Pts',(4.69139991965281,72.070734647621,0.));
#101526=CARTESIAN_POINT('Ctrl Pts',(4.68433692682061,72.0941514461283,0.));
#101527=CARTESIAN_POINT('Ctrl Pts',(4.67723935083088,72.1176009287349,0.));
#101528=CARTESIAN_POINT('Ctrl Pts',(4.67010716859282,72.1410829696129,0.));
#101529=CARTESIAN_POINT('Ctrl Pts',(4.66294035719571,72.1645974434218,0.));
#101530=CARTESIAN_POINT('Ctrl Pts',(4.65573889390825,72.1881442253052,0.));
#101531=CARTESIAN_POINT('Ctrl Pts',(4.64850275618326,72.2117231908816,0.));
#101532=CARTESIAN_POINT('Ctrl Pts',(4.64123192165628,72.2353342162408,0.));
#101533=CARTESIAN_POINT('Ctrl Pts',(4.63392636813843,72.2589771779447,0.));
#101534=CARTESIAN_POINT('Ctrl Pts',(4.62658607361466,72.2826519530254,0.));
#101535=CARTESIAN_POINT('Ctrl Pts',(4.61921101624295,72.306358418981,0.));
#101536=CARTESIAN_POINT('Ctrl Pts',(4.61180117435869,72.330096453767,0.));
#101537=CARTESIAN_POINT('Ctrl Pts',(4.60435652647464,72.3538659357932,0.));
#101538=CARTESIAN_POINT('Ctrl Pts',(4.59687705127341,72.3776667439244,0.));
#101539=CARTESIAN_POINT('Ctrl Pts',(4.58936272760551,72.4014987574789,0.));
#101540=CARTESIAN_POINT('Ctrl Pts',(4.58181353448852,72.4253618562249,0.));
#101541=CARTESIAN_POINT('Ctrl Pts',(4.57422945111095,72.449255920373,0.));
#101542=CARTESIAN_POINT('Ctrl Pts',(4.56661045683367,72.473180830571,0.));
#101543=CARTESIAN_POINT('Ctrl Pts',(4.55895653118214,72.4971364679055,0.));
#101544=CARTESIAN_POINT('Ctrl Pts',(4.55126765384403,72.5211227138997,0.));
#101545=CARTESIAN_POINT('Ctrl Pts',(4.54354380466826,72.5451394505106,0.));
#101546=CARTESIAN_POINT('Ctrl Pts',(4.53578496366802,72.5691865601225,0.));
#101547=CARTESIAN_POINT('Ctrl Pts',(4.52799111102391,72.5932639255406,0.));
#101548=CARTESIAN_POINT('Ctrl Pts',(4.52016222707633,72.6173714299935,0.));
#101549=CARTESIAN_POINT('Ctrl Pts',(4.5122982923226,72.6415089571314,0.));
#101550=CARTESIAN_POINT('Ctrl Pts',(4.50439928741605,72.6656763910241,0.));
#101551=CARTESIAN_POINT('Ctrl Pts',(4.49646519316822,72.689873616155,0.));
#101552=CARTESIAN_POINT('Ctrl Pts',(4.48849599055354,72.7141005174153,0.));
#101553=CARTESIAN_POINT('Ctrl Pts',(4.48049166070224,72.7383569801042,0.));
#101554=CARTESIAN_POINT('Ctrl Pts',(4.47245218489623,72.7626428899287,0.));
#101555=CARTESIAN_POINT('Ctrl Pts',(4.46437754456796,72.7869581329994,0.));
#101556=CARTESIAN_POINT('Ctrl Pts',(4.45626772130139,72.8113025958258,0.));
#101557=CARTESIAN_POINT('Ctrl Pts',(4.44812269683725,72.8356761653064,0.));
#101558=CARTESIAN_POINT('Ctrl Pts',(4.43994245306805,72.8600787287316,0.));
#101559=CARTESIAN_POINT('Ctrl Pts',(4.43172697203342,72.8845101737856,0.));
#101560=CARTESIAN_POINT('Ctrl Pts',(4.42347623591942,72.9089703885464,0.));
#101561=CARTESIAN_POINT('Ctrl Pts',(4.41519022705927,72.9334592614828,0.));
#101562=CARTESIAN_POINT('Ctrl Pts',(4.40686892793966,72.9579766814495,0.));
#101563=CARTESIAN_POINT('Ctrl Pts',(4.39851232119731,72.9825225376839,0.));
#101564=CARTESIAN_POINT('Ctrl Pts',(4.39012038961145,73.0070967198033,0.));
#101565=CARTESIAN_POINT('Ctrl Pts',(4.38169311610154,73.031699117799,0.));
#101566=CARTESIAN_POINT('Ctrl Pts',(4.37323048372607,73.0563296220301,0.));
#101567=CARTESIAN_POINT('Ctrl Pts',(4.36473247568639,73.0809881232111,0.));
#101568=CARTESIAN_POINT('Ctrl Pts',(4.35619907532716,73.1056745124099,0.));
#101569=CARTESIAN_POINT('Ctrl Pts',(4.34763026613155,73.1303886810602,0.));
#101570=CARTESIAN_POINT('Ctrl Pts',(4.3390260317214,73.1551305209692,0.));
#101571=CARTESIAN_POINT('Ctrl Pts',(4.33038635585878,73.1798999243234,0.));
#101572=CARTESIAN_POINT('Ctrl Pts',(4.32171122245219,73.204696783693,0.));
#101573=CARTESIAN_POINT('Ctrl Pts',(4.31300061556103,73.2295209920319,0.));
#101574=CARTESIAN_POINT('Ctrl Pts',(4.30425451938235,73.2543724426562,0.));
#101575=CARTESIAN_POINT('Ctrl Pts',(4.29547291824289,73.2792510292243,0.));
#101576=CARTESIAN_POINT('Ctrl Pts',(4.28665579659303,73.3041566457134,0.));
#101577=CARTESIAN_POINT('Ctrl Pts',(4.27780313900392,73.3290891863959,0.));
#101578=CARTESIAN_POINT('Ctrl Pts',(4.26891493016704,73.354048545808,0.));
#101579=CARTESIAN_POINT('Ctrl Pts',(4.25999115489905,73.3790346187953,0.));
#101580=CARTESIAN_POINT('Ctrl Pts',(4.25103179814892,73.4040473005603,0.));
#101581=CARTESIAN_POINT('Ctrl Pts',(4.24203684500942,73.4290864867103,0.));
#101582=CARTESIAN_POINT('Ctrl Pts',(4.23300628072758,73.4541520732943,0.));
#101583=CARTESIAN_POINT('Ctrl Pts',(4.22394009072754,73.4792439568624,0.));
#101584=CARTESIAN_POINT('Ctrl Pts',(4.21483826059437,73.5043620344107,0.));
#101585=CARTESIAN_POINT('Ctrl Pts',(4.20570077603728,73.5295062032621,0.));
#101586=CARTESIAN_POINT('Ctrl Pts',(4.19652762286127,73.554676360957,0.));
#101587=CARTESIAN_POINT('Ctrl Pts',(4.18731878694239,73.5798724051519,0.));
#101588=CARTESIAN_POINT('Ctrl Pts',(4.17807425419817,73.6050942334773,0.));
#101589=CARTESIAN_POINT('Ctrl Pts',(4.16879401058787,73.6303417435262,0.));
#101590=CARTESIAN_POINT('Ctrl Pts',(4.15947804217791,73.6556148331504,0.));
#101591=CARTESIAN_POINT('Ctrl Pts',(4.15012633519729,73.6809134006909,0.));
#101592=CARTESIAN_POINT('Ctrl Pts',(4.14073887610155,73.7062373452344,0.));
#101593=CARTESIAN_POINT('Ctrl Pts',(4.13131565163575,73.7315865668508,0.));
#101594=CARTESIAN_POINT('Ctrl Pts',(4.12185664890552,73.7569609668501,0.));
#101595=CARTESIAN_POINT('Ctrl Pts',(4.11236185522781,73.7823604472126,0.));
#101596=CARTESIAN_POINT('Ctrl Pts',(4.10283125798725,73.8077849100314,0.));
#101597=CARTESIAN_POINT('Ctrl Pts',(4.09326484448232,73.8332342568978,0.));
#101598=CARTESIAN_POINT('Ctrl Pts',(4.0836626018068,73.8587083884208,0.));
#101599=CARTESIAN_POINT('Ctrl Pts',(4.07402451665254,73.884207203405,0.));
#101600=CARTESIAN_POINT('Ctrl Pts',(4.06435057547335,73.9097305995173,0.));
#101601=CARTESIAN_POINT('Ctrl Pts',(4.05464076484762,73.9352784747665,0.));
#101602=CARTESIAN_POINT('Ctrl Pts',(4.04489507179964,73.9608507287943,0.));
#101603=CARTESIAN_POINT('Ctrl Pts',(4.03511348410661,73.9864472641025,0.));
#101604=CARTESIAN_POINT('Ctrl Pts',(4.02529599070086,74.0120679876396,0.));
#101605=CARTESIAN_POINT('Ctrl Pts',(4.01544258176694,74.0377128111754,0.));
#101606=CARTESIAN_POINT('Ctrl Pts',(4.00696550627606,74.0597159781919,0.));
#101607=CARTESIAN_POINT('Ctrl Pts',(4.00044689712491,74.0765982943431,0.));
#101608=CARTESIAN_POINT('Ctrl Pts',(3.99590266747766,74.0883491449662,0.));
#101609=CARTESIAN_POINT('Ctrl Pts',(3.9933433444657,74.0949615399274,0.));
#101610=CARTESIAN_POINT('Ctrl Pts',(3.99277406492178,74.0964320765798,0.));
#101611=CARTESIAN_POINT('',(5.24987136994593,69.8028570375097,12.));
#101612=CARTESIAN_POINT('',(5.24987136994593,69.8028570375097,0.));
#101613=CARTESIAN_POINT('Ctrl Pts',(3.99277406492178,74.0964320765798,12.));
#101614=CARTESIAN_POINT('Ctrl Pts',(3.9933433444657,74.0949615399274,12.));
#101615=CARTESIAN_POINT('Ctrl Pts',(3.99590266747766,74.0883491449662,12.));
#101616=CARTESIAN_POINT('Ctrl Pts',(4.00044689712491,74.0765982943431,12.));
#101617=CARTESIAN_POINT('Ctrl Pts',(4.00696550627606,74.0597159781919,12.));
#101618=CARTESIAN_POINT('Ctrl Pts',(4.01544258176694,74.0377128111754,12.));
#101619=CARTESIAN_POINT('Ctrl Pts',(4.02529599070086,74.0120679876396,12.));
#101620=CARTESIAN_POINT('Ctrl Pts',(4.03511348410661,73.9864472641025,12.));
#101621=CARTESIAN_POINT('Ctrl Pts',(4.04489507179964,73.9608507287943,12.));
#101622=CARTESIAN_POINT('Ctrl Pts',(4.05464076484762,73.9352784747665,12.));
#101623=CARTESIAN_POINT('Ctrl Pts',(4.06435057547335,73.9097305995173,12.));
#101624=CARTESIAN_POINT('Ctrl Pts',(4.07402451665254,73.884207203405,12.));
#101625=CARTESIAN_POINT('Ctrl Pts',(4.0836626018068,73.8587083884208,12.));
#101626=CARTESIAN_POINT('Ctrl Pts',(4.09326484448232,73.8332342568978,12.));
#101627=CARTESIAN_POINT('Ctrl Pts',(4.10283125798725,73.8077849100314,12.));
#101628=CARTESIAN_POINT('Ctrl Pts',(4.11236185522781,73.7823604472126,12.));
#101629=CARTESIAN_POINT('Ctrl Pts',(4.12185664890552,73.7569609668501,12.));
#101630=CARTESIAN_POINT('Ctrl Pts',(4.13131565163575,73.7315865668508,12.));
#101631=CARTESIAN_POINT('Ctrl Pts',(4.14073887610155,73.7062373452344,12.));
#101632=CARTESIAN_POINT('Ctrl Pts',(4.15012633519729,73.6809134006909,12.));
#101633=CARTESIAN_POINT('Ctrl Pts',(4.15947804217791,73.6556148331504,12.));
#101634=CARTESIAN_POINT('Ctrl Pts',(4.16879401058787,73.6303417435262,12.));
#101635=CARTESIAN_POINT('Ctrl Pts',(4.17807425419817,73.6050942334773,12.));
#101636=CARTESIAN_POINT('Ctrl Pts',(4.18731878694239,73.5798724051519,12.));
#101637=CARTESIAN_POINT('Ctrl Pts',(4.19652762286127,73.554676360957,12.));
#101638=CARTESIAN_POINT('Ctrl Pts',(4.20570077603728,73.5295062032621,12.));
#101639=CARTESIAN_POINT('Ctrl Pts',(4.21483826059437,73.5043620344107,12.));
#101640=CARTESIAN_POINT('Ctrl Pts',(4.22394009072754,73.4792439568624,12.));
#101641=CARTESIAN_POINT('Ctrl Pts',(4.23300628072758,73.4541520732943,12.));
#101642=CARTESIAN_POINT('Ctrl Pts',(4.24203684500942,73.4290864867103,12.));
#101643=CARTESIAN_POINT('Ctrl Pts',(4.25103179814892,73.4040473005603,12.));
#101644=CARTESIAN_POINT('Ctrl Pts',(4.25999115489905,73.3790346187953,12.));
#101645=CARTESIAN_POINT('Ctrl Pts',(4.26891493016704,73.354048545808,12.));
#101646=CARTESIAN_POINT('Ctrl Pts',(4.27780313900392,73.3290891863959,12.));
#101647=CARTESIAN_POINT('Ctrl Pts',(4.28665579659303,73.3041566457134,12.));
#101648=CARTESIAN_POINT('Ctrl Pts',(4.29547291824289,73.2792510292243,12.));
#101649=CARTESIAN_POINT('Ctrl Pts',(4.30425451938235,73.2543724426562,12.));
#101650=CARTESIAN_POINT('Ctrl Pts',(4.31300061556103,73.2295209920319,12.));
#101651=CARTESIAN_POINT('Ctrl Pts',(4.32171122245219,73.204696783693,12.));
#101652=CARTESIAN_POINT('Ctrl Pts',(4.33038635585878,73.1798999243234,12.));
#101653=CARTESIAN_POINT('Ctrl Pts',(4.3390260317214,73.1551305209692,12.));
#101654=CARTESIAN_POINT('Ctrl Pts',(4.34763026613155,73.1303886810602,12.));
#101655=CARTESIAN_POINT('Ctrl Pts',(4.35619907532716,73.1056745124099,12.));
#101656=CARTESIAN_POINT('Ctrl Pts',(4.36473247568639,73.0809881232111,12.));
#101657=CARTESIAN_POINT('Ctrl Pts',(4.37323048372607,73.0563296220301,12.));
#101658=CARTESIAN_POINT('Ctrl Pts',(4.38169311610154,73.031699117799,12.));
#101659=CARTESIAN_POINT('Ctrl Pts',(4.39012038961145,73.0070967198033,12.));
#101660=CARTESIAN_POINT('Ctrl Pts',(4.39851232119731,72.9825225376839,12.));
#101661=CARTESIAN_POINT('Ctrl Pts',(4.40686892793966,72.9579766814495,12.));
#101662=CARTESIAN_POINT('Ctrl Pts',(4.41519022705927,72.9334592614828,12.));
#101663=CARTESIAN_POINT('Ctrl Pts',(4.42347623591942,72.9089703885464,12.));
#101664=CARTESIAN_POINT('Ctrl Pts',(4.43172697203342,72.8845101737856,12.));
#101665=CARTESIAN_POINT('Ctrl Pts',(4.43994245306805,72.8600787287316,12.));
#101666=CARTESIAN_POINT('Ctrl Pts',(4.44812269683725,72.8356761653064,12.));
#101667=CARTESIAN_POINT('Ctrl Pts',(4.45626772130139,72.8113025958258,12.));
#101668=CARTESIAN_POINT('Ctrl Pts',(4.46437754456796,72.7869581329994,12.));
#101669=CARTESIAN_POINT('Ctrl Pts',(4.47245218489623,72.7626428899287,12.));
#101670=CARTESIAN_POINT('Ctrl Pts',(4.48049166070224,72.7383569801042,12.));
#101671=CARTESIAN_POINT('Ctrl Pts',(4.48849599055354,72.7141005174153,12.));
#101672=CARTESIAN_POINT('Ctrl Pts',(4.49646519316822,72.689873616155,12.));
#101673=CARTESIAN_POINT('Ctrl Pts',(4.50439928741605,72.6656763910241,12.));
#101674=CARTESIAN_POINT('Ctrl Pts',(4.5122982923226,72.6415089571314,12.));
#101675=CARTESIAN_POINT('Ctrl Pts',(4.52016222707633,72.6173714299935,12.));
#101676=CARTESIAN_POINT('Ctrl Pts',(4.52799111102391,72.5932639255406,12.));
#101677=CARTESIAN_POINT('Ctrl Pts',(4.53578496366802,72.5691865601225,12.));
#101678=CARTESIAN_POINT('Ctrl Pts',(4.54354380466826,72.5451394505106,12.));
#101679=CARTESIAN_POINT('Ctrl Pts',(4.55126765384403,72.5211227138997,12.));
#101680=CARTESIAN_POINT('Ctrl Pts',(4.55895653118214,72.4971364679055,12.));
#101681=CARTESIAN_POINT('Ctrl Pts',(4.56661045683367,72.473180830571,12.));
#101682=CARTESIAN_POINT('Ctrl Pts',(4.57422945111095,72.449255920373,12.));
#101683=CARTESIAN_POINT('Ctrl Pts',(4.58181353448852,72.4253618562249,12.));
#101684=CARTESIAN_POINT('Ctrl Pts',(4.58936272760551,72.4014987574789,12.));
#101685=CARTESIAN_POINT('Ctrl Pts',(4.59687705127341,72.3776667439244,12.));
#101686=CARTESIAN_POINT('Ctrl Pts',(4.60435652647464,72.3538659357932,12.));
#101687=CARTESIAN_POINT('Ctrl Pts',(4.61180117435869,72.330096453767,12.));
#101688=CARTESIAN_POINT('Ctrl Pts',(4.61921101624295,72.306358418981,12.));
#101689=CARTESIAN_POINT('Ctrl Pts',(4.62658607361466,72.2826519530254,12.));
#101690=CARTESIAN_POINT('Ctrl Pts',(4.63392636813843,72.2589771779447,12.));
#101691=CARTESIAN_POINT('Ctrl Pts',(4.64123192165628,72.2353342162408,12.));
#101692=CARTESIAN_POINT('Ctrl Pts',(4.64850275618326,72.2117231908816,12.));
#101693=CARTESIAN_POINT('Ctrl Pts',(4.65573889390825,72.1881442253052,12.));
#101694=CARTESIAN_POINT('Ctrl Pts',(4.66294035719571,72.1645974434218,12.));
#101695=CARTESIAN_POINT('Ctrl Pts',(4.67010716859282,72.1410829696129,12.));
#101696=CARTESIAN_POINT('Ctrl Pts',(4.67723935083088,72.1176009287349,12.));
#101697=CARTESIAN_POINT('Ctrl Pts',(4.68433692682061,72.0941514461283,12.));
#101698=CARTESIAN_POINT('Ctrl Pts',(4.69139991965281,72.070734647621,12.));
#101699=CARTESIAN_POINT('Ctrl Pts',(4.69842835259998,72.047350659532,12.));
#101700=CARTESIAN_POINT('Ctrl Pts',(4.70542224912313,72.0239996086694,12.));
#101701=CARTESIAN_POINT('Ctrl Pts',(4.71238163287411,72.0006816223335,12.));
#101702=CARTESIAN_POINT('Ctrl Pts',(4.71930652769081,71.9773968283267,12.));
#101703=CARTESIAN_POINT('Ctrl Pts',(4.72619695759779,71.9541453549582,12.));
#101704=CARTESIAN_POINT('Ctrl Pts',(4.73305294680784,71.9309273310469,12.));
#101705=CARTESIAN_POINT('Ctrl Pts',(4.73987451972861,71.9077428859207,12.));
#101706=CARTESIAN_POINT('Ctrl Pts',(4.74666170096546,71.8845921494186,12.));
#101707=CARTESIAN_POINT('Ctrl Pts',(4.75341451531672,71.8614752519008,12.));
#101708=CARTESIAN_POINT('Ctrl Pts',(4.76013298777423,71.8383923242533,12.));
#101709=CARTESIAN_POINT('Ctrl Pts',(4.76681714352504,71.8153434978924,12.));
#101710=CARTESIAN_POINT('Ctrl Pts',(4.77346700795788,71.7923289047636,12.));
#101711=CARTESIAN_POINT('Ctrl Pts',(4.78008260666643,71.7693486773449,12.));
#101712=CARTESIAN_POINT('Ctrl Pts',(4.78666396544451,71.7464029486552,12.));
#101713=CARTESIAN_POINT('Ctrl Pts',(4.79321111028673,71.7234918522604,12.));
#101714=CARTESIAN_POINT('Ctrl Pts',(4.79972406739015,71.7006155222766,12.));
#101715=CARTESIAN_POINT('Ctrl Pts',(4.80620286316089,71.6777740933705,12.));
#101716=CARTESIAN_POINT('Ctrl Pts',(4.81264752421732,71.6549677007613,12.));
#101717=CARTESIAN_POINT('Ctrl Pts',(4.81905807738558,71.6321964802326,12.));
#101718=CARTESIAN_POINT('Ctrl Pts',(4.82543454970027,71.6094605681366,12.));
#101719=CARTESIAN_POINT('Ctrl Pts',(4.83177696840638,71.5867601014,12.));
#101720=CARTESIAN_POINT('Ctrl Pts',(4.83808536096584,71.564095217521,12.));
#101721=CARTESIAN_POINT('Ctrl Pts',(4.84435975506049,71.5414660545739,12.));
#101722=CARTESIAN_POINT('Ctrl Pts',(4.85060017858781,71.5188727512197,12.));
#101723=CARTESIAN_POINT('Ctrl Pts',(4.85680665966181,71.4963154467113,12.));
#101724=CARTESIAN_POINT('Ctrl Pts',(4.86297922661503,71.4737942808982,12.));
#101725=CARTESIAN_POINT('Ctrl Pts',(4.86911790800551,71.4513093942255,12.));
#101726=CARTESIAN_POINT('Ctrl Pts',(4.87522273261908,71.4288609277374,12.));
#101727=CARTESIAN_POINT('Ctrl Pts',(4.88129372946552,71.4064490230899,12.));
#101728=CARTESIAN_POINT('Ctrl Pts',(4.88733092777976,71.3840738225562,12.));
#101729=CARTESIAN_POINT('Ctrl Pts',(4.89333435702414,71.3617354690325,12.));
#101730=CARTESIAN_POINT('Ctrl Pts',(4.89930404689576,71.3394341060359,12.));
#101731=CARTESIAN_POINT('Ctrl Pts',(4.9052400273278,71.3171698777084,12.));
#101732=CARTESIAN_POINT('Ctrl Pts',(4.91114232848604,71.294942928829,12.));
#101733=CARTESIAN_POINT('Ctrl Pts',(4.91701098077037,71.2727534048192,12.));
#101734=CARTESIAN_POINT('Ctrl Pts',(4.92284601481722,71.250601451747,12.));
#101735=CARTESIAN_POINT('Ctrl Pts',(4.92864746150733,71.2284872163273,12.));
#101736=CARTESIAN_POINT('Ctrl Pts',(4.93441535196618,71.2064108459286,12.));
#101737=CARTESIAN_POINT('Ctrl Pts',(4.94014971756115,71.1843724885847,12.));
#101738=CARTESIAN_POINT('Ctrl Pts',(4.94585058990342,71.1623722930001,12.));
#101739=CARTESIAN_POINT('Ctrl Pts',(4.95151800085102,71.1404104085552,12.));
#101740=CARTESIAN_POINT('Ctrl Pts',(4.95715198251685,71.1184869853056,12.));
#101741=CARTESIAN_POINT('Ctrl Pts',(4.96275256726767,71.0966021739907,12.));
#101742=CARTESIAN_POINT('Ctrl Pts',(4.96831978772191,71.0747561260436,12.));
#101743=CARTESIAN_POINT('Ctrl Pts',(4.97385367675159,71.0529489935961,12.));
#101744=CARTESIAN_POINT('Ctrl Pts',(4.97935426748585,71.0311809294821,12.));
#101745=CARTESIAN_POINT('Ctrl Pts',(4.98482159331864,71.0094520872377,12.));
#101746=CARTESIAN_POINT('Ctrl Pts',(4.99025568790665,70.9877626211113,12.));
#101747=CARTESIAN_POINT('Ctrl Pts',(4.99565658516914,70.9661126860773,12.));
#101748=CARTESIAN_POINT('Ctrl Pts',(5.0010243192904,70.9445024378439,12.));
#101749=CARTESIAN_POINT('Ctrl Pts',(5.00635892472514,70.9229320328589,12.));
#101750=CARTESIAN_POINT('Ctrl Pts',(5.01166043620568,70.9014016283124,12.));
#101751=CARTESIAN_POINT('Ctrl Pts',(5.01692888873791,70.8799113821452,12.));
#101752=CARTESIAN_POINT('Ctrl Pts',(5.02216431760061,70.8584614530519,12.));
#101753=CARTESIAN_POINT('Ctrl Pts',(5.02736675834694,70.8370520004843,12.));
#101754=CARTESIAN_POINT('Ctrl Pts',(5.03253624680942,70.8156831846488,12.));
#101755=CARTESIAN_POINT('Ctrl Pts',(5.0376728191048,70.7943551665059,12.));
#101756=CARTESIAN_POINT('Ctrl Pts',(5.0427765116335,70.7730681077983,12.));
#101757=CARTESIAN_POINT('Ctrl Pts',(5.04784736108347,70.7518221710706,12.));
#101758=CARTESIAN_POINT('Ctrl Pts',(5.05288540443483,70.7306175196863,12.));
#101759=CARTESIAN_POINT('Ctrl Pts',(5.05789067897058,70.7094543178438,12.));
#101760=CARTESIAN_POINT('Ctrl Pts',(5.06286322227821,70.6883327305784,12.));
#101761=CARTESIAN_POINT('Ctrl Pts',(5.06780307224073,70.6672529237455,12.));
#101762=CARTESIAN_POINT('Ctrl Pts',(5.07271026703356,70.6462150640015,12.));
#101763=CARTESIAN_POINT('Ctrl Pts',(5.07758484512303,70.6252193187878,12.));
#101764=CARTESIAN_POINT('Ctrl Pts',(5.08242684526687,70.6042658562923,12.));
#101765=CARTESIAN_POINT('Ctrl Pts',(5.08723630652274,70.5833548455014,12.));
#101766=CARTESIAN_POINT('Ctrl Pts',(5.09201326826135,70.5624864562824,12.));
#101767=CARTESIAN_POINT('Ctrl Pts',(5.09675777018184,70.5416608594526,12.));
#101768=CARTESIAN_POINT('Ctrl Pts',(5.10146985232942,70.5208782268497,12.));
#101769=CARTESIAN_POINT('Ctrl Pts',(5.10614955511665,70.500138731399,12.));
#101770=CARTESIAN_POINT('Ctrl Pts',(5.11079691929214,70.4794425469825,12.));
#101771=CARTESIAN_POINT('Ctrl Pts',(5.11541198590933,70.458789848296,12.));
#101772=CARTESIAN_POINT('Ctrl Pts',(5.11999479630212,70.4381808107245,12.));
#101773=CARTESIAN_POINT('Ctrl Pts',(5.12454539205329,70.417615610161,12.));
#101774=CARTESIAN_POINT('Ctrl Pts',(5.12906381499457,70.3970944229851,12.));
#101775=CARTESIAN_POINT('Ctrl Pts',(5.13355010728568,70.3766174264757,12.));
#101776=CARTESIAN_POINT('Ctrl Pts',(5.13800431148904,70.3561847991714,12.));
#101777=CARTESIAN_POINT('Ctrl Pts',(5.1424264706348,70.3357967211796,12.));
#101778=CARTESIAN_POINT('Ctrl Pts',(5.14681662833081,70.3154533746736,12.));
#101779=CARTESIAN_POINT('Ctrl Pts',(5.15117482869255,70.2951549435512,12.));
#101780=CARTESIAN_POINT('Ctrl Pts',(5.1555011161486,70.2749016125105,12.));
#101781=CARTESIAN_POINT('Ctrl Pts',(5.15979553528204,70.2546935662722,12.));
#101782=CARTESIAN_POINT('Ctrl Pts',(5.16405813066977,70.2345309887833,12.));
#101783=CARTESIAN_POINT('Ctrl Pts',(5.16828894670109,70.2144140622953,12.));
#101784=CARTESIAN_POINT('Ctrl Pts',(5.1724880279339,70.1943429691167,12.));
#101785=CARTESIAN_POINT('Ctrl Pts',(5.17665541952384,70.1743178937077,12.));
#101786=CARTESIAN_POINT('Ctrl Pts',(5.18079116757667,70.1543390243892,12.));
#101787=CARTESIAN_POINT('Ctrl Pts',(5.18489531966266,70.1344065558145,12.));
#101788=CARTESIAN_POINT('Ctrl Pts',(5.18896792486566,70.1145206891885,12.));
#101789=CARTESIAN_POINT('Ctrl Pts',(5.19300903271581,70.0946816270997,12.));
#101790=CARTESIAN_POINT('Ctrl Pts',(5.19701869225529,70.0748895689729,12.));
#101791=CARTESIAN_POINT('Ctrl Pts',(5.20099695122657,70.0551447071082,12.));
#101792=CARTESIAN_POINT('Ctrl Pts',(5.20494385478026,70.0354472203546,12.));
#101793=CARTESIAN_POINT('Ctrl Pts',(5.20885944672837,70.0157972802182,12.));
#101794=CARTESIAN_POINT('Ctrl Pts',(5.2127437720326,69.9961950629965,12.));
#101795=CARTESIAN_POINT('Ctrl Pts',(5.2165968788114,69.9766407595385,12.));
#101796=CARTESIAN_POINT('Ctrl Pts',(5.22041882075722,69.9571345870076,12.));
#101797=CARTESIAN_POINT('Ctrl Pts',(5.22420965879982,69.9376767969095,12.));
#101798=CARTESIAN_POINT('Ctrl Pts',(5.22796945602795,69.9182676502048,12.));
#101799=CARTESIAN_POINT('Ctrl Pts',(5.23169827290556,69.8989073936688,12.));
#101800=CARTESIAN_POINT('Ctrl Pts',(5.23539616279621,69.8795962381599,12.));
#101801=CARTESIAN_POINT('Ctrl Pts',(5.23906316634803,69.8603343302743,12.));
#101802=CARTESIAN_POINT('Ctrl Pts',(5.2426993105457,69.841121750752,12.));
#101803=CARTESIAN_POINT('Ctrl Pts',(5.24558355159751,69.8257911792159,12.));
#101804=CARTESIAN_POINT('Ctrl Pts',(5.24773285666377,69.8143154684204,12.));
#101805=CARTESIAN_POINT('Ctrl Pts',(5.24915955997427,69.8066748687772,12.));
#101806=CARTESIAN_POINT('Ctrl Pts',(5.24987136994593,69.8028570375097,12.));
#101807=CARTESIAN_POINT('Ctrl Pts',(2.48034921844894,74.1624659714953,0.));
#101808=CARTESIAN_POINT('Ctrl Pts',(2.48034921844894,74.1624659714953,4.));
#101809=CARTESIAN_POINT('Ctrl Pts',(2.48034921844894,74.1624659714953,8.));
#101810=CARTESIAN_POINT('Ctrl Pts',(2.48034921844894,74.1624659714953,12.));
#101811=CARTESIAN_POINT('Ctrl Pts',(2.52879860312834,74.2610905805697,0.));
#101812=CARTESIAN_POINT('Ctrl Pts',(2.52879860312834,74.2610905805697,4.));
#101813=CARTESIAN_POINT('Ctrl Pts',(2.52879860312834,74.2610905805697,8.));
#101814=CARTESIAN_POINT('Ctrl Pts',(2.52879860312834,74.2610905805697,12.));
#101815=CARTESIAN_POINT('Ctrl Pts',(2.67239300265247,74.404107577982,0.));
#101816=CARTESIAN_POINT('Ctrl Pts',(2.67239300265247,74.404107577982,4.00000000000001));
#101817=CARTESIAN_POINT('Ctrl Pts',(2.67239300265247,74.404107577982,7.99999999999999));
#101818=CARTESIAN_POINT('Ctrl Pts',(2.67239300265247,74.404107577982,12.));
#101819=CARTESIAN_POINT('Ctrl Pts',(2.86656650944678,74.4448761712981,0.));
#101820=CARTESIAN_POINT('Ctrl Pts',(2.86656650944678,74.4448761712981,3.99999999999999));
#101821=CARTESIAN_POINT('Ctrl Pts',(2.86656650944678,74.4448761712981,8.00000000000001));
#101822=CARTESIAN_POINT('Ctrl Pts',(2.86656650944678,74.4448761712981,12.));
#101823=CARTESIAN_POINT('Ctrl Pts',(2.94891377268021,74.441614084874,0.));
#101824=CARTESIAN_POINT('Ctrl Pts',(2.94891377268021,74.441614084874,4.));
#101825=CARTESIAN_POINT('Ctrl Pts',(2.94891377268021,74.441614084874,8.));
#101826=CARTESIAN_POINT('Ctrl Pts',(2.94891377268021,74.441614084874,12.));
#101827=CARTESIAN_POINT('',(2.48034921844894,74.1624659714953,0.));
#101828=CARTESIAN_POINT('',(2.94891377268021,74.4416140848739,0.));
#101829=CARTESIAN_POINT('Ctrl Pts',(2.48034921844894,74.1624659714953,1.88097848788491E-35));
#101830=CARTESIAN_POINT('Ctrl Pts',(2.52879860312834,74.2610905805697,1.88097848788491E-35));
#101831=CARTESIAN_POINT('Ctrl Pts',(2.61085254571356,74.342814579091,1.88097848788492E-35));
#101832=CARTESIAN_POINT('Ctrl Pts',(2.70942211516251,74.3911513436217,1.88097848788491E-35));
#101833=CARTESIAN_POINT('Ctrl Pts',(2.78334929224922,74.4274039170197,1.88097848788491E-35));
#101834=CARTESIAN_POINT('Ctrl Pts',(2.86656650944678,74.4448761712981,1.88097848788491E-35));
#101835=CARTESIAN_POINT('Ctrl Pts',(2.94891377268021,74.441614084874,1.88097848788491E-35));
#101836=CARTESIAN_POINT('',(2.94891377268021,74.4416140848739,12.));
#101837=CARTESIAN_POINT('Ctrl Pts',(2.94891377268021,74.441614084874,0.));
#101838=CARTESIAN_POINT('Ctrl Pts',(2.94891377268021,74.441614084874,4.));
#101839=CARTESIAN_POINT('Ctrl Pts',(2.94891377268021,74.441614084874,8.));
#101840=CARTESIAN_POINT('Ctrl Pts',(2.94891377268021,74.441614084874,12.));
#101841=CARTESIAN_POINT('',(2.48034921844894,74.1624659714953,12.));
#101842=CARTESIAN_POINT('Ctrl Pts',(2.94891377268021,74.441614084874,12.));
#101843=CARTESIAN_POINT('Ctrl Pts',(2.86656650944678,74.4448761712981,12.));
#101844=CARTESIAN_POINT('Ctrl Pts',(2.78334929224922,74.4274039170197,12.));
#101845=CARTESIAN_POINT('Ctrl Pts',(2.70942211516251,74.3911513436217,12.));
#101846=CARTESIAN_POINT('Ctrl Pts',(2.61085254571356,74.342814579091,12.));
#101847=CARTESIAN_POINT('Ctrl Pts',(2.52879860312834,74.2610905805697,12.));
#101848=CARTESIAN_POINT('Ctrl Pts',(2.48034921844894,74.1624659714953,12.));
#101849=CARTESIAN_POINT('Ctrl Pts',(2.48034921844894,74.1624659714953,12.));
#101850=CARTESIAN_POINT('Ctrl Pts',(2.48034921844894,74.1624659714953,8.));
#101851=CARTESIAN_POINT('Ctrl Pts',(2.48034921844894,74.1624659714953,4.));
#101852=CARTESIAN_POINT('Ctrl Pts',(2.48034921844894,74.1624659714953,0.));
#101853=CARTESIAN_POINT('Origin',(1.62512913209676E-11,3.74491326291036E-10,
0.));
#101854=CARTESIAN_POINT('Origin',(1.62512913209676E-11,3.74491326291036E-10,
12.));
#101855=CARTESIAN_POINT('Origin',(1.62512913209676E-11,3.74491326291036E-10,
0.));
#101856=CARTESIAN_POINT('Ctrl Pts',(10.0225374821205,73.8227522002498,-5.55111512312578E-16));
#101857=CARTESIAN_POINT('Ctrl Pts',(10.0225374821205,73.8227522002498,4.));
#101858=CARTESIAN_POINT('Ctrl Pts',(10.0225374821204,73.8227522002498,8.));
#101859=CARTESIAN_POINT('Ctrl Pts',(10.0225374821204,73.8227522002498,12.));
#101860=CARTESIAN_POINT('Ctrl Pts',(10.1314210536415,73.8079696346554,-5.55111512312578E-16));
#101861=CARTESIAN_POINT('Ctrl Pts',(10.1314210536415,73.8079696346554,4.));
#101862=CARTESIAN_POINT('Ctrl Pts',(10.1314210536415,73.8079696346554,8.00000000000001));
#101863=CARTESIAN_POINT('Ctrl Pts',(10.1314210536415,73.8079696346554,12.));
#101864=CARTESIAN_POINT('Ctrl Pts',(10.3125002643518,73.7169567649191,-5.55111512312578E-16));
#101865=CARTESIAN_POINT('Ctrl Pts',(10.3125002643518,73.7169567649191,4.));
#101866=CARTESIAN_POINT('Ctrl Pts',(10.3125002643517,73.7169567649191,7.99999999999999));
#101867=CARTESIAN_POINT('Ctrl Pts',(10.3125002643517,73.7169567649191,12.));
#101868=CARTESIAN_POINT('Ctrl Pts',(10.4125694172277,73.5456341632195,-5.55111512312578E-16));
#101869=CARTESIAN_POINT('Ctrl Pts',(10.4125694172277,73.5456341632195,4.));
#101870=CARTESIAN_POINT('Ctrl Pts',(10.4125694172276,73.5456341632195,8.00000000000001));
#101871=CARTESIAN_POINT('Ctrl Pts',(10.4125694172276,73.5456341632195,12.));
#101872=CARTESIAN_POINT('Ctrl Pts',(10.435509926739,73.4664795929517,-5.55111512312578E-16));
#101873=CARTESIAN_POINT('Ctrl Pts',(10.435509926739,73.4664795929517,4.));
#101874=CARTESIAN_POINT('Ctrl Pts',(10.4355099267389,73.4664795929517,8.));
#101875=CARTESIAN_POINT('Ctrl Pts',(10.4355099267389,73.4664795929517,12.));
#101876=CARTESIAN_POINT('',(10.0225374821205,73.8227522002498,0.));
#101877=CARTESIAN_POINT('',(10.4355099267391,73.4664795929517,2.77555756156289E-16));
#101878=CARTESIAN_POINT('Ctrl Pts',(10.0225374821205,73.8227522002498,-1.38777878078145E-16));
#101879=CARTESIAN_POINT('Ctrl Pts',(10.1314210536415,73.8079696346554,-1.38777878078145E-16));
#101880=CARTESIAN_POINT('Ctrl Pts',(10.2348948883331,73.7559622805204,-1.38777878078144E-16));
#101881=CARTESIAN_POINT('Ctrl Pts',(10.311916459242,73.6777313404381,-1.38777878078144E-16));
#101882=CARTESIAN_POINT('Ctrl Pts',(10.3696826374237,73.6190581353764,-1.38777878078145E-16));
#101883=CARTESIAN_POINT('Ctrl Pts',(10.4125694172277,73.5456341632195,-1.38777878078145E-16));
#101884=CARTESIAN_POINT('Ctrl Pts',(10.435509926739,73.4664795929517,-1.38777878078145E-16));
#101885=CARTESIAN_POINT('',(10.4355099267391,73.4664795929518,12.));
#101886=CARTESIAN_POINT('Ctrl Pts',(10.435509926739,73.4664795929517,-5.55111512312578E-16));
#101887=CARTESIAN_POINT('Ctrl Pts',(10.435509926739,73.4664795929517,4.));
#101888=CARTESIAN_POINT('Ctrl Pts',(10.4355099267389,73.4664795929517,8.));
#101889=CARTESIAN_POINT('Ctrl Pts',(10.4355099267389,73.4664795929517,12.));
#101890=CARTESIAN_POINT('',(10.0225374821204,73.8227522002498,12.));
#101891=CARTESIAN_POINT('Ctrl Pts',(10.4355099267389,73.4664795929517,12.));
#101892=CARTESIAN_POINT('Ctrl Pts',(10.4125694172276,73.5456341632195,12.));
#101893=CARTESIAN_POINT('Ctrl Pts',(10.3696826374237,73.6190581353765,12.));
#101894=CARTESIAN_POINT('Ctrl Pts',(10.311916459242,73.6777313404381,12.));
#101895=CARTESIAN_POINT('Ctrl Pts',(10.2348948883331,73.7559622805204,12.));
#101896=CARTESIAN_POINT('Ctrl Pts',(10.1314210536415,73.8079696346554,12.));
#101897=CARTESIAN_POINT('Ctrl Pts',(10.0225374821204,73.8227522002498,12.));
#101898=CARTESIAN_POINT('Ctrl Pts',(10.0225374821204,73.8227522002498,12.));
#101899=CARTESIAN_POINT('Ctrl Pts',(10.0225374821204,73.8227522002498,8.));
#101900=CARTESIAN_POINT('Ctrl Pts',(10.0225374821205,73.8227522002498,4.));
#101901=CARTESIAN_POINT('Ctrl Pts',(10.0225374821205,73.8227522002498,-5.55111512312578E-16));
#101902=CARTESIAN_POINT('Ctrl Pts',(11.3136138754165,69.079679653846,0.));
#101903=CARTESIAN_POINT('Ctrl Pts',(11.3136138754165,69.079679653846,12.));
#101904=CARTESIAN_POINT('Ctrl Pts',(11.3132375200165,69.0835449954396,0.));
#101905=CARTESIAN_POINT('Ctrl Pts',(11.3132375200165,69.0835449954396,12.));
#101906=CARTESIAN_POINT('Ctrl Pts',(11.3124821678798,69.0912808656811,0.));
#101907=CARTESIAN_POINT('Ctrl Pts',(11.3124821678798,69.0912808656811,12.));
#101908=CARTESIAN_POINT('Ctrl Pts',(11.3113412156661,69.1029002322118,0.));
#101909=CARTESIAN_POINT('Ctrl Pts',(11.3113412156661,69.1029002322118,12.));
#101910=CARTESIAN_POINT('Ctrl Pts',(11.3098040973713,69.118423844466,0.));
#101911=CARTESIAN_POINT('Ctrl Pts',(11.3098040973713,69.118423844466,12.));
#101912=CARTESIAN_POINT('Ctrl Pts',(11.3078562764384,69.1378802251711,0.));
#101913=CARTESIAN_POINT('Ctrl Pts',(11.3078562764384,69.1378802251711,12.));
#101914=CARTESIAN_POINT('Ctrl Pts',(11.3058820128307,69.1573884361,0.));
#101915=CARTESIAN_POINT('Ctrl Pts',(11.3058820128307,69.1573884361,12.));
#101916=CARTESIAN_POINT('Ctrl Pts',(11.3038812726292,69.1769483991721,0.));
#101917=CARTESIAN_POINT('Ctrl Pts',(11.3038812726292,69.1769483991721,12.));
#101918=CARTESIAN_POINT('Ctrl Pts',(11.3018540025638,69.1965599718914,0.));
#101919=CARTESIAN_POINT('Ctrl Pts',(11.3018540025638,69.1965599718914,12.));
#101920=CARTESIAN_POINT('Ctrl Pts',(11.2998001310964,69.2162229488531,0.));
#101921=CARTESIAN_POINT('Ctrl Pts',(11.2998001310964,69.2162229488531,12.));
#101922=CARTESIAN_POINT('Ctrl Pts',(11.2977195764852,69.2359370894907,0.));
#101923=CARTESIAN_POINT('Ctrl Pts',(11.2977195764852,69.2359370894907,12.));
#101924=CARTESIAN_POINT('Ctrl Pts',(11.2956122531375,69.2557021393351,0.));
#101925=CARTESIAN_POINT('Ctrl Pts',(11.2956122531375,69.2557021393351,12.));
#101926=CARTESIAN_POINT('Ctrl Pts',(11.2934780784351,69.275517853148,0.));
#101927=CARTESIAN_POINT('Ctrl Pts',(11.2934780784351,69.275517853148,12.));
#101928=CARTESIAN_POINT('Ctrl Pts',(11.2913169799628,69.295384019272,0.));
#101929=CARTESIAN_POINT('Ctrl Pts',(11.2913169799628,69.295384019272,12.));
#101930=CARTESIAN_POINT('Ctrl Pts',(11.2891288931517,69.3153004517783,0.));
#101931=CARTESIAN_POINT('Ctrl Pts',(11.2891288931517,69.3153004517783,12.));
#101932=CARTESIAN_POINT('Ctrl Pts',(11.2869137578459,69.3352669789587,0.));
#101933=CARTESIAN_POINT('Ctrl Pts',(11.2869137578459,69.3352669789587,12.));
#101934=CARTESIAN_POINT('Ctrl Pts',(11.2846715154524,69.3552834337784,0.));
#101935=CARTESIAN_POINT('Ctrl Pts',(11.2846715154524,69.3552834337784,12.));
#101936=CARTESIAN_POINT('Ctrl Pts',(11.2824021054045,69.3753496420039,0.));
#101937=CARTESIAN_POINT('Ctrl Pts',(11.2824021054045,69.3753496420039,12.));
#101938=CARTESIAN_POINT('Ctrl Pts',(11.2801054633816,69.3954654162281,0.));
#101939=CARTESIAN_POINT('Ctrl Pts',(11.2801054633816,69.3954654162281,12.));
#101940=CARTESIAN_POINT('Ctrl Pts',(11.2777815231469,69.4156305620593,0.));
#101941=CARTESIAN_POINT('Ctrl Pts',(11.2777815231469,69.4156305620593,12.));
#101942=CARTESIAN_POINT('Ctrl Pts',(11.2754302177021,69.4358448819967,0.));
#101943=CARTESIAN_POINT('Ctrl Pts',(11.2754302177021,69.4358448819967,12.));
#101944=CARTESIAN_POINT('Ctrl Pts',(11.2730514806139,69.456108179879,0.));
#101945=CARTESIAN_POINT('Ctrl Pts',(11.2730514806139,69.456108179879,12.));
#101946=CARTESIAN_POINT('Ctrl Pts',(11.270645247528,69.4764202659397,0.));
#101947=CARTESIAN_POINT('Ctrl Pts',(11.270645247528,69.4764202659397,12.));
#101948=CARTESIAN_POINT('Ctrl Pts',(11.2682114561008,69.4967809565929,0.));
#101949=CARTESIAN_POINT('Ctrl Pts',(11.2682114561008,69.4967809565929,12.));
#101950=CARTESIAN_POINT('Ctrl Pts',(11.2657500452716,69.5171900720158,0.));
#101951=CARTESIAN_POINT('Ctrl Pts',(11.2657500452716,69.5171900720158,12.));
#101952=CARTESIAN_POINT('Ctrl Pts',(11.263260954763,69.5376474344771,0.));
#101953=CARTESIAN_POINT('Ctrl Pts',(11.263260954763,69.5376474344771,12.));
#101954=CARTESIAN_POINT('Ctrl Pts',(11.2607441244703,69.5581528662877,0.));
#101955=CARTESIAN_POINT('Ctrl Pts',(11.2607441244703,69.5581528662877,12.));
#101956=CARTESIAN_POINT('Ctrl Pts',(11.2581994939541,69.5787061880857,0.));
#101957=CARTESIAN_POINT('Ctrl Pts',(11.2581994939541,69.5787061880857,12.));
#101958=CARTESIAN_POINT('Ctrl Pts',(11.2556270027016,69.599307219739,0.));
#101959=CARTESIAN_POINT('Ctrl Pts',(11.2556270027016,69.599307219739,12.));
#101960=CARTESIAN_POINT('Ctrl Pts',(11.2530265903557,69.6199557811245,0.));
#101961=CARTESIAN_POINT('Ctrl Pts',(11.2530265903557,69.6199557811245,12.));
#101962=CARTESIAN_POINT('Ctrl Pts',(11.2503981969412,69.6406516928891,0.));
#101963=CARTESIAN_POINT('Ctrl Pts',(11.2503981969412,69.6406516928891,12.));
#101964=CARTESIAN_POINT('Ctrl Pts',(11.2477417631386,69.6613947773534,0.));
#101965=CARTESIAN_POINT('Ctrl Pts',(11.2477417631386,69.6613947773534,12.));
#101966=CARTESIAN_POINT('Ctrl Pts',(11.2450572303841,69.6821848588457,0.));
#101967=CARTESIAN_POINT('Ctrl Pts',(11.2450572303841,69.6821848588457,12.));
#101968=CARTESIAN_POINT('Ctrl Pts',(11.2423445407166,69.7030217632164,0.));
#101969=CARTESIAN_POINT('Ctrl Pts',(11.2423445407166,69.7030217632164,12.));
#101970=CARTESIAN_POINT('Ctrl Pts',(11.239603636686,69.7239053175356,0.));
#101971=CARTESIAN_POINT('Ctrl Pts',(11.239603636686,69.7239053175356,12.));
#101972=CARTESIAN_POINT('Ctrl Pts',(11.2368344612472,69.7448353497408,0.));
#101973=CARTESIAN_POINT('Ctrl Pts',(11.2368344612472,69.7448353497408,12.));
#101974=CARTESIAN_POINT('Ctrl Pts',(11.2340369576456,69.7658116882324,0.));
#101975=CARTESIAN_POINT('Ctrl Pts',(11.2340369576456,69.7658116882324,12.));
#101976=CARTESIAN_POINT('Ctrl Pts',(11.2312110694187,69.7868341618954,0.));
#101977=CARTESIAN_POINT('Ctrl Pts',(11.2312110694187,69.7868341618954,12.));
#101978=CARTESIAN_POINT('Ctrl Pts',(11.2283567404437,69.8079026002768,0.));
#101979=CARTESIAN_POINT('Ctrl Pts',(11.2283567404437,69.8079026002768,12.));
#101980=CARTESIAN_POINT('Ctrl Pts',(11.225473914972,69.8290168337076,0.));
#101981=CARTESIAN_POINT('Ctrl Pts',(11.225473914972,69.8290168337076,12.));
#101982=CARTESIAN_POINT('Ctrl Pts',(11.2225625376736,69.8501766934428,0.));
#101983=CARTESIAN_POINT('Ctrl Pts',(11.2225625376736,69.8501766934428,12.));
#101984=CARTESIAN_POINT('Ctrl Pts',(11.219622553679,69.871382011789,0.));
#101985=CARTESIAN_POINT('Ctrl Pts',(11.219622553679,69.871382011789,12.));
#101986=CARTESIAN_POINT('Ctrl Pts',(11.2166539085523,69.8926326220385,0.));
#101987=CARTESIAN_POINT('Ctrl Pts',(11.2166539085523,69.8926326220385,12.));
#101988=CARTESIAN_POINT('Ctrl Pts',(11.2136565482678,69.9139283584022,0.));
#101989=CARTESIAN_POINT('Ctrl Pts',(11.2136565482678,69.9139283584022,12.));
#101990=CARTESIAN_POINT('Ctrl Pts',(11.2106304191882,69.9352690559405,0.));
#101991=CARTESIAN_POINT('Ctrl Pts',(11.2106304191882,69.9352690559405,12.));
#101992=CARTESIAN_POINT('Ctrl Pts',(11.2075754680449,69.9566545504837,0.));
#101993=CARTESIAN_POINT('Ctrl Pts',(11.2075754680449,69.9566545504837,12.));
#101994=CARTESIAN_POINT('Ctrl Pts',(11.2044916419244,69.97808467858,0.));
#101995=CARTESIAN_POINT('Ctrl Pts',(11.2044916419244,69.97808467858,12.));
#101996=CARTESIAN_POINT('Ctrl Pts',(11.2013788882714,69.9995592775343,0.));
#101997=CARTESIAN_POINT('Ctrl Pts',(11.2013788882714,69.9995592775343,12.));
#101998=CARTESIAN_POINT('Ctrl Pts',(11.1982371548919,70.0210781854243,0.));
#101999=CARTESIAN_POINT('Ctrl Pts',(11.1982371548919,70.0210781854243,12.));
#102000=CARTESIAN_POINT('Ctrl Pts',(11.1950663899576,70.0426412411185,0.));
#102001=CARTESIAN_POINT('Ctrl Pts',(11.1950663899576,70.0426412411185,12.));
#102002=CARTESIAN_POINT('Ctrl Pts',(11.1918665420166,70.0642482842928,0.));
#102003=CARTESIAN_POINT('Ctrl Pts',(11.1918665420166,70.0642482842928,12.));
#102004=CARTESIAN_POINT('Ctrl Pts',(11.1886375599914,70.0858991554283,0.));
#102005=CARTESIAN_POINT('Ctrl Pts',(11.1886375599914,70.0858991554283,12.));
#102006=CARTESIAN_POINT('Ctrl Pts',(11.185379393167,70.1075936957968,0.));
#102007=CARTESIAN_POINT('Ctrl Pts',(11.185379393167,70.1075936957968,12.));
#102008=CARTESIAN_POINT('Ctrl Pts',(11.1820919911846,70.1293317474432,0.));
#102009=CARTESIAN_POINT('Ctrl Pts',(11.1820919911846,70.1293317474432,12.));
#102010=CARTESIAN_POINT('Ctrl Pts',(11.1787753040363,70.1511131531674,0.));
#102011=CARTESIAN_POINT('Ctrl Pts',(11.1787753040363,70.1511131531674,12.));
#102012=CARTESIAN_POINT('Ctrl Pts',(11.1754292820631,70.1729377564956,0.));
#102013=CARTESIAN_POINT('Ctrl Pts',(11.1754292820631,70.1729377564956,12.));
#102014=CARTESIAN_POINT('Ctrl Pts',(11.1720538759499,70.1948054016817,0.));
#102015=CARTESIAN_POINT('Ctrl Pts',(11.1720538759499,70.1948054016817,12.));
#102016=CARTESIAN_POINT('Ctrl Pts',(11.168649036721,70.2167159337095,0.));
#102017=CARTESIAN_POINT('Ctrl Pts',(11.168649036721,70.2167159337095,12.));
#102018=CARTESIAN_POINT('Ctrl Pts',(11.1652147157383,70.2386691982902,0.));
#102019=CARTESIAN_POINT('Ctrl Pts',(11.1652147157383,70.2386691982902,12.));
#102020=CARTESIAN_POINT('Ctrl Pts',(11.1617508647017,70.2606650418589,0.));
#102021=CARTESIAN_POINT('Ctrl Pts',(11.1617508647017,70.2606650418589,12.));
#102022=CARTESIAN_POINT('Ctrl Pts',(11.1582574356522,70.2827033115662,0.));
#102023=CARTESIAN_POINT('Ctrl Pts',(11.1582574356522,70.2827033115662,12.));
#102024=CARTESIAN_POINT('Ctrl Pts',(11.1547343809647,70.3047838552758,0.));
#102025=CARTESIAN_POINT('Ctrl Pts',(11.1547343809647,70.3047838552758,12.));
#102026=CARTESIAN_POINT('Ctrl Pts',(11.1511816533422,70.3269065215591,0.));
#102027=CARTESIAN_POINT('Ctrl Pts',(11.1511816533422,70.3269065215591,12.));
#102028=CARTESIAN_POINT('Ctrl Pts',(11.1475992058124,70.3490711596882,0.));
#102029=CARTESIAN_POINT('Ctrl Pts',(11.1475992058124,70.3490711596882,12.));
#102030=CARTESIAN_POINT('Ctrl Pts',(11.1439869917269,70.3712776196216,0.));
#102031=CARTESIAN_POINT('Ctrl Pts',(11.1439869917269,70.3712776196216,12.));
#102032=CARTESIAN_POINT('Ctrl Pts',(11.1403449647622,70.3935257519945,0.));
#102033=CARTESIAN_POINT('Ctrl Pts',(11.1403449647622,70.3935257519945,12.));
#102034=CARTESIAN_POINT('Ctrl Pts',(11.1366730789122,70.415815408119,0.));
#102035=CARTESIAN_POINT('Ctrl Pts',(11.1366730789122,70.415815408119,12.));
#102036=CARTESIAN_POINT('Ctrl Pts',(11.1329712884845,70.438146439981,0.));
#102037=CARTESIAN_POINT('Ctrl Pts',(11.1329712884845,70.438146439981,12.));
#102038=CARTESIAN_POINT('Ctrl Pts',(11.1292395480975,70.4605187002356,0.));
#102039=CARTESIAN_POINT('Ctrl Pts',(11.1292395480975,70.4605187002356,12.));
#102040=CARTESIAN_POINT('Ctrl Pts',(11.1254778126824,70.4829320421973,0.));
#102041=CARTESIAN_POINT('Ctrl Pts',(11.1254778126824,70.4829320421973,12.));
#102042=CARTESIAN_POINT('Ctrl Pts',(11.121686037483,70.5053863198306,0.));
#102043=CARTESIAN_POINT('Ctrl Pts',(11.121686037483,70.5053863198306,12.));
#102044=CARTESIAN_POINT('Ctrl Pts',(11.117864178048,70.5278813877519,0.));
#102045=CARTESIAN_POINT('Ctrl Pts',(11.117864178048,70.5278813877519,12.));
#102046=CARTESIAN_POINT('Ctrl Pts',(11.1140121902274,70.5504171012247,0.));
#102047=CARTESIAN_POINT('Ctrl Pts',(11.1140121902274,70.5504171012247,12.));
#102048=CARTESIAN_POINT('Ctrl Pts',(11.11013003017,70.5729933161538,0.));
#102049=CARTESIAN_POINT('Ctrl Pts',(11.11013003017,70.5729933161538,12.));
#102050=CARTESIAN_POINT('Ctrl Pts',(11.1062176543257,70.5956098890744,0.));
#102051=CARTESIAN_POINT('Ctrl Pts',(11.1062176543257,70.5956098890744,12.));
#102052=CARTESIAN_POINT('Ctrl Pts',(11.1022750194439,70.6182666771441,0.));
#102053=CARTESIAN_POINT('Ctrl Pts',(11.1022750194439,70.6182666771441,12.));
#102054=CARTESIAN_POINT('Ctrl Pts',(11.0983020825662,70.6409635381446,0.));
#102055=CARTESIAN_POINT('Ctrl Pts',(11.0983020825662,70.6409635381446,12.));
#102056=CARTESIAN_POINT('Ctrl Pts',(11.0942988010231,70.6637003304768,0.));
#102057=CARTESIAN_POINT('Ctrl Pts',(11.0942988010231,70.6637003304768,12.));
#102058=CARTESIAN_POINT('Ctrl Pts',(11.0902651324325,70.686476913156,0.));
#102059=CARTESIAN_POINT('Ctrl Pts',(11.0902651324325,70.686476913156,12.));
#102060=CARTESIAN_POINT('Ctrl Pts',(11.0862010347022,70.7092931457996,0.));
#102061=CARTESIAN_POINT('Ctrl Pts',(11.0862010347022,70.7092931457996,12.));
#102062=CARTESIAN_POINT('Ctrl Pts',(11.0821064660276,70.7321488886229,0.));
#102063=CARTESIAN_POINT('Ctrl Pts',(11.0821064660276,70.7321488886229,12.));
#102064=CARTESIAN_POINT('Ctrl Pts',(11.0779813848851,70.7550440024422,0.));
#102065=CARTESIAN_POINT('Ctrl Pts',(11.0779813848851,70.7550440024422,12.));
#102066=CARTESIAN_POINT('Ctrl Pts',(11.0738257500292,70.7779783486689,0.));
#102067=CARTESIAN_POINT('Ctrl Pts',(11.0738257500292,70.7779783486689,12.));
#102068=CARTESIAN_POINT('Ctrl Pts',(11.0696395204908,70.8009517893042,0.));
#102069=CARTESIAN_POINT('Ctrl Pts',(11.0696395204908,70.8009517893042,12.));
#102070=CARTESIAN_POINT('Ctrl Pts',(11.0654226555798,70.8239641869266,0.));
#102071=CARTESIAN_POINT('Ctrl Pts',(11.0654226555798,70.8239641869266,12.));
#102072=CARTESIAN_POINT('Ctrl Pts',(11.061175114883,70.847015404688,0.));
#102073=CARTESIAN_POINT('Ctrl Pts',(11.061175114883,70.847015404688,12.));
#102074=CARTESIAN_POINT('Ctrl Pts',(11.0568968582566,70.8701053063158,0.));
#102075=CARTESIAN_POINT('Ctrl Pts',(11.0568968582566,70.8701053063158,12.));
#102076=CARTESIAN_POINT('Ctrl Pts',(11.0525878458242,70.8932337561078,0.));
#102077=CARTESIAN_POINT('Ctrl Pts',(11.0525878458242,70.8932337561078,12.));
#102078=CARTESIAN_POINT('Ctrl Pts',(11.0482480379752,70.9164006189283,0.));
#102079=CARTESIAN_POINT('Ctrl Pts',(11.0482480379752,70.9164006189283,12.));
#102080=CARTESIAN_POINT('Ctrl Pts',(11.0438773953686,70.9396057601953,0.));
#102081=CARTESIAN_POINT('Ctrl Pts',(11.0438773953686,70.9396057601953,12.));
#102082=CARTESIAN_POINT('Ctrl Pts',(11.039475878929,70.9628490458779,0.));
#102083=CARTESIAN_POINT('Ctrl Pts',(11.039475878929,70.9628490458779,12.));
#102084=CARTESIAN_POINT('Ctrl Pts',(11.0350434498408,70.9861303424989,0.));
#102085=CARTESIAN_POINT('Ctrl Pts',(11.0350434498408,70.9861303424989,12.));
#102086=CARTESIAN_POINT('Ctrl Pts',(11.0305800695457,71.0094495171295,0.));
#102087=CARTESIAN_POINT('Ctrl Pts',(11.0305800695457,71.0094495171295,12.));
#102088=CARTESIAN_POINT('Ctrl Pts',(11.0260856997414,71.0328064373849,0.));
#102089=CARTESIAN_POINT('Ctrl Pts',(11.0260856997414,71.0328064373849,12.));
#102090=CARTESIAN_POINT('Ctrl Pts',(11.0215603023854,71.0562009714125,0.));
#102091=CARTESIAN_POINT('Ctrl Pts',(11.0215603023854,71.0562009714125,12.));
#102092=CARTESIAN_POINT('Ctrl Pts',(11.0170038396913,71.0796329878896,0.));
#102093=CARTESIAN_POINT('Ctrl Pts',(11.0170038396913,71.0796329878896,12.));
#102094=CARTESIAN_POINT('Ctrl Pts',(11.0124162741223,71.1031023560243,0.));
#102095=CARTESIAN_POINT('Ctrl Pts',(11.0124162741223,71.1031023560243,12.));
#102096=CARTESIAN_POINT('Ctrl Pts',(11.0077975683895,71.1266089455517,0.));
#102097=CARTESIAN_POINT('Ctrl Pts',(11.0077975683895,71.1266089455517,12.));
#102098=CARTESIAN_POINT('Ctrl Pts',(11.0031476854503,71.1501526267288,0.));
#102099=CARTESIAN_POINT('Ctrl Pts',(11.0031476854503,71.1501526267288,12.));
#102100=CARTESIAN_POINT('Ctrl Pts',(10.9984665885127,71.1737332703248,0.));
#102101=CARTESIAN_POINT('Ctrl Pts',(10.9984665885127,71.1737332703248,12.));
#102102=CARTESIAN_POINT('Ctrl Pts',(10.993754241032,71.1973507476188,0.));
#102103=CARTESIAN_POINT('Ctrl Pts',(10.993754241032,71.1973507476188,12.));
#102104=CARTESIAN_POINT('Ctrl Pts',(10.9890106067038,71.221004930401,0.));
#102105=CARTESIAN_POINT('Ctrl Pts',(10.9890106067038,71.221004930401,12.));
#102106=CARTESIAN_POINT('Ctrl Pts',(10.9842356494627,71.2446956909685,0.));
#102107=CARTESIAN_POINT('Ctrl Pts',(10.9842356494627,71.2446956909685,12.));
#102108=CARTESIAN_POINT('Ctrl Pts',(10.9794293334806,71.2684229021209,0.));
#102109=CARTESIAN_POINT('Ctrl Pts',(10.9794293334806,71.2684229021209,12.));
#102110=CARTESIAN_POINT('Ctrl Pts',(10.9745916231711,71.2921864371499,0.));
#102111=CARTESIAN_POINT('Ctrl Pts',(10.9745916231711,71.2921864371499,12.));
#102112=CARTESIAN_POINT('Ctrl Pts',(10.9697224831862,71.3159861698368,0.));
#102113=CARTESIAN_POINT('Ctrl Pts',(10.9697224831862,71.3159861698368,12.));
#102114=CARTESIAN_POINT('Ctrl Pts',(10.96482187841,71.3398219744547,0.));
#102115=CARTESIAN_POINT('Ctrl Pts',(10.96482187841,71.3398219744547,12.));
#102116=CARTESIAN_POINT('Ctrl Pts',(10.9598897739565,71.3636937257651,0.));
#102117=CARTESIAN_POINT('Ctrl Pts',(10.9598897739565,71.3636937257651,12.));
#102118=CARTESIAN_POINT('Ctrl Pts',(10.954926135169,71.3876012990135,0.));
#102119=CARTESIAN_POINT('Ctrl Pts',(10.954926135169,71.3876012990135,12.));
#102120=CARTESIAN_POINT('Ctrl Pts',(10.9499309276235,71.411544569919,0.));
#102121=CARTESIAN_POINT('Ctrl Pts',(10.9499309276235,71.411544569919,12.));
#102122=CARTESIAN_POINT('Ctrl Pts',(10.9449041171269,71.4355234146718,0.));
#102123=CARTESIAN_POINT('Ctrl Pts',(10.9449041171269,71.4355234146718,12.));
#102124=CARTESIAN_POINT('Ctrl Pts',(10.9398456697095,71.4595377099352,0.));
#102125=CARTESIAN_POINT('Ctrl Pts',(10.9398456697095,71.4595377099352,12.));
#102126=CARTESIAN_POINT('Ctrl Pts',(10.9347555516236,71.4835873328425,0.));
#102127=CARTESIAN_POINT('Ctrl Pts',(10.9347555516236,71.4835873328425,12.));
#102128=CARTESIAN_POINT('Ctrl Pts',(10.9296337293425,71.5076721609936,0.));
#102129=CARTESIAN_POINT('Ctrl Pts',(10.9296337293425,71.5076721609936,12.));
#102130=CARTESIAN_POINT('Ctrl Pts',(10.9244801695642,71.5317920724453,0.));
#102131=CARTESIAN_POINT('Ctrl Pts',(10.9244801695642,71.5317920724453,12.));
#102132=CARTESIAN_POINT('Ctrl Pts',(10.9192948392099,71.5559469457082,0.));
#102133=CARTESIAN_POINT('Ctrl Pts',(10.9192948392099,71.5559469457082,12.));
#102134=CARTESIAN_POINT('Ctrl Pts',(10.9140777054169,71.5801366597479,0.));
#102135=CARTESIAN_POINT('Ctrl Pts',(10.9140777054169,71.5801366597479,12.));
#102136=CARTESIAN_POINT('Ctrl Pts',(10.9088287355364,71.604361093983,0.));
#102137=CARTESIAN_POINT('Ctrl Pts',(10.9088287355364,71.604361093983,12.));
#102138=CARTESIAN_POINT('Ctrl Pts',(10.9035478971329,71.6286201282815,0.));
#102139=CARTESIAN_POINT('Ctrl Pts',(10.9035478971329,71.6286201282815,12.));
#102140=CARTESIAN_POINT('Ctrl Pts',(10.8982351579872,71.6529136429515,0.));
#102141=CARTESIAN_POINT('Ctrl Pts',(10.8982351579872,71.6529136429515,12.));
#102142=CARTESIAN_POINT('Ctrl Pts',(10.8928904860967,71.6772415187382,0.));
#102143=CARTESIAN_POINT('Ctrl Pts',(10.8928904860967,71.6772415187382,12.));
#102144=CARTESIAN_POINT('Ctrl Pts',(10.8875138496674,71.7016036368254,0.));
#102145=CARTESIAN_POINT('Ctrl Pts',(10.8875138496674,71.7016036368254,12.));
#102146=CARTESIAN_POINT('Ctrl Pts',(10.8821052171122,71.7259998788337,0.));
#102147=CARTESIAN_POINT('Ctrl Pts',(10.8821052171122,71.7259998788337,12.));
#102148=CARTESIAN_POINT('Ctrl Pts',(10.8766645570496,71.7504301268177,0.));
#102149=CARTESIAN_POINT('Ctrl Pts',(10.8766645570496,71.7504301268177,12.));
#102150=CARTESIAN_POINT('Ctrl Pts',(10.8711918383071,71.7748942632578,0.));
#102151=CARTESIAN_POINT('Ctrl Pts',(10.8711918383071,71.7748942632578,12.));
#102152=CARTESIAN_POINT('Ctrl Pts',(10.8656870299218,71.7993921710546,0.));
#102153=CARTESIAN_POINT('Ctrl Pts',(10.8656870299218,71.7993921710546,12.));
#102154=CARTESIAN_POINT('Ctrl Pts',(10.860150101133,71.8239237335318,0.));
#102155=CARTESIAN_POINT('Ctrl Pts',(10.860150101133,71.8239237335318,12.));
#102156=CARTESIAN_POINT('Ctrl Pts',(10.8545810213799,71.8484888344335,0.));
#102157=CARTESIAN_POINT('Ctrl Pts',(10.8545810213799,71.8484888344335,12.));
#102158=CARTESIAN_POINT('Ctrl Pts',(10.8489797602998,71.8730873579226,0.));
#102159=CARTESIAN_POINT('Ctrl Pts',(10.8489797602998,71.8730873579226,12.));
#102160=CARTESIAN_POINT('Ctrl Pts',(10.8433462877312,71.8977191885726,0.));
#102161=CARTESIAN_POINT('Ctrl Pts',(10.8433462877312,71.8977191885726,12.));
#102162=CARTESIAN_POINT('Ctrl Pts',(10.8376805737158,71.9223842113622,0.));
#102163=CARTESIAN_POINT('Ctrl Pts',(10.8376805737158,71.9223842113622,12.));
#102164=CARTESIAN_POINT('Ctrl Pts',(10.8319825884917,71.9470823116777,0.));
#102165=CARTESIAN_POINT('Ctrl Pts',(10.8319825884917,71.9470823116777,12.));
#102166=CARTESIAN_POINT('Ctrl Pts',(10.8262523024897,71.971813375312,0.));
#102167=CARTESIAN_POINT('Ctrl Pts',(10.8262523024897,71.971813375312,12.));
#102168=CARTESIAN_POINT('Ctrl Pts',(10.8204896863328,71.996577288462,0.));
#102169=CARTESIAN_POINT('Ctrl Pts',(10.8204896863328,71.996577288462,12.));
#102170=CARTESIAN_POINT('Ctrl Pts',(10.8146947108376,72.0213739377231,0.));
#102171=CARTESIAN_POINT('Ctrl Pts',(10.8146947108376,72.0213739377231,12.));
#102172=CARTESIAN_POINT('Ctrl Pts',(10.8088673470187,72.0462032100828,0.));
#102173=CARTESIAN_POINT('Ctrl Pts',(10.8088673470187,72.0462032100828,12.));
#102174=CARTESIAN_POINT('Ctrl Pts',(10.8030075660811,72.0710649929214,0.));
#102175=CARTESIAN_POINT('Ctrl Pts',(10.8030075660811,72.0710649929214,12.));
#102176=CARTESIAN_POINT('Ctrl Pts',(10.7971153394168,72.095959174012,0.));
#102177=CARTESIAN_POINT('Ctrl Pts',(10.7971153394168,72.095959174012,12.));
#102178=CARTESIAN_POINT('Ctrl Pts',(10.7911906386027,72.1208856415171,0.));
#102179=CARTESIAN_POINT('Ctrl Pts',(10.7911906386027,72.1208856415171,12.));
#102180=CARTESIAN_POINT('Ctrl Pts',(10.7852334354015,72.145844283983,0.));
#102181=CARTESIAN_POINT('Ctrl Pts',(10.7852334354015,72.145844283983,12.));
#102182=CARTESIAN_POINT('Ctrl Pts',(10.779243701766,72.17083499033,0.));
#102183=CARTESIAN_POINT('Ctrl Pts',(10.779243701766,72.17083499033,12.));
#102184=CARTESIAN_POINT('Ctrl Pts',(10.7732214098343,72.1958576498556,0.));
#102185=CARTESIAN_POINT('Ctrl Pts',(10.7732214098343,72.1958576498556,12.));
#102186=CARTESIAN_POINT('Ctrl Pts',(10.7671665319254,72.2209121522367,0.));
#102187=CARTESIAN_POINT('Ctrl Pts',(10.7671665319254,72.2209121522367,12.));
#102188=CARTESIAN_POINT('Ctrl Pts',(10.7610790405385,72.2459983875298,0.));
#102189=CARTESIAN_POINT('Ctrl Pts',(10.7610790405385,72.2459983875298,12.));
#102190=CARTESIAN_POINT('Ctrl Pts',(10.7549589083535,72.2711162461679,0.));
#102191=CARTESIAN_POINT('Ctrl Pts',(10.7549589083535,72.2711162461679,12.));
#102192=CARTESIAN_POINT('Ctrl Pts',(10.7488061082368,72.296265618955,0.));
#102193=CARTESIAN_POINT('Ctrl Pts',(10.7488061082368,72.296265618955,12.));
#102194=CARTESIAN_POINT('Ctrl Pts',(10.7426206132375,72.3214463970634,0.));
#102195=CARTESIAN_POINT('Ctrl Pts',(10.7426206132375,72.3214463970634,12.));
#102196=CARTESIAN_POINT('Ctrl Pts',(10.73640239658,72.3466584720311,0.));
#102197=CARTESIAN_POINT('Ctrl Pts',(10.73640239658,72.3466584720311,12.));
#102198=CARTESIAN_POINT('Ctrl Pts',(10.7301514316607,72.3719017357568,0.));
#102199=CARTESIAN_POINT('Ctrl Pts',(10.7301514316607,72.3719017357568,12.));
#102200=CARTESIAN_POINT('Ctrl Pts',(10.7238676920469,72.3971760804935,0.));
#102201=CARTESIAN_POINT('Ctrl Pts',(10.7238676920469,72.3971760804935,12.));
#102202=CARTESIAN_POINT('Ctrl Pts',(10.7175511514789,72.4224813988355,0.));
#102203=CARTESIAN_POINT('Ctrl Pts',(10.7175511514789,72.4224813988355,12.));
#102204=CARTESIAN_POINT('Ctrl Pts',(10.7112017838707,72.4478175837168,0.));
#102205=CARTESIAN_POINT('Ctrl Pts',(10.7112017838707,72.4478175837168,12.));
#102206=CARTESIAN_POINT('Ctrl Pts',(10.7048195633062,72.4731845284238,0.));
#102207=CARTESIAN_POINT('Ctrl Pts',(10.7048195633062,72.4731845284238,12.));
#102208=CARTESIAN_POINT('Ctrl Pts',(10.6984044640399,72.4985821266031,0.));
#102209=CARTESIAN_POINT('Ctrl Pts',(10.6984044640399,72.4985821266031,12.));
#102210=CARTESIAN_POINT('Ctrl Pts',(10.691956460499,72.5240102722662,0.));
#102211=CARTESIAN_POINT('Ctrl Pts',(10.691956460499,72.5240102722662,12.));
#102212=CARTESIAN_POINT('Ctrl Pts',(10.6854755272903,72.5494688597951,0.));
#102213=CARTESIAN_POINT('Ctrl Pts',(10.6854755272903,72.5494688597951,12.));
#102214=CARTESIAN_POINT('Ctrl Pts',(10.6789616392041,72.57495778394,0.));
#102215=CARTESIAN_POINT('Ctrl Pts',(10.6789616392041,72.57495778394,12.));
#102216=CARTESIAN_POINT('Ctrl Pts',(10.6724147711994,72.6004769398004,0.));
#102217=CARTESIAN_POINT('Ctrl Pts',(10.6724147711994,72.6004769398004,12.));
#102218=CARTESIAN_POINT('Ctrl Pts',(10.6658348983944,72.6260262228055,0.));
#102219=CARTESIAN_POINT('Ctrl Pts',(10.6658348983944,72.6260262228055,12.));
#102220=CARTESIAN_POINT('Ctrl Pts',(10.659221996058,72.6516055286908,0.));
#102221=CARTESIAN_POINT('Ctrl Pts',(10.659221996058,72.6516055286908,12.));
#102222=CARTESIAN_POINT('Ctrl Pts',(10.6525760396055,72.6772147534762,0.));
#102223=CARTESIAN_POINT('Ctrl Pts',(10.6525760396055,72.6772147534762,12.));
#102224=CARTESIAN_POINT('Ctrl Pts',(10.6458970045948,72.7028537934332,0.));
#102225=CARTESIAN_POINT('Ctrl Pts',(10.6458970045948,72.7028537934332,12.));
#102226=CARTESIAN_POINT('Ctrl Pts',(10.6391848667354,72.7285225451309,0.));
#102227=CARTESIAN_POINT('Ctrl Pts',(10.6391848667354,72.7285225451309,12.));
#102228=CARTESIAN_POINT('Ctrl Pts',(10.6324396018999,72.7542209054823,0.));
#102229=CARTESIAN_POINT('Ctrl Pts',(10.6324396018999,72.7542209054823,12.));
#102230=CARTESIAN_POINT('Ctrl Pts',(10.6256611861395,72.7799487717914,0.));
#102231=CARTESIAN_POINT('Ctrl Pts',(10.6256611861395,72.7799487717914,12.));
#102232=CARTESIAN_POINT('Ctrl Pts',(10.6188495956973,72.8057060417882,0.));
#102233=CARTESIAN_POINT('Ctrl Pts',(10.6188495956973,72.8057060417882,12.));
#102234=CARTESIAN_POINT('Ctrl Pts',(10.6120048070366,72.8314926136872,0.));
#102235=CARTESIAN_POINT('Ctrl Pts',(10.6120048070366,72.8314926136872,12.));
#102236=CARTESIAN_POINT('Ctrl Pts',(10.6051267968202,72.8573083861328,0.));
#102237=CARTESIAN_POINT('Ctrl Pts',(10.6051267968202,72.8573083861328,12.));
#102238=CARTESIAN_POINT('Ctrl Pts',(10.5982155418625,72.8831532580839,0.));
#102239=CARTESIAN_POINT('Ctrl Pts',(10.5982155418625,72.8831532580839,12.));
#102240=CARTESIAN_POINT('Ctrl Pts',(10.5912710190928,72.9090271287081,0.));
#102241=CARTESIAN_POINT('Ctrl Pts',(10.5912710190928,72.9090271287081,12.));
#102242=CARTESIAN_POINT('Ctrl Pts',(10.5842932055209,72.9349298972823,0.));
#102243=CARTESIAN_POINT('Ctrl Pts',(10.5842932055209,72.9349298972823,12.));
#102244=CARTESIAN_POINT('Ctrl Pts',(10.5772820781959,72.9608614630539,0.));
#102245=CARTESIAN_POINT('Ctrl Pts',(10.5772820781959,72.9608614630539,12.));
#102246=CARTESIAN_POINT('Ctrl Pts',(10.5702376142052,72.9868217252293,0.));
#102247=CARTESIAN_POINT('Ctrl Pts',(10.5702376142052,72.9868217252293,12.));
#102248=CARTESIAN_POINT('Ctrl Pts',(10.5631597907653,73.0128105832635,0.));
#102249=CARTESIAN_POINT('Ctrl Pts',(10.5631597907653,73.0128105832635,12.));
#102250=CARTESIAN_POINT('Ctrl Pts',(10.5560485852975,73.0388279370845,0.));
#102251=CARTESIAN_POINT('Ctrl Pts',(10.5560485852975,73.0388279370845,12.));
#102252=CARTESIAN_POINT('Ctrl Pts',(10.5489039755138,73.0648736873435,0.));
#102253=CARTESIAN_POINT('Ctrl Pts',(10.5489039755138,73.0648736873435,12.));
#102254=CARTESIAN_POINT('Ctrl Pts',(10.5417259395001,73.090947735646,0.));
#102255=CARTESIAN_POINT('Ctrl Pts',(10.5417259395001,73.090947735646,12.));
#102256=CARTESIAN_POINT('Ctrl Pts',(10.5345144558097,73.1170499848012,0.));
#102257=CARTESIAN_POINT('Ctrl Pts',(10.5345144558097,73.1170499848012,12.));
#102258=CARTESIAN_POINT('Ctrl Pts',(10.5272695032649,73.1431803382677,0.));
#102259=CARTESIAN_POINT('Ctrl Pts',(10.5272695032649,73.1431803382677,12.));
#102260=CARTESIAN_POINT('Ctrl Pts',(10.5199910607652,73.169338699611,0.));
#102261=CARTESIAN_POINT('Ctrl Pts',(10.5199910607652,73.169338699611,12.));
#102262=CARTESIAN_POINT('Ctrl Pts',(10.5126791070804,73.1955249719037,0.));
#102263=CARTESIAN_POINT('Ctrl Pts',(10.5126791070804,73.1955249719037,12.));
#102264=CARTESIAN_POINT('Ctrl Pts',(10.505333620691,73.2217390572578,0.));
#102265=CARTESIAN_POINT('Ctrl Pts',(10.505333620691,73.2217390572578,12.));
#102266=CARTESIAN_POINT('Ctrl Pts',(10.4979545795197,73.247980856023,0.));
#102267=CARTESIAN_POINT('Ctrl Pts',(10.4979545795197,73.247980856023,12.));
#102268=CARTESIAN_POINT('Ctrl Pts',(10.4905419611529,73.2742502674361,0.));
#102269=CARTESIAN_POINT('Ctrl Pts',(10.4905419611529,73.2742502674361,12.));
#102270=CARTESIAN_POINT('Ctrl Pts',(10.4830957433311,73.3005471910639,0.));
#102271=CARTESIAN_POINT('Ctrl Pts',(10.4830957433311,73.3005471910639,12.));
#102272=CARTESIAN_POINT('Ctrl Pts',(10.475615904381,73.3268715280609,0.));
#102273=CARTESIAN_POINT('Ctrl Pts',(10.475615904381,73.3268715280609,12.));
#102274=CARTESIAN_POINT('Ctrl Pts',(10.4681024236288,73.353223182365,0.));
#102275=CARTESIAN_POINT('Ctrl Pts',(10.4681024236288,73.353223182365,12.));
#102276=CARTESIAN_POINT('Ctrl Pts',(10.4605552819391,73.3796020622437,0.));
#102277=CARTESIAN_POINT('Ctrl Pts',(10.4605552819391,73.3796020622437,12.));
#102278=CARTESIAN_POINT('Ctrl Pts',(10.4529744618438,73.4060080806578,0.));
#102279=CARTESIAN_POINT('Ctrl Pts',(10.4529744618438,73.4060080806578,12.));
#102280=CARTESIAN_POINT('Ctrl Pts',(10.4453599463534,73.432441151843,0.));
#102281=CARTESIAN_POINT('Ctrl Pts',(10.4453599463534,73.432441151843,12.));
#102282=CARTESIAN_POINT('Ctrl Pts',(10.4377117180212,73.45890118861,0.));
#102283=CARTESIAN_POINT('Ctrl Pts',(10.4377117180212,73.45890118861,12.));
#102284=CARTESIAN_POINT('Ctrl Pts',(10.4300297578648,73.4853880992228,0.));
#102285=CARTESIAN_POINT('Ctrl Pts',(10.4300297578648,73.4853880992228,12.));
#102286=CARTESIAN_POINT('Ctrl Pts',(10.4223140444615,73.5119017847664,0.));
#102287=CARTESIAN_POINT('Ctrl Pts',(10.4223140444615,73.5119017847664,12.));
#102288=CARTESIAN_POINT('Ctrl Pts',(10.4145645526832,73.5384421354746,0.));
#102289=CARTESIAN_POINT('Ctrl Pts',(10.4145645526832,73.5384421354746,12.));
#102290=CARTESIAN_POINT('Ctrl Pts',(10.4067812555539,73.5650090360114,0.));
#102291=CARTESIAN_POINT('Ctrl Pts',(10.4067812555539,73.5650090360114,12.));
#102292=CARTESIAN_POINT('Ctrl Pts',(10.3989641265313,73.5916023719976,0.));
#102293=CARTESIAN_POINT('Ctrl Pts',(10.3989641265313,73.5916023719976,12.));
#102294=CARTESIAN_POINT('Ctrl Pts',(10.3911131417478,73.6182220363295,0.));
#102295=CARTESIAN_POINT('Ctrl Pts',(10.3911131417478,73.6182220363295,12.));
#102296=CARTESIAN_POINT('Ctrl Pts',(10.3832282820362,73.6448679350605,0.));
#102297=CARTESIAN_POINT('Ctrl Pts',(10.3832282820362,73.6448679350605,12.));
#102298=CARTESIAN_POINT('Ctrl Pts',(10.3753095356302,73.6715399947459,0.));
#102299=CARTESIAN_POINT('Ctrl Pts',(10.3753095356302,73.6715399947459,12.));
#102300=CARTESIAN_POINT('Ctrl Pts',(10.3673568984515,73.6982381644571,0.));
#102301=CARTESIAN_POINT('Ctrl Pts',(10.3673568984515,73.6982381644571,12.));
#102302=CARTESIAN_POINT('Ctrl Pts',(10.3593703712542,73.7249624108433,0.));
#102303=CARTESIAN_POINT('Ctrl Pts',(10.3593703712542,73.7249624108433,12.));
#102304=CARTESIAN_POINT('Ctrl Pts',(10.3529540403026,73.7463626541235,0.));
#102305=CARTESIAN_POINT('Ctrl Pts',(10.3529540403026,73.7463626541235,12.));
#102306=CARTESIAN_POINT('Ctrl Pts',(10.3481265449303,73.7624245587416,0.));
#102307=CARTESIAN_POINT('Ctrl Pts',(10.3481265449303,73.7624245587416,12.));
#102308=CARTESIAN_POINT('Ctrl Pts',(10.3449014384439,73.7731377047922,0.));
#102309=CARTESIAN_POINT('Ctrl Pts',(10.3449014384439,73.7731377047922,12.));
#102310=CARTESIAN_POINT('Ctrl Pts',(10.343287191141,73.778495580227,0.));
#102311=CARTESIAN_POINT('Ctrl Pts',(10.343287191141,73.778495580227,12.));
#102312=CARTESIAN_POINT('',(11.3136138754165,69.079679653846,0.));
#102313=CARTESIAN_POINT('Ctrl Pts',(11.3136138754165,69.079679653846,0.));
#102314=CARTESIAN_POINT('Ctrl Pts',(11.3132375200165,69.0835449954396,0.));
#102315=CARTESIAN_POINT('Ctrl Pts',(11.3124821678798,69.0912808656811,0.));
#102316=CARTESIAN_POINT('Ctrl Pts',(11.3113412156661,69.1029002322118,0.));
#102317=CARTESIAN_POINT('Ctrl Pts',(11.3098040973713,69.118423844466,0.));
#102318=CARTESIAN_POINT('Ctrl Pts',(11.3078562764384,69.1378802251711,0.));
#102319=CARTESIAN_POINT('Ctrl Pts',(11.3058820128307,69.1573884361,0.));
#102320=CARTESIAN_POINT('Ctrl Pts',(11.3038812726292,69.1769483991721,0.));
#102321=CARTESIAN_POINT('Ctrl Pts',(11.3018540025638,69.1965599718914,0.));
#102322=CARTESIAN_POINT('Ctrl Pts',(11.2998001310964,69.2162229488531,0.));
#102323=CARTESIAN_POINT('Ctrl Pts',(11.2977195764852,69.2359370894907,0.));
#102324=CARTESIAN_POINT('Ctrl Pts',(11.2956122531375,69.2557021393351,0.));
#102325=CARTESIAN_POINT('Ctrl Pts',(11.2934780784351,69.275517853148,0.));
#102326=CARTESIAN_POINT('Ctrl Pts',(11.2913169799628,69.295384019272,0.));
#102327=CARTESIAN_POINT('Ctrl Pts',(11.2891288931517,69.3153004517783,0.));
#102328=CARTESIAN_POINT('Ctrl Pts',(11.2869137578459,69.3352669789587,0.));
#102329=CARTESIAN_POINT('Ctrl Pts',(11.2846715154524,69.3552834337784,0.));
#102330=CARTESIAN_POINT('Ctrl Pts',(11.2824021054045,69.3753496420039,0.));
#102331=CARTESIAN_POINT('Ctrl Pts',(11.2801054633816,69.3954654162281,0.));
#102332=CARTESIAN_POINT('Ctrl Pts',(11.2777815231469,69.4156305620593,0.));
#102333=CARTESIAN_POINT('Ctrl Pts',(11.2754302177021,69.4358448819967,0.));
#102334=CARTESIAN_POINT('Ctrl Pts',(11.2730514806139,69.456108179879,0.));
#102335=CARTESIAN_POINT('Ctrl Pts',(11.270645247528,69.4764202659397,0.));
#102336=CARTESIAN_POINT('Ctrl Pts',(11.2682114561008,69.4967809565929,0.));
#102337=CARTESIAN_POINT('Ctrl Pts',(11.2657500452716,69.5171900720158,0.));
#102338=CARTESIAN_POINT('Ctrl Pts',(11.263260954763,69.5376474344771,0.));
#102339=CARTESIAN_POINT('Ctrl Pts',(11.2607441244703,69.5581528662877,0.));
#102340=CARTESIAN_POINT('Ctrl Pts',(11.2581994939541,69.5787061880857,0.));
#102341=CARTESIAN_POINT('Ctrl Pts',(11.2556270027016,69.599307219739,0.));
#102342=CARTESIAN_POINT('Ctrl Pts',(11.2530265903557,69.6199557811245,0.));
#102343=CARTESIAN_POINT('Ctrl Pts',(11.2503981969412,69.6406516928891,0.));
#102344=CARTESIAN_POINT('Ctrl Pts',(11.2477417631386,69.6613947773534,0.));
#102345=CARTESIAN_POINT('Ctrl Pts',(11.2450572303841,69.6821848588457,0.));
#102346=CARTESIAN_POINT('Ctrl Pts',(11.2423445407166,69.7030217632164,0.));
#102347=CARTESIAN_POINT('Ctrl Pts',(11.239603636686,69.7239053175356,0.));
#102348=CARTESIAN_POINT('Ctrl Pts',(11.2368344612472,69.7448353497408,0.));
#102349=CARTESIAN_POINT('Ctrl Pts',(11.2340369576456,69.7658116882324,0.));
#102350=CARTESIAN_POINT('Ctrl Pts',(11.2312110694187,69.7868341618954,0.));
#102351=CARTESIAN_POINT('Ctrl Pts',(11.2283567404437,69.8079026002768,0.));
#102352=CARTESIAN_POINT('Ctrl Pts',(11.225473914972,69.8290168337076,0.));
#102353=CARTESIAN_POINT('Ctrl Pts',(11.2225625376736,69.8501766934428,0.));
#102354=CARTESIAN_POINT('Ctrl Pts',(11.219622553679,69.871382011789,0.));
#102355=CARTESIAN_POINT('Ctrl Pts',(11.2166539085523,69.8926326220385,0.));
#102356=CARTESIAN_POINT('Ctrl Pts',(11.2136565482678,69.9139283584022,0.));
#102357=CARTESIAN_POINT('Ctrl Pts',(11.2106304191882,69.9352690559405,0.));
#102358=CARTESIAN_POINT('Ctrl Pts',(11.2075754680449,69.9566545504837,0.));
#102359=CARTESIAN_POINT('Ctrl Pts',(11.2044916419244,69.97808467858,0.));
#102360=CARTESIAN_POINT('Ctrl Pts',(11.2013788882714,69.9995592775343,0.));
#102361=CARTESIAN_POINT('Ctrl Pts',(11.1982371548919,70.0210781854243,0.));
#102362=CARTESIAN_POINT('Ctrl Pts',(11.1950663899576,70.0426412411185,0.));
#102363=CARTESIAN_POINT('Ctrl Pts',(11.1918665420166,70.0642482842928,0.));
#102364=CARTESIAN_POINT('Ctrl Pts',(11.1886375599914,70.0858991554283,0.));
#102365=CARTESIAN_POINT('Ctrl Pts',(11.185379393167,70.1075936957968,0.));
#102366=CARTESIAN_POINT('Ctrl Pts',(11.1820919911846,70.1293317474432,0.));
#102367=CARTESIAN_POINT('Ctrl Pts',(11.1787753040363,70.1511131531674,0.));
#102368=CARTESIAN_POINT('Ctrl Pts',(11.1754292820631,70.1729377564956,0.));
#102369=CARTESIAN_POINT('Ctrl Pts',(11.1720538759499,70.1948054016817,0.));
#102370=CARTESIAN_POINT('Ctrl Pts',(11.168649036721,70.2167159337095,0.));
#102371=CARTESIAN_POINT('Ctrl Pts',(11.1652147157383,70.2386691982902,0.));
#102372=CARTESIAN_POINT('Ctrl Pts',(11.1617508647017,70.2606650418589,0.));
#102373=CARTESIAN_POINT('Ctrl Pts',(11.1582574356522,70.2827033115662,0.));
#102374=CARTESIAN_POINT('Ctrl Pts',(11.1547343809647,70.3047838552758,0.));
#102375=CARTESIAN_POINT('Ctrl Pts',(11.1511816533422,70.3269065215591,0.));
#102376=CARTESIAN_POINT('Ctrl Pts',(11.1475992058124,70.3490711596882,0.));
#102377=CARTESIAN_POINT('Ctrl Pts',(11.1439869917269,70.3712776196216,0.));
#102378=CARTESIAN_POINT('Ctrl Pts',(11.1403449647622,70.3935257519945,0.));
#102379=CARTESIAN_POINT('Ctrl Pts',(11.1366730789122,70.415815408119,0.));
#102380=CARTESIAN_POINT('Ctrl Pts',(11.1329712884845,70.438146439981,0.));
#102381=CARTESIAN_POINT('Ctrl Pts',(11.1292395480975,70.4605187002356,0.));
#102382=CARTESIAN_POINT('Ctrl Pts',(11.1254778126824,70.4829320421973,0.));
#102383=CARTESIAN_POINT('Ctrl Pts',(11.121686037483,70.5053863198306,0.));
#102384=CARTESIAN_POINT('Ctrl Pts',(11.117864178048,70.5278813877519,0.));
#102385=CARTESIAN_POINT('Ctrl Pts',(11.1140121902274,70.5504171012247,0.));
#102386=CARTESIAN_POINT('Ctrl Pts',(11.11013003017,70.5729933161538,0.));
#102387=CARTESIAN_POINT('Ctrl Pts',(11.1062176543257,70.5956098890744,0.));
#102388=CARTESIAN_POINT('Ctrl Pts',(11.1022750194439,70.6182666771441,0.));
#102389=CARTESIAN_POINT('Ctrl Pts',(11.0983020825662,70.6409635381446,0.));
#102390=CARTESIAN_POINT('Ctrl Pts',(11.0942988010231,70.6637003304768,0.));
#102391=CARTESIAN_POINT('Ctrl Pts',(11.0902651324325,70.686476913156,0.));
#102392=CARTESIAN_POINT('Ctrl Pts',(11.0862010347022,70.7092931457996,0.));
#102393=CARTESIAN_POINT('Ctrl Pts',(11.0821064660276,70.7321488886229,0.));
#102394=CARTESIAN_POINT('Ctrl Pts',(11.0779813848851,70.7550440024422,0.));
#102395=CARTESIAN_POINT('Ctrl Pts',(11.0738257500292,70.7779783486689,0.));
#102396=CARTESIAN_POINT('Ctrl Pts',(11.0696395204908,70.8009517893042,0.));
#102397=CARTESIAN_POINT('Ctrl Pts',(11.0654226555798,70.8239641869266,0.));
#102398=CARTESIAN_POINT('Ctrl Pts',(11.061175114883,70.847015404688,0.));
#102399=CARTESIAN_POINT('Ctrl Pts',(11.0568968582566,70.8701053063158,0.));
#102400=CARTESIAN_POINT('Ctrl Pts',(11.0525878458242,70.8932337561078,0.));
#102401=CARTESIAN_POINT('Ctrl Pts',(11.0482480379752,70.9164006189283,0.));
#102402=CARTESIAN_POINT('Ctrl Pts',(11.0438773953686,70.9396057601953,0.));
#102403=CARTESIAN_POINT('Ctrl Pts',(11.039475878929,70.9628490458779,0.));
#102404=CARTESIAN_POINT('Ctrl Pts',(11.0350434498408,70.9861303424989,0.));
#102405=CARTESIAN_POINT('Ctrl Pts',(11.0305800695457,71.0094495171295,0.));
#102406=CARTESIAN_POINT('Ctrl Pts',(11.0260856997414,71.0328064373849,0.));
#102407=CARTESIAN_POINT('Ctrl Pts',(11.0215603023854,71.0562009714125,0.));
#102408=CARTESIAN_POINT('Ctrl Pts',(11.0170038396913,71.0796329878896,0.));
#102409=CARTESIAN_POINT('Ctrl Pts',(11.0124162741223,71.1031023560243,0.));
#102410=CARTESIAN_POINT('Ctrl Pts',(11.0077975683895,71.1266089455517,0.));
#102411=CARTESIAN_POINT('Ctrl Pts',(11.0031476854503,71.1501526267288,0.));
#102412=CARTESIAN_POINT('Ctrl Pts',(10.9984665885127,71.1737332703248,0.));
#102413=CARTESIAN_POINT('Ctrl Pts',(10.993754241032,71.1973507476188,0.));
#102414=CARTESIAN_POINT('Ctrl Pts',(10.9890106067038,71.221004930401,0.));
#102415=CARTESIAN_POINT('Ctrl Pts',(10.9842356494627,71.2446956909685,0.));
#102416=CARTESIAN_POINT('Ctrl Pts',(10.9794293334806,71.2684229021209,0.));
#102417=CARTESIAN_POINT('Ctrl Pts',(10.9745916231711,71.2921864371499,0.));
#102418=CARTESIAN_POINT('Ctrl Pts',(10.9697224831862,71.3159861698368,0.));
#102419=CARTESIAN_POINT('Ctrl Pts',(10.96482187841,71.3398219744547,0.));
#102420=CARTESIAN_POINT('Ctrl Pts',(10.9598897739565,71.3636937257651,0.));
#102421=CARTESIAN_POINT('Ctrl Pts',(10.954926135169,71.3876012990135,0.));
#102422=CARTESIAN_POINT('Ctrl Pts',(10.9499309276235,71.411544569919,0.));
#102423=CARTESIAN_POINT('Ctrl Pts',(10.9449041171269,71.4355234146718,0.));
#102424=CARTESIAN_POINT('Ctrl Pts',(10.9398456697095,71.4595377099352,0.));
#102425=CARTESIAN_POINT('Ctrl Pts',(10.9347555516236,71.4835873328425,0.));
#102426=CARTESIAN_POINT('Ctrl Pts',(10.9296337293425,71.5076721609936,0.));
#102427=CARTESIAN_POINT('Ctrl Pts',(10.9244801695642,71.5317920724453,0.));
#102428=CARTESIAN_POINT('Ctrl Pts',(10.9192948392099,71.5559469457082,0.));
#102429=CARTESIAN_POINT('Ctrl Pts',(10.9140777054169,71.5801366597479,0.));
#102430=CARTESIAN_POINT('Ctrl Pts',(10.9088287355364,71.604361093983,0.));
#102431=CARTESIAN_POINT('Ctrl Pts',(10.9035478971329,71.6286201282815,0.));
#102432=CARTESIAN_POINT('Ctrl Pts',(10.8982351579872,71.6529136429515,0.));
#102433=CARTESIAN_POINT('Ctrl Pts',(10.8928904860967,71.6772415187382,0.));
#102434=CARTESIAN_POINT('Ctrl Pts',(10.8875138496674,71.7016036368254,0.));
#102435=CARTESIAN_POINT('Ctrl Pts',(10.8821052171122,71.7259998788337,0.));
#102436=CARTESIAN_POINT('Ctrl Pts',(10.8766645570496,71.7504301268177,0.));
#102437=CARTESIAN_POINT('Ctrl Pts',(10.8711918383071,71.7748942632578,0.));
#102438=CARTESIAN_POINT('Ctrl Pts',(10.8656870299218,71.7993921710546,0.));
#102439=CARTESIAN_POINT('Ctrl Pts',(10.860150101133,71.8239237335318,0.));
#102440=CARTESIAN_POINT('Ctrl Pts',(10.8545810213799,71.8484888344335,0.));
#102441=CARTESIAN_POINT('Ctrl Pts',(10.8489797602998,71.8730873579226,0.));
#102442=CARTESIAN_POINT('Ctrl Pts',(10.8433462877312,71.8977191885726,0.));
#102443=CARTESIAN_POINT('Ctrl Pts',(10.8376805737158,71.9223842113622,0.));
#102444=CARTESIAN_POINT('Ctrl Pts',(10.8319825884917,71.9470823116777,0.));
#102445=CARTESIAN_POINT('Ctrl Pts',(10.8262523024897,71.971813375312,0.));
#102446=CARTESIAN_POINT('Ctrl Pts',(10.8204896863328,71.996577288462,0.));
#102447=CARTESIAN_POINT('Ctrl Pts',(10.8146947108376,72.0213739377231,0.));
#102448=CARTESIAN_POINT('Ctrl Pts',(10.8088673470187,72.0462032100828,0.));
#102449=CARTESIAN_POINT('Ctrl Pts',(10.8030075660811,72.0710649929214,0.));
#102450=CARTESIAN_POINT('Ctrl Pts',(10.7971153394168,72.095959174012,0.));
#102451=CARTESIAN_POINT('Ctrl Pts',(10.7911906386027,72.1208856415171,0.));
#102452=CARTESIAN_POINT('Ctrl Pts',(10.7852334354015,72.145844283983,0.));
#102453=CARTESIAN_POINT('Ctrl Pts',(10.779243701766,72.17083499033,0.));
#102454=CARTESIAN_POINT('Ctrl Pts',(10.7732214098343,72.1958576498556,0.));
#102455=CARTESIAN_POINT('Ctrl Pts',(10.7671665319254,72.2209121522367,0.));
#102456=CARTESIAN_POINT('Ctrl Pts',(10.7610790405385,72.2459983875298,0.));
#102457=CARTESIAN_POINT('Ctrl Pts',(10.7549589083535,72.2711162461679,0.));
#102458=CARTESIAN_POINT('Ctrl Pts',(10.7488061082368,72.296265618955,0.));
#102459=CARTESIAN_POINT('Ctrl Pts',(10.7426206132375,72.3214463970634,0.));
#102460=CARTESIAN_POINT('Ctrl Pts',(10.73640239658,72.3466584720311,0.));
#102461=CARTESIAN_POINT('Ctrl Pts',(10.7301514316607,72.3719017357568,0.));
#102462=CARTESIAN_POINT('Ctrl Pts',(10.7238676920469,72.3971760804935,0.));
#102463=CARTESIAN_POINT('Ctrl Pts',(10.7175511514789,72.4224813988355,0.));
#102464=CARTESIAN_POINT('Ctrl Pts',(10.7112017838707,72.4478175837168,0.));
#102465=CARTESIAN_POINT('Ctrl Pts',(10.7048195633062,72.4731845284238,0.));
#102466=CARTESIAN_POINT('Ctrl Pts',(10.6984044640399,72.4985821266031,0.));
#102467=CARTESIAN_POINT('Ctrl Pts',(10.691956460499,72.5240102722662,0.));
#102468=CARTESIAN_POINT('Ctrl Pts',(10.6854755272903,72.5494688597951,0.));
#102469=CARTESIAN_POINT('Ctrl Pts',(10.6789616392041,72.57495778394,0.));
#102470=CARTESIAN_POINT('Ctrl Pts',(10.6724147711994,72.6004769398004,0.));
#102471=CARTESIAN_POINT('Ctrl Pts',(10.6658348983944,72.6260262228055,0.));
#102472=CARTESIAN_POINT('Ctrl Pts',(10.659221996058,72.6516055286908,0.));
#102473=CARTESIAN_POINT('Ctrl Pts',(10.6525760396055,72.6772147534762,0.));
#102474=CARTESIAN_POINT('Ctrl Pts',(10.6458970045948,72.7028537934332,0.));
#102475=CARTESIAN_POINT('Ctrl Pts',(10.6391848667354,72.7285225451309,0.));
#102476=CARTESIAN_POINT('Ctrl Pts',(10.6324396018999,72.7542209054823,0.));
#102477=CARTESIAN_POINT('Ctrl Pts',(10.6256611861395,72.7799487717914,0.));
#102478=CARTESIAN_POINT('Ctrl Pts',(10.6188495956973,72.8057060417882,0.));
#102479=CARTESIAN_POINT('Ctrl Pts',(10.6120048070366,72.8314926136872,0.));
#102480=CARTESIAN_POINT('Ctrl Pts',(10.6051267968202,72.8573083861328,0.));
#102481=CARTESIAN_POINT('Ctrl Pts',(10.5982155418625,72.8831532580839,0.));
#102482=CARTESIAN_POINT('Ctrl Pts',(10.5912710190928,72.9090271287081,0.));
#102483=CARTESIAN_POINT('Ctrl Pts',(10.5842932055209,72.9349298972823,0.));
#102484=CARTESIAN_POINT('Ctrl Pts',(10.5772820781959,72.9608614630539,0.));
#102485=CARTESIAN_POINT('Ctrl Pts',(10.5702376142052,72.9868217252293,0.));
#102486=CARTESIAN_POINT('Ctrl Pts',(10.5631597907653,73.0128105832635,0.));
#102487=CARTESIAN_POINT('Ctrl Pts',(10.5560485852975,73.0388279370845,0.));
#102488=CARTESIAN_POINT('Ctrl Pts',(10.5489039755138,73.0648736873435,0.));
#102489=CARTESIAN_POINT('Ctrl Pts',(10.5417259395001,73.090947735646,0.));
#102490=CARTESIAN_POINT('Ctrl Pts',(10.5345144558097,73.1170499848012,0.));
#102491=CARTESIAN_POINT('Ctrl Pts',(10.5272695032649,73.1431803382677,0.));
#102492=CARTESIAN_POINT('Ctrl Pts',(10.5199910607652,73.169338699611,0.));
#102493=CARTESIAN_POINT('Ctrl Pts',(10.5126791070804,73.1955249719037,0.));
#102494=CARTESIAN_POINT('Ctrl Pts',(10.505333620691,73.2217390572578,0.));
#102495=CARTESIAN_POINT('Ctrl Pts',(10.4979545795197,73.247980856023,0.));
#102496=CARTESIAN_POINT('Ctrl Pts',(10.4905419611529,73.2742502674361,0.));
#102497=CARTESIAN_POINT('Ctrl Pts',(10.4830957433311,73.3005471910639,0.));
#102498=CARTESIAN_POINT('Ctrl Pts',(10.475615904381,73.3268715280609,0.));
#102499=CARTESIAN_POINT('Ctrl Pts',(10.4681024236288,73.353223182365,0.));
#102500=CARTESIAN_POINT('Ctrl Pts',(10.4605552819391,73.3796020622437,0.));
#102501=CARTESIAN_POINT('Ctrl Pts',(10.4529744618438,73.4060080806578,0.));
#102502=CARTESIAN_POINT('Ctrl Pts',(10.4464473465487,73.4286663447915,0.));
#102503=CARTESIAN_POINT('Ctrl Pts',(10.4414249334768,73.446052552855,0.));
#102504=CARTESIAN_POINT('Ctrl Pts',(10.4379221501093,73.4581547436539,0.));
#102505=CARTESIAN_POINT('Ctrl Pts',(10.4359488742883,73.4649650361539,0.));
#102506=CARTESIAN_POINT('Ctrl Pts',(10.4355099267391,73.4664795929517,0.));
#102507=CARTESIAN_POINT('',(11.3136138754165,69.079679653846,12.));
#102508=CARTESIAN_POINT('',(11.3136138754165,69.079679653846,0.));
#102509=CARTESIAN_POINT('Ctrl Pts',(10.4355099267391,73.4664795929518,12.));
#102510=CARTESIAN_POINT('Ctrl Pts',(10.4359488742883,73.4649650361539,12.));
#102511=CARTESIAN_POINT('Ctrl Pts',(10.4379221501093,73.4581547436539,12.));
#102512=CARTESIAN_POINT('Ctrl Pts',(10.4414249334768,73.446052552855,12.));
#102513=CARTESIAN_POINT('Ctrl Pts',(10.4464473465487,73.4286663447915,12.));
#102514=CARTESIAN_POINT('Ctrl Pts',(10.4529744618438,73.4060080806578,12.));
#102515=CARTESIAN_POINT('Ctrl Pts',(10.4605552819391,73.3796020622437,12.));
#102516=CARTESIAN_POINT('Ctrl Pts',(10.4681024236288,73.353223182365,12.));
#102517=CARTESIAN_POINT('Ctrl Pts',(10.475615904381,73.3268715280609,12.));
#102518=CARTESIAN_POINT('Ctrl Pts',(10.4830957433311,73.3005471910639,12.));
#102519=CARTESIAN_POINT('Ctrl Pts',(10.4905419611529,73.2742502674361,12.));
#102520=CARTESIAN_POINT('Ctrl Pts',(10.4979545795197,73.247980856023,12.));
#102521=CARTESIAN_POINT('Ctrl Pts',(10.505333620691,73.2217390572578,12.));
#102522=CARTESIAN_POINT('Ctrl Pts',(10.5126791070804,73.1955249719037,12.));
#102523=CARTESIAN_POINT('Ctrl Pts',(10.5199910607652,73.169338699611,12.));
#102524=CARTESIAN_POINT('Ctrl Pts',(10.5272695032649,73.1431803382677,12.));
#102525=CARTESIAN_POINT('Ctrl Pts',(10.5345144558097,73.1170499848012,12.));
#102526=CARTESIAN_POINT('Ctrl Pts',(10.5417259395001,73.090947735646,12.));
#102527=CARTESIAN_POINT('Ctrl Pts',(10.5489039755138,73.0648736873435,12.));
#102528=CARTESIAN_POINT('Ctrl Pts',(10.5560485852975,73.0388279370845,12.));
#102529=CARTESIAN_POINT('Ctrl Pts',(10.5631597907653,73.0128105832635,12.));
#102530=CARTESIAN_POINT('Ctrl Pts',(10.5702376142052,72.9868217252293,12.));
#102531=CARTESIAN_POINT('Ctrl Pts',(10.5772820781959,72.9608614630539,12.));
#102532=CARTESIAN_POINT('Ctrl Pts',(10.5842932055209,72.9349298972823,12.));
#102533=CARTESIAN_POINT('Ctrl Pts',(10.5912710190928,72.9090271287081,12.));
#102534=CARTESIAN_POINT('Ctrl Pts',(10.5982155418625,72.8831532580839,12.));
#102535=CARTESIAN_POINT('Ctrl Pts',(10.6051267968202,72.8573083861328,12.));
#102536=CARTESIAN_POINT('Ctrl Pts',(10.6120048070366,72.8314926136872,12.));
#102537=CARTESIAN_POINT('Ctrl Pts',(10.6188495956973,72.8057060417882,12.));
#102538=CARTESIAN_POINT('Ctrl Pts',(10.6256611861395,72.7799487717914,12.));
#102539=CARTESIAN_POINT('Ctrl Pts',(10.6324396018999,72.7542209054823,12.));
#102540=CARTESIAN_POINT('Ctrl Pts',(10.6391848667354,72.7285225451309,12.));
#102541=CARTESIAN_POINT('Ctrl Pts',(10.6458970045948,72.7028537934332,12.));
#102542=CARTESIAN_POINT('Ctrl Pts',(10.6525760396055,72.6772147534762,12.));
#102543=CARTESIAN_POINT('Ctrl Pts',(10.659221996058,72.6516055286908,12.));
#102544=CARTESIAN_POINT('Ctrl Pts',(10.6658348983944,72.6260262228055,12.));
#102545=CARTESIAN_POINT('Ctrl Pts',(10.6724147711994,72.6004769398004,12.));
#102546=CARTESIAN_POINT('Ctrl Pts',(10.6789616392041,72.57495778394,12.));
#102547=CARTESIAN_POINT('Ctrl Pts',(10.6854755272903,72.5494688597951,12.));
#102548=CARTESIAN_POINT('Ctrl Pts',(10.691956460499,72.5240102722662,12.));
#102549=CARTESIAN_POINT('Ctrl Pts',(10.6984044640399,72.4985821266031,12.));
#102550=CARTESIAN_POINT('Ctrl Pts',(10.7048195633062,72.4731845284238,12.));
#102551=CARTESIAN_POINT('Ctrl Pts',(10.7112017838707,72.4478175837168,12.));
#102552=CARTESIAN_POINT('Ctrl Pts',(10.7175511514789,72.4224813988355,12.));
#102553=CARTESIAN_POINT('Ctrl Pts',(10.7238676920469,72.3971760804935,12.));
#102554=CARTESIAN_POINT('Ctrl Pts',(10.7301514316607,72.3719017357568,12.));
#102555=CARTESIAN_POINT('Ctrl Pts',(10.73640239658,72.3466584720311,12.));
#102556=CARTESIAN_POINT('Ctrl Pts',(10.7426206132375,72.3214463970634,12.));
#102557=CARTESIAN_POINT('Ctrl Pts',(10.7488061082368,72.296265618955,12.));
#102558=CARTESIAN_POINT('Ctrl Pts',(10.7549589083535,72.2711162461679,12.));
#102559=CARTESIAN_POINT('Ctrl Pts',(10.7610790405385,72.2459983875298,12.));
#102560=CARTESIAN_POINT('Ctrl Pts',(10.7671665319254,72.2209121522367,12.));
#102561=CARTESIAN_POINT('Ctrl Pts',(10.7732214098343,72.1958576498556,12.));
#102562=CARTESIAN_POINT('Ctrl Pts',(10.779243701766,72.17083499033,12.));
#102563=CARTESIAN_POINT('Ctrl Pts',(10.7852334354015,72.145844283983,12.));
#102564=CARTESIAN_POINT('Ctrl Pts',(10.7911906386027,72.1208856415171,12.));
#102565=CARTESIAN_POINT('Ctrl Pts',(10.7971153394168,72.095959174012,12.));
#102566=CARTESIAN_POINT('Ctrl Pts',(10.8030075660811,72.0710649929214,12.));
#102567=CARTESIAN_POINT('Ctrl Pts',(10.8088673470187,72.0462032100828,12.));
#102568=CARTESIAN_POINT('Ctrl Pts',(10.8146947108376,72.0213739377231,12.));
#102569=CARTESIAN_POINT('Ctrl Pts',(10.8204896863328,71.996577288462,12.));
#102570=CARTESIAN_POINT('Ctrl Pts',(10.8262523024897,71.971813375312,12.));
#102571=CARTESIAN_POINT('Ctrl Pts',(10.8319825884917,71.9470823116777,12.));
#102572=CARTESIAN_POINT('Ctrl Pts',(10.8376805737158,71.9223842113622,12.));
#102573=CARTESIAN_POINT('Ctrl Pts',(10.8433462877312,71.8977191885726,12.));
#102574=CARTESIAN_POINT('Ctrl Pts',(10.8489797602998,71.8730873579226,12.));
#102575=CARTESIAN_POINT('Ctrl Pts',(10.8545810213799,71.8484888344335,12.));
#102576=CARTESIAN_POINT('Ctrl Pts',(10.860150101133,71.8239237335318,12.));
#102577=CARTESIAN_POINT('Ctrl Pts',(10.8656870299218,71.7993921710546,12.));
#102578=CARTESIAN_POINT('Ctrl Pts',(10.8711918383071,71.7748942632578,12.));
#102579=CARTESIAN_POINT('Ctrl Pts',(10.8766645570496,71.7504301268177,12.));
#102580=CARTESIAN_POINT('Ctrl Pts',(10.8821052171122,71.7259998788337,12.));
#102581=CARTESIAN_POINT('Ctrl Pts',(10.8875138496674,71.7016036368254,12.));
#102582=CARTESIAN_POINT('Ctrl Pts',(10.8928904860967,71.6772415187382,12.));
#102583=CARTESIAN_POINT('Ctrl Pts',(10.8982351579872,71.6529136429515,12.));
#102584=CARTESIAN_POINT('Ctrl Pts',(10.9035478971329,71.6286201282815,12.));
#102585=CARTESIAN_POINT('Ctrl Pts',(10.9088287355364,71.604361093983,12.));
#102586=CARTESIAN_POINT('Ctrl Pts',(10.9140777054169,71.5801366597479,12.));
#102587=CARTESIAN_POINT('Ctrl Pts',(10.9192948392099,71.5559469457082,12.));
#102588=CARTESIAN_POINT('Ctrl Pts',(10.9244801695642,71.5317920724453,12.));
#102589=CARTESIAN_POINT('Ctrl Pts',(10.9296337293425,71.5076721609936,12.));
#102590=CARTESIAN_POINT('Ctrl Pts',(10.9347555516236,71.4835873328425,12.));
#102591=CARTESIAN_POINT('Ctrl Pts',(10.9398456697095,71.4595377099352,12.));
#102592=CARTESIAN_POINT('Ctrl Pts',(10.9449041171269,71.4355234146718,12.));
#102593=CARTESIAN_POINT('Ctrl Pts',(10.9499309276235,71.411544569919,12.));
#102594=CARTESIAN_POINT('Ctrl Pts',(10.954926135169,71.3876012990135,12.));
#102595=CARTESIAN_POINT('Ctrl Pts',(10.9598897739565,71.3636937257651,12.));
#102596=CARTESIAN_POINT('Ctrl Pts',(10.96482187841,71.3398219744547,12.));
#102597=CARTESIAN_POINT('Ctrl Pts',(10.9697224831862,71.3159861698368,12.));
#102598=CARTESIAN_POINT('Ctrl Pts',(10.9745916231711,71.2921864371499,12.));
#102599=CARTESIAN_POINT('Ctrl Pts',(10.9794293334806,71.2684229021209,12.));
#102600=CARTESIAN_POINT('Ctrl Pts',(10.9842356494627,71.2446956909685,12.));
#102601=CARTESIAN_POINT('Ctrl Pts',(10.9890106067038,71.221004930401,12.));
#102602=CARTESIAN_POINT('Ctrl Pts',(10.993754241032,71.1973507476188,12.));
#102603=CARTESIAN_POINT('Ctrl Pts',(10.9984665885127,71.1737332703248,12.));
#102604=CARTESIAN_POINT('Ctrl Pts',(11.0031476854503,71.1501526267288,12.));
#102605=CARTESIAN_POINT('Ctrl Pts',(11.0077975683895,71.1266089455517,12.));
#102606=CARTESIAN_POINT('Ctrl Pts',(11.0124162741223,71.1031023560243,12.));
#102607=CARTESIAN_POINT('Ctrl Pts',(11.0170038396913,71.0796329878896,12.));
#102608=CARTESIAN_POINT('Ctrl Pts',(11.0215603023854,71.0562009714125,12.));
#102609=CARTESIAN_POINT('Ctrl Pts',(11.0260856997414,71.0328064373849,12.));
#102610=CARTESIAN_POINT('Ctrl Pts',(11.0305800695457,71.0094495171295,12.));
#102611=CARTESIAN_POINT('Ctrl Pts',(11.0350434498408,70.9861303424989,12.));
#102612=CARTESIAN_POINT('Ctrl Pts',(11.039475878929,70.9628490458779,12.));
#102613=CARTESIAN_POINT('Ctrl Pts',(11.0438773953686,70.9396057601953,12.));
#102614=CARTESIAN_POINT('Ctrl Pts',(11.0482480379752,70.9164006189283,12.));
#102615=CARTESIAN_POINT('Ctrl Pts',(11.0525878458242,70.8932337561078,12.));
#102616=CARTESIAN_POINT('Ctrl Pts',(11.0568968582566,70.8701053063158,12.));
#102617=CARTESIAN_POINT('Ctrl Pts',(11.061175114883,70.847015404688,12.));
#102618=CARTESIAN_POINT('Ctrl Pts',(11.0654226555798,70.8239641869266,12.));
#102619=CARTESIAN_POINT('Ctrl Pts',(11.0696395204908,70.8009517893042,12.));
#102620=CARTESIAN_POINT('Ctrl Pts',(11.0738257500292,70.7779783486689,12.));
#102621=CARTESIAN_POINT('Ctrl Pts',(11.0779813848851,70.7550440024422,12.));
#102622=CARTESIAN_POINT('Ctrl Pts',(11.0821064660276,70.7321488886229,12.));
#102623=CARTESIAN_POINT('Ctrl Pts',(11.0862010347022,70.7092931457996,12.));
#102624=CARTESIAN_POINT('Ctrl Pts',(11.0902651324325,70.686476913156,12.));
#102625=CARTESIAN_POINT('Ctrl Pts',(11.0942988010231,70.6637003304768,12.));
#102626=CARTESIAN_POINT('Ctrl Pts',(11.0983020825662,70.6409635381446,12.));
#102627=CARTESIAN_POINT('Ctrl Pts',(11.1022750194439,70.6182666771441,12.));
#102628=CARTESIAN_POINT('Ctrl Pts',(11.1062176543257,70.5956098890744,12.));
#102629=CARTESIAN_POINT('Ctrl Pts',(11.11013003017,70.5729933161538,12.));
#102630=CARTESIAN_POINT('Ctrl Pts',(11.1140121902274,70.5504171012247,12.));
#102631=CARTESIAN_POINT('Ctrl Pts',(11.117864178048,70.5278813877519,12.));
#102632=CARTESIAN_POINT('Ctrl Pts',(11.121686037483,70.5053863198306,12.));
#102633=CARTESIAN_POINT('Ctrl Pts',(11.1254778126824,70.4829320421973,12.));
#102634=CARTESIAN_POINT('Ctrl Pts',(11.1292395480975,70.4605187002356,12.));
#102635=CARTESIAN_POINT('Ctrl Pts',(11.1329712884845,70.438146439981,12.));
#102636=CARTESIAN_POINT('Ctrl Pts',(11.1366730789122,70.415815408119,12.));
#102637=CARTESIAN_POINT('Ctrl Pts',(11.1403449647622,70.3935257519945,12.));
#102638=CARTESIAN_POINT('Ctrl Pts',(11.1439869917269,70.3712776196216,12.));
#102639=CARTESIAN_POINT('Ctrl Pts',(11.1475992058124,70.3490711596882,12.));
#102640=CARTESIAN_POINT('Ctrl Pts',(11.1511816533422,70.3269065215591,12.));
#102641=CARTESIAN_POINT('Ctrl Pts',(11.1547343809647,70.3047838552758,12.));
#102642=CARTESIAN_POINT('Ctrl Pts',(11.1582574356522,70.2827033115662,12.));
#102643=CARTESIAN_POINT('Ctrl Pts',(11.1617508647017,70.2606650418589,12.));
#102644=CARTESIAN_POINT('Ctrl Pts',(11.1652147157383,70.2386691982902,12.));
#102645=CARTESIAN_POINT('Ctrl Pts',(11.168649036721,70.2167159337095,12.));
#102646=CARTESIAN_POINT('Ctrl Pts',(11.1720538759499,70.1948054016817,12.));
#102647=CARTESIAN_POINT('Ctrl Pts',(11.1754292820631,70.1729377564956,12.));
#102648=CARTESIAN_POINT('Ctrl Pts',(11.1787753040363,70.1511131531674,12.));
#102649=CARTESIAN_POINT('Ctrl Pts',(11.1820919911846,70.1293317474432,12.));
#102650=CARTESIAN_POINT('Ctrl Pts',(11.185379393167,70.1075936957968,12.));
#102651=CARTESIAN_POINT('Ctrl Pts',(11.1886375599914,70.0858991554283,12.));
#102652=CARTESIAN_POINT('Ctrl Pts',(11.1918665420166,70.0642482842928,12.));
#102653=CARTESIAN_POINT('Ctrl Pts',(11.1950663899576,70.0426412411185,12.));
#102654=CARTESIAN_POINT('Ctrl Pts',(11.1982371548919,70.0210781854243,12.));
#102655=CARTESIAN_POINT('Ctrl Pts',(11.2013788882714,69.9995592775343,12.));
#102656=CARTESIAN_POINT('Ctrl Pts',(11.2044916419244,69.97808467858,12.));
#102657=CARTESIAN_POINT('Ctrl Pts',(11.2075754680449,69.9566545504837,12.));
#102658=CARTESIAN_POINT('Ctrl Pts',(11.2106304191882,69.9352690559405,12.));
#102659=CARTESIAN_POINT('Ctrl Pts',(11.2136565482678,69.9139283584022,12.));
#102660=CARTESIAN_POINT('Ctrl Pts',(11.2166539085523,69.8926326220385,12.));
#102661=CARTESIAN_POINT('Ctrl Pts',(11.219622553679,69.871382011789,12.));
#102662=CARTESIAN_POINT('Ctrl Pts',(11.2225625376736,69.8501766934428,12.));
#102663=CARTESIAN_POINT('Ctrl Pts',(11.225473914972,69.8290168337076,12.));
#102664=CARTESIAN_POINT('Ctrl Pts',(11.2283567404437,69.8079026002768,12.));
#102665=CARTESIAN_POINT('Ctrl Pts',(11.2312110694187,69.7868341618954,12.));
#102666=CARTESIAN_POINT('Ctrl Pts',(11.2340369576456,69.7658116882324,12.));
#102667=CARTESIAN_POINT('Ctrl Pts',(11.2368344612472,69.7448353497408,12.));
#102668=CARTESIAN_POINT('Ctrl Pts',(11.239603636686,69.7239053175356,12.));
#102669=CARTESIAN_POINT('Ctrl Pts',(11.2423445407166,69.7030217632164,12.));
#102670=CARTESIAN_POINT('Ctrl Pts',(11.2450572303841,69.6821848588457,12.));
#102671=CARTESIAN_POINT('Ctrl Pts',(11.2477417631386,69.6613947773534,12.));
#102672=CARTESIAN_POINT('Ctrl Pts',(11.2503981969412,69.6406516928891,12.));
#102673=CARTESIAN_POINT('Ctrl Pts',(11.2530265903557,69.6199557811245,12.));
#102674=CARTESIAN_POINT('Ctrl Pts',(11.2556270027016,69.599307219739,12.));
#102675=CARTESIAN_POINT('Ctrl Pts',(11.2581994939541,69.5787061880857,12.));
#102676=CARTESIAN_POINT('Ctrl Pts',(11.2607441244703,69.5581528662877,12.));
#102677=CARTESIAN_POINT('Ctrl Pts',(11.263260954763,69.5376474344771,12.));
#102678=CARTESIAN_POINT('Ctrl Pts',(11.2657500452716,69.5171900720158,12.));
#102679=CARTESIAN_POINT('Ctrl Pts',(11.2682114561008,69.4967809565929,12.));
#102680=CARTESIAN_POINT('Ctrl Pts',(11.270645247528,69.4764202659397,12.));
#102681=CARTESIAN_POINT('Ctrl Pts',(11.2730514806139,69.456108179879,12.));
#102682=CARTESIAN_POINT('Ctrl Pts',(11.2754302177021,69.4358448819967,12.));
#102683=CARTESIAN_POINT('Ctrl Pts',(11.2777815231469,69.4156305620593,12.));
#102684=CARTESIAN_POINT('Ctrl Pts',(11.2801054633816,69.3954654162281,12.));
#102685=CARTESIAN_POINT('Ctrl Pts',(11.2824021054045,69.3753496420039,12.));
#102686=CARTESIAN_POINT('Ctrl Pts',(11.2846715154524,69.3552834337784,12.));
#102687=CARTESIAN_POINT('Ctrl Pts',(11.2869137578459,69.3352669789587,12.));
#102688=CARTESIAN_POINT('Ctrl Pts',(11.2891288931517,69.3153004517783,12.));
#102689=CARTESIAN_POINT('Ctrl Pts',(11.2913169799628,69.295384019272,12.));
#102690=CARTESIAN_POINT('Ctrl Pts',(11.2934780784351,69.275517853148,12.));
#102691=CARTESIAN_POINT('Ctrl Pts',(11.2956122531375,69.2557021393351,12.));
#102692=CARTESIAN_POINT('Ctrl Pts',(11.2977195764852,69.2359370894907,12.));
#102693=CARTESIAN_POINT('Ctrl Pts',(11.2998001310964,69.2162229488531,12.));
#102694=CARTESIAN_POINT('Ctrl Pts',(11.3018540025638,69.1965599718914,12.));
#102695=CARTESIAN_POINT('Ctrl Pts',(11.3038812726292,69.1769483991721,12.));
#102696=CARTESIAN_POINT('Ctrl Pts',(11.3058820128307,69.1573884361,12.));
#102697=CARTESIAN_POINT('Ctrl Pts',(11.3078562764384,69.1378802251711,12.));
#102698=CARTESIAN_POINT('Ctrl Pts',(11.3098040973713,69.118423844466,12.));
#102699=CARTESIAN_POINT('Ctrl Pts',(11.3113412156661,69.1029002322118,12.));
#102700=CARTESIAN_POINT('Ctrl Pts',(11.3124821678798,69.0912808656811,12.));
#102701=CARTESIAN_POINT('Ctrl Pts',(11.3132375200165,69.0835449954396,12.));
#102702=CARTESIAN_POINT('Ctrl Pts',(11.3136138754165,69.079679653846,12.));
#102703=CARTESIAN_POINT('Ctrl Pts',(8.93459554657839,73.6640787198055,-5.55111512312578E-16));
#102704=CARTESIAN_POINT('Ctrl Pts',(8.93459554657839,73.6640787198055,4.));
#102705=CARTESIAN_POINT('Ctrl Pts',(8.93459554657838,73.6640787198055,8.));
#102706=CARTESIAN_POINT('Ctrl Pts',(8.93459554657838,73.6640787198055,12.));
#102707=CARTESIAN_POINT('Ctrl Pts',(8.99145626777887,73.7581053903595,-5.55111512312578E-16));
#102708=CARTESIAN_POINT('Ctrl Pts',(8.99145626777887,73.7581053903595,4.));
#102709=CARTESIAN_POINT('Ctrl Pts',(8.99145626777886,73.7581053903595,8.));
#102710=CARTESIAN_POINT('Ctrl Pts',(8.99145626777886,73.7581053903595,12.));
#102711=CARTESIAN_POINT('Ctrl Pts',(9.14696952162285,73.8880618019209,-5.55111512312578E-16));
#102712=CARTESIAN_POINT('Ctrl Pts',(9.14696952162285,73.8880618019209,4.));
#102713=CARTESIAN_POINT('Ctrl Pts',(9.14696952162285,73.888061801921,7.99999999999999));
#102714=CARTESIAN_POINT('Ctrl Pts',(9.14696952162285,73.888061801921,12.));
#102715=CARTESIAN_POINT('Ctrl Pts',(9.34395683490519,73.9117532086774,-5.55111512312578E-16));
#102716=CARTESIAN_POINT('Ctrl Pts',(9.34395683490519,73.9117532086774,4.));
#102717=CARTESIAN_POINT('Ctrl Pts',(9.34395683490521,73.9117532086774,8.00000000000001));
#102718=CARTESIAN_POINT('Ctrl Pts',(9.34395683490521,73.9117532086774,12.));
#102719=CARTESIAN_POINT('Ctrl Pts',(9.42570643237553,73.9013264985867,-5.55111512312578E-16));
#102720=CARTESIAN_POINT('Ctrl Pts',(9.42570643237553,73.9013264985867,4.));
#102721=CARTESIAN_POINT('Ctrl Pts',(9.42570643237556,73.9013264985867,8.));
#102722=CARTESIAN_POINT('Ctrl Pts',(9.42570643237556,73.9013264985867,12.));
#102723=CARTESIAN_POINT('',(8.93459554657838,73.6640787198055,0.));
#102724=CARTESIAN_POINT('',(9.4257064323755,73.9013264985864,2.77555756156289E-16));
#102725=CARTESIAN_POINT('Ctrl Pts',(8.93459554657839,73.6640787198055,4.16333634234434E-16));
#102726=CARTESIAN_POINT('Ctrl Pts',(8.99145626777887,73.7581053903595,4.16333634234433E-16));
#102727=CARTESIAN_POINT('Ctrl Pts',(9.08032098426115,73.832366196966,4.16333634234434E-16));
#102728=CARTESIAN_POINT('Ctrl Pts',(9.18272825076411,73.8719282264934,4.16333634234434E-16));
#102729=CARTESIAN_POINT('Ctrl Pts',(9.25953370064133,73.9015997486389,4.16333634234434E-16));
#102730=CARTESIAN_POINT('Ctrl Pts',(9.34395683490519,73.9117532086774,4.16333634234433E-16));
#102731=CARTESIAN_POINT('Ctrl Pts',(9.42570643237553,73.9013264985867,4.16333634234434E-16));
#102732=CARTESIAN_POINT('',(9.42570643237553,73.9013264985864,12.));
#102733=CARTESIAN_POINT('Ctrl Pts',(9.42570643237553,73.9013264985867,-5.55111512312578E-16));
#102734=CARTESIAN_POINT('Ctrl Pts',(9.42570643237553,73.9013264985867,4.));
#102735=CARTESIAN_POINT('Ctrl Pts',(9.42570643237556,73.9013264985867,8.));
#102736=CARTESIAN_POINT('Ctrl Pts',(9.42570643237556,73.9013264985867,12.));
#102737=CARTESIAN_POINT('',(8.93459554657838,73.6640787198055,12.));
#102738=CARTESIAN_POINT('Ctrl Pts',(9.42570643237556,73.9013264985867,12.));
#102739=CARTESIAN_POINT('Ctrl Pts',(9.34395683490521,73.9117532086774,12.));
#102740=CARTESIAN_POINT('Ctrl Pts',(9.25953370064134,73.901599748639,12.));
#102741=CARTESIAN_POINT('Ctrl Pts',(9.18272825076411,73.8719282264934,12.));
#102742=CARTESIAN_POINT('Ctrl Pts',(9.08032098426114,73.8323661969661,12.));
#102743=CARTESIAN_POINT('Ctrl Pts',(8.99145626777886,73.7581053903595,12.));
#102744=CARTESIAN_POINT('Ctrl Pts',(8.93459554657838,73.6640787198055,12.));
#102745=CARTESIAN_POINT('Ctrl Pts',(8.93459554657838,73.6640787198055,12.));
#102746=CARTESIAN_POINT('Ctrl Pts',(8.93459554657838,73.6640787198055,8.));
#102747=CARTESIAN_POINT('Ctrl Pts',(8.93459554657839,73.6640787198055,4.));
#102748=CARTESIAN_POINT('Ctrl Pts',(8.93459554657839,73.6640787198055,-5.55111512312578E-16));
#102749=CARTESIAN_POINT('Origin',(4.88285199465431E-11,3.71649880366789E-10,
0.));
#102750=CARTESIAN_POINT('Origin',(4.88285199465431E-11,3.71649880366789E-10,
12.));
#102751=CARTESIAN_POINT('Origin',(4.88285199465431E-11,3.71649880366789E-10,
0.));
#102752=CARTESIAN_POINT('Ctrl Pts',(16.4184755008034,72.6683126419592,-1.11022302462516E-15));
#102753=CARTESIAN_POINT('Ctrl Pts',(16.4184755008034,72.6683126419592,4.));
#102754=CARTESIAN_POINT('Ctrl Pts',(16.4184755008034,72.6683126419592,8.));
#102755=CARTESIAN_POINT('Ctrl Pts',(16.4184755008034,72.6683126419592,12.));
#102756=CARTESIAN_POINT('Ctrl Pts',(16.5256563519779,72.6440964999409,-1.11022302462516E-15));
#102757=CARTESIAN_POINT('Ctrl Pts',(16.5256563519779,72.6440964999409,3.99999999999999));
#102758=CARTESIAN_POINT('Ctrl Pts',(16.5256563519779,72.6440964999409,8.));
#102759=CARTESIAN_POINT('Ctrl Pts',(16.5256563519779,72.6440964999409,12.));
#102760=CARTESIAN_POINT('Ctrl Pts',(16.6981133841328,72.5376471652843,-1.0371418567521E-15));
#102761=CARTESIAN_POINT('Ctrl Pts',(16.6981133841328,72.5376471652843,4.00000000000001));
#102762=CARTESIAN_POINT('Ctrl Pts',(16.6981133841328,72.5376471652843,8.));
#102763=CARTESIAN_POINT('Ctrl Pts',(16.6981133841328,72.5376471652843,12.));
#102764=CARTESIAN_POINT('Ctrl Pts',(16.7828708182976,72.3582555997243,-8.63611844392621E-16));
#102765=CARTESIAN_POINT('Ctrl Pts',(16.7828708182976,72.3582555997243,3.99999999999999));
#102766=CARTESIAN_POINT('Ctrl Pts',(16.7828708182976,72.3582555997243,8.));
#102767=CARTESIAN_POINT('Ctrl Pts',(16.7828708182976,72.3582555997243,12.));
#102768=CARTESIAN_POINT('Ctrl Pts',(16.7988252568808,72.2774028393484,-7.7995786415518E-16));
#102769=CARTESIAN_POINT('Ctrl Pts',(16.7988252568808,72.2774028393484,4.));
#102770=CARTESIAN_POINT('Ctrl Pts',(16.7988252568808,72.2774028393484,8.));
#102771=CARTESIAN_POINT('Ctrl Pts',(16.7988252568808,72.2774028393484,12.));
#102772=CARTESIAN_POINT('',(16.4184755008034,72.6683126419592,0.));
#102773=CARTESIAN_POINT('',(16.7988252568807,72.2774028393484,2.77555756156289E-16));
#102774=CARTESIAN_POINT('Ctrl Pts',(16.4184755008034,72.6683126419592,-1.38777878078144E-16));
#102775=CARTESIAN_POINT('Ctrl Pts',(16.5256563519779,72.6440964999409,-1.38777878078146E-16));
#102776=CARTESIAN_POINT('Ctrl Pts',(16.624203227495,72.5832683087086,-9.70172107221101E-17));
#102777=CARTESIAN_POINT('Ctrl Pts',(16.6941134995868,72.4986222461608,-2.24569206766341E-17));
#102778=CARTESIAN_POINT('Ctrl Pts',(16.7465462036556,72.43513769925,3.34632968574728E-17));
#102779=CARTESIAN_POINT('Ctrl Pts',(16.7828708182976,72.3582555997243,1.0783330215439E-16));
#102780=CARTESIAN_POINT('Ctrl Pts',(16.7988252568808,72.2774028393484,1.91487282391832E-16));
#102781=CARTESIAN_POINT('',(16.7988252568807,72.2774028393484,12.));
#102782=CARTESIAN_POINT('Ctrl Pts',(16.7988252568808,72.2774028393484,-7.7995786415518E-16));
#102783=CARTESIAN_POINT('Ctrl Pts',(16.7988252568808,72.2774028393484,4.));
#102784=CARTESIAN_POINT('Ctrl Pts',(16.7988252568808,72.2774028393484,8.));
#102785=CARTESIAN_POINT('Ctrl Pts',(16.7988252568808,72.2774028393484,12.));
#102786=CARTESIAN_POINT('',(16.4184755008034,72.6683126419592,12.));
#102787=CARTESIAN_POINT('Ctrl Pts',(16.7988252568808,72.2774028393484,12.));
#102788=CARTESIAN_POINT('Ctrl Pts',(16.7828708182976,72.3582555997243,12.));
#102789=CARTESIAN_POINT('Ctrl Pts',(16.7465462036556,72.43513769925,12.));
#102790=CARTESIAN_POINT('Ctrl Pts',(16.6941134995867,72.4986222461608,12.));
#102791=CARTESIAN_POINT('Ctrl Pts',(16.624203227495,72.5832683087086,12.));
#102792=CARTESIAN_POINT('Ctrl Pts',(16.5256563519779,72.6440964999409,12.));
#102793=CARTESIAN_POINT('Ctrl Pts',(16.4184755008034,72.6683126419592,12.));
#102794=CARTESIAN_POINT('Ctrl Pts',(16.4184755008034,72.6683126419592,12.));
#102795=CARTESIAN_POINT('Ctrl Pts',(16.4184755008034,72.6683126419592,8.));
#102796=CARTESIAN_POINT('Ctrl Pts',(16.4184755008034,72.6683126419592,4.));
#102797=CARTESIAN_POINT('Ctrl Pts',(16.4184755008034,72.6683126419592,-1.11022302462516E-15));
#102798=CARTESIAN_POINT('Ctrl Pts',(17.2912529479484,67.8307641965655,0.));
#102799=CARTESIAN_POINT('Ctrl Pts',(17.2912529479484,67.8307641965655,12.));
#102800=CARTESIAN_POINT('Ctrl Pts',(17.2912149114119,67.8346476309018,0.));
#102801=CARTESIAN_POINT('Ctrl Pts',(17.2912149114119,67.8346476309018,12.));
#102802=CARTESIAN_POINT('Ctrl Pts',(17.2911366591348,67.842419897098,0.));
#102803=CARTESIAN_POINT('Ctrl Pts',(17.2911366591348,67.842419897098,12.));
#102804=CARTESIAN_POINT('Ctrl Pts',(17.291012743109,67.8540944889687,0.));
#102805=CARTESIAN_POINT('Ctrl Pts',(17.291012743109,67.8540944889687,12.));
#102806=CARTESIAN_POINT('Ctrl Pts',(17.2908344459694,67.8696929978782,0.));
#102807=CARTESIAN_POINT('Ctrl Pts',(17.2908344459694,67.8696929978782,12.));
#102808=CARTESIAN_POINT('Ctrl Pts',(17.2905897723949,67.8892451049608,0.));
#102809=CARTESIAN_POINT('Ctrl Pts',(17.2905897723949,67.8892451049608,12.));
#102810=CARTESIAN_POINT('Ctrl Pts',(17.2903232740694,67.9088511496686,0.));
#102811=CARTESIAN_POINT('Ctrl Pts',(17.2903232740694,67.9088511496686,12.));
#102812=CARTESIAN_POINT('Ctrl Pts',(17.2900349103981,67.9285110571741,0.));
#102813=CARTESIAN_POINT('Ctrl Pts',(17.2900349103981,67.9285110571741,12.));
#102814=CARTESIAN_POINT('Ctrl Pts',(17.2897246158941,67.9482246901667,0.));
#102815=CARTESIAN_POINT('Ctrl Pts',(17.2897246158941,67.9482246901667,12.));
#102816=CARTESIAN_POINT('Ctrl Pts',(17.2893923013894,67.9679918502579,0.));
#102817=CARTESIAN_POINT('Ctrl Pts',(17.2893923013894,67.9679918502579,12.));
#102818=CARTESIAN_POINT('Ctrl Pts',(17.2890378644866,67.987812304921,0.));
#102819=CARTESIAN_POINT('Ctrl Pts',(17.2890378644866,67.987812304921,12.));
#102820=CARTESIAN_POINT('Ctrl Pts',(17.28866119774,68.007685808115,0.));
#102821=CARTESIAN_POINT('Ctrl Pts',(17.28866119774,68.007685808115,12.));
#102822=CARTESIAN_POINT('Ctrl Pts',(17.2882621974721,68.0276121227356,0.));
#102823=CARTESIAN_POINT('Ctrl Pts',(17.2882621974721,68.0276121227356,12.));
#102824=CARTESIAN_POINT('Ctrl Pts',(17.2878407730961,68.0475910442424,0.));
#102825=CARTESIAN_POINT('Ctrl Pts',(17.2878407730961,68.0475910442424,12.));
#102826=CARTESIAN_POINT('Ctrl Pts',(17.2873968440839,68.0676223930412,0.));
#102827=CARTESIAN_POINT('Ctrl Pts',(17.2873968440839,68.0676223930412,12.));
#102828=CARTESIAN_POINT('Ctrl Pts',(17.2869303355432,68.0877060033205,0.));
#102829=CARTESIAN_POINT('Ctrl Pts',(17.2869303355432,68.0877060033205,12.));
#102830=CARTESIAN_POINT('Ctrl Pts',(17.2864411745459,68.1078417137877,0.));
#102831=CARTESIAN_POINT('Ctrl Pts',(17.2864411745459,68.1078417137877,12.));
#102832=CARTESIAN_POINT('Ctrl Pts',(17.2859292855705,68.1280293561511,0.));
#102833=CARTESIAN_POINT('Ctrl Pts',(17.2859292855705,68.1280293561511,12.));
#102834=CARTESIAN_POINT('Ctrl Pts',(17.2853945882072,68.1482687493226,0.));
#102835=CARTESIAN_POINT('Ctrl Pts',(17.2853945882072,68.1482687493226,12.));
#102836=CARTESIAN_POINT('Ctrl Pts',(17.2848369995293,68.1685597054232,0.));
#102837=CARTESIAN_POINT('Ctrl Pts',(17.2848369995293,68.1685597054232,12.));
#102838=CARTESIAN_POINT('Ctrl Pts',(17.2842564355799,68.1889020335427,0.));
#102839=CARTESIAN_POINT('Ctrl Pts',(17.2842564355799,68.1889020335427,12.));
#102840=CARTESIAN_POINT('Ctrl Pts',(17.2836528130819,68.2092955440567,0.));
#102841=CARTESIAN_POINT('Ctrl Pts',(17.2836528130819,68.2092955440567,12.));
#102842=CARTESIAN_POINT('Ctrl Pts',(17.2830260513867,68.2297400535294,0.));
#102843=CARTESIAN_POINT('Ctrl Pts',(17.2830260513867,68.2297400535294,12.));
#102844=CARTESIAN_POINT('Ctrl Pts',(17.2823760723874,68.2502353845071,0.));
#102845=CARTESIAN_POINT('Ctrl Pts',(17.2823760723874,68.2502353845071,12.));
#102846=CARTESIAN_POINT('Ctrl Pts',(17.2817027995831,68.2707813631731,0.));
#102847=CARTESIAN_POINT('Ctrl Pts',(17.2817027995831,68.2707813631731,12.));
#102848=CARTESIAN_POINT('Ctrl Pts',(17.2810061574353,68.2913778177261,0.));
#102849=CARTESIAN_POINT('Ctrl Pts',(17.2810061574353,68.2913778177261,12.));
#102850=CARTESIAN_POINT('Ctrl Pts',(17.2802860705815,68.3120245763914,0.));
#102851=CARTESIAN_POINT('Ctrl Pts',(17.2802860705815,68.3120245763914,12.));
#102852=CARTESIAN_POINT('Ctrl Pts',(17.2795424631799,68.3327214657575,0.));
#102853=CARTESIAN_POINT('Ctrl Pts',(17.2795424631799,68.3327214657575,12.));
#102854=CARTESIAN_POINT('Ctrl Pts',(17.2787752592484,68.3534683116515,0.));
#102855=CARTESIAN_POINT('Ctrl Pts',(17.2787752592484,68.3534683116515,12.));
#102856=CARTESIAN_POINT('Ctrl Pts',(17.2779843829608,68.3742649398964,0.));
#102857=CARTESIAN_POINT('Ctrl Pts',(17.2779843829608,68.3742649398964,12.));
#102858=CARTESIAN_POINT('Ctrl Pts',(17.2771697589384,68.3951111770487,0.));
#102859=CARTESIAN_POINT('Ctrl Pts',(17.2771697589384,68.3951111770487,12.));
#102860=CARTESIAN_POINT('Ctrl Pts',(17.2763313126018,68.4160068512753,0.));
#102861=CARTESIAN_POINT('Ctrl Pts',(17.2763313126018,68.4160068512753,12.));
#102862=CARTESIAN_POINT('Ctrl Pts',(17.2754689702992,68.436951792677,0.));
#102863=CARTESIAN_POINT('Ctrl Pts',(17.2754689702992,68.436951792677,12.));
#102864=CARTESIAN_POINT('Ctrl Pts',(17.2745826591119,68.4579458328185,0.));
#102865=CARTESIAN_POINT('Ctrl Pts',(17.2745826591119,68.4579458328185,12.));
#102866=CARTESIAN_POINT('Ctrl Pts',(17.2736723067365,68.4789888044351,0.));
#102867=CARTESIAN_POINT('Ctrl Pts',(17.2736723067365,68.4789888044351,12.));
#102868=CARTESIAN_POINT('Ctrl Pts',(17.2727378413489,68.5000805410911,0.));
#102869=CARTESIAN_POINT('Ctrl Pts',(17.2727378413489,68.5000805410911,12.));
#102870=CARTESIAN_POINT('Ctrl Pts',(17.2717791914544,68.521220876786,0.));
#102871=CARTESIAN_POINT('Ctrl Pts',(17.2717791914544,68.521220876786,12.));
#102872=CARTESIAN_POINT('Ctrl Pts',(17.2707962858919,68.5424096459772,0.));
#102873=CARTESIAN_POINT('Ctrl Pts',(17.2707962858919,68.5424096459772,12.));
#102874=CARTESIAN_POINT('Ctrl Pts',(17.269789053896,68.5636466837517,0.));
#102875=CARTESIAN_POINT('Ctrl Pts',(17.269789053896,68.5636466837517,12.));
#102876=CARTESIAN_POINT('Ctrl Pts',(17.2687574251429,68.5849318259449,0.));
#102877=CARTESIAN_POINT('Ctrl Pts',(17.2687574251429,68.5849318259449,12.));
#102878=CARTESIAN_POINT('Ctrl Pts',(17.2677013298057,68.6062649092764,0.));
#102879=CARTESIAN_POINT('Ctrl Pts',(17.2677013298057,68.6062649092764,12.));
#102880=CARTESIAN_POINT('Ctrl Pts',(17.2666206986084,68.6276457714729,0.));
#102881=CARTESIAN_POINT('Ctrl Pts',(17.2666206986084,68.6276457714729,12.));
#102882=CARTESIAN_POINT('Ctrl Pts',(17.2655154627928,68.6490742512057,0.));
#102883=CARTESIAN_POINT('Ctrl Pts',(17.2655154627928,68.6490742512057,12.));
#102884=CARTESIAN_POINT('Ctrl Pts',(17.2643855540892,68.6705501880249,0.));
#102885=CARTESIAN_POINT('Ctrl Pts',(17.2643855540892,68.6705501880249,12.));
#102886=CARTESIAN_POINT('Ctrl Pts',(17.2632309046892,68.6920734222938,0.));
#102887=CARTESIAN_POINT('Ctrl Pts',(17.2632309046892,68.6920734222938,12.));
#102888=CARTESIAN_POINT('Ctrl Pts',(17.2620514472182,68.7136437951097,0.));
#102889=CARTESIAN_POINT('Ctrl Pts',(17.2620514472182,68.7136437951097,12.));
#102890=CARTESIAN_POINT('Ctrl Pts',(17.2608471147185,68.7352611482547,0.));
#102891=CARTESIAN_POINT('Ctrl Pts',(17.2608471147185,68.7352611482547,12.));
#102892=CARTESIAN_POINT('Ctrl Pts',(17.259617840655,68.7569253242333,0.));
#102893=CARTESIAN_POINT('Ctrl Pts',(17.259617840655,68.7569253242333,12.));
#102894=CARTESIAN_POINT('Ctrl Pts',(17.2583635589198,68.7786361662882,0.));
#102895=CARTESIAN_POINT('Ctrl Pts',(17.2583635589198,68.7786361662882,12.));
#102896=CARTESIAN_POINT('Ctrl Pts',(17.2570842038383,68.8003935184184,0.));
#102897=CARTESIAN_POINT('Ctrl Pts',(17.2570842038383,68.8003935184184,12.));
#102898=CARTESIAN_POINT('Ctrl Pts',(17.2557797101812,68.8221972253941,0.));
#102899=CARTESIAN_POINT('Ctrl Pts',(17.2557797101812,68.8221972253941,12.));
#102900=CARTESIAN_POINT('Ctrl Pts',(17.2544500131624,68.844047132755,0.));
#102901=CARTESIAN_POINT('Ctrl Pts',(17.2544500131624,68.844047132755,12.));
#102902=CARTESIAN_POINT('Ctrl Pts',(17.2530950484258,68.8659430867972,0.));
#102903=CARTESIAN_POINT('Ctrl Pts',(17.2530950484258,68.8659430867972,12.));
#102904=CARTESIAN_POINT('Ctrl Pts',(17.2517147520376,68.8878849345557,0.));
#102905=CARTESIAN_POINT('Ctrl Pts',(17.2517147520376,68.8878849345557,12.));
#102906=CARTESIAN_POINT('Ctrl Pts',(17.2503090604792,68.909872523787,0.));
#102907=CARTESIAN_POINT('Ctrl Pts',(17.2503090604792,68.909872523787,12.));
#102908=CARTESIAN_POINT('Ctrl Pts',(17.248877910643,68.9319057029409,0.));
#102909=CARTESIAN_POINT('Ctrl Pts',(17.248877910643,68.9319057029409,12.));
#102910=CARTESIAN_POINT('Ctrl Pts',(17.2474212398275,68.9539843211619,0.));
#102911=CARTESIAN_POINT('Ctrl Pts',(17.2474212398275,68.9539843211619,12.));
#102912=CARTESIAN_POINT('Ctrl Pts',(17.2459389857327,68.9761082282922,0.));
#102913=CARTESIAN_POINT('Ctrl Pts',(17.2459389857327,68.9761082282922,12.));
#102914=CARTESIAN_POINT('Ctrl Pts',(17.2444310864585,68.9982772748694,0.));
#102915=CARTESIAN_POINT('Ctrl Pts',(17.2444310864585,68.9982772748694,12.));
#102916=CARTESIAN_POINT('Ctrl Pts',(17.2428974805044,69.0204913121225,0.));
#102917=CARTESIAN_POINT('Ctrl Pts',(17.2428974805044,69.0204913121225,12.));
#102918=CARTESIAN_POINT('Ctrl Pts',(17.2413381067723,69.0427501919636,0.));
#102919=CARTESIAN_POINT('Ctrl Pts',(17.2413381067723,69.0427501919636,12.));
#102920=CARTESIAN_POINT('Ctrl Pts',(17.2397529045589,69.065053766986,0.));
#102921=CARTESIAN_POINT('Ctrl Pts',(17.2397529045589,69.065053766986,12.));
#102922=CARTESIAN_POINT('Ctrl Pts',(17.2381418135491,69.0874018904599,0.));
#102923=CARTESIAN_POINT('Ctrl Pts',(17.2381418135491,69.0874018904599,12.));
#102924=CARTESIAN_POINT('Ctrl Pts',(17.2365047738125,69.1097944163245,0.));
#102925=CARTESIAN_POINT('Ctrl Pts',(17.2365047738125,69.1097944163245,12.));
#102926=CARTESIAN_POINT('Ctrl Pts',(17.2348417258015,69.1322311991752,0.));
#102927=CARTESIAN_POINT('Ctrl Pts',(17.2348417258015,69.1322311991752,12.));
#102928=CARTESIAN_POINT('Ctrl Pts',(17.2331526103506,69.1547120942527,0.));
#102929=CARTESIAN_POINT('Ctrl Pts',(17.2331526103506,69.1547120942527,12.));
#102930=CARTESIAN_POINT('Ctrl Pts',(17.23143736867,69.1772369574447,0.));
#102931=CARTESIAN_POINT('Ctrl Pts',(17.23143736867,69.1772369574447,12.));
#102932=CARTESIAN_POINT('Ctrl Pts',(17.2296959423407,69.1998056452828,0.));
#102933=CARTESIAN_POINT('Ctrl Pts',(17.2296959423407,69.1998056452828,12.));
#102934=CARTESIAN_POINT('Ctrl Pts',(17.227928273312,69.222418014938,0.));
#102935=CARTESIAN_POINT('Ctrl Pts',(17.227928273312,69.222418014938,12.));
#102936=CARTESIAN_POINT('Ctrl Pts',(17.226134303902,69.2450739242109,0.));
#102937=CARTESIAN_POINT('Ctrl Pts',(17.226134303902,69.2450739242109,12.));
#102938=CARTESIAN_POINT('Ctrl Pts',(17.224313976797,69.2677732315224,0.));
#102939=CARTESIAN_POINT('Ctrl Pts',(17.224313976797,69.2677732315224,12.));
#102940=CARTESIAN_POINT('Ctrl Pts',(17.2224672350438,69.2905157959166,0.));
#102941=CARTESIAN_POINT('Ctrl Pts',(17.2224672350438,69.2905157959166,12.));
#102942=CARTESIAN_POINT('Ctrl Pts',(17.2205940220459,69.3133014770555,0.));
#102943=CARTESIAN_POINT('Ctrl Pts',(17.2205940220459,69.3133014770555,12.));
#102944=CARTESIAN_POINT('Ctrl Pts',(17.2186942815602,69.3361301352141,0.));
#102945=CARTESIAN_POINT('Ctrl Pts',(17.2186942815602,69.3361301352141,12.));
#102946=CARTESIAN_POINT('Ctrl Pts',(17.2167679576984,69.3590016312692,0.));
#102947=CARTESIAN_POINT('Ctrl Pts',(17.2167679576984,69.3590016312692,12.));
#102948=CARTESIAN_POINT('Ctrl Pts',(17.2148149949252,69.3819158266916,0.));
#102949=CARTESIAN_POINT('Ctrl Pts',(17.2148149949252,69.3819158266916,12.));
#102950=CARTESIAN_POINT('Ctrl Pts',(17.2128353380502,69.404872583548,0.));
#102951=CARTESIAN_POINT('Ctrl Pts',(17.2128353380502,69.404872583548,12.));
#102952=CARTESIAN_POINT('Ctrl Pts',(17.2108289322254,69.4278717644973,0.));
#102953=CARTESIAN_POINT('Ctrl Pts',(17.2108289322254,69.4278717644973,12.));
#102954=CARTESIAN_POINT('Ctrl Pts',(17.2087957229423,69.450913232785,0.));
#102955=CARTESIAN_POINT('Ctrl Pts',(17.2087957229423,69.450913232785,12.));
#102956=CARTESIAN_POINT('Ctrl Pts',(17.2067356560336,69.4739968522313,0.));
#102957=CARTESIAN_POINT('Ctrl Pts',(17.2067356560336,69.4739968522313,12.));
#102958=CARTESIAN_POINT('Ctrl Pts',(17.2046486776708,69.4971224872269,0.));
#102959=CARTESIAN_POINT('Ctrl Pts',(17.2046486776708,69.4971224872269,12.));
#102960=CARTESIAN_POINT('Ctrl Pts',(17.2025347343577,69.5202900027367,0.));
#102961=CARTESIAN_POINT('Ctrl Pts',(17.2025347343577,69.5202900027367,12.));
#102962=CARTESIAN_POINT('Ctrl Pts',(17.2003937729268,69.5434992642944,0.));
#102963=CARTESIAN_POINT('Ctrl Pts',(17.2003937729268,69.5434992642944,12.));
#102964=CARTESIAN_POINT('Ctrl Pts',(17.1982257405377,69.5667501379969,0.));
#102965=CARTESIAN_POINT('Ctrl Pts',(17.1982257405377,69.5667501379969,12.));
#102966=CARTESIAN_POINT('Ctrl Pts',(17.196030584678,69.5900424904921,0.));
#102967=CARTESIAN_POINT('Ctrl Pts',(17.196030584678,69.5900424904921,12.));
#102968=CARTESIAN_POINT('Ctrl Pts',(17.1938082531612,69.6133761889749,0.));
#102969=CARTESIAN_POINT('Ctrl Pts',(17.1938082531612,69.6133761889749,12.));
#102970=CARTESIAN_POINT('Ctrl Pts',(17.1915586941192,69.6367511011898,0.));
#102971=CARTESIAN_POINT('Ctrl Pts',(17.1915586941192,69.6367511011898,12.));
#102972=CARTESIAN_POINT('Ctrl Pts',(17.1892818560002,69.6601670954269,0.));
#102973=CARTESIAN_POINT('Ctrl Pts',(17.1892818560002,69.6601670954269,12.));
#102974=CARTESIAN_POINT('Ctrl Pts',(17.1869776875666,69.6836240405164,0.));
#102975=CARTESIAN_POINT('Ctrl Pts',(17.1869776875666,69.6836240405164,12.));
#102976=CARTESIAN_POINT('Ctrl Pts',(17.1846461378973,69.7071218058178,0.));
#102977=CARTESIAN_POINT('Ctrl Pts',(17.1846461378973,69.7071218058178,12.));
#102978=CARTESIAN_POINT('Ctrl Pts',(17.1822871563842,69.7306602612155,0.));
#102979=CARTESIAN_POINT('Ctrl Pts',(17.1822871563842,69.7306602612155,12.));
#102980=CARTESIAN_POINT('Ctrl Pts',(17.179900692726,69.7542392771234,0.));
#102981=CARTESIAN_POINT('Ctrl Pts',(17.179900692726,69.7542392771234,12.));
#102982=CARTESIAN_POINT('Ctrl Pts',(17.1774866969256,69.777858724479,0.));
#102983=CARTESIAN_POINT('Ctrl Pts',(17.1774866969256,69.777858724479,12.));
#102984=CARTESIAN_POINT('Ctrl Pts',(17.1750451192885,69.8015184747398,0.));
#102985=CARTESIAN_POINT('Ctrl Pts',(17.1750451192885,69.8015184747398,12.));
#102986=CARTESIAN_POINT('Ctrl Pts',(17.1725759104252,69.8252183998702,0.));
#102987=CARTESIAN_POINT('Ctrl Pts',(17.1725759104252,69.8252183998702,12.));
#102988=CARTESIAN_POINT('Ctrl Pts',(17.1700790212474,69.8489583723407,0.));
#102989=CARTESIAN_POINT('Ctrl Pts',(17.1700790212474,69.8489583723407,12.));
#102990=CARTESIAN_POINT('Ctrl Pts',(17.167554402962,69.8727382651286,0.));
#102991=CARTESIAN_POINT('Ctrl Pts',(17.167554402962,69.8727382651286,12.));
#102992=CARTESIAN_POINT('Ctrl Pts',(17.1650020070686,69.8965579517147,0.));
#102993=CARTESIAN_POINT('Ctrl Pts',(17.1650020070686,69.8965579517147,12.));
#102994=CARTESIAN_POINT('Ctrl Pts',(17.1624217853578,69.9204173060781,0.));
#102995=CARTESIAN_POINT('Ctrl Pts',(17.1624217853578,69.9204173060781,12.));
#102996=CARTESIAN_POINT('Ctrl Pts',(17.1598136899144,69.9443162026865,0.));
#102997=CARTESIAN_POINT('Ctrl Pts',(17.1598136899144,69.9443162026865,12.));
#102998=CARTESIAN_POINT('Ctrl Pts',(17.157177673114,69.9682545164939,0.));
#102999=CARTESIAN_POINT('Ctrl Pts',(17.157177673114,69.9682545164939,12.));
#103000=CARTESIAN_POINT('Ctrl Pts',(17.154513687616,69.9922321229424,0.));
#103001=CARTESIAN_POINT('Ctrl Pts',(17.154513687616,69.9922321229424,12.));
#103002=CARTESIAN_POINT('Ctrl Pts',(17.1518216863623,70.0162488979584,0.));
#103003=CARTESIAN_POINT('Ctrl Pts',(17.1518216863623,70.0162488979584,12.));
#103004=CARTESIAN_POINT('Ctrl Pts',(17.1491016225749,70.0403047179483,0.));
#103005=CARTESIAN_POINT('Ctrl Pts',(17.1491016225749,70.0403047179483,12.));
#103006=CARTESIAN_POINT('Ctrl Pts',(17.1463534497594,70.0643994597873,0.));
#103007=CARTESIAN_POINT('Ctrl Pts',(17.1463534497594,70.0643994597873,12.));
#103008=CARTESIAN_POINT('Ctrl Pts',(17.1435771217018,70.0885330008179,0.));
#103009=CARTESIAN_POINT('Ctrl Pts',(17.1435771217018,70.0885330008179,12.));
#103010=CARTESIAN_POINT('Ctrl Pts',(17.1407725924617,70.1127052188522,0.));
#103011=CARTESIAN_POINT('Ctrl Pts',(17.1407725924617,70.1127052188522,12.));
#103012=CARTESIAN_POINT('Ctrl Pts',(17.1379398163709,70.1369159921687,0.));
#103013=CARTESIAN_POINT('Ctrl Pts',(17.1379398163709,70.1369159921687,12.));
#103014=CARTESIAN_POINT('Ctrl Pts',(17.1350787480312,70.1611651995083,0.));
#103015=CARTESIAN_POINT('Ctrl Pts',(17.1350787480312,70.1611651995083,12.));
#103016=CARTESIAN_POINT('Ctrl Pts',(17.1321893423182,70.1854527200631,0.));
#103017=CARTESIAN_POINT('Ctrl Pts',(17.1321893423182,70.1854527200631,12.));
#103018=CARTESIAN_POINT('Ctrl Pts',(17.1292715543778,70.2097784334747,0.));
#103019=CARTESIAN_POINT('Ctrl Pts',(17.1292715543778,70.2097784334747,12.));
#103020=CARTESIAN_POINT('Ctrl Pts',(17.1263253396202,70.2341422198363,0.));
#103021=CARTESIAN_POINT('Ctrl Pts',(17.1263253396202,70.2341422198363,12.));
#103022=CARTESIAN_POINT('Ctrl Pts',(17.1233506537176,70.2585439596901,0.));
#103023=CARTESIAN_POINT('Ctrl Pts',(17.1233506537176,70.2585439596901,12.));
#103024=CARTESIAN_POINT('Ctrl Pts',(17.1203474526031,70.2829835340238,0.));
#103025=CARTESIAN_POINT('Ctrl Pts',(17.1203474526031,70.2829835340238,12.));
#103026=CARTESIAN_POINT('Ctrl Pts',(17.1173156924733,70.3074608242608,0.));
#103027=CARTESIAN_POINT('Ctrl Pts',(17.1173156924733,70.3074608242608,12.));
#103028=CARTESIAN_POINT('Ctrl Pts',(17.1142553297867,70.3319757122568,0.));
#103029=CARTESIAN_POINT('Ctrl Pts',(17.1142553297867,70.3319757122568,12.));
#103030=CARTESIAN_POINT('Ctrl Pts',(17.1111663212568,70.3565280803022,0.));
#103031=CARTESIAN_POINT('Ctrl Pts',(17.1111663212568,70.3565280803022,12.));
#103032=CARTESIAN_POINT('Ctrl Pts',(17.1080486238499,70.3811178111201,0.));
#103033=CARTESIAN_POINT('Ctrl Pts',(17.1080486238499,70.3811178111201,12.));
#103034=CARTESIAN_POINT('Ctrl Pts',(17.1049021947834,70.4057447878624,0.));
#103035=CARTESIAN_POINT('Ctrl Pts',(17.1049021947834,70.4057447878624,12.));
#103036=CARTESIAN_POINT('Ctrl Pts',(17.1017269915292,70.430408894101,0.));
#103037=CARTESIAN_POINT('Ctrl Pts',(17.1017269915292,70.430408894101,12.));
#103038=CARTESIAN_POINT('Ctrl Pts',(17.0985229718124,70.4551100138238,0.));
#103039=CARTESIAN_POINT('Ctrl Pts',(17.0985229718124,70.4551100138238,12.));
#103040=CARTESIAN_POINT('Ctrl Pts',(17.0952900936048,70.4798480314381,0.));
#103041=CARTESIAN_POINT('Ctrl Pts',(17.0952900936048,70.4798480314381,12.));
#103042=CARTESIAN_POINT('Ctrl Pts',(17.0920283151219,70.5046228317677,0.));
#103043=CARTESIAN_POINT('Ctrl Pts',(17.0920283151219,70.5046228317677,12.));
#103044=CARTESIAN_POINT('Ctrl Pts',(17.088737594822,70.5294343000513,0.));
#103045=CARTESIAN_POINT('Ctrl Pts',(17.088737594822,70.5294343000513,12.));
#103046=CARTESIAN_POINT('Ctrl Pts',(17.0854178914087,70.5542823219331,0.));
#103047=CARTESIAN_POINT('Ctrl Pts',(17.0854178914087,70.5542823219331,12.));
#103048=CARTESIAN_POINT('Ctrl Pts',(17.082069163831,70.5791667834582,0.));
#103049=CARTESIAN_POINT('Ctrl Pts',(17.082069163831,70.5791667834582,12.));
#103050=CARTESIAN_POINT('Ctrl Pts',(17.0786913712764,70.6040875710749,0.));
#103051=CARTESIAN_POINT('Ctrl Pts',(17.0786913712764,70.6040875710749,12.));
#103052=CARTESIAN_POINT('Ctrl Pts',(17.0752844731678,70.6290445716337,0.));
#103053=CARTESIAN_POINT('Ctrl Pts',(17.0752844731678,70.6290445716337,12.));
#103054=CARTESIAN_POINT('Ctrl Pts',(17.0718484291624,70.6540376723841,0.));
#103055=CARTESIAN_POINT('Ctrl Pts',(17.0718484291624,70.6540376723841,12.));
#103056=CARTESIAN_POINT('Ctrl Pts',(17.0683831991532,70.6790667609679,0.));
#103057=CARTESIAN_POINT('Ctrl Pts',(17.0683831991532,70.6790667609679,12.));
#103058=CARTESIAN_POINT('Ctrl Pts',(17.0648887432713,70.7041317254125,0.));
#103059=CARTESIAN_POINT('Ctrl Pts',(17.0648887432713,70.7041317254125,12.));
#103060=CARTESIAN_POINT('Ctrl Pts',(17.0613650218787,70.7292324541341,0.));
#103061=CARTESIAN_POINT('Ctrl Pts',(17.0613650218787,70.7292324541341,12.));
#103062=CARTESIAN_POINT('Ctrl Pts',(17.0578119955649,70.7543688359374,0.));
#103063=CARTESIAN_POINT('Ctrl Pts',(17.0578119955649,70.7543688359374,12.));
#103064=CARTESIAN_POINT('Ctrl Pts',(17.0542296251462,70.7795407600127,0.));
#103065=CARTESIAN_POINT('Ctrl Pts',(17.0542296251462,70.7795407600127,12.));
#103066=CARTESIAN_POINT('Ctrl Pts',(17.0506178716664,70.8047481159306,0.));
#103067=CARTESIAN_POINT('Ctrl Pts',(17.0506178716664,70.8047481159306,12.));
#103068=CARTESIAN_POINT('Ctrl Pts',(17.0469766964005,70.8299907936346,0.));
#103069=CARTESIAN_POINT('Ctrl Pts',(17.0469766964005,70.8299907936346,12.));
#103070=CARTESIAN_POINT('Ctrl Pts',(17.0433060608478,70.8552686834435,0.));
#103071=CARTESIAN_POINT('Ctrl Pts',(17.0433060608478,70.8552686834435,12.));
#103072=CARTESIAN_POINT('Ctrl Pts',(17.0396059267279,70.8805816760507,0.));
#103073=CARTESIAN_POINT('Ctrl Pts',(17.0396059267279,70.8805816760507,12.));
#103074=CARTESIAN_POINT('Ctrl Pts',(17.0358762559786,70.9059296625214,0.));
#103075=CARTESIAN_POINT('Ctrl Pts',(17.0358762559786,70.9059296625214,12.));
#103076=CARTESIAN_POINT('Ctrl Pts',(17.0321170107562,70.9313125342872,0.));
#103077=CARTESIAN_POINT('Ctrl Pts',(17.0321170107562,70.9313125342872,12.));
#103078=CARTESIAN_POINT('Ctrl Pts',(17.028328153439,70.9567301831355,0.));
#103079=CARTESIAN_POINT('Ctrl Pts',(17.028328153439,70.9567301831355,12.));
#103080=CARTESIAN_POINT('Ctrl Pts',(17.0245096466228,70.9821825012134,0.));
#103081=CARTESIAN_POINT('Ctrl Pts',(17.0245096466228,70.9821825012134,12.));
#103082=CARTESIAN_POINT('Ctrl Pts',(17.0206614531165,71.0076693810303,0.));
#103083=CARTESIAN_POINT('Ctrl Pts',(17.0206614531165,71.0076693810303,12.));
#103084=CARTESIAN_POINT('Ctrl Pts',(17.0167835359419,71.0331907154575,0.));
#103085=CARTESIAN_POINT('Ctrl Pts',(17.0167835359419,71.0331907154575,12.));
#103086=CARTESIAN_POINT('Ctrl Pts',(17.0128758583335,71.0587463977266,0.));
#103087=CARTESIAN_POINT('Ctrl Pts',(17.0128758583335,71.0587463977266,12.));
#103088=CARTESIAN_POINT('Ctrl Pts',(17.0089383837437,71.0843363214216,0.));
#103089=CARTESIAN_POINT('Ctrl Pts',(17.0089383837437,71.0843363214216,12.));
#103090=CARTESIAN_POINT('Ctrl Pts',(17.0049710758393,71.1099603804779,0.));
#103091=CARTESIAN_POINT('Ctrl Pts',(17.0049710758393,71.1099603804779,12.));
#103092=CARTESIAN_POINT('Ctrl Pts',(17.0009738984935,71.1356184691799,0.));
#103093=CARTESIAN_POINT('Ctrl Pts',(17.0009738984935,71.1356184691799,12.));
#103094=CARTESIAN_POINT('Ctrl Pts',(16.9969468157824,71.1613104821565,0.));
#103095=CARTESIAN_POINT('Ctrl Pts',(16.9969468157824,71.1613104821565,12.));
#103096=CARTESIAN_POINT('Ctrl Pts',(16.9928897919829,71.1870363143742,0.));
#103097=CARTESIAN_POINT('Ctrl Pts',(16.9928897919829,71.1870363143742,12.));
#103098=CARTESIAN_POINT('Ctrl Pts',(16.9888027915743,71.2127958611248,0.));
#103099=CARTESIAN_POINT('Ctrl Pts',(16.9888027915743,71.2127958611248,12.));
#103100=CARTESIAN_POINT('Ctrl Pts',(16.9846857792385,71.2385890180233,0.));
#103101=CARTESIAN_POINT('Ctrl Pts',(16.9846857792385,71.2385890180233,12.));
#103102=CARTESIAN_POINT('Ctrl Pts',(16.9805387198573,71.2644156810209,0.));
#103103=CARTESIAN_POINT('Ctrl Pts',(16.9805387198573,71.2644156810209,12.));
#103104=CARTESIAN_POINT('Ctrl Pts',(16.9763615785138,71.2902757464127,0.));
#103105=CARTESIAN_POINT('Ctrl Pts',(16.9763615785138,71.2902757464127,12.));
#103106=CARTESIAN_POINT('Ctrl Pts',(16.9721543204951,71.3161691108425,0.));
#103107=CARTESIAN_POINT('Ctrl Pts',(16.9721543204951,71.3161691108425,12.));
#103108=CARTESIAN_POINT('Ctrl Pts',(16.9679169112993,71.3420956713072,0.));
#103109=CARTESIAN_POINT('Ctrl Pts',(16.9679169112993,71.3420956713072,12.));
#103110=CARTESIAN_POINT('Ctrl Pts',(16.9636493166395,71.3680553251548,0.));
#103111=CARTESIAN_POINT('Ctrl Pts',(16.9636493166395,71.3680553251548,12.));
#103112=CARTESIAN_POINT('Ctrl Pts',(16.9593515024274,71.3940479700663,0.));
#103113=CARTESIAN_POINT('Ctrl Pts',(16.9593515024274,71.3940479700663,12.));
#103114=CARTESIAN_POINT('Ctrl Pts',(16.9550234347619,71.4200735040374,0.));
#103115=CARTESIAN_POINT('Ctrl Pts',(16.9550234347619,71.4200735040374,12.));
#103116=CARTESIAN_POINT('Ctrl Pts',(16.9506650799188,71.4461318253561,0.));
#103117=CARTESIAN_POINT('Ctrl Pts',(16.9506650799188,71.4461318253561,12.));
#103118=CARTESIAN_POINT('Ctrl Pts',(16.9462764043445,71.4722228325805,0.));
#103119=CARTESIAN_POINT('Ctrl Pts',(16.9462764043445,71.4722228325805,12.));
#103120=CARTESIAN_POINT('Ctrl Pts',(16.9418573746492,71.498346424507,0.));
#103121=CARTESIAN_POINT('Ctrl Pts',(16.9418573746492,71.498346424507,12.));
#103122=CARTESIAN_POINT('Ctrl Pts',(16.9374079576204,71.5245025002154,0.));
#103123=CARTESIAN_POINT('Ctrl Pts',(16.9374079576204,71.5245025002154,12.));
#103124=CARTESIAN_POINT('Ctrl Pts',(16.9329281202379,71.5506909591139,0.));
#103125=CARTESIAN_POINT('Ctrl Pts',(16.9329281202379,71.5506909591139,12.));
#103126=CARTESIAN_POINT('Ctrl Pts',(16.9284178296934,71.5769117009844,0.));
#103127=CARTESIAN_POINT('Ctrl Pts',(16.9284178296934,71.5769117009844,12.));
#103128=CARTESIAN_POINT('Ctrl Pts',(16.923877053407,71.6031646260169,0.));
#103129=CARTESIAN_POINT('Ctrl Pts',(16.923877053407,71.6031646260169,12.));
#103130=CARTESIAN_POINT('Ctrl Pts',(16.9193057590605,71.6294496348644,0.));
#103131=CARTESIAN_POINT('Ctrl Pts',(16.9193057590605,71.6294496348644,12.));
#103132=CARTESIAN_POINT('Ctrl Pts',(16.9147039145715,71.6557666285908,0.));
#103133=CARTESIAN_POINT('Ctrl Pts',(16.9147039145715,71.6557666285908,12.));
#103134=CARTESIAN_POINT('Ctrl Pts',(16.9100714880367,71.6821155085605,0.));
#103135=CARTESIAN_POINT('Ctrl Pts',(16.9100714880367,71.6821155085605,12.));
#103136=CARTESIAN_POINT('Ctrl Pts',(16.9054084476847,71.7084961763355,0.));
#103137=CARTESIAN_POINT('Ctrl Pts',(16.9054084476847,71.7084961763355,12.));
#103138=CARTESIAN_POINT('Ctrl Pts',(16.9007147618344,71.7349085335796,0.));
#103139=CARTESIAN_POINT('Ctrl Pts',(16.9007147618344,71.7349085335796,12.));
#103140=CARTESIAN_POINT('Ctrl Pts',(16.8959903988411,71.761352481924,0.));
#103141=CARTESIAN_POINT('Ctrl Pts',(16.8959903988411,71.761352481924,12.));
#103142=CARTESIAN_POINT('Ctrl Pts',(16.8912353270944,71.7878279229556,0.));
#103143=CARTESIAN_POINT('Ctrl Pts',(16.8912353270944,71.7878279229556,12.));
#103144=CARTESIAN_POINT('Ctrl Pts',(16.8864495151347,71.8143347584977,0.));
#103145=CARTESIAN_POINT('Ctrl Pts',(16.8864495151347,71.8143347584977,12.));
#103146=CARTESIAN_POINT('Ctrl Pts',(16.8816329317473,71.8408728908269,0.));
#103147=CARTESIAN_POINT('Ctrl Pts',(16.8816329317473,71.8408728908269,12.));
#103148=CARTESIAN_POINT('Ctrl Pts',(16.87678554607,71.8674422229151,0.));
#103149=CARTESIAN_POINT('Ctrl Pts',(16.87678554607,71.8674422229151,12.));
#103150=CARTESIAN_POINT('Ctrl Pts',(16.8719073276967,71.8940426586521,0.));
#103151=CARTESIAN_POINT('Ctrl Pts',(16.8719073276967,71.8940426586521,12.));
#103152=CARTESIAN_POINT('Ctrl Pts',(16.8669982467915,71.920674103086,0.));
#103153=CARTESIAN_POINT('Ctrl Pts',(16.8669982467915,71.920674103086,12.));
#103154=CARTESIAN_POINT('Ctrl Pts',(16.8620582738431,71.9473364618889,0.));
#103155=CARTESIAN_POINT('Ctrl Pts',(16.8620582738431,71.9473364618889,12.));
#103156=CARTESIAN_POINT('Ctrl Pts',(16.8570873794264,71.9740296408319,0.));
#103157=CARTESIAN_POINT('Ctrl Pts',(16.8570873794264,71.9740296408319,12.));
#103158=CARTESIAN_POINT('Ctrl Pts',(16.8520855339444,72.0007535452071,0.));
#103159=CARTESIAN_POINT('Ctrl Pts',(16.8520855339444,72.0007535452071,12.));
#103160=CARTESIAN_POINT('Ctrl Pts',(16.8470527074278,72.0275080793742,0.));
#103161=CARTESIAN_POINT('Ctrl Pts',(16.8470527074278,72.0275080793742,12.));
#103162=CARTESIAN_POINT('Ctrl Pts',(16.8419888691984,72.0542931459865,0.));
#103163=CARTESIAN_POINT('Ctrl Pts',(16.8419888691984,72.0542931459865,12.));
#103164=CARTESIAN_POINT('Ctrl Pts',(16.8368939881457,72.0811086466177,0.));
#103165=CARTESIAN_POINT('Ctrl Pts',(16.8368939881457,72.0811086466177,12.));
#103166=CARTESIAN_POINT('Ctrl Pts',(16.8317680333415,72.1079544831569,0.));
#103167=CARTESIAN_POINT('Ctrl Pts',(16.8317680333415,72.1079544831569,12.));
#103168=CARTESIAN_POINT('Ctrl Pts',(16.8266109745801,72.1348305590233,0.));
#103169=CARTESIAN_POINT('Ctrl Pts',(16.8266109745801,72.1348305590233,12.));
#103170=CARTESIAN_POINT('Ctrl Pts',(16.8214227828941,72.1617367803226,0.));
#103171=CARTESIAN_POINT('Ctrl Pts',(16.8214227828941,72.1617367803226,12.));
#103172=CARTESIAN_POINT('Ctrl Pts',(16.8162034312257,72.1886730573389,0.));
#103173=CARTESIAN_POINT('Ctrl Pts',(16.8162034312257,72.1886730573389,12.));
#103174=CARTESIAN_POINT('Ctrl Pts',(16.8109528945876,72.2156393048868,0.));
#103175=CARTESIAN_POINT('Ctrl Pts',(16.8109528945876,72.2156393048868,12.));
#103176=CARTESIAN_POINT('Ctrl Pts',(16.8056711485797,72.242635439009,0.));
#103177=CARTESIAN_POINT('Ctrl Pts',(16.8056711485797,72.242635439009,12.));
#103178=CARTESIAN_POINT('Ctrl Pts',(16.800358168223,72.2696613743687,0.));
#103179=CARTESIAN_POINT('Ctrl Pts',(16.800358168223,72.2696613743687,12.));
#103180=CARTESIAN_POINT('Ctrl Pts',(16.7950139266117,72.2967170212331,0.));
#103181=CARTESIAN_POINT('Ctrl Pts',(16.7950139266117,72.2967170212331,12.));
#103182=CARTESIAN_POINT('Ctrl Pts',(16.7896383937839,72.323802282931,0.));
#103183=CARTESIAN_POINT('Ctrl Pts',(16.7896383937839,72.323802282931,12.));
#103184=CARTESIAN_POINT('Ctrl Pts',(16.7842315351402,72.3509170523038,0.));
#103185=CARTESIAN_POINT('Ctrl Pts',(16.7842315351402,72.3509170523038,12.));
#103186=CARTESIAN_POINT('Ctrl Pts',(16.7787933137551,72.3780612168057,0.));
#103187=CARTESIAN_POINT('Ctrl Pts',(16.7787933137551,72.3780612168057,12.));
#103188=CARTESIAN_POINT('Ctrl Pts',(16.7733236932185,72.4052346648058,0.));
#103189=CARTESIAN_POINT('Ctrl Pts',(16.7733236932185,72.4052346648058,12.));
#103190=CARTESIAN_POINT('Ctrl Pts',(16.7678226404189,72.4324372916884,0.));
#103191=CARTESIAN_POINT('Ctrl Pts',(16.7678226404189,72.4324372916884,12.));
#103192=CARTESIAN_POINT('Ctrl Pts',(16.7622901280741,72.4596690055347,0.));
#103193=CARTESIAN_POINT('Ctrl Pts',(16.7622901280741,72.4596690055347,12.));
#103194=CARTESIAN_POINT('Ctrl Pts',(16.7567261380614,72.4869297342051,0.));
#103195=CARTESIAN_POINT('Ctrl Pts',(16.7567261380614,72.4869297342051,12.));
#103196=CARTESIAN_POINT('Ctrl Pts',(16.7511306618793,72.5142194273203,0.));
#103197=CARTESIAN_POINT('Ctrl Pts',(16.7511306618793,72.5142194273203,12.));
#103198=CARTESIAN_POINT('Ctrl Pts',(16.7455036973724,72.5415380515905,0.));
#103199=CARTESIAN_POINT('Ctrl Pts',(16.7455036973724,72.5415380515905,12.));
#103200=CARTESIAN_POINT('Ctrl Pts',(16.7409769365953,72.563416080574,0.));
#103201=CARTESIAN_POINT('Ctrl Pts',(16.7409769365953,72.563416080574,12.));
#103202=CARTESIAN_POINT('Ctrl Pts',(16.7375676985272,72.5798376087406,0.));
#103203=CARTESIAN_POINT('Ctrl Pts',(16.7375676985272,72.5798376087406,12.));
#103204=CARTESIAN_POINT('Ctrl Pts',(16.7352885767459,72.5907910745874,0.));
#103205=CARTESIAN_POINT('Ctrl Pts',(16.7352885767459,72.5907910745874,12.));
#103206=CARTESIAN_POINT('Ctrl Pts',(16.7341474417544,72.5962692526112,0.));
#103207=CARTESIAN_POINT('Ctrl Pts',(16.7341474417544,72.5962692526112,12.));
#103208=CARTESIAN_POINT('',(17.2912529479484,67.8307641965655,0.));
#103209=CARTESIAN_POINT('Ctrl Pts',(17.2912529479484,67.8307641965655,0.));
#103210=CARTESIAN_POINT('Ctrl Pts',(17.2912149114119,67.8346476309018,0.));
#103211=CARTESIAN_POINT('Ctrl Pts',(17.2911366591348,67.842419897098,0.));
#103212=CARTESIAN_POINT('Ctrl Pts',(17.291012743109,67.8540944889687,0.));
#103213=CARTESIAN_POINT('Ctrl Pts',(17.2908344459694,67.8696929978782,0.));
#103214=CARTESIAN_POINT('Ctrl Pts',(17.2905897723949,67.8892451049608,0.));
#103215=CARTESIAN_POINT('Ctrl Pts',(17.2903232740694,67.9088511496686,0.));
#103216=CARTESIAN_POINT('Ctrl Pts',(17.2900349103981,67.9285110571741,0.));
#103217=CARTESIAN_POINT('Ctrl Pts',(17.2897246158941,67.9482246901667,0.));
#103218=CARTESIAN_POINT('Ctrl Pts',(17.2893923013894,67.9679918502579,0.));
#103219=CARTESIAN_POINT('Ctrl Pts',(17.2890378644866,67.987812304921,0.));
#103220=CARTESIAN_POINT('Ctrl Pts',(17.28866119774,68.007685808115,0.));
#103221=CARTESIAN_POINT('Ctrl Pts',(17.2882621974721,68.0276121227356,0.));
#103222=CARTESIAN_POINT('Ctrl Pts',(17.2878407730961,68.0475910442424,0.));
#103223=CARTESIAN_POINT('Ctrl Pts',(17.2873968440839,68.0676223930412,0.));
#103224=CARTESIAN_POINT('Ctrl Pts',(17.2869303355432,68.0877060033205,0.));
#103225=CARTESIAN_POINT('Ctrl Pts',(17.2864411745459,68.1078417137877,0.));
#103226=CARTESIAN_POINT('Ctrl Pts',(17.2859292855705,68.1280293561511,0.));
#103227=CARTESIAN_POINT('Ctrl Pts',(17.2853945882072,68.1482687493226,0.));
#103228=CARTESIAN_POINT('Ctrl Pts',(17.2848369995293,68.1685597054232,0.));
#103229=CARTESIAN_POINT('Ctrl Pts',(17.2842564355799,68.1889020335427,0.));
#103230=CARTESIAN_POINT('Ctrl Pts',(17.2836528130819,68.2092955440567,0.));
#103231=CARTESIAN_POINT('Ctrl Pts',(17.2830260513867,68.2297400535294,0.));
#103232=CARTESIAN_POINT('Ctrl Pts',(17.2823760723874,68.2502353845071,0.));
#103233=CARTESIAN_POINT('Ctrl Pts',(17.2817027995831,68.2707813631731,0.));
#103234=CARTESIAN_POINT('Ctrl Pts',(17.2810061574353,68.2913778177261,0.));
#103235=CARTESIAN_POINT('Ctrl Pts',(17.2802860705815,68.3120245763914,0.));
#103236=CARTESIAN_POINT('Ctrl Pts',(17.2795424631799,68.3327214657575,0.));
#103237=CARTESIAN_POINT('Ctrl Pts',(17.2787752592484,68.3534683116515,0.));
#103238=CARTESIAN_POINT('Ctrl Pts',(17.2779843829608,68.3742649398964,0.));
#103239=CARTESIAN_POINT('Ctrl Pts',(17.2771697589384,68.3951111770487,0.));
#103240=CARTESIAN_POINT('Ctrl Pts',(17.2763313126018,68.4160068512753,0.));
#103241=CARTESIAN_POINT('Ctrl Pts',(17.2754689702992,68.436951792677,0.));
#103242=CARTESIAN_POINT('Ctrl Pts',(17.2745826591119,68.4579458328185,0.));
#103243=CARTESIAN_POINT('Ctrl Pts',(17.2736723067365,68.4789888044351,0.));
#103244=CARTESIAN_POINT('Ctrl Pts',(17.2727378413489,68.5000805410911,0.));
#103245=CARTESIAN_POINT('Ctrl Pts',(17.2717791914544,68.521220876786,0.));
#103246=CARTESIAN_POINT('Ctrl Pts',(17.2707962858919,68.5424096459772,0.));
#103247=CARTESIAN_POINT('Ctrl Pts',(17.269789053896,68.5636466837517,0.));
#103248=CARTESIAN_POINT('Ctrl Pts',(17.2687574251429,68.5849318259449,0.));
#103249=CARTESIAN_POINT('Ctrl Pts',(17.2677013298057,68.6062649092764,0.));
#103250=CARTESIAN_POINT('Ctrl Pts',(17.2666206986084,68.6276457714729,0.));
#103251=CARTESIAN_POINT('Ctrl Pts',(17.2655154627928,68.6490742512057,0.));
#103252=CARTESIAN_POINT('Ctrl Pts',(17.2643855540892,68.6705501880249,0.));
#103253=CARTESIAN_POINT('Ctrl Pts',(17.2632309046892,68.6920734222938,0.));
#103254=CARTESIAN_POINT('Ctrl Pts',(17.2620514472182,68.7136437951097,0.));
#103255=CARTESIAN_POINT('Ctrl Pts',(17.2608471147185,68.7352611482547,0.));
#103256=CARTESIAN_POINT('Ctrl Pts',(17.259617840655,68.7569253242333,0.));
#103257=CARTESIAN_POINT('Ctrl Pts',(17.2583635589198,68.7786361662882,0.));
#103258=CARTESIAN_POINT('Ctrl Pts',(17.2570842038383,68.8003935184184,0.));
#103259=CARTESIAN_POINT('Ctrl Pts',(17.2557797101812,68.8221972253941,0.));
#103260=CARTESIAN_POINT('Ctrl Pts',(17.2544500131624,68.844047132755,0.));
#103261=CARTESIAN_POINT('Ctrl Pts',(17.2530950484258,68.8659430867972,0.));
#103262=CARTESIAN_POINT('Ctrl Pts',(17.2517147520376,68.8878849345557,0.));
#103263=CARTESIAN_POINT('Ctrl Pts',(17.2503090604792,68.909872523787,0.));
#103264=CARTESIAN_POINT('Ctrl Pts',(17.248877910643,68.9319057029409,0.));
#103265=CARTESIAN_POINT('Ctrl Pts',(17.2474212398275,68.9539843211619,0.));
#103266=CARTESIAN_POINT('Ctrl Pts',(17.2459389857327,68.9761082282922,0.));
#103267=CARTESIAN_POINT('Ctrl Pts',(17.2444310864585,68.9982772748694,0.));
#103268=CARTESIAN_POINT('Ctrl Pts',(17.2428974805044,69.0204913121225,0.));
#103269=CARTESIAN_POINT('Ctrl Pts',(17.2413381067723,69.0427501919636,0.));
#103270=CARTESIAN_POINT('Ctrl Pts',(17.2397529045589,69.065053766986,0.));
#103271=CARTESIAN_POINT('Ctrl Pts',(17.2381418135491,69.0874018904599,0.));
#103272=CARTESIAN_POINT('Ctrl Pts',(17.2365047738125,69.1097944163245,0.));
#103273=CARTESIAN_POINT('Ctrl Pts',(17.2348417258015,69.1322311991752,0.));
#103274=CARTESIAN_POINT('Ctrl Pts',(17.2331526103506,69.1547120942527,0.));
#103275=CARTESIAN_POINT('Ctrl Pts',(17.23143736867,69.1772369574447,0.));
#103276=CARTESIAN_POINT('Ctrl Pts',(17.2296959423407,69.1998056452828,0.));
#103277=CARTESIAN_POINT('Ctrl Pts',(17.227928273312,69.222418014938,0.));
#103278=CARTESIAN_POINT('Ctrl Pts',(17.226134303902,69.2450739242109,0.));
#103279=CARTESIAN_POINT('Ctrl Pts',(17.224313976797,69.2677732315224,0.));
#103280=CARTESIAN_POINT('Ctrl Pts',(17.2224672350438,69.2905157959166,0.));
#103281=CARTESIAN_POINT('Ctrl Pts',(17.2205940220459,69.3133014770555,0.));
#103282=CARTESIAN_POINT('Ctrl Pts',(17.2186942815602,69.3361301352141,0.));
#103283=CARTESIAN_POINT('Ctrl Pts',(17.2167679576984,69.3590016312692,0.));
#103284=CARTESIAN_POINT('Ctrl Pts',(17.2148149949252,69.3819158266916,0.));
#103285=CARTESIAN_POINT('Ctrl Pts',(17.2128353380502,69.404872583548,0.));
#103286=CARTESIAN_POINT('Ctrl Pts',(17.2108289322254,69.4278717644973,0.));
#103287=CARTESIAN_POINT('Ctrl Pts',(17.2087957229423,69.450913232785,0.));
#103288=CARTESIAN_POINT('Ctrl Pts',(17.2067356560336,69.4739968522313,0.));
#103289=CARTESIAN_POINT('Ctrl Pts',(17.2046486776708,69.4971224872269,0.));
#103290=CARTESIAN_POINT('Ctrl Pts',(17.2025347343577,69.5202900027367,0.));
#103291=CARTESIAN_POINT('Ctrl Pts',(17.2003937729268,69.5434992642944,0.));
#103292=CARTESIAN_POINT('Ctrl Pts',(17.1982257405377,69.5667501379969,0.));
#103293=CARTESIAN_POINT('Ctrl Pts',(17.196030584678,69.5900424904921,0.));
#103294=CARTESIAN_POINT('Ctrl Pts',(17.1938082531612,69.6133761889749,0.));
#103295=CARTESIAN_POINT('Ctrl Pts',(17.1915586941192,69.6367511011898,0.));
#103296=CARTESIAN_POINT('Ctrl Pts',(17.1892818560002,69.6601670954269,0.));
#103297=CARTESIAN_POINT('Ctrl Pts',(17.1869776875666,69.6836240405164,0.));
#103298=CARTESIAN_POINT('Ctrl Pts',(17.1846461378973,69.7071218058178,0.));
#103299=CARTESIAN_POINT('Ctrl Pts',(17.1822871563842,69.7306602612155,0.));
#103300=CARTESIAN_POINT('Ctrl Pts',(17.179900692726,69.7542392771234,0.));
#103301=CARTESIAN_POINT('Ctrl Pts',(17.1774866969256,69.777858724479,0.));
#103302=CARTESIAN_POINT('Ctrl Pts',(17.1750451192885,69.8015184747398,0.));
#103303=CARTESIAN_POINT('Ctrl Pts',(17.1725759104252,69.8252183998702,0.));
#103304=CARTESIAN_POINT('Ctrl Pts',(17.1700790212474,69.8489583723407,0.));
#103305=CARTESIAN_POINT('Ctrl Pts',(17.167554402962,69.8727382651286,0.));
#103306=CARTESIAN_POINT('Ctrl Pts',(17.1650020070686,69.8965579517147,0.));
#103307=CARTESIAN_POINT('Ctrl Pts',(17.1624217853578,69.9204173060781,0.));
#103308=CARTESIAN_POINT('Ctrl Pts',(17.1598136899144,69.9443162026865,0.));
#103309=CARTESIAN_POINT('Ctrl Pts',(17.157177673114,69.9682545164939,0.));
#103310=CARTESIAN_POINT('Ctrl Pts',(17.154513687616,69.9922321229424,0.));
#103311=CARTESIAN_POINT('Ctrl Pts',(17.1518216863623,70.0162488979584,0.));
#103312=CARTESIAN_POINT('Ctrl Pts',(17.1491016225749,70.0403047179483,0.));
#103313=CARTESIAN_POINT('Ctrl Pts',(17.1463534497594,70.0643994597873,0.));
#103314=CARTESIAN_POINT('Ctrl Pts',(17.1435771217018,70.0885330008179,0.));
#103315=CARTESIAN_POINT('Ctrl Pts',(17.1407725924617,70.1127052188522,0.));
#103316=CARTESIAN_POINT('Ctrl Pts',(17.1379398163709,70.1369159921687,0.));
#103317=CARTESIAN_POINT('Ctrl Pts',(17.1350787480312,70.1611651995083,0.));
#103318=CARTESIAN_POINT('Ctrl Pts',(17.1321893423182,70.1854527200631,0.));
#103319=CARTESIAN_POINT('Ctrl Pts',(17.1292715543778,70.2097784334747,0.));
#103320=CARTESIAN_POINT('Ctrl Pts',(17.1263253396202,70.2341422198363,0.));
#103321=CARTESIAN_POINT('Ctrl Pts',(17.1233506537176,70.2585439596901,0.));
#103322=CARTESIAN_POINT('Ctrl Pts',(17.1203474526031,70.2829835340238,0.));
#103323=CARTESIAN_POINT('Ctrl Pts',(17.1173156924733,70.3074608242608,0.));
#103324=CARTESIAN_POINT('Ctrl Pts',(17.1142553297867,70.3319757122568,0.));
#103325=CARTESIAN_POINT('Ctrl Pts',(17.1111663212568,70.3565280803022,0.));
#103326=CARTESIAN_POINT('Ctrl Pts',(17.1080486238499,70.3811178111201,0.));
#103327=CARTESIAN_POINT('Ctrl Pts',(17.1049021947834,70.4057447878624,0.));
#103328=CARTESIAN_POINT('Ctrl Pts',(17.1017269915292,70.430408894101,0.));
#103329=CARTESIAN_POINT('Ctrl Pts',(17.0985229718124,70.4551100138238,0.));
#103330=CARTESIAN_POINT('Ctrl Pts',(17.0952900936048,70.4798480314381,0.));
#103331=CARTESIAN_POINT('Ctrl Pts',(17.0920283151219,70.5046228317677,0.));
#103332=CARTESIAN_POINT('Ctrl Pts',(17.088737594822,70.5294343000513,0.));
#103333=CARTESIAN_POINT('Ctrl Pts',(17.0854178914087,70.5542823219331,0.));
#103334=CARTESIAN_POINT('Ctrl Pts',(17.082069163831,70.5791667834582,0.));
#103335=CARTESIAN_POINT('Ctrl Pts',(17.0786913712764,70.6040875710749,0.));
#103336=CARTESIAN_POINT('Ctrl Pts',(17.0752844731678,70.6290445716337,0.));
#103337=CARTESIAN_POINT('Ctrl Pts',(17.0718484291624,70.6540376723841,0.));
#103338=CARTESIAN_POINT('Ctrl Pts',(17.0683831991532,70.6790667609679,0.));
#103339=CARTESIAN_POINT('Ctrl Pts',(17.0648887432713,70.7041317254125,0.));
#103340=CARTESIAN_POINT('Ctrl Pts',(17.0613650218787,70.7292324541341,0.));
#103341=CARTESIAN_POINT('Ctrl Pts',(17.0578119955649,70.7543688359374,0.));
#103342=CARTESIAN_POINT('Ctrl Pts',(17.0542296251462,70.7795407600127,0.));
#103343=CARTESIAN_POINT('Ctrl Pts',(17.0506178716664,70.8047481159306,0.));
#103344=CARTESIAN_POINT('Ctrl Pts',(17.0469766964005,70.8299907936346,0.));
#103345=CARTESIAN_POINT('Ctrl Pts',(17.0433060608478,70.8552686834435,0.));
#103346=CARTESIAN_POINT('Ctrl Pts',(17.0396059267279,70.8805816760507,0.));
#103347=CARTESIAN_POINT('Ctrl Pts',(17.0358762559786,70.9059296625214,0.));
#103348=CARTESIAN_POINT('Ctrl Pts',(17.0321170107562,70.9313125342872,0.));
#103349=CARTESIAN_POINT('Ctrl Pts',(17.028328153439,70.9567301831355,0.));
#103350=CARTESIAN_POINT('Ctrl Pts',(17.0245096466228,70.9821825012134,0.));
#103351=CARTESIAN_POINT('Ctrl Pts',(17.0206614531165,71.0076693810303,0.));
#103352=CARTESIAN_POINT('Ctrl Pts',(17.0167835359419,71.0331907154575,0.));
#103353=CARTESIAN_POINT('Ctrl Pts',(17.0128758583335,71.0587463977266,0.));
#103354=CARTESIAN_POINT('Ctrl Pts',(17.0089383837437,71.0843363214216,0.));
#103355=CARTESIAN_POINT('Ctrl Pts',(17.0049710758393,71.1099603804779,0.));
#103356=CARTESIAN_POINT('Ctrl Pts',(17.0009738984935,71.1356184691799,0.));
#103357=CARTESIAN_POINT('Ctrl Pts',(16.9969468157824,71.1613104821565,0.));
#103358=CARTESIAN_POINT('Ctrl Pts',(16.9928897919829,71.1870363143742,0.));
#103359=CARTESIAN_POINT('Ctrl Pts',(16.9888027915743,71.2127958611248,0.));
#103360=CARTESIAN_POINT('Ctrl Pts',(16.9846857792385,71.2385890180233,0.));
#103361=CARTESIAN_POINT('Ctrl Pts',(16.9805387198573,71.2644156810209,0.));
#103362=CARTESIAN_POINT('Ctrl Pts',(16.9763615785138,71.2902757464127,0.));
#103363=CARTESIAN_POINT('Ctrl Pts',(16.9721543204951,71.3161691108425,0.));
#103364=CARTESIAN_POINT('Ctrl Pts',(16.9679169112993,71.3420956713072,0.));
#103365=CARTESIAN_POINT('Ctrl Pts',(16.9636493166395,71.3680553251548,0.));
#103366=CARTESIAN_POINT('Ctrl Pts',(16.9593515024274,71.3940479700663,0.));
#103367=CARTESIAN_POINT('Ctrl Pts',(16.9550234347619,71.4200735040374,0.));
#103368=CARTESIAN_POINT('Ctrl Pts',(16.9506650799188,71.4461318253561,0.));
#103369=CARTESIAN_POINT('Ctrl Pts',(16.9462764043445,71.4722228325805,0.));
#103370=CARTESIAN_POINT('Ctrl Pts',(16.9418573746492,71.498346424507,0.));
#103371=CARTESIAN_POINT('Ctrl Pts',(16.9374079576204,71.5245025002154,0.));
#103372=CARTESIAN_POINT('Ctrl Pts',(16.9329281202379,71.5506909591139,0.));
#103373=CARTESIAN_POINT('Ctrl Pts',(16.9284178296934,71.5769117009844,0.));
#103374=CARTESIAN_POINT('Ctrl Pts',(16.923877053407,71.6031646260169,0.));
#103375=CARTESIAN_POINT('Ctrl Pts',(16.9193057590605,71.6294496348644,0.));
#103376=CARTESIAN_POINT('Ctrl Pts',(16.9147039145715,71.6557666285908,0.));
#103377=CARTESIAN_POINT('Ctrl Pts',(16.9100714880367,71.6821155085605,0.));
#103378=CARTESIAN_POINT('Ctrl Pts',(16.9054084476847,71.7084961763355,0.));
#103379=CARTESIAN_POINT('Ctrl Pts',(16.9007147618344,71.7349085335796,0.));
#103380=CARTESIAN_POINT('Ctrl Pts',(16.8959903988411,71.761352481924,0.));
#103381=CARTESIAN_POINT('Ctrl Pts',(16.8912353270944,71.7878279229556,0.));
#103382=CARTESIAN_POINT('Ctrl Pts',(16.8864495151347,71.8143347584977,0.));
#103383=CARTESIAN_POINT('Ctrl Pts',(16.8816329317473,71.8408728908269,0.));
#103384=CARTESIAN_POINT('Ctrl Pts',(16.87678554607,71.8674422229151,0.));
#103385=CARTESIAN_POINT('Ctrl Pts',(16.8719073276967,71.8940426586521,0.));
#103386=CARTESIAN_POINT('Ctrl Pts',(16.8669982467915,71.920674103086,0.));
#103387=CARTESIAN_POINT('Ctrl Pts',(16.8620582738431,71.9473364618889,0.));
#103388=CARTESIAN_POINT('Ctrl Pts',(16.8570873794264,71.9740296408319,0.));
#103389=CARTESIAN_POINT('Ctrl Pts',(16.8520855339444,72.0007535452071,0.));
#103390=CARTESIAN_POINT('Ctrl Pts',(16.8470527074278,72.0275080793742,0.));
#103391=CARTESIAN_POINT('Ctrl Pts',(16.8419888691984,72.0542931459865,0.));
#103392=CARTESIAN_POINT('Ctrl Pts',(16.8368939881457,72.0811086466177,0.));
#103393=CARTESIAN_POINT('Ctrl Pts',(16.8317680333415,72.1079544831569,0.));
#103394=CARTESIAN_POINT('Ctrl Pts',(16.8266109745801,72.1348305590233,0.));
#103395=CARTESIAN_POINT('Ctrl Pts',(16.8214227828941,72.1617367803226,0.));
#103396=CARTESIAN_POINT('Ctrl Pts',(16.8162034312257,72.1886730573389,0.));
#103397=CARTESIAN_POINT('Ctrl Pts',(16.8109528945876,72.2156393048868,0.));
#103398=CARTESIAN_POINT('Ctrl Pts',(16.8064254147766,72.2387802230663,0.));
#103399=CARTESIAN_POINT('Ctrl Pts',(16.8029374213802,72.2565380035008,0.));
#103400=CARTESIAN_POINT('Ctrl Pts',(16.8005027425889,72.2688994294959,0.));
#103401=CARTESIAN_POINT('Ctrl Pts',(16.7991305317793,72.2758557890967,0.));
#103402=CARTESIAN_POINT('Ctrl Pts',(16.7988252568807,72.2774028393484,0.));
#103403=CARTESIAN_POINT('',(17.2912529479484,67.8307641965655,12.));
#103404=CARTESIAN_POINT('',(17.2912529479484,67.8307641965655,0.));
#103405=CARTESIAN_POINT('Ctrl Pts',(16.7988252568807,72.2774028393484,12.));
#103406=CARTESIAN_POINT('Ctrl Pts',(16.7991305317793,72.2758557890967,12.));
#103407=CARTESIAN_POINT('Ctrl Pts',(16.8005027425889,72.2688994294959,12.));
#103408=CARTESIAN_POINT('Ctrl Pts',(16.8029374213802,72.2565380035008,12.));
#103409=CARTESIAN_POINT('Ctrl Pts',(16.8064254147766,72.2387802230663,12.));
#103410=CARTESIAN_POINT('Ctrl Pts',(16.8109528945876,72.2156393048868,12.));
#103411=CARTESIAN_POINT('Ctrl Pts',(16.8162034312257,72.1886730573389,12.));
#103412=CARTESIAN_POINT('Ctrl Pts',(16.8214227828941,72.1617367803226,12.));
#103413=CARTESIAN_POINT('Ctrl Pts',(16.8266109745801,72.1348305590233,12.));
#103414=CARTESIAN_POINT('Ctrl Pts',(16.8317680333415,72.1079544831569,12.));
#103415=CARTESIAN_POINT('Ctrl Pts',(16.8368939881457,72.0811086466177,12.));
#103416=CARTESIAN_POINT('Ctrl Pts',(16.8419888691984,72.0542931459865,12.));
#103417=CARTESIAN_POINT('Ctrl Pts',(16.8470527074278,72.0275080793742,12.));
#103418=CARTESIAN_POINT('Ctrl Pts',(16.8520855339444,72.0007535452071,12.));
#103419=CARTESIAN_POINT('Ctrl Pts',(16.8570873794264,71.9740296408319,12.));
#103420=CARTESIAN_POINT('Ctrl Pts',(16.8620582738431,71.9473364618889,12.));
#103421=CARTESIAN_POINT('Ctrl Pts',(16.8669982467915,71.920674103086,12.));
#103422=CARTESIAN_POINT('Ctrl Pts',(16.8719073276967,71.8940426586521,12.));
#103423=CARTESIAN_POINT('Ctrl Pts',(16.87678554607,71.8674422229151,12.));
#103424=CARTESIAN_POINT('Ctrl Pts',(16.8816329317473,71.8408728908269,12.));
#103425=CARTESIAN_POINT('Ctrl Pts',(16.8864495151347,71.8143347584977,12.));
#103426=CARTESIAN_POINT('Ctrl Pts',(16.8912353270944,71.7878279229556,12.));
#103427=CARTESIAN_POINT('Ctrl Pts',(16.8959903988411,71.761352481924,12.));
#103428=CARTESIAN_POINT('Ctrl Pts',(16.9007147618344,71.7349085335796,12.));
#103429=CARTESIAN_POINT('Ctrl Pts',(16.9054084476847,71.7084961763355,12.));
#103430=CARTESIAN_POINT('Ctrl Pts',(16.9100714880367,71.6821155085605,12.));
#103431=CARTESIAN_POINT('Ctrl Pts',(16.9147039145715,71.6557666285908,12.));
#103432=CARTESIAN_POINT('Ctrl Pts',(16.9193057590605,71.6294496348644,12.));
#103433=CARTESIAN_POINT('Ctrl Pts',(16.923877053407,71.6031646260169,12.));
#103434=CARTESIAN_POINT('Ctrl Pts',(16.9284178296934,71.5769117009844,12.));
#103435=CARTESIAN_POINT('Ctrl Pts',(16.9329281202379,71.5506909591139,12.));
#103436=CARTESIAN_POINT('Ctrl Pts',(16.9374079576204,71.5245025002154,12.));
#103437=CARTESIAN_POINT('Ctrl Pts',(16.9418573746492,71.498346424507,12.));
#103438=CARTESIAN_POINT('Ctrl Pts',(16.9462764043445,71.4722228325805,12.));
#103439=CARTESIAN_POINT('Ctrl Pts',(16.9506650799188,71.4461318253561,12.));
#103440=CARTESIAN_POINT('Ctrl Pts',(16.9550234347619,71.4200735040374,12.));
#103441=CARTESIAN_POINT('Ctrl Pts',(16.9593515024274,71.3940479700663,12.));
#103442=CARTESIAN_POINT('Ctrl Pts',(16.9636493166395,71.3680553251548,12.));
#103443=CARTESIAN_POINT('Ctrl Pts',(16.9679169112993,71.3420956713072,12.));
#103444=CARTESIAN_POINT('Ctrl Pts',(16.9721543204951,71.3161691108425,12.));
#103445=CARTESIAN_POINT('Ctrl Pts',(16.9763615785138,71.2902757464127,12.));
#103446=CARTESIAN_POINT('Ctrl Pts',(16.9805387198573,71.2644156810209,12.));
#103447=CARTESIAN_POINT('Ctrl Pts',(16.9846857792385,71.2385890180233,12.));
#103448=CARTESIAN_POINT('Ctrl Pts',(16.9888027915743,71.2127958611248,12.));
#103449=CARTESIAN_POINT('Ctrl Pts',(16.9928897919829,71.1870363143742,12.));
#103450=CARTESIAN_POINT('Ctrl Pts',(16.9969468157824,71.1613104821565,12.));
#103451=CARTESIAN_POINT('Ctrl Pts',(17.0009738984935,71.1356184691799,12.));
#103452=CARTESIAN_POINT('Ctrl Pts',(17.0049710758393,71.1099603804779,12.));
#103453=CARTESIAN_POINT('Ctrl Pts',(17.0089383837437,71.0843363214216,12.));
#103454=CARTESIAN_POINT('Ctrl Pts',(17.0128758583335,71.0587463977266,12.));
#103455=CARTESIAN_POINT('Ctrl Pts',(17.0167835359419,71.0331907154575,12.));
#103456=CARTESIAN_POINT('Ctrl Pts',(17.0206614531165,71.0076693810303,12.));
#103457=CARTESIAN_POINT('Ctrl Pts',(17.0245096466228,70.9821825012134,12.));
#103458=CARTESIAN_POINT('Ctrl Pts',(17.028328153439,70.9567301831355,12.));
#103459=CARTESIAN_POINT('Ctrl Pts',(17.0321170107562,70.9313125342872,12.));
#103460=CARTESIAN_POINT('Ctrl Pts',(17.0358762559786,70.9059296625214,12.));
#103461=CARTESIAN_POINT('Ctrl Pts',(17.0396059267279,70.8805816760507,12.));
#103462=CARTESIAN_POINT('Ctrl Pts',(17.0433060608478,70.8552686834435,12.));
#103463=CARTESIAN_POINT('Ctrl Pts',(17.0469766964005,70.8299907936346,12.));
#103464=CARTESIAN_POINT('Ctrl Pts',(17.0506178716664,70.8047481159306,12.));
#103465=CARTESIAN_POINT('Ctrl Pts',(17.0542296251462,70.7795407600127,12.));
#103466=CARTESIAN_POINT('Ctrl Pts',(17.0578119955649,70.7543688359374,12.));
#103467=CARTESIAN_POINT('Ctrl Pts',(17.0613650218787,70.7292324541341,12.));
#103468=CARTESIAN_POINT('Ctrl Pts',(17.0648887432713,70.7041317254125,12.));
#103469=CARTESIAN_POINT('Ctrl Pts',(17.0683831991532,70.6790667609679,12.));
#103470=CARTESIAN_POINT('Ctrl Pts',(17.0718484291624,70.6540376723841,12.));
#103471=CARTESIAN_POINT('Ctrl Pts',(17.0752844731678,70.6290445716337,12.));
#103472=CARTESIAN_POINT('Ctrl Pts',(17.0786913712764,70.6040875710749,12.));
#103473=CARTESIAN_POINT('Ctrl Pts',(17.082069163831,70.5791667834582,12.));
#103474=CARTESIAN_POINT('Ctrl Pts',(17.0854178914087,70.5542823219331,12.));
#103475=CARTESIAN_POINT('Ctrl Pts',(17.088737594822,70.5294343000513,12.));
#103476=CARTESIAN_POINT('Ctrl Pts',(17.0920283151219,70.5046228317677,12.));
#103477=CARTESIAN_POINT('Ctrl Pts',(17.0952900936048,70.4798480314381,12.));
#103478=CARTESIAN_POINT('Ctrl Pts',(17.0985229718124,70.4551100138238,12.));
#103479=CARTESIAN_POINT('Ctrl Pts',(17.1017269915292,70.430408894101,12.));
#103480=CARTESIAN_POINT('Ctrl Pts',(17.1049021947834,70.4057447878624,12.));
#103481=CARTESIAN_POINT('Ctrl Pts',(17.1080486238499,70.3811178111201,12.));
#103482=CARTESIAN_POINT('Ctrl Pts',(17.1111663212568,70.3565280803022,12.));
#103483=CARTESIAN_POINT('Ctrl Pts',(17.1142553297867,70.3319757122568,12.));
#103484=CARTESIAN_POINT('Ctrl Pts',(17.1173156924733,70.3074608242608,12.));
#103485=CARTESIAN_POINT('Ctrl Pts',(17.1203474526031,70.2829835340238,12.));
#103486=CARTESIAN_POINT('Ctrl Pts',(17.1233506537176,70.2585439596901,12.));
#103487=CARTESIAN_POINT('Ctrl Pts',(17.1263253396202,70.2341422198363,12.));
#103488=CARTESIAN_POINT('Ctrl Pts',(17.1292715543778,70.2097784334747,12.));
#103489=CARTESIAN_POINT('Ctrl Pts',(17.1321893423182,70.1854527200631,12.));
#103490=CARTESIAN_POINT('Ctrl Pts',(17.1350787480312,70.1611651995083,12.));
#103491=CARTESIAN_POINT('Ctrl Pts',(17.1379398163709,70.1369159921687,12.));
#103492=CARTESIAN_POINT('Ctrl Pts',(17.1407725924617,70.1127052188522,12.));
#103493=CARTESIAN_POINT('Ctrl Pts',(17.1435771217018,70.0885330008179,12.));
#103494=CARTESIAN_POINT('Ctrl Pts',(17.1463534497594,70.0643994597873,12.));
#103495=CARTESIAN_POINT('Ctrl Pts',(17.1491016225749,70.0403047179483,12.));
#103496=CARTESIAN_POINT('Ctrl Pts',(17.1518216863623,70.0162488979584,12.));
#103497=CARTESIAN_POINT('Ctrl Pts',(17.154513687616,69.9922321229424,12.));
#103498=CARTESIAN_POINT('Ctrl Pts',(17.157177673114,69.9682545164939,12.));
#103499=CARTESIAN_POINT('Ctrl Pts',(17.1598136899144,69.9443162026865,12.));
#103500=CARTESIAN_POINT('Ctrl Pts',(17.1624217853578,69.9204173060781,12.));
#103501=CARTESIAN_POINT('Ctrl Pts',(17.1650020070686,69.8965579517147,12.));
#103502=CARTESIAN_POINT('Ctrl Pts',(17.167554402962,69.8727382651286,12.));
#103503=CARTESIAN_POINT('Ctrl Pts',(17.1700790212474,69.8489583723407,12.));
#103504=CARTESIAN_POINT('Ctrl Pts',(17.1725759104252,69.8252183998702,12.));
#103505=CARTESIAN_POINT('Ctrl Pts',(17.1750451192885,69.8015184747398,12.));
#103506=CARTESIAN_POINT('Ctrl Pts',(17.1774866969256,69.777858724479,12.));
#103507=CARTESIAN_POINT('Ctrl Pts',(17.179900692726,69.7542392771234,12.));
#103508=CARTESIAN_POINT('Ctrl Pts',(17.1822871563842,69.7306602612155,12.));
#103509=CARTESIAN_POINT('Ctrl Pts',(17.1846461378973,69.7071218058178,12.));
#103510=CARTESIAN_POINT('Ctrl Pts',(17.1869776875666,69.6836240405164,12.));
#103511=CARTESIAN_POINT('Ctrl Pts',(17.1892818560002,69.6601670954269,12.));
#103512=CARTESIAN_POINT('Ctrl Pts',(17.1915586941192,69.6367511011898,12.));
#103513=CARTESIAN_POINT('Ctrl Pts',(17.1938082531612,69.6133761889749,12.));
#103514=CARTESIAN_POINT('Ctrl Pts',(17.196030584678,69.5900424904921,12.));
#103515=CARTESIAN_POINT('Ctrl Pts',(17.1982257405377,69.5667501379969,12.));
#103516=CARTESIAN_POINT('Ctrl Pts',(17.2003937729268,69.5434992642944,12.));
#103517=CARTESIAN_POINT('Ctrl Pts',(17.2025347343577,69.5202900027367,12.));
#103518=CARTESIAN_POINT('Ctrl Pts',(17.2046486776708,69.4971224872269,12.));
#103519=CARTESIAN_POINT('Ctrl Pts',(17.2067356560336,69.4739968522313,12.));
#103520=CARTESIAN_POINT('Ctrl Pts',(17.2087957229423,69.450913232785,12.));
#103521=CARTESIAN_POINT('Ctrl Pts',(17.2108289322254,69.4278717644973,12.));
#103522=CARTESIAN_POINT('Ctrl Pts',(17.2128353380502,69.404872583548,12.));
#103523=CARTESIAN_POINT('Ctrl Pts',(17.2148149949252,69.3819158266916,12.));
#103524=CARTESIAN_POINT('Ctrl Pts',(17.2167679576984,69.3590016312692,12.));
#103525=CARTESIAN_POINT('Ctrl Pts',(17.2186942815602,69.3361301352141,12.));
#103526=CARTESIAN_POINT('Ctrl Pts',(17.2205940220459,69.3133014770555,12.));
#103527=CARTESIAN_POINT('Ctrl Pts',(17.2224672350438,69.2905157959166,12.));
#103528=CARTESIAN_POINT('Ctrl Pts',(17.224313976797,69.2677732315224,12.));
#103529=CARTESIAN_POINT('Ctrl Pts',(17.226134303902,69.2450739242109,12.));
#103530=CARTESIAN_POINT('Ctrl Pts',(17.227928273312,69.222418014938,12.));
#103531=CARTESIAN_POINT('Ctrl Pts',(17.2296959423407,69.1998056452828,12.));
#103532=CARTESIAN_POINT('Ctrl Pts',(17.23143736867,69.1772369574447,12.));
#103533=CARTESIAN_POINT('Ctrl Pts',(17.2331526103506,69.1547120942527,12.));
#103534=CARTESIAN_POINT('Ctrl Pts',(17.2348417258015,69.1322311991752,12.));
#103535=CARTESIAN_POINT('Ctrl Pts',(17.2365047738125,69.1097944163245,12.));
#103536=CARTESIAN_POINT('Ctrl Pts',(17.2381418135491,69.0874018904599,12.));
#103537=CARTESIAN_POINT('Ctrl Pts',(17.2397529045589,69.065053766986,12.));
#103538=CARTESIAN_POINT('Ctrl Pts',(17.2413381067723,69.0427501919636,12.));
#103539=CARTESIAN_POINT('Ctrl Pts',(17.2428974805044,69.0204913121225,12.));
#103540=CARTESIAN_POINT('Ctrl Pts',(17.2444310864585,68.9982772748694,12.));
#103541=CARTESIAN_POINT('Ctrl Pts',(17.2459389857327,68.9761082282922,12.));
#103542=CARTESIAN_POINT('Ctrl Pts',(17.2474212398275,68.9539843211619,12.));
#103543=CARTESIAN_POINT('Ctrl Pts',(17.248877910643,68.9319057029409,12.));
#103544=CARTESIAN_POINT('Ctrl Pts',(17.2503090604792,68.909872523787,12.));
#103545=CARTESIAN_POINT('Ctrl Pts',(17.2517147520376,68.8878849345557,12.));
#103546=CARTESIAN_POINT('Ctrl Pts',(17.2530950484258,68.8659430867972,12.));
#103547=CARTESIAN_POINT('Ctrl Pts',(17.2544500131624,68.844047132755,12.));
#103548=CARTESIAN_POINT('Ctrl Pts',(17.2557797101812,68.8221972253941,12.));
#103549=CARTESIAN_POINT('Ctrl Pts',(17.2570842038383,68.8003935184184,12.));
#103550=CARTESIAN_POINT('Ctrl Pts',(17.2583635589198,68.7786361662882,12.));
#103551=CARTESIAN_POINT('Ctrl Pts',(17.259617840655,68.7569253242333,12.));
#103552=CARTESIAN_POINT('Ctrl Pts',(17.2608471147185,68.7352611482547,12.));
#103553=CARTESIAN_POINT('Ctrl Pts',(17.2620514472182,68.7136437951097,12.));
#103554=CARTESIAN_POINT('Ctrl Pts',(17.2632309046892,68.6920734222938,12.));
#103555=CARTESIAN_POINT('Ctrl Pts',(17.2643855540892,68.6705501880249,12.));
#103556=CARTESIAN_POINT('Ctrl Pts',(17.2655154627928,68.6490742512057,12.));
#103557=CARTESIAN_POINT('Ctrl Pts',(17.2666206986084,68.6276457714729,12.));
#103558=CARTESIAN_POINT('Ctrl Pts',(17.2677013298057,68.6062649092764,12.));
#103559=CARTESIAN_POINT('Ctrl Pts',(17.2687574251429,68.5849318259449,12.));
#103560=CARTESIAN_POINT('Ctrl Pts',(17.269789053896,68.5636466837517,12.));
#103561=CARTESIAN_POINT('Ctrl Pts',(17.2707962858919,68.5424096459772,12.));
#103562=CARTESIAN_POINT('Ctrl Pts',(17.2717791914544,68.521220876786,12.));
#103563=CARTESIAN_POINT('Ctrl Pts',(17.2727378413489,68.5000805410911,12.));
#103564=CARTESIAN_POINT('Ctrl Pts',(17.2736723067365,68.4789888044351,12.));
#103565=CARTESIAN_POINT('Ctrl Pts',(17.2745826591119,68.4579458328185,12.));
#103566=CARTESIAN_POINT('Ctrl Pts',(17.2754689702992,68.436951792677,12.));
#103567=CARTESIAN_POINT('Ctrl Pts',(17.2763313126018,68.4160068512753,12.));
#103568=CARTESIAN_POINT('Ctrl Pts',(17.2771697589384,68.3951111770487,12.));
#103569=CARTESIAN_POINT('Ctrl Pts',(17.2779843829608,68.3742649398964,12.));
#103570=CARTESIAN_POINT('Ctrl Pts',(17.2787752592484,68.3534683116515,12.));
#103571=CARTESIAN_POINT('Ctrl Pts',(17.2795424631799,68.3327214657575,12.));
#103572=CARTESIAN_POINT('Ctrl Pts',(17.2802860705815,68.3120245763914,12.));
#103573=CARTESIAN_POINT('Ctrl Pts',(17.2810061574353,68.2913778177261,12.));
#103574=CARTESIAN_POINT('Ctrl Pts',(17.2817027995831,68.2707813631731,12.));
#103575=CARTESIAN_POINT('Ctrl Pts',(17.2823760723874,68.2502353845071,12.));
#103576=CARTESIAN_POINT('Ctrl Pts',(17.2830260513867,68.2297400535294,12.));
#103577=CARTESIAN_POINT('Ctrl Pts',(17.2836528130819,68.2092955440567,12.));
#103578=CARTESIAN_POINT('Ctrl Pts',(17.2842564355799,68.1889020335427,12.));
#103579=CARTESIAN_POINT('Ctrl Pts',(17.2848369995293,68.1685597054232,12.));
#103580=CARTESIAN_POINT('Ctrl Pts',(17.2853945882072,68.1482687493226,12.));
#103581=CARTESIAN_POINT('Ctrl Pts',(17.2859292855705,68.1280293561511,12.));
#103582=CARTESIAN_POINT('Ctrl Pts',(17.2864411745459,68.1078417137877,12.));
#103583=CARTESIAN_POINT('Ctrl Pts',(17.2869303355432,68.0877060033205,12.));
#103584=CARTESIAN_POINT('Ctrl Pts',(17.2873968440839,68.0676223930412,12.));
#103585=CARTESIAN_POINT('Ctrl Pts',(17.2878407730961,68.0475910442424,12.));
#103586=CARTESIAN_POINT('Ctrl Pts',(17.2882621974721,68.0276121227356,12.));
#103587=CARTESIAN_POINT('Ctrl Pts',(17.28866119774,68.007685808115,12.));
#103588=CARTESIAN_POINT('Ctrl Pts',(17.2890378644866,67.987812304921,12.));
#103589=CARTESIAN_POINT('Ctrl Pts',(17.2893923013894,67.9679918502579,12.));
#103590=CARTESIAN_POINT('Ctrl Pts',(17.2897246158941,67.9482246901667,12.));
#103591=CARTESIAN_POINT('Ctrl Pts',(17.2900349103981,67.9285110571741,12.));
#103592=CARTESIAN_POINT('Ctrl Pts',(17.2903232740694,67.9088511496686,12.));
#103593=CARTESIAN_POINT('Ctrl Pts',(17.2905897723949,67.8892451049608,12.));
#103594=CARTESIAN_POINT('Ctrl Pts',(17.2908344459694,67.8696929978782,12.));
#103595=CARTESIAN_POINT('Ctrl Pts',(17.291012743109,67.8540944889687,12.));
#103596=CARTESIAN_POINT('Ctrl Pts',(17.2911366591348,67.842419897098,12.));
#103597=CARTESIAN_POINT('Ctrl Pts',(17.2912149114119,67.8346476309018,12.));
#103598=CARTESIAN_POINT('Ctrl Pts',(17.2912529479484,67.8307641965655,12.));
#103599=CARTESIAN_POINT('Ctrl Pts',(15.3208442077425,72.6050633494718,0.));
#103600=CARTESIAN_POINT('Ctrl Pts',(15.3208442077425,72.6050633494718,4.));
#103601=CARTESIAN_POINT('Ctrl Pts',(15.3208442077425,72.6050633494718,8.));
#103602=CARTESIAN_POINT('Ctrl Pts',(15.3208442077425,72.6050633494718,12.));
#103603=CARTESIAN_POINT('Ctrl Pts',(15.3856835210424,72.6937764817672,0.));
#103604=CARTESIAN_POINT('Ctrl Pts',(15.3856835210424,72.6937764817672,4.));
#103605=CARTESIAN_POINT('Ctrl Pts',(15.3856835210424,72.6937764817672,8.00000000000001));
#103606=CARTESIAN_POINT('Ctrl Pts',(15.3856835210424,72.6937764817672,12.));
#103607=CARTESIAN_POINT('Ctrl Pts',(15.551931775029,72.8096834307709,0.));
#103608=CARTESIAN_POINT('Ctrl Pts',(15.551931775029,72.8096834307709,4.));
#103609=CARTESIAN_POINT('Ctrl Pts',(15.551931775029,72.809683430771,7.99999999999999));
#103610=CARTESIAN_POINT('Ctrl Pts',(15.551931775029,72.809683430771,12.));
#103611=CARTESIAN_POINT('Ctrl Pts',(15.7502340068144,72.8161171750014,0.));
#103612=CARTESIAN_POINT('Ctrl Pts',(15.7502340068144,72.8161171750014,4.));
#103613=CARTESIAN_POINT('Ctrl Pts',(15.7502340068145,72.8161171750015,8.00000000000001));
#103614=CARTESIAN_POINT('Ctrl Pts',(15.7502340068145,72.8161171750015,12.));
#103615=CARTESIAN_POINT('Ctrl Pts',(15.830763774723,72.7986051948036,0.));
#103616=CARTESIAN_POINT('Ctrl Pts',(15.830763774723,72.7986051948036,4.));
#103617=CARTESIAN_POINT('Ctrl Pts',(15.8307637747231,72.7986051948037,8.));
#103618=CARTESIAN_POINT('Ctrl Pts',(15.8307637747231,72.7986051948037,12.));
#103619=CARTESIAN_POINT('',(15.3208442077425,72.6050633494718,0.));
#103620=CARTESIAN_POINT('',(15.8307637747231,72.7986051948038,0.));
#103621=CARTESIAN_POINT('Ctrl Pts',(15.3208442077425,72.6050633494718,2.77555756156289E-16));
#103622=CARTESIAN_POINT('Ctrl Pts',(15.3856835210424,72.6937764817672,2.77555756156289E-16));
#103623=CARTESIAN_POINT('Ctrl Pts',(15.4806825233205,72.760009024055,2.77555756156289E-16));
#103624=CARTESIAN_POINT('Ctrl Pts',(15.5861481305941,72.7904952137638,2.77555756156289E-16));
#103625=CARTESIAN_POINT('Ctrl Pts',(15.6652473360493,72.8133598560455,2.77555756156289E-16));
#103626=CARTESIAN_POINT('Ctrl Pts',(15.7502340068144,72.8161171750014,2.77555756156289E-16));
#103627=CARTESIAN_POINT('Ctrl Pts',(15.830763774723,72.7986051948036,2.77555756156289E-16));
#103628=CARTESIAN_POINT('',(15.8307637747231,72.7986051948038,12.));
#103629=CARTESIAN_POINT('Ctrl Pts',(15.830763774723,72.7986051948036,0.));
#103630=CARTESIAN_POINT('Ctrl Pts',(15.830763774723,72.7986051948036,4.));
#103631=CARTESIAN_POINT('Ctrl Pts',(15.8307637747231,72.7986051948037,8.));
#103632=CARTESIAN_POINT('Ctrl Pts',(15.8307637747231,72.7986051948037,12.));
#103633=CARTESIAN_POINT('',(15.3208442077425,72.6050633494718,12.));
#103634=CARTESIAN_POINT('Ctrl Pts',(15.8307637747231,72.7986051948037,12.));
#103635=CARTESIAN_POINT('Ctrl Pts',(15.7502340068145,72.8161171750015,12.));
#103636=CARTESIAN_POINT('Ctrl Pts',(15.6652473360493,72.8133598560455,12.));
#103637=CARTESIAN_POINT('Ctrl Pts',(15.5861481305941,72.7904952137639,12.));
#103638=CARTESIAN_POINT('Ctrl Pts',(15.4806825233205,72.7600090240551,12.));
#103639=CARTESIAN_POINT('Ctrl Pts',(15.3856835210424,72.6937764817672,12.));
#103640=CARTESIAN_POINT('Ctrl Pts',(15.3208442077425,72.6050633494718,12.));
#103641=CARTESIAN_POINT('Ctrl Pts',(15.3208442077425,72.6050633494718,12.));
#103642=CARTESIAN_POINT('Ctrl Pts',(15.3208442077425,72.6050633494718,8.));
#103643=CARTESIAN_POINT('Ctrl Pts',(15.3208442077425,72.6050633494718,4.));
#103644=CARTESIAN_POINT('Ctrl Pts',(15.3208442077425,72.6050633494718,0.));
#103645=CARTESIAN_POINT('Origin',(8.10341340518591E-11,3.65979954444617E-10,
0.));
#103646=CARTESIAN_POINT('Origin',(8.10341340518591E-11,3.65979954444617E-10,
12.));
#103647=CARTESIAN_POINT('Origin',(8.10341340518591E-11,3.65979954444617E-10,
0.));
#103648=CARTESIAN_POINT('Ctrl Pts',(22.6894590071785,70.9608233461364,0.));
#103649=CARTESIAN_POINT('Ctrl Pts',(22.6894590071785,70.9608233461364,4.));
#103650=CARTESIAN_POINT('Ctrl Pts',(22.6894590071785,70.9608233461363,8.));
#103651=CARTESIAN_POINT('Ctrl Pts',(22.6894590071785,70.9608233461363,12.));
#103652=CARTESIAN_POINT('Ctrl Pts',(22.7941214270115,70.9273579271571,0.));
#103653=CARTESIAN_POINT('Ctrl Pts',(22.7941214270115,70.9273579271571,4.));
#103654=CARTESIAN_POINT('Ctrl Pts',(22.7941214270115,70.9273579271571,8.));
#103655=CARTESIAN_POINT('Ctrl Pts',(22.7941214270115,70.9273579271571,12.));
#103656=CARTESIAN_POINT('Ctrl Pts',(22.9566438338676,70.8062825417801,0.));
#103657=CARTESIAN_POINT('Ctrl Pts',(22.9566438338676,70.8062825417801,4.00000000000001));
#103658=CARTESIAN_POINT('Ctrl Pts',(22.9566438338677,70.8062825417801,7.99999999999999));
#103659=CARTESIAN_POINT('Ctrl Pts',(22.9566438338677,70.8062825417801,12.));
#103660=CARTESIAN_POINT('Ctrl Pts',(23.0254444386656,70.620187020006,0.));
#103661=CARTESIAN_POINT('Ctrl Pts',(23.0254444386656,70.620187020006,4.));
#103662=CARTESIAN_POINT('Ctrl Pts',(23.0254444386657,70.620187020006,8.00000000000001));
#103663=CARTESIAN_POINT('Ctrl Pts',(23.0254444386657,70.620187020006,12.));
#103664=CARTESIAN_POINT('Ctrl Pts',(23.0342913834094,70.5382514078485,0.));
#103665=CARTESIAN_POINT('Ctrl Pts',(23.0342913834094,70.5382514078485,4.));
#103666=CARTESIAN_POINT('Ctrl Pts',(23.0342913834094,70.5382514078485,8.));
#103667=CARTESIAN_POINT('Ctrl Pts',(23.0342913834094,70.5382514078485,12.));
#103668=CARTESIAN_POINT('',(22.6894590071785,70.9608233461364,0.));
#103669=CARTESIAN_POINT('',(23.0342913834093,70.5382514078485,0.));
#103670=CARTESIAN_POINT('Ctrl Pts',(22.6894590071785,70.9608233461364,0.));
#103671=CARTESIAN_POINT('Ctrl Pts',(22.7941214270115,70.9273579271571,0.));
#103672=CARTESIAN_POINT('Ctrl Pts',(22.8869913737864,70.858171992656,0.));
#103673=CARTESIAN_POINT('Ctrl Pts',(22.9492582831546,70.7677549932088,0.));
#103674=CARTESIAN_POINT('Ctrl Pts',(22.9959584651808,70.6999422436235,0.));
#103675=CARTESIAN_POINT('Ctrl Pts',(23.0254444386656,70.620187020006,0.));
#103676=CARTESIAN_POINT('Ctrl Pts',(23.0342913834094,70.5382514078485,0.));
#103677=CARTESIAN_POINT('',(23.0342913834094,70.5382514078485,12.));
#103678=CARTESIAN_POINT('Ctrl Pts',(23.0342913834094,70.5382514078485,0.));
#103679=CARTESIAN_POINT('Ctrl Pts',(23.0342913834094,70.5382514078485,4.));
#103680=CARTESIAN_POINT('Ctrl Pts',(23.0342913834094,70.5382514078485,8.));
#103681=CARTESIAN_POINT('Ctrl Pts',(23.0342913834094,70.5382514078485,12.));
#103682=CARTESIAN_POINT('',(22.6894590071785,70.9608233461363,12.));
#103683=CARTESIAN_POINT('Ctrl Pts',(23.0342913834094,70.5382514078485,12.));
#103684=CARTESIAN_POINT('Ctrl Pts',(23.0254444386657,70.620187020006,12.));
#103685=CARTESIAN_POINT('Ctrl Pts',(22.9959584651808,70.6999422436235,12.));
#103686=CARTESIAN_POINT('Ctrl Pts',(22.9492582831546,70.7677549932088,12.));
#103687=CARTESIAN_POINT('Ctrl Pts',(22.8869913737864,70.8581719926559,12.));
#103688=CARTESIAN_POINT('Ctrl Pts',(22.7941214270115,70.9273579271571,12.));
#103689=CARTESIAN_POINT('Ctrl Pts',(22.6894590071785,70.9608233461363,12.));
#103690=CARTESIAN_POINT('Ctrl Pts',(22.6894590071785,70.9608233461363,12.));
#103691=CARTESIAN_POINT('Ctrl Pts',(22.6894590071785,70.9608233461363,8.));
#103692=CARTESIAN_POINT('Ctrl Pts',(22.6894590071785,70.9608233461364,4.));
#103693=CARTESIAN_POINT('Ctrl Pts',(22.6894590071785,70.9608233461364,0.));
#103694=CARTESIAN_POINT('Ctrl Pts',(23.1372951448024,66.0656156664138,0.));
#103695=CARTESIAN_POINT('Ctrl Pts',(23.1372951448024,66.0656156664138,12.));
#103696=CARTESIAN_POINT('Ctrl Pts',(23.1375957166104,66.0694876382127,0.));
#103697=CARTESIAN_POINT('Ctrl Pts',(23.1375957166104,66.0694876382127,12.));
#103698=CARTESIAN_POINT('Ctrl Pts',(23.1381951597399,66.0772371487248,0.));
#103699=CARTESIAN_POINT('Ctrl Pts',(23.1381951597399,66.0772371487248,12.));
#103700=CARTESIAN_POINT('Ctrl Pts',(23.1390892229778,66.0888781152421,0.));
#103701=CARTESIAN_POINT('Ctrl Pts',(23.1390892229778,66.0888781152421,12.));
#103702=CARTESIAN_POINT('Ctrl Pts',(23.1402711039425,66.1044328067355,0.));
#103703=CARTESIAN_POINT('Ctrl Pts',(23.1402711039425,66.1044328067355,12.));
#103704=CARTESIAN_POINT('Ctrl Pts',(23.1417314398398,66.1239318368548,0.));
#103705=CARTESIAN_POINT('Ctrl Pts',(23.1417314398398,66.1239318368548,12.));
#103706=CARTESIAN_POINT('Ctrl Pts',(23.1431747350098,66.1434865015027,0.));
#103707=CARTESIAN_POINT('Ctrl Pts',(23.1431747350098,66.1434865015027,12.));
#103708=CARTESIAN_POINT('Ctrl Pts',(23.1446009424903,66.1630967296747,0.));
#103709=CARTESIAN_POINT('Ctrl Pts',(23.1446009424903,66.1630967296747,12.));
#103710=CARTESIAN_POINT('Ctrl Pts',(23.1460099850763,66.18276239029,0.));
#103711=CARTESIAN_POINT('Ctrl Pts',(23.1460099850763,66.18276239029,12.));
#103712=CARTESIAN_POINT('Ctrl Pts',(23.1474017566484,66.2024832934866,0.));
#103713=CARTESIAN_POINT('Ctrl Pts',(23.1474017566484,66.2024832934866,12.));
#103714=CARTESIAN_POINT('Ctrl Pts',(23.1487761349328,66.2222592165473,0.));
#103715=CARTESIAN_POINT('Ctrl Pts',(23.1487761349328,66.2222592165473,12.));
#103716=CARTESIAN_POINT('Ctrl Pts',(23.1501329914487,66.2420899237317,0.));
#103717=CARTESIAN_POINT('Ctrl Pts',(23.1501329914487,66.2420899237317,12.));
#103718=CARTESIAN_POINT('Ctrl Pts',(23.1514722022483,66.2619751878741,0.));
#103719=CARTESIAN_POINT('Ctrl Pts',(23.1514722022483,66.2619751878741,12.));
#103720=CARTESIAN_POINT('Ctrl Pts',(23.1527936592625,66.2819148131072,0.));
#103721=CARTESIAN_POINT('Ctrl Pts',(23.1527936592625,66.2819148131072,12.));
#103722=CARTESIAN_POINT('Ctrl Pts',(23.154097266617,66.301908627539,0.));
#103723=CARTESIAN_POINT('Ctrl Pts',(23.154097266617,66.301908627539,12.));
#103724=CARTESIAN_POINT('Ctrl Pts',(23.1553829352531,66.3219564725161,0.));
#103725=CARTESIAN_POINT('Ctrl Pts',(23.1553829352531,66.3219564725161,12.));
#103726=CARTESIAN_POINT('Ctrl Pts',(23.1566505784626,66.3420581937159,0.));
#103727=CARTESIAN_POINT('Ctrl Pts',(23.1566505784626,66.3420581937159,12.));
#103728=CARTESIAN_POINT('Ctrl Pts',(23.1579001063438,66.3622136300692,0.));
#103729=CARTESIAN_POINT('Ctrl Pts',(23.1579001063438,66.3622136300692,12.));
#103730=CARTESIAN_POINT('Ctrl Pts',(23.15913142301,66.382422608185,0.));
#103731=CARTESIAN_POINT('Ctrl Pts',(23.15913142301,66.382422608185,12.));
#103732=CARTESIAN_POINT('Ctrl Pts',(23.1603444294754,66.402684948127,0.));
#103733=CARTESIAN_POINT('Ctrl Pts',(23.1603444294754,66.402684948127,12.));
#103734=CARTESIAN_POINT('Ctrl Pts',(23.1615390254635,66.4230004670288,0.));
#103735=CARTESIAN_POINT('Ctrl Pts',(23.1615390254635,66.4230004670288,12.));
#103736=CARTESIAN_POINT('Ctrl Pts',(23.1627151114875,66.4433689832454,0.));
#103737=CARTESIAN_POINT('Ctrl Pts',(23.1627151114875,66.4433689832454,12.));
#103738=CARTESIAN_POINT('Ctrl Pts',(23.163872591218,66.4637903210682,0.));
#103739=CARTESIAN_POINT('Ctrl Pts',(23.163872591218,66.4637903210682,12.));
#103740=CARTESIAN_POINT('Ctrl Pts',(23.1650113713792,66.4842643105263,0.));
#103741=CARTESIAN_POINT('Ctrl Pts',(23.1650113713792,66.4842643105263,12.));
#103742=CARTESIAN_POINT('Ctrl Pts',(23.1661313606123,66.5047907851319,0.));
#103743=CARTESIAN_POINT('Ctrl Pts',(23.1661313606123,66.5047907851319,12.));
#103744=CARTESIAN_POINT('Ctrl Pts',(23.1672324686927,66.5253695803209,0.));
#103745=CARTESIAN_POINT('Ctrl Pts',(23.1672324686927,66.5253695803209,12.));
#103746=CARTESIAN_POINT('Ctrl Pts',(23.1683146055736,66.5460005315406,0.));
#103747=CARTESIAN_POINT('Ctrl Pts',(23.1683146055736,66.5460005315406,12.));
#103748=CARTESIAN_POINT('Ctrl Pts',(23.169377680588,66.5666834726495,0.));
#103749=CARTESIAN_POINT('Ctrl Pts',(23.169377680588,66.5666834726495,12.));
#103750=CARTESIAN_POINT('Ctrl Pts',(23.1704216028626,66.5874182367597,0.));
#103751=CARTESIAN_POINT('Ctrl Pts',(23.1704216028626,66.5874182367597,12.));
#103752=CARTESIAN_POINT('Ctrl Pts',(23.1714462816794,66.6082046569657,0.));
#103753=CARTESIAN_POINT('Ctrl Pts',(23.1714462816794,66.6082046569657,12.));
#103754=CARTESIAN_POINT('Ctrl Pts',(23.1724516268299,66.6290425670538,0.));
#103755=CARTESIAN_POINT('Ctrl Pts',(23.1724516268299,66.6290425670538,12.));
#103756=CARTESIAN_POINT('Ctrl Pts',(23.1734375490421,66.6499318023445,0.));
#103757=CARTESIAN_POINT('Ctrl Pts',(23.1734375490421,66.6499318023445,12.));
#103758=CARTESIAN_POINT('Ctrl Pts',(23.174403960137,66.6708722000046,0.));
#103759=CARTESIAN_POINT('Ctrl Pts',(23.174403960137,66.6708722000046,12.));
#103760=CARTESIAN_POINT('Ctrl Pts',(23.1753507727931,66.691863598595,0.));
#103761=CARTESIAN_POINT('Ctrl Pts',(23.1753507727931,66.691863598595,12.));
#103762=CARTESIAN_POINT('Ctrl Pts',(23.1762779004043,66.712905837789,0.));
#103763=CARTESIAN_POINT('Ctrl Pts',(23.1762779004043,66.712905837789,12.));
#103764=CARTESIAN_POINT('Ctrl Pts',(23.1771852569136,66.7339987580441,0.));
#103765=CARTESIAN_POINT('Ctrl Pts',(23.1771852569136,66.7339987580441,12.));
#103766=CARTESIAN_POINT('Ctrl Pts',(23.1780727566309,66.7551422002229,0.));
#103767=CARTESIAN_POINT('Ctrl Pts',(23.1780727566309,66.7551422002229,12.));
#103768=CARTESIAN_POINT('Ctrl Pts',(23.1789403142375,66.7763360056146,0.));
#103769=CARTESIAN_POINT('Ctrl Pts',(23.1789403142375,66.7763360056146,12.));
#103770=CARTESIAN_POINT('Ctrl Pts',(23.1797878448645,66.7975800161014,0.));
#103771=CARTESIAN_POINT('Ctrl Pts',(23.1797878448645,66.7975800161014,12.));
#103772=CARTESIAN_POINT('Ctrl Pts',(23.1806152641475,66.8188740742727,0.));
#103773=CARTESIAN_POINT('Ctrl Pts',(23.1806152641475,66.8188740742727,12.));
#103774=CARTESIAN_POINT('Ctrl Pts',(23.1814224882948,66.840218023555,0.));
#103775=CARTESIAN_POINT('Ctrl Pts',(23.1814224882948,66.840218023555,12.));
#103776=CARTESIAN_POINT('Ctrl Pts',(23.1822094341508,66.8616117083304,0.));
#103777=CARTESIAN_POINT('Ctrl Pts',(23.1822094341508,66.8616117083304,12.));
#103778=CARTESIAN_POINT('Ctrl Pts',(23.1829760191582,66.8830549738768,0.));
#103779=CARTESIAN_POINT('Ctrl Pts',(23.1829760191582,66.8830549738768,12.));
#103780=CARTESIAN_POINT('Ctrl Pts',(23.1837221613231,66.904547666305,0.));
#103781=CARTESIAN_POINT('Ctrl Pts',(23.1837221613231,66.904547666305,12.));
#103782=CARTESIAN_POINT('Ctrl Pts',(23.1844477791816,66.9260896324955,0.));
#103783=CARTESIAN_POINT('Ctrl Pts',(23.1844477791816,66.9260896324955,12.));
#103784=CARTESIAN_POINT('Ctrl Pts',(23.1851527917665,66.9476807200225,0.));
#103785=CARTESIAN_POINT('Ctrl Pts',(23.1851527917665,66.9476807200225,12.));
#103786=CARTESIAN_POINT('Ctrl Pts',(23.1858371185852,66.9693207771059,0.));
#103787=CARTESIAN_POINT('Ctrl Pts',(23.1858371185852,66.9693207771059,12.));
#103788=CARTESIAN_POINT('Ctrl Pts',(23.1865006796291,66.9910096526483,0.));
#103789=CARTESIAN_POINT('Ctrl Pts',(23.1865006796291,66.9910096526483,12.));
#103790=CARTESIAN_POINT('Ctrl Pts',(23.1871433953795,67.0127471962507,0.));
#103791=CARTESIAN_POINT('Ctrl Pts',(23.1871433953795,67.0127471962507,12.));
#103792=CARTESIAN_POINT('Ctrl Pts',(23.1877651868155,67.0345332582297,0.));
#103793=CARTESIAN_POINT('Ctrl Pts',(23.1877651868155,67.0345332582297,12.));
#103794=CARTESIAN_POINT('Ctrl Pts',(23.1883659754267,67.0563676896312,0.));
#103795=CARTESIAN_POINT('Ctrl Pts',(23.1883659754267,67.0563676896312,12.));
#103796=CARTESIAN_POINT('Ctrl Pts',(23.1889456832115,67.0782503422293,0.));
#103797=CARTESIAN_POINT('Ctrl Pts',(23.1889456832115,67.0782503422293,12.));
#103798=CARTESIAN_POINT('Ctrl Pts',(23.1895042326625,67.1001810685138,0.));
#103799=CARTESIAN_POINT('Ctrl Pts',(23.1895042326625,67.1001810685138,12.));
#103800=CARTESIAN_POINT('Ctrl Pts',(23.1900415467574,67.122159721674,0.));
#103801=CARTESIAN_POINT('Ctrl Pts',(23.1900415467574,67.122159721674,12.));
#103802=CARTESIAN_POINT('Ctrl Pts',(23.1905575489505,67.1441861555819,0.));
#103803=CARTESIAN_POINT('Ctrl Pts',(23.1905575489505,67.1441861555819,12.));
#103804=CARTESIAN_POINT('Ctrl Pts',(23.1910521631658,67.1662602247641,0.));
#103805=CARTESIAN_POINT('Ctrl Pts',(23.1910521631658,67.1662602247641,12.));
#103806=CARTESIAN_POINT('Ctrl Pts',(23.1915253137923,67.1883817844039,0.));
#103807=CARTESIAN_POINT('Ctrl Pts',(23.1915253137923,67.1883817844039,12.));
#103808=CARTESIAN_POINT('Ctrl Pts',(23.1919769256803,67.2105506903448,0.));
#103809=CARTESIAN_POINT('Ctrl Pts',(23.1919769256803,67.2105506903448,12.));
#103810=CARTESIAN_POINT('Ctrl Pts',(23.1924069241385,67.232766799088,0.));
#103811=CARTESIAN_POINT('Ctrl Pts',(23.1924069241385,67.232766799088,12.));
#103812=CARTESIAN_POINT('Ctrl Pts',(23.1928152349343,67.2550299677888,0.));
#103813=CARTESIAN_POINT('Ctrl Pts',(23.1928152349343,67.2550299677888,12.));
#103814=CARTESIAN_POINT('Ctrl Pts',(23.1932017842954,67.2773400542477,0.));
#103815=CARTESIAN_POINT('Ctrl Pts',(23.1932017842954,67.2773400542477,12.));
#103816=CARTESIAN_POINT('Ctrl Pts',(23.193566498902,67.2996969169099,0.));
#103817=CARTESIAN_POINT('Ctrl Pts',(23.193566498902,67.2996969169099,12.));
#103818=CARTESIAN_POINT('Ctrl Pts',(23.1939093058802,67.3221004148604,0.));
#103819=CARTESIAN_POINT('Ctrl Pts',(23.1939093058802,67.3221004148604,12.));
#103820=CARTESIAN_POINT('Ctrl Pts',(23.1942301327978,67.3445504078178,0.));
#103821=CARTESIAN_POINT('Ctrl Pts',(23.1942301327978,67.3445504078178,12.));
#103822=CARTESIAN_POINT('Ctrl Pts',(23.1945289076608,67.3670467561205,0.));
#103823=CARTESIAN_POINT('Ctrl Pts',(23.1945289076608,67.3670467561205,12.));
#103824=CARTESIAN_POINT('Ctrl Pts',(23.1948055589123,67.3895893207168,0.));
#103825=CARTESIAN_POINT('Ctrl Pts',(23.1948055589123,67.3895893207168,12.));
#103826=CARTESIAN_POINT('Ctrl Pts',(23.1950600154259,67.4121779631666,0.));
#103827=CARTESIAN_POINT('Ctrl Pts',(23.1950600154259,67.4121779631666,12.));
#103828=CARTESIAN_POINT('Ctrl Pts',(23.1952922065009,67.4348125456389,0.));
#103829=CARTESIAN_POINT('Ctrl Pts',(23.1952922065009,67.4348125456389,12.));
#103830=CARTESIAN_POINT('Ctrl Pts',(23.1955020618591,67.4574929309079,0.));
#103831=CARTESIAN_POINT('Ctrl Pts',(23.1955020618591,67.4574929309079,12.));
#103832=CARTESIAN_POINT('Ctrl Pts',(23.1956895116446,67.4802189823424,0.));
#103833=CARTESIAN_POINT('Ctrl Pts',(23.1956895116446,67.4802189823424,12.));
#103834=CARTESIAN_POINT('Ctrl Pts',(23.1958544864224,67.5029905638974,0.));
#103835=CARTESIAN_POINT('Ctrl Pts',(23.1958544864224,67.5029905638974,12.));
#103836=CARTESIAN_POINT('Ctrl Pts',(23.1959969171709,67.525807540117,0.));
#103837=CARTESIAN_POINT('Ctrl Pts',(23.1959969171709,67.525807540117,12.));
#103838=CARTESIAN_POINT('Ctrl Pts',(23.1961167352776,67.5486697761301,0.));
#103839=CARTESIAN_POINT('Ctrl Pts',(23.1961167352776,67.5486697761301,12.));
#103840=CARTESIAN_POINT('Ctrl Pts',(23.1962138725358,67.5715771376454,0.));
#103841=CARTESIAN_POINT('Ctrl Pts',(23.1962138725358,67.5715771376454,12.));
#103842=CARTESIAN_POINT('Ctrl Pts',(23.1962882611443,67.5945294909398,0.));
#103843=CARTESIAN_POINT('Ctrl Pts',(23.1962882611443,67.5945294909398,12.));
#103844=CARTESIAN_POINT('Ctrl Pts',(23.1963398337055,67.6175267028517,0.));
#103845=CARTESIAN_POINT('Ctrl Pts',(23.1963398337055,67.6175267028517,12.));
#103846=CARTESIAN_POINT('Ctrl Pts',(23.1963685232176,67.6405686407828,0.));
#103847=CARTESIAN_POINT('Ctrl Pts',(23.1963685232176,67.6405686407828,12.));
#103848=CARTESIAN_POINT('Ctrl Pts',(23.1963742630709,67.6636551726948,0.));
#103849=CARTESIAN_POINT('Ctrl Pts',(23.1963742630709,67.6636551726948,12.));
#103850=CARTESIAN_POINT('Ctrl Pts',(23.1963569870456,67.6867861671045,0.));
#103851=CARTESIAN_POINT('Ctrl Pts',(23.1963569870456,67.6867861671045,12.));
#103852=CARTESIAN_POINT('Ctrl Pts',(23.1963166293116,67.7099614930712,0.));
#103853=CARTESIAN_POINT('Ctrl Pts',(23.1963166293116,67.7099614930712,12.));
#103854=CARTESIAN_POINT('Ctrl Pts',(23.1962531244261,67.7331810201931,0.));
#103855=CARTESIAN_POINT('Ctrl Pts',(23.1962531244261,67.7331810201931,12.));
#103856=CARTESIAN_POINT('Ctrl Pts',(23.1961664073273,67.7564446186115,0.));
#103857=CARTESIAN_POINT('Ctrl Pts',(23.1961664073273,67.7564446186115,12.));
#103858=CARTESIAN_POINT('Ctrl Pts',(23.1960564133308,67.7797521590056,0.));
#103859=CARTESIAN_POINT('Ctrl Pts',(23.1960564133308,67.7797521590056,12.));
#103860=CARTESIAN_POINT('Ctrl Pts',(23.1959230781265,67.8031035125873,0.));
#103861=CARTESIAN_POINT('Ctrl Pts',(23.1959230781265,67.8031035125873,12.));
#103862=CARTESIAN_POINT('Ctrl Pts',(23.1957663377797,67.8264985510884,0.));
#103863=CARTESIAN_POINT('Ctrl Pts',(23.1957663377797,67.8264985510884,12.));
#103864=CARTESIAN_POINT('Ctrl Pts',(23.1955861287275,67.8499371467578,0.));
#103865=CARTESIAN_POINT('Ctrl Pts',(23.1955861287275,67.8499371467578,12.));
#103866=CARTESIAN_POINT('Ctrl Pts',(23.1953823877726,67.8734191723639,0.));
#103867=CARTESIAN_POINT('Ctrl Pts',(23.1953823877726,67.8734191723639,12.));
#103868=CARTESIAN_POINT('Ctrl Pts',(23.19515505208,67.8969445011908,0.));
#103869=CARTESIAN_POINT('Ctrl Pts',(23.19515505208,67.8969445011908,12.));
#103870=CARTESIAN_POINT('Ctrl Pts',(23.1949040591748,67.9205130070337,0.));
#103871=CARTESIAN_POINT('Ctrl Pts',(23.1949040591748,67.9205130070337,12.));
#103872=CARTESIAN_POINT('Ctrl Pts',(23.1946293469436,67.9441245641871,0.));
#103873=CARTESIAN_POINT('Ctrl Pts',(23.1946293469436,67.9441245641871,12.));
#103874=CARTESIAN_POINT('Ctrl Pts',(23.1943308536307,67.9677790474414,0.));
#103875=CARTESIAN_POINT('Ctrl Pts',(23.1943308536307,67.9677790474414,12.));
#103876=CARTESIAN_POINT('Ctrl Pts',(23.1940085178319,67.9914763320878,0.));
#103877=CARTESIAN_POINT('Ctrl Pts',(23.1940085178319,67.9914763320878,12.));
#103878=CARTESIAN_POINT('Ctrl Pts',(23.193662278492,68.0152162939123,0.));
#103879=CARTESIAN_POINT('Ctrl Pts',(23.193662278492,68.0152162939123,12.));
#103880=CARTESIAN_POINT('Ctrl Pts',(23.1932920749021,68.0389988091926,0.));
#103881=CARTESIAN_POINT('Ctrl Pts',(23.1932920749021,68.0389988091926,12.));
#103882=CARTESIAN_POINT('Ctrl Pts',(23.1928978467017,68.0628237546853,0.));
#103883=CARTESIAN_POINT('Ctrl Pts',(23.1928978467017,68.0628237546853,12.));
#103884=CARTESIAN_POINT('Ctrl Pts',(23.1924795338745,68.086691007624,0.));
#103885=CARTESIAN_POINT('Ctrl Pts',(23.1924795338745,68.086691007624,12.));
#103886=CARTESIAN_POINT('Ctrl Pts',(23.1920370767423,68.1106004457223,0.));
#103887=CARTESIAN_POINT('Ctrl Pts',(23.1920370767423,68.1106004457223,12.));
#103888=CARTESIAN_POINT('Ctrl Pts',(23.1915704159623,68.1345519471695,0.));
#103889=CARTESIAN_POINT('Ctrl Pts',(23.1915704159623,68.1345519471695,12.));
#103890=CARTESIAN_POINT('Ctrl Pts',(23.1910794925252,68.1585453906259,0.));
#103891=CARTESIAN_POINT('Ctrl Pts',(23.1910794925252,68.1585453906259,12.));
#103892=CARTESIAN_POINT('Ctrl Pts',(23.1905642477571,68.182580655213,0.));
#103893=CARTESIAN_POINT('Ctrl Pts',(23.1905642477571,68.182580655213,12.));
#103894=CARTESIAN_POINT('Ctrl Pts',(23.1900246233164,68.2066576205113,0.));
#103895=CARTESIAN_POINT('Ctrl Pts',(23.1900246233164,68.2066576205113,12.));
#103896=CARTESIAN_POINT('Ctrl Pts',(23.1894605611869,68.2307761665629,0.));
#103897=CARTESIAN_POINT('Ctrl Pts',(23.1894605611869,68.2307761665629,12.));
#103898=CARTESIAN_POINT('Ctrl Pts',(23.1888720036756,68.2549361738679,0.));
#103899=CARTESIAN_POINT('Ctrl Pts',(23.1888720036756,68.2549361738679,12.));
#103900=CARTESIAN_POINT('Ctrl Pts',(23.1882588934108,68.2791375233798,0.));
#103901=CARTESIAN_POINT('Ctrl Pts',(23.1882588934108,68.2791375233798,12.));
#103902=CARTESIAN_POINT('Ctrl Pts',(23.1876211733439,68.3033800964946,0.));
#103903=CARTESIAN_POINT('Ctrl Pts',(23.1876211733439,68.3033800964946,12.));
#103904=CARTESIAN_POINT('Ctrl Pts',(23.1869587867463,68.3276637750494,0.));
#103905=CARTESIAN_POINT('Ctrl Pts',(23.1869587867463,68.3276637750494,12.));
#103906=CARTESIAN_POINT('Ctrl Pts',(23.1862716772034,68.3519884413253,0.));
#103907=CARTESIAN_POINT('Ctrl Pts',(23.1862716772034,68.3519884413253,12.));
#103908=CARTESIAN_POINT('Ctrl Pts',(23.1855597886117,68.3763539780442,0.));
#103909=CARTESIAN_POINT('Ctrl Pts',(23.1855597886117,68.3763539780442,12.));
#103910=CARTESIAN_POINT('Ctrl Pts',(23.1848230651775,68.4007602683649,0.));
#103911=CARTESIAN_POINT('Ctrl Pts',(23.1848230651775,68.4007602683649,12.));
#103912=CARTESIAN_POINT('Ctrl Pts',(23.184061451419,68.4252071958725,0.));
#103913=CARTESIAN_POINT('Ctrl Pts',(23.184061451419,68.4252071958725,12.));
#103914=CARTESIAN_POINT('Ctrl Pts',(23.1832748921629,68.4496946445756,0.));
#103915=CARTESIAN_POINT('Ctrl Pts',(23.1832748921629,68.4496946445756,12.));
#103916=CARTESIAN_POINT('Ctrl Pts',(23.1824633325384,68.4742224989099,0.));
#103917=CARTESIAN_POINT('Ctrl Pts',(23.1824633325384,68.4742224989099,12.));
#103918=CARTESIAN_POINT('Ctrl Pts',(23.1816267179751,68.4987906437357,0.));
#103919=CARTESIAN_POINT('Ctrl Pts',(23.1816267179751,68.4987906437357,12.));
#103920=CARTESIAN_POINT('Ctrl Pts',(23.180764994201,68.5233989643344,0.));
#103921=CARTESIAN_POINT('Ctrl Pts',(23.180764994201,68.5233989643344,12.));
#103922=CARTESIAN_POINT('Ctrl Pts',(23.1798781072449,68.548047346398,0.));
#103923=CARTESIAN_POINT('Ctrl Pts',(23.1798781072449,68.548047346398,12.));
#103924=CARTESIAN_POINT('Ctrl Pts',(23.1789660034339,68.572735676027,0.));
#103925=CARTESIAN_POINT('Ctrl Pts',(23.1789660034339,68.572735676027,12.));
#103926=CARTESIAN_POINT('Ctrl Pts',(23.1780286293873,68.5974638397322,0.));
#103927=CARTESIAN_POINT('Ctrl Pts',(23.1780286293873,68.5974638397322,12.));
#103928=CARTESIAN_POINT('Ctrl Pts',(23.1770659320136,68.6222317244337,0.));
#103929=CARTESIAN_POINT('Ctrl Pts',(23.1770659320136,68.6222317244337,12.));
#103930=CARTESIAN_POINT('Ctrl Pts',(23.1760778585093,68.6470392174567,0.));
#103931=CARTESIAN_POINT('Ctrl Pts',(23.1760778585093,68.6470392174567,12.));
#103932=CARTESIAN_POINT('Ctrl Pts',(23.1750643563605,68.6718862065227,0.));
#103933=CARTESIAN_POINT('Ctrl Pts',(23.1750643563605,68.6718862065227,12.));
#103934=CARTESIAN_POINT('Ctrl Pts',(23.1740253733423,68.6967725797458,0.));
#103935=CARTESIAN_POINT('Ctrl Pts',(23.1740253733423,68.6967725797458,12.));
#103936=CARTESIAN_POINT('Ctrl Pts',(23.1729608575115,68.7216982256357,0.));
#103937=CARTESIAN_POINT('Ctrl Pts',(23.1729608575115,68.7216982256357,12.));
#103938=CARTESIAN_POINT('Ctrl Pts',(23.1718707572046,68.7466630330968,0.));
#103939=CARTESIAN_POINT('Ctrl Pts',(23.1718707572046,68.7466630330968,12.));
#103940=CARTESIAN_POINT('Ctrl Pts',(23.1707550210359,68.7716668914246,0.));
#103941=CARTESIAN_POINT('Ctrl Pts',(23.1707550210359,68.7716668914246,12.));
#103942=CARTESIAN_POINT('Ctrl Pts',(23.1696135978992,68.7967096902981,0.));
#103943=CARTESIAN_POINT('Ctrl Pts',(23.1696135978992,68.7967096902981,12.));
#103944=CARTESIAN_POINT('Ctrl Pts',(23.1684464369681,68.8217913197735,0.));
#103945=CARTESIAN_POINT('Ctrl Pts',(23.1684464369681,68.8217913197735,12.));
#103946=CARTESIAN_POINT('Ctrl Pts',(23.1672534876885,68.8469116702885,0.));
#103947=CARTESIAN_POINT('Ctrl Pts',(23.1672534876885,68.8469116702885,12.));
#103948=CARTESIAN_POINT('Ctrl Pts',(23.1660346997762,68.8720706326606,0.));
#103949=CARTESIAN_POINT('Ctrl Pts',(23.1660346997762,68.8720706326606,12.));
#103950=CARTESIAN_POINT('Ctrl Pts',(23.1647900232151,68.8972680980844,0.));
#103951=CARTESIAN_POINT('Ctrl Pts',(23.1647900232151,68.8972680980844,12.));
#103952=CARTESIAN_POINT('Ctrl Pts',(23.1635194082581,68.9225039581249,0.));
#103953=CARTESIAN_POINT('Ctrl Pts',(23.1635194082581,68.9225039581249,12.));
#103954=CARTESIAN_POINT('Ctrl Pts',(23.162222805429,68.9477781047103,0.));
#103955=CARTESIAN_POINT('Ctrl Pts',(23.162222805429,68.9477781047103,12.));
#103956=CARTESIAN_POINT('Ctrl Pts',(23.1609001655153,68.9730904301363,0.));
#103957=CARTESIAN_POINT('Ctrl Pts',(23.1609001655153,68.9730904301363,12.));
#103958=CARTESIAN_POINT('Ctrl Pts',(23.1595514395654,68.9984408270653,0.));
#103959=CARTESIAN_POINT('Ctrl Pts',(23.1595514395654,68.9984408270653,12.));
#103960=CARTESIAN_POINT('Ctrl Pts',(23.1581765788869,69.0238291885245,0.));
#103961=CARTESIAN_POINT('Ctrl Pts',(23.1581765788869,69.0238291885245,12.));
#103962=CARTESIAN_POINT('Ctrl Pts',(23.1567755350472,69.0492554078999,0.));
#103963=CARTESIAN_POINT('Ctrl Pts',(23.1567755350472,69.0492554078999,12.));
#103964=CARTESIAN_POINT('Ctrl Pts',(23.1553482598767,69.0747193789292,0.));
#103965=CARTESIAN_POINT('Ctrl Pts',(23.1553482598767,69.0747193789292,12.));
#103966=CARTESIAN_POINT('Ctrl Pts',(23.1538947054619,69.1002209957037,0.));
#103967=CARTESIAN_POINT('Ctrl Pts',(23.1538947054619,69.1002209957037,12.));
#103968=CARTESIAN_POINT('Ctrl Pts',(23.1524148241413,69.1257601526693,0.));
#103969=CARTESIAN_POINT('Ctrl Pts',(23.1524148241413,69.1257601526693,12.));
#103970=CARTESIAN_POINT('Ctrl Pts',(23.1509085685032,69.1513367446231,0.));
#103971=CARTESIAN_POINT('Ctrl Pts',(23.1509085685032,69.1513367446231,12.));
#103972=CARTESIAN_POINT('Ctrl Pts',(23.1493758913857,69.176950666708,0.));
#103973=CARTESIAN_POINT('Ctrl Pts',(23.1493758913857,69.176950666708,12.));
#103974=CARTESIAN_POINT('Ctrl Pts',(23.1478167458787,69.2026018144023,0.));
#103975=CARTESIAN_POINT('Ctrl Pts',(23.1478167458787,69.2026018144023,12.));
#103976=CARTESIAN_POINT('Ctrl Pts',(23.1462310853205,69.2282900835234,0.));
#103977=CARTESIAN_POINT('Ctrl Pts',(23.1462310853205,69.2282900835234,12.));
#103978=CARTESIAN_POINT('Ctrl Pts',(23.1446188632931,69.2540153702311,0.));
#103979=CARTESIAN_POINT('Ctrl Pts',(23.1446188632931,69.2540153702311,12.));
#103980=CARTESIAN_POINT('Ctrl Pts',(23.142980033622,69.2797775710275,0.));
#103981=CARTESIAN_POINT('Ctrl Pts',(23.142980033622,69.2797775710275,12.));
#103982=CARTESIAN_POINT('Ctrl Pts',(23.1413145503762,69.3055765827544,0.));
#103983=CARTESIAN_POINT('Ctrl Pts',(23.1413145503762,69.3055765827544,12.));
#103984=CARTESIAN_POINT('Ctrl Pts',(23.1396223678725,69.3314123025863,0.));
#103985=CARTESIAN_POINT('Ctrl Pts',(23.1396223678725,69.3314123025863,12.));
#103986=CARTESIAN_POINT('Ctrl Pts',(23.1379034406717,69.3572846280289,0.));
#103987=CARTESIAN_POINT('Ctrl Pts',(23.1379034406717,69.3572846280289,12.));
#103988=CARTESIAN_POINT('Ctrl Pts',(23.1361577235708,69.3831934569176,0.));
#103989=CARTESIAN_POINT('Ctrl Pts',(23.1361577235708,69.3831934569176,12.));
#103990=CARTESIAN_POINT('Ctrl Pts',(23.1343851715988,69.4091386874129,0.));
#103991=CARTESIAN_POINT('Ctrl Pts',(23.1343851715988,69.4091386874129,12.));
#103992=CARTESIAN_POINT('Ctrl Pts',(23.1325857400145,69.4351202179948,0.));
#103993=CARTESIAN_POINT('Ctrl Pts',(23.1325857400145,69.4351202179948,12.));
#103994=CARTESIAN_POINT('Ctrl Pts',(23.1307593843063,69.4611379474492,0.));
#103995=CARTESIAN_POINT('Ctrl Pts',(23.1307593843063,69.4611379474492,12.));
#103996=CARTESIAN_POINT('Ctrl Pts',(23.1289060601927,69.4871917748665,0.));
#103997=CARTESIAN_POINT('Ctrl Pts',(23.1289060601927,69.4871917748665,12.));
#103998=CARTESIAN_POINT('Ctrl Pts',(23.1270257236207,69.5132815996548,0.));
#103999=CARTESIAN_POINT('Ctrl Pts',(23.1270257236207,69.5132815996548,12.));
#104000=CARTESIAN_POINT('Ctrl Pts',(23.1251183307678,69.5394073215467,0.));
#104001=CARTESIAN_POINT('Ctrl Pts',(23.1251183307678,69.5394073215467,12.));
#104002=CARTESIAN_POINT('Ctrl Pts',(23.1231838380452,69.565568840605,0.));
#104003=CARTESIAN_POINT('Ctrl Pts',(23.1231838380452,69.565568840605,12.));
#104004=CARTESIAN_POINT('Ctrl Pts',(23.1212222021049,69.5917660572255,0.));
#104005=CARTESIAN_POINT('Ctrl Pts',(23.1212222021049,69.5917660572255,12.));
#104006=CARTESIAN_POINT('Ctrl Pts',(23.1192333798437,69.617998872135,0.));
#104007=CARTESIAN_POINT('Ctrl Pts',(23.1192333798437,69.617998872135,12.));
#104008=CARTESIAN_POINT('Ctrl Pts',(23.1172173283855,69.6442671863751,0.));
#104009=CARTESIAN_POINT('Ctrl Pts',(23.1172173283855,69.6442671863751,12.));
#104010=CARTESIAN_POINT('Ctrl Pts',(23.1151740050678,69.6705709012842,0.));
#104011=CARTESIAN_POINT('Ctrl Pts',(23.1151740050678,69.6705709012842,12.));
#104012=CARTESIAN_POINT('Ctrl Pts',(23.1131033674301,69.6969099184766,0.));
#104013=CARTESIAN_POINT('Ctrl Pts',(23.1131033674301,69.6969099184766,12.));
#104014=CARTESIAN_POINT('Ctrl Pts',(23.1110053732049,69.7232841398207,0.));
#104015=CARTESIAN_POINT('Ctrl Pts',(23.1110053732049,69.7232841398207,12.));
#104016=CARTESIAN_POINT('Ctrl Pts',(23.1088799803093,69.7496934674083,0.));
#104017=CARTESIAN_POINT('Ctrl Pts',(23.1088799803093,69.7496934674083,12.));
#104018=CARTESIAN_POINT('Ctrl Pts',(23.1067271468614,69.7761378035979,0.));
#104019=CARTESIAN_POINT('Ctrl Pts',(23.1067271468614,69.7761378035979,12.));
#104020=CARTESIAN_POINT('Ctrl Pts',(23.1045468311994,69.8026170510582,0.));
#104021=CARTESIAN_POINT('Ctrl Pts',(23.1045468311994,69.8026170510582,12.));
#104022=CARTESIAN_POINT('Ctrl Pts',(23.1023389919052,69.8291311128121,0.));
#104023=CARTESIAN_POINT('Ctrl Pts',(23.1023389919052,69.8291311128121,12.));
#104024=CARTESIAN_POINT('Ctrl Pts',(23.100103587824,69.8556798922688,0.));
#104025=CARTESIAN_POINT('Ctrl Pts',(23.100103587824,69.8556798922688,12.));
#104026=CARTESIAN_POINT('Ctrl Pts',(23.0978405781018,69.882263293276,0.));
#104027=CARTESIAN_POINT('Ctrl Pts',(23.0978405781018,69.882263293276,12.));
#104028=CARTESIAN_POINT('Ctrl Pts',(23.0955499221555,69.9088812200704,0.));
#104029=CARTESIAN_POINT('Ctrl Pts',(23.0955499221555,69.9088812200704,12.));
#104030=CARTESIAN_POINT('Ctrl Pts',(23.0932315796066,69.9355335771722,0.));
#104031=CARTESIAN_POINT('Ctrl Pts',(23.0932315796066,69.9355335771722,12.));
#104032=CARTESIAN_POINT('Ctrl Pts',(23.090885510225,69.9622202692871,0.));
#104033=CARTESIAN_POINT('Ctrl Pts',(23.090885510225,69.9622202692871,12.));
#104034=CARTESIAN_POINT('Ctrl Pts',(23.0885116738798,69.9889412012143,0.));
#104035=CARTESIAN_POINT('Ctrl Pts',(23.0885116738798,69.9889412012143,12.));
#104036=CARTESIAN_POINT('Ctrl Pts',(23.0861100304731,70.0156962777173,0.));
#104037=CARTESIAN_POINT('Ctrl Pts',(23.0861100304731,70.0156962777173,12.));
#104038=CARTESIAN_POINT('Ctrl Pts',(23.0836805399377,70.0424854035125,0.));
#104039=CARTESIAN_POINT('Ctrl Pts',(23.0836805399377,70.0424854035125,12.));
#104040=CARTESIAN_POINT('Ctrl Pts',(23.081223162377,70.0693084835388,0.));
#104041=CARTESIAN_POINT('Ctrl Pts',(23.081223162377,70.0693084835388,12.));
#104042=CARTESIAN_POINT('Ctrl Pts',(23.0787378581778,70.096165423165,0.));
#104043=CARTESIAN_POINT('Ctrl Pts',(23.0787378581778,70.096165423165,12.));
#104044=CARTESIAN_POINT('Ctrl Pts',(23.076224588139,70.1230561284222,0.));
#104045=CARTESIAN_POINT('Ctrl Pts',(23.076224588139,70.1230561284222,12.));
#104046=CARTESIAN_POINT('Ctrl Pts',(23.0736833135934,70.1499805062159,0.));
#104047=CARTESIAN_POINT('Ctrl Pts',(23.0736833135934,70.1499805062159,12.));
#104048=CARTESIAN_POINT('Ctrl Pts',(23.0711139965432,70.176938464556,0.));
#104049=CARTESIAN_POINT('Ctrl Pts',(23.0711139965432,70.176938464556,12.));
#104050=CARTESIAN_POINT('Ctrl Pts',(23.0685165993681,70.2039299120456,0.));
#104051=CARTESIAN_POINT('Ctrl Pts',(23.0685165993681,70.2039299120456,12.));
#104052=CARTESIAN_POINT('Ctrl Pts',(23.0658910845425,70.2309547573789,0.));
#104053=CARTESIAN_POINT('Ctrl Pts',(23.0658910845425,70.2309547573789,12.));
#104054=CARTESIAN_POINT('Ctrl Pts',(23.0632374143276,70.2580129087878,0.));
#104055=CARTESIAN_POINT('Ctrl Pts',(23.0632374143276,70.2580129087878,12.));
#104056=CARTESIAN_POINT('Ctrl Pts',(23.0605555505326,70.2851042736081,0.));
#104057=CARTESIAN_POINT('Ctrl Pts',(23.0605555505326,70.2851042736081,12.));
#104058=CARTESIAN_POINT('Ctrl Pts',(23.0578454541116,70.3122287575374,0.));
#104059=CARTESIAN_POINT('Ctrl Pts',(23.0578454541116,70.3122287575374,12.));
#104060=CARTESIAN_POINT('Ctrl Pts',(23.0551070854942,70.3393862652353,0.));
#104061=CARTESIAN_POINT('Ctrl Pts',(23.0551070854942,70.3393862652353,12.));
#104062=CARTESIAN_POINT('Ctrl Pts',(23.0523404053188,70.3665767016596,0.));
#104063=CARTESIAN_POINT('Ctrl Pts',(23.0523404053188,70.3665767016596,12.));
#104064=CARTESIAN_POINT('Ctrl Pts',(23.0495453750773,70.39379997323,0.));
#104065=CARTESIAN_POINT('Ctrl Pts',(23.0495453750773,70.39379997323,12.));
#104066=CARTESIAN_POINT('Ctrl Pts',(23.0467219577288,70.421055988934,0.));
#104067=CARTESIAN_POINT('Ctrl Pts',(23.0467219577288,70.421055988934,12.));
#104068=CARTESIAN_POINT('Ctrl Pts',(23.0438701184995,70.4483446617553,0.));
#104069=CARTESIAN_POINT('Ctrl Pts',(23.0438701184995,70.4483446617553,12.));
#104070=CARTESIAN_POINT('Ctrl Pts',(23.0409898250726,70.4756659090104,0.));
#104071=CARTESIAN_POINT('Ctrl Pts',(23.0409898250726,70.4756659090104,12.));
#104072=CARTESIAN_POINT('Ctrl Pts',(23.0380810458237,70.5030196491883,0.));
#104073=CARTESIAN_POINT('Ctrl Pts',(23.0380810458237,70.5030196491883,12.));
#104074=CARTESIAN_POINT('Ctrl Pts',(23.0351437484309,70.5304057994537,0.));
#104075=CARTESIAN_POINT('Ctrl Pts',(23.0351437484309,70.5304057994537,12.));
#104076=CARTESIAN_POINT('Ctrl Pts',(23.0321778982705,70.5578242727606,0.));
#104077=CARTESIAN_POINT('Ctrl Pts',(23.0321778982705,70.5578242727606,12.));
#104078=CARTESIAN_POINT('Ctrl Pts',(23.0291834570688,70.5852749754168,0.));
#104079=CARTESIAN_POINT('Ctrl Pts',(23.0291834570688,70.5852749754168,12.));
#104080=CARTESIAN_POINT('Ctrl Pts',(23.0261603810187,70.6127578036869,0.));
#104081=CARTESIAN_POINT('Ctrl Pts',(23.0261603810187,70.6127578036869,12.));
#104082=CARTESIAN_POINT('Ctrl Pts',(23.0231086235262,70.6402726486718,0.));
#104083=CARTESIAN_POINT('Ctrl Pts',(23.0231086235262,70.6402726486718,12.));
#104084=CARTESIAN_POINT('Ctrl Pts',(23.0200281385906,70.6678194023389,0.));
#104085=CARTESIAN_POINT('Ctrl Pts',(23.0200281385906,70.6678194023389,12.));
#104086=CARTESIAN_POINT('Ctrl Pts',(23.0169188841083,70.6953979633561,0.));
#104087=CARTESIAN_POINT('Ctrl Pts',(23.0169188841083,70.6953979633561,12.));
#104088=CARTESIAN_POINT('Ctrl Pts',(23.0137808248898,70.7230082425324,0.));
#104089=CARTESIAN_POINT('Ctrl Pts',(23.0137808248898,70.7230082425324,12.));
#104090=CARTESIAN_POINT('Ctrl Pts',(23.0106139365941,70.7506501695822,0.));
#104091=CARTESIAN_POINT('Ctrl Pts',(23.0106139365941,70.7506501695822,12.));
#104092=CARTESIAN_POINT('Ctrl Pts',(23.007418206361,70.7783236950588,0.));
#104093=CARTESIAN_POINT('Ctrl Pts',(23.007418206361,70.7783236950588,12.));
#104094=CARTESIAN_POINT('Ctrl Pts',(23.004193629142,70.806028785987,0.));
#104095=CARTESIAN_POINT('Ctrl Pts',(23.004193629142,70.806028785987,12.));
#104096=CARTESIAN_POINT('Ctrl Pts',(23.0015908899222,70.8282180956627,0.));
#104097=CARTESIAN_POINT('Ctrl Pts',(23.0015908899222,70.8282180956627,12.));
#104098=CARTESIAN_POINT('Ctrl Pts',(22.9996258555187,70.8448742696329,0.));
#104099=CARTESIAN_POINT('Ctrl Pts',(22.9996258555187,70.8448742696329,12.));
#104100=CARTESIAN_POINT('Ctrl Pts',(22.9983100639353,70.8559846927868,0.));
#104101=CARTESIAN_POINT('Ctrl Pts',(22.9983100639353,70.8559846927868,12.));
#104102=CARTESIAN_POINT('Ctrl Pts',(22.9976507259816,70.8615414811572,0.));
#104103=CARTESIAN_POINT('Ctrl Pts',(22.9976507259816,70.8615414811572,12.));
#104104=CARTESIAN_POINT('',(23.1372951448024,66.0656156664138,0.));
#104105=CARTESIAN_POINT('Ctrl Pts',(23.1372951448024,66.0656156664138,0.));
#104106=CARTESIAN_POINT('Ctrl Pts',(23.1375957166104,66.0694876382127,0.));
#104107=CARTESIAN_POINT('Ctrl Pts',(23.1381951597399,66.0772371487248,0.));
#104108=CARTESIAN_POINT('Ctrl Pts',(23.1390892229778,66.0888781152421,0.));
#104109=CARTESIAN_POINT('Ctrl Pts',(23.1402711039425,66.1044328067355,0.));
#104110=CARTESIAN_POINT('Ctrl Pts',(23.1417314398398,66.1239318368548,0.));
#104111=CARTESIAN_POINT('Ctrl Pts',(23.1431747350098,66.1434865015027,0.));
#104112=CARTESIAN_POINT('Ctrl Pts',(23.1446009424903,66.1630967296747,0.));
#104113=CARTESIAN_POINT('Ctrl Pts',(23.1460099850763,66.18276239029,0.));
#104114=CARTESIAN_POINT('Ctrl Pts',(23.1474017566484,66.2024832934866,0.));
#104115=CARTESIAN_POINT('Ctrl Pts',(23.1487761349328,66.2222592165473,0.));
#104116=CARTESIAN_POINT('Ctrl Pts',(23.1501329914487,66.2420899237317,0.));
#104117=CARTESIAN_POINT('Ctrl Pts',(23.1514722022483,66.2619751878741,0.));
#104118=CARTESIAN_POINT('Ctrl Pts',(23.1527936592625,66.2819148131072,0.));
#104119=CARTESIAN_POINT('Ctrl Pts',(23.154097266617,66.301908627539,0.));
#104120=CARTESIAN_POINT('Ctrl Pts',(23.1553829352531,66.3219564725161,0.));
#104121=CARTESIAN_POINT('Ctrl Pts',(23.1566505784626,66.3420581937159,0.));
#104122=CARTESIAN_POINT('Ctrl Pts',(23.1579001063438,66.3622136300692,0.));
#104123=CARTESIAN_POINT('Ctrl Pts',(23.15913142301,66.382422608185,0.));
#104124=CARTESIAN_POINT('Ctrl Pts',(23.1603444294754,66.402684948127,0.));
#104125=CARTESIAN_POINT('Ctrl Pts',(23.1615390254635,66.4230004670288,0.));
#104126=CARTESIAN_POINT('Ctrl Pts',(23.1627151114875,66.4433689832454,0.));
#104127=CARTESIAN_POINT('Ctrl Pts',(23.163872591218,66.4637903210682,0.));
#104128=CARTESIAN_POINT('Ctrl Pts',(23.1650113713792,66.4842643105263,0.));
#104129=CARTESIAN_POINT('Ctrl Pts',(23.1661313606123,66.5047907851319,0.));
#104130=CARTESIAN_POINT('Ctrl Pts',(23.1672324686927,66.5253695803209,0.));
#104131=CARTESIAN_POINT('Ctrl Pts',(23.1683146055736,66.5460005315406,0.));
#104132=CARTESIAN_POINT('Ctrl Pts',(23.169377680588,66.5666834726495,0.));
#104133=CARTESIAN_POINT('Ctrl Pts',(23.1704216028626,66.5874182367597,0.));
#104134=CARTESIAN_POINT('Ctrl Pts',(23.1714462816794,66.6082046569657,0.));
#104135=CARTESIAN_POINT('Ctrl Pts',(23.1724516268299,66.6290425670538,0.));
#104136=CARTESIAN_POINT('Ctrl Pts',(23.1734375490421,66.6499318023445,0.));
#104137=CARTESIAN_POINT('Ctrl Pts',(23.174403960137,66.6708722000046,0.));
#104138=CARTESIAN_POINT('Ctrl Pts',(23.1753507727931,66.691863598595,0.));
#104139=CARTESIAN_POINT('Ctrl Pts',(23.1762779004043,66.712905837789,0.));
#104140=CARTESIAN_POINT('Ctrl Pts',(23.1771852569136,66.7339987580441,0.));
#104141=CARTESIAN_POINT('Ctrl Pts',(23.1780727566309,66.7551422002229,0.));
#104142=CARTESIAN_POINT('Ctrl Pts',(23.1789403142375,66.7763360056146,0.));
#104143=CARTESIAN_POINT('Ctrl Pts',(23.1797878448645,66.7975800161014,0.));
#104144=CARTESIAN_POINT('Ctrl Pts',(23.1806152641475,66.8188740742727,0.));
#104145=CARTESIAN_POINT('Ctrl Pts',(23.1814224882948,66.840218023555,0.));
#104146=CARTESIAN_POINT('Ctrl Pts',(23.1822094341508,66.8616117083304,0.));
#104147=CARTESIAN_POINT('Ctrl Pts',(23.1829760191582,66.8830549738768,0.));
#104148=CARTESIAN_POINT('Ctrl Pts',(23.1837221613231,66.904547666305,0.));
#104149=CARTESIAN_POINT('Ctrl Pts',(23.1844477791816,66.9260896324955,0.));
#104150=CARTESIAN_POINT('Ctrl Pts',(23.1851527917665,66.9476807200225,0.));
#104151=CARTESIAN_POINT('Ctrl Pts',(23.1858371185852,66.9693207771059,0.));
#104152=CARTESIAN_POINT('Ctrl Pts',(23.1865006796291,66.9910096526483,0.));
#104153=CARTESIAN_POINT('Ctrl Pts',(23.1871433953795,67.0127471962507,0.));
#104154=CARTESIAN_POINT('Ctrl Pts',(23.1877651868155,67.0345332582297,0.));
#104155=CARTESIAN_POINT('Ctrl Pts',(23.1883659754267,67.0563676896312,0.));
#104156=CARTESIAN_POINT('Ctrl Pts',(23.1889456832115,67.0782503422293,0.));
#104157=CARTESIAN_POINT('Ctrl Pts',(23.1895042326625,67.1001810685138,0.));
#104158=CARTESIAN_POINT('Ctrl Pts',(23.1900415467574,67.122159721674,0.));
#104159=CARTESIAN_POINT('Ctrl Pts',(23.1905575489505,67.1441861555819,0.));
#104160=CARTESIAN_POINT('Ctrl Pts',(23.1910521631658,67.1662602247641,0.));
#104161=CARTESIAN_POINT('Ctrl Pts',(23.1915253137923,67.1883817844039,0.));
#104162=CARTESIAN_POINT('Ctrl Pts',(23.1919769256803,67.2105506903448,0.));
#104163=CARTESIAN_POINT('Ctrl Pts',(23.1924069241385,67.232766799088,0.));
#104164=CARTESIAN_POINT('Ctrl Pts',(23.1928152349343,67.2550299677888,0.));
#104165=CARTESIAN_POINT('Ctrl Pts',(23.1932017842954,67.2773400542477,0.));
#104166=CARTESIAN_POINT('Ctrl Pts',(23.193566498902,67.2996969169099,0.));
#104167=CARTESIAN_POINT('Ctrl Pts',(23.1939093058802,67.3221004148604,0.));
#104168=CARTESIAN_POINT('Ctrl Pts',(23.1942301327978,67.3445504078178,0.));
#104169=CARTESIAN_POINT('Ctrl Pts',(23.1945289076608,67.3670467561205,0.));
#104170=CARTESIAN_POINT('Ctrl Pts',(23.1948055589123,67.3895893207168,0.));
#104171=CARTESIAN_POINT('Ctrl Pts',(23.1950600154259,67.4121779631666,0.));
#104172=CARTESIAN_POINT('Ctrl Pts',(23.1952922065009,67.4348125456389,0.));
#104173=CARTESIAN_POINT('Ctrl Pts',(23.1955020618591,67.4574929309079,0.));
#104174=CARTESIAN_POINT('Ctrl Pts',(23.1956895116446,67.4802189823424,0.));
#104175=CARTESIAN_POINT('Ctrl Pts',(23.1958544864224,67.5029905638974,0.));
#104176=CARTESIAN_POINT('Ctrl Pts',(23.1959969171709,67.525807540117,0.));
#104177=CARTESIAN_POINT('Ctrl Pts',(23.1961167352776,67.5486697761301,0.));
#104178=CARTESIAN_POINT('Ctrl Pts',(23.1962138725358,67.5715771376454,0.));
#104179=CARTESIAN_POINT('Ctrl Pts',(23.1962882611443,67.5945294909398,0.));
#104180=CARTESIAN_POINT('Ctrl Pts',(23.1963398337055,67.6175267028517,0.));
#104181=CARTESIAN_POINT('Ctrl Pts',(23.1963685232176,67.6405686407828,0.));
#104182=CARTESIAN_POINT('Ctrl Pts',(23.1963742630709,67.6636551726948,0.));
#104183=CARTESIAN_POINT('Ctrl Pts',(23.1963569870456,67.6867861671045,0.));
#104184=CARTESIAN_POINT('Ctrl Pts',(23.1963166293116,67.7099614930712,0.));
#104185=CARTESIAN_POINT('Ctrl Pts',(23.1962531244261,67.7331810201931,0.));
#104186=CARTESIAN_POINT('Ctrl Pts',(23.1961664073273,67.7564446186115,0.));
#104187=CARTESIAN_POINT('Ctrl Pts',(23.1960564133308,67.7797521590056,0.));
#104188=CARTESIAN_POINT('Ctrl Pts',(23.1959230781265,67.8031035125873,0.));
#104189=CARTESIAN_POINT('Ctrl Pts',(23.1957663377797,67.8264985510884,0.));
#104190=CARTESIAN_POINT('Ctrl Pts',(23.1955861287275,67.8499371467578,0.));
#104191=CARTESIAN_POINT('Ctrl Pts',(23.1953823877726,67.8734191723639,0.));
#104192=CARTESIAN_POINT('Ctrl Pts',(23.19515505208,67.8969445011908,0.));
#104193=CARTESIAN_POINT('Ctrl Pts',(23.1949040591748,67.9205130070337,0.));
#104194=CARTESIAN_POINT('Ctrl Pts',(23.1946293469436,67.9441245641871,0.));
#104195=CARTESIAN_POINT('Ctrl Pts',(23.1943308536307,67.9677790474414,0.));
#104196=CARTESIAN_POINT('Ctrl Pts',(23.1940085178319,67.9914763320878,0.));
#104197=CARTESIAN_POINT('Ctrl Pts',(23.193662278492,68.0152162939123,0.));
#104198=CARTESIAN_POINT('Ctrl Pts',(23.1932920749021,68.0389988091926,0.));
#104199=CARTESIAN_POINT('Ctrl Pts',(23.1928978467017,68.0628237546853,0.));
#104200=CARTESIAN_POINT('Ctrl Pts',(23.1924795338745,68.086691007624,0.));
#104201=CARTESIAN_POINT('Ctrl Pts',(23.1920370767423,68.1106004457223,0.));
#104202=CARTESIAN_POINT('Ctrl Pts',(23.1915704159623,68.1345519471695,0.));
#104203=CARTESIAN_POINT('Ctrl Pts',(23.1910794925252,68.1585453906259,0.));
#104204=CARTESIAN_POINT('Ctrl Pts',(23.1905642477571,68.182580655213,0.));
#104205=CARTESIAN_POINT('Ctrl Pts',(23.1900246233164,68.2066576205113,0.));
#104206=CARTESIAN_POINT('Ctrl Pts',(23.1894605611869,68.2307761665629,0.));
#104207=CARTESIAN_POINT('Ctrl Pts',(23.1888720036756,68.2549361738679,0.));
#104208=CARTESIAN_POINT('Ctrl Pts',(23.1882588934108,68.2791375233798,0.));
#104209=CARTESIAN_POINT('Ctrl Pts',(23.1876211733439,68.3033800964946,0.));
#104210=CARTESIAN_POINT('Ctrl Pts',(23.1869587867463,68.3276637750494,0.));
#104211=CARTESIAN_POINT('Ctrl Pts',(23.1862716772034,68.3519884413253,0.));
#104212=CARTESIAN_POINT('Ctrl Pts',(23.1855597886117,68.3763539780442,0.));
#104213=CARTESIAN_POINT('Ctrl Pts',(23.1848230651775,68.4007602683649,0.));
#104214=CARTESIAN_POINT('Ctrl Pts',(23.184061451419,68.4252071958725,0.));
#104215=CARTESIAN_POINT('Ctrl Pts',(23.1832748921629,68.4496946445756,0.));
#104216=CARTESIAN_POINT('Ctrl Pts',(23.1824633325384,68.4742224989099,0.));
#104217=CARTESIAN_POINT('Ctrl Pts',(23.1816267179751,68.4987906437357,0.));
#104218=CARTESIAN_POINT('Ctrl Pts',(23.180764994201,68.5233989643344,0.));
#104219=CARTESIAN_POINT('Ctrl Pts',(23.1798781072449,68.548047346398,0.));
#104220=CARTESIAN_POINT('Ctrl Pts',(23.1789660034339,68.572735676027,0.));
#104221=CARTESIAN_POINT('Ctrl Pts',(23.1780286293873,68.5974638397322,0.));
#104222=CARTESIAN_POINT('Ctrl Pts',(23.1770659320136,68.6222317244337,0.));
#104223=CARTESIAN_POINT('Ctrl Pts',(23.1760778585093,68.6470392174567,0.));
#104224=CARTESIAN_POINT('Ctrl Pts',(23.1750643563605,68.6718862065227,0.));
#104225=CARTESIAN_POINT('Ctrl Pts',(23.1740253733423,68.6967725797458,0.));
#104226=CARTESIAN_POINT('Ctrl Pts',(23.1729608575115,68.7216982256357,0.));
#104227=CARTESIAN_POINT('Ctrl Pts',(23.1718707572046,68.7466630330968,0.));
#104228=CARTESIAN_POINT('Ctrl Pts',(23.1707550210359,68.7716668914246,0.));
#104229=CARTESIAN_POINT('Ctrl Pts',(23.1696135978992,68.7967096902981,0.));
#104230=CARTESIAN_POINT('Ctrl Pts',(23.1684464369681,68.8217913197735,0.));
#104231=CARTESIAN_POINT('Ctrl Pts',(23.1672534876885,68.8469116702885,0.));
#104232=CARTESIAN_POINT('Ctrl Pts',(23.1660346997762,68.8720706326606,0.));
#104233=CARTESIAN_POINT('Ctrl Pts',(23.1647900232151,68.8972680980844,0.));
#104234=CARTESIAN_POINT('Ctrl Pts',(23.1635194082581,68.9225039581249,0.));
#104235=CARTESIAN_POINT('Ctrl Pts',(23.162222805429,68.9477781047103,0.));
#104236=CARTESIAN_POINT('Ctrl Pts',(23.1609001655153,68.9730904301363,0.));
#104237=CARTESIAN_POINT('Ctrl Pts',(23.1595514395654,68.9984408270653,0.));
#104238=CARTESIAN_POINT('Ctrl Pts',(23.1581765788869,69.0238291885245,0.));
#104239=CARTESIAN_POINT('Ctrl Pts',(23.1567755350472,69.0492554078999,0.));
#104240=CARTESIAN_POINT('Ctrl Pts',(23.1553482598767,69.0747193789292,0.));
#104241=CARTESIAN_POINT('Ctrl Pts',(23.1538947054619,69.1002209957037,0.));
#104242=CARTESIAN_POINT('Ctrl Pts',(23.1524148241413,69.1257601526693,0.));
#104243=CARTESIAN_POINT('Ctrl Pts',(23.1509085685032,69.1513367446231,0.));
#104244=CARTESIAN_POINT('Ctrl Pts',(23.1493758913857,69.176950666708,0.));
#104245=CARTESIAN_POINT('Ctrl Pts',(23.1478167458787,69.2026018144023,0.));
#104246=CARTESIAN_POINT('Ctrl Pts',(23.1462310853205,69.2282900835234,0.));
#104247=CARTESIAN_POINT('Ctrl Pts',(23.1446188632931,69.2540153702311,0.));
#104248=CARTESIAN_POINT('Ctrl Pts',(23.142980033622,69.2797775710275,0.));
#104249=CARTESIAN_POINT('Ctrl Pts',(23.1413145503762,69.3055765827544,0.));
#104250=CARTESIAN_POINT('Ctrl Pts',(23.1396223678725,69.3314123025863,0.));
#104251=CARTESIAN_POINT('Ctrl Pts',(23.1379034406717,69.3572846280289,0.));
#104252=CARTESIAN_POINT('Ctrl Pts',(23.1361577235708,69.3831934569176,0.));
#104253=CARTESIAN_POINT('Ctrl Pts',(23.1343851715988,69.4091386874129,0.));
#104254=CARTESIAN_POINT('Ctrl Pts',(23.1325857400145,69.4351202179948,0.));
#104255=CARTESIAN_POINT('Ctrl Pts',(23.1307593843063,69.4611379474492,0.));
#104256=CARTESIAN_POINT('Ctrl Pts',(23.1289060601927,69.4871917748665,0.));
#104257=CARTESIAN_POINT('Ctrl Pts',(23.1270257236207,69.5132815996548,0.));
#104258=CARTESIAN_POINT('Ctrl Pts',(23.1251183307678,69.5394073215467,0.));
#104259=CARTESIAN_POINT('Ctrl Pts',(23.1231838380452,69.565568840605,0.));
#104260=CARTESIAN_POINT('Ctrl Pts',(23.1212222021049,69.5917660572255,0.));
#104261=CARTESIAN_POINT('Ctrl Pts',(23.1192333798437,69.617998872135,0.));
#104262=CARTESIAN_POINT('Ctrl Pts',(23.1172173283855,69.6442671863751,0.));
#104263=CARTESIAN_POINT('Ctrl Pts',(23.1151740050678,69.6705709012842,0.));
#104264=CARTESIAN_POINT('Ctrl Pts',(23.1131033674301,69.6969099184766,0.));
#104265=CARTESIAN_POINT('Ctrl Pts',(23.1110053732049,69.7232841398207,0.));
#104266=CARTESIAN_POINT('Ctrl Pts',(23.1088799803093,69.7496934674083,0.));
#104267=CARTESIAN_POINT('Ctrl Pts',(23.1067271468614,69.7761378035979,0.));
#104268=CARTESIAN_POINT('Ctrl Pts',(23.1045468311994,69.8026170510582,0.));
#104269=CARTESIAN_POINT('Ctrl Pts',(23.1023389919052,69.8291311128121,0.));
#104270=CARTESIAN_POINT('Ctrl Pts',(23.100103587824,69.8556798922688,0.));
#104271=CARTESIAN_POINT('Ctrl Pts',(23.0978405781018,69.882263293276,0.));
#104272=CARTESIAN_POINT('Ctrl Pts',(23.0955499221555,69.9088812200704,0.));
#104273=CARTESIAN_POINT('Ctrl Pts',(23.0932315796066,69.9355335771722,0.));
#104274=CARTESIAN_POINT('Ctrl Pts',(23.090885510225,69.9622202692871,0.));
#104275=CARTESIAN_POINT('Ctrl Pts',(23.0885116738798,69.9889412012143,0.));
#104276=CARTESIAN_POINT('Ctrl Pts',(23.0861100304731,70.0156962777173,0.));
#104277=CARTESIAN_POINT('Ctrl Pts',(23.0836805399377,70.0424854035125,0.));
#104278=CARTESIAN_POINT('Ctrl Pts',(23.081223162377,70.0693084835388,0.));
#104279=CARTESIAN_POINT('Ctrl Pts',(23.0787378581778,70.096165423165,0.));
#104280=CARTESIAN_POINT('Ctrl Pts',(23.076224588139,70.1230561284222,0.));
#104281=CARTESIAN_POINT('Ctrl Pts',(23.0736833135934,70.1499805062159,0.));
#104282=CARTESIAN_POINT('Ctrl Pts',(23.0711139965432,70.176938464556,0.));
#104283=CARTESIAN_POINT('Ctrl Pts',(23.0685165993681,70.2039299120456,0.));
#104284=CARTESIAN_POINT('Ctrl Pts',(23.0658910845425,70.2309547573789,0.));
#104285=CARTESIAN_POINT('Ctrl Pts',(23.0632374143276,70.2580129087878,0.));
#104286=CARTESIAN_POINT('Ctrl Pts',(23.0605555505326,70.2851042736081,0.));
#104287=CARTESIAN_POINT('Ctrl Pts',(23.0578454541116,70.3122287575374,0.));
#104288=CARTESIAN_POINT('Ctrl Pts',(23.0551070854942,70.3393862652353,0.));
#104289=CARTESIAN_POINT('Ctrl Pts',(23.0523404053188,70.3665767016596,0.));
#104290=CARTESIAN_POINT('Ctrl Pts',(23.0495453750773,70.39379997323,0.));
#104291=CARTESIAN_POINT('Ctrl Pts',(23.0467219577288,70.421055988934,0.));
#104292=CARTESIAN_POINT('Ctrl Pts',(23.0438701184995,70.4483446617553,0.));
#104293=CARTESIAN_POINT('Ctrl Pts',(23.0409898250726,70.4756659090104,0.));
#104294=CARTESIAN_POINT('Ctrl Pts',(23.038496437601,70.4991133648755,0.));
#104295=CARTESIAN_POINT('Ctrl Pts',(23.0365694096158,70.5171075702494,0.));
#104296=CARTESIAN_POINT('Ctrl Pts',(23.0352213647764,70.529634153525,0.));
#104297=CARTESIAN_POINT('Ctrl Pts',(23.034460662331,70.5366836381296,0.));
#104298=CARTESIAN_POINT('Ctrl Pts',(23.0342913834094,70.5382514078485,0.));
#104299=CARTESIAN_POINT('',(23.1372951448024,66.0656156664138,12.));
#104300=CARTESIAN_POINT('',(23.1372951448024,66.0656156664138,0.));
#104301=CARTESIAN_POINT('Ctrl Pts',(23.0342913834094,70.5382514078485,12.));
#104302=CARTESIAN_POINT('Ctrl Pts',(23.034460662331,70.5366836381296,12.));
#104303=CARTESIAN_POINT('Ctrl Pts',(23.0352213647764,70.529634153525,12.));
#104304=CARTESIAN_POINT('Ctrl Pts',(23.0365694096158,70.5171075702494,12.));
#104305=CARTESIAN_POINT('Ctrl Pts',(23.038496437601,70.4991133648755,12.));
#104306=CARTESIAN_POINT('Ctrl Pts',(23.0409898250726,70.4756659090104,12.));
#104307=CARTESIAN_POINT('Ctrl Pts',(23.0438701184995,70.4483446617553,12.));
#104308=CARTESIAN_POINT('Ctrl Pts',(23.0467219577288,70.421055988934,12.));
#104309=CARTESIAN_POINT('Ctrl Pts',(23.0495453750773,70.39379997323,12.));
#104310=CARTESIAN_POINT('Ctrl Pts',(23.0523404053188,70.3665767016596,12.));
#104311=CARTESIAN_POINT('Ctrl Pts',(23.0551070854942,70.3393862652353,12.));
#104312=CARTESIAN_POINT('Ctrl Pts',(23.0578454541116,70.3122287575374,12.));
#104313=CARTESIAN_POINT('Ctrl Pts',(23.0605555505326,70.2851042736081,12.));
#104314=CARTESIAN_POINT('Ctrl Pts',(23.0632374143276,70.2580129087878,12.));
#104315=CARTESIAN_POINT('Ctrl Pts',(23.0658910845425,70.2309547573789,12.));
#104316=CARTESIAN_POINT('Ctrl Pts',(23.0685165993681,70.2039299120456,12.));
#104317=CARTESIAN_POINT('Ctrl Pts',(23.0711139965432,70.176938464556,12.));
#104318=CARTESIAN_POINT('Ctrl Pts',(23.0736833135934,70.1499805062159,12.));
#104319=CARTESIAN_POINT('Ctrl Pts',(23.076224588139,70.1230561284222,12.));
#104320=CARTESIAN_POINT('Ctrl Pts',(23.0787378581778,70.096165423165,12.));
#104321=CARTESIAN_POINT('Ctrl Pts',(23.081223162377,70.0693084835388,12.));
#104322=CARTESIAN_POINT('Ctrl Pts',(23.0836805399377,70.0424854035125,12.));
#104323=CARTESIAN_POINT('Ctrl Pts',(23.0861100304731,70.0156962777173,12.));
#104324=CARTESIAN_POINT('Ctrl Pts',(23.0885116738798,69.9889412012143,12.));
#104325=CARTESIAN_POINT('Ctrl Pts',(23.090885510225,69.9622202692871,12.));
#104326=CARTESIAN_POINT('Ctrl Pts',(23.0932315796066,69.9355335771722,12.));
#104327=CARTESIAN_POINT('Ctrl Pts',(23.0955499221555,69.9088812200704,12.));
#104328=CARTESIAN_POINT('Ctrl Pts',(23.0978405781018,69.882263293276,12.));
#104329=CARTESIAN_POINT('Ctrl Pts',(23.100103587824,69.8556798922688,12.));
#104330=CARTESIAN_POINT('Ctrl Pts',(23.1023389919052,69.8291311128121,12.));
#104331=CARTESIAN_POINT('Ctrl Pts',(23.1045468311994,69.8026170510582,12.));
#104332=CARTESIAN_POINT('Ctrl Pts',(23.1067271468614,69.7761378035979,12.));
#104333=CARTESIAN_POINT('Ctrl Pts',(23.1088799803093,69.7496934674083,12.));
#104334=CARTESIAN_POINT('Ctrl Pts',(23.1110053732049,69.7232841398207,12.));
#104335=CARTESIAN_POINT('Ctrl Pts',(23.1131033674301,69.6969099184766,12.));
#104336=CARTESIAN_POINT('Ctrl Pts',(23.1151740050678,69.6705709012842,12.));
#104337=CARTESIAN_POINT('Ctrl Pts',(23.1172173283855,69.6442671863751,12.));
#104338=CARTESIAN_POINT('Ctrl Pts',(23.1192333798437,69.617998872135,12.));
#104339=CARTESIAN_POINT('Ctrl Pts',(23.1212222021049,69.5917660572255,12.));
#104340=CARTESIAN_POINT('Ctrl Pts',(23.1231838380452,69.565568840605,12.));
#104341=CARTESIAN_POINT('Ctrl Pts',(23.1251183307678,69.5394073215467,12.));
#104342=CARTESIAN_POINT('Ctrl Pts',(23.1270257236207,69.5132815996548,12.));
#104343=CARTESIAN_POINT('Ctrl Pts',(23.1289060601927,69.4871917748665,12.));
#104344=CARTESIAN_POINT('Ctrl Pts',(23.1307593843063,69.4611379474492,12.));
#104345=CARTESIAN_POINT('Ctrl Pts',(23.1325857400145,69.4351202179948,12.));
#104346=CARTESIAN_POINT('Ctrl Pts',(23.1343851715988,69.4091386874129,12.));
#104347=CARTESIAN_POINT('Ctrl Pts',(23.1361577235708,69.3831934569176,12.));
#104348=CARTESIAN_POINT('Ctrl Pts',(23.1379034406717,69.3572846280289,12.));
#104349=CARTESIAN_POINT('Ctrl Pts',(23.1396223678725,69.3314123025863,12.));
#104350=CARTESIAN_POINT('Ctrl Pts',(23.1413145503762,69.3055765827544,12.));
#104351=CARTESIAN_POINT('Ctrl Pts',(23.142980033622,69.2797775710275,12.));
#104352=CARTESIAN_POINT('Ctrl Pts',(23.1446188632931,69.2540153702311,12.));
#104353=CARTESIAN_POINT('Ctrl Pts',(23.1462310853205,69.2282900835234,12.));
#104354=CARTESIAN_POINT('Ctrl Pts',(23.1478167458787,69.2026018144023,12.));
#104355=CARTESIAN_POINT('Ctrl Pts',(23.1493758913857,69.176950666708,12.));
#104356=CARTESIAN_POINT('Ctrl Pts',(23.1509085685032,69.1513367446231,12.));
#104357=CARTESIAN_POINT('Ctrl Pts',(23.1524148241413,69.1257601526693,12.));
#104358=CARTESIAN_POINT('Ctrl Pts',(23.1538947054619,69.1002209957037,12.));
#104359=CARTESIAN_POINT('Ctrl Pts',(23.1553482598767,69.0747193789292,12.));
#104360=CARTESIAN_POINT('Ctrl Pts',(23.1567755350472,69.0492554078999,12.));
#104361=CARTESIAN_POINT('Ctrl Pts',(23.1581765788869,69.0238291885245,12.));
#104362=CARTESIAN_POINT('Ctrl Pts',(23.1595514395654,68.9984408270653,12.));
#104363=CARTESIAN_POINT('Ctrl Pts',(23.1609001655153,68.9730904301363,12.));
#104364=CARTESIAN_POINT('Ctrl Pts',(23.162222805429,68.9477781047103,12.));
#104365=CARTESIAN_POINT('Ctrl Pts',(23.1635194082581,68.9225039581249,12.));
#104366=CARTESIAN_POINT('Ctrl Pts',(23.1647900232151,68.8972680980844,12.));
#104367=CARTESIAN_POINT('Ctrl Pts',(23.1660346997762,68.8720706326606,12.));
#104368=CARTESIAN_POINT('Ctrl Pts',(23.1672534876885,68.8469116702885,12.));
#104369=CARTESIAN_POINT('Ctrl Pts',(23.1684464369681,68.8217913197735,12.));
#104370=CARTESIAN_POINT('Ctrl Pts',(23.1696135978992,68.7967096902981,12.));
#104371=CARTESIAN_POINT('Ctrl Pts',(23.1707550210359,68.7716668914246,12.));
#104372=CARTESIAN_POINT('Ctrl Pts',(23.1718707572046,68.7466630330968,12.));
#104373=CARTESIAN_POINT('Ctrl Pts',(23.1729608575115,68.7216982256357,12.));
#104374=CARTESIAN_POINT('Ctrl Pts',(23.1740253733423,68.6967725797458,12.));
#104375=CARTESIAN_POINT('Ctrl Pts',(23.1750643563605,68.6718862065227,12.));
#104376=CARTESIAN_POINT('Ctrl Pts',(23.1760778585093,68.6470392174567,12.));
#104377=CARTESIAN_POINT('Ctrl Pts',(23.1770659320136,68.6222317244337,12.));
#104378=CARTESIAN_POINT('Ctrl Pts',(23.1780286293873,68.5974638397322,12.));
#104379=CARTESIAN_POINT('Ctrl Pts',(23.1789660034339,68.572735676027,12.));
#104380=CARTESIAN_POINT('Ctrl Pts',(23.1798781072449,68.548047346398,12.));
#104381=CARTESIAN_POINT('Ctrl Pts',(23.180764994201,68.5233989643344,12.));
#104382=CARTESIAN_POINT('Ctrl Pts',(23.1816267179751,68.4987906437357,12.));
#104383=CARTESIAN_POINT('Ctrl Pts',(23.1824633325384,68.4742224989099,12.));
#104384=CARTESIAN_POINT('Ctrl Pts',(23.1832748921629,68.4496946445756,12.));
#104385=CARTESIAN_POINT('Ctrl Pts',(23.184061451419,68.4252071958725,12.));
#104386=CARTESIAN_POINT('Ctrl Pts',(23.1848230651775,68.4007602683649,12.));
#104387=CARTESIAN_POINT('Ctrl Pts',(23.1855597886117,68.3763539780442,12.));
#104388=CARTESIAN_POINT('Ctrl Pts',(23.1862716772034,68.3519884413253,12.));
#104389=CARTESIAN_POINT('Ctrl Pts',(23.1869587867463,68.3276637750494,12.));
#104390=CARTESIAN_POINT('Ctrl Pts',(23.1876211733439,68.3033800964946,12.));
#104391=CARTESIAN_POINT('Ctrl Pts',(23.1882588934108,68.2791375233798,12.));
#104392=CARTESIAN_POINT('Ctrl Pts',(23.1888720036756,68.2549361738679,12.));
#104393=CARTESIAN_POINT('Ctrl Pts',(23.1894605611869,68.2307761665629,12.));
#104394=CARTESIAN_POINT('Ctrl Pts',(23.1900246233164,68.2066576205113,12.));
#104395=CARTESIAN_POINT('Ctrl Pts',(23.1905642477571,68.182580655213,12.));
#104396=CARTESIAN_POINT('Ctrl Pts',(23.1910794925252,68.1585453906259,12.));
#104397=CARTESIAN_POINT('Ctrl Pts',(23.1915704159623,68.1345519471695,12.));
#104398=CARTESIAN_POINT('Ctrl Pts',(23.1920370767423,68.1106004457223,12.));
#104399=CARTESIAN_POINT('Ctrl Pts',(23.1924795338745,68.086691007624,12.));
#104400=CARTESIAN_POINT('Ctrl Pts',(23.1928978467017,68.0628237546853,12.));
#104401=CARTESIAN_POINT('Ctrl Pts',(23.1932920749021,68.0389988091926,12.));
#104402=CARTESIAN_POINT('Ctrl Pts',(23.193662278492,68.0152162939123,12.));
#104403=CARTESIAN_POINT('Ctrl Pts',(23.1940085178319,67.9914763320878,12.));
#104404=CARTESIAN_POINT('Ctrl Pts',(23.1943308536307,67.9677790474414,12.));
#104405=CARTESIAN_POINT('Ctrl Pts',(23.1946293469436,67.9441245641871,12.));
#104406=CARTESIAN_POINT('Ctrl Pts',(23.1949040591748,67.9205130070337,12.));
#104407=CARTESIAN_POINT('Ctrl Pts',(23.19515505208,67.8969445011908,12.));
#104408=CARTESIAN_POINT('Ctrl Pts',(23.1953823877726,67.8734191723639,12.));
#104409=CARTESIAN_POINT('Ctrl Pts',(23.1955861287275,67.8499371467578,12.));
#104410=CARTESIAN_POINT('Ctrl Pts',(23.1957663377797,67.8264985510884,12.));
#104411=CARTESIAN_POINT('Ctrl Pts',(23.1959230781265,67.8031035125873,12.));
#104412=CARTESIAN_POINT('Ctrl Pts',(23.1960564133308,67.7797521590056,12.));
#104413=CARTESIAN_POINT('Ctrl Pts',(23.1961664073273,67.7564446186115,12.));
#104414=CARTESIAN_POINT('Ctrl Pts',(23.1962531244261,67.7331810201931,12.));
#104415=CARTESIAN_POINT('Ctrl Pts',(23.1963166293116,67.7099614930712,12.));
#104416=CARTESIAN_POINT('Ctrl Pts',(23.1963569870456,67.6867861671045,12.));
#104417=CARTESIAN_POINT('Ctrl Pts',(23.1963742630709,67.6636551726948,12.));
#104418=CARTESIAN_POINT('Ctrl Pts',(23.1963685232176,67.6405686407828,12.));
#104419=CARTESIAN_POINT('Ctrl Pts',(23.1963398337055,67.6175267028517,12.));
#104420=CARTESIAN_POINT('Ctrl Pts',(23.1962882611443,67.5945294909398,12.));
#104421=CARTESIAN_POINT('Ctrl Pts',(23.1962138725358,67.5715771376454,12.));
#104422=CARTESIAN_POINT('Ctrl Pts',(23.1961167352776,67.5486697761301,12.));
#104423=CARTESIAN_POINT('Ctrl Pts',(23.1959969171709,67.525807540117,12.));
#104424=CARTESIAN_POINT('Ctrl Pts',(23.1958544864224,67.5029905638974,12.));
#104425=CARTESIAN_POINT('Ctrl Pts',(23.1956895116446,67.4802189823424,12.));
#104426=CARTESIAN_POINT('Ctrl Pts',(23.1955020618591,67.4574929309079,12.));
#104427=CARTESIAN_POINT('Ctrl Pts',(23.1952922065009,67.4348125456389,12.));
#104428=CARTESIAN_POINT('Ctrl Pts',(23.1950600154259,67.4121779631666,12.));
#104429=CARTESIAN_POINT('Ctrl Pts',(23.1948055589123,67.3895893207168,12.));
#104430=CARTESIAN_POINT('Ctrl Pts',(23.1945289076608,67.3670467561205,12.));
#104431=CARTESIAN_POINT('Ctrl Pts',(23.1942301327978,67.3445504078178,12.));
#104432=CARTESIAN_POINT('Ctrl Pts',(23.1939093058802,67.3221004148604,12.));
#104433=CARTESIAN_POINT('Ctrl Pts',(23.193566498902,67.2996969169099,12.));
#104434=CARTESIAN_POINT('Ctrl Pts',(23.1932017842954,67.2773400542477,12.));
#104435=CARTESIAN_POINT('Ctrl Pts',(23.1928152349343,67.2550299677888,12.));
#104436=CARTESIAN_POINT('Ctrl Pts',(23.1924069241385,67.232766799088,12.));
#104437=CARTESIAN_POINT('Ctrl Pts',(23.1919769256803,67.2105506903448,12.));
#104438=CARTESIAN_POINT('Ctrl Pts',(23.1915253137923,67.1883817844039,12.));
#104439=CARTESIAN_POINT('Ctrl Pts',(23.1910521631658,67.1662602247641,12.));
#104440=CARTESIAN_POINT('Ctrl Pts',(23.1905575489505,67.1441861555819,12.));
#104441=CARTESIAN_POINT('Ctrl Pts',(23.1900415467574,67.122159721674,12.));
#104442=CARTESIAN_POINT('Ctrl Pts',(23.1895042326625,67.1001810685138,12.));
#104443=CARTESIAN_POINT('Ctrl Pts',(23.1889456832115,67.0782503422293,12.));
#104444=CARTESIAN_POINT('Ctrl Pts',(23.1883659754267,67.0563676896312,12.));
#104445=CARTESIAN_POINT('Ctrl Pts',(23.1877651868155,67.0345332582297,12.));
#104446=CARTESIAN_POINT('Ctrl Pts',(23.1871433953795,67.0127471962507,12.));
#104447=CARTESIAN_POINT('Ctrl Pts',(23.1865006796291,66.9910096526483,12.));
#104448=CARTESIAN_POINT('Ctrl Pts',(23.1858371185852,66.9693207771059,12.));
#104449=CARTESIAN_POINT('Ctrl Pts',(23.1851527917665,66.9476807200225,12.));
#104450=CARTESIAN_POINT('Ctrl Pts',(23.1844477791816,66.9260896324955,12.));
#104451=CARTESIAN_POINT('Ctrl Pts',(23.1837221613231,66.904547666305,12.));
#104452=CARTESIAN_POINT('Ctrl Pts',(23.1829760191582,66.8830549738768,12.));
#104453=CARTESIAN_POINT('Ctrl Pts',(23.1822094341508,66.8616117083304,12.));
#104454=CARTESIAN_POINT('Ctrl Pts',(23.1814224882948,66.840218023555,12.));
#104455=CARTESIAN_POINT('Ctrl Pts',(23.1806152641475,66.8188740742727,12.));
#104456=CARTESIAN_POINT('Ctrl Pts',(23.1797878448645,66.7975800161014,12.));
#104457=CARTESIAN_POINT('Ctrl Pts',(23.1789403142375,66.7763360056146,12.));
#104458=CARTESIAN_POINT('Ctrl Pts',(23.1780727566309,66.7551422002229,12.));
#104459=CARTESIAN_POINT('Ctrl Pts',(23.1771852569136,66.7339987580441,12.));
#104460=CARTESIAN_POINT('Ctrl Pts',(23.1762779004043,66.712905837789,12.));
#104461=CARTESIAN_POINT('Ctrl Pts',(23.1753507727931,66.691863598595,12.));
#104462=CARTESIAN_POINT('Ctrl Pts',(23.174403960137,66.6708722000046,12.));
#104463=CARTESIAN_POINT('Ctrl Pts',(23.1734375490421,66.6499318023445,12.));
#104464=CARTESIAN_POINT('Ctrl Pts',(23.1724516268299,66.6290425670538,12.));
#104465=CARTESIAN_POINT('Ctrl Pts',(23.1714462816794,66.6082046569657,12.));
#104466=CARTESIAN_POINT('Ctrl Pts',(23.1704216028626,66.5874182367597,12.));
#104467=CARTESIAN_POINT('Ctrl Pts',(23.169377680588,66.5666834726495,12.));
#104468=CARTESIAN_POINT('Ctrl Pts',(23.1683146055736,66.5460005315406,12.));
#104469=CARTESIAN_POINT('Ctrl Pts',(23.1672324686927,66.5253695803209,12.));
#104470=CARTESIAN_POINT('Ctrl Pts',(23.1661313606123,66.5047907851319,12.));
#104471=CARTESIAN_POINT('Ctrl Pts',(23.1650113713792,66.4842643105263,12.));
#104472=CARTESIAN_POINT('Ctrl Pts',(23.163872591218,66.4637903210682,12.));
#104473=CARTESIAN_POINT('Ctrl Pts',(23.1627151114875,66.4433689832454,12.));
#104474=CARTESIAN_POINT('Ctrl Pts',(23.1615390254635,66.4230004670288,12.));
#104475=CARTESIAN_POINT('Ctrl Pts',(23.1603444294754,66.402684948127,12.));
#104476=CARTESIAN_POINT('Ctrl Pts',(23.15913142301,66.382422608185,12.));
#104477=CARTESIAN_POINT('Ctrl Pts',(23.1579001063438,66.3622136300692,12.));
#104478=CARTESIAN_POINT('Ctrl Pts',(23.1566505784626,66.3420581937159,12.));
#104479=CARTESIAN_POINT('Ctrl Pts',(23.1553829352531,66.3219564725161,12.));
#104480=CARTESIAN_POINT('Ctrl Pts',(23.154097266617,66.301908627539,12.));
#104481=CARTESIAN_POINT('Ctrl Pts',(23.1527936592625,66.2819148131072,12.));
#104482=CARTESIAN_POINT('Ctrl Pts',(23.1514722022483,66.2619751878741,12.));
#104483=CARTESIAN_POINT('Ctrl Pts',(23.1501329914487,66.2420899237317,12.));
#104484=CARTESIAN_POINT('Ctrl Pts',(23.1487761349328,66.2222592165473,12.));
#104485=CARTESIAN_POINT('Ctrl Pts',(23.1474017566484,66.2024832934866,12.));
#104486=CARTESIAN_POINT('Ctrl Pts',(23.1460099850763,66.18276239029,12.));
#104487=CARTESIAN_POINT('Ctrl Pts',(23.1446009424903,66.1630967296747,12.));
#104488=CARTESIAN_POINT('Ctrl Pts',(23.1431747350098,66.1434865015027,12.));
#104489=CARTESIAN_POINT('Ctrl Pts',(23.1417314398398,66.1239318368548,12.));
#104490=CARTESIAN_POINT('Ctrl Pts',(23.1402711039425,66.1044328067355,12.));
#104491=CARTESIAN_POINT('Ctrl Pts',(23.1390892229778,66.0888781152421,12.));
#104492=CARTESIAN_POINT('Ctrl Pts',(23.1381951597399,66.0772371487248,12.));
#104493=CARTESIAN_POINT('Ctrl Pts',(23.1375957166104,66.0694876382127,12.));
#104494=CARTESIAN_POINT('Ctrl Pts',(23.1372951448024,66.0656156664138,12.));
#104495=CARTESIAN_POINT('Ctrl Pts',(21.5904919935065,70.993479606912,-5.55111512312578E-16));
#104496=CARTESIAN_POINT('Ctrl Pts',(21.5904919935065,70.993479606912,4.));
#104497=CARTESIAN_POINT('Ctrl Pts',(21.5904919935065,70.993479606912,8.));
#104498=CARTESIAN_POINT('Ctrl Pts',(21.5904919935065,70.993479606912,12.));
#104499=CARTESIAN_POINT('Ctrl Pts',(21.6628164325804,71.0762040404458,-5.55111512312578E-16));
#104500=CARTESIAN_POINT('Ctrl Pts',(21.6628164325804,71.0762040404458,3.99999999999999));
#104501=CARTESIAN_POINT('Ctrl Pts',(21.6628164325804,71.0762040404458,8.));
#104502=CARTESIAN_POINT('Ctrl Pts',(21.6628164325804,71.0762040404458,12.));
#104503=CARTESIAN_POINT('Ctrl Pts',(21.8385342042358,71.1771795679078,-5.55111512312578E-16));
#104504=CARTESIAN_POINT('Ctrl Pts',(21.8385342042358,71.1771795679078,4.00000000000001));
#104505=CARTESIAN_POINT('Ctrl Pts',(21.8385342042358,71.1771795679079,7.99999999999999));
#104506=CARTESIAN_POINT('Ctrl Pts',(21.8385342042358,71.1771795679079,12.));
#104507=CARTESIAN_POINT('Ctrl Pts',(22.0366423876805,71.1663065220502,-5.55111512312578E-16));
#104508=CARTESIAN_POINT('Ctrl Pts',(22.0366423876805,71.1663065220502,3.99999999999999));
#104509=CARTESIAN_POINT('Ctrl Pts',(22.0366423876805,71.1663065220503,8.00000000000001));
#104510=CARTESIAN_POINT('Ctrl Pts',(22.0366423876805,71.1663065220503,12.));
#104511=CARTESIAN_POINT('Ctrl Pts',(22.1153394458685,71.1418425484888,-5.55111512312578E-16));
#104512=CARTESIAN_POINT('Ctrl Pts',(22.1153394458685,71.1418425484888,4.));
#104513=CARTESIAN_POINT('Ctrl Pts',(22.1153394458685,71.1418425484888,8.));
#104514=CARTESIAN_POINT('Ctrl Pts',(22.1153394458685,71.1418425484888,12.));
#104515=CARTESIAN_POINT('',(21.5904919935065,70.993479606912,0.));
#104516=CARTESIAN_POINT('',(22.1153394458686,71.1418425484891,0.));
#104517=CARTESIAN_POINT('Ctrl Pts',(21.5904919935065,70.993479606912,0.));
#104518=CARTESIAN_POINT('Ctrl Pts',(21.6628164325804,71.0762040404458,-6.93334779979405E-31));
#104519=CARTESIAN_POINT('Ctrl Pts',(21.7632265878121,71.1339043418527,3.85185988877447E-31));
#104520=CARTESIAN_POINT('Ctrl Pts',(21.8709478979137,71.1550826601348,1.54074395550979E-31));
#104521=CARTESIAN_POINT('Ctrl Pts',(21.9517388804899,71.1709663988463,-3.08148791101957E-32));
#104522=CARTESIAN_POINT('Ctrl Pts',(22.0366423876805,71.1663065220502,-9.55261252416069E-31));
#104523=CARTESIAN_POINT('Ctrl Pts',(22.1153394458685,71.1418425484888,4.62223186652938E-32));
#104524=CARTESIAN_POINT('',(22.1153394458686,71.1418425484891,12.));
#104525=CARTESIAN_POINT('Ctrl Pts',(22.1153394458685,71.1418425484888,-5.55111512312578E-16));
#104526=CARTESIAN_POINT('Ctrl Pts',(22.1153394458685,71.1418425484888,4.));
#104527=CARTESIAN_POINT('Ctrl Pts',(22.1153394458685,71.1418425484888,8.));
#104528=CARTESIAN_POINT('Ctrl Pts',(22.1153394458685,71.1418425484888,12.));
#104529=CARTESIAN_POINT('',(21.5904919935065,70.993479606912,12.));
#104530=CARTESIAN_POINT('Ctrl Pts',(22.1153394458685,71.1418425484888,12.));
#104531=CARTESIAN_POINT('Ctrl Pts',(22.0366423876805,71.1663065220503,12.));
#104532=CARTESIAN_POINT('Ctrl Pts',(21.9517388804899,71.1709663988464,12.));
#104533=CARTESIAN_POINT('Ctrl Pts',(21.8709478979137,71.1550826601348,12.));
#104534=CARTESIAN_POINT('Ctrl Pts',(21.7632265878121,71.1339043418527,12.));
#104535=CARTESIAN_POINT('Ctrl Pts',(21.6628164325804,71.0762040404458,12.));
#104536=CARTESIAN_POINT('Ctrl Pts',(21.5904919935065,70.993479606912,12.));
#104537=CARTESIAN_POINT('Ctrl Pts',(21.5904919935065,70.993479606912,12.));
#104538=CARTESIAN_POINT('Ctrl Pts',(21.5904919935065,70.993479606912,8.));
#104539=CARTESIAN_POINT('Ctrl Pts',(21.5904919935065,70.993479606912,4.));
#104540=CARTESIAN_POINT('Ctrl Pts',(21.5904919935065,70.993479606912,-5.55111512312578E-16));
#104541=CARTESIAN_POINT('Origin',(1.12623029467293E-10,3.57524700084383E-10,
0.));
#104542=CARTESIAN_POINT('Origin',(1.12623029467293E-10,3.57524700084383E-10,
12.));
#104543=CARTESIAN_POINT('Origin',(1.12623029467293E-10,3.57524700084383E-10,
0.));
#104544=CARTESIAN_POINT('Ctrl Pts',(28.787762030239,68.7132793373328,0.));
#104545=CARTESIAN_POINT('Ctrl Pts',(28.787762030239,68.7132793373328,4.));
#104546=CARTESIAN_POINT('Ctrl Pts',(28.787762030239,68.7132793373328,8.));
#104547=CARTESIAN_POINT('Ctrl Pts',(28.787762030239,68.7132793373328,12.));
#104548=CARTESIAN_POINT('Ctrl Pts',(28.8891094745185,68.670819333438,0.));
#104549=CARTESIAN_POINT('Ctrl Pts',(28.8891094745185,68.670819333438,4.));
#104550=CARTESIAN_POINT('Ctrl Pts',(28.8891094745185,68.670819333438,8.));
#104551=CARTESIAN_POINT('Ctrl Pts',(28.8891094745185,68.670819333438,12.));
#104552=CARTESIAN_POINT('Ctrl Pts',(29.0404604348956,68.5360395709812,0.));
#104553=CARTESIAN_POINT('Ctrl Pts',(29.0404604348956,68.5360395709812,4.));
#104554=CARTESIAN_POINT('Ctrl Pts',(29.0404604348956,68.5360395709812,7.99999999999999));
#104555=CARTESIAN_POINT('Ctrl Pts',(29.0404604348956,68.5360395709812,12.));
#104556=CARTESIAN_POINT('Ctrl Pts',(29.0927805237117,68.3446561754308,0.));
#104557=CARTESIAN_POINT('Ctrl Pts',(29.0927805237117,68.3446561754308,4.));
#104558=CARTESIAN_POINT('Ctrl Pts',(29.0927805237117,68.3446561754308,8.00000000000001));
#104559=CARTESIAN_POINT('Ctrl Pts',(29.0927805237117,68.3446561754308,12.));
#104560=CARTESIAN_POINT('Ctrl Pts',(29.0944526440247,68.2622612909745,0.));
#104561=CARTESIAN_POINT('Ctrl Pts',(29.0944526440247,68.2622612909745,4.));
#104562=CARTESIAN_POINT('Ctrl Pts',(29.0944526440247,68.2622612909745,8.));
#104563=CARTESIAN_POINT('Ctrl Pts',(29.0944526440247,68.2622612909745,12.));
#104564=CARTESIAN_POINT('',(28.787762030239,68.7132793373328,0.));
#104565=CARTESIAN_POINT('',(29.0944526440248,68.2622612909745,0.));
#104566=CARTESIAN_POINT('Ctrl Pts',(28.787762030239,68.7132793373328,0.));
#104567=CARTESIAN_POINT('Ctrl Pts',(28.8891094745185,68.670819333438,0.));
#104568=CARTESIAN_POINT('Ctrl Pts',(28.9755957375911,68.5938023263198,0.));
#104569=CARTESIAN_POINT('Ctrl Pts',(29.0297453895418,68.4983025002323,0.));
#104570=CARTESIAN_POINT('Ctrl Pts',(29.0703576285048,68.4266776306667,0.));
#104571=CARTESIAN_POINT('Ctrl Pts',(29.0927805237117,68.3446561754308,0.));
#104572=CARTESIAN_POINT('Ctrl Pts',(29.0944526440247,68.2622612909745,0.));
#104573=CARTESIAN_POINT('',(29.0944526440248,68.2622612909745,12.));
#104574=CARTESIAN_POINT('Ctrl Pts',(29.0944526440247,68.2622612909745,0.));
#104575=CARTESIAN_POINT('Ctrl Pts',(29.0944526440247,68.2622612909745,4.));
#104576=CARTESIAN_POINT('Ctrl Pts',(29.0944526440247,68.2622612909745,8.));
#104577=CARTESIAN_POINT('Ctrl Pts',(29.0944526440247,68.2622612909745,12.));
#104578=CARTESIAN_POINT('',(28.787762030239,68.7132793373328,12.));
#104579=CARTESIAN_POINT('Ctrl Pts',(29.0944526440247,68.2622612909745,12.));
#104580=CARTESIAN_POINT('Ctrl Pts',(29.0927805237117,68.3446561754308,12.));
#104581=CARTESIAN_POINT('Ctrl Pts',(29.0703576285048,68.4266776306667,12.));
#104582=CARTESIAN_POINT('Ctrl Pts',(29.0297453895418,68.4983025002323,12.));
#104583=CARTESIAN_POINT('Ctrl Pts',(28.9755957375911,68.5938023263198,12.));
#104584=CARTESIAN_POINT('Ctrl Pts',(28.8891094745185,68.670819333438,12.));
#104585=CARTESIAN_POINT('Ctrl Pts',(28.787762030239,68.7132793373328,12.));
#104586=CARTESIAN_POINT('Ctrl Pts',(28.787762030239,68.7132793373328,12.));
#104587=CARTESIAN_POINT('Ctrl Pts',(28.787762030239,68.7132793373328,8.));
#104588=CARTESIAN_POINT('Ctrl Pts',(28.787762030239,68.7132793373328,4.));
#104589=CARTESIAN_POINT('Ctrl Pts',(28.787762030239,68.7132793373328,0.));
#104590=CARTESIAN_POINT('Ctrl Pts',(28.8072485549236,63.7976679095314,0.));
#104591=CARTESIAN_POINT('Ctrl Pts',(28.8072485549236,63.7976679095314,12.));
#104592=CARTESIAN_POINT('Ctrl Pts',(28.8078854475432,63.8014989507494,0.));
#104593=CARTESIAN_POINT('Ctrl Pts',(28.8078854475432,63.8014989507494,12.));
#104594=CARTESIAN_POINT('Ctrl Pts',(28.8091580239553,63.8091667271232,0.));
#104595=CARTESIAN_POINT('Ctrl Pts',(28.8091580239553,63.8091667271232,12.));
#104596=CARTESIAN_POINT('Ctrl Pts',(28.8110632620957,63.8206854735028,0.));
#104597=CARTESIAN_POINT('Ctrl Pts',(28.8110632620957,63.8206854735028,12.));
#104598=CARTESIAN_POINT('Ctrl Pts',(28.8135963263368,63.8360779669856,0.));
#104599=CARTESIAN_POINT('Ctrl Pts',(28.8135963263368,63.8360779669856,12.));
#104600=CARTESIAN_POINT('Ctrl Pts',(28.8167505576681,63.8553755207487,0.));
#104601=CARTESIAN_POINT('Ctrl Pts',(28.8167505576681,63.8553755207487,12.));
#104602=CARTESIAN_POINT('Ctrl Pts',(28.8198926619857,63.8747299825313,0.));
#104603=CARTESIAN_POINT('Ctrl Pts',(28.8198926619857,63.8747299825313,12.));
#104604=CARTESIAN_POINT('Ctrl Pts',(28.823022586318,63.8941412856924,0.));
#104605=CARTESIAN_POINT('Ctrl Pts',(28.823022586318,63.8941412856924,12.));
#104606=CARTESIAN_POINT('Ctrl Pts',(28.8261402423291,63.9136093063786,0.));
#104607=CARTESIAN_POINT('Ctrl Pts',(28.8261402423291,63.9136093063786,12.));
#104608=CARTESIAN_POINT('Ctrl Pts',(28.8292455077559,63.9331338646996,0.));
#104609=CARTESIAN_POINT('Ctrl Pts',(28.8292455077559,63.9331338646996,12.));
#104610=CARTESIAN_POINT('Ctrl Pts',(28.8323382413789,63.9527147494423,0.));
#104611=CARTESIAN_POINT('Ctrl Pts',(28.8323382413789,63.9527147494423,12.));
#104612=CARTESIAN_POINT('Ctrl Pts',(28.83541829466,63.9723517369614,0.));
#104613=CARTESIAN_POINT('Ctrl Pts',(28.83541829466,63.9723517369614,12.));
#104614=CARTESIAN_POINT('Ctrl Pts',(28.8384855243242,63.9920446117582,0.));
#104615=CARTESIAN_POINT('Ctrl Pts',(28.8384855243242,63.9920446117582,12.));
#104616=CARTESIAN_POINT('Ctrl Pts',(28.8415398056428,64.0117931881298,0.));
#104617=CARTESIAN_POINT('Ctrl Pts',(28.8415398056428,64.0117931881298,12.));
#104618=CARTESIAN_POINT('Ctrl Pts',(28.844581028125,64.0315973031942,0.));
#104619=CARTESIAN_POINT('Ctrl Pts',(28.844581028125,64.0315973031942,12.));
#104620=CARTESIAN_POINT('Ctrl Pts',(28.8476090892232,64.0514568066637,0.));
#104621=CARTESIAN_POINT('Ctrl Pts',(28.8476090892232,64.0514568066637,12.));
#104622=CARTESIAN_POINT('Ctrl Pts',(28.8506238891092,64.0713715523599,0.));
#104623=CARTESIAN_POINT('Ctrl Pts',(28.8506238891092,64.0713715523599,12.));
#104624=CARTESIAN_POINT('Ctrl Pts',(28.8536253241853,64.0913413876622,0.));
#104625=CARTESIAN_POINT('Ctrl Pts',(28.8536253241853,64.0913413876622,12.));
#104626=CARTESIAN_POINT('Ctrl Pts',(28.8566132838178,64.1113661481965,0.));
#104627=CARTESIAN_POINT('Ctrl Pts',(28.8566132838178,64.1113661481965,12.));
#104628=CARTESIAN_POINT('Ctrl Pts',(28.8595876537148,64.1314456633381,0.));
#104629=CARTESIAN_POINT('Ctrl Pts',(28.8595876537148,64.1314456633381,12.));
#104630=CARTESIAN_POINT('Ctrl Pts',(28.8625483180437,64.1515797596564,0.));
#104631=CARTESIAN_POINT('Ctrl Pts',(28.8625483180437,64.1515797596564,12.));
#104632=CARTESIAN_POINT('Ctrl Pts',(28.8654951618649,64.1717682648685,0.));
#104633=CARTESIAN_POINT('Ctrl Pts',(28.8654951618649,64.1717682648685,12.));
#104634=CARTESIAN_POINT('Ctrl Pts',(28.8684280739014,64.1920110123299,0.));
#104635=CARTESIAN_POINT('Ctrl Pts',(28.8684280739014,64.1920110123299,12.));
#104636=CARTESIAN_POINT('Ctrl Pts',(28.8713469464185,64.2123078408461,0.));
#104637=CARTESIAN_POINT('Ctrl Pts',(28.8713469464185,64.2123078408461,12.));
#104638=CARTESIAN_POINT('Ctrl Pts',(28.8742516738946,64.2326585925252,0.));
#104639=CARTESIAN_POINT('Ctrl Pts',(28.8742516738946,64.2326585925252,12.));
#104640=CARTESIAN_POINT('Ctrl Pts',(28.877142152106,64.2530631112929,0.));
#104641=CARTESIAN_POINT('Ctrl Pts',(28.877142152106,64.2530631112929,12.));
#104642=CARTESIAN_POINT('Ctrl Pts',(28.8800182770064,64.2735212410711,0.));
#104643=CARTESIAN_POINT('Ctrl Pts',(28.8800182770064,64.2735212410711,12.));
#104644=CARTESIAN_POINT('Ctrl Pts',(28.882879943794,64.2940328242521,0.));
#104645=CARTESIAN_POINT('Ctrl Pts',(28.882879943794,64.2940328242521,12.));
#104646=CARTESIAN_POINT('Ctrl Pts',(28.8857270473959,64.3145977025037,0.));
#104647=CARTESIAN_POINT('Ctrl Pts',(28.8857270473959,64.3145977025037,12.));
#104648=CARTESIAN_POINT('Ctrl Pts',(28.8885594828926,64.3352157174619,0.));
#104649=CARTESIAN_POINT('Ctrl Pts',(28.8885594828926,64.3352157174619,12.));
#104650=CARTESIAN_POINT('Ctrl Pts',(28.8913771459323,64.3558867114076,0.));
#104651=CARTESIAN_POINT('Ctrl Pts',(28.8913771459323,64.3558867114076,12.));
#104652=CARTESIAN_POINT('Ctrl Pts',(28.89417993323,64.3766105280688,0.));
#104653=CARTESIAN_POINT('Ctrl Pts',(28.89417993323,64.3766105280688,12.));
#104654=CARTESIAN_POINT('Ctrl Pts',(28.8969677427504,64.397387012917,0.));
#104655=CARTESIAN_POINT('Ctrl Pts',(28.8969677427504,64.397387012917,12.));
#104656=CARTESIAN_POINT('Ctrl Pts',(28.899740473434,64.4182160127379,0.));
#104657=CARTESIAN_POINT('Ctrl Pts',(28.899740473434,64.4182160127379,12.));
#104658=CARTESIAN_POINT('Ctrl Pts',(28.9024980250307,64.4390973753634,0.));
#104659=CARTESIAN_POINT('Ctrl Pts',(28.9024980250307,64.4390973753634,12.));
#104660=CARTESIAN_POINT('Ctrl Pts',(28.9052402979062,64.4600309493583,0.));
#104661=CARTESIAN_POINT('Ctrl Pts',(28.9052402979062,64.4600309493583,12.));
#104662=CARTESIAN_POINT('Ctrl Pts',(28.9079671928264,64.4810165836592,0.));
#104663=CARTESIAN_POINT('Ctrl Pts',(28.9079671928264,64.4810165836592,12.));
#104664=CARTESIAN_POINT('Ctrl Pts',(28.910678610965,64.5020541275951,0.));
#104665=CARTESIAN_POINT('Ctrl Pts',(28.910678610965,64.5020541275951,12.));
#104666=CARTESIAN_POINT('Ctrl Pts',(28.9133744539949,64.523143431047,0.));
#104667=CARTESIAN_POINT('Ctrl Pts',(28.9133744539949,64.523143431047,12.));
#104668=CARTESIAN_POINT('Ctrl Pts',(28.9160546241538,64.5442843445559,0.));
#104669=CARTESIAN_POINT('Ctrl Pts',(28.9160546241538,64.5442843445559,12.));
#104670=CARTESIAN_POINT('Ctrl Pts',(28.9187190243224,64.5654767194472,0.));
#104671=CARTESIAN_POINT('Ctrl Pts',(28.9187190243224,64.5654767194472,12.));
#104672=CARTESIAN_POINT('Ctrl Pts',(28.9213675580985,64.5867204079426,0.));
#104673=CARTESIAN_POINT('Ctrl Pts',(28.9213675580985,64.5867204079426,12.));
#104674=CARTESIAN_POINT('Ctrl Pts',(28.9240001297542,64.6080152631039,0.));
#104675=CARTESIAN_POINT('Ctrl Pts',(28.9240001297542,64.6080152631039,12.));
#104676=CARTESIAN_POINT('Ctrl Pts',(28.926616644195,64.629361138774,0.));
#104677=CARTESIAN_POINT('Ctrl Pts',(28.926616644195,64.629361138774,12.));
#104678=CARTESIAN_POINT('Ctrl Pts',(28.9292170069221,64.6507578895161,0.));
#104679=CARTESIAN_POINT('Ctrl Pts',(28.9292170069221,64.6507578895161,12.));
#104680=CARTESIAN_POINT('Ctrl Pts',(28.9318011239915,64.672205370541,0.));
#104681=CARTESIAN_POINT('Ctrl Pts',(28.9318011239915,64.672205370541,12.));
#104682=CARTESIAN_POINT('Ctrl Pts',(28.9343689019882,64.6937034376617,0.));
#104683=CARTESIAN_POINT('Ctrl Pts',(28.9343689019882,64.6937034376617,12.));
#104684=CARTESIAN_POINT('Ctrl Pts',(28.9369202480392,64.715251947329,0.));
#104685=CARTESIAN_POINT('Ctrl Pts',(28.9369202480392,64.715251947329,12.));
#104686=CARTESIAN_POINT('Ctrl Pts',(28.9394550698204,64.7368507566467,0.));
#104687=CARTESIAN_POINT('Ctrl Pts',(28.9394550698204,64.7368507566467,12.));
#104688=CARTESIAN_POINT('Ctrl Pts',(28.9419732755655,64.758499723388,0.));
#104689=CARTESIAN_POINT('Ctrl Pts',(28.9419732755655,64.758499723388,12.));
#104690=CARTESIAN_POINT('Ctrl Pts',(28.944474774081,64.7801987060084,0.));
#104691=CARTESIAN_POINT('Ctrl Pts',(28.944474774081,64.7801987060084,12.));
#104692=CARTESIAN_POINT('Ctrl Pts',(28.9469594747431,64.8019475636442,0.));
#104693=CARTESIAN_POINT('Ctrl Pts',(28.9469594747431,64.8019475636442,12.));
#104694=CARTESIAN_POINT('Ctrl Pts',(28.9494272874831,64.8237461561019,0.));
#104695=CARTESIAN_POINT('Ctrl Pts',(28.9494272874831,64.8237461561019,12.));
#104696=CARTESIAN_POINT('Ctrl Pts',(28.9518781227765,64.8455943438423,0.));
#104697=CARTESIAN_POINT('Ctrl Pts',(28.9518781227765,64.8455943438423,12.));
#104698=CARTESIAN_POINT('Ctrl Pts',(28.9543118916328,64.8674919879648,0.));
#104699=CARTESIAN_POINT('Ctrl Pts',(28.9543118916328,64.8674919879648,12.));
#104700=CARTESIAN_POINT('Ctrl Pts',(28.9567285055866,64.8894389501801,0.));
#104701=CARTESIAN_POINT('Ctrl Pts',(28.9567285055866,64.8894389501801,12.));
#104702=CARTESIAN_POINT('Ctrl Pts',(28.9591278766934,64.9114350928125,0.));
#104703=CARTESIAN_POINT('Ctrl Pts',(28.9591278766934,64.9114350928125,12.));
#104704=CARTESIAN_POINT('Ctrl Pts',(28.9615099175249,64.9334802788038,0.));
#104705=CARTESIAN_POINT('Ctrl Pts',(28.9615099175249,64.9334802788038,12.));
#104706=CARTESIAN_POINT('Ctrl Pts',(28.9638745411677,64.955574371711,0.));
#104707=CARTESIAN_POINT('Ctrl Pts',(28.9638745411677,64.955574371711,12.));
#104708=CARTESIAN_POINT('Ctrl Pts',(28.9662216612217,64.9777172357027,0.));
#104709=CARTESIAN_POINT('Ctrl Pts',(28.9662216612217,64.9777172357027,12.));
#104710=CARTESIAN_POINT('Ctrl Pts',(28.9685511918018,64.9999087355504,0.));
#104711=CARTESIAN_POINT('Ctrl Pts',(28.9685511918018,64.9999087355504,12.));
#104712=CARTESIAN_POINT('Ctrl Pts',(28.97086304753,65.022148736628,0.));
#104713=CARTESIAN_POINT('Ctrl Pts',(28.97086304753,65.022148736628,12.));
#104714=CARTESIAN_POINT('Ctrl Pts',(28.9731571435282,65.0444371049082,0.));
#104715=CARTESIAN_POINT('Ctrl Pts',(28.9731571435282,65.0444371049082,12.));
#104716=CARTESIAN_POINT('Ctrl Pts',(28.9754333954135,65.0667737069563,0.));
#104717=CARTESIAN_POINT('Ctrl Pts',(28.9754333954135,65.0667737069563,12.));
#104718=CARTESIAN_POINT('Ctrl Pts',(28.9776917192933,65.0891584099168,0.));
#104719=CARTESIAN_POINT('Ctrl Pts',(28.9776917192933,65.0891584099168,12.));
#104720=CARTESIAN_POINT('Ctrl Pts',(28.9799320317641,65.1115910815037,0.));
#104721=CARTESIAN_POINT('Ctrl Pts',(28.9799320317641,65.1115910815037,12.));
#104722=CARTESIAN_POINT('Ctrl Pts',(28.9821542499042,65.1340715900028,0.));
#104723=CARTESIAN_POINT('Ctrl Pts',(28.9821542499042,65.1340715900028,12.));
#104724=CARTESIAN_POINT('Ctrl Pts',(28.9843582912692,65.1565998042697,0.));
#104725=CARTESIAN_POINT('Ctrl Pts',(28.9843582912692,65.1565998042697,12.));
#104726=CARTESIAN_POINT('Ctrl Pts',(28.9865440738883,65.1791755937256,0.));
#104727=CARTESIAN_POINT('Ctrl Pts',(28.9865440738883,65.1791755937256,12.));
#104728=CARTESIAN_POINT('Ctrl Pts',(28.9887115162633,65.2017988283479,0.));
#104729=CARTESIAN_POINT('Ctrl Pts',(28.9887115162633,65.2017988283479,12.));
#104730=CARTESIAN_POINT('Ctrl Pts',(28.9908605373663,65.2244693786609,0.));
#104731=CARTESIAN_POINT('Ctrl Pts',(28.9908605373663,65.2244693786609,12.));
#104732=CARTESIAN_POINT('Ctrl Pts',(28.9929910566325,65.2471871157397,0.));
#104733=CARTESIAN_POINT('Ctrl Pts',(28.9929910566325,65.2471871157397,12.));
#104734=CARTESIAN_POINT('Ctrl Pts',(28.9951029939557,65.2699519112064,0.));
#104735=CARTESIAN_POINT('Ctrl Pts',(28.9951029939557,65.2699519112064,12.));
#104736=CARTESIAN_POINT('Ctrl Pts',(28.9971962696845,65.2927636372254,0.));
#104737=CARTESIAN_POINT('Ctrl Pts',(28.9971962696845,65.2927636372254,12.));
#104738=CARTESIAN_POINT('Ctrl Pts',(28.9992708046211,65.3156221664916,0.));
#104739=CARTESIAN_POINT('Ctrl Pts',(28.9992708046211,65.3156221664916,12.));
#104740=CARTESIAN_POINT('Ctrl Pts',(29.0013265200185,65.3385273722241,0.));
#104741=CARTESIAN_POINT('Ctrl Pts',(29.0013265200185,65.3385273722241,12.));
#104742=CARTESIAN_POINT('Ctrl Pts',(29.003363337573,65.3614791281692,0.));
#104743=CARTESIAN_POINT('Ctrl Pts',(29.003363337573,65.3614791281692,12.));
#104744=CARTESIAN_POINT('Ctrl Pts',(29.0053811794207,65.3844773085961,0.));
#104745=CARTESIAN_POINT('Ctrl Pts',(29.0053811794207,65.3844773085961,12.));
#104746=CARTESIAN_POINT('Ctrl Pts',(29.0073799681342,65.4075217882934,0.));
#104747=CARTESIAN_POINT('Ctrl Pts',(29.0073799681342,65.4075217882934,12.));
#104748=CARTESIAN_POINT('Ctrl Pts',(29.0093596267215,65.4306124425562,0.));
#104749=CARTESIAN_POINT('Ctrl Pts',(29.0093596267215,65.4306124425562,12.));
#104750=CARTESIAN_POINT('Ctrl Pts',(29.0113200786239,65.4537491471828,0.));
#104751=CARTESIAN_POINT('Ctrl Pts',(29.0113200786239,65.4537491471828,12.));
#104752=CARTESIAN_POINT('Ctrl Pts',(29.013261247709,65.4769317784789,0.));
#104753=CARTESIAN_POINT('Ctrl Pts',(29.013261247709,65.4769317784789,12.));
#104754=CARTESIAN_POINT('Ctrl Pts',(29.0151830582675,65.5001602132535,0.));
#104755=CARTESIAN_POINT('Ctrl Pts',(29.0151830582675,65.5001602132535,12.));
#104756=CARTESIAN_POINT('Ctrl Pts',(29.0170854350095,65.5234343288136,0.));
#104757=CARTESIAN_POINT('Ctrl Pts',(29.0170854350095,65.5234343288136,12.));
#104758=CARTESIAN_POINT('Ctrl Pts',(29.0189683030642,65.5467540029514,0.));
#104759=CARTESIAN_POINT('Ctrl Pts',(29.0189683030642,65.5467540029514,12.));
#104760=CARTESIAN_POINT('Ctrl Pts',(29.0208315879764,65.5701191139418,0.));
#104761=CARTESIAN_POINT('Ctrl Pts',(29.0208315879764,65.5701191139418,12.));
#104762=CARTESIAN_POINT('Ctrl Pts',(29.0226752157003,65.5935295405453,0.));
#104763=CARTESIAN_POINT('Ctrl Pts',(29.0226752157003,65.5935295405453,12.));
#104764=CARTESIAN_POINT('Ctrl Pts',(29.0244991125958,65.6169851620046,0.));
#104765=CARTESIAN_POINT('Ctrl Pts',(29.0244991125958,65.6169851620046,12.));
#104766=CARTESIAN_POINT('Ctrl Pts',(29.0263032054266,65.6404858580403,0.));
#104767=CARTESIAN_POINT('Ctrl Pts',(29.0263032054266,65.6404858580403,12.));
#104768=CARTESIAN_POINT('Ctrl Pts',(29.0280874213596,65.6640315088388,0.));
#104769=CARTESIAN_POINT('Ctrl Pts',(29.0280874213596,65.6640315088388,12.));
#104770=CARTESIAN_POINT('Ctrl Pts',(29.0298516879611,65.6876219950493,0.));
#104771=CARTESIAN_POINT('Ctrl Pts',(29.0298516879611,65.6876219950493,12.));
#104772=CARTESIAN_POINT('Ctrl Pts',(29.0315959331919,65.7112571977891,0.));
#104773=CARTESIAN_POINT('Ctrl Pts',(29.0315959331919,65.7112571977891,12.));
#104774=CARTESIAN_POINT('Ctrl Pts',(29.0333200854027,65.7349369986384,0.));
#104775=CARTESIAN_POINT('Ctrl Pts',(29.0333200854027,65.7349369986384,12.));
#104776=CARTESIAN_POINT('Ctrl Pts',(29.035024073333,65.7586612796368,0.));
#104777=CARTESIAN_POINT('Ctrl Pts',(29.035024073333,65.7586612796368,12.));
#104778=CARTESIAN_POINT('Ctrl Pts',(29.0367078261102,65.7824299232705,0.));
#104779=CARTESIAN_POINT('Ctrl Pts',(29.0367078261102,65.7824299232705,12.));
#104780=CARTESIAN_POINT('Ctrl Pts',(29.0383712732469,65.8062428124713,0.));
#104781=CARTESIAN_POINT('Ctrl Pts',(29.0383712732469,65.8062428124713,12.));
#104782=CARTESIAN_POINT('Ctrl Pts',(29.0400143446338,65.8300998306191,0.));
#104783=CARTESIAN_POINT('Ctrl Pts',(29.0400143446338,65.8300998306191,12.));
#104784=CARTESIAN_POINT('Ctrl Pts',(29.0416369705375,65.854000861539,0.));
#104785=CARTESIAN_POINT('Ctrl Pts',(29.0416369705375,65.854000861539,12.));
#104786=CARTESIAN_POINT('Ctrl Pts',(29.0432390815977,65.8779457894961,0.));
#104787=CARTESIAN_POINT('Ctrl Pts',(29.0432390815977,65.8779457894961,12.));
#104788=CARTESIAN_POINT('Ctrl Pts',(29.0448206088288,65.9019344991854,0.));
#104789=CARTESIAN_POINT('Ctrl Pts',(29.0448206088288,65.9019344991854,12.));
#104790=CARTESIAN_POINT('Ctrl Pts',(29.0463814836157,65.9259668757307,0.));
#104791=CARTESIAN_POINT('Ctrl Pts',(29.0463814836157,65.9259668757307,12.));
#104792=CARTESIAN_POINT('Ctrl Pts',(29.0479216377081,65.9500428046868,0.));
#104793=CARTESIAN_POINT('Ctrl Pts',(29.0479216377081,65.9500428046868,12.));
#104794=CARTESIAN_POINT('Ctrl Pts',(29.0494410032172,65.974162172037,0.));
#104795=CARTESIAN_POINT('Ctrl Pts',(29.0494410032172,65.974162172037,12.));
#104796=CARTESIAN_POINT('Ctrl Pts',(29.0509395126142,65.9983248641879,0.));
#104797=CARTESIAN_POINT('Ctrl Pts',(29.0509395126142,65.9983248641879,12.));
#104798=CARTESIAN_POINT('Ctrl Pts',(29.0524170987307,66.0225307679591,0.));
#104799=CARTESIAN_POINT('Ctrl Pts',(29.0524170987307,66.0225307679591,12.));
#104800=CARTESIAN_POINT('Ctrl Pts',(29.0538736947552,66.0467797705815,0.));
#104801=CARTESIAN_POINT('Ctrl Pts',(29.0538736947552,66.0467797705815,12.));
#104802=CARTESIAN_POINT('Ctrl Pts',(29.0553092342278,66.0710717597009,0.));
#104803=CARTESIAN_POINT('Ctrl Pts',(29.0553092342278,66.0710717597009,12.));
#104804=CARTESIAN_POINT('Ctrl Pts',(29.0567236510373,66.0954066233754,0.));
#104805=CARTESIAN_POINT('Ctrl Pts',(29.0567236510373,66.0954066233754,12.));
#104806=CARTESIAN_POINT('Ctrl Pts',(29.0581168794189,66.1197842500711,0.));
#104807=CARTESIAN_POINT('Ctrl Pts',(29.0581168794189,66.1197842500711,12.));
#104808=CARTESIAN_POINT('Ctrl Pts',(29.0594888539555,66.1442045286516,0.));
#104809=CARTESIAN_POINT('Ctrl Pts',(29.0594888539555,66.1442045286516,12.));
#104810=CARTESIAN_POINT('Ctrl Pts',(29.0608395095745,66.1686673483755,0.));
#104811=CARTESIAN_POINT('Ctrl Pts',(29.0608395095745,66.1686673483755,12.));
#104812=CARTESIAN_POINT('Ctrl Pts',(29.062168781542,66.1931725989008,0.));
#104813=CARTESIAN_POINT('Ctrl Pts',(29.062168781542,66.1931725989008,12.));
#104814=CARTESIAN_POINT('Ctrl Pts',(29.0634766054599,66.2177201702819,0.));
#104815=CARTESIAN_POINT('Ctrl Pts',(29.0634766054599,66.2177201702819,12.));
#104816=CARTESIAN_POINT('Ctrl Pts',(29.0647629172645,66.2423099529668,0.));
#104817=CARTESIAN_POINT('Ctrl Pts',(29.0647629172645,66.2423099529668,12.));
#104818=CARTESIAN_POINT('Ctrl Pts',(29.0660276532272,66.2669418377866,0.));
#104819=CARTESIAN_POINT('Ctrl Pts',(29.0660276532272,66.2669418377866,12.));
#104820=CARTESIAN_POINT('Ctrl Pts',(29.0672707499527,66.2916157159528,0.));
#104821=CARTESIAN_POINT('Ctrl Pts',(29.0672707499527,66.2916157159528,12.));
#104822=CARTESIAN_POINT('Ctrl Pts',(29.0684921443718,66.3163314790607,0.));
#104823=CARTESIAN_POINT('Ctrl Pts',(29.0684921443718,66.3163314790607,12.));
#104824=CARTESIAN_POINT('Ctrl Pts',(29.0696917737397,66.3410890190879,0.));
#104825=CARTESIAN_POINT('Ctrl Pts',(29.0696917737397,66.3410890190879,12.));
#104826=CARTESIAN_POINT('Ctrl Pts',(29.0708695756335,66.3658882283906,0.));
#104827=CARTESIAN_POINT('Ctrl Pts',(29.0708695756335,66.3658882283906,12.));
#104828=CARTESIAN_POINT('Ctrl Pts',(29.0720254879535,66.3907289996942,0.));
#104829=CARTESIAN_POINT('Ctrl Pts',(29.0720254879535,66.3907289996942,12.));
#104830=CARTESIAN_POINT('Ctrl Pts',(29.0731594489218,66.4156112260904,0.));
#104831=CARTESIAN_POINT('Ctrl Pts',(29.0731594489218,66.4156112260904,12.));
#104832=CARTESIAN_POINT('Ctrl Pts',(29.0742713970762,66.4405348010404,0.));
#104833=CARTESIAN_POINT('Ctrl Pts',(29.0742713970762,66.4405348010404,12.));
#104834=CARTESIAN_POINT('Ctrl Pts',(29.0753612712669,66.4654996183739,0.));
#104835=CARTESIAN_POINT('Ctrl Pts',(29.0753612712669,66.4654996183739,12.));
#104836=CARTESIAN_POINT('Ctrl Pts',(29.0764290106553,66.4905055722864,0.));
#104837=CARTESIAN_POINT('Ctrl Pts',(29.0764290106553,66.4905055722864,12.));
#104838=CARTESIAN_POINT('Ctrl Pts',(29.0774745547146,66.5155525573308,0.));
#104839=CARTESIAN_POINT('Ctrl Pts',(29.0774745547146,66.5155525573308,12.));
#104840=CARTESIAN_POINT('Ctrl Pts',(29.0784978432294,66.5406404684116,0.));
#104841=CARTESIAN_POINT('Ctrl Pts',(29.0784978432294,66.5406404684116,12.));
#104842=CARTESIAN_POINT('Ctrl Pts',(29.0794988162892,66.5657692007894,0.));
#104843=CARTESIAN_POINT('Ctrl Pts',(29.0794988162892,66.5657692007894,12.));
#104844=CARTESIAN_POINT('Ctrl Pts',(29.0804774142852,66.5909386500796,0.));
#104845=CARTESIAN_POINT('Ctrl Pts',(29.0804774142852,66.5909386500796,12.));
#104846=CARTESIAN_POINT('Ctrl Pts',(29.0814335779085,66.6161487122504,0.));
#104847=CARTESIAN_POINT('Ctrl Pts',(29.0814335779085,66.6161487122504,12.));
#104848=CARTESIAN_POINT('Ctrl Pts',(29.0823672481508,66.6413992836148,0.));
#104849=CARTESIAN_POINT('Ctrl Pts',(29.0823672481508,66.6413992836148,12.));
#104850=CARTESIAN_POINT('Ctrl Pts',(29.0832783663048,66.6666902608246,0.));
#104851=CARTESIAN_POINT('Ctrl Pts',(29.0832783663048,66.6666902608246,12.));
#104852=CARTESIAN_POINT('Ctrl Pts',(29.0841668739585,66.6920215408744,0.));
#104853=CARTESIAN_POINT('Ctrl Pts',(29.0841668739585,66.6920215408744,12.));
#104854=CARTESIAN_POINT('Ctrl Pts',(29.0850327129913,66.7173930211015,0.));
#104855=CARTESIAN_POINT('Ctrl Pts',(29.0850327129913,66.7173930211015,12.));
#104856=CARTESIAN_POINT('Ctrl Pts',(29.0858758255729,66.7428045991841,0.));
#104857=CARTESIAN_POINT('Ctrl Pts',(29.0858758255729,66.7428045991841,12.));
#104858=CARTESIAN_POINT('Ctrl Pts',(29.0866961541629,66.7682561731349,0.));
#104859=CARTESIAN_POINT('Ctrl Pts',(29.0866961541629,66.7682561731349,12.));
#104860=CARTESIAN_POINT('Ctrl Pts',(29.0874936415137,66.7937476412941,0.));
#104861=CARTESIAN_POINT('Ctrl Pts',(29.0874936415137,66.7937476412941,12.));
#104862=CARTESIAN_POINT('Ctrl Pts',(29.0882682306636,66.8192789023323,0.));
#104863=CARTESIAN_POINT('Ctrl Pts',(29.0882682306636,66.8192789023323,12.));
#104864=CARTESIAN_POINT('Ctrl Pts',(29.0890198649327,66.8448498552508,0.));
#104865=CARTESIAN_POINT('Ctrl Pts',(29.0890198649327,66.8448498552508,12.));
#104866=CARTESIAN_POINT('Ctrl Pts',(29.0897484879207,66.8704603993794,0.));
#104867=CARTESIAN_POINT('Ctrl Pts',(29.0897484879207,66.8704603993794,12.));
#104868=CARTESIAN_POINT('Ctrl Pts',(29.0904540435063,66.8961104343703,0.));
#104869=CARTESIAN_POINT('Ctrl Pts',(29.0904540435063,66.8961104343703,12.));
#104870=CARTESIAN_POINT('Ctrl Pts',(29.0911364758484,66.9217998601881,0.));
#104871=CARTESIAN_POINT('Ctrl Pts',(29.0911364758484,66.9217998601881,12.));
#104872=CARTESIAN_POINT('Ctrl Pts',(29.0917957293824,66.9475285771133,0.));
#104873=CARTESIAN_POINT('Ctrl Pts',(29.0917957293824,66.9475285771133,12.));
#104874=CARTESIAN_POINT('Ctrl Pts',(29.092431748817,66.9732964857467,0.));
#104875=CARTESIAN_POINT('Ctrl Pts',(29.092431748817,66.9732964857467,12.));
#104876=CARTESIAN_POINT('Ctrl Pts',(29.0930444791328,66.9991034870084,0.));
#104877=CARTESIAN_POINT('Ctrl Pts',(29.0930444791328,66.9991034870084,12.));
#104878=CARTESIAN_POINT('Ctrl Pts',(29.0936338655828,67.0249494821361,0.));
#104879=CARTESIAN_POINT('Ctrl Pts',(29.0936338655828,67.0249494821361,12.));
#104880=CARTESIAN_POINT('Ctrl Pts',(29.0941998536957,67.0508343726771,0.));
#104881=CARTESIAN_POINT('Ctrl Pts',(29.0941998536957,67.0508343726771,12.));
#104882=CARTESIAN_POINT('Ctrl Pts',(29.0947423892725,67.0767580604872,0.));
#104883=CARTESIAN_POINT('Ctrl Pts',(29.0947423892725,67.0767580604872,12.));
#104884=CARTESIAN_POINT('Ctrl Pts',(29.0952614183777,67.1027204477304,0.));
#104885=CARTESIAN_POINT('Ctrl Pts',(29.0952614183777,67.1027204477304,12.));
#104886=CARTESIAN_POINT('Ctrl Pts',(29.0957568873357,67.1287214368743,0.));
#104887=CARTESIAN_POINT('Ctrl Pts',(29.0957568873357,67.1287214368743,12.));
#104888=CARTESIAN_POINT('Ctrl Pts',(29.0962287427274,67.1547609306845,0.));
#104889=CARTESIAN_POINT('Ctrl Pts',(29.0962287427274,67.1547609306845,12.));
#104890=CARTESIAN_POINT('Ctrl Pts',(29.0966769313893,67.1808388322116,0.));
#104891=CARTESIAN_POINT('Ctrl Pts',(29.0966769313893,67.1808388322116,12.));
#104892=CARTESIAN_POINT('Ctrl Pts',(29.0971014004134,67.2069550447895,0.));
#104893=CARTESIAN_POINT('Ctrl Pts',(29.0971014004134,67.2069550447895,12.));
#104894=CARTESIAN_POINT('Ctrl Pts',(29.0975020971473,67.2331094720482,0.));
#104895=CARTESIAN_POINT('Ctrl Pts',(29.0975020971473,67.2331094720482,12.));
#104896=CARTESIAN_POINT('Ctrl Pts',(29.0978789691964,67.2593020179216,0.));
#104897=CARTESIAN_POINT('Ctrl Pts',(29.0978789691964,67.2593020179216,12.));
#104898=CARTESIAN_POINT('Ctrl Pts',(29.0982319644276,67.2855325866516,0.));
#104899=CARTESIAN_POINT('Ctrl Pts',(29.0982319644276,67.2855325866516,12.));
#104900=CARTESIAN_POINT('Ctrl Pts',(29.0985610309768,67.311801082791,0.));
#104901=CARTESIAN_POINT('Ctrl Pts',(29.0985610309768,67.311801082791,12.));
#104902=CARTESIAN_POINT('Ctrl Pts',(29.0988661172526,67.3381074112013,0.));
#104903=CARTESIAN_POINT('Ctrl Pts',(29.0988661172526,67.3381074112013,12.));
#104904=CARTESIAN_POINT('Ctrl Pts',(29.0991471719172,67.3644514770373,0.));
#104905=CARTESIAN_POINT('Ctrl Pts',(29.0991471719172,67.3644514770373,12.));
#104906=CARTESIAN_POINT('Ctrl Pts',(29.0994041438715,67.3908331857313,0.));
#104907=CARTESIAN_POINT('Ctrl Pts',(29.0994041438715,67.3908331857313,12.));
#104908=CARTESIAN_POINT('Ctrl Pts',(29.0996369822418,67.4172524429726,0.));
#104909=CARTESIAN_POINT('Ctrl Pts',(29.0996369822418,67.4172524429726,12.));
#104910=CARTESIAN_POINT('Ctrl Pts',(29.0998456363687,67.4437091546869,0.));
#104911=CARTESIAN_POINT('Ctrl Pts',(29.0998456363687,67.4437091546869,12.));
#104912=CARTESIAN_POINT('Ctrl Pts',(29.1000300557961,67.4702032270063,0.));
#104913=CARTESIAN_POINT('Ctrl Pts',(29.1000300557961,67.4702032270063,12.));
#104914=CARTESIAN_POINT('Ctrl Pts',(29.1001901902914,67.496734566311,0.));
#104915=CARTESIAN_POINT('Ctrl Pts',(29.1001901902914,67.496734566311,12.));
#104916=CARTESIAN_POINT('Ctrl Pts',(29.1003259898686,67.5233030792714,0.));
#104917=CARTESIAN_POINT('Ctrl Pts',(29.1003259898686,67.5233030792714,12.));
#104918=CARTESIAN_POINT('Ctrl Pts',(29.1004374048149,67.5499086728891,0.));
#104919=CARTESIAN_POINT('Ctrl Pts',(29.1004374048149,67.5499086728891,12.));
#104920=CARTESIAN_POINT('Ctrl Pts',(29.1005243857137,67.5765512545276,0.));
#104921=CARTESIAN_POINT('Ctrl Pts',(29.1005243857137,67.5765512545276,12.));
#104922=CARTESIAN_POINT('Ctrl Pts',(29.1005868834863,67.6032307319614,0.));
#104923=CARTESIAN_POINT('Ctrl Pts',(29.1005868834863,67.6032307319614,12.));
#104924=CARTESIAN_POINT('Ctrl Pts',(29.1006248493576,67.6299470133286,0.));
#104925=CARTESIAN_POINT('Ctrl Pts',(29.1006248493576,67.6299470133286,12.));
#104926=CARTESIAN_POINT('Ctrl Pts',(29.1006382347811,67.6567000070319,0.));
#104927=CARTESIAN_POINT('Ctrl Pts',(29.1006382347811,67.6567000070319,12.));
#104928=CARTESIAN_POINT('Ctrl Pts',(29.1006269913746,67.6834896216458,0.));
#104929=CARTESIAN_POINT('Ctrl Pts',(29.1006269913746,67.6834896216458,12.));
#104930=CARTESIAN_POINT('Ctrl Pts',(29.1005910708624,67.7103157658297,0.));
#104931=CARTESIAN_POINT('Ctrl Pts',(29.1005910708624,67.7103157658297,12.));
#104932=CARTESIAN_POINT('Ctrl Pts',(29.1005304249988,67.7371783482039,0.));
#104933=CARTESIAN_POINT('Ctrl Pts',(29.1005304249988,67.7371783482039,12.));
#104934=CARTESIAN_POINT('Ctrl Pts',(29.1004450055647,67.7640772773397,0.));
#104935=CARTESIAN_POINT('Ctrl Pts',(29.1004450055647,67.7640772773397,12.));
#104936=CARTESIAN_POINT('Ctrl Pts',(29.1003347645299,67.7910124620148,0.));
#104937=CARTESIAN_POINT('Ctrl Pts',(29.1003347645299,67.7910124620148,12.));
#104938=CARTESIAN_POINT('Ctrl Pts',(29.1001996541846,67.8179838114109,0.));
#104939=CARTESIAN_POINT('Ctrl Pts',(29.1001996541846,67.8179838114109,12.));
#104940=CARTESIAN_POINT('Ctrl Pts',(29.1000396272868,67.844991235333,0.));
#104941=CARTESIAN_POINT('Ctrl Pts',(29.1000396272868,67.844991235333,12.));
#104942=CARTESIAN_POINT('Ctrl Pts',(29.0998546372027,67.8720346444111,0.));
#104943=CARTESIAN_POINT('Ctrl Pts',(29.0998546372027,67.8720346444111,12.));
#104944=CARTESIAN_POINT('Ctrl Pts',(29.0996446380617,67.8991139503168,0.));
#104945=CARTESIAN_POINT('Ctrl Pts',(29.0996446380617,67.8991139503168,12.));
#104946=CARTESIAN_POINT('Ctrl Pts',(29.0994095844208,67.9262290652797,0.));
#104947=CARTESIAN_POINT('Ctrl Pts',(29.0994095844208,67.9262290652797,12.));
#104948=CARTESIAN_POINT('Ctrl Pts',(29.0991494309394,67.9533799016122,0.));
#104949=CARTESIAN_POINT('Ctrl Pts',(29.0991494309394,67.9533799016122,12.));
#104950=CARTESIAN_POINT('Ctrl Pts',(29.0988641320243,67.9805663711845,0.));
#104951=CARTESIAN_POINT('Ctrl Pts',(29.0988641320243,67.9805663711845,12.));
#104952=CARTESIAN_POINT('Ctrl Pts',(29.0985536415537,68.0077883850136,0.));
#104953=CARTESIAN_POINT('Ctrl Pts',(29.0985536415537,68.0077883850136,12.));
#104954=CARTESIAN_POINT('Ctrl Pts',(29.0982179124112,68.0350458525589,0.));
#104955=CARTESIAN_POINT('Ctrl Pts',(29.0982179124112,68.0350458525589,12.));
#104956=CARTESIAN_POINT('Ctrl Pts',(29.0978568968677,68.0623386822917,0.));
#104957=CARTESIAN_POINT('Ctrl Pts',(29.0978568968677,68.0623386822917,12.));
#104958=CARTESIAN_POINT('Ctrl Pts',(29.0974705474279,68.089666782962,0.));
#104959=CARTESIAN_POINT('Ctrl Pts',(29.0974705474279,68.089666782962,12.));
#104960=CARTESIAN_POINT('Ctrl Pts',(29.097058817574,68.1170300647019,0.));
#104961=CARTESIAN_POINT('Ctrl Pts',(29.097058817574,68.1170300647019,12.));
#104962=CARTESIAN_POINT('Ctrl Pts',(29.096621662474,68.1444284400734,0.));
#104963=CARTESIAN_POINT('Ctrl Pts',(29.096621662474,68.1444284400734,12.));
#104964=CARTESIAN_POINT('Ctrl Pts',(29.0961590399023,68.1718618254221,0.));
#104965=CARTESIAN_POINT('Ctrl Pts',(29.0961590399023,68.1718618254221,12.));
#104966=CARTESIAN_POINT('Ctrl Pts',(29.0956709104588,68.1993301411959,0.));
#104967=CARTESIAN_POINT('Ctrl Pts',(29.0956709104588,68.1993301411959,12.));
#104968=CARTESIAN_POINT('Ctrl Pts',(29.0951572355352,68.22683330895,0.));
#104969=CARTESIAN_POINT('Ctrl Pts',(29.0951572355352,68.22683330895,12.));
#104970=CARTESIAN_POINT('Ctrl Pts',(29.0946179757132,68.2543712489815,0.));
#104971=CARTESIAN_POINT('Ctrl Pts',(29.0946179757132,68.2543712489815,12.));
#104972=CARTESIAN_POINT('Ctrl Pts',(29.0940530889141,68.2819438775932,0.));
#104973=CARTESIAN_POINT('Ctrl Pts',(29.0940530889141,68.2819438775932,12.));
#104974=CARTESIAN_POINT('Ctrl Pts',(29.0934625288442,68.3095511047852,0.));
#104975=CARTESIAN_POINT('Ctrl Pts',(29.0934625288442,68.3095511047852,12.));
#104976=CARTESIAN_POINT('Ctrl Pts',(29.0928462428218,68.3371928310351,0.));
#104977=CARTESIAN_POINT('Ctrl Pts',(29.0928462428218,68.3371928310351,12.));
#104978=CARTESIAN_POINT('Ctrl Pts',(29.0922041749393,68.3648689519188,0.));
#104979=CARTESIAN_POINT('Ctrl Pts',(29.0922041749393,68.3648689519188,12.));
#104980=CARTESIAN_POINT('Ctrl Pts',(29.0915362699549,68.3925793638241,0.));
#104981=CARTESIAN_POINT('Ctrl Pts',(29.0915362699549,68.3925793638241,12.));
#104982=CARTESIAN_POINT('Ctrl Pts',(29.0908424770941,68.4203239694742,0.));
#104983=CARTESIAN_POINT('Ctrl Pts',(29.0908424770941,68.4203239694742,12.));
#104984=CARTESIAN_POINT('Ctrl Pts',(29.0901227535274,68.4481026830845,0.));
#104985=CARTESIAN_POINT('Ctrl Pts',(29.0901227535274,68.4481026830845,12.));
#104986=CARTESIAN_POINT('Ctrl Pts',(29.0893770688807,68.4759154367582,0.));
#104987=CARTESIAN_POINT('Ctrl Pts',(29.0893770688807,68.4759154367582,12.));
#104988=CARTESIAN_POINT('Ctrl Pts',(29.0886054060334,68.5037621823575,0.));
#104989=CARTESIAN_POINT('Ctrl Pts',(29.0886054060334,68.5037621823575,12.));
#104990=CARTESIAN_POINT('Ctrl Pts',(29.0878077570819,68.5316428874729,0.));
#104991=CARTESIAN_POINT('Ctrl Pts',(29.0878077570819,68.5316428874729,12.));
#104992=CARTESIAN_POINT('Ctrl Pts',(29.0871488478365,68.5539746037961,0.));
#104993=CARTESIAN_POINT('Ctrl Pts',(29.0871488478365,68.5539746037961,12.));
#104994=CARTESIAN_POINT('Ctrl Pts',(29.0866429721958,68.5707386600286,0.));
#104995=CARTESIAN_POINT('Ctrl Pts',(29.0866429721958,68.5707386600286,12.));
#104996=CARTESIAN_POINT('Ctrl Pts',(29.0863005247789,68.5819214834609,0.));
#104997=CARTESIAN_POINT('Ctrl Pts',(29.0863005247789,68.5819214834609,12.));
#104998=CARTESIAN_POINT('Ctrl Pts',(29.0861280018229,68.5875145916629,0.));
#104999=CARTESIAN_POINT('Ctrl Pts',(29.0861280018229,68.5875145916629,12.));
#105000=CARTESIAN_POINT('',(28.8072485549236,63.7976679095314,0.));
#105001=CARTESIAN_POINT('Ctrl Pts',(28.8072485549236,63.7976679095314,0.));
#105002=CARTESIAN_POINT('Ctrl Pts',(28.8078854475432,63.8014989507494,0.));
#105003=CARTESIAN_POINT('Ctrl Pts',(28.8091580239553,63.8091667271232,0.));
#105004=CARTESIAN_POINT('Ctrl Pts',(28.8110632620957,63.8206854735028,0.));
#105005=CARTESIAN_POINT('Ctrl Pts',(28.8135963263368,63.8360779669856,0.));
#105006=CARTESIAN_POINT('Ctrl Pts',(28.8167505576681,63.8553755207487,0.));
#105007=CARTESIAN_POINT('Ctrl Pts',(28.8198926619857,63.8747299825313,0.));
#105008=CARTESIAN_POINT('Ctrl Pts',(28.823022586318,63.8941412856924,0.));
#105009=CARTESIAN_POINT('Ctrl Pts',(28.8261402423291,63.9136093063786,0.));
#105010=CARTESIAN_POINT('Ctrl Pts',(28.8292455077559,63.9331338646996,0.));
#105011=CARTESIAN_POINT('Ctrl Pts',(28.8323382413789,63.9527147494423,0.));
#105012=CARTESIAN_POINT('Ctrl Pts',(28.83541829466,63.9723517369614,0.));
#105013=CARTESIAN_POINT('Ctrl Pts',(28.8384855243242,63.9920446117582,0.));
#105014=CARTESIAN_POINT('Ctrl Pts',(28.8415398056428,64.0117931881298,0.));
#105015=CARTESIAN_POINT('Ctrl Pts',(28.844581028125,64.0315973031942,0.));
#105016=CARTESIAN_POINT('Ctrl Pts',(28.8476090892232,64.0514568066637,0.));
#105017=CARTESIAN_POINT('Ctrl Pts',(28.8506238891092,64.0713715523599,0.));
#105018=CARTESIAN_POINT('Ctrl Pts',(28.8536253241853,64.0913413876622,0.));
#105019=CARTESIAN_POINT('Ctrl Pts',(28.8566132838178,64.1113661481965,0.));
#105020=CARTESIAN_POINT('Ctrl Pts',(28.8595876537148,64.1314456633381,0.));
#105021=CARTESIAN_POINT('Ctrl Pts',(28.8625483180437,64.1515797596564,0.));
#105022=CARTESIAN_POINT('Ctrl Pts',(28.8654951618649,64.1717682648685,0.));
#105023=CARTESIAN_POINT('Ctrl Pts',(28.8684280739014,64.1920110123299,0.));
#105024=CARTESIAN_POINT('Ctrl Pts',(28.8713469464185,64.2123078408461,0.));
#105025=CARTESIAN_POINT('Ctrl Pts',(28.8742516738946,64.2326585925252,0.));
#105026=CARTESIAN_POINT('Ctrl Pts',(28.877142152106,64.2530631112929,0.));
#105027=CARTESIAN_POINT('Ctrl Pts',(28.8800182770064,64.2735212410711,0.));
#105028=CARTESIAN_POINT('Ctrl Pts',(28.882879943794,64.2940328242521,0.));
#105029=CARTESIAN_POINT('Ctrl Pts',(28.8857270473959,64.3145977025037,0.));
#105030=CARTESIAN_POINT('Ctrl Pts',(28.8885594828926,64.3352157174619,0.));
#105031=CARTESIAN_POINT('Ctrl Pts',(28.8913771459323,64.3558867114076,0.));
#105032=CARTESIAN_POINT('Ctrl Pts',(28.89417993323,64.3766105280688,0.));
#105033=CARTESIAN_POINT('Ctrl Pts',(28.8969677427504,64.397387012917,0.));
#105034=CARTESIAN_POINT('Ctrl Pts',(28.899740473434,64.4182160127379,0.));
#105035=CARTESIAN_POINT('Ctrl Pts',(28.9024980250307,64.4390973753634,0.));
#105036=CARTESIAN_POINT('Ctrl Pts',(28.9052402979062,64.4600309493583,0.));
#105037=CARTESIAN_POINT('Ctrl Pts',(28.9079671928264,64.4810165836592,0.));
#105038=CARTESIAN_POINT('Ctrl Pts',(28.910678610965,64.5020541275951,0.));
#105039=CARTESIAN_POINT('Ctrl Pts',(28.9133744539949,64.523143431047,0.));
#105040=CARTESIAN_POINT('Ctrl Pts',(28.9160546241538,64.5442843445559,0.));
#105041=CARTESIAN_POINT('Ctrl Pts',(28.9187190243224,64.5654767194472,0.));
#105042=CARTESIAN_POINT('Ctrl Pts',(28.9213675580985,64.5867204079426,0.));
#105043=CARTESIAN_POINT('Ctrl Pts',(28.9240001297542,64.6080152631039,0.));
#105044=CARTESIAN_POINT('Ctrl Pts',(28.926616644195,64.629361138774,0.));
#105045=CARTESIAN_POINT('Ctrl Pts',(28.9292170069221,64.6507578895161,0.));
#105046=CARTESIAN_POINT('Ctrl Pts',(28.9318011239915,64.672205370541,0.));
#105047=CARTESIAN_POINT('Ctrl Pts',(28.9343689019882,64.6937034376617,0.));
#105048=CARTESIAN_POINT('Ctrl Pts',(28.9369202480392,64.715251947329,0.));
#105049=CARTESIAN_POINT('Ctrl Pts',(28.9394550698204,64.7368507566467,0.));
#105050=CARTESIAN_POINT('Ctrl Pts',(28.9419732755655,64.758499723388,0.));
#105051=CARTESIAN_POINT('Ctrl Pts',(28.944474774081,64.7801987060084,0.));
#105052=CARTESIAN_POINT('Ctrl Pts',(28.9469594747431,64.8019475636442,0.));
#105053=CARTESIAN_POINT('Ctrl Pts',(28.9494272874831,64.8237461561019,0.));
#105054=CARTESIAN_POINT('Ctrl Pts',(28.9518781227765,64.8455943438423,0.));
#105055=CARTESIAN_POINT('Ctrl Pts',(28.9543118916328,64.8674919879648,0.));
#105056=CARTESIAN_POINT('Ctrl Pts',(28.9567285055866,64.8894389501801,0.));
#105057=CARTESIAN_POINT('Ctrl Pts',(28.9591278766934,64.9114350928125,0.));
#105058=CARTESIAN_POINT('Ctrl Pts',(28.9615099175249,64.9334802788038,0.));
#105059=CARTESIAN_POINT('Ctrl Pts',(28.9638745411677,64.955574371711,0.));
#105060=CARTESIAN_POINT('Ctrl Pts',(28.9662216612217,64.9777172357027,0.));
#105061=CARTESIAN_POINT('Ctrl Pts',(28.9685511918018,64.9999087355504,0.));
#105062=CARTESIAN_POINT('Ctrl Pts',(28.97086304753,65.022148736628,0.));
#105063=CARTESIAN_POINT('Ctrl Pts',(28.9731571435282,65.0444371049082,0.));
#105064=CARTESIAN_POINT('Ctrl Pts',(28.9754333954135,65.0667737069563,0.));
#105065=CARTESIAN_POINT('Ctrl Pts',(28.9776917192933,65.0891584099168,0.));
#105066=CARTESIAN_POINT('Ctrl Pts',(28.9799320317641,65.1115910815037,0.));
#105067=CARTESIAN_POINT('Ctrl Pts',(28.9821542499042,65.1340715900028,0.));
#105068=CARTESIAN_POINT('Ctrl Pts',(28.9843582912692,65.1565998042697,0.));
#105069=CARTESIAN_POINT('Ctrl Pts',(28.9865440738883,65.1791755937256,0.));
#105070=CARTESIAN_POINT('Ctrl Pts',(28.9887115162633,65.2017988283479,0.));
#105071=CARTESIAN_POINT('Ctrl Pts',(28.9908605373663,65.2244693786609,0.));
#105072=CARTESIAN_POINT('Ctrl Pts',(28.9929910566325,65.2471871157397,0.));
#105073=CARTESIAN_POINT('Ctrl Pts',(28.9951029939557,65.2699519112064,0.));
#105074=CARTESIAN_POINT('Ctrl Pts',(28.9971962696845,65.2927636372254,0.));
#105075=CARTESIAN_POINT('Ctrl Pts',(28.9992708046211,65.3156221664916,0.));
#105076=CARTESIAN_POINT('Ctrl Pts',(29.0013265200185,65.3385273722241,0.));
#105077=CARTESIAN_POINT('Ctrl Pts',(29.003363337573,65.3614791281692,0.));
#105078=CARTESIAN_POINT('Ctrl Pts',(29.0053811794207,65.3844773085961,0.));
#105079=CARTESIAN_POINT('Ctrl Pts',(29.0073799681342,65.4075217882934,0.));
#105080=CARTESIAN_POINT('Ctrl Pts',(29.0093596267215,65.4306124425562,0.));
#105081=CARTESIAN_POINT('Ctrl Pts',(29.0113200786239,65.4537491471828,0.));
#105082=CARTESIAN_POINT('Ctrl Pts',(29.013261247709,65.4769317784789,0.));
#105083=CARTESIAN_POINT('Ctrl Pts',(29.0151830582675,65.5001602132535,0.));
#105084=CARTESIAN_POINT('Ctrl Pts',(29.0170854350095,65.5234343288136,0.));
#105085=CARTESIAN_POINT('Ctrl Pts',(29.0189683030642,65.5467540029514,0.));
#105086=CARTESIAN_POINT('Ctrl Pts',(29.0208315879764,65.5701191139418,0.));
#105087=CARTESIAN_POINT('Ctrl Pts',(29.0226752157003,65.5935295405453,0.));
#105088=CARTESIAN_POINT('Ctrl Pts',(29.0244991125958,65.6169851620046,0.));
#105089=CARTESIAN_POINT('Ctrl Pts',(29.0263032054266,65.6404858580403,0.));
#105090=CARTESIAN_POINT('Ctrl Pts',(29.0280874213596,65.6640315088388,0.));
#105091=CARTESIAN_POINT('Ctrl Pts',(29.0298516879611,65.6876219950493,0.));
#105092=CARTESIAN_POINT('Ctrl Pts',(29.0315959331919,65.7112571977891,0.));
#105093=CARTESIAN_POINT('Ctrl Pts',(29.0333200854027,65.7349369986384,0.));
#105094=CARTESIAN_POINT('Ctrl Pts',(29.035024073333,65.7586612796368,0.));
#105095=CARTESIAN_POINT('Ctrl Pts',(29.0367078261102,65.7824299232705,0.));
#105096=CARTESIAN_POINT('Ctrl Pts',(29.0383712732469,65.8062428124713,0.));
#105097=CARTESIAN_POINT('Ctrl Pts',(29.0400143446338,65.8300998306191,0.));
#105098=CARTESIAN_POINT('Ctrl Pts',(29.0416369705375,65.854000861539,0.));
#105099=CARTESIAN_POINT('Ctrl Pts',(29.0432390815977,65.8779457894961,0.));
#105100=CARTESIAN_POINT('Ctrl Pts',(29.0448206088288,65.9019344991854,0.));
#105101=CARTESIAN_POINT('Ctrl Pts',(29.0463814836157,65.9259668757307,0.));
#105102=CARTESIAN_POINT('Ctrl Pts',(29.0479216377081,65.9500428046868,0.));
#105103=CARTESIAN_POINT('Ctrl Pts',(29.0494410032172,65.974162172037,0.));
#105104=CARTESIAN_POINT('Ctrl Pts',(29.0509395126142,65.9983248641879,0.));
#105105=CARTESIAN_POINT('Ctrl Pts',(29.0524170987307,66.0225307679591,0.));
#105106=CARTESIAN_POINT('Ctrl Pts',(29.0538736947552,66.0467797705815,0.));
#105107=CARTESIAN_POINT('Ctrl Pts',(29.0553092342278,66.0710717597009,0.));
#105108=CARTESIAN_POINT('Ctrl Pts',(29.0567236510373,66.0954066233754,0.));
#105109=CARTESIAN_POINT('Ctrl Pts',(29.0581168794189,66.1197842500711,0.));
#105110=CARTESIAN_POINT('Ctrl Pts',(29.0594888539555,66.1442045286516,0.));
#105111=CARTESIAN_POINT('Ctrl Pts',(29.0608395095745,66.1686673483755,0.));
#105112=CARTESIAN_POINT('Ctrl Pts',(29.062168781542,66.1931725989008,0.));
#105113=CARTESIAN_POINT('Ctrl Pts',(29.0634766054599,66.2177201702819,0.));
#105114=CARTESIAN_POINT('Ctrl Pts',(29.0647629172645,66.2423099529668,0.));
#105115=CARTESIAN_POINT('Ctrl Pts',(29.0660276532272,66.2669418377866,0.));
#105116=CARTESIAN_POINT('Ctrl Pts',(29.0672707499527,66.2916157159528,0.));
#105117=CARTESIAN_POINT('Ctrl Pts',(29.0684921443718,66.3163314790607,0.));
#105118=CARTESIAN_POINT('Ctrl Pts',(29.0696917737397,66.3410890190879,0.));
#105119=CARTESIAN_POINT('Ctrl Pts',(29.0708695756335,66.3658882283906,0.));
#105120=CARTESIAN_POINT('Ctrl Pts',(29.0720254879535,66.3907289996942,0.));
#105121=CARTESIAN_POINT('Ctrl Pts',(29.0731594489218,66.4156112260904,0.));
#105122=CARTESIAN_POINT('Ctrl Pts',(29.0742713970762,66.4405348010404,0.));
#105123=CARTESIAN_POINT('Ctrl Pts',(29.0753612712669,66.4654996183739,0.));
#105124=CARTESIAN_POINT('Ctrl Pts',(29.0764290106553,66.4905055722864,0.));
#105125=CARTESIAN_POINT('Ctrl Pts',(29.0774745547146,66.5155525573308,0.));
#105126=CARTESIAN_POINT('Ctrl Pts',(29.0784978432294,66.5406404684116,0.));
#105127=CARTESIAN_POINT('Ctrl Pts',(29.0794988162892,66.5657692007894,0.));
#105128=CARTESIAN_POINT('Ctrl Pts',(29.0804774142852,66.5909386500796,0.));
#105129=CARTESIAN_POINT('Ctrl Pts',(29.0814335779085,66.6161487122504,0.));
#105130=CARTESIAN_POINT('Ctrl Pts',(29.0823672481508,66.6413992836148,0.));
#105131=CARTESIAN_POINT('Ctrl Pts',(29.0832783663048,66.6666902608246,0.));
#105132=CARTESIAN_POINT('Ctrl Pts',(29.0841668739585,66.6920215408744,0.));
#105133=CARTESIAN_POINT('Ctrl Pts',(29.0850327129913,66.7173930211015,0.));
#105134=CARTESIAN_POINT('Ctrl Pts',(29.0858758255729,66.7428045991841,0.));
#105135=CARTESIAN_POINT('Ctrl Pts',(29.0866961541629,66.7682561731349,0.));
#105136=CARTESIAN_POINT('Ctrl Pts',(29.0874936415137,66.7937476412941,0.));
#105137=CARTESIAN_POINT('Ctrl Pts',(29.0882682306636,66.8192789023323,0.));
#105138=CARTESIAN_POINT('Ctrl Pts',(29.0890198649327,66.8448498552508,0.));
#105139=CARTESIAN_POINT('Ctrl Pts',(29.0897484879207,66.8704603993794,0.));
#105140=CARTESIAN_POINT('Ctrl Pts',(29.0904540435063,66.8961104343703,0.));
#105141=CARTESIAN_POINT('Ctrl Pts',(29.0911364758484,66.9217998601881,0.));
#105142=CARTESIAN_POINT('Ctrl Pts',(29.0917957293824,66.9475285771133,0.));
#105143=CARTESIAN_POINT('Ctrl Pts',(29.092431748817,66.9732964857467,0.));
#105144=CARTESIAN_POINT('Ctrl Pts',(29.0930444791328,66.9991034870084,0.));
#105145=CARTESIAN_POINT('Ctrl Pts',(29.0936338655828,67.0249494821361,0.));
#105146=CARTESIAN_POINT('Ctrl Pts',(29.0941998536957,67.0508343726771,0.));
#105147=CARTESIAN_POINT('Ctrl Pts',(29.0947423892725,67.0767580604872,0.));
#105148=CARTESIAN_POINT('Ctrl Pts',(29.0952614183777,67.1027204477304,0.));
#105149=CARTESIAN_POINT('Ctrl Pts',(29.0957568873357,67.1287214368743,0.));
#105150=CARTESIAN_POINT('Ctrl Pts',(29.0962287427274,67.1547609306845,0.));
#105151=CARTESIAN_POINT('Ctrl Pts',(29.0966769313893,67.1808388322116,0.));
#105152=CARTESIAN_POINT('Ctrl Pts',(29.0971014004134,67.2069550447895,0.));
#105153=CARTESIAN_POINT('Ctrl Pts',(29.0975020971473,67.2331094720482,0.));
#105154=CARTESIAN_POINT('Ctrl Pts',(29.0978789691964,67.2593020179216,0.));
#105155=CARTESIAN_POINT('Ctrl Pts',(29.0982319644276,67.2855325866516,0.));
#105156=CARTESIAN_POINT('Ctrl Pts',(29.0985610309768,67.311801082791,0.));
#105157=CARTESIAN_POINT('Ctrl Pts',(29.0988661172526,67.3381074112013,0.));
#105158=CARTESIAN_POINT('Ctrl Pts',(29.0991471719172,67.3644514770373,0.));
#105159=CARTESIAN_POINT('Ctrl Pts',(29.0994041438715,67.3908331857313,0.));
#105160=CARTESIAN_POINT('Ctrl Pts',(29.0996369822418,67.4172524429726,0.));
#105161=CARTESIAN_POINT('Ctrl Pts',(29.0998456363687,67.4437091546869,0.));
#105162=CARTESIAN_POINT('Ctrl Pts',(29.1000300557961,67.4702032270063,0.));
#105163=CARTESIAN_POINT('Ctrl Pts',(29.1001901902914,67.496734566311,0.));
#105164=CARTESIAN_POINT('Ctrl Pts',(29.1003259898686,67.5233030792714,0.));
#105165=CARTESIAN_POINT('Ctrl Pts',(29.1004374048149,67.5499086728891,0.));
#105166=CARTESIAN_POINT('Ctrl Pts',(29.1005243857137,67.5765512545276,0.));
#105167=CARTESIAN_POINT('Ctrl Pts',(29.1005868834863,67.6032307319614,0.));
#105168=CARTESIAN_POINT('Ctrl Pts',(29.1006248493576,67.6299470133286,0.));
#105169=CARTESIAN_POINT('Ctrl Pts',(29.1006382347811,67.6567000070319,0.));
#105170=CARTESIAN_POINT('Ctrl Pts',(29.1006269913746,67.6834896216458,0.));
#105171=CARTESIAN_POINT('Ctrl Pts',(29.1005910708624,67.7103157658297,0.));
#105172=CARTESIAN_POINT('Ctrl Pts',(29.1005304249988,67.7371783482039,0.));
#105173=CARTESIAN_POINT('Ctrl Pts',(29.1004450055647,67.7640772773397,0.));
#105174=CARTESIAN_POINT('Ctrl Pts',(29.1003347645299,67.7910124620148,0.));
#105175=CARTESIAN_POINT('Ctrl Pts',(29.1001996541846,67.8179838114109,0.));
#105176=CARTESIAN_POINT('Ctrl Pts',(29.1000396272868,67.844991235333,0.));
#105177=CARTESIAN_POINT('Ctrl Pts',(29.0998546372027,67.8720346444111,0.));
#105178=CARTESIAN_POINT('Ctrl Pts',(29.0996446380617,67.8991139503168,0.));
#105179=CARTESIAN_POINT('Ctrl Pts',(29.0994095844208,67.9262290652797,0.));
#105180=CARTESIAN_POINT('Ctrl Pts',(29.0991494309394,67.9533799016122,0.));
#105181=CARTESIAN_POINT('Ctrl Pts',(29.0988641320243,67.9805663711845,0.));
#105182=CARTESIAN_POINT('Ctrl Pts',(29.0985536415537,68.0077883850136,0.));
#105183=CARTESIAN_POINT('Ctrl Pts',(29.0982179124112,68.0350458525589,0.));
#105184=CARTESIAN_POINT('Ctrl Pts',(29.0978568968677,68.0623386822917,0.));
#105185=CARTESIAN_POINT('Ctrl Pts',(29.0974705474279,68.089666782962,0.));
#105186=CARTESIAN_POINT('Ctrl Pts',(29.097058817574,68.1170300647019,0.));
#105187=CARTESIAN_POINT('Ctrl Pts',(29.096621662474,68.1444284400734,0.));
#105188=CARTESIAN_POINT('Ctrl Pts',(29.0961590399023,68.1718618254221,0.));
#105189=CARTESIAN_POINT('Ctrl Pts',(29.0956709104588,68.1993301411959,0.));
#105190=CARTESIAN_POINT('Ctrl Pts',(29.0952305915108,68.2229056854495,0.));
#105191=CARTESIAN_POINT('Ctrl Pts',(29.0948791947834,68.2409993689947,0.));
#105192=CARTESIAN_POINT('Ctrl Pts',(29.094628043331,68.2535957746884,0.));
#105193=CARTESIAN_POINT('Ctrl Pts',(29.0944846386548,68.2606847334625,0.));
#105194=CARTESIAN_POINT('Ctrl Pts',(29.0944526440248,68.2622612909745,0.));
#105195=CARTESIAN_POINT('',(28.8072485549236,63.7976679095314,12.));
#105196=CARTESIAN_POINT('',(28.8072485549236,63.7976679095314,0.));
#105197=CARTESIAN_POINT('Ctrl Pts',(29.0944526440248,68.2622612909745,12.));
#105198=CARTESIAN_POINT('Ctrl Pts',(29.0944846386548,68.2606847334625,12.));
#105199=CARTESIAN_POINT('Ctrl Pts',(29.094628043331,68.2535957746884,12.));
#105200=CARTESIAN_POINT('Ctrl Pts',(29.0948791947834,68.2409993689947,12.));
#105201=CARTESIAN_POINT('Ctrl Pts',(29.0952305915108,68.2229056854495,12.));
#105202=CARTESIAN_POINT('Ctrl Pts',(29.0956709104588,68.1993301411959,12.));
#105203=CARTESIAN_POINT('Ctrl Pts',(29.0961590399023,68.1718618254221,12.));
#105204=CARTESIAN_POINT('Ctrl Pts',(29.096621662474,68.1444284400734,12.));
#105205=CARTESIAN_POINT('Ctrl Pts',(29.097058817574,68.1170300647019,12.));
#105206=CARTESIAN_POINT('Ctrl Pts',(29.0974705474279,68.089666782962,12.));
#105207=CARTESIAN_POINT('Ctrl Pts',(29.0978568968677,68.0623386822917,12.));
#105208=CARTESIAN_POINT('Ctrl Pts',(29.0982179124112,68.0350458525589,12.));
#105209=CARTESIAN_POINT('Ctrl Pts',(29.0985536415537,68.0077883850136,12.));
#105210=CARTESIAN_POINT('Ctrl Pts',(29.0988641320243,67.9805663711845,12.));
#105211=CARTESIAN_POINT('Ctrl Pts',(29.0991494309394,67.9533799016122,12.));
#105212=CARTESIAN_POINT('Ctrl Pts',(29.0994095844208,67.9262290652797,12.));
#105213=CARTESIAN_POINT('Ctrl Pts',(29.0996446380617,67.8991139503168,12.));
#105214=CARTESIAN_POINT('Ctrl Pts',(29.0998546372027,67.8720346444111,12.));
#105215=CARTESIAN_POINT('Ctrl Pts',(29.1000396272868,67.844991235333,12.));
#105216=CARTESIAN_POINT('Ctrl Pts',(29.1001996541846,67.8179838114109,12.));
#105217=CARTESIAN_POINT('Ctrl Pts',(29.1003347645299,67.7910124620148,12.));
#105218=CARTESIAN_POINT('Ctrl Pts',(29.1004450055647,67.7640772773397,12.));
#105219=CARTESIAN_POINT('Ctrl Pts',(29.1005304249988,67.7371783482039,12.));
#105220=CARTESIAN_POINT('Ctrl Pts',(29.1005910708624,67.7103157658297,12.));
#105221=CARTESIAN_POINT('Ctrl Pts',(29.1006269913746,67.6834896216458,12.));
#105222=CARTESIAN_POINT('Ctrl Pts',(29.1006382347811,67.6567000070319,12.));
#105223=CARTESIAN_POINT('Ctrl Pts',(29.1006248493576,67.6299470133286,12.));
#105224=CARTESIAN_POINT('Ctrl Pts',(29.1005868834863,67.6032307319614,12.));
#105225=CARTESIAN_POINT('Ctrl Pts',(29.1005243857137,67.5765512545276,12.));
#105226=CARTESIAN_POINT('Ctrl Pts',(29.1004374048149,67.5499086728891,12.));
#105227=CARTESIAN_POINT('Ctrl Pts',(29.1003259898686,67.5233030792714,12.));
#105228=CARTESIAN_POINT('Ctrl Pts',(29.1001901902914,67.496734566311,12.));
#105229=CARTESIAN_POINT('Ctrl Pts',(29.1000300557961,67.4702032270063,12.));
#105230=CARTESIAN_POINT('Ctrl Pts',(29.0998456363687,67.4437091546869,12.));
#105231=CARTESIAN_POINT('Ctrl Pts',(29.0996369822418,67.4172524429726,12.));
#105232=CARTESIAN_POINT('Ctrl Pts',(29.0994041438715,67.3908331857313,12.));
#105233=CARTESIAN_POINT('Ctrl Pts',(29.0991471719172,67.3644514770373,12.));
#105234=CARTESIAN_POINT('Ctrl Pts',(29.0988661172526,67.3381074112013,12.));
#105235=CARTESIAN_POINT('Ctrl Pts',(29.0985610309768,67.311801082791,12.));
#105236=CARTESIAN_POINT('Ctrl Pts',(29.0982319644276,67.2855325866516,12.));
#105237=CARTESIAN_POINT('Ctrl Pts',(29.0978789691964,67.2593020179216,12.));
#105238=CARTESIAN_POINT('Ctrl Pts',(29.0975020971473,67.2331094720482,12.));
#105239=CARTESIAN_POINT('Ctrl Pts',(29.0971014004134,67.2069550447895,12.));
#105240=CARTESIAN_POINT('Ctrl Pts',(29.0966769313893,67.1808388322116,12.));
#105241=CARTESIAN_POINT('Ctrl Pts',(29.0962287427274,67.1547609306845,12.));
#105242=CARTESIAN_POINT('Ctrl Pts',(29.0957568873357,67.1287214368743,12.));
#105243=CARTESIAN_POINT('Ctrl Pts',(29.0952614183777,67.1027204477304,12.));
#105244=CARTESIAN_POINT('Ctrl Pts',(29.0947423892725,67.0767580604872,12.));
#105245=CARTESIAN_POINT('Ctrl Pts',(29.0941998536957,67.0508343726771,12.));
#105246=CARTESIAN_POINT('Ctrl Pts',(29.0936338655828,67.0249494821361,12.));
#105247=CARTESIAN_POINT('Ctrl Pts',(29.0930444791328,66.9991034870084,12.));
#105248=CARTESIAN_POINT('Ctrl Pts',(29.092431748817,66.9732964857467,12.));
#105249=CARTESIAN_POINT('Ctrl Pts',(29.0917957293824,66.9475285771133,12.));
#105250=CARTESIAN_POINT('Ctrl Pts',(29.0911364758484,66.9217998601881,12.));
#105251=CARTESIAN_POINT('Ctrl Pts',(29.0904540435063,66.8961104343703,12.));
#105252=CARTESIAN_POINT('Ctrl Pts',(29.0897484879207,66.8704603993794,12.));
#105253=CARTESIAN_POINT('Ctrl Pts',(29.0890198649327,66.8448498552508,12.));
#105254=CARTESIAN_POINT('Ctrl Pts',(29.0882682306636,66.8192789023323,12.));
#105255=CARTESIAN_POINT('Ctrl Pts',(29.0874936415137,66.7937476412941,12.));
#105256=CARTESIAN_POINT('Ctrl Pts',(29.0866961541629,66.7682561731349,12.));
#105257=CARTESIAN_POINT('Ctrl Pts',(29.0858758255729,66.7428045991841,12.));
#105258=CARTESIAN_POINT('Ctrl Pts',(29.0850327129913,66.7173930211015,12.));
#105259=CARTESIAN_POINT('Ctrl Pts',(29.0841668739585,66.6920215408744,12.));
#105260=CARTESIAN_POINT('Ctrl Pts',(29.0832783663048,66.6666902608246,12.));
#105261=CARTESIAN_POINT('Ctrl Pts',(29.0823672481508,66.6413992836148,12.));
#105262=CARTESIAN_POINT('Ctrl Pts',(29.0814335779085,66.6161487122504,12.));
#105263=CARTESIAN_POINT('Ctrl Pts',(29.0804774142852,66.5909386500796,12.));
#105264=CARTESIAN_POINT('Ctrl Pts',(29.0794988162892,66.5657692007894,12.));
#105265=CARTESIAN_POINT('Ctrl Pts',(29.0784978432294,66.5406404684116,12.));
#105266=CARTESIAN_POINT('Ctrl Pts',(29.0774745547146,66.5155525573308,12.));
#105267=CARTESIAN_POINT('Ctrl Pts',(29.0764290106553,66.4905055722864,12.));
#105268=CARTESIAN_POINT('Ctrl Pts',(29.0753612712669,66.4654996183739,12.));
#105269=CARTESIAN_POINT('Ctrl Pts',(29.0742713970762,66.4405348010404,12.));
#105270=CARTESIAN_POINT('Ctrl Pts',(29.0731594489218,66.4156112260904,12.));
#105271=CARTESIAN_POINT('Ctrl Pts',(29.0720254879535,66.3907289996942,12.));
#105272=CARTESIAN_POINT('Ctrl Pts',(29.0708695756335,66.3658882283906,12.));
#105273=CARTESIAN_POINT('Ctrl Pts',(29.0696917737397,66.3410890190879,12.));
#105274=CARTESIAN_POINT('Ctrl Pts',(29.0684921443718,66.3163314790607,12.));
#105275=CARTESIAN_POINT('Ctrl Pts',(29.0672707499527,66.2916157159528,12.));
#105276=CARTESIAN_POINT('Ctrl Pts',(29.0660276532272,66.2669418377866,12.));
#105277=CARTESIAN_POINT('Ctrl Pts',(29.0647629172645,66.2423099529668,12.));
#105278=CARTESIAN_POINT('Ctrl Pts',(29.0634766054599,66.2177201702819,12.));
#105279=CARTESIAN_POINT('Ctrl Pts',(29.062168781542,66.1931725989008,12.));
#105280=CARTESIAN_POINT('Ctrl Pts',(29.0608395095745,66.1686673483755,12.));
#105281=CARTESIAN_POINT('Ctrl Pts',(29.0594888539555,66.1442045286516,12.));
#105282=CARTESIAN_POINT('Ctrl Pts',(29.0581168794189,66.1197842500711,12.));
#105283=CARTESIAN_POINT('Ctrl Pts',(29.0567236510373,66.0954066233754,12.));
#105284=CARTESIAN_POINT('Ctrl Pts',(29.0553092342278,66.0710717597009,12.));
#105285=CARTESIAN_POINT('Ctrl Pts',(29.0538736947552,66.0467797705815,12.));
#105286=CARTESIAN_POINT('Ctrl Pts',(29.0524170987307,66.0225307679591,12.));
#105287=CARTESIAN_POINT('Ctrl Pts',(29.0509395126142,65.9983248641879,12.));
#105288=CARTESIAN_POINT('Ctrl Pts',(29.0494410032172,65.974162172037,12.));
#105289=CARTESIAN_POINT('Ctrl Pts',(29.0479216377081,65.9500428046868,12.));
#105290=CARTESIAN_POINT('Ctrl Pts',(29.0463814836157,65.9259668757307,12.));
#105291=CARTESIAN_POINT('Ctrl Pts',(29.0448206088288,65.9019344991854,12.));
#105292=CARTESIAN_POINT('Ctrl Pts',(29.0432390815977,65.8779457894961,12.));
#105293=CARTESIAN_POINT('Ctrl Pts',(29.0416369705375,65.854000861539,12.));
#105294=CARTESIAN_POINT('Ctrl Pts',(29.0400143446338,65.8300998306191,12.));
#105295=CARTESIAN_POINT('Ctrl Pts',(29.0383712732469,65.8062428124713,12.));
#105296=CARTESIAN_POINT('Ctrl Pts',(29.0367078261102,65.7824299232705,12.));
#105297=CARTESIAN_POINT('Ctrl Pts',(29.035024073333,65.7586612796368,12.));
#105298=CARTESIAN_POINT('Ctrl Pts',(29.0333200854027,65.7349369986384,12.));
#105299=CARTESIAN_POINT('Ctrl Pts',(29.0315959331919,65.7112571977891,12.));
#105300=CARTESIAN_POINT('Ctrl Pts',(29.0298516879611,65.6876219950493,12.));
#105301=CARTESIAN_POINT('Ctrl Pts',(29.0280874213596,65.6640315088388,12.));
#105302=CARTESIAN_POINT('Ctrl Pts',(29.0263032054266,65.6404858580403,12.));
#105303=CARTESIAN_POINT('Ctrl Pts',(29.0244991125958,65.6169851620046,12.));
#105304=CARTESIAN_POINT('Ctrl Pts',(29.0226752157003,65.5935295405453,12.));
#105305=CARTESIAN_POINT('Ctrl Pts',(29.0208315879764,65.5701191139418,12.));
#105306=CARTESIAN_POINT('Ctrl Pts',(29.0189683030642,65.5467540029514,12.));
#105307=CARTESIAN_POINT('Ctrl Pts',(29.0170854350095,65.5234343288136,12.));
#105308=CARTESIAN_POINT('Ctrl Pts',(29.0151830582675,65.5001602132535,12.));
#105309=CARTESIAN_POINT('Ctrl Pts',(29.013261247709,65.4769317784789,12.));
#105310=CARTESIAN_POINT('Ctrl Pts',(29.0113200786239,65.4537491471828,12.));
#105311=CARTESIAN_POINT('Ctrl Pts',(29.0093596267215,65.4306124425562,12.));
#105312=CARTESIAN_POINT('Ctrl Pts',(29.0073799681342,65.4075217882934,12.));
#105313=CARTESIAN_POINT('Ctrl Pts',(29.0053811794207,65.3844773085961,12.));
#105314=CARTESIAN_POINT('Ctrl Pts',(29.003363337573,65.3614791281692,12.));
#105315=CARTESIAN_POINT('Ctrl Pts',(29.0013265200185,65.3385273722241,12.));
#105316=CARTESIAN_POINT('Ctrl Pts',(28.9992708046211,65.3156221664916,12.));
#105317=CARTESIAN_POINT('Ctrl Pts',(28.9971962696845,65.2927636372254,12.));
#105318=CARTESIAN_POINT('Ctrl Pts',(28.9951029939557,65.2699519112064,12.));
#105319=CARTESIAN_POINT('Ctrl Pts',(28.9929910566325,65.2471871157397,12.));
#105320=CARTESIAN_POINT('Ctrl Pts',(28.9908605373663,65.2244693786609,12.));
#105321=CARTESIAN_POINT('Ctrl Pts',(28.9887115162633,65.2017988283479,12.));
#105322=CARTESIAN_POINT('Ctrl Pts',(28.9865440738883,65.1791755937256,12.));
#105323=CARTESIAN_POINT('Ctrl Pts',(28.9843582912692,65.1565998042697,12.));
#105324=CARTESIAN_POINT('Ctrl Pts',(28.9821542499042,65.1340715900028,12.));
#105325=CARTESIAN_POINT('Ctrl Pts',(28.9799320317641,65.1115910815037,12.));
#105326=CARTESIAN_POINT('Ctrl Pts',(28.9776917192933,65.0891584099168,12.));
#105327=CARTESIAN_POINT('Ctrl Pts',(28.9754333954135,65.0667737069563,12.));
#105328=CARTESIAN_POINT('Ctrl Pts',(28.9731571435282,65.0444371049082,12.));
#105329=CARTESIAN_POINT('Ctrl Pts',(28.97086304753,65.022148736628,12.));
#105330=CARTESIAN_POINT('Ctrl Pts',(28.9685511918018,64.9999087355504,12.));
#105331=CARTESIAN_POINT('Ctrl Pts',(28.9662216612217,64.9777172357027,12.));
#105332=CARTESIAN_POINT('Ctrl Pts',(28.9638745411677,64.955574371711,12.));
#105333=CARTESIAN_POINT('Ctrl Pts',(28.9615099175249,64.9334802788038,12.));
#105334=CARTESIAN_POINT('Ctrl Pts',(28.9591278766934,64.9114350928125,12.));
#105335=CARTESIAN_POINT('Ctrl Pts',(28.9567285055866,64.8894389501801,12.));
#105336=CARTESIAN_POINT('Ctrl Pts',(28.9543118916328,64.8674919879648,12.));
#105337=CARTESIAN_POINT('Ctrl Pts',(28.9518781227765,64.8455943438423,12.));
#105338=CARTESIAN_POINT('Ctrl Pts',(28.9494272874831,64.8237461561019,12.));
#105339=CARTESIAN_POINT('Ctrl Pts',(28.9469594747431,64.8019475636442,12.));
#105340=CARTESIAN_POINT('Ctrl Pts',(28.944474774081,64.7801987060084,12.));
#105341=CARTESIAN_POINT('Ctrl Pts',(28.9419732755655,64.758499723388,12.));
#105342=CARTESIAN_POINT('Ctrl Pts',(28.9394550698204,64.7368507566467,12.));
#105343=CARTESIAN_POINT('Ctrl Pts',(28.9369202480392,64.715251947329,12.));
#105344=CARTESIAN_POINT('Ctrl Pts',(28.9343689019882,64.6937034376617,12.));
#105345=CARTESIAN_POINT('Ctrl Pts',(28.9318011239915,64.672205370541,12.));
#105346=CARTESIAN_POINT('Ctrl Pts',(28.9292170069221,64.6507578895161,12.));
#105347=CARTESIAN_POINT('Ctrl Pts',(28.926616644195,64.629361138774,12.));
#105348=CARTESIAN_POINT('Ctrl Pts',(28.9240001297542,64.6080152631039,12.));
#105349=CARTESIAN_POINT('Ctrl Pts',(28.9213675580985,64.5867204079426,12.));
#105350=CARTESIAN_POINT('Ctrl Pts',(28.9187190243224,64.5654767194472,12.));
#105351=CARTESIAN_POINT('Ctrl Pts',(28.9160546241538,64.5442843445559,12.));
#105352=CARTESIAN_POINT('Ctrl Pts',(28.9133744539949,64.523143431047,12.));
#105353=CARTESIAN_POINT('Ctrl Pts',(28.910678610965,64.5020541275951,12.));
#105354=CARTESIAN_POINT('Ctrl Pts',(28.9079671928264,64.4810165836592,12.));
#105355=CARTESIAN_POINT('Ctrl Pts',(28.9052402979062,64.4600309493583,12.));
#105356=CARTESIAN_POINT('Ctrl Pts',(28.9024980250307,64.4390973753634,12.));
#105357=CARTESIAN_POINT('Ctrl Pts',(28.899740473434,64.4182160127379,12.));
#105358=CARTESIAN_POINT('Ctrl Pts',(28.8969677427504,64.397387012917,12.));
#105359=CARTESIAN_POINT('Ctrl Pts',(28.89417993323,64.3766105280688,12.));
#105360=CARTESIAN_POINT('Ctrl Pts',(28.8913771459323,64.3558867114076,12.));
#105361=CARTESIAN_POINT('Ctrl Pts',(28.8885594828926,64.3352157174619,12.));
#105362=CARTESIAN_POINT('Ctrl Pts',(28.8857270473959,64.3145977025037,12.));
#105363=CARTESIAN_POINT('Ctrl Pts',(28.882879943794,64.2940328242521,12.));
#105364=CARTESIAN_POINT('Ctrl Pts',(28.8800182770064,64.2735212410711,12.));
#105365=CARTESIAN_POINT('Ctrl Pts',(28.877142152106,64.2530631112929,12.));
#105366=CARTESIAN_POINT('Ctrl Pts',(28.8742516738946,64.2326585925252,12.));
#105367=CARTESIAN_POINT('Ctrl Pts',(28.8713469464185,64.2123078408461,12.));
#105368=CARTESIAN_POINT('Ctrl Pts',(28.8684280739014,64.1920110123299,12.));
#105369=CARTESIAN_POINT('Ctrl Pts',(28.8654951618649,64.1717682648685,12.));
#105370=CARTESIAN_POINT('Ctrl Pts',(28.8625483180437,64.1515797596564,12.));
#105371=CARTESIAN_POINT('Ctrl Pts',(28.8595876537148,64.1314456633381,12.));
#105372=CARTESIAN_POINT('Ctrl Pts',(28.8566132838178,64.1113661481965,12.));
#105373=CARTESIAN_POINT('Ctrl Pts',(28.8536253241853,64.0913413876622,12.));
#105374=CARTESIAN_POINT('Ctrl Pts',(28.8506238891092,64.0713715523599,12.));
#105375=CARTESIAN_POINT('Ctrl Pts',(28.8476090892232,64.0514568066637,12.));
#105376=CARTESIAN_POINT('Ctrl Pts',(28.844581028125,64.0315973031942,12.));
#105377=CARTESIAN_POINT('Ctrl Pts',(28.8415398056428,64.0117931881298,12.));
#105378=CARTESIAN_POINT('Ctrl Pts',(28.8384855243242,63.9920446117582,12.));
#105379=CARTESIAN_POINT('Ctrl Pts',(28.83541829466,63.9723517369614,12.));
#105380=CARTESIAN_POINT('Ctrl Pts',(28.8323382413789,63.9527147494423,12.));
#105381=CARTESIAN_POINT('Ctrl Pts',(28.8292455077559,63.9331338646996,12.));
#105382=CARTESIAN_POINT('Ctrl Pts',(28.8261402423291,63.9136093063786,12.));
#105383=CARTESIAN_POINT('Ctrl Pts',(28.823022586318,63.8941412856924,12.));
#105384=CARTESIAN_POINT('Ctrl Pts',(28.8198926619857,63.8747299825313,12.));
#105385=CARTESIAN_POINT('Ctrl Pts',(28.8167505576681,63.8553755207487,12.));
#105386=CARTESIAN_POINT('Ctrl Pts',(28.8135963263368,63.8360779669856,12.));
#105387=CARTESIAN_POINT('Ctrl Pts',(28.8110632620957,63.8206854735028,12.));
#105388=CARTESIAN_POINT('Ctrl Pts',(28.8091580239553,63.8091667271232,12.));
#105389=CARTESIAN_POINT('Ctrl Pts',(28.8078854475432,63.8014989507494,12.));
#105390=CARTESIAN_POINT('Ctrl Pts',(28.8072485549236,63.7976679095314,12.));
#105391=CARTESIAN_POINT('Ctrl Pts',(27.6958230985043,68.8415926175085,-2.22044604925031E-15));
#105392=CARTESIAN_POINT('Ctrl Pts',(27.6958230985043,68.8415926175085,4.));
#105393=CARTESIAN_POINT('Ctrl Pts',(27.6958230985043,68.8415926175085,8.));
#105394=CARTESIAN_POINT('Ctrl Pts',(27.6958230985043,68.8415926175085,12.));
#105395=CARTESIAN_POINT('Ctrl Pts',(27.7750822307002,68.9176987693915,-2.22044604925031E-15));
#105396=CARTESIAN_POINT('Ctrl Pts',(27.7750822307002,68.9176987693915,4.));
#105397=CARTESIAN_POINT('Ctrl Pts',(27.7750822307002,68.9176987693915,8.));
#105398=CARTESIAN_POINT('Ctrl Pts',(27.7750822307002,68.9176987693915,12.));
#105399=CARTESIAN_POINT('Ctrl Pts',(27.9589320265197,69.002974546758,-2.00119860333522E-15));
#105400=CARTESIAN_POINT('Ctrl Pts',(27.9589320265197,69.002974546758,4.));
#105401=CARTESIAN_POINT('Ctrl Pts',(27.9589320265197,69.002974546758,7.99999999999999));
#105402=CARTESIAN_POINT('Ctrl Pts',(27.9589320265197,69.002974546758,12.));
#105403=CARTESIAN_POINT('Ctrl Pts',(28.1553386138881,68.9748773050759,-1.48061250865807E-15));
#105404=CARTESIAN_POINT('Ctrl Pts',(28.1553386138881,68.9748773050759,4.));
#105405=CARTESIAN_POINT('Ctrl Pts',(28.1553386138881,68.9748773050759,8.00000000000001));
#105406=CARTESIAN_POINT('Ctrl Pts',(28.1553386138881,68.9748773050759,12.));
#105407=CARTESIAN_POINT('Ctrl Pts',(28.2316040302242,68.9436475237613,-1.22965056797476E-15));
#105408=CARTESIAN_POINT('Ctrl Pts',(28.2316040302242,68.9436475237613,4.));
#105409=CARTESIAN_POINT('Ctrl Pts',(28.2316040302242,68.9436475237612,8.));
#105410=CARTESIAN_POINT('Ctrl Pts',(28.2316040302242,68.9436475237612,12.));
#105411=CARTESIAN_POINT('',(27.6958230985043,68.8415926175085,2.77555756156289E-16));
#105412=CARTESIAN_POINT('',(28.2316040302242,68.9436475237612,2.77555756156289E-16));
#105413=CARTESIAN_POINT('Ctrl Pts',(27.6958230985043,68.8415926175085,-1.12534929619454E-16));
#105414=CARTESIAN_POINT('Ctrl Pts',(27.7750822307002,68.9176987693915,-1.12534929619455E-16));
#105415=CARTESIAN_POINT('Ctrl Pts',(27.8801392568828,68.9664277850295,1.27493251891736E-17));
#105416=CARTESIAN_POINT('Ctrl Pts',(27.9892964598977,68.9781370393455,2.36429873471121E-16));
#105417=CARTESIAN_POINT('Ctrl Pts',(28.0711643621588,68.9869189800825,4.04190284682582E-16));
#105418=CARTESIAN_POINT('Ctrl Pts',(28.1553386138881,68.9748773050759,6.27298610972785E-16));
#105419=CARTESIAN_POINT('Ctrl Pts',(28.2316040302242,68.9436475237613,8.78260551656101E-16));
#105420=CARTESIAN_POINT('',(28.2316040302242,68.9436475237612,12.));
#105421=CARTESIAN_POINT('Ctrl Pts',(28.2316040302242,68.9436475237613,-1.22965056797476E-15));
#105422=CARTESIAN_POINT('Ctrl Pts',(28.2316040302242,68.9436475237613,4.));
#105423=CARTESIAN_POINT('Ctrl Pts',(28.2316040302242,68.9436475237612,8.));
#105424=CARTESIAN_POINT('Ctrl Pts',(28.2316040302242,68.9436475237612,12.));
#105425=CARTESIAN_POINT('',(27.6958230985043,68.8415926175085,12.));
#105426=CARTESIAN_POINT('Ctrl Pts',(28.2316040302242,68.9436475237612,12.));
#105427=CARTESIAN_POINT('Ctrl Pts',(28.1553386138881,68.9748773050759,12.));
#105428=CARTESIAN_POINT('Ctrl Pts',(28.0711643621588,68.9869189800825,12.));
#105429=CARTESIAN_POINT('Ctrl Pts',(27.9892964598977,68.9781370393455,12.));
#105430=CARTESIAN_POINT('Ctrl Pts',(27.8801392568828,68.9664277850295,12.));
#105431=CARTESIAN_POINT('Ctrl Pts',(27.7750822307002,68.9176987693915,12.));
#105432=CARTESIAN_POINT('Ctrl Pts',(27.6958230985043,68.8415926175085,12.));
#105433=CARTESIAN_POINT('Ctrl Pts',(27.6958230985043,68.8415926175085,12.));
#105434=CARTESIAN_POINT('Ctrl Pts',(27.6958230985043,68.8415926175085,8.));
#105435=CARTESIAN_POINT('Ctrl Pts',(27.6958230985043,68.8415926175085,4.));
#105436=CARTESIAN_POINT('Ctrl Pts',(27.6958230985043,68.8415926175085,-2.22044604925031E-15));
#105437=CARTESIAN_POINT('Origin',(1.43354795624835E-10,3.4634846687719E-10,
0.));
#105438=CARTESIAN_POINT('Origin',(1.43354795624835E-10,3.4634846687719E-10,
12.));
#105439=CARTESIAN_POINT('Origin',(1.43354795624835E-10,3.4634846687719E-10,
0.));
#105440=CARTESIAN_POINT('Ctrl Pts',(34.6669728017236,65.9427857825597,0.));
#105441=CARTESIAN_POINT('Ctrl Pts',(34.6669728017236,65.9427857825597,4.));
#105442=CARTESIAN_POINT('Ctrl Pts',(34.6669728017236,65.9427857825597,8.));
#105443=CARTESIAN_POINT('Ctrl Pts',(34.6669728017236,65.9427857825597,12.));
#105444=CARTESIAN_POINT('Ctrl Pts',(34.7642339552035,65.8916543400169,0.));
#105445=CARTESIAN_POINT('Ctrl Pts',(34.7642339552035,65.8916543400169,4.));
#105446=CARTESIAN_POINT('Ctrl Pts',(34.7642339552035,65.8916543400169,8.));
#105447=CARTESIAN_POINT('Ctrl Pts',(34.7642339552035,65.8916543400169,12.));
#105448=CARTESIAN_POINT('Ctrl Pts',(34.9032616822024,65.7441961270804,0.));
#105449=CARTESIAN_POINT('Ctrl Pts',(34.9032616822024,65.7441961270804,4.));
#105450=CARTESIAN_POINT('Ctrl Pts',(34.9032616822024,65.7441961270803,7.99999999999999));
#105451=CARTESIAN_POINT('Ctrl Pts',(34.9032616822024,65.7441961270803,12.));
#105452=CARTESIAN_POINT('Ctrl Pts',(34.9387029822715,65.5489812297285,0.));
#105453=CARTESIAN_POINT('Ctrl Pts',(34.9387029822715,65.5489812297285,4.));
#105454=CARTESIAN_POINT('Ctrl Pts',(34.9387029822716,65.5489812297284,8.00000000000001));
#105455=CARTESIAN_POINT('Ctrl Pts',(34.9387029822716,65.5489812297284,12.));
#105456=CARTESIAN_POINT('Ctrl Pts',(34.9331875523085,65.4667541477953,0.));
#105457=CARTESIAN_POINT('Ctrl Pts',(34.9331875523085,65.4667541477953,4.));
#105458=CARTESIAN_POINT('Ctrl Pts',(34.9331875523085,65.4667541477952,8.));
#105459=CARTESIAN_POINT('Ctrl Pts',(34.9331875523085,65.4667541477952,12.));
#105460=CARTESIAN_POINT('',(34.6669728017236,65.9427857825597,0.));
#105461=CARTESIAN_POINT('',(34.9331875523085,65.4667541477953,0.));
#105462=CARTESIAN_POINT('Ctrl Pts',(34.6669728017236,65.9427857825597,2.77555756156289E-16));
#105463=CARTESIAN_POINT('Ctrl Pts',(34.7642339552035,65.8916543400169,2.77555756156289E-16));
#105464=CARTESIAN_POINT('Ctrl Pts',(34.8436783706314,65.8073925040532,2.77555756156289E-16));
#105465=CARTESIAN_POINT('Ctrl Pts',(34.8892986466537,65.7075366486885,2.77555756156289E-16));
#105466=CARTESIAN_POINT('Ctrl Pts',(34.9235138536705,65.632644757165,2.77555756156289E-16));
#105467=CARTESIAN_POINT('Ctrl Pts',(34.9387029822715,65.5489812297285,2.77555756156289E-16));
#105468=CARTESIAN_POINT('Ctrl Pts',(34.9331875523085,65.4667541477953,2.77555756156289E-16));
#105469=CARTESIAN_POINT('',(34.9331875523085,65.4667541477952,12.));
#105470=CARTESIAN_POINT('Ctrl Pts',(34.9331875523085,65.4667541477953,0.));
#105471=CARTESIAN_POINT('Ctrl Pts',(34.9331875523085,65.4667541477953,4.));
#105472=CARTESIAN_POINT('Ctrl Pts',(34.9331875523085,65.4667541477952,8.));
#105473=CARTESIAN_POINT('Ctrl Pts',(34.9331875523085,65.4667541477952,12.));
#105474=CARTESIAN_POINT('',(34.6669728017236,65.9427857825597,12.));
#105475=CARTESIAN_POINT('Ctrl Pts',(34.9331875523085,65.4667541477952,12.));
#105476=CARTESIAN_POINT('Ctrl Pts',(34.9387029822716,65.5489812297284,12.));
#105477=CARTESIAN_POINT('Ctrl Pts',(34.9235138536705,65.6326447571649,12.));
#105478=CARTESIAN_POINT('Ctrl Pts',(34.8892986466538,65.7075366486884,12.));
#105479=CARTESIAN_POINT('Ctrl Pts',(34.8436783706315,65.8073925040531,12.));
#105480=CARTESIAN_POINT('Ctrl Pts',(34.7642339552035,65.8916543400169,12.));
#105481=CARTESIAN_POINT('Ctrl Pts',(34.6669728017236,65.9427857825597,12.));
#105482=CARTESIAN_POINT('Ctrl Pts',(34.6669728017236,65.9427857825597,12.));
#105483=CARTESIAN_POINT('Ctrl Pts',(34.6669728017236,65.9427857825597,8.));
#105484=CARTESIAN_POINT('Ctrl Pts',(34.6669728017236,65.9427857825597,4.));
#105485=CARTESIAN_POINT('Ctrl Pts',(34.6669728017236,65.9427857825597,0.));
#105486=CARTESIAN_POINT('Ctrl Pts',(34.2579614092497,61.0441813777723,0.));
#105487=CARTESIAN_POINT('Ctrl Pts',(34.2579614092497,61.0441813777723,12.));
#105488=CARTESIAN_POINT('Ctrl Pts',(34.2589297755434,61.0479423318725,0.));
#105489=CARTESIAN_POINT('Ctrl Pts',(34.2589297755434,61.0479423318725,12.));
#105490=CARTESIAN_POINT('Ctrl Pts',(34.2608658001631,61.0554700176998,0.));
#105491=CARTESIAN_POINT('Ctrl Pts',(34.2608658001631,61.0554700176998,12.));
#105492=CARTESIAN_POINT('Ctrl Pts',(34.2637677131934,61.0667788793266,0.));
#105493=CARTESIAN_POINT('Ctrl Pts',(34.2637677131934,61.0667788793266,12.));
#105494=CARTESIAN_POINT('Ctrl Pts',(34.2676326825626,61.0818920286293,0.));
#105495=CARTESIAN_POINT('Ctrl Pts',(34.2676326825626,61.0818920286293,12.));
#105496=CARTESIAN_POINT('Ctrl Pts',(34.2724568037227,61.1008412399997,0.));
#105497=CARTESIAN_POINT('Ctrl Pts',(34.2724568037227,61.1008412399997,12.));
#105498=CARTESIAN_POINT('Ctrl Pts',(34.277273803877,61.1198481997764,0.));
#105499=CARTESIAN_POINT('Ctrl Pts',(34.277273803877,61.1198481997764,12.));
#105500=CARTESIAN_POINT('Ctrl Pts',(34.2820836244469,61.1389128461886,0.));
#105501=CARTESIAN_POINT('Ctrl Pts',(34.2820836244469,61.1389128461886,12.));
#105502=CARTESIAN_POINT('Ctrl Pts',(34.2868861666384,61.1580350635533,0.));
#105503=CARTESIAN_POINT('Ctrl Pts',(34.2868861666384,61.1580350635533,12.));
#105504=CARTESIAN_POINT('Ctrl Pts',(34.2916812929751,61.1772146833205,0.));
#105505=CARTESIAN_POINT('Ctrl Pts',(34.2916812929751,61.1772146833205,12.));
#105506=CARTESIAN_POINT('Ctrl Pts',(34.2964688443663,61.1964515073891,0.));
#105507=CARTESIAN_POINT('Ctrl Pts',(34.2964688443663,61.1964515073891,12.));
#105508=CARTESIAN_POINT('Ctrl Pts',(34.3012486533474,61.2157453259107,0.));
#105509=CARTESIAN_POINT('Ctrl Pts',(34.3012486533474,61.2157453259107,12.));
#105510=CARTESIAN_POINT('Ctrl Pts',(34.3060205584064,61.2350959366939,0.));
#105511=CARTESIAN_POINT('Ctrl Pts',(34.3060205584064,61.2350959366939,12.));
#105512=CARTESIAN_POINT('Ctrl Pts',(34.3107844191043,61.2545031656133,0.));
#105513=CARTESIAN_POINT('Ctrl Pts',(34.3107844191043,61.2545031656133,12.));
#105514=CARTESIAN_POINT('Ctrl Pts',(34.3155401111747,61.2739668600365,0.));
#105515=CARTESIAN_POINT('Ctrl Pts',(34.3155401111747,61.2739668600365,12.));
#105516=CARTESIAN_POINT('Ctrl Pts',(34.3202875193617,61.2934868791855,0.));
#105517=CARTESIAN_POINT('Ctrl Pts',(34.3202875193617,61.2934868791855,12.));
#105518=CARTESIAN_POINT('Ctrl Pts',(34.3250265314768,61.3130630861386,0.));
#105519=CARTESIAN_POINT('Ctrl Pts',(34.3250265314768,61.3130630861386,12.));
#105520=CARTESIAN_POINT('Ctrl Pts',(34.3297570310146,61.3326953378851,0.));
#105521=CARTESIAN_POINT('Ctrl Pts',(34.3297570310146,61.3326953378851,12.));
#105522=CARTESIAN_POINT('Ctrl Pts',(34.3344788934363,61.3523834803188,0.));
#105523=CARTESIAN_POINT('Ctrl Pts',(34.3344788934363,61.3523834803188,12.));
#105524=CARTESIAN_POINT('Ctrl Pts',(34.339191990014,61.3721273534257,0.));
#105525=CARTESIAN_POINT('Ctrl Pts',(34.339191990014,61.3721273534257,12.));
#105526=CARTESIAN_POINT('Ctrl Pts',(34.3438961902405,61.3919267945302,0.));
#105527=CARTESIAN_POINT('Ctrl Pts',(34.3438961902405,61.3919267945302,12.));
#105528=CARTESIAN_POINT('Ctrl Pts',(34.3485913645979,61.4117816420229,0.));
#105529=CARTESIAN_POINT('Ctrl Pts',(34.3485913645979,61.4117816420229,12.));
#105530=CARTESIAN_POINT('Ctrl Pts',(34.3532773877089,61.4316917395918,0.));
#105531=CARTESIAN_POINT('Ctrl Pts',(34.3532773877089,61.4316917395918,12.));
#105532=CARTESIAN_POINT('Ctrl Pts',(34.3579541381996,61.4516569360454,0.));
#105533=CARTESIAN_POINT('Ctrl Pts',(34.3579541381996,61.4516569360454,12.));
#105534=CARTESIAN_POINT('Ctrl Pts',(34.3626214971888,61.4716770832897,0.));
#105535=CARTESIAN_POINT('Ctrl Pts',(34.3626214971888,61.4716770832897,12.));
#105536=CARTESIAN_POINT('Ctrl Pts',(34.3672793472465,61.4917520349278,0.));
#105537=CARTESIAN_POINT('Ctrl Pts',(34.3672793472465,61.4917520349278,12.));
#105538=CARTESIAN_POINT('Ctrl Pts',(34.3719275711195,61.5118816445437,0.));
#105539=CARTESIAN_POINT('Ctrl Pts',(34.3719275711195,61.5118816445437,12.));
#105540=CARTESIAN_POINT('Ctrl Pts',(34.376566050668,61.5320657642638,0.));
#105541=CARTESIAN_POINT('Ctrl Pts',(34.376566050668,61.5320657642638,12.));
#105542=CARTESIAN_POINT('Ctrl Pts',(34.3811946674197,61.5523042455158,0.));
#105543=CARTESIAN_POINT('Ctrl Pts',(34.3811946674197,61.5523042455158,12.));
#105544=CARTESIAN_POINT('Ctrl Pts',(34.3858133030518,61.5725969396829,0.));
#105545=CARTESIAN_POINT('Ctrl Pts',(34.3858133030518,61.5725969396829,12.));
#105546=CARTESIAN_POINT('Ctrl Pts',(34.3904218398636,61.5929436987409,0.));
#105547=CARTESIAN_POINT('Ctrl Pts',(34.3904218398636,61.5929436987409,12.));
#105548=CARTESIAN_POINT('Ctrl Pts',(34.3950201613432,61.6133443760142,0.));
#105549=CARTESIAN_POINT('Ctrl Pts',(34.3950201613432,61.6133443760142,12.));
#105550=CARTESIAN_POINT('Ctrl Pts',(34.3996081523753,61.6337988264556,0.));
#105551=CARTESIAN_POINT('Ctrl Pts',(34.3996081523753,61.6337988264556,12.));
#105552=CARTESIAN_POINT('Ctrl Pts',(34.4041856989316,61.6543069062416,0.));
#105553=CARTESIAN_POINT('Ctrl Pts',(34.4041856989316,61.6543069062416,12.));
#105554=CARTESIAN_POINT('Ctrl Pts',(34.4087526878812,61.6748684725205,0.));
#105555=CARTESIAN_POINT('Ctrl Pts',(34.4087526878812,61.6748684725205,12.));
#105556=CARTESIAN_POINT('Ctrl Pts',(34.4133090067703,61.695483383117,0.));
#105557=CARTESIAN_POINT('Ctrl Pts',(34.4133090067703,61.695483383117,12.));
#105558=CARTESIAN_POINT('Ctrl Pts',(34.4178545435766,61.7161514961915,0.));
#105559=CARTESIAN_POINT('Ctrl Pts',(34.4178545435766,61.7161514961915,12.));
#105560=CARTESIAN_POINT('Ctrl Pts',(34.4223891867179,61.7368726702596,0.));
#105561=CARTESIAN_POINT('Ctrl Pts',(34.4223891867179,61.7368726702596,12.));
#105562=CARTESIAN_POINT('Ctrl Pts',(34.4269128251576,61.7576467643432,0.));
#105563=CARTESIAN_POINT('Ctrl Pts',(34.4269128251576,61.7576467643432,12.));
#105564=CARTESIAN_POINT('Ctrl Pts',(34.4314253484791,61.7784736380727,0.));
#105565=CARTESIAN_POINT('Ctrl Pts',(34.4314253484791,61.7784736380727,12.));
#105566=CARTESIAN_POINT('Ctrl Pts',(34.4359266469749,61.7993531518037,0.));
#105567=CARTESIAN_POINT('Ctrl Pts',(34.4359266469749,61.7993531518037,12.));
#105568=CARTESIAN_POINT('Ctrl Pts',(34.4404166117299,61.8202851667222,0.));
#105569=CARTESIAN_POINT('Ctrl Pts',(34.4404166117299,61.8202851667222,12.));
#105570=CARTESIAN_POINT('Ctrl Pts',(34.4448951345739,61.8412695447926,0.));
#105571=CARTESIAN_POINT('Ctrl Pts',(34.4448951345739,61.8412695447926,12.));
#105572=CARTESIAN_POINT('Ctrl Pts',(34.449362108036,61.8623061487018,0.));
#105573=CARTESIAN_POINT('Ctrl Pts',(34.449362108036,61.8623061487018,12.));
#105574=CARTESIAN_POINT('Ctrl Pts',(34.4538174253012,61.8833948418025,0.));
#105575=CARTESIAN_POINT('Ctrl Pts',(34.4538174253012,61.8833948418025,12.));
#105576=CARTESIAN_POINT('Ctrl Pts',(34.4582609801637,61.9045354880445,0.));
#105577=CARTESIAN_POINT('Ctrl Pts',(34.4582609801637,61.9045354880445,12.));
#105578=CARTESIAN_POINT('Ctrl Pts',(34.4626926669974,61.9257279519308,0.));
#105579=CARTESIAN_POINT('Ctrl Pts',(34.4626926669974,61.9257279519308,12.));
#105580=CARTESIAN_POINT('Ctrl Pts',(34.4671123807717,61.9469720985531,0.));
#105581=CARTESIAN_POINT('Ctrl Pts',(34.4671123807717,61.9469720985531,12.));
#105582=CARTESIAN_POINT('Ctrl Pts',(34.4715200170592,61.9682677936054,0.));
#105583=CARTESIAN_POINT('Ctrl Pts',(34.4715200170592,61.9682677936054,12.));
#105584=CARTESIAN_POINT('Ctrl Pts',(34.4759154720473,61.9896149034001,0.));
#105585=CARTESIAN_POINT('Ctrl Pts',(34.4759154720473,61.9896149034001,12.));
#105586=CARTESIAN_POINT('Ctrl Pts',(34.4802986425528,62.0110132948794,0.));
#105587=CARTESIAN_POINT('Ctrl Pts',(34.4802986425528,62.0110132948794,12.));
#105588=CARTESIAN_POINT('Ctrl Pts',(34.4846694260199,62.0324628356141,0.));
#105589=CARTESIAN_POINT('Ctrl Pts',(34.4846694260199,62.0324628356141,12.));
#105590=CARTESIAN_POINT('Ctrl Pts',(34.4890277205039,62.0539633937939,0.));
#105591=CARTESIAN_POINT('Ctrl Pts',(34.4890277205039,62.0539633937939,12.));
#105592=CARTESIAN_POINT('Ctrl Pts',(34.4933734246592,62.0755148382135,0.));
#105593=CARTESIAN_POINT('Ctrl Pts',(34.4933734246592,62.0755148382135,12.));
#105594=CARTESIAN_POINT('Ctrl Pts',(34.4977064377282,62.0971170382567,0.));
#105595=CARTESIAN_POINT('Ctrl Pts',(34.4977064377282,62.0971170382567,12.));
#105596=CARTESIAN_POINT('Ctrl Pts',(34.5020266595293,62.1187698638707,0.));
#105597=CARTESIAN_POINT('Ctrl Pts',(34.5020266595293,62.1187698638707,12.));
#105598=CARTESIAN_POINT('Ctrl Pts',(34.5063339904533,62.1404731855687,0.));
#105599=CARTESIAN_POINT('Ctrl Pts',(34.5063339904533,62.1404731855687,12.));
#105600=CARTESIAN_POINT('Ctrl Pts',(34.5106283314594,62.1622268744337,0.));
#105601=CARTESIAN_POINT('Ctrl Pts',(34.5106283314594,62.1622268744337,12.));
#105602=CARTESIAN_POINT('Ctrl Pts',(34.5149095840729,62.1840308021171,0.));
#105603=CARTESIAN_POINT('Ctrl Pts',(34.5149095840729,62.1840308021171,12.));
#105604=CARTESIAN_POINT('Ctrl Pts',(34.5191776503843,62.2058848408346,0.));
#105605=CARTESIAN_POINT('Ctrl Pts',(34.5191776503843,62.2058848408346,12.));
#105606=CARTESIAN_POINT('Ctrl Pts',(34.5234324330492,62.2277888633576,0.));
#105607=CARTESIAN_POINT('Ctrl Pts',(34.5234324330492,62.2277888633576,12.));
#105608=CARTESIAN_POINT('Ctrl Pts',(34.527673835281,62.2497427430136,0.));
#105609=CARTESIAN_POINT('Ctrl Pts',(34.527673835281,62.2497427430136,12.));
#105610=CARTESIAN_POINT('Ctrl Pts',(34.5319017608434,62.2717463536828,0.));
#105611=CARTESIAN_POINT('Ctrl Pts',(34.5319017608434,62.2717463536828,12.));
#105612=CARTESIAN_POINT('Ctrl Pts',(34.536116114045,62.2937995697927,0.));
#105613=CARTESIAN_POINT('Ctrl Pts',(34.536116114045,62.2937995697927,12.));
#105614=CARTESIAN_POINT('Ctrl Pts',(34.5403167997333,62.3159022663052,0.));
#105615=CARTESIAN_POINT('Ctrl Pts',(34.5403167997333,62.3159022663052,12.));
#105616=CARTESIAN_POINT('Ctrl Pts',(34.5445037232928,62.3380543187067,0.));
#105617=CARTESIAN_POINT('Ctrl Pts',(34.5445037232928,62.3380543187067,12.));
#105618=CARTESIAN_POINT('Ctrl Pts',(34.5486767906376,62.3602556030114,0.));
#105619=CARTESIAN_POINT('Ctrl Pts',(34.5486767906376,62.3602556030114,12.));
#105620=CARTESIAN_POINT('Ctrl Pts',(34.552835908207,62.3825059957593,0.));
#105621=CARTESIAN_POINT('Ctrl Pts',(34.552835908207,62.3825059957593,12.));
#105622=CARTESIAN_POINT('Ctrl Pts',(34.5569809829615,62.4048053740129,0.));
#105623=CARTESIAN_POINT('Ctrl Pts',(34.5569809829615,62.4048053740129,12.));
#105624=CARTESIAN_POINT('Ctrl Pts',(34.5611119223807,62.4271536153473,0.));
#105625=CARTESIAN_POINT('Ctrl Pts',(34.5611119223807,62.4271536153473,12.));
#105626=CARTESIAN_POINT('Ctrl Pts',(34.5652286344606,62.4495505978415,0.));
#105627=CARTESIAN_POINT('Ctrl Pts',(34.5652286344606,62.4495505978415,12.));
#105628=CARTESIAN_POINT('Ctrl Pts',(34.5693310277064,62.471996200083,0.));
#105629=CARTESIAN_POINT('Ctrl Pts',(34.5693310277064,62.471996200083,12.));
#105630=CARTESIAN_POINT('Ctrl Pts',(34.5734190111279,62.494490301164,0.));
#105631=CARTESIAN_POINT('Ctrl Pts',(34.5734190111279,62.494490301164,12.));
#105632=CARTESIAN_POINT('Ctrl Pts',(34.5774924942351,62.5170327806774,0.));
#105633=CARTESIAN_POINT('Ctrl Pts',(34.5774924942351,62.5170327806774,12.));
#105634=CARTESIAN_POINT('Ctrl Pts',(34.5815513870363,62.5396235187053,0.));
#105635=CARTESIAN_POINT('Ctrl Pts',(34.5815513870363,62.5396235187053,12.));
#105636=CARTESIAN_POINT('Ctrl Pts',(34.5855956000343,62.5622623958125,0.));
#105637=CARTESIAN_POINT('Ctrl Pts',(34.5855956000343,62.5622623958125,12.));
#105638=CARTESIAN_POINT('Ctrl Pts',(34.5896250442199,62.5849492930501,0.));
#105639=CARTESIAN_POINT('Ctrl Pts',(34.5896250442199,62.5849492930501,12.));
#105640=CARTESIAN_POINT('Ctrl Pts',(34.5936396310671,62.6076840919521,0.));
#105641=CARTESIAN_POINT('Ctrl Pts',(34.5936396310671,62.6076840919521,12.));
#105642=CARTESIAN_POINT('Ctrl Pts',(34.5976392725303,62.6304666745319,0.));
#105643=CARTESIAN_POINT('Ctrl Pts',(34.5976392725303,62.6304666745319,12.));
#105644=CARTESIAN_POINT('Ctrl Pts',(34.6016238810419,62.6532969232695,0.));
#105645=CARTESIAN_POINT('Ctrl Pts',(34.6016238810419,62.6532969232695,12.));
#105646=CARTESIAN_POINT('Ctrl Pts',(34.6055933695093,62.6761747211081,0.));
#105647=CARTESIAN_POINT('Ctrl Pts',(34.6055933695093,62.6761747211081,12.));
#105648=CARTESIAN_POINT('Ctrl Pts',(34.6095476513095,62.6990999514597,0.));
#105649=CARTESIAN_POINT('Ctrl Pts',(34.6095476513095,62.6990999514597,12.));
#105650=CARTESIAN_POINT('Ctrl Pts',(34.6134866402842,62.7220724982005,0.));
#105651=CARTESIAN_POINT('Ctrl Pts',(34.6134866402842,62.7220724982005,12.));
#105652=CARTESIAN_POINT('Ctrl Pts',(34.6174102507368,62.7450922456662,0.));
#105653=CARTESIAN_POINT('Ctrl Pts',(34.6174102507368,62.7450922456662,12.));
#105654=CARTESIAN_POINT('Ctrl Pts',(34.6213183974302,62.7681590786398,0.));
#105655=CARTESIAN_POINT('Ctrl Pts',(34.6213183974302,62.7681590786398,12.));
#105656=CARTESIAN_POINT('Ctrl Pts',(34.6252109955836,62.7912728823483,0.));
#105657=CARTESIAN_POINT('Ctrl Pts',(34.6252109955836,62.7912728823483,12.));
#105658=CARTESIAN_POINT('Ctrl Pts',(34.629087960866,62.8144335424671,0.));
#105659=CARTESIAN_POINT('Ctrl Pts',(34.629087960866,62.8144335424671,12.));
#105660=CARTESIAN_POINT('Ctrl Pts',(34.6329492093931,62.8376409451167,0.));
#105661=CARTESIAN_POINT('Ctrl Pts',(34.6329492093931,62.8376409451167,12.));
#105662=CARTESIAN_POINT('Ctrl Pts',(34.6367946577241,62.8608949768583,0.));
#105663=CARTESIAN_POINT('Ctrl Pts',(34.6367946577241,62.8608949768583,12.));
#105664=CARTESIAN_POINT('Ctrl Pts',(34.6406242228606,62.8841955246819,0.));
#105665=CARTESIAN_POINT('Ctrl Pts',(34.6406242228606,62.8841955246819,12.));
#105666=CARTESIAN_POINT('Ctrl Pts',(34.6444378222425,62.9075424760042,0.));
#105667=CARTESIAN_POINT('Ctrl Pts',(34.6444378222425,62.9075424760042,12.));
#105668=CARTESIAN_POINT('Ctrl Pts',(34.6482353737433,62.9309357186733,0.));
#105669=CARTESIAN_POINT('Ctrl Pts',(34.6482353737433,62.9309357186733,12.));
#105670=CARTESIAN_POINT('Ctrl Pts',(34.6520167956656,62.9543751409648,0.));
#105671=CARTESIAN_POINT('Ctrl Pts',(34.6520167956656,62.9543751409648,12.));
#105672=CARTESIAN_POINT('Ctrl Pts',(34.6557820067389,62.9778606315777,0.));
#105673=CARTESIAN_POINT('Ctrl Pts',(34.6557820067389,62.9778606315777,12.));
#105674=CARTESIAN_POINT('Ctrl Pts',(34.6595309261185,63.0013920796225,0.));
#105675=CARTESIAN_POINT('Ctrl Pts',(34.6595309261185,63.0013920796225,12.));
#105676=CARTESIAN_POINT('Ctrl Pts',(34.6632634733819,63.0249693746198,0.));
#105677=CARTESIAN_POINT('Ctrl Pts',(34.6632634733819,63.0249693746198,12.));
#105678=CARTESIAN_POINT('Ctrl Pts',(34.6669795685225,63.0485924065039,0.));
#105679=CARTESIAN_POINT('Ctrl Pts',(34.6669795685225,63.0485924065039,12.));
#105680=CARTESIAN_POINT('Ctrl Pts',(34.670679131947,63.0722610656194,0.));
#105681=CARTESIAN_POINT('Ctrl Pts',(34.670679131947,63.0722610656194,12.));
#105682=CARTESIAN_POINT('Ctrl Pts',(34.6743620844721,63.0959752427169,0.));
#105683=CARTESIAN_POINT('Ctrl Pts',(34.6743620844721,63.0959752427169,12.));
#105684=CARTESIAN_POINT('Ctrl Pts',(34.6780283473252,63.119734828943,0.));
#105685=CARTESIAN_POINT('Ctrl Pts',(34.6780283473252,63.119734828943,12.));
#105686=CARTESIAN_POINT('Ctrl Pts',(34.68167784214,63.1435397158385,0.));
#105687=CARTESIAN_POINT('Ctrl Pts',(34.68167784214,63.1435397158385,12.));
#105688=CARTESIAN_POINT('Ctrl Pts',(34.6853104909516,63.1673897953425,0.));
#105689=CARTESIAN_POINT('Ctrl Pts',(34.6853104909516,63.1673897953425,12.));
#105690=CARTESIAN_POINT('Ctrl Pts',(34.6889262161923,63.1912849597885,0.));
#105691=CARTESIAN_POINT('Ctrl Pts',(34.6889262161923,63.1912849597885,12.));
#105692=CARTESIAN_POINT('Ctrl Pts',(34.6925249406898,63.2152251019014,0.));
#105693=CARTESIAN_POINT('Ctrl Pts',(34.6925249406898,63.2152251019014,12.));
#105694=CARTESIAN_POINT('Ctrl Pts',(34.696106587667,63.2392101147854,0.));
#105695=CARTESIAN_POINT('Ctrl Pts',(34.696106587667,63.2392101147854,12.));
#105696=CARTESIAN_POINT('Ctrl Pts',(34.6996710807384,63.2632398919234,0.));
#105697=CARTESIAN_POINT('Ctrl Pts',(34.6996710807384,63.2632398919234,12.));
#105698=CARTESIAN_POINT('Ctrl Pts',(34.7032183439045,63.2873143271813,0.));
#105699=CARTESIAN_POINT('Ctrl Pts',(34.7032183439045,63.2873143271813,12.));
#105700=CARTESIAN_POINT('Ctrl Pts',(34.7067483015492,63.311433314805,0.));
#105701=CARTESIAN_POINT('Ctrl Pts',(34.7067483015492,63.311433314805,12.));
#105702=CARTESIAN_POINT('Ctrl Pts',(34.7102608784372,63.3355967494169,0.));
#105703=CARTESIAN_POINT('Ctrl Pts',(34.7102608784372,63.3355967494169,12.));
#105704=CARTESIAN_POINT('Ctrl Pts',(34.7137559997143,63.359804526005,0.));
#105705=CARTESIAN_POINT('Ctrl Pts',(34.7137559997143,63.359804526005,12.));
#105706=CARTESIAN_POINT('Ctrl Pts',(34.7172335909037,63.3840565399207,0.));
#105707=CARTESIAN_POINT('Ctrl Pts',(34.7172335909037,63.3840565399207,12.));
#105708=CARTESIAN_POINT('Ctrl Pts',(34.7206935779007,63.4083526868837,0.));
#105709=CARTESIAN_POINT('Ctrl Pts',(34.7206935779007,63.4083526868837,12.));
#105710=CARTESIAN_POINT('Ctrl Pts',(34.7241358869702,63.4326928629797,0.));
#105711=CARTESIAN_POINT('Ctrl Pts',(34.7241358869702,63.4326928629797,12.));
#105712=CARTESIAN_POINT('Ctrl Pts',(34.7275604447438,63.4570769646568,0.));
#105713=CARTESIAN_POINT('Ctrl Pts',(34.7275604447438,63.4570769646568,12.));
#105714=CARTESIAN_POINT('Ctrl Pts',(34.7309671782212,63.481504888716,0.));
#105715=CARTESIAN_POINT('Ctrl Pts',(34.7309671782212,63.481504888716,12.));
#105716=CARTESIAN_POINT('Ctrl Pts',(34.7343560147663,63.5059765323082,0.));
#105717=CARTESIAN_POINT('Ctrl Pts',(34.7343560147663,63.5059765323082,12.));
#105718=CARTESIAN_POINT('Ctrl Pts',(34.7377268821022,63.5304917929378,0.));
#105719=CARTESIAN_POINT('Ctrl Pts',(34.7377268821022,63.5304917929378,12.));
#105720=CARTESIAN_POINT('Ctrl Pts',(34.7410797083079,63.5550505684621,0.));
#105721=CARTESIAN_POINT('Ctrl Pts',(34.7410797083079,63.5550505684621,12.));
#105722=CARTESIAN_POINT('Ctrl Pts',(34.7444144218162,63.5796527570874,0.));
#105723=CARTESIAN_POINT('Ctrl Pts',(34.7444144218162,63.5796527570874,12.));
#105724=CARTESIAN_POINT('Ctrl Pts',(34.7477309514142,63.6042982573599,0.));
#105725=CARTESIAN_POINT('Ctrl Pts',(34.7477309514142,63.6042982573599,12.));
#105726=CARTESIAN_POINT('Ctrl Pts',(34.7510292262415,63.628986968162,0.));
#105727=CARTESIAN_POINT('Ctrl Pts',(34.7510292262415,63.628986968162,12.));
#105728=CARTESIAN_POINT('Ctrl Pts',(34.7543091757841,63.6537187887174,0.));
#105729=CARTESIAN_POINT('Ctrl Pts',(34.7543091757841,63.6537187887174,12.));
#105730=CARTESIAN_POINT('Ctrl Pts',(34.7575707298718,63.6784936185893,0.));
#105731=CARTESIAN_POINT('Ctrl Pts',(34.7575707298718,63.6784936185893,12.));
#105732=CARTESIAN_POINT('Ctrl Pts',(34.7608138186757,63.7033113576782,0.));
#105733=CARTESIAN_POINT('Ctrl Pts',(34.7608138186757,63.7033113576782,12.));
#105734=CARTESIAN_POINT('Ctrl Pts',(34.7640383727094,63.7281719062135,0.));
#105735=CARTESIAN_POINT('Ctrl Pts',(34.7640383727094,63.7281719062135,12.));
#105736=CARTESIAN_POINT('Ctrl Pts',(34.7672443228266,63.7530751647479,0.));
#105737=CARTESIAN_POINT('Ctrl Pts',(34.7672443228266,63.7530751647479,12.));
#105738=CARTESIAN_POINT('Ctrl Pts',(34.7704316002165,63.7780210341619,0.));
#105739=CARTESIAN_POINT('Ctrl Pts',(34.7704316002165,63.7780210341619,12.));
#105740=CARTESIAN_POINT('Ctrl Pts',(34.7736001363991,63.8030094156635,0.));
#105741=CARTESIAN_POINT('Ctrl Pts',(34.7736001363991,63.8030094156635,12.));
#105742=CARTESIAN_POINT('Ctrl Pts',(34.7767498632244,63.8280402107858,0.));
#105743=CARTESIAN_POINT('Ctrl Pts',(34.7767498632244,63.8280402107858,12.));
#105744=CARTESIAN_POINT('Ctrl Pts',(34.7798807128716,63.8531133213794,0.));
#105745=CARTESIAN_POINT('Ctrl Pts',(34.7798807128716,63.8531133213794,12.));
#105746=CARTESIAN_POINT('Ctrl Pts',(34.7829926178495,63.8782286496059,0.));
#105747=CARTESIAN_POINT('Ctrl Pts',(34.7829926178495,63.8782286496059,12.));
#105748=CARTESIAN_POINT('Ctrl Pts',(34.7860855109908,63.9033860979429,0.));
#105749=CARTESIAN_POINT('Ctrl Pts',(34.7860855109908,63.9033860979429,12.));
#105750=CARTESIAN_POINT('Ctrl Pts',(34.7891593254485,63.9285855691839,0.));
#105751=CARTESIAN_POINT('Ctrl Pts',(34.7891593254485,63.9285855691839,12.));
#105752=CARTESIAN_POINT('Ctrl Pts',(34.7922139946943,63.9538269664366,0.));
#105753=CARTESIAN_POINT('Ctrl Pts',(34.7922139946943,63.9538269664366,12.));
#105754=CARTESIAN_POINT('Ctrl Pts',(34.7952494525182,63.9791101931169,0.));
#105755=CARTESIAN_POINT('Ctrl Pts',(34.7952494525182,63.9791101931169,12.));
#105756=CARTESIAN_POINT('Ctrl Pts',(34.79826563303,64.0044351529413,0.));
#105757=CARTESIAN_POINT('Ctrl Pts',(34.79826563303,64.0044351529413,12.));
#105758=CARTESIAN_POINT('Ctrl Pts',(34.8012624706533,64.0298017499305,0.));
#105759=CARTESIAN_POINT('Ctrl Pts',(34.8012624706533,64.0298017499305,12.));
#105760=CARTESIAN_POINT('Ctrl Pts',(34.8042399001214,64.0552098884101,0.));
#105761=CARTESIAN_POINT('Ctrl Pts',(34.8042399001214,64.0552098884101,12.));
#105762=CARTESIAN_POINT('Ctrl Pts',(34.8071978564748,64.0806594730085,0.));
#105763=CARTESIAN_POINT('Ctrl Pts',(34.8071978564748,64.0806594730085,12.));
#105764=CARTESIAN_POINT('Ctrl Pts',(34.8101362750595,64.1061504086512,0.));
#105765=CARTESIAN_POINT('Ctrl Pts',(34.8101362750595,64.1061504086512,12.));
#105766=CARTESIAN_POINT('Ctrl Pts',(34.8130550915284,64.1316826005502,0.));
#105767=CARTESIAN_POINT('Ctrl Pts',(34.8130550915284,64.1316826005502,12.));
#105768=CARTESIAN_POINT('Ctrl Pts',(34.8159542418372,64.1572559542085,0.));
#105769=CARTESIAN_POINT('Ctrl Pts',(34.8159542418372,64.1572559542085,12.));
#105770=CARTESIAN_POINT('Ctrl Pts',(34.8188336622418,64.1828703754237,0.));
#105771=CARTESIAN_POINT('Ctrl Pts',(34.8188336622418,64.1828703754237,12.));
#105772=CARTESIAN_POINT('Ctrl Pts',(34.8216932892969,64.2085257702885,0.));
#105773=CARTESIAN_POINT('Ctrl Pts',(34.8216932892969,64.2085257702885,12.));
#105774=CARTESIAN_POINT('Ctrl Pts',(34.8245330598559,64.2342220451878,0.));
#105775=CARTESIAN_POINT('Ctrl Pts',(34.8245330598559,64.2342220451878,12.));
#105776=CARTESIAN_POINT('Ctrl Pts',(34.8273529110742,64.259959106791,0.));
#105777=CARTESIAN_POINT('Ctrl Pts',(34.8273529110742,64.259959106791,12.));
#105778=CARTESIAN_POINT('Ctrl Pts',(34.8301527804052,64.2857368620513,0.));
#105779=CARTESIAN_POINT('Ctrl Pts',(34.8301527804052,64.2857368620513,12.));
#105780=CARTESIAN_POINT('Ctrl Pts',(34.8329326055916,64.3115552182056,0.));
#105781=CARTESIAN_POINT('Ctrl Pts',(34.8329326055916,64.3115552182056,12.));
#105782=CARTESIAN_POINT('Ctrl Pts',(34.8356923246617,64.3374140827708,0.));
#105783=CARTESIAN_POINT('Ctrl Pts',(34.8356923246617,64.3374140827708,12.));
#105784=CARTESIAN_POINT('Ctrl Pts',(34.8384318759249,64.3633133635385,0.));
#105785=CARTESIAN_POINT('Ctrl Pts',(34.8384318759249,64.3633133635385,12.));
#105786=CARTESIAN_POINT('Ctrl Pts',(34.8411511979705,64.3892529685614,0.));
#105787=CARTESIAN_POINT('Ctrl Pts',(34.8411511979705,64.3892529685614,12.));
#105788=CARTESIAN_POINT('Ctrl Pts',(34.8438502296669,64.4152328061526,0.));
#105789=CARTESIAN_POINT('Ctrl Pts',(34.8438502296669,64.4152328061526,12.));
#105790=CARTESIAN_POINT('Ctrl Pts',(34.8465289101626,64.4412527848979,0.));
#105791=CARTESIAN_POINT('Ctrl Pts',(34.8465289101626,64.4412527848979,12.));
#105792=CARTESIAN_POINT('Ctrl Pts',(34.8491871788898,64.4673128136631,0.));
#105793=CARTESIAN_POINT('Ctrl Pts',(34.8491871788898,64.4673128136631,12.));
#105794=CARTESIAN_POINT('Ctrl Pts',(34.851824975568,64.4934128015983,0.));
#105795=CARTESIAN_POINT('Ctrl Pts',(34.851824975568,64.4934128015983,12.));
#105796=CARTESIAN_POINT('Ctrl Pts',(34.8544422402114,64.5195526581398,0.));
#105797=CARTESIAN_POINT('Ctrl Pts',(34.8544422402114,64.5195526581398,12.));
#105798=CARTESIAN_POINT('Ctrl Pts',(34.8570389131334,64.5457322930074,0.));
#105799=CARTESIAN_POINT('Ctrl Pts',(34.8570389131334,64.5457322930074,12.));
#105800=CARTESIAN_POINT('Ctrl Pts',(34.859614934925,64.5719516161914,0.));
#105801=CARTESIAN_POINT('Ctrl Pts',(34.859614934925,64.5719516161914,12.));
#105802=CARTESIAN_POINT('Ctrl Pts',(34.8621702464397,64.5982105379374,0.));
#105803=CARTESIAN_POINT('Ctrl Pts',(34.8621702464397,64.5982105379374,12.));
#105804=CARTESIAN_POINT('Ctrl Pts',(34.8647047887774,64.6245089687276,0.));
#105805=CARTESIAN_POINT('Ctrl Pts',(34.8647047887774,64.6245089687276,12.));
#105806=CARTESIAN_POINT('Ctrl Pts',(34.8672185032724,64.6508468192609,0.));
#105807=CARTESIAN_POINT('Ctrl Pts',(34.8672185032724,64.6508468192609,12.));
#105808=CARTESIAN_POINT('Ctrl Pts',(34.8697113314797,64.6772240004241,0.));
#105809=CARTESIAN_POINT('Ctrl Pts',(34.8697113314797,64.6772240004241,12.));
#105810=CARTESIAN_POINT('Ctrl Pts',(34.8721832151981,64.7036404233319,0.));
#105811=CARTESIAN_POINT('Ctrl Pts',(34.8721832151981,64.7036404233319,12.));
#105812=CARTESIAN_POINT('Ctrl Pts',(34.8746340964976,64.7300959993662,0.));
#105813=CARTESIAN_POINT('Ctrl Pts',(34.8746340964976,64.7300959993662,12.));
#105814=CARTESIAN_POINT('Ctrl Pts',(34.8770639177494,64.7565906402154,0.));
#105815=CARTESIAN_POINT('Ctrl Pts',(34.8770639177494,64.7565906402154,12.));
#105816=CARTESIAN_POINT('Ctrl Pts',(34.8794726216511,64.7831242579023,0.));
#105817=CARTESIAN_POINT('Ctrl Pts',(34.8794726216511,64.7831242579023,12.));
#105818=CARTESIAN_POINT('Ctrl Pts',(34.8818601512726,64.8096967648299,0.));
#105819=CARTESIAN_POINT('Ctrl Pts',(34.8818601512726,64.8096967648299,12.));
#105820=CARTESIAN_POINT('Ctrl Pts',(34.8842264500184,64.8363080737369,0.));
#105821=CARTESIAN_POINT('Ctrl Pts',(34.8842264500184,64.8363080737369,12.));
#105822=CARTESIAN_POINT('Ctrl Pts',(34.8865714615433,64.8629580976057,0.));
#105823=CARTESIAN_POINT('Ctrl Pts',(34.8865714615433,64.8629580976057,12.));
#105824=CARTESIAN_POINT('Ctrl Pts',(34.8888951296809,64.8896467495755,0.));
#105825=CARTESIAN_POINT('Ctrl Pts',(34.8888951296809,64.8896467495755,12.));
#105826=CARTESIAN_POINT('Ctrl Pts',(34.8911973983785,64.9163739428606,0.));
#105827=CARTESIAN_POINT('Ctrl Pts',(34.8911973983785,64.9163739428606,12.));
#105828=CARTESIAN_POINT('Ctrl Pts',(34.8934782116097,64.9431395906341,0.));
#105829=CARTESIAN_POINT('Ctrl Pts',(34.8934782116097,64.9431395906341,12.));
#105830=CARTESIAN_POINT('Ctrl Pts',(34.8957375133702,64.9699436060178,0.));
#105831=CARTESIAN_POINT('Ctrl Pts',(34.8957375133702,64.9699436060178,12.));
#105832=CARTESIAN_POINT('Ctrl Pts',(34.8979752478623,64.9967859023225,0.));
#105833=CARTESIAN_POINT('Ctrl Pts',(34.8979752478623,64.9967859023225,12.));
#105834=CARTESIAN_POINT('Ctrl Pts',(34.9001913596422,65.0236663932338,0.));
#105835=CARTESIAN_POINT('Ctrl Pts',(34.9001913596422,65.0236663932338,12.));
#105836=CARTESIAN_POINT('Ctrl Pts',(34.9023857937866,65.0505849930173,0.));
#105837=CARTESIAN_POINT('Ctrl Pts',(34.9023857937866,65.0505849930173,12.));
#105838=CARTESIAN_POINT('Ctrl Pts',(34.9045584960503,65.0775416167073,0.));
#105839=CARTESIAN_POINT('Ctrl Pts',(34.9045584960503,65.0775416167073,12.));
#105840=CARTESIAN_POINT('Ctrl Pts',(34.9067094130387,65.1045361803097,0.));
#105841=CARTESIAN_POINT('Ctrl Pts',(34.9067094130387,65.1045361803097,12.));
#105842=CARTESIAN_POINT('Ctrl Pts',(34.9088384918321,65.1315686003485,0.));
#105843=CARTESIAN_POINT('Ctrl Pts',(34.9088384918321,65.1315686003485,12.));
#105844=CARTESIAN_POINT('Ctrl Pts',(34.9109456796201,65.1586387934216,0.));
#105845=CARTESIAN_POINT('Ctrl Pts',(34.9109456796201,65.1586387934216,12.));
#105846=CARTESIAN_POINT('Ctrl Pts',(34.9130309233017,65.1857466757082,0.));
#105847=CARTESIAN_POINT('Ctrl Pts',(34.9130309233017,65.1857466757082,12.));
#105848=CARTESIAN_POINT('Ctrl Pts',(34.9150941691754,65.2128921625838,0.));
#105849=CARTESIAN_POINT('Ctrl Pts',(34.9150941691754,65.2128921625838,12.));
#105850=CARTESIAN_POINT('Ctrl Pts',(34.9171353624131,65.2400751679586,0.));
#105851=CARTESIAN_POINT('Ctrl Pts',(34.9171353624131,65.2400751679586,12.));
#105852=CARTESIAN_POINT('Ctrl Pts',(34.9191544474898,65.2672956048121,0.));
#105853=CARTESIAN_POINT('Ctrl Pts',(34.9191544474898,65.2672956048121,12.));
#105854=CARTESIAN_POINT('Ctrl Pts',(34.921151369138,65.2945533863812,0.));
#105855=CARTESIAN_POINT('Ctrl Pts',(34.921151369138,65.2945533863812,12.));
#105856=CARTESIAN_POINT('Ctrl Pts',(34.9231260731846,65.3218484271941,0.));
#105857=CARTESIAN_POINT('Ctrl Pts',(34.9231260731846,65.3218484271941,12.));
#105858=CARTESIAN_POINT('Ctrl Pts',(34.9250785073473,65.3491806440529,0.));
#105859=CARTESIAN_POINT('Ctrl Pts',(34.9250785073473,65.3491806440529,12.));
#105860=CARTESIAN_POINT('Ctrl Pts',(34.9270086222703,65.3765499573019,0.));
#105861=CARTESIAN_POINT('Ctrl Pts',(34.9270086222703,65.3765499573019,12.));
#105862=CARTESIAN_POINT('Ctrl Pts',(34.92891637177,65.4039562911255,0.));
#105863=CARTESIAN_POINT('Ctrl Pts',(34.92891637177,65.4039562911255,12.));
#105864=CARTESIAN_POINT('Ctrl Pts',(34.9308017105481,65.4313995707423,0.));
#105865=CARTESIAN_POINT('Ctrl Pts',(34.9308017105481,65.4313995707423,12.));
#105866=CARTESIAN_POINT('Ctrl Pts',(34.9326645923897,65.4588797201884,0.));
#105867=CARTESIAN_POINT('Ctrl Pts',(34.9326645923897,65.4588797201884,12.));
#105868=CARTESIAN_POINT('Ctrl Pts',(34.9345049680816,65.4863966597524,0.));
#105869=CARTESIAN_POINT('Ctrl Pts',(34.9345049680816,65.4863966597524,12.));
#105870=CARTESIAN_POINT('Ctrl Pts',(34.9363227836621,65.5139503038116,0.));
#105871=CARTESIAN_POINT('Ctrl Pts',(34.9363227836621,65.5139503038116,12.));
#105872=CARTESIAN_POINT('Ctrl Pts',(34.9381179779763,65.5415405578138,0.));
#105873=CARTESIAN_POINT('Ctrl Pts',(34.9381179779763,65.5415405578138,12.));
#105874=CARTESIAN_POINT('Ctrl Pts',(34.9398904862278,65.5691673226051,0.));
#105875=CARTESIAN_POINT('Ctrl Pts',(34.9398904862278,65.5691673226051,12.));
#105876=CARTESIAN_POINT('Ctrl Pts',(34.9416402443551,65.5968304997821,0.));
#105877=CARTESIAN_POINT('Ctrl Pts',(34.9416402443551,65.5968304997821,12.));
#105878=CARTESIAN_POINT('Ctrl Pts',(34.9433671932982,65.6245299968635,0.));
#105879=CARTESIAN_POINT('Ctrl Pts',(34.9433671932982,65.6245299968635,12.));
#105880=CARTESIAN_POINT('Ctrl Pts',(34.9450712829142,65.652265732124,0.));
#105881=CARTESIAN_POINT('Ctrl Pts',(34.9450712829142,65.652265732124,12.));
#105882=CARTESIAN_POINT('Ctrl Pts',(34.9467524770271,65.6800376405722,0.));
#105883=CARTESIAN_POINT('Ctrl Pts',(34.9467524770271,65.6800376405722,12.));
#105884=CARTESIAN_POINT('Ctrl Pts',(34.9484107543857,65.707845675746,0.));
#105885=CARTESIAN_POINT('Ctrl Pts',(34.9484107543857,65.707845675746,12.));
#105886=CARTESIAN_POINT('Ctrl Pts',(34.9500461042919,65.7356898060478,0.));
#105887=CARTESIAN_POINT('Ctrl Pts',(34.9500461042919,65.7356898060478,12.));
#105888=CARTESIAN_POINT('Ctrl Pts',(34.9513360397181,65.757993971173,0.));
#105889=CARTESIAN_POINT('Ctrl Pts',(34.9513360397181,65.757993971173,12.));
#105890=CARTESIAN_POINT('Ctrl Pts',(34.9522931728594,65.7747383250775,0.));
#105891=CARTESIAN_POINT('Ctrl Pts',(34.9522931728594,65.7747383250775,12.));
#105892=CARTESIAN_POINT('Ctrl Pts',(34.9529266758405,65.7859084407494,0.));
#105893=CARTESIAN_POINT('Ctrl Pts',(34.9529266758405,65.7859084407494,12.));
#105894=CARTESIAN_POINT('Ctrl Pts',(34.9532422808861,65.7914953018525,0.));
#105895=CARTESIAN_POINT('Ctrl Pts',(34.9532422808861,65.7914953018525,12.));
#105896=CARTESIAN_POINT('',(34.2579614092497,61.0441813777723,0.));
#105897=CARTESIAN_POINT('Ctrl Pts',(34.2579614092497,61.0441813777723,0.));
#105898=CARTESIAN_POINT('Ctrl Pts',(34.2589297755434,61.0479423318725,0.));
#105899=CARTESIAN_POINT('Ctrl Pts',(34.2608658001631,61.0554700176998,0.));
#105900=CARTESIAN_POINT('Ctrl Pts',(34.2637677131934,61.0667788793266,0.));
#105901=CARTESIAN_POINT('Ctrl Pts',(34.2676326825626,61.0818920286293,0.));
#105902=CARTESIAN_POINT('Ctrl Pts',(34.2724568037227,61.1008412399997,0.));
#105903=CARTESIAN_POINT('Ctrl Pts',(34.277273803877,61.1198481997764,0.));
#105904=CARTESIAN_POINT('Ctrl Pts',(34.2820836244469,61.1389128461886,0.));
#105905=CARTESIAN_POINT('Ctrl Pts',(34.2868861666384,61.1580350635533,0.));
#105906=CARTESIAN_POINT('Ctrl Pts',(34.2916812929751,61.1772146833205,0.));
#105907=CARTESIAN_POINT('Ctrl Pts',(34.2964688443663,61.1964515073891,0.));
#105908=CARTESIAN_POINT('Ctrl Pts',(34.3012486533474,61.2157453259107,0.));
#105909=CARTESIAN_POINT('Ctrl Pts',(34.3060205584064,61.2350959366939,0.));
#105910=CARTESIAN_POINT('Ctrl Pts',(34.3107844191043,61.2545031656133,0.));
#105911=CARTESIAN_POINT('Ctrl Pts',(34.3155401111747,61.2739668600365,0.));
#105912=CARTESIAN_POINT('Ctrl Pts',(34.3202875193617,61.2934868791855,0.));
#105913=CARTESIAN_POINT('Ctrl Pts',(34.3250265314768,61.3130630861386,0.));
#105914=CARTESIAN_POINT('Ctrl Pts',(34.3297570310146,61.3326953378851,0.));
#105915=CARTESIAN_POINT('Ctrl Pts',(34.3344788934363,61.3523834803188,0.));
#105916=CARTESIAN_POINT('Ctrl Pts',(34.339191990014,61.3721273534257,0.));
#105917=CARTESIAN_POINT('Ctrl Pts',(34.3438961902405,61.3919267945302,0.));
#105918=CARTESIAN_POINT('Ctrl Pts',(34.3485913645979,61.4117816420229,0.));
#105919=CARTESIAN_POINT('Ctrl Pts',(34.3532773877089,61.4316917395918,0.));
#105920=CARTESIAN_POINT('Ctrl Pts',(34.3579541381996,61.4516569360454,0.));
#105921=CARTESIAN_POINT('Ctrl Pts',(34.3626214971888,61.4716770832897,0.));
#105922=CARTESIAN_POINT('Ctrl Pts',(34.3672793472465,61.4917520349278,0.));
#105923=CARTESIAN_POINT('Ctrl Pts',(34.3719275711195,61.5118816445437,0.));
#105924=CARTESIAN_POINT('Ctrl Pts',(34.376566050668,61.5320657642638,0.));
#105925=CARTESIAN_POINT('Ctrl Pts',(34.3811946674197,61.5523042455158,0.));
#105926=CARTESIAN_POINT('Ctrl Pts',(34.3858133030518,61.5725969396829,0.));
#105927=CARTESIAN_POINT('Ctrl Pts',(34.3904218398636,61.5929436987409,0.));
#105928=CARTESIAN_POINT('Ctrl Pts',(34.3950201613432,61.6133443760142,0.));
#105929=CARTESIAN_POINT('Ctrl Pts',(34.3996081523753,61.6337988264556,0.));
#105930=CARTESIAN_POINT('Ctrl Pts',(34.4041856989316,61.6543069062416,0.));
#105931=CARTESIAN_POINT('Ctrl Pts',(34.4087526878812,61.6748684725205,0.));
#105932=CARTESIAN_POINT('Ctrl Pts',(34.4133090067703,61.695483383117,0.));
#105933=CARTESIAN_POINT('Ctrl Pts',(34.4178545435766,61.7161514961915,0.));
#105934=CARTESIAN_POINT('Ctrl Pts',(34.4223891867179,61.7368726702596,0.));
#105935=CARTESIAN_POINT('Ctrl Pts',(34.4269128251576,61.7576467643432,0.));
#105936=CARTESIAN_POINT('Ctrl Pts',(34.4314253484791,61.7784736380727,0.));
#105937=CARTESIAN_POINT('Ctrl Pts',(34.4359266469749,61.7993531518037,0.));
#105938=CARTESIAN_POINT('Ctrl Pts',(34.4404166117299,61.8202851667222,0.));
#105939=CARTESIAN_POINT('Ctrl Pts',(34.4448951345739,61.8412695447926,0.));
#105940=CARTESIAN_POINT('Ctrl Pts',(34.449362108036,61.8623061487018,0.));
#105941=CARTESIAN_POINT('Ctrl Pts',(34.4538174253012,61.8833948418025,0.));
#105942=CARTESIAN_POINT('Ctrl Pts',(34.4582609801637,61.9045354880445,0.));
#105943=CARTESIAN_POINT('Ctrl Pts',(34.4626926669974,61.9257279519308,0.));
#105944=CARTESIAN_POINT('Ctrl Pts',(34.4671123807717,61.9469720985531,0.));
#105945=CARTESIAN_POINT('Ctrl Pts',(34.4715200170592,61.9682677936054,0.));
#105946=CARTESIAN_POINT('Ctrl Pts',(34.4759154720473,61.9896149034001,0.));
#105947=CARTESIAN_POINT('Ctrl Pts',(34.4802986425528,62.0110132948794,0.));
#105948=CARTESIAN_POINT('Ctrl Pts',(34.4846694260199,62.0324628356141,0.));
#105949=CARTESIAN_POINT('Ctrl Pts',(34.4890277205039,62.0539633937939,0.));
#105950=CARTESIAN_POINT('Ctrl Pts',(34.4933734246592,62.0755148382135,0.));
#105951=CARTESIAN_POINT('Ctrl Pts',(34.4977064377282,62.0971170382567,0.));
#105952=CARTESIAN_POINT('Ctrl Pts',(34.5020266595293,62.1187698638707,0.));
#105953=CARTESIAN_POINT('Ctrl Pts',(34.5063339904533,62.1404731855687,0.));
#105954=CARTESIAN_POINT('Ctrl Pts',(34.5106283314594,62.1622268744337,0.));
#105955=CARTESIAN_POINT('Ctrl Pts',(34.5149095840729,62.1840308021171,0.));
#105956=CARTESIAN_POINT('Ctrl Pts',(34.5191776503843,62.2058848408346,0.));
#105957=CARTESIAN_POINT('Ctrl Pts',(34.5234324330492,62.2277888633576,0.));
#105958=CARTESIAN_POINT('Ctrl Pts',(34.527673835281,62.2497427430136,0.));
#105959=CARTESIAN_POINT('Ctrl Pts',(34.5319017608434,62.2717463536828,0.));
#105960=CARTESIAN_POINT('Ctrl Pts',(34.536116114045,62.2937995697927,0.));
#105961=CARTESIAN_POINT('Ctrl Pts',(34.5403167997333,62.3159022663052,0.));
#105962=CARTESIAN_POINT('Ctrl Pts',(34.5445037232928,62.3380543187067,0.));
#105963=CARTESIAN_POINT('Ctrl Pts',(34.5486767906376,62.3602556030114,0.));
#105964=CARTESIAN_POINT('Ctrl Pts',(34.552835908207,62.3825059957593,0.));
#105965=CARTESIAN_POINT('Ctrl Pts',(34.5569809829615,62.4048053740129,0.));
#105966=CARTESIAN_POINT('Ctrl Pts',(34.5611119223807,62.4271536153473,0.));
#105967=CARTESIAN_POINT('Ctrl Pts',(34.5652286344606,62.4495505978415,0.));
#105968=CARTESIAN_POINT('Ctrl Pts',(34.5693310277064,62.471996200083,0.));
#105969=CARTESIAN_POINT('Ctrl Pts',(34.5734190111279,62.494490301164,0.));
#105970=CARTESIAN_POINT('Ctrl Pts',(34.5774924942351,62.5170327806774,0.));
#105971=CARTESIAN_POINT('Ctrl Pts',(34.5815513870363,62.5396235187053,0.));
#105972=CARTESIAN_POINT('Ctrl Pts',(34.5855956000343,62.5622623958125,0.));
#105973=CARTESIAN_POINT('Ctrl Pts',(34.5896250442199,62.5849492930501,0.));
#105974=CARTESIAN_POINT('Ctrl Pts',(34.5936396310671,62.6076840919521,0.));
#105975=CARTESIAN_POINT('Ctrl Pts',(34.5976392725303,62.6304666745319,0.));
#105976=CARTESIAN_POINT('Ctrl Pts',(34.6016238810419,62.6532969232695,0.));
#105977=CARTESIAN_POINT('Ctrl Pts',(34.6055933695093,62.6761747211081,0.));
#105978=CARTESIAN_POINT('Ctrl Pts',(34.6095476513095,62.6990999514597,0.));
#105979=CARTESIAN_POINT('Ctrl Pts',(34.6134866402842,62.7220724982005,0.));
#105980=CARTESIAN_POINT('Ctrl Pts',(34.6174102507368,62.7450922456662,0.));
#105981=CARTESIAN_POINT('Ctrl Pts',(34.6213183974302,62.7681590786398,0.));
#105982=CARTESIAN_POINT('Ctrl Pts',(34.6252109955836,62.7912728823483,0.));
#105983=CARTESIAN_POINT('Ctrl Pts',(34.629087960866,62.8144335424671,0.));
#105984=CARTESIAN_POINT('Ctrl Pts',(34.6329492093931,62.8376409451167,0.));
#105985=CARTESIAN_POINT('Ctrl Pts',(34.6367946577241,62.8608949768583,0.));
#105986=CARTESIAN_POINT('Ctrl Pts',(34.6406242228606,62.8841955246819,0.));
#105987=CARTESIAN_POINT('Ctrl Pts',(34.6444378222425,62.9075424760042,0.));
#105988=CARTESIAN_POINT('Ctrl Pts',(34.6482353737433,62.9309357186733,0.));
#105989=CARTESIAN_POINT('Ctrl Pts',(34.6520167956656,62.9543751409648,0.));
#105990=CARTESIAN_POINT('Ctrl Pts',(34.6557820067389,62.9778606315777,0.));
#105991=CARTESIAN_POINT('Ctrl Pts',(34.6595309261185,63.0013920796225,0.));
#105992=CARTESIAN_POINT('Ctrl Pts',(34.6632634733819,63.0249693746198,0.));
#105993=CARTESIAN_POINT('Ctrl Pts',(34.6669795685225,63.0485924065039,0.));
#105994=CARTESIAN_POINT('Ctrl Pts',(34.670679131947,63.0722610656194,0.));
#105995=CARTESIAN_POINT('Ctrl Pts',(34.6743620844721,63.0959752427169,0.));
#105996=CARTESIAN_POINT('Ctrl Pts',(34.6780283473252,63.119734828943,0.));
#105997=CARTESIAN_POINT('Ctrl Pts',(34.68167784214,63.1435397158385,0.));
#105998=CARTESIAN_POINT('Ctrl Pts',(34.6853104909516,63.1673897953425,0.));
#105999=CARTESIAN_POINT('Ctrl Pts',(34.6889262161923,63.1912849597885,0.));
#106000=CARTESIAN_POINT('Ctrl Pts',(34.6925249406898,63.2152251019014,0.));
#106001=CARTESIAN_POINT('Ctrl Pts',(34.696106587667,63.2392101147854,0.));
#106002=CARTESIAN_POINT('Ctrl Pts',(34.6996710807384,63.2632398919234,0.));
#106003=CARTESIAN_POINT('Ctrl Pts',(34.7032183439045,63.2873143271813,0.));
#106004=CARTESIAN_POINT('Ctrl Pts',(34.7067483015492,63.311433314805,0.));
#106005=CARTESIAN_POINT('Ctrl Pts',(34.7102608784372,63.3355967494169,0.));
#106006=CARTESIAN_POINT('Ctrl Pts',(34.7137559997143,63.359804526005,0.));
#106007=CARTESIAN_POINT('Ctrl Pts',(34.7172335909037,63.3840565399207,0.));
#106008=CARTESIAN_POINT('Ctrl Pts',(34.7206935779007,63.4083526868837,0.));
#106009=CARTESIAN_POINT('Ctrl Pts',(34.7241358869702,63.4326928629797,0.));
#106010=CARTESIAN_POINT('Ctrl Pts',(34.7275604447438,63.4570769646568,0.));
#106011=CARTESIAN_POINT('Ctrl Pts',(34.7309671782212,63.481504888716,0.));
#106012=CARTESIAN_POINT('Ctrl Pts',(34.7343560147663,63.5059765323082,0.));
#106013=CARTESIAN_POINT('Ctrl Pts',(34.7377268821022,63.5304917929378,0.));
#106014=CARTESIAN_POINT('Ctrl Pts',(34.7410797083079,63.5550505684621,0.));
#106015=CARTESIAN_POINT('Ctrl Pts',(34.7444144218162,63.5796527570874,0.));
#106016=CARTESIAN_POINT('Ctrl Pts',(34.7477309514142,63.6042982573599,0.));
#106017=CARTESIAN_POINT('Ctrl Pts',(34.7510292262415,63.628986968162,0.));
#106018=CARTESIAN_POINT('Ctrl Pts',(34.7543091757841,63.6537187887174,0.));
#106019=CARTESIAN_POINT('Ctrl Pts',(34.7575707298718,63.6784936185893,0.));
#106020=CARTESIAN_POINT('Ctrl Pts',(34.7608138186757,63.7033113576782,0.));
#106021=CARTESIAN_POINT('Ctrl Pts',(34.7640383727094,63.7281719062135,0.));
#106022=CARTESIAN_POINT('Ctrl Pts',(34.7672443228266,63.7530751647479,0.));
#106023=CARTESIAN_POINT('Ctrl Pts',(34.7704316002165,63.7780210341619,0.));
#106024=CARTESIAN_POINT('Ctrl Pts',(34.7736001363991,63.8030094156635,0.));
#106025=CARTESIAN_POINT('Ctrl Pts',(34.7767498632244,63.8280402107858,0.));
#106026=CARTESIAN_POINT('Ctrl Pts',(34.7798807128716,63.8531133213794,0.));
#106027=CARTESIAN_POINT('Ctrl Pts',(34.7829926178495,63.8782286496059,0.));
#106028=CARTESIAN_POINT('Ctrl Pts',(34.7860855109908,63.9033860979429,0.));
#106029=CARTESIAN_POINT('Ctrl Pts',(34.7891593254485,63.9285855691839,0.));
#106030=CARTESIAN_POINT('Ctrl Pts',(34.7922139946943,63.9538269664366,0.));
#106031=CARTESIAN_POINT('Ctrl Pts',(34.7952494525182,63.9791101931169,0.));
#106032=CARTESIAN_POINT('Ctrl Pts',(34.79826563303,64.0044351529413,0.));
#106033=CARTESIAN_POINT('Ctrl Pts',(34.8012624706533,64.0298017499305,0.));
#106034=CARTESIAN_POINT('Ctrl Pts',(34.8042399001214,64.0552098884101,0.));
#106035=CARTESIAN_POINT('Ctrl Pts',(34.8071978564748,64.0806594730085,0.));
#106036=CARTESIAN_POINT('Ctrl Pts',(34.8101362750595,64.1061504086512,0.));
#106037=CARTESIAN_POINT('Ctrl Pts',(34.8130550915284,64.1316826005502,0.));
#106038=CARTESIAN_POINT('Ctrl Pts',(34.8159542418372,64.1572559542085,0.));
#106039=CARTESIAN_POINT('Ctrl Pts',(34.8188336622418,64.1828703754237,0.));
#106040=CARTESIAN_POINT('Ctrl Pts',(34.8216932892969,64.2085257702885,0.));
#106041=CARTESIAN_POINT('Ctrl Pts',(34.8245330598559,64.2342220451878,0.));
#106042=CARTESIAN_POINT('Ctrl Pts',(34.8273529110742,64.259959106791,0.));
#106043=CARTESIAN_POINT('Ctrl Pts',(34.8301527804052,64.2857368620513,0.));
#106044=CARTESIAN_POINT('Ctrl Pts',(34.8329326055916,64.3115552182056,0.));
#106045=CARTESIAN_POINT('Ctrl Pts',(34.8356923246617,64.3374140827708,0.));
#106046=CARTESIAN_POINT('Ctrl Pts',(34.8384318759249,64.3633133635385,0.));
#106047=CARTESIAN_POINT('Ctrl Pts',(34.8411511979705,64.3892529685614,0.));
#106048=CARTESIAN_POINT('Ctrl Pts',(34.8438502296669,64.4152328061526,0.));
#106049=CARTESIAN_POINT('Ctrl Pts',(34.8465289101626,64.4412527848979,0.));
#106050=CARTESIAN_POINT('Ctrl Pts',(34.8491871788898,64.4673128136631,0.));
#106051=CARTESIAN_POINT('Ctrl Pts',(34.851824975568,64.4934128015983,0.));
#106052=CARTESIAN_POINT('Ctrl Pts',(34.8544422402114,64.5195526581398,0.));
#106053=CARTESIAN_POINT('Ctrl Pts',(34.8570389131334,64.5457322930074,0.));
#106054=CARTESIAN_POINT('Ctrl Pts',(34.859614934925,64.5719516161914,0.));
#106055=CARTESIAN_POINT('Ctrl Pts',(34.8621702464397,64.5982105379374,0.));
#106056=CARTESIAN_POINT('Ctrl Pts',(34.8647047887774,64.6245089687276,0.));
#106057=CARTESIAN_POINT('Ctrl Pts',(34.8672185032724,64.6508468192609,0.));
#106058=CARTESIAN_POINT('Ctrl Pts',(34.8697113314797,64.6772240004241,0.));
#106059=CARTESIAN_POINT('Ctrl Pts',(34.8721832151981,64.7036404233319,0.));
#106060=CARTESIAN_POINT('Ctrl Pts',(34.8746340964976,64.7300959993662,0.));
#106061=CARTESIAN_POINT('Ctrl Pts',(34.8770639177494,64.7565906402154,0.));
#106062=CARTESIAN_POINT('Ctrl Pts',(34.8794726216511,64.7831242579023,0.));
#106063=CARTESIAN_POINT('Ctrl Pts',(34.8818601512726,64.8096967648299,0.));
#106064=CARTESIAN_POINT('Ctrl Pts',(34.8842264500184,64.8363080737369,0.));
#106065=CARTESIAN_POINT('Ctrl Pts',(34.8865714615433,64.8629580976057,0.));
#106066=CARTESIAN_POINT('Ctrl Pts',(34.8888951296809,64.8896467495755,0.));
#106067=CARTESIAN_POINT('Ctrl Pts',(34.8911973983785,64.9163739428606,0.));
#106068=CARTESIAN_POINT('Ctrl Pts',(34.8934782116097,64.9431395906341,0.));
#106069=CARTESIAN_POINT('Ctrl Pts',(34.8957375133702,64.9699436060178,0.));
#106070=CARTESIAN_POINT('Ctrl Pts',(34.8979752478623,64.9967859023225,0.));
#106071=CARTESIAN_POINT('Ctrl Pts',(34.9001913596422,65.0236663932338,0.));
#106072=CARTESIAN_POINT('Ctrl Pts',(34.9023857937866,65.0505849930173,0.));
#106073=CARTESIAN_POINT('Ctrl Pts',(34.9045584960503,65.0775416167073,0.));
#106074=CARTESIAN_POINT('Ctrl Pts',(34.9067094130387,65.1045361803097,0.));
#106075=CARTESIAN_POINT('Ctrl Pts',(34.9088384918321,65.1315686003485,0.));
#106076=CARTESIAN_POINT('Ctrl Pts',(34.9109456796201,65.1586387934216,0.));
#106077=CARTESIAN_POINT('Ctrl Pts',(34.9130309233017,65.1857466757082,0.));
#106078=CARTESIAN_POINT('Ctrl Pts',(34.9150941691754,65.2128921625838,0.));
#106079=CARTESIAN_POINT('Ctrl Pts',(34.9171353624131,65.2400751679586,0.));
#106080=CARTESIAN_POINT('Ctrl Pts',(34.9191544474898,65.2672956048121,0.));
#106081=CARTESIAN_POINT('Ctrl Pts',(34.921151369138,65.2945533863812,0.));
#106082=CARTESIAN_POINT('Ctrl Pts',(34.9231260731846,65.3218484271941,0.));
#106083=CARTESIAN_POINT('Ctrl Pts',(34.9250785073473,65.3491806440529,0.));
#106084=CARTESIAN_POINT('Ctrl Pts',(34.9270086222703,65.3765499573019,0.));
#106085=CARTESIAN_POINT('Ctrl Pts',(34.92891637177,65.4039562911255,0.));
#106086=CARTESIAN_POINT('Ctrl Pts',(34.9305324724386,65.4274804996405,0.));
#106087=CARTESIAN_POINT('Ctrl Pts',(34.9317593813102,65.4455359574998,0.));
#106088=CARTESIAN_POINT('Ctrl Pts',(34.9326070346591,65.4581063193582,0.));
#106089=CARTESIAN_POINT('Ctrl Pts',(34.9330820191483,65.4651808010449,0.));
#106090=CARTESIAN_POINT('Ctrl Pts',(34.9331875523085,65.4667541477953,0.));
#106091=CARTESIAN_POINT('',(34.2579614092497,61.0441813777723,12.));
#106092=CARTESIAN_POINT('',(34.2579614092497,61.0441813777723,0.));
#106093=CARTESIAN_POINT('Ctrl Pts',(34.9331875523085,65.4667541477952,12.));
#106094=CARTESIAN_POINT('Ctrl Pts',(34.9330820191483,65.4651808010449,12.));
#106095=CARTESIAN_POINT('Ctrl Pts',(34.9326070346591,65.4581063193582,12.));
#106096=CARTESIAN_POINT('Ctrl Pts',(34.9317593813102,65.4455359574998,12.));
#106097=CARTESIAN_POINT('Ctrl Pts',(34.9305324724386,65.4274804996405,12.));
#106098=CARTESIAN_POINT('Ctrl Pts',(34.92891637177,65.4039562911255,12.));
#106099=CARTESIAN_POINT('Ctrl Pts',(34.9270086222703,65.3765499573019,12.));
#106100=CARTESIAN_POINT('Ctrl Pts',(34.9250785073473,65.3491806440529,12.));
#106101=CARTESIAN_POINT('Ctrl Pts',(34.9231260731846,65.3218484271941,12.));
#106102=CARTESIAN_POINT('Ctrl Pts',(34.921151369138,65.2945533863812,12.));
#106103=CARTESIAN_POINT('Ctrl Pts',(34.9191544474898,65.2672956048121,12.));
#106104=CARTESIAN_POINT('Ctrl Pts',(34.9171353624131,65.2400751679586,12.));
#106105=CARTESIAN_POINT('Ctrl Pts',(34.9150941691754,65.2128921625838,12.));
#106106=CARTESIAN_POINT('Ctrl Pts',(34.9130309233017,65.1857466757082,12.));
#106107=CARTESIAN_POINT('Ctrl Pts',(34.9109456796201,65.1586387934216,12.));
#106108=CARTESIAN_POINT('Ctrl Pts',(34.9088384918321,65.1315686003485,12.));
#106109=CARTESIAN_POINT('Ctrl Pts',(34.9067094130387,65.1045361803097,12.));
#106110=CARTESIAN_POINT('Ctrl Pts',(34.9045584960503,65.0775416167073,12.));
#106111=CARTESIAN_POINT('Ctrl Pts',(34.9023857937866,65.0505849930173,12.));
#106112=CARTESIAN_POINT('Ctrl Pts',(34.9001913596422,65.0236663932338,12.));
#106113=CARTESIAN_POINT('Ctrl Pts',(34.8979752478623,64.9967859023225,12.));
#106114=CARTESIAN_POINT('Ctrl Pts',(34.8957375133702,64.9699436060178,12.));
#106115=CARTESIAN_POINT('Ctrl Pts',(34.8934782116097,64.9431395906341,12.));
#106116=CARTESIAN_POINT('Ctrl Pts',(34.8911973983785,64.9163739428606,12.));
#106117=CARTESIAN_POINT('Ctrl Pts',(34.8888951296809,64.8896467495755,12.));
#106118=CARTESIAN_POINT('Ctrl Pts',(34.8865714615433,64.8629580976057,12.));
#106119=CARTESIAN_POINT('Ctrl Pts',(34.8842264500184,64.8363080737369,12.));
#106120=CARTESIAN_POINT('Ctrl Pts',(34.8818601512726,64.8096967648299,12.));
#106121=CARTESIAN_POINT('Ctrl Pts',(34.8794726216511,64.7831242579023,12.));
#106122=CARTESIAN_POINT('Ctrl Pts',(34.8770639177494,64.7565906402154,12.));
#106123=CARTESIAN_POINT('Ctrl Pts',(34.8746340964976,64.7300959993662,12.));
#106124=CARTESIAN_POINT('Ctrl Pts',(34.8721832151981,64.7036404233319,12.));
#106125=CARTESIAN_POINT('Ctrl Pts',(34.8697113314797,64.6772240004241,12.));
#106126=CARTESIAN_POINT('Ctrl Pts',(34.8672185032724,64.6508468192609,12.));
#106127=CARTESIAN_POINT('Ctrl Pts',(34.8647047887774,64.6245089687276,12.));
#106128=CARTESIAN_POINT('Ctrl Pts',(34.8621702464397,64.5982105379374,12.));
#106129=CARTESIAN_POINT('Ctrl Pts',(34.859614934925,64.5719516161914,12.));
#106130=CARTESIAN_POINT('Ctrl Pts',(34.8570389131334,64.5457322930074,12.));
#106131=CARTESIAN_POINT('Ctrl Pts',(34.8544422402114,64.5195526581398,12.));
#106132=CARTESIAN_POINT('Ctrl Pts',(34.851824975568,64.4934128015983,12.));
#106133=CARTESIAN_POINT('Ctrl Pts',(34.8491871788898,64.4673128136631,12.));
#106134=CARTESIAN_POINT('Ctrl Pts',(34.8465289101626,64.4412527848979,12.));
#106135=CARTESIAN_POINT('Ctrl Pts',(34.8438502296669,64.4152328061526,12.));
#106136=CARTESIAN_POINT('Ctrl Pts',(34.8411511979705,64.3892529685614,12.));
#106137=CARTESIAN_POINT('Ctrl Pts',(34.8384318759249,64.3633133635385,12.));
#106138=CARTESIAN_POINT('Ctrl Pts',(34.8356923246617,64.3374140827708,12.));
#106139=CARTESIAN_POINT('Ctrl Pts',(34.8329326055916,64.3115552182056,12.));
#106140=CARTESIAN_POINT('Ctrl Pts',(34.8301527804052,64.2857368620513,12.));
#106141=CARTESIAN_POINT('Ctrl Pts',(34.8273529110742,64.259959106791,12.));
#106142=CARTESIAN_POINT('Ctrl Pts',(34.8245330598559,64.2342220451878,12.));
#106143=CARTESIAN_POINT('Ctrl Pts',(34.8216932892969,64.2085257702885,12.));
#106144=CARTESIAN_POINT('Ctrl Pts',(34.8188336622418,64.1828703754237,12.));
#106145=CARTESIAN_POINT('Ctrl Pts',(34.8159542418372,64.1572559542085,12.));
#106146=CARTESIAN_POINT('Ctrl Pts',(34.8130550915284,64.1316826005502,12.));
#106147=CARTESIAN_POINT('Ctrl Pts',(34.8101362750595,64.1061504086512,12.));
#106148=CARTESIAN_POINT('Ctrl Pts',(34.8071978564748,64.0806594730085,12.));
#106149=CARTESIAN_POINT('Ctrl Pts',(34.8042399001214,64.0552098884101,12.));
#106150=CARTESIAN_POINT('Ctrl Pts',(34.8012624706533,64.0298017499305,12.));
#106151=CARTESIAN_POINT('Ctrl Pts',(34.79826563303,64.0044351529413,12.));
#106152=CARTESIAN_POINT('Ctrl Pts',(34.7952494525182,63.9791101931169,12.));
#106153=CARTESIAN_POINT('Ctrl Pts',(34.7922139946943,63.9538269664366,12.));
#106154=CARTESIAN_POINT('Ctrl Pts',(34.7891593254485,63.9285855691839,12.));
#106155=CARTESIAN_POINT('Ctrl Pts',(34.7860855109908,63.9033860979429,12.));
#106156=CARTESIAN_POINT('Ctrl Pts',(34.7829926178495,63.8782286496059,12.));
#106157=CARTESIAN_POINT('Ctrl Pts',(34.7798807128716,63.8531133213794,12.));
#106158=CARTESIAN_POINT('Ctrl Pts',(34.7767498632244,63.8280402107858,12.));
#106159=CARTESIAN_POINT('Ctrl Pts',(34.7736001363991,63.8030094156635,12.));
#106160=CARTESIAN_POINT('Ctrl Pts',(34.7704316002165,63.7780210341619,12.));
#106161=CARTESIAN_POINT('Ctrl Pts',(34.7672443228266,63.7530751647479,12.));
#106162=CARTESIAN_POINT('Ctrl Pts',(34.7640383727094,63.7281719062135,12.));
#106163=CARTESIAN_POINT('Ctrl Pts',(34.7608138186757,63.7033113576782,12.));
#106164=CARTESIAN_POINT('Ctrl Pts',(34.7575707298718,63.6784936185893,12.));
#106165=CARTESIAN_POINT('Ctrl Pts',(34.7543091757841,63.6537187887174,12.));
#106166=CARTESIAN_POINT('Ctrl Pts',(34.7510292262415,63.628986968162,12.));
#106167=CARTESIAN_POINT('Ctrl Pts',(34.7477309514142,63.6042982573599,12.));
#106168=CARTESIAN_POINT('Ctrl Pts',(34.7444144218162,63.5796527570874,12.));
#106169=CARTESIAN_POINT('Ctrl Pts',(34.7410797083079,63.5550505684621,12.));
#106170=CARTESIAN_POINT('Ctrl Pts',(34.7377268821022,63.5304917929378,12.));
#106171=CARTESIAN_POINT('Ctrl Pts',(34.7343560147663,63.5059765323082,12.));
#106172=CARTESIAN_POINT('Ctrl Pts',(34.7309671782212,63.481504888716,12.));
#106173=CARTESIAN_POINT('Ctrl Pts',(34.7275604447438,63.4570769646568,12.));
#106174=CARTESIAN_POINT('Ctrl Pts',(34.7241358869702,63.4326928629797,12.));
#106175=CARTESIAN_POINT('Ctrl Pts',(34.7206935779007,63.4083526868837,12.));
#106176=CARTESIAN_POINT('Ctrl Pts',(34.7172335909037,63.3840565399207,12.));
#106177=CARTESIAN_POINT('Ctrl Pts',(34.7137559997143,63.359804526005,12.));
#106178=CARTESIAN_POINT('Ctrl Pts',(34.7102608784372,63.3355967494169,12.));
#106179=CARTESIAN_POINT('Ctrl Pts',(34.7067483015492,63.311433314805,12.));
#106180=CARTESIAN_POINT('Ctrl Pts',(34.7032183439045,63.2873143271813,12.));
#106181=CARTESIAN_POINT('Ctrl Pts',(34.6996710807384,63.2632398919234,12.));
#106182=CARTESIAN_POINT('Ctrl Pts',(34.696106587667,63.2392101147854,12.));
#106183=CARTESIAN_POINT('Ctrl Pts',(34.6925249406898,63.2152251019014,12.));
#106184=CARTESIAN_POINT('Ctrl Pts',(34.6889262161923,63.1912849597885,12.));
#106185=CARTESIAN_POINT('Ctrl Pts',(34.6853104909516,63.1673897953425,12.));
#106186=CARTESIAN_POINT('Ctrl Pts',(34.68167784214,63.1435397158385,12.));
#106187=CARTESIAN_POINT('Ctrl Pts',(34.6780283473252,63.119734828943,12.));
#106188=CARTESIAN_POINT('Ctrl Pts',(34.6743620844721,63.0959752427169,12.));
#106189=CARTESIAN_POINT('Ctrl Pts',(34.670679131947,63.0722610656194,12.));
#106190=CARTESIAN_POINT('Ctrl Pts',(34.6669795685225,63.0485924065039,12.));
#106191=CARTESIAN_POINT('Ctrl Pts',(34.6632634733819,63.0249693746198,12.));
#106192=CARTESIAN_POINT('Ctrl Pts',(34.6595309261185,63.0013920796225,12.));
#106193=CARTESIAN_POINT('Ctrl Pts',(34.6557820067389,62.9778606315777,12.));
#106194=CARTESIAN_POINT('Ctrl Pts',(34.6520167956656,62.9543751409648,12.));
#106195=CARTESIAN_POINT('Ctrl Pts',(34.6482353737433,62.9309357186733,12.));
#106196=CARTESIAN_POINT('Ctrl Pts',(34.6444378222425,62.9075424760042,12.));
#106197=CARTESIAN_POINT('Ctrl Pts',(34.6406242228606,62.8841955246819,12.));
#106198=CARTESIAN_POINT('Ctrl Pts',(34.6367946577241,62.8608949768583,12.));
#106199=CARTESIAN_POINT('Ctrl Pts',(34.6329492093931,62.8376409451167,12.));
#106200=CARTESIAN_POINT('Ctrl Pts',(34.629087960866,62.8144335424671,12.));
#106201=CARTESIAN_POINT('Ctrl Pts',(34.6252109955836,62.7912728823483,12.));
#106202=CARTESIAN_POINT('Ctrl Pts',(34.6213183974302,62.7681590786398,12.));
#106203=CARTESIAN_POINT('Ctrl Pts',(34.6174102507368,62.7450922456662,12.));
#106204=CARTESIAN_POINT('Ctrl Pts',(34.6134866402842,62.7220724982005,12.));
#106205=CARTESIAN_POINT('Ctrl Pts',(34.6095476513095,62.6990999514597,12.));
#106206=CARTESIAN_POINT('Ctrl Pts',(34.6055933695093,62.6761747211081,12.));
#106207=CARTESIAN_POINT('Ctrl Pts',(34.6016238810419,62.6532969232695,12.));
#106208=CARTESIAN_POINT('Ctrl Pts',(34.5976392725303,62.6304666745319,12.));
#106209=CARTESIAN_POINT('Ctrl Pts',(34.5936396310671,62.6076840919521,12.));
#106210=CARTESIAN_POINT('Ctrl Pts',(34.5896250442199,62.5849492930501,12.));
#106211=CARTESIAN_POINT('Ctrl Pts',(34.5855956000343,62.5622623958125,12.));
#106212=CARTESIAN_POINT('Ctrl Pts',(34.5815513870363,62.5396235187053,12.));
#106213=CARTESIAN_POINT('Ctrl Pts',(34.5774924942351,62.5170327806774,12.));
#106214=CARTESIAN_POINT('Ctrl Pts',(34.5734190111279,62.494490301164,12.));
#106215=CARTESIAN_POINT('Ctrl Pts',(34.5693310277064,62.471996200083,12.));
#106216=CARTESIAN_POINT('Ctrl Pts',(34.5652286344606,62.4495505978415,12.));
#106217=CARTESIAN_POINT('Ctrl Pts',(34.5611119223807,62.4271536153473,12.));
#106218=CARTESIAN_POINT('Ctrl Pts',(34.5569809829615,62.4048053740129,12.));
#106219=CARTESIAN_POINT('Ctrl Pts',(34.552835908207,62.3825059957593,12.));
#106220=CARTESIAN_POINT('Ctrl Pts',(34.5486767906376,62.3602556030114,12.));
#106221=CARTESIAN_POINT('Ctrl Pts',(34.5445037232928,62.3380543187067,12.));
#106222=CARTESIAN_POINT('Ctrl Pts',(34.5403167997333,62.3159022663052,12.));
#106223=CARTESIAN_POINT('Ctrl Pts',(34.536116114045,62.2937995697927,12.));
#106224=CARTESIAN_POINT('Ctrl Pts',(34.5319017608434,62.2717463536828,12.));
#106225=CARTESIAN_POINT('Ctrl Pts',(34.527673835281,62.2497427430136,12.));
#106226=CARTESIAN_POINT('Ctrl Pts',(34.5234324330492,62.2277888633576,12.));
#106227=CARTESIAN_POINT('Ctrl Pts',(34.5191776503843,62.2058848408346,12.));
#106228=CARTESIAN_POINT('Ctrl Pts',(34.5149095840729,62.1840308021171,12.));
#106229=CARTESIAN_POINT('Ctrl Pts',(34.5106283314594,62.1622268744337,12.));
#106230=CARTESIAN_POINT('Ctrl Pts',(34.5063339904533,62.1404731855687,12.));
#106231=CARTESIAN_POINT('Ctrl Pts',(34.5020266595293,62.1187698638707,12.));
#106232=CARTESIAN_POINT('Ctrl Pts',(34.4977064377282,62.0971170382567,12.));
#106233=CARTESIAN_POINT('Ctrl Pts',(34.4933734246592,62.0755148382135,12.));
#106234=CARTESIAN_POINT('Ctrl Pts',(34.4890277205039,62.0539633937939,12.));
#106235=CARTESIAN_POINT('Ctrl Pts',(34.4846694260199,62.0324628356141,12.));
#106236=CARTESIAN_POINT('Ctrl Pts',(34.4802986425528,62.0110132948794,12.));
#106237=CARTESIAN_POINT('Ctrl Pts',(34.4759154720473,61.9896149034001,12.));
#106238=CARTESIAN_POINT('Ctrl Pts',(34.4715200170592,61.9682677936054,12.));
#106239=CARTESIAN_POINT('Ctrl Pts',(34.4671123807717,61.9469720985531,12.));
#106240=CARTESIAN_POINT('Ctrl Pts',(34.4626926669974,61.9257279519308,12.));
#106241=CARTESIAN_POINT('Ctrl Pts',(34.4582609801637,61.9045354880445,12.));
#106242=CARTESIAN_POINT('Ctrl Pts',(34.4538174253012,61.8833948418025,12.));
#106243=CARTESIAN_POINT('Ctrl Pts',(34.449362108036,61.8623061487018,12.));
#106244=CARTESIAN_POINT('Ctrl Pts',(34.4448951345739,61.8412695447926,12.));
#106245=CARTESIAN_POINT('Ctrl Pts',(34.4404166117299,61.8202851667222,12.));
#106246=CARTESIAN_POINT('Ctrl Pts',(34.4359266469749,61.7993531518037,12.));
#106247=CARTESIAN_POINT('Ctrl Pts',(34.4314253484791,61.7784736380727,12.));
#106248=CARTESIAN_POINT('Ctrl Pts',(34.4269128251576,61.7576467643432,12.));
#106249=CARTESIAN_POINT('Ctrl Pts',(34.4223891867179,61.7368726702596,12.));
#106250=CARTESIAN_POINT('Ctrl Pts',(34.4178545435766,61.7161514961915,12.));
#106251=CARTESIAN_POINT('Ctrl Pts',(34.4133090067703,61.695483383117,12.));
#106252=CARTESIAN_POINT('Ctrl Pts',(34.4087526878812,61.6748684725205,12.));
#106253=CARTESIAN_POINT('Ctrl Pts',(34.4041856989316,61.6543069062416,12.));
#106254=CARTESIAN_POINT('Ctrl Pts',(34.3996081523753,61.6337988264556,12.));
#106255=CARTESIAN_POINT('Ctrl Pts',(34.3950201613432,61.6133443760142,12.));
#106256=CARTESIAN_POINT('Ctrl Pts',(34.3904218398636,61.5929436987409,12.));
#106257=CARTESIAN_POINT('Ctrl Pts',(34.3858133030518,61.5725969396829,12.));
#106258=CARTESIAN_POINT('Ctrl Pts',(34.3811946674197,61.5523042455158,12.));
#106259=CARTESIAN_POINT('Ctrl Pts',(34.376566050668,61.5320657642638,12.));
#106260=CARTESIAN_POINT('Ctrl Pts',(34.3719275711195,61.5118816445437,12.));
#106261=CARTESIAN_POINT('Ctrl Pts',(34.3672793472465,61.4917520349278,12.));
#106262=CARTESIAN_POINT('Ctrl Pts',(34.3626214971888,61.4716770832897,12.));
#106263=CARTESIAN_POINT('Ctrl Pts',(34.3579541381996,61.4516569360454,12.));
#106264=CARTESIAN_POINT('Ctrl Pts',(34.3532773877089,61.4316917395918,12.));
#106265=CARTESIAN_POINT('Ctrl Pts',(34.3485913645979,61.4117816420229,12.));
#106266=CARTESIAN_POINT('Ctrl Pts',(34.3438961902405,61.3919267945302,12.));
#106267=CARTESIAN_POINT('Ctrl Pts',(34.339191990014,61.3721273534257,12.));
#106268=CARTESIAN_POINT('Ctrl Pts',(34.3344788934363,61.3523834803188,12.));
#106269=CARTESIAN_POINT('Ctrl Pts',(34.3297570310146,61.3326953378851,12.));
#106270=CARTESIAN_POINT('Ctrl Pts',(34.3250265314768,61.3130630861386,12.));
#106271=CARTESIAN_POINT('Ctrl Pts',(34.3202875193617,61.2934868791855,12.));
#106272=CARTESIAN_POINT('Ctrl Pts',(34.3155401111747,61.2739668600365,12.));
#106273=CARTESIAN_POINT('Ctrl Pts',(34.3107844191043,61.2545031656133,12.));
#106274=CARTESIAN_POINT('Ctrl Pts',(34.3060205584064,61.2350959366939,12.));
#106275=CARTESIAN_POINT('Ctrl Pts',(34.3012486533474,61.2157453259107,12.));
#106276=CARTESIAN_POINT('Ctrl Pts',(34.2964688443663,61.1964515073891,12.));
#106277=CARTESIAN_POINT('Ctrl Pts',(34.2916812929751,61.1772146833205,12.));
#106278=CARTESIAN_POINT('Ctrl Pts',(34.2868861666384,61.1580350635533,12.));
#106279=CARTESIAN_POINT('Ctrl Pts',(34.2820836244469,61.1389128461886,12.));
#106280=CARTESIAN_POINT('Ctrl Pts',(34.277273803877,61.1198481997764,12.));
#106281=CARTESIAN_POINT('Ctrl Pts',(34.2724568037227,61.1008412399997,12.));
#106282=CARTESIAN_POINT('Ctrl Pts',(34.2676326825626,61.0818920286293,12.));
#106283=CARTESIAN_POINT('Ctrl Pts',(34.2637677131934,61.0667788793266,12.));
#106284=CARTESIAN_POINT('Ctrl Pts',(34.2608658001631,61.0554700176998,12.));
#106285=CARTESIAN_POINT('Ctrl Pts',(34.2589297755434,61.0479423318725,12.));
#106286=CARTESIAN_POINT('Ctrl Pts',(34.2579614092497,61.0441813777723,12.));
#106287=CARTESIAN_POINT('Ctrl Pts',(33.5903722665274,66.1657795405958,-1.11022302462516E-15));
#106288=CARTESIAN_POINT('Ctrl Pts',(33.5903722665274,66.1657795405958,4.));
#106289=CARTESIAN_POINT('Ctrl Pts',(33.5903722665274,66.1657795405958,8.));
#106290=CARTESIAN_POINT('Ctrl Pts',(33.5903722665274,66.1657795405958,12.));
#106291=CARTESIAN_POINT('Ctrl Pts',(33.6759628819914,66.2346881970577,-1.11022302462516E-15));
#106292=CARTESIAN_POINT('Ctrl Pts',(33.6759628819914,66.2346881970577,4.));
#106293=CARTESIAN_POINT('Ctrl Pts',(33.6759628819914,66.2346881970577,8.));
#106294=CARTESIAN_POINT('Ctrl Pts',(33.6759628819914,66.2346881970577,12.));
#106295=CARTESIAN_POINT('Ctrl Pts',(33.8665453669327,66.3036153738441,-1.11022302462516E-15));
#106296=CARTESIAN_POINT('Ctrl Pts',(33.8665453669327,66.3036153738441,4.00000000000001));
#106297=CARTESIAN_POINT('Ctrl Pts',(33.8665453669327,66.3036153738441,7.99999999999999));
#106298=CARTESIAN_POINT('Ctrl Pts',(33.8665453669327,66.3036153738441,12.));
#106299=CARTESIAN_POINT('Ctrl Pts',(34.0597557125855,66.2585076236399,-1.11022302462516E-15));
#106300=CARTESIAN_POINT('Ctrl Pts',(34.0597557125855,66.2585076236399,4.));
#106301=CARTESIAN_POINT('Ctrl Pts',(34.0597557125855,66.2585076236399,8.00000000000001));
#106302=CARTESIAN_POINT('Ctrl Pts',(34.0597557125855,66.2585076236399,12.));
#106303=CARTESIAN_POINT('Ctrl Pts',(34.1330090612009,66.220749712065,-1.11022302462516E-15));
#106304=CARTESIAN_POINT('Ctrl Pts',(34.1330090612009,66.220749712065,4.));
#106305=CARTESIAN_POINT('Ctrl Pts',(34.1330090612009,66.220749712065,8.));
#106306=CARTESIAN_POINT('Ctrl Pts',(34.1330090612009,66.220749712065,12.));
#106307=CARTESIAN_POINT('',(33.5903722665274,66.1657795405958,0.));
#106308=CARTESIAN_POINT('',(34.133009061201,66.2207497120651,0.));
#106309=CARTESIAN_POINT('Ctrl Pts',(33.5903722665274,66.1657795405958,0.));
#106310=CARTESIAN_POINT('Ctrl Pts',(33.6759628819914,66.2346881970577,-7.70371977754894E-31));
#106311=CARTESIAN_POINT('Ctrl Pts',(33.7848671591007,66.2740751552214,6.16297582203915E-31));
#106312=CARTESIAN_POINT('Ctrl Pts',(33.894629513177,66.2762262188575,3.08148791101958E-31));
#106313=CARTESIAN_POINT('Ctrl Pts',(33.9769512787343,66.2778395165845,-6.16297582203913E-32));
#106314=CARTESIAN_POINT('Ctrl Pts',(34.0597557125855,66.2585076236399,-1.4482993181792E-30));
#106315=CARTESIAN_POINT('Ctrl Pts',(34.1330090612009,66.220749712065,-6.16297582203914E-32));
#106316=CARTESIAN_POINT('',(34.133009061201,66.2207497120651,12.));
#106317=CARTESIAN_POINT('Ctrl Pts',(34.1330090612009,66.220749712065,-1.11022302462516E-15));
#106318=CARTESIAN_POINT('Ctrl Pts',(34.1330090612009,66.220749712065,4.));
#106319=CARTESIAN_POINT('Ctrl Pts',(34.1330090612009,66.220749712065,8.));
#106320=CARTESIAN_POINT('Ctrl Pts',(34.1330090612009,66.220749712065,12.));
#106321=CARTESIAN_POINT('',(33.5903722665274,66.1657795405958,12.));
#106322=CARTESIAN_POINT('Ctrl Pts',(34.1330090612009,66.220749712065,12.));
#106323=CARTESIAN_POINT('Ctrl Pts',(34.0597557125855,66.2585076236399,12.));
#106324=CARTESIAN_POINT('Ctrl Pts',(33.9769512787343,66.2778395165845,12.));
#106325=CARTESIAN_POINT('Ctrl Pts',(33.894629513177,66.2762262188575,12.));
#106326=CARTESIAN_POINT('Ctrl Pts',(33.7848671591007,66.2740751552214,12.));
#106327=CARTESIAN_POINT('Ctrl Pts',(33.6759628819914,66.2346881970577,12.));
#106328=CARTESIAN_POINT('Ctrl Pts',(33.5903722665274,66.1657795405958,12.));
#106329=CARTESIAN_POINT('Ctrl Pts',(33.5903722665274,66.1657795405958,12.));
#106330=CARTESIAN_POINT('Ctrl Pts',(33.5903722665274,66.1657795405958,8.));
#106331=CARTESIAN_POINT('Ctrl Pts',(33.5903722665274,66.1657795405958,4.));
#106332=CARTESIAN_POINT('Ctrl Pts',(33.5903722665274,66.1657795405958,-1.11022302462516E-15));
#106333=CARTESIAN_POINT('Origin',(1.72995545227681E-10,3.3253631270614E-10,
0.));
#106334=CARTESIAN_POINT('Origin',(1.72995545227681E-10,3.3253631270614E-10,
12.));
#106335=CARTESIAN_POINT('Origin',(1.72995545227681E-10,3.3253631270614E-10,
0.));
#106336=CARTESIAN_POINT('Ctrl Pts',(40.2823469776964,62.6704278106387,-5.55111512312578E-16));
#106337=CARTESIAN_POINT('Ctrl Pts',(40.2823469776964,62.6704278106387,4.));
#106338=CARTESIAN_POINT('Ctrl Pts',(40.2823469776964,62.6704278106387,8.));
#106339=CARTESIAN_POINT('Ctrl Pts',(40.2823469776964,62.6704278106387,12.));
#106340=CARTESIAN_POINT('Ctrl Pts',(40.3747816242709,62.6110140705997,-5.55111512312578E-16));
#106341=CARTESIAN_POINT('Ctrl Pts',(40.3747816242709,62.6110140705997,4.));
#106342=CARTESIAN_POINT('Ctrl Pts',(40.3747816242709,62.6110140705997,8.00000000000001));
#106343=CARTESIAN_POINT('Ctrl Pts',(40.3747816242709,62.6110140705997,12.));
#106344=CARTESIAN_POINT('Ctrl Pts',(40.5004281293558,62.4519997852059,-5.55111512312578E-16));
#106345=CARTESIAN_POINT('Ctrl Pts',(40.5004281293558,62.4519997852059,4.));
#106346=CARTESIAN_POINT('Ctrl Pts',(40.5004281293558,62.4519997852059,7.99999999999999));
#106347=CARTESIAN_POINT('Ctrl Pts',(40.5004281293558,62.4519997852059,12.));
#106348=CARTESIAN_POINT('Ctrl Pts',(40.5187208145704,62.2544389573108,-5.55111512312578E-16));
#106349=CARTESIAN_POINT('Ctrl Pts',(40.5187208145704,62.2544389573108,4.));
#106350=CARTESIAN_POINT('Ctrl Pts',(40.5187208145704,62.2544389573108,8.00000000000001));
#106351=CARTESIAN_POINT('Ctrl Pts',(40.5187208145704,62.2544389573108,12.));
#106352=CARTESIAN_POINT('Ctrl Pts',(40.5060598100835,62.1730054756444,-5.55111512312578E-16));
#106353=CARTESIAN_POINT('Ctrl Pts',(40.5060598100835,62.1730054756444,4.));
#106354=CARTESIAN_POINT('Ctrl Pts',(40.5060598100835,62.1730054756444,8.));
#106355=CARTESIAN_POINT('Ctrl Pts',(40.5060598100835,62.1730054756444,12.));
#106356=CARTESIAN_POINT('',(40.2823469776964,62.6704278106387,0.));
#106357=CARTESIAN_POINT('',(40.5060598100837,62.1730054756444,2.77555756156289E-16));
#106358=CARTESIAN_POINT('Ctrl Pts',(40.2823469776964,62.6704278106387,-1.38777878078145E-16));
#106359=CARTESIAN_POINT('Ctrl Pts',(40.3747816242709,62.6110140705997,-1.38777878078145E-16));
#106360=CARTESIAN_POINT('Ctrl Pts',(40.4465796271766,62.5201487646603,-1.38777878078144E-16));
#106361=CARTESIAN_POINT('Ctrl Pts',(40.4833233215531,62.4166968325982,-1.38777878078145E-16));
#106362=CARTESIAN_POINT('Ctrl Pts',(40.5108810923356,62.3391078835515,-1.38777878078145E-16));
#106363=CARTESIAN_POINT('Ctrl Pts',(40.5187208145704,62.2544389573108,-1.38777878078145E-16));
#106364=CARTESIAN_POINT('Ctrl Pts',(40.5060598100835,62.1730054756444,-1.38777878078145E-16));
#106365=CARTESIAN_POINT('',(40.5060598100837,62.1730054756444,12.));
#106366=CARTESIAN_POINT('Ctrl Pts',(40.5060598100835,62.1730054756444,-5.55111512312578E-16));
#106367=CARTESIAN_POINT('Ctrl Pts',(40.5060598100835,62.1730054756444,4.));
#106368=CARTESIAN_POINT('Ctrl Pts',(40.5060598100835,62.1730054756444,8.));
#106369=CARTESIAN_POINT('Ctrl Pts',(40.5060598100835,62.1730054756444,12.));
#106370=CARTESIAN_POINT('',(40.2823469776964,62.6704278106387,12.));
#106371=CARTESIAN_POINT('Ctrl Pts',(40.5060598100835,62.1730054756444,12.));
#106372=CARTESIAN_POINT('Ctrl Pts',(40.5187208145704,62.2544389573108,12.));
#106373=CARTESIAN_POINT('Ctrl Pts',(40.5108810923356,62.3391078835515,12.));
#106374=CARTESIAN_POINT('Ctrl Pts',(40.4833233215531,62.4166968325982,12.));
#106375=CARTESIAN_POINT('Ctrl Pts',(40.4465796271766,62.5201487646603,12.));
#106376=CARTESIAN_POINT('Ctrl Pts',(40.3747816242709,62.6110140705997,12.));
#106377=CARTESIAN_POINT('Ctrl Pts',(40.2823469776964,62.6704278106387,12.));
#106378=CARTESIAN_POINT('Ctrl Pts',(40.2823469776964,62.6704278106387,12.));
#106379=CARTESIAN_POINT('Ctrl Pts',(40.2823469776964,62.6704278106387,8.));
#106380=CARTESIAN_POINT('Ctrl Pts',(40.2823469776964,62.6704278106387,4.));
#106381=CARTESIAN_POINT('Ctrl Pts',(40.2823469776964,62.6704278106387,-5.55111512312578E-16));
#106382=CARTESIAN_POINT('Ctrl Pts',(39.4479504917287,57.8261117662439,0.));
#106383=CARTESIAN_POINT('Ctrl Pts',(39.4479504917287,57.8261117662439,12.));
#106384=CARTESIAN_POINT('Ctrl Pts',(39.4492429618443,57.8297740100947,0.));
#106385=CARTESIAN_POINT('Ctrl Pts',(39.4492429618443,57.8297740100947,12.));
#106386=CARTESIAN_POINT('Ctrl Pts',(39.4518277003553,57.8371043151411,0.));
#106387=CARTESIAN_POINT('Ctrl Pts',(39.4518277003553,57.8371043151411,12.));
#106388=CARTESIAN_POINT('Ctrl Pts',(39.4557042029652,57.8481172247496,0.));
#106389=CARTESIAN_POINT('Ctrl Pts',(39.4557042029652,57.8481172247496,12.));
#106390=CARTESIAN_POINT('Ctrl Pts',(39.4608716627117,57.8628360096803,0.));
#106391=CARTESIAN_POINT('Ctrl Pts',(39.4608716627117,57.8628360096803,12.));
#106392=CARTESIAN_POINT('Ctrl Pts',(39.4673289592259,57.8812926637177,0.));
#106393=CARTESIAN_POINT('Ctrl Pts',(39.4673289592259,57.8812926637177,12.));
#106394=CARTESIAN_POINT('Ctrl Pts',(39.473784194937,57.8998074670478,0.));
#106395=CARTESIAN_POINT('Ctrl Pts',(39.473784194937,57.8998074670478,12.));
#106396=CARTESIAN_POINT('Ctrl Pts',(39.4802373061058,57.9183803632404,0.));
#106397=CARTESIAN_POINT('Ctrl Pts',(39.4802373061058,57.9183803632404,12.));
#106398=CARTESIAN_POINT('Ctrl Pts',(39.4866881842317,57.9370112456631,0.));
#106399=CARTESIAN_POINT('Ctrl Pts',(39.4866881842317,57.9370112456631,12.));
#106400=CARTESIAN_POINT('Ctrl Pts',(39.4931366776714,57.9556999583892,0.));
#106401=CARTESIAN_POINT('Ctrl Pts',(39.4931366776714,57.9556999583892,12.));
#106402=CARTESIAN_POINT('Ctrl Pts',(39.499582610674,57.974446317937,0.));
#106403=CARTESIAN_POINT('Ctrl Pts',(39.499582610674,57.974446317937,12.));
#106404=CARTESIAN_POINT('Ctrl Pts',(39.5060257981225,57.9932501298522,0.));
#106405=CARTESIAN_POINT('Ctrl Pts',(39.5060257981225,57.9932501298522,12.));
#106406=CARTESIAN_POINT('Ctrl Pts',(39.5124660614976,58.0121112067896,0.));
#106407=CARTESIAN_POINT('Ctrl Pts',(39.5124660614976,58.0121112067896,12.));
#106408=CARTESIAN_POINT('Ctrl Pts',(39.5189032457184,58.0310293875262,0.));
#106409=CARTESIAN_POINT('Ctrl Pts',(39.5189032457184,58.0310293875262,12.));
#106410=CARTESIAN_POINT('Ctrl Pts',(39.5253372136887,58.0500045308412,0.));
#106411=CARTESIAN_POINT('Ctrl Pts',(39.5253372136887,58.0500045308412,12.));
#106412=CARTESIAN_POINT('Ctrl Pts',(39.5317678383217,58.0690365065374,0.));
#106413=CARTESIAN_POINT('Ctrl Pts',(39.5317678383217,58.0690365065374,12.));
#106414=CARTESIAN_POINT('Ctrl Pts',(39.5381949959221,58.0881251879921,0.));
#106415=CARTESIAN_POINT('Ctrl Pts',(39.5381949959221,58.0881251879921,12.));
#106416=CARTESIAN_POINT('Ctrl Pts',(39.5446185579638,58.1072704428928,0.));
#106417=CARTESIAN_POINT('Ctrl Pts',(39.5446185579638,58.1072704428928,12.));
#106418=CARTESIAN_POINT('Ctrl Pts',(39.5510383869505,58.126472128574,0.));
#106419=CARTESIAN_POINT('Ctrl Pts',(39.5510383869505,58.126472128574,12.));
#106420=CARTESIAN_POINT('Ctrl Pts',(39.5574543406981,58.1457300968499,0.));
#106421=CARTESIAN_POINT('Ctrl Pts',(39.5574543406981,58.1457300968499,12.));
#106422=CARTESIAN_POINT('Ctrl Pts',(39.563866275018,58.1650441970387,0.));
#106423=CARTESIAN_POINT('Ctrl Pts',(39.563866275018,58.1650441970387,12.));
#106424=CARTESIAN_POINT('Ctrl Pts',(39.5702740467999,58.1844142794338,0.));
#106425=CARTESIAN_POINT('Ctrl Pts',(39.5702740467999,58.1844142794338,12.));
#106426=CARTESIAN_POINT('Ctrl Pts',(39.57667751752,58.2038401992457,0.));
#106427=CARTESIAN_POINT('Ctrl Pts',(39.57667751752,58.2038401992457,12.));
#106428=CARTESIAN_POINT('Ctrl Pts',(39.5830765530891,58.2233218164366,0.));
#106429=CARTESIAN_POINT('Ctrl Pts',(39.5830765530891,58.2233218164366,12.));
#106430=CARTESIAN_POINT('Ctrl Pts',(39.5894710221713,58.2428589938369,0.));
#106431=CARTESIAN_POINT('Ctrl Pts',(39.5894710221713,58.2428589938369,12.));
#106432=CARTESIAN_POINT('Ctrl Pts',(39.5958607950239,58.2624515958419,0.));
#106433=CARTESIAN_POINT('Ctrl Pts',(39.5958607950239,58.2624515958419,12.));
#106434=CARTESIAN_POINT('Ctrl Pts',(39.6022457420789,58.2820994868118,0.));
#106435=CARTESIAN_POINT('Ctrl Pts',(39.6022457420789,58.2820994868118,12.));
#106436=CARTESIAN_POINT('Ctrl Pts',(39.6086257327583,58.3018025297324,0.));
#106437=CARTESIAN_POINT('Ctrl Pts',(39.6086257327583,58.3018025297324,12.));
#106438=CARTESIAN_POINT('Ctrl Pts',(39.6150006360914,58.3215605869221,0.));
#106439=CARTESIAN_POINT('Ctrl Pts',(39.6150006360914,58.3215605869221,12.));
#106440=CARTESIAN_POINT('Ctrl Pts',(39.6213703212531,58.3413735206424,0.));
#106441=CARTESIAN_POINT('Ctrl Pts',(39.6213703212531,58.3413735206424,12.));
#106442=CARTESIAN_POINT('Ctrl Pts',(39.6277346580892,58.3612411936905,0.));
#106443=CARTESIAN_POINT('Ctrl Pts',(39.6277346580892,58.3612411936905,12.));
#106444=CARTESIAN_POINT('Ctrl Pts',(39.6340935177476,58.3811634701037,0.));
#106445=CARTESIAN_POINT('Ctrl Pts',(39.6340935177476,58.3811634701037,12.));
#106446=CARTESIAN_POINT('Ctrl Pts',(39.6404467729094,58.4011402154196,0.));
#106447=CARTESIAN_POINT('Ctrl Pts',(39.6404467729094,58.4011402154196,12.));
#106448=CARTESIAN_POINT('Ctrl Pts',(39.6467942974451,58.4211712963004,0.));
#106449=CARTESIAN_POINT('Ctrl Pts',(39.6467942974451,58.4211712963004,12.));
#106450=CARTESIAN_POINT('Ctrl Pts',(39.653135966204,58.4412565802979,0.));
#106451=CARTESIAN_POINT('Ctrl Pts',(39.653135966204,58.4412565802979,12.));
#106452=CARTESIAN_POINT('Ctrl Pts',(39.6594716547689,58.4613959355788,0.));
#106453=CARTESIAN_POINT('Ctrl Pts',(39.6594716547689,58.4613959355788,12.));
#106454=CARTESIAN_POINT('Ctrl Pts',(39.6658012391815,58.4815892306066,0.));
#106455=CARTESIAN_POINT('Ctrl Pts',(39.6658012391815,58.4815892306066,12.));
#106456=CARTESIAN_POINT('Ctrl Pts',(39.6721245959531,58.5018363341604,0.));
#106457=CARTESIAN_POINT('Ctrl Pts',(39.6721245959531,58.5018363341604,12.));
#106458=CARTESIAN_POINT('Ctrl Pts',(39.6784416021826,58.5221371154761,0.));
#106459=CARTESIAN_POINT('Ctrl Pts',(39.6784416021826,58.5221371154761,12.));
#106460=CARTESIAN_POINT('Ctrl Pts',(39.6847521356395,58.5424914443415,0.));
#106461=CARTESIAN_POINT('Ctrl Pts',(39.6847521356395,58.5424914443415,12.));
#106462=CARTESIAN_POINT('Ctrl Pts',(39.6910560748629,58.5628991912052,0.));
#106463=CARTESIAN_POINT('Ctrl Pts',(39.6910560748629,58.5628991912052,12.));
#106464=CARTESIAN_POINT('Ctrl Pts',(39.6973532992539,58.5833602272744,0.));
#106465=CARTESIAN_POINT('Ctrl Pts',(39.6973532992539,58.5833602272744,12.));
#106466=CARTESIAN_POINT('Ctrl Pts',(39.7036436890232,58.6038744244659,0.));
#106467=CARTESIAN_POINT('Ctrl Pts',(39.7036436890232,58.6038744244659,12.));
#106468=CARTESIAN_POINT('Ctrl Pts',(39.7099271251413,58.6244416553562,0.));
#106469=CARTESIAN_POINT('Ctrl Pts',(39.7099271251413,58.6244416553562,12.));
#106470=CARTESIAN_POINT('Ctrl Pts',(39.7162034892899,58.6450617931274,0.));
#106471=CARTESIAN_POINT('Ctrl Pts',(39.7162034892899,58.6450617931274,12.));
#106472=CARTESIAN_POINT('Ctrl Pts',(39.72247266381,58.6657347115034,0.));
#106473=CARTESIAN_POINT('Ctrl Pts',(39.72247266381,58.6657347115034,12.));
#106474=CARTESIAN_POINT('Ctrl Pts',(39.7287345316681,58.6864602847088,0.));
#106475=CARTESIAN_POINT('Ctrl Pts',(39.7287345316681,58.6864602847088,12.));
#106476=CARTESIAN_POINT('Ctrl Pts',(39.7349889764749,58.7072383875027,0.));
#106477=CARTESIAN_POINT('Ctrl Pts',(39.7349889764749,58.7072383875027,12.));
#106478=CARTESIAN_POINT('Ctrl Pts',(39.7412358824953,58.7280688951916,0.));
#106479=CARTESIAN_POINT('Ctrl Pts',(39.7412358824953,58.7280688951916,12.));
#106480=CARTESIAN_POINT('Ctrl Pts',(39.7474751346598,58.7489516836445,0.));
#106481=CARTESIAN_POINT('Ctrl Pts',(39.7474751346598,58.7489516836445,12.));
#106482=CARTESIAN_POINT('Ctrl Pts',(39.7537066185812,58.7698866293029,0.));
#106483=CARTESIAN_POINT('Ctrl Pts',(39.7537066185812,58.7698866293029,12.));
#106484=CARTESIAN_POINT('Ctrl Pts',(39.759930220552,58.7908736091798,0.));
#106485=CARTESIAN_POINT('Ctrl Pts',(39.759930220552,58.7908736091798,12.));
#106486=CARTESIAN_POINT('Ctrl Pts',(39.7661458275274,58.8119125008517,0.));
#106487=CARTESIAN_POINT('Ctrl Pts',(39.7661458275274,58.8119125008517,12.));
#106488=CARTESIAN_POINT('Ctrl Pts',(39.772353327112,58.8330031824453,0.));
#106489=CARTESIAN_POINT('Ctrl Pts',(39.772353327112,58.8330031824453,12.));
#106490=CARTESIAN_POINT('Ctrl Pts',(39.7785526075478,58.8541455326231,0.));
#106491=CARTESIAN_POINT('Ctrl Pts',(39.7785526075478,58.8541455326231,12.));
#106492=CARTESIAN_POINT('Ctrl Pts',(39.7847435576996,58.8753394305586,0.));
#106493=CARTESIAN_POINT('Ctrl Pts',(39.7847435576996,58.8753394305586,12.));
#106494=CARTESIAN_POINT('Ctrl Pts',(39.7909260670517,58.8965847559391,0.));
#106495=CARTESIAN_POINT('Ctrl Pts',(39.7909260670517,58.8965847559391,12.));
#106496=CARTESIAN_POINT('Ctrl Pts',(39.7971000257044,58.9178813889704,0.));
#106497=CARTESIAN_POINT('Ctrl Pts',(39.7971000257044,58.9178813889704,12.));
#106498=CARTESIAN_POINT('Ctrl Pts',(39.8032653243712,58.9392292103747,0.));
#106499=CARTESIAN_POINT('Ctrl Pts',(39.8032653243712,58.9392292103747,12.));
#106500=CARTESIAN_POINT('Ctrl Pts',(39.8094218543782,58.9606281013875,0.));
#106501=CARTESIAN_POINT('Ctrl Pts',(39.8094218543782,58.9606281013875,12.));
#106502=CARTESIAN_POINT('Ctrl Pts',(39.8155695076626,58.9820779437485,0.));
#106503=CARTESIAN_POINT('Ctrl Pts',(39.8155695076626,58.9820779437485,12.));
#106504=CARTESIAN_POINT('Ctrl Pts',(39.821708176766,59.0035786197024,0.));
#106505=CARTESIAN_POINT('Ctrl Pts',(39.821708176766,59.0035786197024,12.));
#106506=CARTESIAN_POINT('Ctrl Pts',(39.8278377548262,59.0251300119973,0.));
#106507=CARTESIAN_POINT('Ctrl Pts',(39.8278377548262,59.0251300119973,12.));
#106508=CARTESIAN_POINT('Ctrl Pts',(39.8339581355715,59.0467320038784,0.));
#106509=CARTESIAN_POINT('Ctrl Pts',(39.8339581355715,59.0467320038784,12.));
#106510=CARTESIAN_POINT('Ctrl Pts',(39.8400692133139,59.0683844790764,0.));
#106511=CARTESIAN_POINT('Ctrl Pts',(39.8400692133139,59.0683844790764,12.));
#106512=CARTESIAN_POINT('Ctrl Pts',(39.8461708829456,59.0900873217981,0.));
#106513=CARTESIAN_POINT('Ctrl Pts',(39.8461708829456,59.0900873217981,12.));
#106514=CARTESIAN_POINT('Ctrl Pts',(39.8522630399328,59.1118404167292,0.));
#106515=CARTESIAN_POINT('Ctrl Pts',(39.8522630399328,59.1118404167292,12.));
#106516=CARTESIAN_POINT('Ctrl Pts',(39.8583455803105,59.1336436490342,0.));
#106517=CARTESIAN_POINT('Ctrl Pts',(39.8583455803105,59.1336436490342,12.));
#106518=CARTESIAN_POINT('Ctrl Pts',(39.8644184006786,59.1554969043522,0.));
#106519=CARTESIAN_POINT('Ctrl Pts',(39.8644184006786,59.1554969043522,12.));
#106520=CARTESIAN_POINT('Ctrl Pts',(39.8704813981988,59.1774000687879,0.));
#106521=CARTESIAN_POINT('Ctrl Pts',(39.8704813981988,59.1774000687879,12.));
#106522=CARTESIAN_POINT('Ctrl Pts',(39.8765344705909,59.1993530289029,0.));
#106523=CARTESIAN_POINT('Ctrl Pts',(39.8765344705909,59.1993530289029,12.));
#106524=CARTESIAN_POINT('Ctrl Pts',(39.8825775161267,59.2213556717209,0.));
#106525=CARTESIAN_POINT('Ctrl Pts',(39.8825775161267,59.2213556717209,12.));
#106526=CARTESIAN_POINT('Ctrl Pts',(39.8886104336242,59.2434078847247,0.));
#106527=CARTESIAN_POINT('Ctrl Pts',(39.8886104336242,59.2434078847247,12.));
#106528=CARTESIAN_POINT('Ctrl Pts',(39.8946331224438,59.2655095558521,0.));
#106529=CARTESIAN_POINT('Ctrl Pts',(39.8946331224438,59.2655095558521,12.));
#106530=CARTESIAN_POINT('Ctrl Pts',(39.9006454824845,59.2876605734847,0.));
#106531=CARTESIAN_POINT('Ctrl Pts',(39.9006454824845,59.2876605734847,12.));
#106532=CARTESIAN_POINT('Ctrl Pts',(39.9066474141803,59.3098608264419,0.));
#106533=CARTESIAN_POINT('Ctrl Pts',(39.9066474141803,59.3098608264419,12.));
#106534=CARTESIAN_POINT('Ctrl Pts',(39.9126388184936,59.3321102039852,0.));
#106535=CARTESIAN_POINT('Ctrl Pts',(39.9126388184936,59.3321102039852,12.));
#106536=CARTESIAN_POINT('Ctrl Pts',(39.9186195969104,59.3544085958151,0.));
#106537=CARTESIAN_POINT('Ctrl Pts',(39.9186195969104,59.3544085958151,12.));
#106538=CARTESIAN_POINT('Ctrl Pts',(39.9245896514367,59.3767558920675,0.));
#106539=CARTESIAN_POINT('Ctrl Pts',(39.9245896514367,59.3767558920675,12.));
#106540=CARTESIAN_POINT('Ctrl Pts',(39.9305488845958,59.3991519833016,0.));
#106541=CARTESIAN_POINT('Ctrl Pts',(39.9305488845958,59.3991519833016,12.));
#106542=CARTESIAN_POINT('Ctrl Pts',(39.9364971994242,59.4215967604968,0.));
#106543=CARTESIAN_POINT('Ctrl Pts',(39.9364971994242,59.4215967604968,12.));
#106544=CARTESIAN_POINT('Ctrl Pts',(39.9424344994672,59.4440901150582,0.));
#106545=CARTESIAN_POINT('Ctrl Pts',(39.9424344994672,59.4440901150582,12.));
#106546=CARTESIAN_POINT('Ctrl Pts',(39.9483606887737,59.4666319388133,0.));
#106547=CARTESIAN_POINT('Ctrl Pts',(39.9483606887737,59.4666319388133,12.));
#106548=CARTESIAN_POINT('Ctrl Pts',(39.9542756718922,59.4892221240069,0.));
#106549=CARTESIAN_POINT('Ctrl Pts',(39.9542756718922,59.4892221240069,12.));
#106550=CARTESIAN_POINT('Ctrl Pts',(39.9601793538682,59.5118605632891,0.));
#106551=CARTESIAN_POINT('Ctrl Pts',(39.9601793538682,59.5118605632891,12.));
#106552=CARTESIAN_POINT('Ctrl Pts',(39.9660716402403,59.5345471497129,0.));
#106553=CARTESIAN_POINT('Ctrl Pts',(39.9660716402403,59.5345471497129,12.));
#106554=CARTESIAN_POINT('Ctrl Pts',(39.9719524370345,59.5572817767388,0.));
#106555=CARTESIAN_POINT('Ctrl Pts',(39.9719524370345,59.5572817767388,12.));
#106556=CARTESIAN_POINT('Ctrl Pts',(39.9778216507605,59.5800643382315,0.));
#106557=CARTESIAN_POINT('Ctrl Pts',(39.9778216507605,59.5800643382315,12.));
#106558=CARTESIAN_POINT('Ctrl Pts',(39.9836791884079,59.6028947284562,0.));
#106559=CARTESIAN_POINT('Ctrl Pts',(39.9836791884079,59.6028947284562,12.));
#106560=CARTESIAN_POINT('Ctrl Pts',(39.9895249574448,59.6257728420669,0.));
#106561=CARTESIAN_POINT('Ctrl Pts',(39.9895249574448,59.6257728420669,12.));
#106562=CARTESIAN_POINT('Ctrl Pts',(39.9953588658131,59.6486985741041,0.));
#106563=CARTESIAN_POINT('Ctrl Pts',(39.9953588658131,59.6486985741041,12.));
#106564=CARTESIAN_POINT('Ctrl Pts',(40.0011808219241,59.6716718200005,0.));
#106565=CARTESIAN_POINT('Ctrl Pts',(40.0011808219241,59.6716718200005,12.));
#106566=CARTESIAN_POINT('Ctrl Pts',(40.0069907346537,59.6946924755773,0.));
#106567=CARTESIAN_POINT('Ctrl Pts',(40.0069907346537,59.6946924755773,12.));
#106568=CARTESIAN_POINT('Ctrl Pts',(40.0127885133403,59.7177604370403,0.));
#106569=CARTESIAN_POINT('Ctrl Pts',(40.0127885133403,59.7177604370403,12.));
#106570=CARTESIAN_POINT('Ctrl Pts',(40.0185740677821,59.7408756009679,0.));
#106571=CARTESIAN_POINT('Ctrl Pts',(40.0185740677821,59.7408756009679,12.));
#106572=CARTESIAN_POINT('Ctrl Pts',(40.0243473082337,59.7640378643106,0.));
#106573=CARTESIAN_POINT('Ctrl Pts',(40.0243473082337,59.7640378643106,12.));
#106574=CARTESIAN_POINT('Ctrl Pts',(40.0301081454002,59.7872471243942,0.));
#106575=CARTESIAN_POINT('Ctrl Pts',(40.0301081454002,59.7872471243942,12.));
#106576=CARTESIAN_POINT('Ctrl Pts',(40.035856490434,59.8105032789179,0.));
#106577=CARTESIAN_POINT('Ctrl Pts',(40.035856490434,59.8105032789179,12.));
#106578=CARTESIAN_POINT('Ctrl Pts',(40.0415922549314,59.8338062259493,0.));
#106579=CARTESIAN_POINT('Ctrl Pts',(40.0415922549314,59.8338062259493,12.));
#106580=CARTESIAN_POINT('Ctrl Pts',(40.0473153509324,59.8571558639145,0.));
#106581=CARTESIAN_POINT('Ctrl Pts',(40.0473153509324,59.8571558639145,12.));
#106582=CARTESIAN_POINT('Ctrl Pts',(40.053025690916,59.8805520915972,0.));
#106583=CARTESIAN_POINT('Ctrl Pts',(40.053025690916,59.8805520915972,12.));
#106584=CARTESIAN_POINT('Ctrl Pts',(40.0587231877959,59.9039948081428,0.));
#106585=CARTESIAN_POINT('Ctrl Pts',(40.0587231877959,59.9039948081428,12.));
#106586=CARTESIAN_POINT('Ctrl Pts',(40.0644077549158,59.927483913055,0.));
#106587=CARTESIAN_POINT('Ctrl Pts',(40.0644077549158,59.927483913055,12.));
#106588=CARTESIAN_POINT('Ctrl Pts',(40.0700793060475,59.9510193061929,0.));
#106589=CARTESIAN_POINT('Ctrl Pts',(40.0700793060475,59.9510193061929,12.));
#106590=CARTESIAN_POINT('Ctrl Pts',(40.0757377553893,59.974600887759,0.));
#106591=CARTESIAN_POINT('Ctrl Pts',(40.0757377553893,59.974600887759,12.));
#106592=CARTESIAN_POINT('Ctrl Pts',(40.0813830175629,59.9982285582991,0.));
#106593=CARTESIAN_POINT('Ctrl Pts',(40.0813830175629,59.9982285582991,12.));
#106594=CARTESIAN_POINT('Ctrl Pts',(40.0870150076078,60.0219022187066,0.));
#106595=CARTESIAN_POINT('Ctrl Pts',(40.0870150076078,60.0219022187066,12.));
#106596=CARTESIAN_POINT('Ctrl Pts',(40.0926336409787,60.0456217702203,0.));
#106597=CARTESIAN_POINT('Ctrl Pts',(40.0926336409787,60.0456217702203,12.));
#106598=CARTESIAN_POINT('Ctrl Pts',(40.0982388335421,60.0693871144207,0.));
#106599=CARTESIAN_POINT('Ctrl Pts',(40.0982388335421,60.0693871144207,12.));
#106600=CARTESIAN_POINT('Ctrl Pts',(40.1038305015763,60.0931981532194,0.));
#106601=CARTESIAN_POINT('Ctrl Pts',(40.1038305015763,60.0931981532194,12.));
#106602=CARTESIAN_POINT('Ctrl Pts',(40.1094085617672,60.1170547888572,0.));
#106603=CARTESIAN_POINT('Ctrl Pts',(40.1094085617672,60.1170547888572,12.));
#106604=CARTESIAN_POINT('Ctrl Pts',(40.1149729312036,60.1409569239093,0.));
#106605=CARTESIAN_POINT('Ctrl Pts',(40.1149729312036,60.1409569239093,12.));
#106606=CARTESIAN_POINT('Ctrl Pts',(40.120523527374,60.164904461283,0.));
#106607=CARTESIAN_POINT('Ctrl Pts',(40.120523527374,60.164904461283,12.));
#106608=CARTESIAN_POINT('Ctrl Pts',(40.1260602681644,60.1888973042151,0.));
#106609=CARTESIAN_POINT('Ctrl Pts',(40.1260602681644,60.1888973042151,12.));
#106610=CARTESIAN_POINT('Ctrl Pts',(40.1315830718575,60.2129353562618,0.));
#106611=CARTESIAN_POINT('Ctrl Pts',(40.1315830718575,60.2129353562618,12.));
#106612=CARTESIAN_POINT('Ctrl Pts',(40.13709185713,60.2370185212957,0.));
#106613=CARTESIAN_POINT('Ctrl Pts',(40.13709185713,60.2370185212957,12.));
#106614=CARTESIAN_POINT('Ctrl Pts',(40.1425865430468,60.2611467035109,0.));
#106615=CARTESIAN_POINT('Ctrl Pts',(40.1425865430468,60.2611467035109,12.));
#106616=CARTESIAN_POINT('Ctrl Pts',(40.1480670490583,60.2853198074216,0.));
#106617=CARTESIAN_POINT('Ctrl Pts',(40.1480670490583,60.2853198074216,12.));
#106618=CARTESIAN_POINT('Ctrl Pts',(40.1535332949978,60.3095377378589,0.));
#106619=CARTESIAN_POINT('Ctrl Pts',(40.1535332949978,60.3095377378589,12.));
#106620=CARTESIAN_POINT('Ctrl Pts',(40.158985201081,60.3338003999616,0.));
#106621=CARTESIAN_POINT('Ctrl Pts',(40.158985201081,60.3338003999616,12.));
#106622=CARTESIAN_POINT('Ctrl Pts',(40.1644226879043,60.3581076991731,0.));
#106623=CARTESIAN_POINT('Ctrl Pts',(40.1644226879043,60.3581076991731,12.));
#106624=CARTESIAN_POINT('Ctrl Pts',(40.1698456764387,60.382459541246,0.));
#106625=CARTESIAN_POINT('Ctrl Pts',(40.1698456764387,60.382459541246,12.));
#106626=CARTESIAN_POINT('Ctrl Pts',(40.1752540880273,60.4068558322415,0.));
#106627=CARTESIAN_POINT('Ctrl Pts',(40.1752540880273,60.4068558322415,12.));
#106628=CARTESIAN_POINT('Ctrl Pts',(40.1806478443828,60.4312964785269,0.));
#106629=CARTESIAN_POINT('Ctrl Pts',(40.1806478443828,60.4312964785269,12.));
#106630=CARTESIAN_POINT('Ctrl Pts',(40.1860268675875,60.4557813867677,0.));
#106631=CARTESIAN_POINT('Ctrl Pts',(40.1860268675875,60.4557813867677,12.));
#106632=CARTESIAN_POINT('Ctrl Pts',(40.1913910800911,60.4803104639211,0.));
#106633=CARTESIAN_POINT('Ctrl Pts',(40.1913910800911,60.4803104639211,12.));
#106634=CARTESIAN_POINT('Ctrl Pts',(40.1967404047055,60.5048836172424,0.));
#106635=CARTESIAN_POINT('Ctrl Pts',(40.1967404047055,60.5048836172424,12.));
#106636=CARTESIAN_POINT('Ctrl Pts',(40.2020747646012,60.5295007542838,0.));
#106637=CARTESIAN_POINT('Ctrl Pts',(40.2020747646012,60.5295007542838,12.));
#106638=CARTESIAN_POINT('Ctrl Pts',(40.2073940833054,60.5541617828927,0.));
#106639=CARTESIAN_POINT('Ctrl Pts',(40.2073940833054,60.5541617828927,12.));
#106640=CARTESIAN_POINT('Ctrl Pts',(40.2126982847012,60.5788666112043,0.));
#106641=CARTESIAN_POINT('Ctrl Pts',(40.2126982847012,60.5788666112043,12.));
#106642=CARTESIAN_POINT('Ctrl Pts',(40.2179872930271,60.6036151476347,0.));
#106643=CARTESIAN_POINT('Ctrl Pts',(40.2179872930271,60.6036151476347,12.));
#106644=CARTESIAN_POINT('Ctrl Pts',(40.2232610328717,60.6284073008865,0.));
#106645=CARTESIAN_POINT('Ctrl Pts',(40.2232610328717,60.6284073008865,12.));
#106646=CARTESIAN_POINT('Ctrl Pts',(40.2285194291702,60.6532429799494,0.));
#106647=CARTESIAN_POINT('Ctrl Pts',(40.2285194291702,60.6532429799494,12.));
#106648=CARTESIAN_POINT('Ctrl Pts',(40.2337624072029,60.678122094098,0.));
#106649=CARTESIAN_POINT('Ctrl Pts',(40.2337624072029,60.678122094098,12.));
#106650=CARTESIAN_POINT('Ctrl Pts',(40.2389898925937,60.7030445528863,0.));
#106651=CARTESIAN_POINT('Ctrl Pts',(40.2389898925937,60.7030445528863,12.));
#106652=CARTESIAN_POINT('Ctrl Pts',(40.2442018113116,60.7280102661401,0.));
#106653=CARTESIAN_POINT('Ctrl Pts',(40.2442018113116,60.7280102661401,12.));
#106654=CARTESIAN_POINT('Ctrl Pts',(40.2493980896646,60.7530191439603,0.));
#106655=CARTESIAN_POINT('Ctrl Pts',(40.2493980896646,60.7530191439603,12.));
#106656=CARTESIAN_POINT('Ctrl Pts',(40.2545786542957,60.7780710967253,0.));
#106657=CARTESIAN_POINT('Ctrl Pts',(40.2545786542957,60.7780710967253,12.));
#106658=CARTESIAN_POINT('Ctrl Pts',(40.2597434321803,60.8031660350879,0.));
#106659=CARTESIAN_POINT('Ctrl Pts',(40.2597434321803,60.8031660350879,12.));
#106660=CARTESIAN_POINT('Ctrl Pts',(40.2648923506245,60.8283038699703,0.));
#106661=CARTESIAN_POINT('Ctrl Pts',(40.2648923506245,60.8283038699703,12.));
#106662=CARTESIAN_POINT('Ctrl Pts',(40.2700253372644,60.8534845125535,0.));
#106663=CARTESIAN_POINT('Ctrl Pts',(40.2700253372644,60.8534845125535,12.));
#106664=CARTESIAN_POINT('Ctrl Pts',(40.2751423200637,60.8787078742817,0.));
#106665=CARTESIAN_POINT('Ctrl Pts',(40.2751423200637,60.8787078742817,12.));
#106666=CARTESIAN_POINT('Ctrl Pts',(40.2802432273104,60.903973866867,0.));
#106667=CARTESIAN_POINT('Ctrl Pts',(40.2802432273104,60.903973866867,12.));
#106668=CARTESIAN_POINT('Ctrl Pts',(40.2853279876161,60.9292824022888,0.));
#106669=CARTESIAN_POINT('Ctrl Pts',(40.2853279876161,60.9292824022888,12.));
#106670=CARTESIAN_POINT('Ctrl Pts',(40.2903965299155,60.9546333927919,0.));
#106671=CARTESIAN_POINT('Ctrl Pts',(40.2903965299155,60.9546333927919,12.));
#106672=CARTESIAN_POINT('Ctrl Pts',(40.2954487834688,60.9800267508781,0.));
#106673=CARTESIAN_POINT('Ctrl Pts',(40.2954487834688,60.9800267508781,12.));
#106674=CARTESIAN_POINT('Ctrl Pts',(40.3004846778577,61.005462389306,0.));
#106675=CARTESIAN_POINT('Ctrl Pts',(40.3004846778577,61.005462389306,12.));
#106676=CARTESIAN_POINT('Ctrl Pts',(40.3055041429772,61.0309402210915,0.));
#106677=CARTESIAN_POINT('Ctrl Pts',(40.3055041429772,61.0309402210915,12.));
#106678=CARTESIAN_POINT('Ctrl Pts',(40.3105071090308,61.0564601595047,0.));
#106679=CARTESIAN_POINT('Ctrl Pts',(40.3105071090308,61.0564601595047,12.));
#106680=CARTESIAN_POINT('Ctrl Pts',(40.3154935065263,61.0820221180647,0.));
#106681=CARTESIAN_POINT('Ctrl Pts',(40.3154935065263,61.0820221180647,12.));
#106682=CARTESIAN_POINT('Ctrl Pts',(40.3204632662729,61.1076260105265,0.));
#106683=CARTESIAN_POINT('Ctrl Pts',(40.3204632662729,61.1076260105265,12.));
#106684=CARTESIAN_POINT('Ctrl Pts',(40.3254163193805,61.1332717508799,0.));
#106685=CARTESIAN_POINT('Ctrl Pts',(40.3254163193805,61.1332717508799,12.));
#106686=CARTESIAN_POINT('Ctrl Pts',(40.3303525972621,61.1589592533623,0.));
#106687=CARTESIAN_POINT('Ctrl Pts',(40.3303525972621,61.1589592533623,12.));
#106688=CARTESIAN_POINT('Ctrl Pts',(40.3352720316373,61.184688432465,0.));
#106689=CARTESIAN_POINT('Ctrl Pts',(40.3352720316373,61.184688432465,12.));
#106690=CARTESIAN_POINT('Ctrl Pts',(40.3401745545369,61.2104592029376,0.));
#106691=CARTESIAN_POINT('Ctrl Pts',(40.3401745545369,61.2104592029376,12.));
#106692=CARTESIAN_POINT('Ctrl Pts',(40.3450600983104,61.2362714797891,0.));
#106693=CARTESIAN_POINT('Ctrl Pts',(40.3450600983104,61.2362714797891,12.));
#106694=CARTESIAN_POINT('Ctrl Pts',(40.3499285956297,61.262125178285,0.));
#106695=CARTESIAN_POINT('Ctrl Pts',(40.3499285956297,61.262125178285,12.));
#106696=CARTESIAN_POINT('Ctrl Pts',(40.3547799794672,61.2880202139358,0.));
#106697=CARTESIAN_POINT('Ctrl Pts',(40.3547799794672,61.2880202139358,12.));
#106698=CARTESIAN_POINT('Ctrl Pts',(40.3596141830786,61.3139565024838,0.));
#106699=CARTESIAN_POINT('Ctrl Pts',(40.3596141830786,61.3139565024838,12.));
#106700=CARTESIAN_POINT('Ctrl Pts',(40.364431139986,61.3399339598852,0.));
#106701=CARTESIAN_POINT('Ctrl Pts',(40.364431139986,61.3399339598852,12.));
#106702=CARTESIAN_POINT('Ctrl Pts',(40.3692307839642,61.3659525022917,0.));
#106703=CARTESIAN_POINT('Ctrl Pts',(40.3692307839642,61.3659525022917,12.));
#106704=CARTESIAN_POINT('Ctrl Pts',(40.3740130490233,61.3920120460232,0.));
#106705=CARTESIAN_POINT('Ctrl Pts',(40.3740130490233,61.3920120460232,12.));
#106706=CARTESIAN_POINT('Ctrl Pts',(40.3787778694372,61.418112507605,0.));
#106707=CARTESIAN_POINT('Ctrl Pts',(40.3787778694372,61.418112507605,12.));
#106708=CARTESIAN_POINT('Ctrl Pts',(40.3835251797725,61.4442538038053,0.));
#106709=CARTESIAN_POINT('Ctrl Pts',(40.3835251797725,61.4442538038053,12.));
#106710=CARTESIAN_POINT('Ctrl Pts',(40.3882549149229,61.4704358516711,0.));
#106711=CARTESIAN_POINT('Ctrl Pts',(40.3882549149229,61.4704358516711,12.));
#106712=CARTESIAN_POINT('Ctrl Pts',(40.3929670101363,61.4966585685545,0.));
#106713=CARTESIAN_POINT('Ctrl Pts',(40.3929670101363,61.4966585685545,12.));
#106714=CARTESIAN_POINT('Ctrl Pts',(40.3976614010648,61.5229218721532,0.));
#106715=CARTESIAN_POINT('Ctrl Pts',(40.3976614010648,61.5229218721532,12.));
#106716=CARTESIAN_POINT('Ctrl Pts',(40.4023380237227,61.5492256804709,0.));
#106717=CARTESIAN_POINT('Ctrl Pts',(40.4023380237227,61.5492256804709,12.));
#106718=CARTESIAN_POINT('Ctrl Pts',(40.4069968143953,61.5755699117318,0.));
#106719=CARTESIAN_POINT('Ctrl Pts',(40.4069968143953,61.5755699117318,12.));
#106720=CARTESIAN_POINT('Ctrl Pts',(40.4116377095595,61.6019544843009,0.));
#106721=CARTESIAN_POINT('Ctrl Pts',(40.4116377095595,61.6019544843009,12.));
#106722=CARTESIAN_POINT('Ctrl Pts',(40.4162606458119,61.628379316608,0.));
#106723=CARTESIAN_POINT('Ctrl Pts',(40.4162606458119,61.628379316608,12.));
#106724=CARTESIAN_POINT('Ctrl Pts',(40.420865559772,61.6548443270397,0.));
#106725=CARTESIAN_POINT('Ctrl Pts',(40.420865559772,61.6548443270397,12.));
#106726=CARTESIAN_POINT('Ctrl Pts',(40.4254523880766,61.6813494339295,0.));
#106727=CARTESIAN_POINT('Ctrl Pts',(40.4254523880766,61.6813494339295,12.));
#106728=CARTESIAN_POINT('Ctrl Pts',(40.4300210675848,61.7078945557812,0.));
#106729=CARTESIAN_POINT('Ctrl Pts',(40.4300210675848,61.7078945557812,12.));
#106730=CARTESIAN_POINT('Ctrl Pts',(40.4345715355411,61.7344796114409,0.));
#106731=CARTESIAN_POINT('Ctrl Pts',(40.4345715355411,61.7344796114409,12.));
#106732=CARTESIAN_POINT('Ctrl Pts',(40.4391037297589,61.7611045202875,0.));
#106733=CARTESIAN_POINT('Ctrl Pts',(40.4391037297589,61.7611045202875,12.));
#106734=CARTESIAN_POINT('Ctrl Pts',(40.4436175887942,61.7877692024064,0.));
#106735=CARTESIAN_POINT('Ctrl Pts',(40.4436175887942,61.7877692024064,12.));
#106736=CARTESIAN_POINT('Ctrl Pts',(40.448113052135,61.8144735787767,0.));
#106737=CARTESIAN_POINT('Ctrl Pts',(40.448113052135,61.8144735787767,12.));
#106738=CARTESIAN_POINT('Ctrl Pts',(40.4525900597877,61.8412175708524,0.));
#106739=CARTESIAN_POINT('Ctrl Pts',(40.4525900597877,61.8412175708524,12.));
#106740=CARTESIAN_POINT('Ctrl Pts',(40.4570485518735,61.8680011001513,0.));
#106741=CARTESIAN_POINT('Ctrl Pts',(40.4570485518735,61.8680011001513,12.));
#106742=CARTESIAN_POINT('Ctrl Pts',(40.4614884681884,61.8948240877998,0.));
#106743=CARTESIAN_POINT('Ctrl Pts',(40.4614884681884,61.8948240877998,12.));
#106744=CARTESIAN_POINT('Ctrl Pts',(40.4659097478595,61.9216864541758,0.));
#106745=CARTESIAN_POINT('Ctrl Pts',(40.4659097478595,61.9216864541758,12.));
#106746=CARTESIAN_POINT('Ctrl Pts',(40.4703123287642,61.9485881182957,0.));
#106747=CARTESIAN_POINT('Ctrl Pts',(40.4703123287642,61.9485881182957,12.));
#106748=CARTESIAN_POINT('Ctrl Pts',(40.4746961480045,61.9755289983094,0.));
#106749=CARTESIAN_POINT('Ctrl Pts',(40.4746961480045,61.9755289983094,12.));
#106750=CARTESIAN_POINT('Ctrl Pts',(40.4790611429613,62.0025090126008,0.));
#106751=CARTESIAN_POINT('Ctrl Pts',(40.4790611429613,62.0025090126008,12.));
#106752=CARTESIAN_POINT('Ctrl Pts',(40.4834072522181,62.0295280807449,0.));
#106753=CARTESIAN_POINT('Ctrl Pts',(40.4834072522181,62.0295280807449,12.));
#106754=CARTESIAN_POINT('Ctrl Pts',(40.4877344164407,62.0565861244171,0.));
#106755=CARTESIAN_POINT('Ctrl Pts',(40.4877344164407,62.0565861244171,12.));
#106756=CARTESIAN_POINT('Ctrl Pts',(40.4920425795184,62.0836830685665,0.));
#106757=CARTESIAN_POINT('Ctrl Pts',(40.4920425795184,62.0836830685665,12.));
#106758=CARTESIAN_POINT('Ctrl Pts',(40.4963316888356,62.110818841691,0.));
#106759=CARTESIAN_POINT('Ctrl Pts',(40.4963316888356,62.110818841691,12.));
#106760=CARTESIAN_POINT('Ctrl Pts',(40.5006016927489,62.137993373242,0.));
#106761=CARTESIAN_POINT('Ctrl Pts',(40.5006016927489,62.137993373242,12.));
#106762=CARTESIAN_POINT('Ctrl Pts',(40.5048525385985,62.1652065915724,0.));
#106763=CARTESIAN_POINT('Ctrl Pts',(40.5048525385985,62.1652065915724,12.));
#106764=CARTESIAN_POINT('Ctrl Pts',(40.5090841704111,62.1924584215634,0.));
#106765=CARTESIAN_POINT('Ctrl Pts',(40.5090841704111,62.1924584215634,12.));
#106766=CARTESIAN_POINT('Ctrl Pts',(40.5132965269679,62.2197487826212,0.));
#106767=CARTESIAN_POINT('Ctrl Pts',(40.5132965269679,62.2197487826212,12.));
#106768=CARTESIAN_POINT('Ctrl Pts',(40.5174895391059,62.2470775858834,0.));
#106769=CARTESIAN_POINT('Ctrl Pts',(40.5174895391059,62.2470775858834,12.));
#106770=CARTESIAN_POINT('Ctrl Pts',(40.5216631336335,62.2744447382207,0.));
#106771=CARTESIAN_POINT('Ctrl Pts',(40.5216631336335,62.2744447382207,12.));
#106772=CARTESIAN_POINT('Ctrl Pts',(40.5258172381564,62.3018501471877,0.));
#106773=CARTESIAN_POINT('Ctrl Pts',(40.5258172381564,62.3018501471877,12.));
#106774=CARTESIAN_POINT('Ctrl Pts',(40.5299517857793,62.3292937258021,0.));
#106775=CARTESIAN_POINT('Ctrl Pts',(40.5299517857793,62.3292937258021,12.));
#106776=CARTESIAN_POINT('Ctrl Pts',(40.5340667194272,62.35677539702,0.));
#106777=CARTESIAN_POINT('Ctrl Pts',(40.5340667194272,62.35677539702,12.));
#106778=CARTESIAN_POINT('Ctrl Pts',(40.5381619973972,62.3842950992505,0.));
#106779=CARTESIAN_POINT('Ctrl Pts',(40.5381619973972,62.3842950992505,12.));
#106780=CARTESIAN_POINT('Ctrl Pts',(40.5422375944697,62.4118527880601,0.));
#106781=CARTESIAN_POINT('Ctrl Pts',(40.5422375944697,62.4118527880601,12.));
#106782=CARTESIAN_POINT('Ctrl Pts',(40.5462934972334,62.439448432904,0.));
#106783=CARTESIAN_POINT('Ctrl Pts',(40.5462934972334,62.439448432904,12.));
#106784=CARTESIAN_POINT('Ctrl Pts',(40.5495224601437,62.4615552986669,0.));
#106785=CARTESIAN_POINT('Ctrl Pts',(40.5495224601437,62.4615552986669,12.));
#106786=CARTESIAN_POINT('Ctrl Pts',(40.5519353177058,62.4781525155997,0.));
#106787=CARTESIAN_POINT('Ctrl Pts',(40.5519353177058,62.4781525155997,12.));
#106788=CARTESIAN_POINT('Ctrl Pts',(40.5535399497448,62.4892249121863,0.));
#106789=CARTESIAN_POINT('Ctrl Pts',(40.5535399497448,62.4892249121863,12.));
#106790=CARTESIAN_POINT('Ctrl Pts',(40.554341280847,62.494763006804,0.));
#106791=CARTESIAN_POINT('Ctrl Pts',(40.554341280847,62.494763006804,12.));
#106792=CARTESIAN_POINT('',(39.4479504917287,57.8261117662439,0.));
#106793=CARTESIAN_POINT('Ctrl Pts',(39.4479504917287,57.8261117662439,0.));
#106794=CARTESIAN_POINT('Ctrl Pts',(39.4492429618443,57.8297740100947,0.));
#106795=CARTESIAN_POINT('Ctrl Pts',(39.4518277003553,57.8371043151411,0.));
#106796=CARTESIAN_POINT('Ctrl Pts',(39.4557042029652,57.8481172247496,0.));
#106797=CARTESIAN_POINT('Ctrl Pts',(39.4608716627117,57.8628360096803,0.));
#106798=CARTESIAN_POINT('Ctrl Pts',(39.4673289592259,57.8812926637177,0.));
#106799=CARTESIAN_POINT('Ctrl Pts',(39.473784194937,57.8998074670478,0.));
#106800=CARTESIAN_POINT('Ctrl Pts',(39.4802373061058,57.9183803632404,0.));
#106801=CARTESIAN_POINT('Ctrl Pts',(39.4866881842317,57.9370112456631,0.));
#106802=CARTESIAN_POINT('Ctrl Pts',(39.4931366776714,57.9556999583892,0.));
#106803=CARTESIAN_POINT('Ctrl Pts',(39.499582610674,57.974446317937,0.));
#106804=CARTESIAN_POINT('Ctrl Pts',(39.5060257981225,57.9932501298522,0.));
#106805=CARTESIAN_POINT('Ctrl Pts',(39.5124660614976,58.0121112067896,0.));
#106806=CARTESIAN_POINT('Ctrl Pts',(39.5189032457184,58.0310293875262,0.));
#106807=CARTESIAN_POINT('Ctrl Pts',(39.5253372136887,58.0500045308412,0.));
#106808=CARTESIAN_POINT('Ctrl Pts',(39.5317678383217,58.0690365065374,0.));
#106809=CARTESIAN_POINT('Ctrl Pts',(39.5381949959221,58.0881251879921,0.));
#106810=CARTESIAN_POINT('Ctrl Pts',(39.5446185579638,58.1072704428928,0.));
#106811=CARTESIAN_POINT('Ctrl Pts',(39.5510383869505,58.126472128574,0.));
#106812=CARTESIAN_POINT('Ctrl Pts',(39.5574543406981,58.1457300968499,0.));
#106813=CARTESIAN_POINT('Ctrl Pts',(39.563866275018,58.1650441970387,0.));
#106814=CARTESIAN_POINT('Ctrl Pts',(39.5702740467999,58.1844142794338,0.));
#106815=CARTESIAN_POINT('Ctrl Pts',(39.57667751752,58.2038401992457,0.));
#106816=CARTESIAN_POINT('Ctrl Pts',(39.5830765530891,58.2233218164366,0.));
#106817=CARTESIAN_POINT('Ctrl Pts',(39.5894710221713,58.2428589938369,0.));
#106818=CARTESIAN_POINT('Ctrl Pts',(39.5958607950239,58.2624515958419,0.));
#106819=CARTESIAN_POINT('Ctrl Pts',(39.6022457420789,58.2820994868118,0.));
#106820=CARTESIAN_POINT('Ctrl Pts',(39.6086257327583,58.3018025297324,0.));
#106821=CARTESIAN_POINT('Ctrl Pts',(39.6150006360914,58.3215605869221,0.));
#106822=CARTESIAN_POINT('Ctrl Pts',(39.6213703212531,58.3413735206424,0.));
#106823=CARTESIAN_POINT('Ctrl Pts',(39.6277346580892,58.3612411936905,0.));
#106824=CARTESIAN_POINT('Ctrl Pts',(39.6340935177476,58.3811634701037,0.));
#106825=CARTESIAN_POINT('Ctrl Pts',(39.6404467729094,58.4011402154196,0.));
#106826=CARTESIAN_POINT('Ctrl Pts',(39.6467942974451,58.4211712963004,0.));
#106827=CARTESIAN_POINT('Ctrl Pts',(39.653135966204,58.4412565802979,0.));
#106828=CARTESIAN_POINT('Ctrl Pts',(39.6594716547689,58.4613959355788,0.));
#106829=CARTESIAN_POINT('Ctrl Pts',(39.6658012391815,58.4815892306066,0.));
#106830=CARTESIAN_POINT('Ctrl Pts',(39.6721245959531,58.5018363341604,0.));
#106831=CARTESIAN_POINT('Ctrl Pts',(39.6784416021826,58.5221371154761,0.));
#106832=CARTESIAN_POINT('Ctrl Pts',(39.6847521356395,58.5424914443415,0.));
#106833=CARTESIAN_POINT('Ctrl Pts',(39.6910560748629,58.5628991912052,0.));
#106834=CARTESIAN_POINT('Ctrl Pts',(39.6973532992539,58.5833602272744,0.));
#106835=CARTESIAN_POINT('Ctrl Pts',(39.7036436890232,58.6038744244659,0.));
#106836=CARTESIAN_POINT('Ctrl Pts',(39.7099271251413,58.6244416553562,0.));
#106837=CARTESIAN_POINT('Ctrl Pts',(39.7162034892899,58.6450617931274,0.));
#106838=CARTESIAN_POINT('Ctrl Pts',(39.72247266381,58.6657347115034,0.));
#106839=CARTESIAN_POINT('Ctrl Pts',(39.7287345316681,58.6864602847088,0.));
#106840=CARTESIAN_POINT('Ctrl Pts',(39.7349889764749,58.7072383875027,0.));
#106841=CARTESIAN_POINT('Ctrl Pts',(39.7412358824953,58.7280688951916,0.));
#106842=CARTESIAN_POINT('Ctrl Pts',(39.7474751346598,58.7489516836445,0.));
#106843=CARTESIAN_POINT('Ctrl Pts',(39.7537066185812,58.7698866293029,0.));
#106844=CARTESIAN_POINT('Ctrl Pts',(39.759930220552,58.7908736091798,0.));
#106845=CARTESIAN_POINT('Ctrl Pts',(39.7661458275274,58.8119125008517,0.));
#106846=CARTESIAN_POINT('Ctrl Pts',(39.772353327112,58.8330031824453,0.));
#106847=CARTESIAN_POINT('Ctrl Pts',(39.7785526075478,58.8541455326231,0.));
#106848=CARTESIAN_POINT('Ctrl Pts',(39.7847435576996,58.8753394305586,0.));
#106849=CARTESIAN_POINT('Ctrl Pts',(39.7909260670517,58.8965847559391,0.));
#106850=CARTESIAN_POINT('Ctrl Pts',(39.7971000257044,58.9178813889704,0.));
#106851=CARTESIAN_POINT('Ctrl Pts',(39.8032653243712,58.9392292103747,0.));
#106852=CARTESIAN_POINT('Ctrl Pts',(39.8094218543782,58.9606281013875,0.));
#106853=CARTESIAN_POINT('Ctrl Pts',(39.8155695076626,58.9820779437485,0.));
#106854=CARTESIAN_POINT('Ctrl Pts',(39.821708176766,59.0035786197024,0.));
#106855=CARTESIAN_POINT('Ctrl Pts',(39.8278377548262,59.0251300119973,0.));
#106856=CARTESIAN_POINT('Ctrl Pts',(39.8339581355715,59.0467320038784,0.));
#106857=CARTESIAN_POINT('Ctrl Pts',(39.8400692133139,59.0683844790764,0.));
#106858=CARTESIAN_POINT('Ctrl Pts',(39.8461708829456,59.0900873217981,0.));
#106859=CARTESIAN_POINT('Ctrl Pts',(39.8522630399328,59.1118404167292,0.));
#106860=CARTESIAN_POINT('Ctrl Pts',(39.8583455803105,59.1336436490342,0.));
#106861=CARTESIAN_POINT('Ctrl Pts',(39.8644184006786,59.1554969043522,0.));
#106862=CARTESIAN_POINT('Ctrl Pts',(39.8704813981988,59.1774000687879,0.));
#106863=CARTESIAN_POINT('Ctrl Pts',(39.8765344705909,59.1993530289029,0.));
#106864=CARTESIAN_POINT('Ctrl Pts',(39.8825775161267,59.2213556717209,0.));
#106865=CARTESIAN_POINT('Ctrl Pts',(39.8886104336242,59.2434078847247,0.));
#106866=CARTESIAN_POINT('Ctrl Pts',(39.8946331224438,59.2655095558521,0.));
#106867=CARTESIAN_POINT('Ctrl Pts',(39.9006454824845,59.2876605734847,0.));
#106868=CARTESIAN_POINT('Ctrl Pts',(39.9066474141803,59.3098608264419,0.));
#106869=CARTESIAN_POINT('Ctrl Pts',(39.9126388184936,59.3321102039852,0.));
#106870=CARTESIAN_POINT('Ctrl Pts',(39.9186195969104,59.3544085958151,0.));
#106871=CARTESIAN_POINT('Ctrl Pts',(39.9245896514367,59.3767558920675,0.));
#106872=CARTESIAN_POINT('Ctrl Pts',(39.9305488845958,59.3991519833016,0.));
#106873=CARTESIAN_POINT('Ctrl Pts',(39.9364971994242,59.4215967604968,0.));
#106874=CARTESIAN_POINT('Ctrl Pts',(39.9424344994672,59.4440901150582,0.));
#106875=CARTESIAN_POINT('Ctrl Pts',(39.9483606887737,59.4666319388133,0.));
#106876=CARTESIAN_POINT('Ctrl Pts',(39.9542756718922,59.4892221240069,0.));
#106877=CARTESIAN_POINT('Ctrl Pts',(39.9601793538682,59.5118605632891,0.));
#106878=CARTESIAN_POINT('Ctrl Pts',(39.9660716402403,59.5345471497129,0.));
#106879=CARTESIAN_POINT('Ctrl Pts',(39.9719524370345,59.5572817767388,0.));
#106880=CARTESIAN_POINT('Ctrl Pts',(39.9778216507605,59.5800643382315,0.));
#106881=CARTESIAN_POINT('Ctrl Pts',(39.9836791884079,59.6028947284562,0.));
#106882=CARTESIAN_POINT('Ctrl Pts',(39.9895249574448,59.6257728420669,0.));
#106883=CARTESIAN_POINT('Ctrl Pts',(39.9953588658131,59.6486985741041,0.));
#106884=CARTESIAN_POINT('Ctrl Pts',(40.0011808219241,59.6716718200005,0.));
#106885=CARTESIAN_POINT('Ctrl Pts',(40.0069907346537,59.6946924755773,0.));
#106886=CARTESIAN_POINT('Ctrl Pts',(40.0127885133403,59.7177604370403,0.));
#106887=CARTESIAN_POINT('Ctrl Pts',(40.0185740677821,59.7408756009679,0.));
#106888=CARTESIAN_POINT('Ctrl Pts',(40.0243473082337,59.7640378643106,0.));
#106889=CARTESIAN_POINT('Ctrl Pts',(40.0301081454002,59.7872471243942,0.));
#106890=CARTESIAN_POINT('Ctrl Pts',(40.035856490434,59.8105032789179,0.));
#106891=CARTESIAN_POINT('Ctrl Pts',(40.0415922549314,59.8338062259493,0.));
#106892=CARTESIAN_POINT('Ctrl Pts',(40.0473153509324,59.8571558639145,0.));
#106893=CARTESIAN_POINT('Ctrl Pts',(40.053025690916,59.8805520915972,0.));
#106894=CARTESIAN_POINT('Ctrl Pts',(40.0587231877959,59.9039948081428,0.));
#106895=CARTESIAN_POINT('Ctrl Pts',(40.0644077549158,59.927483913055,0.));
#106896=CARTESIAN_POINT('Ctrl Pts',(40.0700793060475,59.9510193061929,0.));
#106897=CARTESIAN_POINT('Ctrl Pts',(40.0757377553893,59.974600887759,0.));
#106898=CARTESIAN_POINT('Ctrl Pts',(40.0813830175629,59.9982285582991,0.));
#106899=CARTESIAN_POINT('Ctrl Pts',(40.0870150076078,60.0219022187066,0.));
#106900=CARTESIAN_POINT('Ctrl Pts',(40.0926336409787,60.0456217702203,0.));
#106901=CARTESIAN_POINT('Ctrl Pts',(40.0982388335421,60.0693871144207,0.));
#106902=CARTESIAN_POINT('Ctrl Pts',(40.1038305015763,60.0931981532194,0.));
#106903=CARTESIAN_POINT('Ctrl Pts',(40.1094085617672,60.1170547888572,0.));
#106904=CARTESIAN_POINT('Ctrl Pts',(40.1149729312036,60.1409569239093,0.));
#106905=CARTESIAN_POINT('Ctrl Pts',(40.120523527374,60.164904461283,0.));
#106906=CARTESIAN_POINT('Ctrl Pts',(40.1260602681644,60.1888973042151,0.));
#106907=CARTESIAN_POINT('Ctrl Pts',(40.1315830718575,60.2129353562618,0.));
#106908=CARTESIAN_POINT('Ctrl Pts',(40.13709185713,60.2370185212957,0.));
#106909=CARTESIAN_POINT('Ctrl Pts',(40.1425865430468,60.2611467035109,0.));
#106910=CARTESIAN_POINT('Ctrl Pts',(40.1480670490583,60.2853198074216,0.));
#106911=CARTESIAN_POINT('Ctrl Pts',(40.1535332949978,60.3095377378589,0.));
#106912=CARTESIAN_POINT('Ctrl Pts',(40.158985201081,60.3338003999616,0.));
#106913=CARTESIAN_POINT('Ctrl Pts',(40.1644226879043,60.3581076991731,0.));
#106914=CARTESIAN_POINT('Ctrl Pts',(40.1698456764387,60.382459541246,0.));
#106915=CARTESIAN_POINT('Ctrl Pts',(40.1752540880273,60.4068558322415,0.));
#106916=CARTESIAN_POINT('Ctrl Pts',(40.1806478443828,60.4312964785269,0.));
#106917=CARTESIAN_POINT('Ctrl Pts',(40.1860268675875,60.4557813867677,0.));
#106918=CARTESIAN_POINT('Ctrl Pts',(40.1913910800911,60.4803104639211,0.));
#106919=CARTESIAN_POINT('Ctrl Pts',(40.1967404047055,60.5048836172424,0.));
#106920=CARTESIAN_POINT('Ctrl Pts',(40.2020747646012,60.5295007542838,0.));
#106921=CARTESIAN_POINT('Ctrl Pts',(40.2073940833054,60.5541617828927,0.));
#106922=CARTESIAN_POINT('Ctrl Pts',(40.2126982847012,60.5788666112043,0.));
#106923=CARTESIAN_POINT('Ctrl Pts',(40.2179872930271,60.6036151476347,0.));
#106924=CARTESIAN_POINT('Ctrl Pts',(40.2232610328717,60.6284073008865,0.));
#106925=CARTESIAN_POINT('Ctrl Pts',(40.2285194291702,60.6532429799494,0.));
#106926=CARTESIAN_POINT('Ctrl Pts',(40.2337624072029,60.678122094098,0.));
#106927=CARTESIAN_POINT('Ctrl Pts',(40.2389898925937,60.7030445528863,0.));
#106928=CARTESIAN_POINT('Ctrl Pts',(40.2442018113116,60.7280102661401,0.));
#106929=CARTESIAN_POINT('Ctrl Pts',(40.2493980896646,60.7530191439603,0.));
#106930=CARTESIAN_POINT('Ctrl Pts',(40.2545786542957,60.7780710967253,0.));
#106931=CARTESIAN_POINT('Ctrl Pts',(40.2597434321803,60.8031660350879,0.));
#106932=CARTESIAN_POINT('Ctrl Pts',(40.2648923506245,60.8283038699703,0.));
#106933=CARTESIAN_POINT('Ctrl Pts',(40.2700253372644,60.8534845125535,0.));
#106934=CARTESIAN_POINT('Ctrl Pts',(40.2751423200637,60.8787078742817,0.));
#106935=CARTESIAN_POINT('Ctrl Pts',(40.2802432273104,60.903973866867,0.));
#106936=CARTESIAN_POINT('Ctrl Pts',(40.2853279876161,60.9292824022888,0.));
#106937=CARTESIAN_POINT('Ctrl Pts',(40.2903965299155,60.9546333927919,0.));
#106938=CARTESIAN_POINT('Ctrl Pts',(40.2954487834688,60.9800267508781,0.));
#106939=CARTESIAN_POINT('Ctrl Pts',(40.3004846778577,61.005462389306,0.));
#106940=CARTESIAN_POINT('Ctrl Pts',(40.3055041429772,61.0309402210915,0.));
#106941=CARTESIAN_POINT('Ctrl Pts',(40.3105071090308,61.0564601595047,0.));
#106942=CARTESIAN_POINT('Ctrl Pts',(40.3154935065263,61.0820221180647,0.));
#106943=CARTESIAN_POINT('Ctrl Pts',(40.3204632662729,61.1076260105265,0.));
#106944=CARTESIAN_POINT('Ctrl Pts',(40.3254163193805,61.1332717508799,0.));
#106945=CARTESIAN_POINT('Ctrl Pts',(40.3303525972621,61.1589592533623,0.));
#106946=CARTESIAN_POINT('Ctrl Pts',(40.3352720316373,61.184688432465,0.));
#106947=CARTESIAN_POINT('Ctrl Pts',(40.3401745545369,61.2104592029376,0.));
#106948=CARTESIAN_POINT('Ctrl Pts',(40.3450600983104,61.2362714797891,0.));
#106949=CARTESIAN_POINT('Ctrl Pts',(40.3499285956297,61.262125178285,0.));
#106950=CARTESIAN_POINT('Ctrl Pts',(40.3547799794672,61.2880202139358,0.));
#106951=CARTESIAN_POINT('Ctrl Pts',(40.3596141830786,61.3139565024838,0.));
#106952=CARTESIAN_POINT('Ctrl Pts',(40.364431139986,61.3399339598852,0.));
#106953=CARTESIAN_POINT('Ctrl Pts',(40.3692307839642,61.3659525022917,0.));
#106954=CARTESIAN_POINT('Ctrl Pts',(40.3740130490233,61.3920120460232,0.));
#106955=CARTESIAN_POINT('Ctrl Pts',(40.3787778694372,61.418112507605,0.));
#106956=CARTESIAN_POINT('Ctrl Pts',(40.3835251797725,61.4442538038053,0.));
#106957=CARTESIAN_POINT('Ctrl Pts',(40.3882549149229,61.4704358516711,0.));
#106958=CARTESIAN_POINT('Ctrl Pts',(40.3929670101363,61.4966585685545,0.));
#106959=CARTESIAN_POINT('Ctrl Pts',(40.3976614010648,61.5229218721532,0.));
#106960=CARTESIAN_POINT('Ctrl Pts',(40.4023380237227,61.5492256804709,0.));
#106961=CARTESIAN_POINT('Ctrl Pts',(40.4069968143953,61.5755699117318,0.));
#106962=CARTESIAN_POINT('Ctrl Pts',(40.4116377095595,61.6019544843009,0.));
#106963=CARTESIAN_POINT('Ctrl Pts',(40.4162606458119,61.628379316608,0.));
#106964=CARTESIAN_POINT('Ctrl Pts',(40.420865559772,61.6548443270397,0.));
#106965=CARTESIAN_POINT('Ctrl Pts',(40.4254523880766,61.6813494339295,0.));
#106966=CARTESIAN_POINT('Ctrl Pts',(40.4300210675848,61.7078945557812,0.));
#106967=CARTESIAN_POINT('Ctrl Pts',(40.4345715355411,61.7344796114409,0.));
#106968=CARTESIAN_POINT('Ctrl Pts',(40.4391037297589,61.7611045202875,0.));
#106969=CARTESIAN_POINT('Ctrl Pts',(40.4436175887942,61.7877692024064,0.));
#106970=CARTESIAN_POINT('Ctrl Pts',(40.448113052135,61.8144735787767,0.));
#106971=CARTESIAN_POINT('Ctrl Pts',(40.4525900597877,61.8412175708524,0.));
#106972=CARTESIAN_POINT('Ctrl Pts',(40.4570485518735,61.8680011001513,0.));
#106973=CARTESIAN_POINT('Ctrl Pts',(40.4614884681884,61.8948240877998,0.));
#106974=CARTESIAN_POINT('Ctrl Pts',(40.4659097478595,61.9216864541758,0.));
#106975=CARTESIAN_POINT('Ctrl Pts',(40.4703123287642,61.9485881182957,0.));
#106976=CARTESIAN_POINT('Ctrl Pts',(40.4746961480045,61.9755289983094,0.));
#106977=CARTESIAN_POINT('Ctrl Pts',(40.4790611429613,62.0025090126008,0.));
#106978=CARTESIAN_POINT('Ctrl Pts',(40.4834072522181,62.0295280807449,0.));
#106979=CARTESIAN_POINT('Ctrl Pts',(40.4877344164407,62.0565861244171,0.));
#106980=CARTESIAN_POINT('Ctrl Pts',(40.4920425795184,62.0836830685665,0.));
#106981=CARTESIAN_POINT('Ctrl Pts',(40.4963316888356,62.110818841691,0.));
#106982=CARTESIAN_POINT('Ctrl Pts',(40.4999919096189,62.1341126810362,0.));
#106983=CARTESIAN_POINT('Ctrl Pts',(40.5027877865723,62.1519925002733,0.));
#106984=CARTESIAN_POINT('Ctrl Pts',(40.5047277935687,62.1644411502524,0.));
#106985=CARTESIAN_POINT('Ctrl Pts',(40.5058175523044,62.1714473137745,0.));
#106986=CARTESIAN_POINT('Ctrl Pts',(40.5060598100837,62.1730054756444,0.));
#106987=CARTESIAN_POINT('',(39.4479504917287,57.8261117662439,12.));
#106988=CARTESIAN_POINT('',(39.4479504917287,57.8261117662439,0.));
#106989=CARTESIAN_POINT('Ctrl Pts',(40.5060598100837,62.1730054756444,12.));
#106990=CARTESIAN_POINT('Ctrl Pts',(40.5058175523044,62.1714473137745,12.));
#106991=CARTESIAN_POINT('Ctrl Pts',(40.5047277935687,62.1644411502524,12.));
#106992=CARTESIAN_POINT('Ctrl Pts',(40.5027877865723,62.1519925002733,12.));
#106993=CARTESIAN_POINT('Ctrl Pts',(40.4999919096189,62.1341126810362,12.));
#106994=CARTESIAN_POINT('Ctrl Pts',(40.4963316888356,62.110818841691,12.));
#106995=CARTESIAN_POINT('Ctrl Pts',(40.4920425795184,62.0836830685665,12.));
#106996=CARTESIAN_POINT('Ctrl Pts',(40.4877344164407,62.0565861244171,12.));
#106997=CARTESIAN_POINT('Ctrl Pts',(40.4834072522181,62.0295280807449,12.));
#106998=CARTESIAN_POINT('Ctrl Pts',(40.4790611429613,62.0025090126008,12.));
#106999=CARTESIAN_POINT('Ctrl Pts',(40.4746961480045,61.9755289983094,12.));
#107000=CARTESIAN_POINT('Ctrl Pts',(40.4703123287642,61.9485881182957,12.));
#107001=CARTESIAN_POINT('Ctrl Pts',(40.4659097478595,61.9216864541758,12.));
#107002=CARTESIAN_POINT('Ctrl Pts',(40.4614884681884,61.8948240877998,12.));
#107003=CARTESIAN_POINT('Ctrl Pts',(40.4570485518735,61.8680011001513,12.));
#107004=CARTESIAN_POINT('Ctrl Pts',(40.4525900597877,61.8412175708524,12.));
#107005=CARTESIAN_POINT('Ctrl Pts',(40.448113052135,61.8144735787767,12.));
#107006=CARTESIAN_POINT('Ctrl Pts',(40.4436175887942,61.7877692024064,12.));
#107007=CARTESIAN_POINT('Ctrl Pts',(40.4391037297589,61.7611045202875,12.));
#107008=CARTESIAN_POINT('Ctrl Pts',(40.4345715355411,61.7344796114409,12.));
#107009=CARTESIAN_POINT('Ctrl Pts',(40.4300210675848,61.7078945557812,12.));
#107010=CARTESIAN_POINT('Ctrl Pts',(40.4254523880766,61.6813494339295,12.));
#107011=CARTESIAN_POINT('Ctrl Pts',(40.420865559772,61.6548443270397,12.));
#107012=CARTESIAN_POINT('Ctrl Pts',(40.4162606458119,61.628379316608,12.));
#107013=CARTESIAN_POINT('Ctrl Pts',(40.4116377095595,61.6019544843009,12.));
#107014=CARTESIAN_POINT('Ctrl Pts',(40.4069968143953,61.5755699117318,12.));
#107015=CARTESIAN_POINT('Ctrl Pts',(40.4023380237227,61.5492256804709,12.));
#107016=CARTESIAN_POINT('Ctrl Pts',(40.3976614010648,61.5229218721532,12.));
#107017=CARTESIAN_POINT('Ctrl Pts',(40.3929670101363,61.4966585685545,12.));
#107018=CARTESIAN_POINT('Ctrl Pts',(40.3882549149229,61.4704358516711,12.));
#107019=CARTESIAN_POINT('Ctrl Pts',(40.3835251797725,61.4442538038053,12.));
#107020=CARTESIAN_POINT('Ctrl Pts',(40.3787778694372,61.418112507605,12.));
#107021=CARTESIAN_POINT('Ctrl Pts',(40.3740130490233,61.3920120460232,12.));
#107022=CARTESIAN_POINT('Ctrl Pts',(40.3692307839642,61.3659525022917,12.));
#107023=CARTESIAN_POINT('Ctrl Pts',(40.364431139986,61.3399339598852,12.));
#107024=CARTESIAN_POINT('Ctrl Pts',(40.3596141830786,61.3139565024838,12.));
#107025=CARTESIAN_POINT('Ctrl Pts',(40.3547799794672,61.2880202139358,12.));
#107026=CARTESIAN_POINT('Ctrl Pts',(40.3499285956297,61.262125178285,12.));
#107027=CARTESIAN_POINT('Ctrl Pts',(40.3450600983104,61.2362714797891,12.));
#107028=CARTESIAN_POINT('Ctrl Pts',(40.3401745545369,61.2104592029376,12.));
#107029=CARTESIAN_POINT('Ctrl Pts',(40.3352720316373,61.184688432465,12.));
#107030=CARTESIAN_POINT('Ctrl Pts',(40.3303525972621,61.1589592533623,12.));
#107031=CARTESIAN_POINT('Ctrl Pts',(40.3254163193805,61.1332717508799,12.));
#107032=CARTESIAN_POINT('Ctrl Pts',(40.3204632662729,61.1076260105265,12.));
#107033=CARTESIAN_POINT('Ctrl Pts',(40.3154935065263,61.0820221180647,12.));
#107034=CARTESIAN_POINT('Ctrl Pts',(40.3105071090308,61.0564601595047,12.));
#107035=CARTESIAN_POINT('Ctrl Pts',(40.3055041429772,61.0309402210915,12.));
#107036=CARTESIAN_POINT('Ctrl Pts',(40.3004846778577,61.005462389306,12.));
#107037=CARTESIAN_POINT('Ctrl Pts',(40.2954487834688,60.9800267508781,12.));
#107038=CARTESIAN_POINT('Ctrl Pts',(40.2903965299155,60.9546333927919,12.));
#107039=CARTESIAN_POINT('Ctrl Pts',(40.2853279876161,60.9292824022888,12.));
#107040=CARTESIAN_POINT('Ctrl Pts',(40.2802432273104,60.903973866867,12.));
#107041=CARTESIAN_POINT('Ctrl Pts',(40.2751423200637,60.8787078742817,12.));
#107042=CARTESIAN_POINT('Ctrl Pts',(40.2700253372644,60.8534845125535,12.));
#107043=CARTESIAN_POINT('Ctrl Pts',(40.2648923506245,60.8283038699703,12.));
#107044=CARTESIAN_POINT('Ctrl Pts',(40.2597434321803,60.8031660350879,12.));
#107045=CARTESIAN_POINT('Ctrl Pts',(40.2545786542957,60.7780710967253,12.));
#107046=CARTESIAN_POINT('Ctrl Pts',(40.2493980896646,60.7530191439603,12.));
#107047=CARTESIAN_POINT('Ctrl Pts',(40.2442018113116,60.7280102661401,12.));
#107048=CARTESIAN_POINT('Ctrl Pts',(40.2389898925937,60.7030445528863,12.));
#107049=CARTESIAN_POINT('Ctrl Pts',(40.2337624072029,60.678122094098,12.));
#107050=CARTESIAN_POINT('Ctrl Pts',(40.2285194291702,60.6532429799494,12.));
#107051=CARTESIAN_POINT('Ctrl Pts',(40.2232610328717,60.6284073008865,12.));
#107052=CARTESIAN_POINT('Ctrl Pts',(40.2179872930271,60.6036151476347,12.));
#107053=CARTESIAN_POINT('Ctrl Pts',(40.2126982847012,60.5788666112043,12.));
#107054=CARTESIAN_POINT('Ctrl Pts',(40.2073940833054,60.5541617828927,12.));
#107055=CARTESIAN_POINT('Ctrl Pts',(40.2020747646012,60.5295007542838,12.));
#107056=CARTESIAN_POINT('Ctrl Pts',(40.1967404047055,60.5048836172424,12.));
#107057=CARTESIAN_POINT('Ctrl Pts',(40.1913910800911,60.4803104639211,12.));
#107058=CARTESIAN_POINT('Ctrl Pts',(40.1860268675875,60.4557813867677,12.));
#107059=CARTESIAN_POINT('Ctrl Pts',(40.1806478443828,60.4312964785269,12.));
#107060=CARTESIAN_POINT('Ctrl Pts',(40.1752540880273,60.4068558322415,12.));
#107061=CARTESIAN_POINT('Ctrl Pts',(40.1698456764387,60.382459541246,12.));
#107062=CARTESIAN_POINT('Ctrl Pts',(40.1644226879043,60.3581076991731,12.));
#107063=CARTESIAN_POINT('Ctrl Pts',(40.158985201081,60.3338003999616,12.));
#107064=CARTESIAN_POINT('Ctrl Pts',(40.1535332949978,60.3095377378589,12.));
#107065=CARTESIAN_POINT('Ctrl Pts',(40.1480670490583,60.2853198074216,12.));
#107066=CARTESIAN_POINT('Ctrl Pts',(40.1425865430468,60.2611467035109,12.));
#107067=CARTESIAN_POINT('Ctrl Pts',(40.13709185713,60.2370185212957,12.));
#107068=CARTESIAN_POINT('Ctrl Pts',(40.1315830718575,60.2129353562618,12.));
#107069=CARTESIAN_POINT('Ctrl Pts',(40.1260602681644,60.1888973042151,12.));
#107070=CARTESIAN_POINT('Ctrl Pts',(40.120523527374,60.164904461283,12.));
#107071=CARTESIAN_POINT('Ctrl Pts',(40.1149729312036,60.1409569239093,12.));
#107072=CARTESIAN_POINT('Ctrl Pts',(40.1094085617672,60.1170547888572,12.));
#107073=CARTESIAN_POINT('Ctrl Pts',(40.1038305015763,60.0931981532194,12.));
#107074=CARTESIAN_POINT('Ctrl Pts',(40.0982388335421,60.0693871144207,12.));
#107075=CARTESIAN_POINT('Ctrl Pts',(40.0926336409787,60.0456217702203,12.));
#107076=CARTESIAN_POINT('Ctrl Pts',(40.0870150076078,60.0219022187066,12.));
#107077=CARTESIAN_POINT('Ctrl Pts',(40.0813830175629,59.9982285582991,12.));
#107078=CARTESIAN_POINT('Ctrl Pts',(40.0757377553893,59.974600887759,12.));
#107079=CARTESIAN_POINT('Ctrl Pts',(40.0700793060475,59.9510193061929,12.));
#107080=CARTESIAN_POINT('Ctrl Pts',(40.0644077549158,59.927483913055,12.));
#107081=CARTESIAN_POINT('Ctrl Pts',(40.0587231877959,59.9039948081428,12.));
#107082=CARTESIAN_POINT('Ctrl Pts',(40.053025690916,59.8805520915972,12.));
#107083=CARTESIAN_POINT('Ctrl Pts',(40.0473153509324,59.8571558639145,12.));
#107084=CARTESIAN_POINT('Ctrl Pts',(40.0415922549314,59.8338062259493,12.));
#107085=CARTESIAN_POINT('Ctrl Pts',(40.035856490434,59.8105032789179,12.));
#107086=CARTESIAN_POINT('Ctrl Pts',(40.0301081454002,59.7872471243942,12.));
#107087=CARTESIAN_POINT('Ctrl Pts',(40.0243473082337,59.7640378643106,12.));
#107088=CARTESIAN_POINT('Ctrl Pts',(40.0185740677821,59.7408756009679,12.));
#107089=CARTESIAN_POINT('Ctrl Pts',(40.0127885133403,59.7177604370403,12.));
#107090=CARTESIAN_POINT('Ctrl Pts',(40.0069907346537,59.6946924755773,12.));
#107091=CARTESIAN_POINT('Ctrl Pts',(40.0011808219241,59.6716718200005,12.));
#107092=CARTESIAN_POINT('Ctrl Pts',(39.9953588658131,59.6486985741041,12.));
#107093=CARTESIAN_POINT('Ctrl Pts',(39.9895249574448,59.6257728420669,12.));
#107094=CARTESIAN_POINT('Ctrl Pts',(39.9836791884079,59.6028947284562,12.));
#107095=CARTESIAN_POINT('Ctrl Pts',(39.9778216507605,59.5800643382315,12.));
#107096=CARTESIAN_POINT('Ctrl Pts',(39.9719524370345,59.5572817767388,12.));
#107097=CARTESIAN_POINT('Ctrl Pts',(39.9660716402403,59.5345471497129,12.));
#107098=CARTESIAN_POINT('Ctrl Pts',(39.9601793538682,59.5118605632891,12.));
#107099=CARTESIAN_POINT('Ctrl Pts',(39.9542756718922,59.4892221240069,12.));
#107100=CARTESIAN_POINT('Ctrl Pts',(39.9483606887737,59.4666319388133,12.));
#107101=CARTESIAN_POINT('Ctrl Pts',(39.9424344994672,59.4440901150582,12.));
#107102=CARTESIAN_POINT('Ctrl Pts',(39.9364971994242,59.4215967604968,12.));
#107103=CARTESIAN_POINT('Ctrl Pts',(39.9305488845958,59.3991519833016,12.));
#107104=CARTESIAN_POINT('Ctrl Pts',(39.9245896514367,59.3767558920675,12.));
#107105=CARTESIAN_POINT('Ctrl Pts',(39.9186195969104,59.3544085958151,12.));
#107106=CARTESIAN_POINT('Ctrl Pts',(39.9126388184936,59.3321102039852,12.));
#107107=CARTESIAN_POINT('Ctrl Pts',(39.9066474141803,59.3098608264419,12.));
#107108=CARTESIAN_POINT('Ctrl Pts',(39.9006454824845,59.2876605734847,12.));
#107109=CARTESIAN_POINT('Ctrl Pts',(39.8946331224438,59.2655095558521,12.));
#107110=CARTESIAN_POINT('Ctrl Pts',(39.8886104336242,59.2434078847247,12.));
#107111=CARTESIAN_POINT('Ctrl Pts',(39.8825775161267,59.2213556717209,12.));
#107112=CARTESIAN_POINT('Ctrl Pts',(39.8765344705909,59.1993530289029,12.));
#107113=CARTESIAN_POINT('Ctrl Pts',(39.8704813981988,59.1774000687879,12.));
#107114=CARTESIAN_POINT('Ctrl Pts',(39.8644184006786,59.1554969043522,12.));
#107115=CARTESIAN_POINT('Ctrl Pts',(39.8583455803105,59.1336436490342,12.));
#107116=CARTESIAN_POINT('Ctrl Pts',(39.8522630399328,59.1118404167292,12.));
#107117=CARTESIAN_POINT('Ctrl Pts',(39.8461708829456,59.0900873217981,12.));
#107118=CARTESIAN_POINT('Ctrl Pts',(39.8400692133139,59.0683844790764,12.));
#107119=CARTESIAN_POINT('Ctrl Pts',(39.8339581355715,59.0467320038784,12.));
#107120=CARTESIAN_POINT('Ctrl Pts',(39.8278377548262,59.0251300119973,12.));
#107121=CARTESIAN_POINT('Ctrl Pts',(39.821708176766,59.0035786197024,12.));
#107122=CARTESIAN_POINT('Ctrl Pts',(39.8155695076626,58.9820779437485,12.));
#107123=CARTESIAN_POINT('Ctrl Pts',(39.8094218543782,58.9606281013875,12.));
#107124=CARTESIAN_POINT('Ctrl Pts',(39.8032653243712,58.9392292103747,12.));
#107125=CARTESIAN_POINT('Ctrl Pts',(39.7971000257044,58.9178813889704,12.));
#107126=CARTESIAN_POINT('Ctrl Pts',(39.7909260670517,58.8965847559391,12.));
#107127=CARTESIAN_POINT('Ctrl Pts',(39.7847435576996,58.8753394305586,12.));
#107128=CARTESIAN_POINT('Ctrl Pts',(39.7785526075478,58.8541455326231,12.));
#107129=CARTESIAN_POINT('Ctrl Pts',(39.772353327112,58.8330031824453,12.));
#107130=CARTESIAN_POINT('Ctrl Pts',(39.7661458275274,58.8119125008517,12.));
#107131=CARTESIAN_POINT('Ctrl Pts',(39.759930220552,58.7908736091798,12.));
#107132=CARTESIAN_POINT('Ctrl Pts',(39.7537066185812,58.7698866293029,12.));
#107133=CARTESIAN_POINT('Ctrl Pts',(39.7474751346598,58.7489516836445,12.));
#107134=CARTESIAN_POINT('Ctrl Pts',(39.7412358824953,58.7280688951916,12.));
#107135=CARTESIAN_POINT('Ctrl Pts',(39.7349889764749,58.7072383875027,12.));
#107136=CARTESIAN_POINT('Ctrl Pts',(39.7287345316681,58.6864602847088,12.));
#107137=CARTESIAN_POINT('Ctrl Pts',(39.72247266381,58.6657347115034,12.));
#107138=CARTESIAN_POINT('Ctrl Pts',(39.7162034892899,58.6450617931274,12.));
#107139=CARTESIAN_POINT('Ctrl Pts',(39.7099271251413,58.6244416553562,12.));
#107140=CARTESIAN_POINT('Ctrl Pts',(39.7036436890232,58.6038744244659,12.));
#107141=CARTESIAN_POINT('Ctrl Pts',(39.6973532992539,58.5833602272744,12.));
#107142=CARTESIAN_POINT('Ctrl Pts',(39.6910560748629,58.5628991912052,12.));
#107143=CARTESIAN_POINT('Ctrl Pts',(39.6847521356395,58.5424914443415,12.));
#107144=CARTESIAN_POINT('Ctrl Pts',(39.6784416021826,58.5221371154761,12.));
#107145=CARTESIAN_POINT('Ctrl Pts',(39.6721245959531,58.5018363341604,12.));
#107146=CARTESIAN_POINT('Ctrl Pts',(39.6658012391815,58.4815892306066,12.));
#107147=CARTESIAN_POINT('Ctrl Pts',(39.6594716547689,58.4613959355788,12.));
#107148=CARTESIAN_POINT('Ctrl Pts',(39.653135966204,58.4412565802979,12.));
#107149=CARTESIAN_POINT('Ctrl Pts',(39.6467942974451,58.4211712963004,12.));
#107150=CARTESIAN_POINT('Ctrl Pts',(39.6404467729094,58.4011402154196,12.));
#107151=CARTESIAN_POINT('Ctrl Pts',(39.6340935177476,58.3811634701037,12.));
#107152=CARTESIAN_POINT('Ctrl Pts',(39.6277346580892,58.3612411936905,12.));
#107153=CARTESIAN_POINT('Ctrl Pts',(39.6213703212531,58.3413735206424,12.));
#107154=CARTESIAN_POINT('Ctrl Pts',(39.6150006360914,58.3215605869221,12.));
#107155=CARTESIAN_POINT('Ctrl Pts',(39.6086257327583,58.3018025297324,12.));
#107156=CARTESIAN_POINT('Ctrl Pts',(39.6022457420789,58.2820994868118,12.));
#107157=CARTESIAN_POINT('Ctrl Pts',(39.5958607950239,58.2624515958419,12.));
#107158=CARTESIAN_POINT('Ctrl Pts',(39.5894710221713,58.2428589938369,12.));
#107159=CARTESIAN_POINT('Ctrl Pts',(39.5830765530891,58.2233218164366,12.));
#107160=CARTESIAN_POINT('Ctrl Pts',(39.57667751752,58.2038401992457,12.));
#107161=CARTESIAN_POINT('Ctrl Pts',(39.5702740467999,58.1844142794338,12.));
#107162=CARTESIAN_POINT('Ctrl Pts',(39.563866275018,58.1650441970387,12.));
#107163=CARTESIAN_POINT('Ctrl Pts',(39.5574543406981,58.1457300968499,12.));
#107164=CARTESIAN_POINT('Ctrl Pts',(39.5510383869505,58.126472128574,12.));
#107165=CARTESIAN_POINT('Ctrl Pts',(39.5446185579638,58.1072704428928,12.));
#107166=CARTESIAN_POINT('Ctrl Pts',(39.5381949959221,58.0881251879921,12.));
#107167=CARTESIAN_POINT('Ctrl Pts',(39.5317678383217,58.0690365065374,12.));
#107168=CARTESIAN_POINT('Ctrl Pts',(39.5253372136887,58.0500045308412,12.));
#107169=CARTESIAN_POINT('Ctrl Pts',(39.5189032457184,58.0310293875262,12.));
#107170=CARTESIAN_POINT('Ctrl Pts',(39.5124660614976,58.0121112067896,12.));
#107171=CARTESIAN_POINT('Ctrl Pts',(39.5060257981225,57.9932501298522,12.));
#107172=CARTESIAN_POINT('Ctrl Pts',(39.499582610674,57.974446317937,12.));
#107173=CARTESIAN_POINT('Ctrl Pts',(39.4931366776714,57.9556999583892,12.));
#107174=CARTESIAN_POINT('Ctrl Pts',(39.4866881842317,57.9370112456631,12.));
#107175=CARTESIAN_POINT('Ctrl Pts',(39.4802373061058,57.9183803632404,12.));
#107176=CARTESIAN_POINT('Ctrl Pts',(39.473784194937,57.8998074670478,12.));
#107177=CARTESIAN_POINT('Ctrl Pts',(39.4673289592259,57.8812926637177,12.));
#107178=CARTESIAN_POINT('Ctrl Pts',(39.4608716627117,57.8628360096803,12.));
#107179=CARTESIAN_POINT('Ctrl Pts',(39.4557042029652,57.8481172247496,12.));
#107180=CARTESIAN_POINT('Ctrl Pts',(39.4518277003553,57.8371043151411,12.));
#107181=CARTESIAN_POINT('Ctrl Pts',(39.4492429618443,57.8297740100947,12.));
#107182=CARTESIAN_POINT('Ctrl Pts',(39.4479504917287,57.8261117662439,12.));
#107183=CARTESIAN_POINT('Ctrl Pts',(39.2292784191814,62.9864049293895,-5.55111512312578E-16));
#107184=CARTESIAN_POINT('Ctrl Pts',(39.2292784191814,62.9864049293895,4.));
#107185=CARTESIAN_POINT('Ctrl Pts',(39.2292784191814,62.9864049293895,8.));
#107186=CARTESIAN_POINT('Ctrl Pts',(39.2292784191814,62.9864049293895,12.));
#107187=CARTESIAN_POINT('Ctrl Pts',(39.3205491216487,63.0475916539466,-5.55111512312578E-16));
#107188=CARTESIAN_POINT('Ctrl Pts',(39.3205491216487,63.0475916539466,4.));
#107189=CARTESIAN_POINT('Ctrl Pts',(39.3205491216487,63.0475916539466,8.));
#107190=CARTESIAN_POINT('Ctrl Pts',(39.3205491216487,63.0475916539466,12.));
#107191=CARTESIAN_POINT('Ctrl Pts',(39.5164137621552,63.0996457958587,-5.55111512312578E-16));
#107192=CARTESIAN_POINT('Ctrl Pts',(39.5164137621552,63.0996457958587,4.00000000000001));
#107193=CARTESIAN_POINT('Ctrl Pts',(39.5164137621552,63.0996457958587,8.));
#107194=CARTESIAN_POINT('Ctrl Pts',(39.5164137621552,63.0996457958587,12.));
#107195=CARTESIAN_POINT('Ctrl Pts',(39.704957504468,63.0378706912078,-5.55111512312578E-16));
#107196=CARTESIAN_POINT('Ctrl Pts',(39.704957504468,63.0378706912078,4.));
#107197=CARTESIAN_POINT('Ctrl Pts',(39.704957504468,63.0378706912078,8.00000000000001));
#107198=CARTESIAN_POINT('Ctrl Pts',(39.704957504468,63.0378706912078,12.));
#107199=CARTESIAN_POINT('Ctrl Pts',(39.7746412831482,62.9938720098785,-5.55111512312578E-16));
#107200=CARTESIAN_POINT('Ctrl Pts',(39.7746412831482,62.9938720098785,4.));
#107201=CARTESIAN_POINT('Ctrl Pts',(39.7746412831482,62.9938720098785,8.));
#107202=CARTESIAN_POINT('Ctrl Pts',(39.7746412831482,62.9938720098785,12.));
#107203=CARTESIAN_POINT('',(39.2292784191814,62.9864049293895,2.77555756156289E-16));
#107204=CARTESIAN_POINT('',(39.774641283148,62.9938720098781,0.));
#107205=CARTESIAN_POINT('Ctrl Pts',(39.2292784191814,62.9864049293895,-1.38777878078145E-16));
#107206=CARTESIAN_POINT('Ctrl Pts',(39.3205491216487,63.0475916539466,-1.38777878078145E-16));
#107207=CARTESIAN_POINT('Ctrl Pts',(39.4324717733667,63.0773368778964,-1.38777878078144E-16));
#107208=CARTESIAN_POINT('Ctrl Pts',(39.5420039277153,63.0699133682745,-1.38777878078145E-16));
#107209=CARTESIAN_POINT('Ctrl Pts',(39.6241530434768,63.0643457360582,-1.38777878078145E-16));
#107210=CARTESIAN_POINT('Ctrl Pts',(39.704957504468,63.0378706912078,-1.38777878078145E-16));
#107211=CARTESIAN_POINT('Ctrl Pts',(39.7746412831482,62.9938720098785,-1.38777878078145E-16));
#107212=CARTESIAN_POINT('',(39.774641283148,62.9938720098781,12.));
#107213=CARTESIAN_POINT('Ctrl Pts',(39.7746412831482,62.9938720098785,-5.55111512312578E-16));
#107214=CARTESIAN_POINT('Ctrl Pts',(39.7746412831482,62.9938720098785,4.));
#107215=CARTESIAN_POINT('Ctrl Pts',(39.7746412831482,62.9938720098785,8.));
#107216=CARTESIAN_POINT('Ctrl Pts',(39.7746412831482,62.9938720098785,12.));
#107217=CARTESIAN_POINT('',(39.2292784191814,62.9864049293895,12.));
#107218=CARTESIAN_POINT('Ctrl Pts',(39.7746412831482,62.9938720098785,12.));
#107219=CARTESIAN_POINT('Ctrl Pts',(39.704957504468,63.0378706912078,12.));
#107220=CARTESIAN_POINT('Ctrl Pts',(39.6241530434768,63.0643457360582,12.));
#107221=CARTESIAN_POINT('Ctrl Pts',(39.5420039277153,63.0699133682745,12.));
#107222=CARTESIAN_POINT('Ctrl Pts',(39.4324717733667,63.0773368778964,12.));
#107223=CARTESIAN_POINT('Ctrl Pts',(39.3205491216487,63.0475916539466,12.));
#107224=CARTESIAN_POINT('Ctrl Pts',(39.2292784191814,62.9864049293895,12.));
#107225=CARTESIAN_POINT('Ctrl Pts',(39.2292784191814,62.9864049293895,12.));
#107226=CARTESIAN_POINT('Ctrl Pts',(39.2292784191814,62.9864049293895,8.));
#107227=CARTESIAN_POINT('Ctrl Pts',(39.2292784191814,62.9864049293895,4.));
#107228=CARTESIAN_POINT('Ctrl Pts',(39.2292784191814,62.9864049293895,-5.55111512312578E-16));
#107229=CARTESIAN_POINT('Origin',(2.01319694273778E-10,3.16193356404481E-10,
0.));
#107230=CARTESIAN_POINT('Origin',(2.01319694273778E-10,3.16193356404481E-10,
12.));
#107231=CARTESIAN_POINT('Origin',(2.01319694273778E-10,3.16193356404481E-10,
0.));
#107232=CARTESIAN_POINT('Ctrl Pts',(45.5911481700231,58.9211100416396,0.));
#107233=CARTESIAN_POINT('Ctrl Pts',(45.5911481700231,58.9211100416396,4.));
#107234=CARTESIAN_POINT('Ctrl Pts',(45.591148170023,58.9211100416396,8.));
#107235=CARTESIAN_POINT('Ctrl Pts',(45.591148170023,58.9211100416396,12.));
#107236=CARTESIAN_POINT('Ctrl Pts',(45.6780528262179,58.8538661785412,0.));
#107237=CARTESIAN_POINT('Ctrl Pts',(45.6780528262179,58.8538661785412,4.));
#107238=CARTESIAN_POINT('Ctrl Pts',(45.6780528262179,58.8538661785413,8.00000000000001));
#107239=CARTESIAN_POINT('Ctrl Pts',(45.6780528262179,58.8538661785413,12.));
#107240=CARTESIAN_POINT('Ctrl Pts',(45.7893619681938,58.6845061116498,0.));
#107241=CARTESIAN_POINT('Ctrl Pts',(45.7893619681938,58.6845061116498,4.));
#107242=CARTESIAN_POINT('Ctrl Pts',(45.7893619681937,58.6845061116498,7.99999999999999));
#107243=CARTESIAN_POINT('Ctrl Pts',(45.7893619681937,58.6845061116498,12.));
#107244=CARTESIAN_POINT('Ctrl Pts',(45.7903667155981,58.4861028141708,0.));
#107245=CARTESIAN_POINT('Ctrl Pts',(45.7903667155981,58.4861028141708,4.));
#107246=CARTESIAN_POINT('Ctrl Pts',(45.790366715598,58.486102814171,8.00000000000001));
#107247=CARTESIAN_POINT('Ctrl Pts',(45.790366715598,58.486102814171,12.));
#107248=CARTESIAN_POINT('Ctrl Pts',(45.7706564944768,58.4060826907376,0.));
#107249=CARTESIAN_POINT('Ctrl Pts',(45.7706564944768,58.4060826907376,4.));
#107250=CARTESIAN_POINT('Ctrl Pts',(45.7706564944767,58.4060826907378,8.));
#107251=CARTESIAN_POINT('Ctrl Pts',(45.7706564944767,58.4060826907378,12.));
#107252=CARTESIAN_POINT('',(45.5911481700231,58.9211100416396,0.));
#107253=CARTESIAN_POINT('',(45.7706564944766,58.4060826907377,0.));
#107254=CARTESIAN_POINT('Ctrl Pts',(45.5911481700231,58.9211100416396,2.77555756156289E-16));
#107255=CARTESIAN_POINT('Ctrl Pts',(45.6780528262179,58.8538661785412,2.77555756156289E-16));
#107256=CARTESIAN_POINT('Ctrl Pts',(45.7416580502041,58.7570889974604,2.77555756156289E-16));
#107257=CARTESIAN_POINT('Ctrl Pts',(45.7692455126976,58.6508283125143,2.77555756156289E-16));
#107258=CARTESIAN_POINT('Ctrl Pts',(45.7899361095677,58.5711327988047,2.77555756156289E-16));
#107259=CARTESIAN_POINT('Ctrl Pts',(45.7903667155981,58.4861028141708,2.77555756156289E-16));
#107260=CARTESIAN_POINT('Ctrl Pts',(45.7706564944768,58.4060826907376,2.77555756156289E-16));
#107261=CARTESIAN_POINT('',(45.7706564944766,58.4060826907378,12.));
#107262=CARTESIAN_POINT('Ctrl Pts',(45.7706564944768,58.4060826907376,0.));
#107263=CARTESIAN_POINT('Ctrl Pts',(45.7706564944768,58.4060826907376,4.));
#107264=CARTESIAN_POINT('Ctrl Pts',(45.7706564944767,58.4060826907378,8.));
#107265=CARTESIAN_POINT('Ctrl Pts',(45.7706564944767,58.4060826907378,12.));
#107266=CARTESIAN_POINT('',(45.591148170023,58.9211100416396,12.));
#107267=CARTESIAN_POINT('Ctrl Pts',(45.7706564944767,58.4060826907378,12.));
#107268=CARTESIAN_POINT('Ctrl Pts',(45.790366715598,58.486102814171,12.));
#107269=CARTESIAN_POINT('Ctrl Pts',(45.7899361095676,58.5711327988048,12.));
#107270=CARTESIAN_POINT('Ctrl Pts',(45.7692455126975,58.6508283125143,12.));
#107271=CARTESIAN_POINT('Ctrl Pts',(45.7416580502041,58.7570889974605,12.));
#107272=CARTESIAN_POINT('Ctrl Pts',(45.6780528262179,58.8538661785413,12.));
#107273=CARTESIAN_POINT('Ctrl Pts',(45.591148170023,58.9211100416396,12.));
#107274=CARTESIAN_POINT('Ctrl Pts',(45.591148170023,58.9211100416396,12.));
#107275=CARTESIAN_POINT('Ctrl Pts',(45.591148170023,58.9211100416396,8.));
#107276=CARTESIAN_POINT('Ctrl Pts',(45.5911481700231,58.9211100416396,4.));
#107277=CARTESIAN_POINT('Ctrl Pts',(45.5911481700231,58.9211100416396,0.));
#107278=CARTESIAN_POINT('Ctrl Pts',(44.3377168516418,54.1679505278134,0.));
#107279=CARTESIAN_POINT('Ctrl Pts',(44.3377168516418,54.1679505278134,12.));
#107280=CARTESIAN_POINT('Ctrl Pts',(44.3393235891014,54.1714861895278,0.));
#107281=CARTESIAN_POINT('Ctrl Pts',(44.3393235891014,54.1714861895278,12.));
#107282=CARTESIAN_POINT('Ctrl Pts',(44.3425373700829,54.1785633257456,0.));
#107283=CARTESIAN_POINT('Ctrl Pts',(44.3425373700829,54.1785633257456,12.));
#107284=CARTESIAN_POINT('Ctrl Pts',(44.3473589597467,54.189196468444,0.));
#107285=CARTESIAN_POINT('Ctrl Pts',(44.3473589597467,54.189196468444,12.));
#107286=CARTESIAN_POINT('Ctrl Pts',(44.3537895823819,54.203408870162,0.));
#107287=CARTESIAN_POINT('Ctrl Pts',(44.3537895823819,54.203408870162,12.));
#107288=CARTESIAN_POINT('Ctrl Pts',(44.3618309103245,54.2212325005847,0.));
#107289=CARTESIAN_POINT('Ctrl Pts',(44.3618309103245,54.2212325005847,12.));
#107290=CARTESIAN_POINT('Ctrl Pts',(44.3698752533509,54.2391142386354,0.));
#107291=CARTESIAN_POINT('Ctrl Pts',(44.3698752533509,54.2391142386354,12.));
#107292=CARTESIAN_POINT('Ctrl Pts',(44.3779225430461,54.2570540336536,0.));
#107293=CARTESIAN_POINT('Ctrl Pts',(44.3779225430461,54.2570540336536,12.));
#107294=CARTESIAN_POINT('Ctrl Pts',(44.3859726620288,54.2750517888695,0.));
#107295=CARTESIAN_POINT('Ctrl Pts',(44.3859726620288,54.2750517888695,12.));
#107296=CARTESIAN_POINT('Ctrl Pts',(44.3940254456427,54.2931073621661,0.));
#107297=CARTESIAN_POINT('Ctrl Pts',(44.3940254456427,54.2931073621661,12.));
#107298=CARTESIAN_POINT('Ctrl Pts',(44.4020807028143,54.3112205860776,0.));
#107299=CARTESIAN_POINT('Ctrl Pts',(44.4020807028143,54.3112205860776,12.));
#107300=CARTESIAN_POINT('Ctrl Pts',(44.4101382321834,54.3293912830237,0.));
#107301=CARTESIAN_POINT('Ctrl Pts',(44.4101382321834,54.3293912830237,12.));
#107302=CARTESIAN_POINT('Ctrl Pts',(44.4181978395814,54.347619281931,0.));
#107303=CARTESIAN_POINT('Ctrl Pts',(44.4181978395814,54.347619281931,12.));
#107304=CARTESIAN_POINT('Ctrl Pts',(44.4262593564664,54.3659044357064,0.));
#107305=CARTESIAN_POINT('Ctrl Pts',(44.4262593564664,54.3659044357064,12.));
#107306=CARTESIAN_POINT('Ctrl Pts',(44.4343226339554,54.3842466156151,0.));
#107307=CARTESIAN_POINT('Ctrl Pts',(44.4343226339554,54.3842466156151,12.));
#107308=CARTESIAN_POINT('Ctrl Pts',(44.442387534098,54.4026457030316,0.));
#107309=CARTESIAN_POINT('Ctrl Pts',(44.442387534098,54.4026457030316,12.));
#107310=CARTESIAN_POINT('Ctrl Pts',(44.4504539226336,54.4211015825959,0.));
#107311=CARTESIAN_POINT('Ctrl Pts',(44.4504539226336,54.4211015825959,12.));
#107312=CARTESIAN_POINT('Ctrl Pts',(44.4585216599933,54.4396141337008,0.));
#107313=CARTESIAN_POINT('Ctrl Pts',(44.4585216599933,54.4396141337008,12.));
#107314=CARTESIAN_POINT('Ctrl Pts',(44.4665905967701,54.4581832262072,0.));
#107315=CARTESIAN_POINT('Ctrl Pts',(44.4665905967701,54.4581832262072,12.));
#107316=CARTESIAN_POINT('Ctrl Pts',(44.4746605784056,54.4768087248854,0.));
#107317=CARTESIAN_POINT('Ctrl Pts',(44.4746605784056,54.4768087248854,12.));
#107318=CARTESIAN_POINT('Ctrl Pts',(44.482731448127,54.4954904921938,0.));
#107319=CARTESIAN_POINT('Ctrl Pts',(44.482731448127,54.4954904921938,12.));
#107320=CARTESIAN_POINT('Ctrl Pts',(44.4908030503209,54.5142283914684,0.));
#107321=CARTESIAN_POINT('Ctrl Pts',(44.4908030503209,54.5142283914684,12.));
#107322=CARTESIAN_POINT('Ctrl Pts',(44.4988752343714,54.5330222905438,0.));
#107323=CARTESIAN_POINT('Ctrl Pts',(44.4988752343714,54.5330222905438,12.));
#107324=CARTESIAN_POINT('Ctrl Pts',(44.5069478544945,54.5518720616016,0.));
#107325=CARTESIAN_POINT('Ctrl Pts',(44.5069478544945,54.5518720616016,12.));
#107326=CARTESIAN_POINT('Ctrl Pts',(44.5150207678988,54.5707775794412,0.));
#107327=CARTESIAN_POINT('Ctrl Pts',(44.5150207678988,54.5707775794412,12.));
#107328=CARTESIAN_POINT('Ctrl Pts',(44.5230938335167,54.5897387202815,0.));
#107329=CARTESIAN_POINT('Ctrl Pts',(44.5230938335167,54.5897387202815,12.));
#107330=CARTESIAN_POINT('Ctrl Pts',(44.5311669104514,54.6087553602914,0.));
#107331=CARTESIAN_POINT('Ctrl Pts',(44.5311669104514,54.6087553602914,12.));
#107332=CARTESIAN_POINT('Ctrl Pts',(44.5392398566802,54.6278273743587,0.));
#107333=CARTESIAN_POINT('Ctrl Pts',(44.5392398566802,54.6278273743587,12.));
#107334=CARTESIAN_POINT('Ctrl Pts',(44.5473125297311,54.6469546367408,0.));
#107335=CARTESIAN_POINT('Ctrl Pts',(44.5473125297311,54.6469546367408,12.));
#107336=CARTESIAN_POINT('Ctrl Pts',(44.5553847872721,54.6661370216252,0.));
#107337=CARTESIAN_POINT('Ctrl Pts',(44.5553847872721,54.6661370216252,12.));
#107338=CARTESIAN_POINT('Ctrl Pts',(44.5634564876863,54.6853744036751,0.));
#107339=CARTESIAN_POINT('Ctrl Pts',(44.5634564876863,54.6853744036751,12.));
#107340=CARTESIAN_POINT('Ctrl Pts',(44.5715274907619,54.7046666586754,0.));
#107341=CARTESIAN_POINT('Ctrl Pts',(44.5715274907619,54.7046666586754,12.));
#107342=CARTESIAN_POINT('Ctrl Pts',(44.5795976579454,54.7240136637717,0.));
#107343=CARTESIAN_POINT('Ctrl Pts',(44.5795976579454,54.7240136637717,12.));
#107344=CARTESIAN_POINT('Ctrl Pts',(44.5876668519661,54.7434152971267,0.));
#107345=CARTESIAN_POINT('Ctrl Pts',(44.5876668519661,54.7434152971267,12.));
#107346=CARTESIAN_POINT('Ctrl Pts',(44.5957349366058,54.7628714377037,0.));
#107347=CARTESIAN_POINT('Ctrl Pts',(44.5957349366058,54.7628714377037,12.));
#107348=CARTESIAN_POINT('Ctrl Pts',(44.6038017764309,54.7823819650149,0.));
#107349=CARTESIAN_POINT('Ctrl Pts',(44.6038017764309,54.7823819650149,12.));
#107350=CARTESIAN_POINT('Ctrl Pts',(44.6118672364906,54.8019467588278,0.));
#107351=CARTESIAN_POINT('Ctrl Pts',(44.6118672364906,54.8019467588278,12.));
#107352=CARTESIAN_POINT('Ctrl Pts',(44.6199311823293,54.8215656991837,0.));
#107353=CARTESIAN_POINT('Ctrl Pts',(44.6199311823293,54.8215656991837,12.));
#107354=CARTESIAN_POINT('Ctrl Pts',(44.6279934801168,54.8412386665276,0.));
#107355=CARTESIAN_POINT('Ctrl Pts',(44.6279934801168,54.8412386665276,12.));
#107356=CARTESIAN_POINT('Ctrl Pts',(44.6360539967392,54.860965541796,0.));
#107357=CARTESIAN_POINT('Ctrl Pts',(44.6360539967392,54.860965541796,12.));
#107358=CARTESIAN_POINT('Ctrl Pts',(44.6441125999063,54.8807462065164,0.));
#107359=CARTESIAN_POINT('Ctrl Pts',(44.6441125999063,54.8807462065164,12.));
#107360=CARTESIAN_POINT('Ctrl Pts',(44.6521691582533,54.9005805428969,0.));
#107361=CARTESIAN_POINT('Ctrl Pts',(44.6521691582533,54.9005805428969,12.));
#107362=CARTESIAN_POINT('Ctrl Pts',(44.6602235412836,54.9204684337822,0.));
#107363=CARTESIAN_POINT('Ctrl Pts',(44.6602235412836,54.9204684337822,12.));
#107364=CARTESIAN_POINT('Ctrl Pts',(44.6682756193147,54.9404097626077,0.));
#107365=CARTESIAN_POINT('Ctrl Pts',(44.6682756193147,54.9404097626077,12.));
#107366=CARTESIAN_POINT('Ctrl Pts',(44.6763252634258,54.9604044133501,0.));
#107367=CARTESIAN_POINT('Ctrl Pts',(44.6763252634258,54.9604044133501,12.));
#107368=CARTESIAN_POINT('Ctrl Pts',(44.6843723454,54.9804522704686,0.));
#107369=CARTESIAN_POINT('Ctrl Pts',(44.6843723454,54.9804522704686,12.));
#107370=CARTESIAN_POINT('Ctrl Pts',(44.6924167376869,55.0005532188667,0.));
#107371=CARTESIAN_POINT('Ctrl Pts',(44.6924167376869,55.0005532188667,12.));
#107372=CARTESIAN_POINT('Ctrl Pts',(44.7004583134249,55.0207071439237,0.));
#107373=CARTESIAN_POINT('Ctrl Pts',(44.7004583134249,55.0207071439237,12.));
#107374=CARTESIAN_POINT('Ctrl Pts',(44.7084969464513,55.0409139315078,0.));
#107375=CARTESIAN_POINT('Ctrl Pts',(44.7084969464513,55.0409139315078,12.));
#107376=CARTESIAN_POINT('Ctrl Pts',(44.7165325113159,55.0611734679894,0.));
#107377=CARTESIAN_POINT('Ctrl Pts',(44.7165325113159,55.0611734679894,12.));
#107378=CARTESIAN_POINT('Ctrl Pts',(44.7245648832979,55.0814856402496,0.));
#107379=CARTESIAN_POINT('Ctrl Pts',(44.7245648832979,55.0814856402496,12.));
#107380=CARTESIAN_POINT('Ctrl Pts',(44.7325939384035,55.1018503356796,0.));
#107381=CARTESIAN_POINT('Ctrl Pts',(44.7325939384035,55.1018503356796,12.));
#107382=CARTESIAN_POINT('Ctrl Pts',(44.7406195533479,55.1222674421743,0.));
#107383=CARTESIAN_POINT('Ctrl Pts',(44.7406195533479,55.1222674421743,12.));
#107384=CARTESIAN_POINT('Ctrl Pts',(44.7486416055419,55.14273684812,0.));
#107385=CARTESIAN_POINT('Ctrl Pts',(44.7486416055419,55.14273684812,12.));
#107386=CARTESIAN_POINT('Ctrl Pts',(44.7566599730773,55.1632584423815,0.));
#107387=CARTESIAN_POINT('Ctrl Pts',(44.7566599730773,55.1632584423815,12.));
#107388=CARTESIAN_POINT('Ctrl Pts',(44.7646745347109,55.1838321142779,0.));
#107389=CARTESIAN_POINT('Ctrl Pts',(44.7646745347109,55.1838321142779,12.));
#107390=CARTESIAN_POINT('Ctrl Pts',(44.7726851698618,55.2044577535866,0.));
#107391=CARTESIAN_POINT('Ctrl Pts',(44.7726851698618,55.2044577535866,12.));
#107392=CARTESIAN_POINT('Ctrl Pts',(44.7806917586077,55.2251352505475,0.));
#107393=CARTESIAN_POINT('Ctrl Pts',(44.7806917586077,55.2251352505475,12.));
#107394=CARTESIAN_POINT('Ctrl Pts',(44.7886941816823,55.2458644958617,0.));
#107395=CARTESIAN_POINT('Ctrl Pts',(44.7886941816823,55.2458644958617,12.));
#107396=CARTESIAN_POINT('Ctrl Pts',(44.7966923204741,55.2666453806883,0.));
#107397=CARTESIAN_POINT('Ctrl Pts',(44.7966923204741,55.2666453806883,12.));
#107398=CARTESIAN_POINT('Ctrl Pts',(44.8046860570245,55.287477796635,0.));
#107399=CARTESIAN_POINT('Ctrl Pts',(44.8046860570245,55.287477796635,12.));
#107400=CARTESIAN_POINT('Ctrl Pts',(44.812675274021,55.3083616357605,0.));
#107401=CARTESIAN_POINT('Ctrl Pts',(44.812675274021,55.3083616357605,12.));
#107402=CARTESIAN_POINT('Ctrl Pts',(44.8206598547888,55.3292967905726,0.));
#107403=CARTESIAN_POINT('Ctrl Pts',(44.8206598547888,55.3292967905726,12.));
#107404=CARTESIAN_POINT('Ctrl Pts',(44.8286396832849,55.350283154023,0.));
#107405=CARTESIAN_POINT('Ctrl Pts',(44.8286396832849,55.350283154023,12.));
#107406=CARTESIAN_POINT('Ctrl Pts',(44.8366146440896,55.3713206194962,0.));
#107407=CARTESIAN_POINT('Ctrl Pts',(44.8366146440896,55.3713206194962,12.));
#107408=CARTESIAN_POINT('Ctrl Pts',(44.8445846224033,55.3924090808002,0.));
#107409=CARTESIAN_POINT('Ctrl Pts',(44.8445846224033,55.3924090808002,12.));
#107410=CARTESIAN_POINT('Ctrl Pts',(44.8525495040397,55.4135484321706,0.));
#107411=CARTESIAN_POINT('Ctrl Pts',(44.8525495040397,55.4135484321706,12.));
#107412=CARTESIAN_POINT('Ctrl Pts',(44.8605091754208,55.4347385682697,0.));
#107413=CARTESIAN_POINT('Ctrl Pts',(44.8605091754208,55.4347385682697,12.));
#107414=CARTESIAN_POINT('Ctrl Pts',(44.8684635235727,55.4559793841838,0.));
#107415=CARTESIAN_POINT('Ctrl Pts',(44.8684635235727,55.4559793841838,12.));
#107416=CARTESIAN_POINT('Ctrl Pts',(44.8764124361218,55.4772707754139,0.));
#107417=CARTESIAN_POINT('Ctrl Pts',(44.8764124361218,55.4772707754139,12.));
#107418=CARTESIAN_POINT('Ctrl Pts',(44.8843558012903,55.4986126378676,0.));
#107419=CARTESIAN_POINT('Ctrl Pts',(44.8843558012903,55.4986126378676,12.));
#107420=CARTESIAN_POINT('Ctrl Pts',(44.8922935078905,55.5200048678648,0.));
#107421=CARTESIAN_POINT('Ctrl Pts',(44.8922935078905,55.5200048678648,12.));
#107422=CARTESIAN_POINT('Ctrl Pts',(44.9002254453192,55.541447362135,0.));
#107423=CARTESIAN_POINT('Ctrl Pts',(44.9002254453192,55.541447362135,12.));
#107424=CARTESIAN_POINT('Ctrl Pts',(44.9081515035525,55.5629400178136,0.));
#107425=CARTESIAN_POINT('Ctrl Pts',(44.9081515035525,55.5629400178136,12.));
#107426=CARTESIAN_POINT('Ctrl Pts',(44.9160715731425,55.5844827324315,0.));
#107427=CARTESIAN_POINT('Ctrl Pts',(44.9160715731425,55.5844827324315,12.));
#107428=CARTESIAN_POINT('Ctrl Pts',(44.9239855452119,55.6060754039089,0.));
#107429=CARTESIAN_POINT('Ctrl Pts',(44.9239855452119,55.6060754039089,12.));
#107430=CARTESIAN_POINT('Ctrl Pts',(44.9318933114483,55.6277179305604,0.));
#107431=CARTESIAN_POINT('Ctrl Pts',(44.9318933114483,55.6277179305604,12.));
#107432=CARTESIAN_POINT('Ctrl Pts',(44.9397947640996,55.6494102110922,0.));
#107433=CARTESIAN_POINT('Ctrl Pts',(44.9397947640996,55.6494102110922,12.));
#107434=CARTESIAN_POINT('Ctrl Pts',(44.9476897959694,55.671152144599,0.));
#107435=CARTESIAN_POINT('Ctrl Pts',(44.9476897959694,55.671152144599,12.));
#107436=CARTESIAN_POINT('Ctrl Pts',(44.9555783004133,55.6929436305522,0.));
#107437=CARTESIAN_POINT('Ctrl Pts',(44.9555783004133,55.6929436305522,12.));
#107438=CARTESIAN_POINT('Ctrl Pts',(44.9634601713352,55.7147845687969,0.));
#107439=CARTESIAN_POINT('Ctrl Pts',(44.9634601713352,55.7147845687969,12.));
#107440=CARTESIAN_POINT('Ctrl Pts',(44.9713353031827,55.7366748595582,0.));
#107441=CARTESIAN_POINT('Ctrl Pts',(44.9713353031827,55.7366748595582,12.));
#107442=CARTESIAN_POINT('Ctrl Pts',(44.979203590942,55.7586144034376,0.));
#107443=CARTESIAN_POINT('Ctrl Pts',(44.979203590942,55.7586144034376,12.));
#107444=CARTESIAN_POINT('Ctrl Pts',(44.9870649301333,55.7806031014093,0.));
#107445=CARTESIAN_POINT('Ctrl Pts',(44.9870649301333,55.7806031014093,12.));
#107446=CARTESIAN_POINT('Ctrl Pts',(44.9949192168073,55.8026408548078,0.));
#107447=CARTESIAN_POINT('Ctrl Pts',(44.9949192168073,55.8026408548078,12.));
#107448=CARTESIAN_POINT('Ctrl Pts',(45.002766347541,55.8247275653257,0.));
#107449=CARTESIAN_POINT('Ctrl Pts',(45.002766347541,55.8247275653257,12.));
#107450=CARTESIAN_POINT('Ctrl Pts',(45.0106062194325,55.8468631350195,0.));
#107451=CARTESIAN_POINT('Ctrl Pts',(45.0106062194325,55.8468631350195,12.));
#107452=CARTESIAN_POINT('Ctrl Pts',(45.0184387300968,55.8690474663058,0.));
#107453=CARTESIAN_POINT('Ctrl Pts',(45.0184387300968,55.8690474663058,12.));
#107454=CARTESIAN_POINT('Ctrl Pts',(45.0262637776623,55.8912804619588,0.));
#107455=CARTESIAN_POINT('Ctrl Pts',(45.0262637776623,55.8912804619588,12.));
#107456=CARTESIAN_POINT('Ctrl Pts',(45.0340812607675,55.9135620250977,0.));
#107457=CARTESIAN_POINT('Ctrl Pts',(45.0340812607675,55.9135620250977,12.));
#107458=CARTESIAN_POINT('Ctrl Pts',(45.041891078557,55.9358920591861,0.));
#107459=CARTESIAN_POINT('Ctrl Pts',(45.041891078557,55.9358920591861,12.));
#107460=CARTESIAN_POINT('Ctrl Pts',(45.0496931306766,55.958270468037,0.));
#107461=CARTESIAN_POINT('Ctrl Pts',(45.0496931306766,55.958270468037,12.));
#107462=CARTESIAN_POINT('Ctrl Pts',(45.0574873172696,55.9806971558099,0.));
#107463=CARTESIAN_POINT('Ctrl Pts',(45.0574873172696,55.9806971558099,12.));
#107464=CARTESIAN_POINT('Ctrl Pts',(45.0652735389728,56.0031720270074,0.));
#107465=CARTESIAN_POINT('Ctrl Pts',(45.0652735389728,56.0031720270074,12.));
#107466=CARTESIAN_POINT('Ctrl Pts',(45.0730516969142,56.025694986463,0.));
#107467=CARTESIAN_POINT('Ctrl Pts',(45.0730516969142,56.025694986463,12.));
#107468=CARTESIAN_POINT('Ctrl Pts',(45.0808216927082,56.0482659393412,0.));
#107469=CARTESIAN_POINT('Ctrl Pts',(45.0808216927082,56.0482659393412,12.));
#107470=CARTESIAN_POINT('Ctrl Pts',(45.0885834284513,56.070884791141,0.));
#107471=CARTESIAN_POINT('Ctrl Pts',(45.0885834284513,56.070884791141,12.));
#107472=CARTESIAN_POINT('Ctrl Pts',(45.0963368067177,56.0935514476946,0.));
#107473=CARTESIAN_POINT('Ctrl Pts',(45.0963368067177,56.0935514476946,12.));
#107474=CARTESIAN_POINT('Ctrl Pts',(45.1040817305563,56.1162658151621,0.));
#107475=CARTESIAN_POINT('Ctrl Pts',(45.1040817305563,56.1162658151621,12.));
#107476=CARTESIAN_POINT('Ctrl Pts',(45.1118181034888,56.1390278000226,0.));
#107477=CARTESIAN_POINT('Ctrl Pts',(45.1118181034888,56.1390278000226,12.));
#107478=CARTESIAN_POINT('Ctrl Pts',(45.119545829506,56.1618373090729,0.));
#107479=CARTESIAN_POINT('Ctrl Pts',(45.119545829506,56.1618373090729,12.));
#107480=CARTESIAN_POINT('Ctrl Pts',(45.1272648130627,56.1846942494321,0.));
#107481=CARTESIAN_POINT('Ctrl Pts',(45.1272648130627,56.1846942494321,12.));
#107482=CARTESIAN_POINT('Ctrl Pts',(45.1349749590736,56.2075985285391,0.));
#107483=CARTESIAN_POINT('Ctrl Pts',(45.1349749590736,56.2075985285391,12.));
#107484=CARTESIAN_POINT('Ctrl Pts',(45.1426761729107,56.2305500541491,0.));
#107485=CARTESIAN_POINT('Ctrl Pts',(45.1426761729107,56.2305500541491,12.));
#107486=CARTESIAN_POINT('Ctrl Pts',(45.150368360401,56.2535487343227,0.));
#107487=CARTESIAN_POINT('Ctrl Pts',(45.150368360401,56.2535487343227,12.));
#107488=CARTESIAN_POINT('Ctrl Pts',(45.158051427823,56.2765944774252,0.));
#107489=CARTESIAN_POINT('Ctrl Pts',(45.158051427823,56.2765944774252,12.));
#107490=CARTESIAN_POINT('Ctrl Pts',(45.1657252819018,56.2996871921321,0.));
#107491=CARTESIAN_POINT('Ctrl Pts',(45.1657252819018,56.2996871921321,12.));
#107492=CARTESIAN_POINT('Ctrl Pts',(45.1733898298062,56.3228267874265,0.));
#107493=CARTESIAN_POINT('Ctrl Pts',(45.1733898298062,56.3228267874265,12.));
#107494=CARTESIAN_POINT('Ctrl Pts',(45.1810449791451,56.3460131725962,0.));
#107495=CARTESIAN_POINT('Ctrl Pts',(45.1810449791451,56.3460131725962,12.));
#107496=CARTESIAN_POINT('Ctrl Pts',(45.1886906379664,56.3692462572228,0.));
#107497=CARTESIAN_POINT('Ctrl Pts',(45.1886906379664,56.3692462572228,12.));
#107498=CARTESIAN_POINT('Ctrl Pts',(45.1963267147527,56.3925259511804,0.));
#107499=CARTESIAN_POINT('Ctrl Pts',(45.1963267147527,56.3925259511804,12.));
#107500=CARTESIAN_POINT('Ctrl Pts',(45.2039531184172,56.4158521646412,0.));
#107501=CARTESIAN_POINT('Ctrl Pts',(45.2039531184172,56.4158521646412,12.));
#107502=CARTESIAN_POINT('Ctrl Pts',(45.2115697583002,56.4392248080733,0.));
#107503=CARTESIAN_POINT('Ctrl Pts',(45.2115697583002,56.4392248080733,12.));
#107504=CARTESIAN_POINT('Ctrl Pts',(45.2191765441666,56.4626437922385,0.));
#107505=CARTESIAN_POINT('Ctrl Pts',(45.2191765441666,56.4626437922385,12.));
#107506=CARTESIAN_POINT('Ctrl Pts',(45.2267733862046,56.4861090281819,0.));
#107507=CARTESIAN_POINT('Ctrl Pts',(45.2267733862046,56.4861090281819,12.));
#107508=CARTESIAN_POINT('Ctrl Pts',(45.2343601950222,56.5096204272299,0.));
#107509=CARTESIAN_POINT('Ctrl Pts',(45.2343601950222,56.5096204272299,12.));
#107510=CARTESIAN_POINT('Ctrl Pts',(45.2419368816423,56.533177900995,0.));
#107511=CARTESIAN_POINT('Ctrl Pts',(45.2419368816423,56.533177900995,12.));
#107512=CARTESIAN_POINT('Ctrl Pts',(45.2495033574997,56.5567813613752,0.));
#107513=CARTESIAN_POINT('Ctrl Pts',(45.2495033574997,56.5567813613752,12.));
#107514=CARTESIAN_POINT('Ctrl Pts',(45.2570595344382,56.5804307205507,0.));
#107515=CARTESIAN_POINT('Ctrl Pts',(45.2570595344382,56.5804307205507,12.));
#107516=CARTESIAN_POINT('Ctrl Pts',(45.2646053247094,56.604125890975,0.));
#107517=CARTESIAN_POINT('Ctrl Pts',(45.2646053247094,56.604125890975,12.));
#107518=CARTESIAN_POINT('Ctrl Pts',(45.2721406409706,56.6278667853716,0.));
#107519=CARTESIAN_POINT('Ctrl Pts',(45.2721406409706,56.6278667853716,12.));
#107520=CARTESIAN_POINT('Ctrl Pts',(45.2796653962795,56.6516533167398,0.));
#107521=CARTESIAN_POINT('Ctrl Pts',(45.2796653962795,56.6516533167398,12.));
#107522=CARTESIAN_POINT('Ctrl Pts',(45.2871795040912,56.6754853983535,0.));
#107523=CARTESIAN_POINT('Ctrl Pts',(45.2871795040912,56.6754853983535,12.));
#107524=CARTESIAN_POINT('Ctrl Pts',(45.2946828782557,56.6993629437597,0.));
#107525=CARTESIAN_POINT('Ctrl Pts',(45.2946828782557,56.6993629437597,12.));
#107526=CARTESIAN_POINT('Ctrl Pts',(45.3021754330169,56.7232858667697,0.));
#107527=CARTESIAN_POINT('Ctrl Pts',(45.3021754330169,56.7232858667697,12.));
#107528=CARTESIAN_POINT('Ctrl Pts',(45.3096570830107,56.747254081454,0.));
#107529=CARTESIAN_POINT('Ctrl Pts',(45.3096570830107,56.747254081454,12.));
#107530=CARTESIAN_POINT('Ctrl Pts',(45.3171277432592,56.771267502148,0.));
#107531=CARTESIAN_POINT('Ctrl Pts',(45.3171277432592,56.771267502148,12.));
#107532=CARTESIAN_POINT('Ctrl Pts',(45.3245873291682,56.7953260434521,0.));
#107533=CARTESIAN_POINT('Ctrl Pts',(45.3245873291682,56.7953260434521,12.));
#107534=CARTESIAN_POINT('Ctrl Pts',(45.3320357565241,56.8194296202293,0.));
#107535=CARTESIAN_POINT('Ctrl Pts',(45.3320357565241,56.8194296202293,12.));
#107536=CARTESIAN_POINT('Ctrl Pts',(45.3394729414932,56.8435781475982,0.));
#107537=CARTESIAN_POINT('Ctrl Pts',(45.3394729414932,56.8435781475982,12.));
#107538=CARTESIAN_POINT('Ctrl Pts',(45.3468988006201,56.8677715409266,0.));
#107539=CARTESIAN_POINT('Ctrl Pts',(45.3468988006201,56.8677715409266,12.));
#107540=CARTESIAN_POINT('Ctrl Pts',(45.3543132508234,56.8920097158371,0.));
#107541=CARTESIAN_POINT('Ctrl Pts',(45.3543132508234,56.8920097158371,12.));
#107542=CARTESIAN_POINT('Ctrl Pts',(45.3617162093918,56.916292588208,0.));
#107543=CARTESIAN_POINT('Ctrl Pts',(45.3617162093918,56.916292588208,12.));
#107544=CARTESIAN_POINT('Ctrl Pts',(45.3691075939827,56.9406200741714,0.));
#107545=CARTESIAN_POINT('Ctrl Pts',(45.3691075939827,56.9406200741714,12.));
#107546=CARTESIAN_POINT('Ctrl Pts',(45.3764873226202,56.9649920901079,0.));
#107547=CARTESIAN_POINT('Ctrl Pts',(45.3764873226202,56.9649920901079,12.));
#107548=CARTESIAN_POINT('Ctrl Pts',(45.3838553136957,56.9894085526383,0.));
#107549=CARTESIAN_POINT('Ctrl Pts',(45.3838553136957,56.9894085526383,12.));
#107550=CARTESIAN_POINT('Ctrl Pts',(45.3912114859624,57.0138693786287,0.));
#107551=CARTESIAN_POINT('Ctrl Pts',(45.3912114859624,57.0138693786287,12.));
#107552=CARTESIAN_POINT('Ctrl Pts',(45.3985557585316,57.0383744851917,0.));
#107553=CARTESIAN_POINT('Ctrl Pts',(45.3985557585316,57.0383744851917,12.));
#107554=CARTESIAN_POINT('Ctrl Pts',(45.4058880508693,57.0629237896848,0.));
#107555=CARTESIAN_POINT('Ctrl Pts',(45.4058880508693,57.0629237896848,12.));
#107556=CARTESIAN_POINT('Ctrl Pts',(45.4132082827945,57.0875172097048,0.));
#107557=CARTESIAN_POINT('Ctrl Pts',(45.4132082827945,57.0875172097048,12.));
#107558=CARTESIAN_POINT('Ctrl Pts',(45.4205163744778,57.1121546630776,0.));
#107559=CARTESIAN_POINT('Ctrl Pts',(45.4205163744778,57.1121546630776,12.));
#107560=CARTESIAN_POINT('Ctrl Pts',(45.4278122464387,57.1368360678629,0.));
#107561=CARTESIAN_POINT('Ctrl Pts',(45.4278122464387,57.1368360678629,12.));
#107562=CARTESIAN_POINT('Ctrl Pts',(45.4350958195434,57.1615613423586,0.));
#107563=CARTESIAN_POINT('Ctrl Pts',(45.4350958195434,57.1615613423586,12.));
#107564=CARTESIAN_POINT('Ctrl Pts',(45.4423670150035,57.1863304051011,0.));
#107565=CARTESIAN_POINT('Ctrl Pts',(45.4423670150035,57.1863304051011,12.));
#107566=CARTESIAN_POINT('Ctrl Pts',(45.4496257543758,57.2111431748629,0.));
#107567=CARTESIAN_POINT('Ctrl Pts',(45.4496257543758,57.2111431748629,12.));
#107568=CARTESIAN_POINT('Ctrl Pts',(45.4568719595639,57.2359995706441,0.));
#107569=CARTESIAN_POINT('Ctrl Pts',(45.4568719595639,57.2359995706441,12.));
#107570=CARTESIAN_POINT('Ctrl Pts',(45.4641055528137,57.2608995116727,0.));
#107571=CARTESIAN_POINT('Ctrl Pts',(45.4641055528137,57.2608995116727,12.));
#107572=CARTESIAN_POINT('Ctrl Pts',(45.4713264567059,57.2858429174056,0.));
#107573=CARTESIAN_POINT('Ctrl Pts',(45.4713264567059,57.2858429174056,12.));
#107574=CARTESIAN_POINT('Ctrl Pts',(45.4785345941505,57.3108297075262,0.));
#107575=CARTESIAN_POINT('Ctrl Pts',(45.4785345941505,57.3108297075262,12.));
#107576=CARTESIAN_POINT('Ctrl Pts',(45.4857298883826,57.3358598019391,0.));
#107577=CARTESIAN_POINT('Ctrl Pts',(45.4857298883826,57.3358598019391,12.));
#107578=CARTESIAN_POINT('Ctrl Pts',(45.4929122629576,57.360933120758,0.));
#107579=CARTESIAN_POINT('Ctrl Pts',(45.4929122629576,57.360933120758,12.));
#107580=CARTESIAN_POINT('Ctrl Pts',(45.5000816417516,57.3860495843043,0.));
#107581=CARTESIAN_POINT('Ctrl Pts',(45.5000816417516,57.3860495843043,12.));
#107582=CARTESIAN_POINT('Ctrl Pts',(45.5072379489637,57.4112091131193,0.));
#107583=CARTESIAN_POINT('Ctrl Pts',(45.5072379489637,57.4112091131193,12.));
#107584=CARTESIAN_POINT('Ctrl Pts',(45.5143811091209,57.4364116279708,0.));
#107585=CARTESIAN_POINT('Ctrl Pts',(45.5143811091209,57.4364116279708,12.));
#107586=CARTESIAN_POINT('Ctrl Pts',(45.5215110470824,57.4616570498566,0.));
#107587=CARTESIAN_POINT('Ctrl Pts',(45.5215110470824,57.4616570498566,12.));
#107588=CARTESIAN_POINT('Ctrl Pts',(45.5286276880479,57.4869453000055,0.));
#107589=CARTESIAN_POINT('Ctrl Pts',(45.5286276880479,57.4869453000055,12.));
#107590=CARTESIAN_POINT('Ctrl Pts',(45.5357309575603,57.5122762998732,0.));
#107591=CARTESIAN_POINT('Ctrl Pts',(45.5357309575603,57.5122762998732,12.));
#107592=CARTESIAN_POINT('Ctrl Pts',(45.5428207814832,57.5376499711338,0.));
#107593=CARTESIAN_POINT('Ctrl Pts',(45.5428207814832,57.5376499711338,12.));
#107594=CARTESIAN_POINT('Ctrl Pts',(45.5498970859829,57.5630662356671,0.));
#107595=CARTESIAN_POINT('Ctrl Pts',(45.5498970859829,57.5630662356671,12.));
#107596=CARTESIAN_POINT('Ctrl Pts',(45.5569597975095,57.5885250155432,0.));
#107597=CARTESIAN_POINT('Ctrl Pts',(45.5569597975095,57.5885250155432,12.));
#107598=CARTESIAN_POINT('Ctrl Pts',(45.5640088427819,57.6140262330048,0.));
#107599=CARTESIAN_POINT('Ctrl Pts',(45.5640088427819,57.6140262330048,12.));
#107600=CARTESIAN_POINT('Ctrl Pts',(45.5710441487683,57.6395698104416,0.));
#107601=CARTESIAN_POINT('Ctrl Pts',(45.5710441487683,57.6395698104416,12.));
#107602=CARTESIAN_POINT('Ctrl Pts',(45.5780656427172,57.6651556704249,0.));
#107603=CARTESIAN_POINT('Ctrl Pts',(45.5780656427172,57.6651556704249,12.));
#107604=CARTESIAN_POINT('Ctrl Pts',(45.5850732521902,57.6907837357426,0.));
#107605=CARTESIAN_POINT('Ctrl Pts',(45.5850732521902,57.6907837357426,12.));
#107606=CARTESIAN_POINT('Ctrl Pts',(45.5920669050987,57.7164539294316,0.));
#107607=CARTESIAN_POINT('Ctrl Pts',(45.5920669050987,57.7164539294316,12.));
#107608=CARTESIAN_POINT('Ctrl Pts',(45.5990465297341,57.7421661748022,0.));
#107609=CARTESIAN_POINT('Ctrl Pts',(45.5990465297341,57.7421661748022,12.));
#107610=CARTESIAN_POINT('Ctrl Pts',(45.6060120548199,57.7679203954735,0.));
#107611=CARTESIAN_POINT('Ctrl Pts',(45.6060120548199,57.7679203954735,12.));
#107612=CARTESIAN_POINT('Ctrl Pts',(45.6129634094677,57.7937165153379,0.));
#107613=CARTESIAN_POINT('Ctrl Pts',(45.6129634094677,57.7937165153379,12.));
#107614=CARTESIAN_POINT('Ctrl Pts',(45.619900523078,57.819554458484,0.));
#107615=CARTESIAN_POINT('Ctrl Pts',(45.619900523078,57.819554458484,12.));
#107616=CARTESIAN_POINT('Ctrl Pts',(45.6268233252543,57.8454341491236,0.));
#107617=CARTESIAN_POINT('Ctrl Pts',(45.6268233252543,57.8454341491236,12.));
#107618=CARTESIAN_POINT('Ctrl Pts',(45.6337317457253,57.8713555115232,0.));
#107619=CARTESIAN_POINT('Ctrl Pts',(45.6337317457253,57.8713555115232,12.));
#107620=CARTESIAN_POINT('Ctrl Pts',(45.6406257142384,57.8973184699038,0.));
#107621=CARTESIAN_POINT('Ctrl Pts',(45.6406257142384,57.8973184699038,12.));
#107622=CARTESIAN_POINT('Ctrl Pts',(45.6475051605542,57.923322948432,0.));
#107623=CARTESIAN_POINT('Ctrl Pts',(45.6475051605542,57.923322948432,12.));
#107624=CARTESIAN_POINT('Ctrl Pts',(45.6543700146688,57.9493688714249,0.));
#107625=CARTESIAN_POINT('Ctrl Pts',(45.6543700146688,57.9493688714249,12.));
#107626=CARTESIAN_POINT('Ctrl Pts',(45.6612202069927,57.975456163507,0.));
#107627=CARTESIAN_POINT('Ctrl Pts',(45.6612202069927,57.975456163507,12.));
#107628=CARTESIAN_POINT('Ctrl Pts',(45.6680556685494,58.0015847497838,0.));
#107629=CARTESIAN_POINT('Ctrl Pts',(45.6680556685494,58.0015847497838,12.));
#107630=CARTESIAN_POINT('Ctrl Pts',(45.6748763311635,58.0277545560001,0.));
#107631=CARTESIAN_POINT('Ctrl Pts',(45.6748763311635,58.0277545560001,12.));
#107632=CARTESIAN_POINT('Ctrl Pts',(45.6816821276662,58.0539655087095,0.));
#107633=CARTESIAN_POINT('Ctrl Pts',(45.6816821276662,58.0539655087095,12.));
#107634=CARTESIAN_POINT('Ctrl Pts',(45.6884729914465,58.0802175348939,0.));
#107635=CARTESIAN_POINT('Ctrl Pts',(45.6884729914465,58.0802175348939,12.));
#107636=CARTESIAN_POINT('Ctrl Pts',(45.6952488560133,58.1065105615884,0.));
#107637=CARTESIAN_POINT('Ctrl Pts',(45.6952488560133,58.1065105615884,12.));
#107638=CARTESIAN_POINT('Ctrl Pts',(45.7020096545174,58.1328445154667,0.));
#107639=CARTESIAN_POINT('Ctrl Pts',(45.7020096545174,58.1328445154667,12.));
#107640=CARTESIAN_POINT('Ctrl Pts',(45.708755319378,58.159219322515,0.));
#107641=CARTESIAN_POINT('Ctrl Pts',(45.708755319378,58.159219322515,12.));
#107642=CARTESIAN_POINT('Ctrl Pts',(45.7154857816507,58.1856349074723,0.));
#107643=CARTESIAN_POINT('Ctrl Pts',(45.7154857816507,58.1856349074723,12.));
#107644=CARTESIAN_POINT('Ctrl Pts',(45.7222009715431,58.2120911942819,0.));
#107645=CARTESIAN_POINT('Ctrl Pts',(45.7222009715431,58.2120911942819,12.));
#107646=CARTESIAN_POINT('Ctrl Pts',(45.7289008195612,58.2385881070959,0.));
#107647=CARTESIAN_POINT('Ctrl Pts',(45.7289008195612,58.2385881070959,12.));
#107648=CARTESIAN_POINT('Ctrl Pts',(45.7355852575127,58.2651255711481,0.));
#107649=CARTESIAN_POINT('Ctrl Pts',(45.7355852575127,58.2651255711481,12.));
#107650=CARTESIAN_POINT('Ctrl Pts',(45.7422542194625,58.2917035135833,0.));
#107651=CARTESIAN_POINT('Ctrl Pts',(45.7422542194625,58.2917035135833,12.));
#107652=CARTESIAN_POINT('Ctrl Pts',(45.7489076429725,58.3183218645265,0.));
#107653=CARTESIAN_POINT('Ctrl Pts',(45.7489076429725,58.3183218645265,12.));
#107654=CARTESIAN_POINT('Ctrl Pts',(45.7555454693956,58.3449805573335,0.));
#107655=CARTESIAN_POINT('Ctrl Pts',(45.7555454693956,58.3449805573335,12.));
#107656=CARTESIAN_POINT('Ctrl Pts',(45.762167641136,58.3716795262252,0.));
#107657=CARTESIAN_POINT('Ctrl Pts',(45.762167641136,58.3716795262252,12.));
#107658=CARTESIAN_POINT('Ctrl Pts',(45.7687740994899,58.3984187044166,0.));
#107659=CARTESIAN_POINT('Ctrl Pts',(45.7687740994899,58.3984187044166,12.));
#107660=CARTESIAN_POINT('Ctrl Pts',(45.77536478215,58.4251980219532,0.));
#107661=CARTESIAN_POINT('Ctrl Pts',(45.77536478215,58.4251980219532,12.));
#107662=CARTESIAN_POINT('Ctrl Pts',(45.7819396211062,58.4520174038836,0.));
#107663=CARTESIAN_POINT('Ctrl Pts',(45.7819396211062,58.4520174038836,12.));
#107664=CARTESIAN_POINT('Ctrl Pts',(45.7884985397138,58.4788767677114,0.));
#107665=CARTESIAN_POINT('Ctrl Pts',(45.7884985397138,58.4788767677114,12.));
#107666=CARTESIAN_POINT('Ctrl Pts',(45.7950414569431,58.5057760270407,0.));
#107667=CARTESIAN_POINT('Ctrl Pts',(45.7950414569431,58.5057760270407,12.));
#107668=CARTESIAN_POINT('Ctrl Pts',(45.801568292618,58.5327150960874,0.));
#107669=CARTESIAN_POINT('Ctrl Pts',(45.801568292618,58.5327150960874,12.));
#107670=CARTESIAN_POINT('Ctrl Pts',(45.8080789725167,58.5596938940308,0.));
#107671=CARTESIAN_POINT('Ctrl Pts',(45.8080789725167,58.5596938940308,12.));
#107672=CARTESIAN_POINT('Ctrl Pts',(45.8145734330666,58.5867123490943,0.));
#107673=CARTESIAN_POINT('Ctrl Pts',(45.8145734330666,58.5867123490943,12.));
#107674=CARTESIAN_POINT('Ctrl Pts',(45.8210516273556,58.6137704035561,0.));
#107675=CARTESIAN_POINT('Ctrl Pts',(45.8210516273556,58.6137704035561,12.));
#107676=CARTESIAN_POINT('Ctrl Pts',(45.8275135263874,58.64086801535,0.));
#107677=CARTESIAN_POINT('Ctrl Pts',(45.8275135263874,58.64086801535,12.));
#107678=CARTESIAN_POINT('Ctrl Pts',(45.8339591141396,58.668005155216,0.));
#107679=CARTESIAN_POINT('Ctrl Pts',(45.8339591141396,58.668005155216,12.));
#107680=CARTESIAN_POINT('Ctrl Pts',(45.8391025301766,58.6897464750196,0.));
#107681=CARTESIAN_POINT('Ctrl Pts',(45.8391025301766,58.6897464750196,12.));
#107682=CARTESIAN_POINT('Ctrl Pts',(45.8429527488565,58.7060702401382,0.));
#107683=CARTESIAN_POINT('Ctrl Pts',(45.8429527488565,58.7060702401382,12.));
#107684=CARTESIAN_POINT('Ctrl Pts',(45.8455162977347,58.7169606500157,0.));
#107685=CARTESIAN_POINT('Ctrl Pts',(45.8455162977347,58.7169606500157,12.));
#107686=CARTESIAN_POINT('Ctrl Pts',(45.8467972562798,58.722407829904,0.));
#107687=CARTESIAN_POINT('Ctrl Pts',(45.8467972562798,58.722407829904,12.));
#107688=CARTESIAN_POINT('',(44.3377168516418,54.1679505278134,0.));
#107689=CARTESIAN_POINT('Ctrl Pts',(44.3377168516418,54.1679505278134,0.));
#107690=CARTESIAN_POINT('Ctrl Pts',(44.3393235891014,54.1714861895278,0.));
#107691=CARTESIAN_POINT('Ctrl Pts',(44.3425373700829,54.1785633257456,0.));
#107692=CARTESIAN_POINT('Ctrl Pts',(44.3473589597467,54.189196468444,0.));
#107693=CARTESIAN_POINT('Ctrl Pts',(44.3537895823819,54.203408870162,0.));
#107694=CARTESIAN_POINT('Ctrl Pts',(44.3618309103245,54.2212325005847,0.));
#107695=CARTESIAN_POINT('Ctrl Pts',(44.3698752533509,54.2391142386354,0.));
#107696=CARTESIAN_POINT('Ctrl Pts',(44.3779225430461,54.2570540336536,0.));
#107697=CARTESIAN_POINT('Ctrl Pts',(44.3859726620288,54.2750517888695,0.));
#107698=CARTESIAN_POINT('Ctrl Pts',(44.3940254456427,54.2931073621661,0.));
#107699=CARTESIAN_POINT('Ctrl Pts',(44.4020807028143,54.3112205860776,0.));
#107700=CARTESIAN_POINT('Ctrl Pts',(44.4101382321834,54.3293912830237,0.));
#107701=CARTESIAN_POINT('Ctrl Pts',(44.4181978395814,54.347619281931,0.));
#107702=CARTESIAN_POINT('Ctrl Pts',(44.4262593564664,54.3659044357064,0.));
#107703=CARTESIAN_POINT('Ctrl Pts',(44.4343226339554,54.3842466156151,0.));
#107704=CARTESIAN_POINT('Ctrl Pts',(44.442387534098,54.4026457030316,0.));
#107705=CARTESIAN_POINT('Ctrl Pts',(44.4504539226336,54.4211015825959,0.));
#107706=CARTESIAN_POINT('Ctrl Pts',(44.4585216599933,54.4396141337008,0.));
#107707=CARTESIAN_POINT('Ctrl Pts',(44.4665905967701,54.4581832262072,0.));
#107708=CARTESIAN_POINT('Ctrl Pts',(44.4746605784056,54.4768087248854,0.));
#107709=CARTESIAN_POINT('Ctrl Pts',(44.482731448127,54.4954904921938,0.));
#107710=CARTESIAN_POINT('Ctrl Pts',(44.4908030503209,54.5142283914684,0.));
#107711=CARTESIAN_POINT('Ctrl Pts',(44.4988752343714,54.5330222905438,0.));
#107712=CARTESIAN_POINT('Ctrl Pts',(44.5069478544945,54.5518720616016,0.));
#107713=CARTESIAN_POINT('Ctrl Pts',(44.5150207678988,54.5707775794412,0.));
#107714=CARTESIAN_POINT('Ctrl Pts',(44.5230938335167,54.5897387202815,0.));
#107715=CARTESIAN_POINT('Ctrl Pts',(44.5311669104514,54.6087553602914,0.));
#107716=CARTESIAN_POINT('Ctrl Pts',(44.5392398566802,54.6278273743587,0.));
#107717=CARTESIAN_POINT('Ctrl Pts',(44.5473125297311,54.6469546367408,0.));
#107718=CARTESIAN_POINT('Ctrl Pts',(44.5553847872721,54.6661370216252,0.));
#107719=CARTESIAN_POINT('Ctrl Pts',(44.5634564876863,54.6853744036751,0.));
#107720=CARTESIAN_POINT('Ctrl Pts',(44.5715274907619,54.7046666586754,0.));
#107721=CARTESIAN_POINT('Ctrl Pts',(44.5795976579454,54.7240136637717,0.));
#107722=CARTESIAN_POINT('Ctrl Pts',(44.5876668519661,54.7434152971267,0.));
#107723=CARTESIAN_POINT('Ctrl Pts',(44.5957349366058,54.7628714377037,0.));
#107724=CARTESIAN_POINT('Ctrl Pts',(44.6038017764309,54.7823819650149,0.));
#107725=CARTESIAN_POINT('Ctrl Pts',(44.6118672364906,54.8019467588278,0.));
#107726=CARTESIAN_POINT('Ctrl Pts',(44.6199311823293,54.8215656991837,0.));
#107727=CARTESIAN_POINT('Ctrl Pts',(44.6279934801168,54.8412386665276,0.));
#107728=CARTESIAN_POINT('Ctrl Pts',(44.6360539967392,54.860965541796,0.));
#107729=CARTESIAN_POINT('Ctrl Pts',(44.6441125999063,54.8807462065164,0.));
#107730=CARTESIAN_POINT('Ctrl Pts',(44.6521691582533,54.9005805428969,0.));
#107731=CARTESIAN_POINT('Ctrl Pts',(44.6602235412836,54.9204684337822,0.));
#107732=CARTESIAN_POINT('Ctrl Pts',(44.6682756193147,54.9404097626077,0.));
#107733=CARTESIAN_POINT('Ctrl Pts',(44.6763252634258,54.9604044133501,0.));
#107734=CARTESIAN_POINT('Ctrl Pts',(44.6843723454,54.9804522704686,0.));
#107735=CARTESIAN_POINT('Ctrl Pts',(44.6924167376869,55.0005532188667,0.));
#107736=CARTESIAN_POINT('Ctrl Pts',(44.7004583134249,55.0207071439237,0.));
#107737=CARTESIAN_POINT('Ctrl Pts',(44.7084969464513,55.0409139315078,0.));
#107738=CARTESIAN_POINT('Ctrl Pts',(44.7165325113159,55.0611734679894,0.));
#107739=CARTESIAN_POINT('Ctrl Pts',(44.7245648832979,55.0814856402496,0.));
#107740=CARTESIAN_POINT('Ctrl Pts',(44.7325939384035,55.1018503356796,0.));
#107741=CARTESIAN_POINT('Ctrl Pts',(44.7406195533479,55.1222674421743,0.));
#107742=CARTESIAN_POINT('Ctrl Pts',(44.7486416055419,55.14273684812,0.));
#107743=CARTESIAN_POINT('Ctrl Pts',(44.7566599730773,55.1632584423815,0.));
#107744=CARTESIAN_POINT('Ctrl Pts',(44.7646745347109,55.1838321142779,0.));
#107745=CARTESIAN_POINT('Ctrl Pts',(44.7726851698618,55.2044577535866,0.));
#107746=CARTESIAN_POINT('Ctrl Pts',(44.7806917586077,55.2251352505475,0.));
#107747=CARTESIAN_POINT('Ctrl Pts',(44.7886941816823,55.2458644958617,0.));
#107748=CARTESIAN_POINT('Ctrl Pts',(44.7966923204741,55.2666453806883,0.));
#107749=CARTESIAN_POINT('Ctrl Pts',(44.8046860570245,55.287477796635,0.));
#107750=CARTESIAN_POINT('Ctrl Pts',(44.812675274021,55.3083616357605,0.));
#107751=CARTESIAN_POINT('Ctrl Pts',(44.8206598547888,55.3292967905726,0.));
#107752=CARTESIAN_POINT('Ctrl Pts',(44.8286396832849,55.350283154023,0.));
#107753=CARTESIAN_POINT('Ctrl Pts',(44.8366146440896,55.3713206194962,0.));
#107754=CARTESIAN_POINT('Ctrl Pts',(44.8445846224033,55.3924090808002,0.));
#107755=CARTESIAN_POINT('Ctrl Pts',(44.8525495040397,55.4135484321706,0.));
#107756=CARTESIAN_POINT('Ctrl Pts',(44.8605091754208,55.4347385682697,0.));
#107757=CARTESIAN_POINT('Ctrl Pts',(44.8684635235727,55.4559793841838,0.));
#107758=CARTESIAN_POINT('Ctrl Pts',(44.8764124361218,55.4772707754139,0.));
#107759=CARTESIAN_POINT('Ctrl Pts',(44.8843558012903,55.4986126378676,0.));
#107760=CARTESIAN_POINT('Ctrl Pts',(44.8922935078905,55.5200048678648,0.));
#107761=CARTESIAN_POINT('Ctrl Pts',(44.9002254453192,55.541447362135,0.));
#107762=CARTESIAN_POINT('Ctrl Pts',(44.9081515035525,55.5629400178136,0.));
#107763=CARTESIAN_POINT('Ctrl Pts',(44.9160715731425,55.5844827324315,0.));
#107764=CARTESIAN_POINT('Ctrl Pts',(44.9239855452119,55.6060754039089,0.));
#107765=CARTESIAN_POINT('Ctrl Pts',(44.9318933114483,55.6277179305604,0.));
#107766=CARTESIAN_POINT('Ctrl Pts',(44.9397947640996,55.6494102110922,0.));
#107767=CARTESIAN_POINT('Ctrl Pts',(44.9476897959694,55.671152144599,0.));
#107768=CARTESIAN_POINT('Ctrl Pts',(44.9555783004133,55.6929436305522,0.));
#107769=CARTESIAN_POINT('Ctrl Pts',(44.9634601713352,55.7147845687969,0.));
#107770=CARTESIAN_POINT('Ctrl Pts',(44.9713353031827,55.7366748595582,0.));
#107771=CARTESIAN_POINT('Ctrl Pts',(44.979203590942,55.7586144034376,0.));
#107772=CARTESIAN_POINT('Ctrl Pts',(44.9870649301333,55.7806031014093,0.));
#107773=CARTESIAN_POINT('Ctrl Pts',(44.9949192168073,55.8026408548078,0.));
#107774=CARTESIAN_POINT('Ctrl Pts',(45.002766347541,55.8247275653257,0.));
#107775=CARTESIAN_POINT('Ctrl Pts',(45.0106062194325,55.8468631350195,0.));
#107776=CARTESIAN_POINT('Ctrl Pts',(45.0184387300968,55.8690474663058,0.));
#107777=CARTESIAN_POINT('Ctrl Pts',(45.0262637776623,55.8912804619588,0.));
#107778=CARTESIAN_POINT('Ctrl Pts',(45.0340812607675,55.9135620250977,0.));
#107779=CARTESIAN_POINT('Ctrl Pts',(45.041891078557,55.9358920591861,0.));
#107780=CARTESIAN_POINT('Ctrl Pts',(45.0496931306766,55.958270468037,0.));
#107781=CARTESIAN_POINT('Ctrl Pts',(45.0574873172696,55.9806971558099,0.));
#107782=CARTESIAN_POINT('Ctrl Pts',(45.0652735389728,56.0031720270074,0.));
#107783=CARTESIAN_POINT('Ctrl Pts',(45.0730516969142,56.025694986463,0.));
#107784=CARTESIAN_POINT('Ctrl Pts',(45.0808216927082,56.0482659393412,0.));
#107785=CARTESIAN_POINT('Ctrl Pts',(45.0885834284513,56.070884791141,0.));
#107786=CARTESIAN_POINT('Ctrl Pts',(45.0963368067177,56.0935514476946,0.));
#107787=CARTESIAN_POINT('Ctrl Pts',(45.1040817305563,56.1162658151621,0.));
#107788=CARTESIAN_POINT('Ctrl Pts',(45.1118181034888,56.1390278000226,0.));
#107789=CARTESIAN_POINT('Ctrl Pts',(45.119545829506,56.1618373090729,0.));
#107790=CARTESIAN_POINT('Ctrl Pts',(45.1272648130627,56.1846942494321,0.));
#107791=CARTESIAN_POINT('Ctrl Pts',(45.1349749590736,56.2075985285391,0.));
#107792=CARTESIAN_POINT('Ctrl Pts',(45.1426761729107,56.2305500541491,0.));
#107793=CARTESIAN_POINT('Ctrl Pts',(45.150368360401,56.2535487343227,0.));
#107794=CARTESIAN_POINT('Ctrl Pts',(45.158051427823,56.2765944774252,0.));
#107795=CARTESIAN_POINT('Ctrl Pts',(45.1657252819018,56.2996871921321,0.));
#107796=CARTESIAN_POINT('Ctrl Pts',(45.1733898298062,56.3228267874265,0.));
#107797=CARTESIAN_POINT('Ctrl Pts',(45.1810449791451,56.3460131725962,0.));
#107798=CARTESIAN_POINT('Ctrl Pts',(45.1886906379664,56.3692462572228,0.));
#107799=CARTESIAN_POINT('Ctrl Pts',(45.1963267147527,56.3925259511804,0.));
#107800=CARTESIAN_POINT('Ctrl Pts',(45.2039531184172,56.4158521646412,0.));
#107801=CARTESIAN_POINT('Ctrl Pts',(45.2115697583002,56.4392248080733,0.));
#107802=CARTESIAN_POINT('Ctrl Pts',(45.2191765441666,56.4626437922385,0.));
#107803=CARTESIAN_POINT('Ctrl Pts',(45.2267733862046,56.4861090281819,0.));
#107804=CARTESIAN_POINT('Ctrl Pts',(45.2343601950222,56.5096204272299,0.));
#107805=CARTESIAN_POINT('Ctrl Pts',(45.2419368816423,56.533177900995,0.));
#107806=CARTESIAN_POINT('Ctrl Pts',(45.2495033574997,56.5567813613752,0.));
#107807=CARTESIAN_POINT('Ctrl Pts',(45.2570595344382,56.5804307205507,0.));
#107808=CARTESIAN_POINT('Ctrl Pts',(45.2646053247094,56.604125890975,0.));
#107809=CARTESIAN_POINT('Ctrl Pts',(45.2721406409706,56.6278667853716,0.));
#107810=CARTESIAN_POINT('Ctrl Pts',(45.2796653962795,56.6516533167398,0.));
#107811=CARTESIAN_POINT('Ctrl Pts',(45.2871795040912,56.6754853983535,0.));
#107812=CARTESIAN_POINT('Ctrl Pts',(45.2946828782557,56.6993629437597,0.));
#107813=CARTESIAN_POINT('Ctrl Pts',(45.3021754330169,56.7232858667697,0.));
#107814=CARTESIAN_POINT('Ctrl Pts',(45.3096570830107,56.747254081454,0.));
#107815=CARTESIAN_POINT('Ctrl Pts',(45.3171277432592,56.771267502148,0.));
#107816=CARTESIAN_POINT('Ctrl Pts',(45.3245873291682,56.7953260434521,0.));
#107817=CARTESIAN_POINT('Ctrl Pts',(45.3320357565241,56.8194296202293,0.));
#107818=CARTESIAN_POINT('Ctrl Pts',(45.3394729414932,56.8435781475982,0.));
#107819=CARTESIAN_POINT('Ctrl Pts',(45.3468988006201,56.8677715409266,0.));
#107820=CARTESIAN_POINT('Ctrl Pts',(45.3543132508234,56.8920097158371,0.));
#107821=CARTESIAN_POINT('Ctrl Pts',(45.3617162093918,56.916292588208,0.));
#107822=CARTESIAN_POINT('Ctrl Pts',(45.3691075939827,56.9406200741714,0.));
#107823=CARTESIAN_POINT('Ctrl Pts',(45.3764873226202,56.9649920901079,0.));
#107824=CARTESIAN_POINT('Ctrl Pts',(45.3838553136957,56.9894085526383,0.));
#107825=CARTESIAN_POINT('Ctrl Pts',(45.3912114859624,57.0138693786287,0.));
#107826=CARTESIAN_POINT('Ctrl Pts',(45.3985557585316,57.0383744851917,0.));
#107827=CARTESIAN_POINT('Ctrl Pts',(45.4058880508693,57.0629237896848,0.));
#107828=CARTESIAN_POINT('Ctrl Pts',(45.4132082827945,57.0875172097048,0.));
#107829=CARTESIAN_POINT('Ctrl Pts',(45.4205163744778,57.1121546630776,0.));
#107830=CARTESIAN_POINT('Ctrl Pts',(45.4278122464387,57.1368360678629,0.));
#107831=CARTESIAN_POINT('Ctrl Pts',(45.4350958195434,57.1615613423586,0.));
#107832=CARTESIAN_POINT('Ctrl Pts',(45.4423670150035,57.1863304051011,0.));
#107833=CARTESIAN_POINT('Ctrl Pts',(45.4496257543758,57.2111431748629,0.));
#107834=CARTESIAN_POINT('Ctrl Pts',(45.4568719595639,57.2359995706441,0.));
#107835=CARTESIAN_POINT('Ctrl Pts',(45.4641055528137,57.2608995116727,0.));
#107836=CARTESIAN_POINT('Ctrl Pts',(45.4713264567059,57.2858429174056,0.));
#107837=CARTESIAN_POINT('Ctrl Pts',(45.4785345941505,57.3108297075262,0.));
#107838=CARTESIAN_POINT('Ctrl Pts',(45.4857298883826,57.3358598019391,0.));
#107839=CARTESIAN_POINT('Ctrl Pts',(45.4929122629576,57.360933120758,0.));
#107840=CARTESIAN_POINT('Ctrl Pts',(45.5000816417516,57.3860495843043,0.));
#107841=CARTESIAN_POINT('Ctrl Pts',(45.5072379489637,57.4112091131193,0.));
#107842=CARTESIAN_POINT('Ctrl Pts',(45.5143811091209,57.4364116279708,0.));
#107843=CARTESIAN_POINT('Ctrl Pts',(45.5215110470824,57.4616570498566,0.));
#107844=CARTESIAN_POINT('Ctrl Pts',(45.5286276880479,57.4869453000055,0.));
#107845=CARTESIAN_POINT('Ctrl Pts',(45.5357309575603,57.5122762998732,0.));
#107846=CARTESIAN_POINT('Ctrl Pts',(45.5428207814832,57.5376499711338,0.));
#107847=CARTESIAN_POINT('Ctrl Pts',(45.5498970859829,57.5630662356671,0.));
#107848=CARTESIAN_POINT('Ctrl Pts',(45.5569597975095,57.5885250155432,0.));
#107849=CARTESIAN_POINT('Ctrl Pts',(45.5640088427819,57.6140262330048,0.));
#107850=CARTESIAN_POINT('Ctrl Pts',(45.5710441487683,57.6395698104416,0.));
#107851=CARTESIAN_POINT('Ctrl Pts',(45.5780656427172,57.6651556704249,0.));
#107852=CARTESIAN_POINT('Ctrl Pts',(45.5850732521902,57.6907837357426,0.));
#107853=CARTESIAN_POINT('Ctrl Pts',(45.5920669050987,57.7164539294316,0.));
#107854=CARTESIAN_POINT('Ctrl Pts',(45.5990465297341,57.7421661748022,0.));
#107855=CARTESIAN_POINT('Ctrl Pts',(45.6060120548199,57.7679203954735,0.));
#107856=CARTESIAN_POINT('Ctrl Pts',(45.6129634094677,57.7937165153379,0.));
#107857=CARTESIAN_POINT('Ctrl Pts',(45.619900523078,57.819554458484,0.));
#107858=CARTESIAN_POINT('Ctrl Pts',(45.6268233252543,57.8454341491236,0.));
#107859=CARTESIAN_POINT('Ctrl Pts',(45.6337317457253,57.8713555115232,0.));
#107860=CARTESIAN_POINT('Ctrl Pts',(45.6406257142384,57.8973184699038,0.));
#107861=CARTESIAN_POINT('Ctrl Pts',(45.6475051605542,57.923322948432,0.));
#107862=CARTESIAN_POINT('Ctrl Pts',(45.6543700146688,57.9493688714249,0.));
#107863=CARTESIAN_POINT('Ctrl Pts',(45.6612202069927,57.975456163507,0.));
#107864=CARTESIAN_POINT('Ctrl Pts',(45.6680556685494,58.0015847497838,0.));
#107865=CARTESIAN_POINT('Ctrl Pts',(45.6748763311635,58.0277545560001,0.));
#107866=CARTESIAN_POINT('Ctrl Pts',(45.6816821276662,58.0539655087095,0.));
#107867=CARTESIAN_POINT('Ctrl Pts',(45.6884729914465,58.0802175348939,0.));
#107868=CARTESIAN_POINT('Ctrl Pts',(45.6952488560133,58.1065105615884,0.));
#107869=CARTESIAN_POINT('Ctrl Pts',(45.7020096545174,58.1328445154667,0.));
#107870=CARTESIAN_POINT('Ctrl Pts',(45.708755319378,58.159219322515,0.));
#107871=CARTESIAN_POINT('Ctrl Pts',(45.7154857816507,58.1856349074723,0.));
#107872=CARTESIAN_POINT('Ctrl Pts',(45.7222009715431,58.2120911942819,0.));
#107873=CARTESIAN_POINT('Ctrl Pts',(45.7289008195612,58.2385881070959,0.));
#107874=CARTESIAN_POINT('Ctrl Pts',(45.7355852575127,58.2651255711481,0.));
#107875=CARTESIAN_POINT('Ctrl Pts',(45.7422542194625,58.2917035135833,0.));
#107876=CARTESIAN_POINT('Ctrl Pts',(45.7489076429725,58.3183218645265,0.));
#107877=CARTESIAN_POINT('Ctrl Pts',(45.7555454693956,58.3449805573335,0.));
#107878=CARTESIAN_POINT('Ctrl Pts',(45.7612219538034,58.3678667473265,0.));
#107879=CARTESIAN_POINT('Ctrl Pts',(45.7655655205267,58.385434851721,0.));
#107880=CARTESIAN_POINT('Ctrl Pts',(45.7685831165459,58.3976670480779,0.));
#107881=CARTESIAN_POINT('Ctrl Pts',(45.7702793558062,58.4045515723007,0.));
#107882=CARTESIAN_POINT('Ctrl Pts',(45.7706564944766,58.4060826907377,0.));
#107883=CARTESIAN_POINT('',(44.3377168516418,54.1679505278134,12.));
#107884=CARTESIAN_POINT('',(44.3377168516418,54.1679505278134,0.));
#107885=CARTESIAN_POINT('Ctrl Pts',(45.7706564944766,58.4060826907378,12.));
#107886=CARTESIAN_POINT('Ctrl Pts',(45.7702793558062,58.4045515723008,12.));
#107887=CARTESIAN_POINT('Ctrl Pts',(45.7685831165459,58.397667048078,12.));
#107888=CARTESIAN_POINT('Ctrl Pts',(45.7655655205267,58.385434851721,12.));
#107889=CARTESIAN_POINT('Ctrl Pts',(45.7612219538034,58.3678667473266,12.));
#107890=CARTESIAN_POINT('Ctrl Pts',(45.7555454693956,58.3449805573335,12.));
#107891=CARTESIAN_POINT('Ctrl Pts',(45.7489076429725,58.3183218645265,12.));
#107892=CARTESIAN_POINT('Ctrl Pts',(45.7422542194625,58.2917035135833,12.));
#107893=CARTESIAN_POINT('Ctrl Pts',(45.7355852575127,58.2651255711481,12.));
#107894=CARTESIAN_POINT('Ctrl Pts',(45.7289008195612,58.2385881070959,12.));
#107895=CARTESIAN_POINT('Ctrl Pts',(45.7222009715431,58.2120911942819,12.));
#107896=CARTESIAN_POINT('Ctrl Pts',(45.7154857816507,58.1856349074723,12.));
#107897=CARTESIAN_POINT('Ctrl Pts',(45.708755319378,58.159219322515,12.));
#107898=CARTESIAN_POINT('Ctrl Pts',(45.7020096545174,58.1328445154667,12.));
#107899=CARTESIAN_POINT('Ctrl Pts',(45.6952488560133,58.1065105615884,12.));
#107900=CARTESIAN_POINT('Ctrl Pts',(45.6884729914465,58.0802175348939,12.));
#107901=CARTESIAN_POINT('Ctrl Pts',(45.6816821276662,58.0539655087095,12.));
#107902=CARTESIAN_POINT('Ctrl Pts',(45.6748763311635,58.0277545560001,12.));
#107903=CARTESIAN_POINT('Ctrl Pts',(45.6680556685494,58.0015847497838,12.));
#107904=CARTESIAN_POINT('Ctrl Pts',(45.6612202069927,57.975456163507,12.));
#107905=CARTESIAN_POINT('Ctrl Pts',(45.6543700146688,57.9493688714249,12.));
#107906=CARTESIAN_POINT('Ctrl Pts',(45.6475051605542,57.923322948432,12.));
#107907=CARTESIAN_POINT('Ctrl Pts',(45.6406257142384,57.8973184699038,12.));
#107908=CARTESIAN_POINT('Ctrl Pts',(45.6337317457253,57.8713555115232,12.));
#107909=CARTESIAN_POINT('Ctrl Pts',(45.6268233252543,57.8454341491236,12.));
#107910=CARTESIAN_POINT('Ctrl Pts',(45.619900523078,57.819554458484,12.));
#107911=CARTESIAN_POINT('Ctrl Pts',(45.6129634094677,57.7937165153379,12.));
#107912=CARTESIAN_POINT('Ctrl Pts',(45.6060120548199,57.7679203954735,12.));
#107913=CARTESIAN_POINT('Ctrl Pts',(45.5990465297341,57.7421661748022,12.));
#107914=CARTESIAN_POINT('Ctrl Pts',(45.5920669050987,57.7164539294316,12.));
#107915=CARTESIAN_POINT('Ctrl Pts',(45.5850732521902,57.6907837357426,12.));
#107916=CARTESIAN_POINT('Ctrl Pts',(45.5780656427172,57.6651556704249,12.));
#107917=CARTESIAN_POINT('Ctrl Pts',(45.5710441487683,57.6395698104416,12.));
#107918=CARTESIAN_POINT('Ctrl Pts',(45.5640088427819,57.6140262330048,12.));
#107919=CARTESIAN_POINT('Ctrl Pts',(45.5569597975095,57.5885250155432,12.));
#107920=CARTESIAN_POINT('Ctrl Pts',(45.5498970859829,57.5630662356671,12.));
#107921=CARTESIAN_POINT('Ctrl Pts',(45.5428207814832,57.5376499711338,12.));
#107922=CARTESIAN_POINT('Ctrl Pts',(45.5357309575603,57.5122762998732,12.));
#107923=CARTESIAN_POINT('Ctrl Pts',(45.5286276880479,57.4869453000055,12.));
#107924=CARTESIAN_POINT('Ctrl Pts',(45.5215110470824,57.4616570498566,12.));
#107925=CARTESIAN_POINT('Ctrl Pts',(45.5143811091209,57.4364116279708,12.));
#107926=CARTESIAN_POINT('Ctrl Pts',(45.5072379489637,57.4112091131193,12.));
#107927=CARTESIAN_POINT('Ctrl Pts',(45.5000816417516,57.3860495843043,12.));
#107928=CARTESIAN_POINT('Ctrl Pts',(45.4929122629576,57.360933120758,12.));
#107929=CARTESIAN_POINT('Ctrl Pts',(45.4857298883826,57.3358598019391,12.));
#107930=CARTESIAN_POINT('Ctrl Pts',(45.4785345941505,57.3108297075262,12.));
#107931=CARTESIAN_POINT('Ctrl Pts',(45.4713264567059,57.2858429174056,12.));
#107932=CARTESIAN_POINT('Ctrl Pts',(45.4641055528137,57.2608995116727,12.));
#107933=CARTESIAN_POINT('Ctrl Pts',(45.4568719595639,57.2359995706441,12.));
#107934=CARTESIAN_POINT('Ctrl Pts',(45.4496257543758,57.2111431748629,12.));
#107935=CARTESIAN_POINT('Ctrl Pts',(45.4423670150035,57.1863304051011,12.));
#107936=CARTESIAN_POINT('Ctrl Pts',(45.4350958195434,57.1615613423586,12.));
#107937=CARTESIAN_POINT('Ctrl Pts',(45.4278122464387,57.1368360678629,12.));
#107938=CARTESIAN_POINT('Ctrl Pts',(45.4205163744778,57.1121546630776,12.));
#107939=CARTESIAN_POINT('Ctrl Pts',(45.4132082827945,57.0875172097048,12.));
#107940=CARTESIAN_POINT('Ctrl Pts',(45.4058880508693,57.0629237896848,12.));
#107941=CARTESIAN_POINT('Ctrl Pts',(45.3985557585316,57.0383744851917,12.));
#107942=CARTESIAN_POINT('Ctrl Pts',(45.3912114859624,57.0138693786287,12.));
#107943=CARTESIAN_POINT('Ctrl Pts',(45.3838553136957,56.9894085526383,12.));
#107944=CARTESIAN_POINT('Ctrl Pts',(45.3764873226202,56.9649920901079,12.));
#107945=CARTESIAN_POINT('Ctrl Pts',(45.3691075939827,56.9406200741714,12.));
#107946=CARTESIAN_POINT('Ctrl Pts',(45.3617162093918,56.916292588208,12.));
#107947=CARTESIAN_POINT('Ctrl Pts',(45.3543132508234,56.8920097158371,12.));
#107948=CARTESIAN_POINT('Ctrl Pts',(45.3468988006201,56.8677715409266,12.));
#107949=CARTESIAN_POINT('Ctrl Pts',(45.3394729414932,56.8435781475982,12.));
#107950=CARTESIAN_POINT('Ctrl Pts',(45.3320357565241,56.8194296202293,12.));
#107951=CARTESIAN_POINT('Ctrl Pts',(45.3245873291682,56.7953260434521,12.));
#107952=CARTESIAN_POINT('Ctrl Pts',(45.3171277432592,56.771267502148,12.));
#107953=CARTESIAN_POINT('Ctrl Pts',(45.3096570830107,56.747254081454,12.));
#107954=CARTESIAN_POINT('Ctrl Pts',(45.3021754330169,56.7232858667697,12.));
#107955=CARTESIAN_POINT('Ctrl Pts',(45.2946828782557,56.6993629437597,12.));
#107956=CARTESIAN_POINT('Ctrl Pts',(45.2871795040912,56.6754853983535,12.));
#107957=CARTESIAN_POINT('Ctrl Pts',(45.2796653962795,56.6516533167398,12.));
#107958=CARTESIAN_POINT('Ctrl Pts',(45.2721406409706,56.6278667853716,12.));
#107959=CARTESIAN_POINT('Ctrl Pts',(45.2646053247094,56.604125890975,12.));
#107960=CARTESIAN_POINT('Ctrl Pts',(45.2570595344382,56.5804307205507,12.));
#107961=CARTESIAN_POINT('Ctrl Pts',(45.2495033574997,56.5567813613752,12.));
#107962=CARTESIAN_POINT('Ctrl Pts',(45.2419368816423,56.533177900995,12.));
#107963=CARTESIAN_POINT('Ctrl Pts',(45.2343601950222,56.5096204272299,12.));
#107964=CARTESIAN_POINT('Ctrl Pts',(45.2267733862046,56.4861090281819,12.));
#107965=CARTESIAN_POINT('Ctrl Pts',(45.2191765441666,56.4626437922385,12.));
#107966=CARTESIAN_POINT('Ctrl Pts',(45.2115697583002,56.4392248080733,12.));
#107967=CARTESIAN_POINT('Ctrl Pts',(45.2039531184172,56.4158521646412,12.));
#107968=CARTESIAN_POINT('Ctrl Pts',(45.1963267147527,56.3925259511804,12.));
#107969=CARTESIAN_POINT('Ctrl Pts',(45.1886906379664,56.3692462572228,12.));
#107970=CARTESIAN_POINT('Ctrl Pts',(45.1810449791451,56.3460131725962,12.));
#107971=CARTESIAN_POINT('Ctrl Pts',(45.1733898298062,56.3228267874265,12.));
#107972=CARTESIAN_POINT('Ctrl Pts',(45.1657252819018,56.2996871921321,12.));
#107973=CARTESIAN_POINT('Ctrl Pts',(45.158051427823,56.2765944774252,12.));
#107974=CARTESIAN_POINT('Ctrl Pts',(45.150368360401,56.2535487343227,12.));
#107975=CARTESIAN_POINT('Ctrl Pts',(45.1426761729107,56.2305500541491,12.));
#107976=CARTESIAN_POINT('Ctrl Pts',(45.1349749590736,56.2075985285391,12.));
#107977=CARTESIAN_POINT('Ctrl Pts',(45.1272648130627,56.1846942494321,12.));
#107978=CARTESIAN_POINT('Ctrl Pts',(45.119545829506,56.1618373090729,12.));
#107979=CARTESIAN_POINT('Ctrl Pts',(45.1118181034888,56.1390278000226,12.));
#107980=CARTESIAN_POINT('Ctrl Pts',(45.1040817305563,56.1162658151621,12.));
#107981=CARTESIAN_POINT('Ctrl Pts',(45.0963368067177,56.0935514476946,12.));
#107982=CARTESIAN_POINT('Ctrl Pts',(45.0885834284513,56.070884791141,12.));
#107983=CARTESIAN_POINT('Ctrl Pts',(45.0808216927082,56.0482659393412,12.));
#107984=CARTESIAN_POINT('Ctrl Pts',(45.0730516969142,56.025694986463,12.));
#107985=CARTESIAN_POINT('Ctrl Pts',(45.0652735389728,56.0031720270074,12.));
#107986=CARTESIAN_POINT('Ctrl Pts',(45.0574873172696,55.9806971558099,12.));
#107987=CARTESIAN_POINT('Ctrl Pts',(45.0496931306766,55.958270468037,12.));
#107988=CARTESIAN_POINT('Ctrl Pts',(45.041891078557,55.9358920591861,12.));
#107989=CARTESIAN_POINT('Ctrl Pts',(45.0340812607675,55.9135620250977,12.));
#107990=CARTESIAN_POINT('Ctrl Pts',(45.0262637776623,55.8912804619588,12.));
#107991=CARTESIAN_POINT('Ctrl Pts',(45.0184387300968,55.8690474663058,12.));
#107992=CARTESIAN_POINT('Ctrl Pts',(45.0106062194325,55.8468631350195,12.));
#107993=CARTESIAN_POINT('Ctrl Pts',(45.002766347541,55.8247275653257,12.));
#107994=CARTESIAN_POINT('Ctrl Pts',(44.9949192168073,55.8026408548078,12.));
#107995=CARTESIAN_POINT('Ctrl Pts',(44.9870649301333,55.7806031014093,12.));
#107996=CARTESIAN_POINT('Ctrl Pts',(44.979203590942,55.7586144034376,12.));
#107997=CARTESIAN_POINT('Ctrl Pts',(44.9713353031827,55.7366748595582,12.));
#107998=CARTESIAN_POINT('Ctrl Pts',(44.9634601713352,55.7147845687969,12.));
#107999=CARTESIAN_POINT('Ctrl Pts',(44.9555783004133,55.6929436305522,12.));
#108000=CARTESIAN_POINT('Ctrl Pts',(44.9476897959694,55.671152144599,12.));
#108001=CARTESIAN_POINT('Ctrl Pts',(44.9397947640996,55.6494102110922,12.));
#108002=CARTESIAN_POINT('Ctrl Pts',(44.9318933114483,55.6277179305604,12.));
#108003=CARTESIAN_POINT('Ctrl Pts',(44.9239855452119,55.6060754039089,12.));
#108004=CARTESIAN_POINT('Ctrl Pts',(44.9160715731425,55.5844827324315,12.));
#108005=CARTESIAN_POINT('Ctrl Pts',(44.9081515035525,55.5629400178136,12.));
#108006=CARTESIAN_POINT('Ctrl Pts',(44.9002254453192,55.541447362135,12.));
#108007=CARTESIAN_POINT('Ctrl Pts',(44.8922935078905,55.5200048678648,12.));
#108008=CARTESIAN_POINT('Ctrl Pts',(44.8843558012903,55.4986126378676,12.));
#108009=CARTESIAN_POINT('Ctrl Pts',(44.8764124361218,55.4772707754139,12.));
#108010=CARTESIAN_POINT('Ctrl Pts',(44.8684635235727,55.4559793841838,12.));
#108011=CARTESIAN_POINT('Ctrl Pts',(44.8605091754208,55.4347385682697,12.));
#108012=CARTESIAN_POINT('Ctrl Pts',(44.8525495040397,55.4135484321706,12.));
#108013=CARTESIAN_POINT('Ctrl Pts',(44.8445846224033,55.3924090808002,12.));
#108014=CARTESIAN_POINT('Ctrl Pts',(44.8366146440896,55.3713206194962,12.));
#108015=CARTESIAN_POINT('Ctrl Pts',(44.8286396832849,55.350283154023,12.));
#108016=CARTESIAN_POINT('Ctrl Pts',(44.8206598547888,55.3292967905726,12.));
#108017=CARTESIAN_POINT('Ctrl Pts',(44.812675274021,55.3083616357605,12.));
#108018=CARTESIAN_POINT('Ctrl Pts',(44.8046860570245,55.287477796635,12.));
#108019=CARTESIAN_POINT('Ctrl Pts',(44.7966923204741,55.2666453806883,12.));
#108020=CARTESIAN_POINT('Ctrl Pts',(44.7886941816823,55.2458644958617,12.));
#108021=CARTESIAN_POINT('Ctrl Pts',(44.7806917586077,55.2251352505475,12.));
#108022=CARTESIAN_POINT('Ctrl Pts',(44.7726851698618,55.2044577535866,12.));
#108023=CARTESIAN_POINT('Ctrl Pts',(44.7646745347109,55.1838321142779,12.));
#108024=CARTESIAN_POINT('Ctrl Pts',(44.7566599730773,55.1632584423815,12.));
#108025=CARTESIAN_POINT('Ctrl Pts',(44.7486416055419,55.14273684812,12.));
#108026=CARTESIAN_POINT('Ctrl Pts',(44.7406195533479,55.1222674421743,12.));
#108027=CARTESIAN_POINT('Ctrl Pts',(44.7325939384035,55.1018503356796,12.));
#108028=CARTESIAN_POINT('Ctrl Pts',(44.7245648832979,55.0814856402496,12.));
#108029=CARTESIAN_POINT('Ctrl Pts',(44.7165325113159,55.0611734679894,12.));
#108030=CARTESIAN_POINT('Ctrl Pts',(44.7084969464513,55.0409139315078,12.));
#108031=CARTESIAN_POINT('Ctrl Pts',(44.7004583134249,55.0207071439237,12.));
#108032=CARTESIAN_POINT('Ctrl Pts',(44.6924167376869,55.0005532188667,12.));
#108033=CARTESIAN_POINT('Ctrl Pts',(44.6843723454,54.9804522704686,12.));
#108034=CARTESIAN_POINT('Ctrl Pts',(44.6763252634258,54.9604044133501,12.));
#108035=CARTESIAN_POINT('Ctrl Pts',(44.6682756193147,54.9404097626077,12.));
#108036=CARTESIAN_POINT('Ctrl Pts',(44.6602235412836,54.9204684337822,12.));
#108037=CARTESIAN_POINT('Ctrl Pts',(44.6521691582533,54.9005805428969,12.));
#108038=CARTESIAN_POINT('Ctrl Pts',(44.6441125999063,54.8807462065164,12.));
#108039=CARTESIAN_POINT('Ctrl Pts',(44.6360539967392,54.860965541796,12.));
#108040=CARTESIAN_POINT('Ctrl Pts',(44.6279934801168,54.8412386665276,12.));
#108041=CARTESIAN_POINT('Ctrl Pts',(44.6199311823293,54.8215656991837,12.));
#108042=CARTESIAN_POINT('Ctrl Pts',(44.6118672364906,54.8019467588278,12.));
#108043=CARTESIAN_POINT('Ctrl Pts',(44.6038017764309,54.7823819650149,12.));
#108044=CARTESIAN_POINT('Ctrl Pts',(44.5957349366058,54.7628714377037,12.));
#108045=CARTESIAN_POINT('Ctrl Pts',(44.5876668519661,54.7434152971267,12.));
#108046=CARTESIAN_POINT('Ctrl Pts',(44.5795976579454,54.7240136637717,12.));
#108047=CARTESIAN_POINT('Ctrl Pts',(44.5715274907619,54.7046666586754,12.));
#108048=CARTESIAN_POINT('Ctrl Pts',(44.5634564876863,54.6853744036751,12.));
#108049=CARTESIAN_POINT('Ctrl Pts',(44.5553847872721,54.6661370216252,12.));
#108050=CARTESIAN_POINT('Ctrl Pts',(44.5473125297311,54.6469546367408,12.));
#108051=CARTESIAN_POINT('Ctrl Pts',(44.5392398566802,54.6278273743587,12.));
#108052=CARTESIAN_POINT('Ctrl Pts',(44.5311669104514,54.6087553602914,12.));
#108053=CARTESIAN_POINT('Ctrl Pts',(44.5230938335167,54.5897387202815,12.));
#108054=CARTESIAN_POINT('Ctrl Pts',(44.5150207678988,54.5707775794412,12.));
#108055=CARTESIAN_POINT('Ctrl Pts',(44.5069478544945,54.5518720616016,12.));
#108056=CARTESIAN_POINT('Ctrl Pts',(44.4988752343714,54.5330222905438,12.));
#108057=CARTESIAN_POINT('Ctrl Pts',(44.4908030503209,54.5142283914684,12.));
#108058=CARTESIAN_POINT('Ctrl Pts',(44.482731448127,54.4954904921938,12.));
#108059=CARTESIAN_POINT('Ctrl Pts',(44.4746605784056,54.4768087248854,12.));
#108060=CARTESIAN_POINT('Ctrl Pts',(44.4665905967701,54.4581832262072,12.));
#108061=CARTESIAN_POINT('Ctrl Pts',(44.4585216599933,54.4396141337008,12.));
#108062=CARTESIAN_POINT('Ctrl Pts',(44.4504539226336,54.4211015825959,12.));
#108063=CARTESIAN_POINT('Ctrl Pts',(44.442387534098,54.4026457030316,12.));
#108064=CARTESIAN_POINT('Ctrl Pts',(44.4343226339554,54.3842466156151,12.));
#108065=CARTESIAN_POINT('Ctrl Pts',(44.4262593564664,54.3659044357064,12.));
#108066=CARTESIAN_POINT('Ctrl Pts',(44.4181978395814,54.347619281931,12.));
#108067=CARTESIAN_POINT('Ctrl Pts',(44.4101382321834,54.3293912830237,12.));
#108068=CARTESIAN_POINT('Ctrl Pts',(44.4020807028143,54.3112205860776,12.));
#108069=CARTESIAN_POINT('Ctrl Pts',(44.3940254456427,54.2931073621661,12.));
#108070=CARTESIAN_POINT('Ctrl Pts',(44.3859726620288,54.2750517888695,12.));
#108071=CARTESIAN_POINT('Ctrl Pts',(44.3779225430461,54.2570540336536,12.));
#108072=CARTESIAN_POINT('Ctrl Pts',(44.3698752533509,54.2391142386354,12.));
#108073=CARTESIAN_POINT('Ctrl Pts',(44.3618309103245,54.2212325005847,12.));
#108074=CARTESIAN_POINT('Ctrl Pts',(44.3537895823819,54.203408870162,12.));
#108075=CARTESIAN_POINT('Ctrl Pts',(44.3473589597467,54.189196468444,12.));
#108076=CARTESIAN_POINT('Ctrl Pts',(44.3425373700829,54.1785633257456,12.));
#108077=CARTESIAN_POINT('Ctrl Pts',(44.3393235891014,54.1714861895278,12.));
#108078=CARTESIAN_POINT('Ctrl Pts',(44.3377168516418,54.1679505278134,12.));
#108079=CARTESIAN_POINT('Ctrl Pts',(44.5696260757798,59.3276657444395,-5.55111512312578E-16));
#108080=CARTESIAN_POINT('Ctrl Pts',(44.5696260757798,59.3276657444395,4.));
#108081=CARTESIAN_POINT('Ctrl Pts',(44.5696260757798,59.3276657444395,8.));
#108082=CARTESIAN_POINT('Ctrl Pts',(44.5696260757798,59.3276657444395,12.));
#108083=CARTESIAN_POINT('Ctrl Pts',(44.6658822400938,59.380664869172,-5.55111512312578E-16));
#108084=CARTESIAN_POINT('Ctrl Pts',(44.6658822400938,59.380664869172,4.));
#108085=CARTESIAN_POINT('Ctrl Pts',(44.6658822400938,59.3806648691719,8.));
#108086=CARTESIAN_POINT('Ctrl Pts',(44.6658822400938,59.3806648691719,12.));
#108087=CARTESIAN_POINT('Ctrl Pts',(44.8655383388343,59.4154499491516,-5.55111512312578E-16));
#108088=CARTESIAN_POINT('Ctrl Pts',(44.8655383388343,59.4154499491516,4.));
#108089=CARTESIAN_POINT('Ctrl Pts',(44.8655383388343,59.4154499491515,8.));
#108090=CARTESIAN_POINT('Ctrl Pts',(44.8655383388343,59.4154499491515,12.));
#108091=CARTESIAN_POINT('Ctrl Pts',(45.0479805952319,59.3374774995079,-5.55111512312578E-16));
#108092=CARTESIAN_POINT('Ctrl Pts',(45.0479805952319,59.3374774995079,4.));
#108093=CARTESIAN_POINT('Ctrl Pts',(45.0479805952318,59.3374774995078,8.));
#108094=CARTESIAN_POINT('Ctrl Pts',(45.0479805952318,59.3374774995078,12.));
#108095=CARTESIAN_POINT('Ctrl Pts',(45.1135644683449,59.2875729049564,-5.55111512312578E-16));
#108096=CARTESIAN_POINT('Ctrl Pts',(45.1135644683449,59.2875729049564,4.));
#108097=CARTESIAN_POINT('Ctrl Pts',(45.1135644683448,59.2875729049563,8.));
#108098=CARTESIAN_POINT('Ctrl Pts',(45.1135644683448,59.2875729049563,12.));
#108099=CARTESIAN_POINT('',(44.5696260757798,59.3276657444395,2.77555756156289E-16));
#108100=CARTESIAN_POINT('',(45.1135644683448,59.2875729049562,0.));
#108101=CARTESIAN_POINT('Ctrl Pts',(44.5696260757798,59.3276657444395,-4.16333634234434E-16));
#108102=CARTESIAN_POINT('Ctrl Pts',(44.6658822400938,59.380664869172,-4.16333634234434E-16));
#108103=CARTESIAN_POINT('Ctrl Pts',(44.7799714393741,59.4005420577317,-4.16333634234434E-16));
#108104=CARTESIAN_POINT('Ctrl Pts',(44.888439792175,59.3836004611084,-4.16333634234434E-16));
#108105=CARTESIAN_POINT('Ctrl Pts',(44.9697910567758,59.3708942636409,-4.16333634234434E-16));
#108106=CARTESIAN_POINT('Ctrl Pts',(45.0479805952319,59.3374774995079,-4.16333634234434E-16));
#108107=CARTESIAN_POINT('Ctrl Pts',(45.1135644683449,59.2875729049564,-4.16333634234434E-16));
#108108=CARTESIAN_POINT('',(45.1135644683447,59.2875729049563,12.));
#108109=CARTESIAN_POINT('Ctrl Pts',(45.1135644683449,59.2875729049564,-5.55111512312578E-16));
#108110=CARTESIAN_POINT('Ctrl Pts',(45.1135644683449,59.2875729049564,4.));
#108111=CARTESIAN_POINT('Ctrl Pts',(45.1135644683448,59.2875729049563,8.));
#108112=CARTESIAN_POINT('Ctrl Pts',(45.1135644683448,59.2875729049563,12.));
#108113=CARTESIAN_POINT('',(44.5696260757798,59.3276657444395,12.));
#108114=CARTESIAN_POINT('Ctrl Pts',(45.1135644683448,59.2875729049563,12.));
#108115=CARTESIAN_POINT('Ctrl Pts',(45.0479805952318,59.3374774995078,12.));
#108116=CARTESIAN_POINT('Ctrl Pts',(44.9697910567757,59.3708942636408,12.));
#108117=CARTESIAN_POINT('Ctrl Pts',(44.888439792175,59.3836004611083,12.));
#108118=CARTESIAN_POINT('Ctrl Pts',(44.7799714393741,59.4005420577317,12.));
#108119=CARTESIAN_POINT('Ctrl Pts',(44.6658822400938,59.3806648691719,12.));
#108120=CARTESIAN_POINT('Ctrl Pts',(44.5696260757798,59.3276657444395,12.));
#108121=CARTESIAN_POINT('Ctrl Pts',(44.5696260757798,59.3276657444395,12.));
#108122=CARTESIAN_POINT('Ctrl Pts',(44.5696260757798,59.3276657444395,8.));
#108123=CARTESIAN_POINT('Ctrl Pts',(44.5696260757798,59.3276657444395,4.));
#108124=CARTESIAN_POINT('Ctrl Pts',(44.5696260757798,59.3276657444395,-5.55111512312578E-16));
#108125=CARTESIAN_POINT('Origin',(2.28111678886296E-10,2.97443977737815E-10,
0.));
#108126=CARTESIAN_POINT('Origin',(2.28111678886296E-10,2.97443977737815E-10,
12.));
#108127=CARTESIAN_POINT('Origin',(2.28111678886296E-10,2.97443977737815E-10,
0.));
#108128=CARTESIAN_POINT('Ctrl Pts',(50.5529731960876,54.7233670476849,0.));
#108129=CARTESIAN_POINT('Ctrl Pts',(50.5529731960876,54.7233670476849,4.));
#108130=CARTESIAN_POINT('Ctrl Pts',(50.5529731960876,54.7233670476849,8.));
#108131=CARTESIAN_POINT('Ctrl Pts',(50.5529731960876,54.7233670476849,12.));
#108132=CARTESIAN_POINT('Ctrl Pts',(50.6336864649947,54.6488048279283,0.));
#108133=CARTESIAN_POINT('Ctrl Pts',(50.6336864649947,54.6488048279283,4.));
#108134=CARTESIAN_POINT('Ctrl Pts',(50.6336864649947,54.6488048279283,8.));
#108135=CARTESIAN_POINT('Ctrl Pts',(50.6336864649947,54.6488048279283,12.));
#108136=CARTESIAN_POINT('Ctrl Pts',(50.7298112257545,54.4703879751555,0.));
#108137=CARTESIAN_POINT('Ctrl Pts',(50.7298112257545,54.4703879751555,4.00000000000001));
#108138=CARTESIAN_POINT('Ctrl Pts',(50.7298112257545,54.4703879751555,8.));
#108139=CARTESIAN_POINT('Ctrl Pts',(50.7298112257545,54.4703879751555,12.));
#108140=CARTESIAN_POINT('Ctrl Pts',(50.7135202769403,54.2726521137411,0.));
#108141=CARTESIAN_POINT('Ctrl Pts',(50.7135202769403,54.2726521137411,4.));
#108142=CARTESIAN_POINT('Ctrl Pts',(50.7135202769403,54.2726521137411,8.));
#108143=CARTESIAN_POINT('Ctrl Pts',(50.7135202769403,54.2726521137411,12.));
#108144=CARTESIAN_POINT('Ctrl Pts',(50.6869108458687,54.1946543499979,0.));
#108145=CARTESIAN_POINT('Ctrl Pts',(50.6869108458687,54.1946543499979,4.));
#108146=CARTESIAN_POINT('Ctrl Pts',(50.6869108458687,54.1946543499979,8.));
#108147=CARTESIAN_POINT('Ctrl Pts',(50.6869108458687,54.1946543499979,12.));
#108148=CARTESIAN_POINT('',(50.5529731960876,54.7233670476849,0.));
#108149=CARTESIAN_POINT('',(50.6869108458688,54.1946543499978,0.));
#108150=CARTESIAN_POINT('Ctrl Pts',(50.5529731960876,54.7233670476849,1.38777878078145E-16));
#108151=CARTESIAN_POINT('Ctrl Pts',(50.6336864649947,54.6488048279283,1.38777878078144E-16));
#108152=CARTESIAN_POINT('Ctrl Pts',(50.6886148997146,54.5468523406296,1.38777878078145E-16));
#108153=CARTESIAN_POINT('Ctrl Pts',(50.7068361639613,54.4385916056111,1.38777878078145E-16));
#108154=CARTESIAN_POINT('Ctrl Pts',(50.7205021121464,54.3573960543472,1.38777878078145E-16));
#108155=CARTESIAN_POINT('Ctrl Pts',(50.7135202769403,54.2726521137411,1.38777878078144E-16));
#108156=CARTESIAN_POINT('Ctrl Pts',(50.6869108458687,54.1946543499979,1.38777878078145E-16));
#108157=CARTESIAN_POINT('',(50.6869108458688,54.1946543499978,12.));
#108158=CARTESIAN_POINT('Ctrl Pts',(50.6869108458687,54.1946543499979,0.));
#108159=CARTESIAN_POINT('Ctrl Pts',(50.6869108458687,54.1946543499979,4.));
#108160=CARTESIAN_POINT('Ctrl Pts',(50.6869108458687,54.1946543499979,8.));
#108161=CARTESIAN_POINT('Ctrl Pts',(50.6869108458687,54.1946543499979,12.));
#108162=CARTESIAN_POINT('',(50.5529731960876,54.7233670476849,12.));
#108163=CARTESIAN_POINT('Ctrl Pts',(50.6869108458687,54.1946543499979,12.));
#108164=CARTESIAN_POINT('Ctrl Pts',(50.7135202769403,54.2726521137411,12.));
#108165=CARTESIAN_POINT('Ctrl Pts',(50.7205021121464,54.3573960543472,12.));
#108166=CARTESIAN_POINT('Ctrl Pts',(50.7068361639613,54.4385916056111,12.));
#108167=CARTESIAN_POINT('Ctrl Pts',(50.6886148997146,54.5468523406296,12.));
#108168=CARTESIAN_POINT('Ctrl Pts',(50.6336864649947,54.6488048279283,12.));
#108169=CARTESIAN_POINT('Ctrl Pts',(50.5529731960876,54.7233670476849,12.));
#108170=CARTESIAN_POINT('Ctrl Pts',(50.5529731960876,54.7233670476849,12.));
#108171=CARTESIAN_POINT('Ctrl Pts',(50.5529731960876,54.7233670476849,8.));
#108172=CARTESIAN_POINT('Ctrl Pts',(50.5529731960876,54.7233670476849,4.));
#108173=CARTESIAN_POINT('Ctrl Pts',(50.5529731960876,54.7233670476849,0.));
#108174=CARTESIAN_POINT('Ctrl Pts',(48.8900464144686,50.0975384783634,0.));
#108175=CARTESIAN_POINT('Ctrl Pts',(48.8900464144686,50.0975384783634,12.));
#108176=CARTESIAN_POINT('Ctrl Pts',(48.8919551910299,50.1009206494209,0.));
#108177=CARTESIAN_POINT('Ctrl Pts',(48.8919551910299,50.1009206494209,12.));
#108178=CARTESIAN_POINT('Ctrl Pts',(48.8957735556681,50.1076907555303,0.));
#108179=CARTESIAN_POINT('Ctrl Pts',(48.8957735556681,50.1076907555303,12.));
#108180=CARTESIAN_POINT('Ctrl Pts',(48.9015035371772,50.1178632066821,0.));
#108181=CARTESIAN_POINT('Ctrl Pts',(48.9015035371772,50.1178632066821,12.));
#108182=CARTESIAN_POINT('Ctrl Pts',(48.9091483817797,50.1314610602286,0.));
#108183=CARTESIAN_POINT('Ctrl Pts',(48.9091483817797,50.1314610602286,12.));
#108184=CARTESIAN_POINT('Ctrl Pts',(48.9187125417897,50.148516018447,0.));
#108185=CARTESIAN_POINT('Ctrl Pts',(48.9187125417897,50.148516018447,12.));
#108186=CARTESIAN_POINT('Ctrl Pts',(48.9282847698237,50.1656286003943,0.));
#108187=CARTESIAN_POINT('Ctrl Pts',(48.9282847698237,50.1656286003943,12.));
#108188=CARTESIAN_POINT('Ctrl Pts',(48.9378649933116,50.1827987615659,0.));
#108189=CARTESIAN_POINT('Ctrl Pts',(48.9378649933116,50.1827987615659,12.));
#108190=CARTESIAN_POINT('Ctrl Pts',(48.9474530868847,50.2000264157903,0.));
#108191=CARTESIAN_POINT('Ctrl Pts',(48.9474530868847,50.2000264157903,12.));
#108192=CARTESIAN_POINT('Ctrl Pts',(48.9570488741273,50.2173114358423,0.));
#108193=CARTESIAN_POINT('Ctrl Pts',(48.9570488741273,50.2173114358423,12.));
#108194=CARTESIAN_POINT('Ctrl Pts',(48.9666521500969,50.2346536715465,0.));
#108195=CARTESIAN_POINT('Ctrl Pts',(48.9666521500969,50.2346536715465,12.));
#108196=CARTESIAN_POINT('Ctrl Pts',(48.9762626987227,50.252052963548,0.));
#108197=CARTESIAN_POINT('Ctrl Pts',(48.9762626987227,50.252052963548,12.));
#108198=CARTESIAN_POINT('Ctrl Pts',(48.9858803116649,50.2695091583473,0.));
#108199=CARTESIAN_POINT('Ctrl Pts',(48.9858803116649,50.2695091583473,12.));
#108200=CARTESIAN_POINT('Ctrl Pts',(48.9955048082028,50.2870221241003,0.));
#108201=CARTESIAN_POINT('Ctrl Pts',(48.9955048082028,50.2870221241003,12.));
#108202=CARTESIAN_POINT('Ctrl Pts',(49.0051360288002,50.3045917455383,0.));
#108203=CARTESIAN_POINT('Ctrl Pts',(49.0051360288002,50.3045917455383,12.));
#108204=CARTESIAN_POINT('Ctrl Pts',(49.0147738256925,50.3222179165102,0.));
#108205=CARTESIAN_POINT('Ctrl Pts',(49.0147738256925,50.3222179165102,12.));
#108206=CARTESIAN_POINT('Ctrl Pts',(49.0244180550759,50.3399005337967,0.));
#108207=CARTESIAN_POINT('Ctrl Pts',(49.0244180550759,50.3399005337967,12.));
#108208=CARTESIAN_POINT('Ctrl Pts',(49.034068567401,50.3576394894136,0.));
#108209=CARTESIAN_POINT('Ctrl Pts',(49.034068567401,50.3576394894136,12.));
#108210=CARTESIAN_POINT('Ctrl Pts',(49.0437252024868,50.3754346667389,0.));
#108211=CARTESIAN_POINT('Ctrl Pts',(49.0437252024868,50.3754346667389,12.));
#108212=CARTESIAN_POINT('Ctrl Pts',(49.0533877945771,50.393285944528,0.));
#108213=CARTESIAN_POINT('Ctrl Pts',(49.0533877945771,50.393285944528,12.));
#108214=CARTESIAN_POINT('Ctrl Pts',(49.0630561755082,50.4111931994264,0.));
#108215=CARTESIAN_POINT('Ctrl Pts',(49.0630561755082,50.4111931994264,12.));
#108216=CARTESIAN_POINT('Ctrl Pts',(49.0727301783477,50.4291563088528,0.));
#108217=CARTESIAN_POINT('Ctrl Pts',(49.0727301783477,50.4291563088528,12.));
#108218=CARTESIAN_POINT('Ctrl Pts',(49.0824096415339,50.4471751542717,0.));
#108219=CARTESIAN_POINT('Ctrl Pts',(49.0824096415339,50.4471751542717,12.));
#108220=CARTESIAN_POINT('Ctrl Pts',(49.0920944086973,50.465249621057,0.));
#108221=CARTESIAN_POINT('Ctrl Pts',(49.0920944086973,50.465249621057,12.));
#108222=CARTESIAN_POINT('Ctrl Pts',(49.1017843266782,50.4833795969296,0.));
#108223=CARTESIAN_POINT('Ctrl Pts',(49.1017843266782,50.4833795969296,12.));
#108224=CARTESIAN_POINT('Ctrl Pts',(49.1114792441573,50.5015649708742,0.));
#108225=CARTESIAN_POINT('Ctrl Pts',(49.1114792441573,50.5015649708742,12.));
#108226=CARTESIAN_POINT('Ctrl Pts',(49.1211790099817,50.5198056318111,0.));
#108227=CARTESIAN_POINT('Ctrl Pts',(49.1211790099817,50.5198056318111,12.));
#108228=CARTESIAN_POINT('Ctrl Pts',(49.1308834717645,50.5381014674822,0.));
#108229=CARTESIAN_POINT('Ctrl Pts',(49.1308834717645,50.5381014674822,12.));
#108230=CARTESIAN_POINT('Ctrl Pts',(49.1405924766169,50.5564523650406,0.));
#108231=CARTESIAN_POINT('Ctrl Pts',(49.1405924766169,50.5564523650406,12.));
#108232=CARTESIAN_POINT('Ctrl Pts',(49.1503058717831,50.5748582115575,0.));
#108233=CARTESIAN_POINT('Ctrl Pts',(49.1503058717831,50.5748582115575,12.));
#108234=CARTESIAN_POINT('Ctrl Pts',(49.1600235052613,50.593318894516,0.));
#108235=CARTESIAN_POINT('Ctrl Pts',(49.1600235052613,50.593318894516,12.));
#108236=CARTESIAN_POINT('Ctrl Pts',(49.1697452265473,50.6118343023937,0.));
#108237=CARTESIAN_POINT('Ctrl Pts',(49.1697452265473,50.6118343023937,12.));
#108238=CARTESIAN_POINT('Ctrl Pts',(49.1794708869074,50.6304043248796,0.));
#108239=CARTESIAN_POINT('Ctrl Pts',(49.1794708869074,50.6304043248796,12.));
#108240=CARTESIAN_POINT('Ctrl Pts',(49.1892003389743,50.6490288525639,0.));
#108241=CARTESIAN_POINT('Ctrl Pts',(49.1892003389743,50.6490288525639,12.));
#108242=CARTESIAN_POINT('Ctrl Pts',(49.1989334364991,50.6677077767427,0.));
#108243=CARTESIAN_POINT('Ctrl Pts',(49.1989334364991,50.6677077767427,12.));
#108244=CARTESIAN_POINT('Ctrl Pts',(49.2086700340625,50.6864409891905,0.));
#108245=CARTESIAN_POINT('Ctrl Pts',(49.2086700340625,50.6864409891905,12.));
#108246=CARTESIAN_POINT('Ctrl Pts',(49.218409986748,50.7052283818941,0.));
#108247=CARTESIAN_POINT('Ctrl Pts',(49.218409986748,50.7052283818941,12.));
#108248=CARTESIAN_POINT('Ctrl Pts',(49.2281531501569,50.7240698470698,0.));
#108249=CARTESIAN_POINT('Ctrl Pts',(49.2281531501569,50.7240698470698,12.));
#108250=CARTESIAN_POINT('Ctrl Pts',(49.2378993805482,50.7429652772816,0.));
#108251=CARTESIAN_POINT('Ctrl Pts',(49.2378993805482,50.7429652772816,12.));
#108252=CARTESIAN_POINT('Ctrl Pts',(49.2476485349373,50.7619145655207,0.));
#108253=CARTESIAN_POINT('Ctrl Pts',(49.2476485349373,50.7619145655207,12.));
#108254=CARTESIAN_POINT('Ctrl Pts',(49.2574004712122,50.7809176052954,0.));
#108255=CARTESIAN_POINT('Ctrl Pts',(49.2574004712122,50.7809176052954,12.));
#108256=CARTESIAN_POINT('Ctrl Pts',(49.2671550482415,50.7999742907111,0.));
#108257=CARTESIAN_POINT('Ctrl Pts',(49.2671550482415,50.7999742907111,12.));
#108258=CARTESIAN_POINT('Ctrl Pts',(49.2769121258144,50.8190845164319,0.));
#108259=CARTESIAN_POINT('Ctrl Pts',(49.2769121258144,50.8190845164319,12.));
#108260=CARTESIAN_POINT('Ctrl Pts',(49.2866715645828,50.8382481776392,0.));
#108261=CARTESIAN_POINT('Ctrl Pts',(49.2866715645828,50.8382481776392,12.));
#108262=CARTESIAN_POINT('Ctrl Pts',(49.2964332260043,50.8574651699877,0.));
#108263=CARTESIAN_POINT('Ctrl Pts',(49.2964332260043,50.8574651699877,12.));
#108264=CARTESIAN_POINT('Ctrl Pts',(49.3061969722798,50.8767353895509,0.));
#108265=CARTESIAN_POINT('Ctrl Pts',(49.3061969722798,50.8767353895509,12.));
#108266=CARTESIAN_POINT('Ctrl Pts',(49.3159626663129,50.8960587327869,0.));
#108267=CARTESIAN_POINT('Ctrl Pts',(49.3159626663129,50.8960587327869,12.));
#108268=CARTESIAN_POINT('Ctrl Pts',(49.325730171735,50.9154350965681,0.));
#108269=CARTESIAN_POINT('Ctrl Pts',(49.325730171735,50.9154350965681,12.));
#108270=CARTESIAN_POINT('Ctrl Pts',(49.3354993529163,50.9348643781928,0.));
#108271=CARTESIAN_POINT('Ctrl Pts',(49.3354993529163,50.9348643781928,12.));
#108272=CARTESIAN_POINT('Ctrl Pts',(49.3452700749804,50.9543464753974,0.));
#108273=CARTESIAN_POINT('Ctrl Pts',(49.3452700749804,50.9543464753974,12.));
#108274=CARTESIAN_POINT('Ctrl Pts',(49.3550422038221,50.9738812863636,0.));
#108275=CARTESIAN_POINT('Ctrl Pts',(49.3550422038221,50.9738812863636,12.));
#108276=CARTESIAN_POINT('Ctrl Pts',(49.3648156061049,50.9934687097179,0.));
#108277=CARTESIAN_POINT('Ctrl Pts',(49.3648156061049,50.9934687097179,12.));
#108278=CARTESIAN_POINT('Ctrl Pts',(49.3745901492428,51.0131086445268,0.));
#108279=CARTESIAN_POINT('Ctrl Pts',(49.3745901492428,51.0131086445268,12.));
#108280=CARTESIAN_POINT('Ctrl Pts',(49.3843657013851,51.0328009902857,0.));
#108281=CARTESIAN_POINT('Ctrl Pts',(49.3843657013851,51.0328009902857,12.));
#108282=CARTESIAN_POINT('Ctrl Pts',(49.3941421314014,51.0525456469072,0.));
#108283=CARTESIAN_POINT('Ctrl Pts',(49.3941421314014,51.0525456469072,12.));
#108284=CARTESIAN_POINT('Ctrl Pts',(49.4039193088635,51.0723425146987,0.));
#108285=CARTESIAN_POINT('Ctrl Pts',(49.4039193088635,51.0723425146987,12.));
#108286=CARTESIAN_POINT('Ctrl Pts',(49.4136971040428,51.0921914943663,0.));
#108287=CARTESIAN_POINT('Ctrl Pts',(49.4136971040428,51.0921914943663,12.));
#108288=CARTESIAN_POINT('Ctrl Pts',(49.4234753879071,51.1120924870196,0.));
#108289=CARTESIAN_POINT('Ctrl Pts',(49.4234753879071,51.1120924870196,12.));
#108290=CARTESIAN_POINT('Ctrl Pts',(49.4332540321178,51.1320453941702,0.));
#108291=CARTESIAN_POINT('Ctrl Pts',(49.4332540321178,51.1320453941702,12.));
#108292=CARTESIAN_POINT('Ctrl Pts',(49.4430329090288,51.1520501177291,0.));
#108293=CARTESIAN_POINT('Ctrl Pts',(49.4430329090288,51.1520501177291,12.));
#108294=CARTESIAN_POINT('Ctrl Pts',(49.4528118916833,51.1721065599972,0.));
#108295=CARTESIAN_POINT('Ctrl Pts',(49.4528118916833,51.1721065599972,12.));
#108296=CARTESIAN_POINT('Ctrl Pts',(49.4625908538076,51.1922146236686,0.));
#108297=CARTESIAN_POINT('Ctrl Pts',(49.4625908538076,51.1922146236686,12.));
#108298=CARTESIAN_POINT('Ctrl Pts',(49.4723696698022,51.2123742118288,0.));
#108299=CARTESIAN_POINT('Ctrl Pts',(49.4723696698022,51.2123742118288,12.));
#108300=CARTESIAN_POINT('Ctrl Pts',(49.4821482147357,51.2325852279507,0.));
#108301=CARTESIAN_POINT('Ctrl Pts',(49.4821482147357,51.2325852279507,12.));
#108302=CARTESIAN_POINT('Ctrl Pts',(49.4919263643357,51.2528475758841,0.));
#108303=CARTESIAN_POINT('Ctrl Pts',(49.4919263643357,51.2528475758841,12.));
#108304=CARTESIAN_POINT('Ctrl Pts',(49.5017039949841,51.2731611598465,0.));
#108305=CARTESIAN_POINT('Ctrl Pts',(49.5017039949841,51.2731611598465,12.));
#108306=CARTESIAN_POINT('Ctrl Pts',(49.5114809837111,51.2935258844278,0.));
#108307=CARTESIAN_POINT('Ctrl Pts',(49.5114809837111,51.2935258844278,12.));
#108308=CARTESIAN_POINT('Ctrl Pts',(49.5212572081901,51.3139416545903,0.));
#108309=CARTESIAN_POINT('Ctrl Pts',(49.5212572081901,51.3139416545903,12.));
#108310=CARTESIAN_POINT('Ctrl Pts',(49.5310325467334,51.3344083756659,0.));
#108311=CARTESIAN_POINT('Ctrl Pts',(49.5310325467334,51.3344083756659,12.));
#108312=CARTESIAN_POINT('Ctrl Pts',(49.5408068782871,51.354925953347,0.));
#108313=CARTESIAN_POINT('Ctrl Pts',(49.5408068782871,51.354925953347,12.));
#108314=CARTESIAN_POINT('Ctrl Pts',(49.5505800824268,51.3754942936796,0.));
#108315=CARTESIAN_POINT('Ctrl Pts',(49.5505800824268,51.3754942936796,12.));
#108316=CARTESIAN_POINT('Ctrl Pts',(49.5603520393514,51.3961133030688,0.));
#108317=CARTESIAN_POINT('Ctrl Pts',(49.5603520393514,51.3961133030688,12.));
#108318=CARTESIAN_POINT('Ctrl Pts',(49.5701226298779,51.4167828882765,0.));
#108319=CARTESIAN_POINT('Ctrl Pts',(49.5701226298779,51.4167828882765,12.));
#108320=CARTESIAN_POINT('Ctrl Pts',(49.579891735436,51.4375029564191,0.));
#108321=CARTESIAN_POINT('Ctrl Pts',(49.579891735436,51.4375029564191,12.));
#108322=CARTESIAN_POINT('Ctrl Pts',(49.5896592380634,51.4582734149562,0.));
#108323=CARTESIAN_POINT('Ctrl Pts',(49.5896592380634,51.4582734149562,12.));
#108324=CARTESIAN_POINT('Ctrl Pts',(49.5994250204003,51.4790941716859,0.));
#108325=CARTESIAN_POINT('Ctrl Pts',(49.5994250204003,51.4790941716859,12.));
#108326=CARTESIAN_POINT('Ctrl Pts',(49.609188965684,51.4999651347496,0.));
#108327=CARTESIAN_POINT('Ctrl Pts',(49.609188965684,51.4999651347496,12.));
#108328=CARTESIAN_POINT('Ctrl Pts',(49.6189509577441,51.5208862126303,0.));
#108329=CARTESIAN_POINT('Ctrl Pts',(49.6189509577441,51.5208862126303,12.));
#108330=CARTESIAN_POINT('Ctrl Pts',(49.6287108809975,51.5418573141494,0.));
#108331=CARTESIAN_POINT('Ctrl Pts',(49.6287108809975,51.5418573141494,12.));
#108332=CARTESIAN_POINT('Ctrl Pts',(49.6384686204443,51.5628783484556,0.));
#108333=CARTESIAN_POINT('Ctrl Pts',(49.6384686204443,51.5628783484556,12.));
#108334=CARTESIAN_POINT('Ctrl Pts',(49.6482240616627,51.5839492250218,0.));
#108335=CARTESIAN_POINT('Ctrl Pts',(49.6482240616627,51.5839492250218,12.));
#108336=CARTESIAN_POINT('Ctrl Pts',(49.6579770908063,51.6050698536525,0.));
#108337=CARTESIAN_POINT('Ctrl Pts',(49.6579770908063,51.6050698536525,12.));
#108338=CARTESIAN_POINT('Ctrl Pts',(49.6677275945975,51.6262401444799,0.));
#108339=CARTESIAN_POINT('Ctrl Pts',(49.6677275945975,51.6262401444799,12.));
#108340=CARTESIAN_POINT('Ctrl Pts',(49.6774754603235,51.6474600079611,0.));
#108341=CARTESIAN_POINT('Ctrl Pts',(49.6774754603235,51.6474600079611,12.));
#108342=CARTESIAN_POINT('Ctrl Pts',(49.6872205758314,51.6687293548656,0.));
#108343=CARTESIAN_POINT('Ctrl Pts',(49.6872205758314,51.6687293548656,12.));
#108344=CARTESIAN_POINT('Ctrl Pts',(49.6969628295236,51.6900480962744,0.));
#108345=CARTESIAN_POINT('Ctrl Pts',(49.6969628295236,51.6900480962744,12.));
#108346=CARTESIAN_POINT('Ctrl Pts',(49.7067021103534,51.7114161435848,0.));
#108347=CARTESIAN_POINT('Ctrl Pts',(49.7067021103534,51.7114161435848,12.));
#108348=CARTESIAN_POINT('Ctrl Pts',(49.7164383078206,51.7328334085084,0.));
#108349=CARTESIAN_POINT('Ctrl Pts',(49.7164383078206,51.7328334085084,12.));
#108350=CARTESIAN_POINT('Ctrl Pts',(49.7261713119672,51.754299803068,0.));
#108351=CARTESIAN_POINT('Ctrl Pts',(49.7261713119672,51.754299803068,12.));
#108352=CARTESIAN_POINT('Ctrl Pts',(49.7359010133741,51.7758152395857,0.));
#108353=CARTESIAN_POINT('Ctrl Pts',(49.7359010133741,51.7758152395857,12.));
#108354=CARTESIAN_POINT('Ctrl Pts',(49.7456273031555,51.7973796306826,0.));
#108355=CARTESIAN_POINT('Ctrl Pts',(49.7456273031555,51.7973796306826,12.));
#108356=CARTESIAN_POINT('Ctrl Pts',(49.7553500729563,51.8189928892841,0.));
#108357=CARTESIAN_POINT('Ctrl Pts',(49.7553500729563,51.8189928892841,12.));
#108358=CARTESIAN_POINT('Ctrl Pts',(49.7650692149464,51.8406549286177,0.));
#108359=CARTESIAN_POINT('Ctrl Pts',(49.7650692149464,51.8406549286177,12.));
#108360=CARTESIAN_POINT('Ctrl Pts',(49.7747846218177,51.8623656622092,0.));
#108361=CARTESIAN_POINT('Ctrl Pts',(49.7747846218177,51.8623656622092,12.));
#108362=CARTESIAN_POINT('Ctrl Pts',(49.78449618678,51.8841250038716,0.));
#108363=CARTESIAN_POINT('Ctrl Pts',(49.78449618678,51.8841250038716,12.));
#108364=CARTESIAN_POINT('Ctrl Pts',(49.7942038035568,51.9059328677051,0.));
#108365=CARTESIAN_POINT('Ctrl Pts',(49.7942038035568,51.9059328677051,12.));
#108366=CARTESIAN_POINT('Ctrl Pts',(49.8039073663808,51.9277891681014,0.));
#108367=CARTESIAN_POINT('Ctrl Pts',(49.8039073663808,51.9277891681014,12.));
#108368=CARTESIAN_POINT('Ctrl Pts',(49.8136067699896,51.9496938197418,0.));
#108369=CARTESIAN_POINT('Ctrl Pts',(49.8136067699896,51.9496938197418,12.));
#108370=CARTESIAN_POINT('Ctrl Pts',(49.8233019096224,51.9716467375938,0.));
#108371=CARTESIAN_POINT('Ctrl Pts',(49.8233019096224,51.9716467375938,12.));
#108372=CARTESIAN_POINT('Ctrl Pts',(49.8329926810172,51.9936478369008,0.));
#108373=CARTESIAN_POINT('Ctrl Pts',(49.8329926810172,51.9936478369008,12.));
#108374=CARTESIAN_POINT('Ctrl Pts',(49.8426789804068,52.015697033182,0.));
#108375=CARTESIAN_POINT('Ctrl Pts',(49.8426789804068,52.015697033182,12.));
#108376=CARTESIAN_POINT('Ctrl Pts',(49.8523607045146,52.0377942422373,0.));
#108377=CARTESIAN_POINT('Ctrl Pts',(49.8523607045146,52.0377942422373,12.));
#108378=CARTESIAN_POINT('Ctrl Pts',(49.8620377505498,52.059939380145,0.));
#108379=CARTESIAN_POINT('Ctrl Pts',(49.8620377505498,52.059939380145,12.));
#108380=CARTESIAN_POINT('Ctrl Pts',(49.871710016205,52.0821323632588,0.));
#108381=CARTESIAN_POINT('Ctrl Pts',(49.871710016205,52.0821323632588,12.));
#108382=CARTESIAN_POINT('Ctrl Pts',(49.8813773996523,52.1043731081968,0.));
#108383=CARTESIAN_POINT('Ctrl Pts',(49.8813773996523,52.1043731081968,12.));
#108384=CARTESIAN_POINT('Ctrl Pts',(49.8910397995404,52.1266615318414,0.));
#108385=CARTESIAN_POINT('Ctrl Pts',(49.8910397995404,52.1266615318414,12.));
#108386=CARTESIAN_POINT('Ctrl Pts',(49.90069711499,52.1489975513449,0.));
#108387=CARTESIAN_POINT('Ctrl Pts',(49.90069711499,52.1489975513449,12.));
#108388=CARTESIAN_POINT('Ctrl Pts',(49.9103492455904,52.1713810841277,0.));
#108389=CARTESIAN_POINT('Ctrl Pts',(49.9103492455904,52.1713810841277,12.));
#108390=CARTESIAN_POINT('Ctrl Pts',(49.919996091396,52.1938120478752,0.));
#108391=CARTESIAN_POINT('Ctrl Pts',(49.919996091396,52.1938120478752,12.));
#108392=CARTESIAN_POINT('Ctrl Pts',(49.9296375529241,52.2162903605272,0.));
#108393=CARTESIAN_POINT('Ctrl Pts',(49.9296375529241,52.2162903605272,12.));
#108394=CARTESIAN_POINT('Ctrl Pts',(49.9392735311507,52.238815940277,0.));
#108395=CARTESIAN_POINT('Ctrl Pts',(49.9392735311507,52.238815940277,12.));
#108396=CARTESIAN_POINT('Ctrl Pts',(49.9489039275064,52.2613887055773,0.));
#108397=CARTESIAN_POINT('Ctrl Pts',(49.9489039275064,52.2613887055773,12.));
#108398=CARTESIAN_POINT('Ctrl Pts',(49.9585286438734,52.2840085751385,0.));
#108399=CARTESIAN_POINT('Ctrl Pts',(49.9585286438734,52.2840085751385,12.));
#108400=CARTESIAN_POINT('Ctrl Pts',(49.9681475825824,52.3066754679265,0.));
#108401=CARTESIAN_POINT('Ctrl Pts',(49.9681475825824,52.3066754679265,12.));
#108402=CARTESIAN_POINT('Ctrl Pts',(49.9777606464103,52.3293893031524,0.));
#108403=CARTESIAN_POINT('Ctrl Pts',(49.9777606464103,52.3293893031524,12.));
#108404=CARTESIAN_POINT('Ctrl Pts',(49.9873677385769,52.3521500002711,0.));
#108405=CARTESIAN_POINT('Ctrl Pts',(49.9873677385769,52.3521500002711,12.));
#108406=CARTESIAN_POINT('Ctrl Pts',(49.9969687627402,52.3749574789865,0.));
#108407=CARTESIAN_POINT('Ctrl Pts',(49.9969687627402,52.3749574789865,12.));
#108408=CARTESIAN_POINT('Ctrl Pts',(50.0065636229934,52.3978116592505,0.));
#108409=CARTESIAN_POINT('Ctrl Pts',(50.0065636229934,52.3978116592505,12.));
#108410=CARTESIAN_POINT('Ctrl Pts',(50.0161522238619,52.420712461261,0.));
#108411=CARTESIAN_POINT('Ctrl Pts',(50.0161522238619,52.420712461261,12.));
#108412=CARTESIAN_POINT('Ctrl Pts',(50.0257344703008,52.4436598054523,0.));
#108413=CARTESIAN_POINT('Ctrl Pts',(50.0257344703008,52.4436598054523,12.));
#108414=CARTESIAN_POINT('Ctrl Pts',(50.0353102676933,52.4666536124926,0.));
#108415=CARTESIAN_POINT('Ctrl Pts',(50.0353102676933,52.4666536124926,12.));
#108416=CARTESIAN_POINT('Ctrl Pts',(50.0448795218453,52.4896938032896,0.));
#108417=CARTESIAN_POINT('Ctrl Pts',(50.0448795218453,52.4896938032896,12.));
#108418=CARTESIAN_POINT('Ctrl Pts',(50.0544421389824,52.5127802989903,0.));
#108419=CARTESIAN_POINT('Ctrl Pts',(50.0544421389824,52.5127802989903,12.));
#108420=CARTESIAN_POINT('Ctrl Pts',(50.0639980257477,52.5359130209789,0.));
#108421=CARTESIAN_POINT('Ctrl Pts',(50.0639980257477,52.5359130209789,12.));
#108422=CARTESIAN_POINT('Ctrl Pts',(50.0735470891996,52.5590918908691,0.));
#108423=CARTESIAN_POINT('Ctrl Pts',(50.0735470891996,52.5590918908691,12.));
#108424=CARTESIAN_POINT('Ctrl Pts',(50.0830892368095,52.5823168304981,0.));
#108425=CARTESIAN_POINT('Ctrl Pts',(50.0830892368095,52.5823168304981,12.));
#108426=CARTESIAN_POINT('Ctrl Pts',(50.0926243764569,52.6055877619338,0.));
#108427=CARTESIAN_POINT('Ctrl Pts',(50.0926243764569,52.6055877619338,12.));
#108428=CARTESIAN_POINT('Ctrl Pts',(50.1021524164261,52.6289046074743,0.));
#108429=CARTESIAN_POINT('Ctrl Pts',(50.1021524164261,52.6289046074743,12.));
#108430=CARTESIAN_POINT('Ctrl Pts',(50.1116732654041,52.6522672896462,0.));
#108431=CARTESIAN_POINT('Ctrl Pts',(50.1116732654041,52.6522672896462,12.));
#108432=CARTESIAN_POINT('Ctrl Pts',(50.1211868324781,52.6756757311979,0.));
#108433=CARTESIAN_POINT('Ctrl Pts',(50.1211868324781,52.6756757311979,12.));
#108434=CARTESIAN_POINT('Ctrl Pts',(50.1306930271343,52.6991298550928,0.));
#108435=CARTESIAN_POINT('Ctrl Pts',(50.1306930271343,52.6991298550928,12.));
#108436=CARTESIAN_POINT('Ctrl Pts',(50.1401917592532,52.7226295845156,0.));
#108437=CARTESIAN_POINT('Ctrl Pts',(50.1401917592532,52.7226295845156,12.));
#108438=CARTESIAN_POINT('Ctrl Pts',(50.1496829391068,52.7461748428733,0.));
#108439=CARTESIAN_POINT('Ctrl Pts',(50.1496829391068,52.7461748428733,12.));
#108440=CARTESIAN_POINT('Ctrl Pts',(50.1591664773561,52.769765553794,0.));
#108441=CARTESIAN_POINT('Ctrl Pts',(50.1591664773561,52.769765553794,12.));
#108442=CARTESIAN_POINT('Ctrl Pts',(50.1686422850493,52.793401641121,0.));
#108443=CARTESIAN_POINT('Ctrl Pts',(50.1686422850493,52.793401641121,12.));
#108444=CARTESIAN_POINT('Ctrl Pts',(50.1781102736215,52.8170830289052,0.));
#108445=CARTESIAN_POINT('Ctrl Pts',(50.1781102736215,52.8170830289052,12.));
#108446=CARTESIAN_POINT('Ctrl Pts',(50.1875703548893,52.8408096414101,0.));
#108447=CARTESIAN_POINT('Ctrl Pts',(50.1875703548893,52.8408096414101,12.));
#108448=CARTESIAN_POINT('Ctrl Pts',(50.1970224410476,52.8645814031137,0.));
#108449=CARTESIAN_POINT('Ctrl Pts',(50.1970224410476,52.8645814031137,12.));
#108450=CARTESIAN_POINT('Ctrl Pts',(50.2064664446663,52.8883982387068,0.));
#108451=CARTESIAN_POINT('Ctrl Pts',(50.2064664446663,52.8883982387068,12.));
#108452=CARTESIAN_POINT('Ctrl Pts',(50.2159022786876,52.9122600730882,0.));
#108453=CARTESIAN_POINT('Ctrl Pts',(50.2159022786876,52.9122600730882,12.));
#108454=CARTESIAN_POINT('Ctrl Pts',(50.2253298564237,52.9361668313539,0.));
#108455=CARTESIAN_POINT('Ctrl Pts',(50.2253298564237,52.9361668313539,12.));
#108456=CARTESIAN_POINT('Ctrl Pts',(50.2347490915553,52.9601184388027,0.));
#108457=CARTESIAN_POINT('Ctrl Pts',(50.2347490915553,52.9601184388027,12.));
#108458=CARTESIAN_POINT('Ctrl Pts',(50.2441598981286,52.9841148209404,0.));
#108459=CARTESIAN_POINT('Ctrl Pts',(50.2441598981286,52.9841148209404,12.));
#108460=CARTESIAN_POINT('Ctrl Pts',(50.2535621905553,53.0081559034802,0.));
#108461=CARTESIAN_POINT('Ctrl Pts',(50.2535621905553,53.0081559034802,12.));
#108462=CARTESIAN_POINT('Ctrl Pts',(50.262955883611,53.0322416123404,0.));
#108463=CARTESIAN_POINT('Ctrl Pts',(50.262955883611,53.0322416123404,12.));
#108464=CARTESIAN_POINT('Ctrl Pts',(50.272340892437,53.0563718736361,0.));
#108465=CARTESIAN_POINT('Ctrl Pts',(50.272340892437,53.0563718736361,12.));
#108466=CARTESIAN_POINT('Ctrl Pts',(50.2817171325354,53.0805466136791,0.));
#108467=CARTESIAN_POINT('Ctrl Pts',(50.2817171325354,53.0805466136791,12.));
#108468=CARTESIAN_POINT('Ctrl Pts',(50.2910845197615,53.1047657589806,0.));
#108469=CARTESIAN_POINT('Ctrl Pts',(50.2910845197615,53.1047657589806,12.));
#108470=CARTESIAN_POINT('Ctrl Pts',(50.3004429703188,53.1290292362482,0.));
#108471=CARTESIAN_POINT('Ctrl Pts',(50.3004429703188,53.1290292362482,12.));
#108472=CARTESIAN_POINT('Ctrl Pts',(50.3097924007535,53.153336972382,0.));
#108473=CARTESIAN_POINT('Ctrl Pts',(50.3097924007535,53.153336972382,12.));
#108474=CARTESIAN_POINT('Ctrl Pts',(50.3191327279497,53.1776888944622,0.));
#108475=CARTESIAN_POINT('Ctrl Pts',(50.3191327279497,53.1776888944622,12.));
#108476=CARTESIAN_POINT('Ctrl Pts',(50.3284638691285,53.202084929748,0.));
#108477=CARTESIAN_POINT('Ctrl Pts',(50.3284638691285,53.202084929748,12.));
#108478=CARTESIAN_POINT('Ctrl Pts',(50.3377857418522,53.2265250056896,0.));
#108479=CARTESIAN_POINT('Ctrl Pts',(50.3377857418522,53.2265250056896,12.));
#108480=CARTESIAN_POINT('Ctrl Pts',(50.3470982640293,53.2510090499341,0.));
#108481=CARTESIAN_POINT('Ctrl Pts',(50.3470982640293,53.2510090499341,12.));
#108482=CARTESIAN_POINT('Ctrl Pts',(50.3564013539198,53.2755369903291,0.));
#108483=CARTESIAN_POINT('Ctrl Pts',(50.3564013539198,53.2755369903291,12.));
#108484=CARTESIAN_POINT('Ctrl Pts',(50.3656949301423,53.3001087549222,0.));
#108485=CARTESIAN_POINT('Ctrl Pts',(50.3656949301423,53.3001087549222,12.));
#108486=CARTESIAN_POINT('Ctrl Pts',(50.3749789116777,53.3247242719575,0.));
#108487=CARTESIAN_POINT('Ctrl Pts',(50.3749789116777,53.3247242719575,12.));
#108488=CARTESIAN_POINT('Ctrl Pts',(50.384253217845,53.3493834698685,0.));
#108489=CARTESIAN_POINT('Ctrl Pts',(50.384253217845,53.3493834698685,12.));
#108490=CARTESIAN_POINT('Ctrl Pts',(50.393517768283,53.3740862772673,0.));
#108491=CARTESIAN_POINT('Ctrl Pts',(50.393517768283,53.3740862772673,12.));
#108492=CARTESIAN_POINT('Ctrl Pts',(50.4027724829296,53.3988326229308,0.));
#108493=CARTESIAN_POINT('Ctrl Pts',(50.4027724829296,53.3988326229308,12.));
#108494=CARTESIAN_POINT('Ctrl Pts',(50.4120172820054,53.4236224357846,0.));
#108495=CARTESIAN_POINT('Ctrl Pts',(50.4120172820054,53.4236224357846,12.));
#108496=CARTESIAN_POINT('Ctrl Pts',(50.4212520859924,53.4484556448787,0.));
#108497=CARTESIAN_POINT('Ctrl Pts',(50.4212520859924,53.4484556448787,12.));
#108498=CARTESIAN_POINT('Ctrl Pts',(50.4304768156677,53.4733321794199,0.));
#108499=CARTESIAN_POINT('Ctrl Pts',(50.4304768156677,53.4733321794199,12.));
#108500=CARTESIAN_POINT('Ctrl Pts',(50.4396913921389,53.4982519688032,0.));
#108501=CARTESIAN_POINT('Ctrl Pts',(50.4396913921389,53.4982519688032,12.));
#108502=CARTESIAN_POINT('Ctrl Pts',(50.4488957368841,53.5232149426415,0.));
#108503=CARTESIAN_POINT('Ctrl Pts',(50.4488957368841,53.5232149426415,12.));
#108504=CARTESIAN_POINT('Ctrl Pts',(50.4580897717835,53.5482210307864,0.));
#108505=CARTESIAN_POINT('Ctrl Pts',(50.4580897717835,53.5482210307864,12.));
#108506=CARTESIAN_POINT('Ctrl Pts',(50.4672734191749,53.5732701633603,0.));
#108507=CARTESIAN_POINT('Ctrl Pts',(50.4672734191749,53.5732701633603,12.));
#108508=CARTESIAN_POINT('Ctrl Pts',(50.4764466018064,53.5983622707231,0.));
#108509=CARTESIAN_POINT('Ctrl Pts',(50.4764466018064,53.5983622707231,12.));
#108510=CARTESIAN_POINT('Ctrl Pts',(50.4856092427309,53.6234972834055,0.));
#108511=CARTESIAN_POINT('Ctrl Pts',(50.4856092427309,53.6234972834055,12.));
#108512=CARTESIAN_POINT('Ctrl Pts',(50.4947612652147,53.6486751320434,0.));
#108513=CARTESIAN_POINT('Ctrl Pts',(50.4947612652147,53.6486751320434,12.));
#108514=CARTESIAN_POINT('Ctrl Pts',(50.5039025926531,53.6738957473158,0.));
#108515=CARTESIAN_POINT('Ctrl Pts',(50.5039025926531,53.6738957473158,12.));
#108516=CARTESIAN_POINT('Ctrl Pts',(50.5130331484563,53.6991590598551,0.));
#108517=CARTESIAN_POINT('Ctrl Pts',(50.5130331484563,53.6991590598551,12.));
#108518=CARTESIAN_POINT('Ctrl Pts',(50.5221528560427,53.7244650002382,0.));
#108519=CARTESIAN_POINT('Ctrl Pts',(50.5221528560427,53.7244650002382,12.));
#108520=CARTESIAN_POINT('Ctrl Pts',(50.5312616390789,53.7498134991714,0.));
#108521=CARTESIAN_POINT('Ctrl Pts',(50.5312616390789,53.7498134991714,12.));
#108522=CARTESIAN_POINT('Ctrl Pts',(50.5403594216706,53.7752044876313,0.));
#108523=CARTESIAN_POINT('Ctrl Pts',(50.5403594216706,53.7752044876313,12.));
#108524=CARTESIAN_POINT('Ctrl Pts',(50.5494461285762,53.8006378970198,0.));
#108525=CARTESIAN_POINT('Ctrl Pts',(50.5494461285762,53.8006378970198,12.));
#108526=CARTESIAN_POINT('Ctrl Pts',(50.5585216854082,53.8261136593064,0.));
#108527=CARTESIAN_POINT('Ctrl Pts',(50.5585216854082,53.8261136593064,12.));
#108528=CARTESIAN_POINT('Ctrl Pts',(50.567586018852,53.8516317071783,0.));
#108529=CARTESIAN_POINT('Ctrl Pts',(50.567586018852,53.8516317071783,12.));
#108530=CARTESIAN_POINT('Ctrl Pts',(50.5766390561861,53.8771919737007,0.));
#108531=CARTESIAN_POINT('Ctrl Pts',(50.5766390561861,53.8771919737007,12.));
#108532=CARTESIAN_POINT('Ctrl Pts',(50.5856807248133,53.9027943919814,0.));
#108533=CARTESIAN_POINT('Ctrl Pts',(50.5856807248133,53.9027943919814,12.));
#108534=CARTESIAN_POINT('Ctrl Pts',(50.5947109517476,53.9284388947996,0.));
#108535=CARTESIAN_POINT('Ctrl Pts',(50.5947109517476,53.9284388947996,12.));
#108536=CARTESIAN_POINT('Ctrl Pts',(50.603729663215,53.9541254143131,0.));
#108537=CARTESIAN_POINT('Ctrl Pts',(50.603729663215,53.9541254143131,12.));
#108538=CARTESIAN_POINT('Ctrl Pts',(50.6127367839738,53.9798538815561,0.));
#108539=CARTESIAN_POINT('Ctrl Pts',(50.6127367839738,53.9798538815561,12.));
#108540=CARTESIAN_POINT('Ctrl Pts',(50.6217322378686,54.0056242268443,0.));
#108541=CARTESIAN_POINT('Ctrl Pts',(50.6217322378686,54.0056242268443,12.));
#108542=CARTESIAN_POINT('Ctrl Pts',(50.630715949059,54.0314363806751,0.));
#108543=CARTESIAN_POINT('Ctrl Pts',(50.630715949059,54.0314363806751,12.));
#108544=CARTESIAN_POINT('Ctrl Pts',(50.6396878430961,54.0572902745101,0.));
#108545=CARTESIAN_POINT('Ctrl Pts',(50.6396878430961,54.0572902745101,12.));
#108546=CARTESIAN_POINT('Ctrl Pts',(50.6486478479459,54.0831858415182,0.));
#108547=CARTESIAN_POINT('Ctrl Pts',(50.6486478479459,54.0831858415182,12.));
#108548=CARTESIAN_POINT('Ctrl Pts',(50.657595895318,54.1091230175319,0.));
#108549=CARTESIAN_POINT('Ctrl Pts',(50.657595895318,54.1091230175319,12.));
#108550=CARTESIAN_POINT('Ctrl Pts',(50.6665319209798,54.1351017412722,0.));
#108551=CARTESIAN_POINT('Ctrl Pts',(50.6665319209798,54.1351017412722,12.));
#108552=CARTESIAN_POINT('Ctrl Pts',(50.6754558618218,54.1611219522299,0.));
#108553=CARTESIAN_POINT('Ctrl Pts',(50.6754558618218,54.1611219522299,12.));
#108554=CARTESIAN_POINT('Ctrl Pts',(50.6843676535428,54.1871835889908,0.));
#108555=CARTESIAN_POINT('Ctrl Pts',(50.6843676535428,54.1871835889908,12.));
#108556=CARTESIAN_POINT('Ctrl Pts',(50.6932672279758,54.2132865872968,0.));
#108557=CARTESIAN_POINT('Ctrl Pts',(50.6932672279758,54.2132865872968,12.));
#108558=CARTESIAN_POINT('Ctrl Pts',(50.7021545108369,54.2394308784093,0.));
#108559=CARTESIAN_POINT('Ctrl Pts',(50.7021545108369,54.2394308784093,12.));
#108560=CARTESIAN_POINT('Ctrl Pts',(50.7110294185832,54.2656163868258,0.));
#108561=CARTESIAN_POINT('Ctrl Pts',(50.7110294185832,54.2656163868258,12.));
#108562=CARTESIAN_POINT('Ctrl Pts',(50.7198918629632,54.2918430335414,0.));
#108563=CARTESIAN_POINT('Ctrl Pts',(50.7198918629632,54.2918430335414,12.));
#108564=CARTESIAN_POINT('Ctrl Pts',(50.7287417566296,54.3181107400862,0.));
#108565=CARTESIAN_POINT('Ctrl Pts',(50.7287417566296,54.3181107400862,12.));
#108566=CARTESIAN_POINT('Ctrl Pts',(50.7375790185988,54.344419432416,0.));
#108567=CARTESIAN_POINT('Ctrl Pts',(50.7375790185988,54.344419432416,12.));
#108568=CARTESIAN_POINT('Ctrl Pts',(50.7464035792846,54.3707690445679,0.));
#108569=CARTESIAN_POINT('Ctrl Pts',(50.7464035792846,54.3707690445679,12.));
#108570=CARTESIAN_POINT('Ctrl Pts',(50.7552153869224,54.3971595231285,0.));
#108571=CARTESIAN_POINT('Ctrl Pts',(50.7552153869224,54.3971595231285,12.));
#108572=CARTESIAN_POINT('Ctrl Pts',(50.7640144089601,54.4235908287188,0.));
#108573=CARTESIAN_POINT('Ctrl Pts',(50.7640144089601,54.4235908287188,12.));
#108574=CARTESIAN_POINT('Ctrl Pts',(50.772800626886,54.4500629335867,0.));
#108575=CARTESIAN_POINT('Ctrl Pts',(50.772800626886,54.4500629335867,12.));
#108576=CARTESIAN_POINT('Ctrl Pts',(50.7798193515479,54.4712732428597,0.));
#108577=CARTESIAN_POINT('Ctrl Pts',(50.7798193515479,54.4712732428597,12.));
#108578=CARTESIAN_POINT('Ctrl Pts',(50.7850776288567,54.4871993224549,0.));
#108579=CARTESIAN_POINT('Ctrl Pts',(50.7850776288567,54.4871993224549,12.));
#108580=CARTESIAN_POINT('Ctrl Pts',(50.7885805844191,54.4978248630284,0.));
#108581=CARTESIAN_POINT('Ctrl Pts',(50.7885805844191,54.4978248630284,12.));
#108582=CARTESIAN_POINT('Ctrl Pts',(50.7903314215393,54.5031396718592,0.));
#108583=CARTESIAN_POINT('Ctrl Pts',(50.7903314215393,54.5031396718592,12.));
#108584=CARTESIAN_POINT('',(48.8900464144686,50.0975384783634,0.));
#108585=CARTESIAN_POINT('Ctrl Pts',(48.8900464144686,50.0975384783634,0.));
#108586=CARTESIAN_POINT('Ctrl Pts',(48.8919551910299,50.1009206494209,0.));
#108587=CARTESIAN_POINT('Ctrl Pts',(48.8957735556681,50.1076907555303,0.));
#108588=CARTESIAN_POINT('Ctrl Pts',(48.9015035371772,50.1178632066821,0.));
#108589=CARTESIAN_POINT('Ctrl Pts',(48.9091483817797,50.1314610602286,0.));
#108590=CARTESIAN_POINT('Ctrl Pts',(48.9187125417897,50.148516018447,0.));
#108591=CARTESIAN_POINT('Ctrl Pts',(48.9282847698237,50.1656286003943,0.));
#108592=CARTESIAN_POINT('Ctrl Pts',(48.9378649933116,50.1827987615659,0.));
#108593=CARTESIAN_POINT('Ctrl Pts',(48.9474530868847,50.2000264157903,0.));
#108594=CARTESIAN_POINT('Ctrl Pts',(48.9570488741273,50.2173114358423,0.));
#108595=CARTESIAN_POINT('Ctrl Pts',(48.9666521500969,50.2346536715465,0.));
#108596=CARTESIAN_POINT('Ctrl Pts',(48.9762626987227,50.252052963548,0.));
#108597=CARTESIAN_POINT('Ctrl Pts',(48.9858803116649,50.2695091583473,0.));
#108598=CARTESIAN_POINT('Ctrl Pts',(48.9955048082028,50.2870221241003,0.));
#108599=CARTESIAN_POINT('Ctrl Pts',(49.0051360288002,50.3045917455383,0.));
#108600=CARTESIAN_POINT('Ctrl Pts',(49.0147738256925,50.3222179165102,0.));
#108601=CARTESIAN_POINT('Ctrl Pts',(49.0244180550759,50.3399005337967,0.));
#108602=CARTESIAN_POINT('Ctrl Pts',(49.034068567401,50.3576394894136,0.));
#108603=CARTESIAN_POINT('Ctrl Pts',(49.0437252024868,50.3754346667389,0.));
#108604=CARTESIAN_POINT('Ctrl Pts',(49.0533877945771,50.393285944528,0.));
#108605=CARTESIAN_POINT('Ctrl Pts',(49.0630561755082,50.4111931994264,0.));
#108606=CARTESIAN_POINT('Ctrl Pts',(49.0727301783477,50.4291563088528,0.));
#108607=CARTESIAN_POINT('Ctrl Pts',(49.0824096415339,50.4471751542717,0.));
#108608=CARTESIAN_POINT('Ctrl Pts',(49.0920944086973,50.465249621057,0.));
#108609=CARTESIAN_POINT('Ctrl Pts',(49.1017843266782,50.4833795969296,0.));
#108610=CARTESIAN_POINT('Ctrl Pts',(49.1114792441573,50.5015649708742,0.));
#108611=CARTESIAN_POINT('Ctrl Pts',(49.1211790099817,50.5198056318111,0.));
#108612=CARTESIAN_POINT('Ctrl Pts',(49.1308834717645,50.5381014674822,0.));
#108613=CARTESIAN_POINT('Ctrl Pts',(49.1405924766169,50.5564523650406,0.));
#108614=CARTESIAN_POINT('Ctrl Pts',(49.1503058717831,50.5748582115575,0.));
#108615=CARTESIAN_POINT('Ctrl Pts',(49.1600235052613,50.593318894516,0.));
#108616=CARTESIAN_POINT('Ctrl Pts',(49.1697452265473,50.6118343023937,0.));
#108617=CARTESIAN_POINT('Ctrl Pts',(49.1794708869074,50.6304043248796,0.));
#108618=CARTESIAN_POINT('Ctrl Pts',(49.1892003389743,50.6490288525639,0.));
#108619=CARTESIAN_POINT('Ctrl Pts',(49.1989334364991,50.6677077767427,0.));
#108620=CARTESIAN_POINT('Ctrl Pts',(49.2086700340625,50.6864409891905,0.));
#108621=CARTESIAN_POINT('Ctrl Pts',(49.218409986748,50.7052283818941,0.));
#108622=CARTESIAN_POINT('Ctrl Pts',(49.2281531501569,50.7240698470698,0.));
#108623=CARTESIAN_POINT('Ctrl Pts',(49.2378993805482,50.7429652772816,0.));
#108624=CARTESIAN_POINT('Ctrl Pts',(49.2476485349373,50.7619145655207,0.));
#108625=CARTESIAN_POINT('Ctrl Pts',(49.2574004712122,50.7809176052954,0.));
#108626=CARTESIAN_POINT('Ctrl Pts',(49.2671550482415,50.7999742907111,0.));
#108627=CARTESIAN_POINT('Ctrl Pts',(49.2769121258144,50.8190845164319,0.));
#108628=CARTESIAN_POINT('Ctrl Pts',(49.2866715645828,50.8382481776392,0.));
#108629=CARTESIAN_POINT('Ctrl Pts',(49.2964332260043,50.8574651699877,0.));
#108630=CARTESIAN_POINT('Ctrl Pts',(49.3061969722798,50.8767353895509,0.));
#108631=CARTESIAN_POINT('Ctrl Pts',(49.3159626663129,50.8960587327869,0.));
#108632=CARTESIAN_POINT('Ctrl Pts',(49.325730171735,50.9154350965681,0.));
#108633=CARTESIAN_POINT('Ctrl Pts',(49.3354993529163,50.9348643781928,0.));
#108634=CARTESIAN_POINT('Ctrl Pts',(49.3452700749804,50.9543464753974,0.));
#108635=CARTESIAN_POINT('Ctrl Pts',(49.3550422038221,50.9738812863636,0.));
#108636=CARTESIAN_POINT('Ctrl Pts',(49.3648156061049,50.9934687097179,0.));
#108637=CARTESIAN_POINT('Ctrl Pts',(49.3745901492428,51.0131086445268,0.));
#108638=CARTESIAN_POINT('Ctrl Pts',(49.3843657013851,51.0328009902857,0.));
#108639=CARTESIAN_POINT('Ctrl Pts',(49.3941421314014,51.0525456469072,0.));
#108640=CARTESIAN_POINT('Ctrl Pts',(49.4039193088635,51.0723425146987,0.));
#108641=CARTESIAN_POINT('Ctrl Pts',(49.4136971040428,51.0921914943663,0.));
#108642=CARTESIAN_POINT('Ctrl Pts',(49.4234753879071,51.1120924870196,0.));
#108643=CARTESIAN_POINT('Ctrl Pts',(49.4332540321178,51.1320453941702,0.));
#108644=CARTESIAN_POINT('Ctrl Pts',(49.4430329090288,51.1520501177291,0.));
#108645=CARTESIAN_POINT('Ctrl Pts',(49.4528118916833,51.1721065599972,0.));
#108646=CARTESIAN_POINT('Ctrl Pts',(49.4625908538076,51.1922146236686,0.));
#108647=CARTESIAN_POINT('Ctrl Pts',(49.4723696698022,51.2123742118288,0.));
#108648=CARTESIAN_POINT('Ctrl Pts',(49.4821482147357,51.2325852279507,0.));
#108649=CARTESIAN_POINT('Ctrl Pts',(49.4919263643357,51.2528475758841,0.));
#108650=CARTESIAN_POINT('Ctrl Pts',(49.5017039949841,51.2731611598465,0.));
#108651=CARTESIAN_POINT('Ctrl Pts',(49.5114809837111,51.2935258844278,0.));
#108652=CARTESIAN_POINT('Ctrl Pts',(49.5212572081901,51.3139416545903,0.));
#108653=CARTESIAN_POINT('Ctrl Pts',(49.5310325467334,51.3344083756659,0.));
#108654=CARTESIAN_POINT('Ctrl Pts',(49.5408068782871,51.354925953347,0.));
#108655=CARTESIAN_POINT('Ctrl Pts',(49.5505800824268,51.3754942936796,0.));
#108656=CARTESIAN_POINT('Ctrl Pts',(49.5603520393514,51.3961133030688,0.));
#108657=CARTESIAN_POINT('Ctrl Pts',(49.5701226298779,51.4167828882765,0.));
#108658=CARTESIAN_POINT('Ctrl Pts',(49.579891735436,51.4375029564191,0.));
#108659=CARTESIAN_POINT('Ctrl Pts',(49.5896592380634,51.4582734149562,0.));
#108660=CARTESIAN_POINT('Ctrl Pts',(49.5994250204003,51.4790941716859,0.));
#108661=CARTESIAN_POINT('Ctrl Pts',(49.609188965684,51.4999651347496,0.));
#108662=CARTESIAN_POINT('Ctrl Pts',(49.6189509577441,51.5208862126303,0.));
#108663=CARTESIAN_POINT('Ctrl Pts',(49.6287108809975,51.5418573141494,0.));
#108664=CARTESIAN_POINT('Ctrl Pts',(49.6384686204443,51.5628783484556,0.));
#108665=CARTESIAN_POINT('Ctrl Pts',(49.6482240616627,51.5839492250218,0.));
#108666=CARTESIAN_POINT('Ctrl Pts',(49.6579770908063,51.6050698536525,0.));
#108667=CARTESIAN_POINT('Ctrl Pts',(49.6677275945975,51.6262401444799,0.));
#108668=CARTESIAN_POINT('Ctrl Pts',(49.6774754603235,51.6474600079611,0.));
#108669=CARTESIAN_POINT('Ctrl Pts',(49.6872205758314,51.6687293548656,0.));
#108670=CARTESIAN_POINT('Ctrl Pts',(49.6969628295236,51.6900480962744,0.));
#108671=CARTESIAN_POINT('Ctrl Pts',(49.7067021103534,51.7114161435848,0.));
#108672=CARTESIAN_POINT('Ctrl Pts',(49.7164383078206,51.7328334085084,0.));
#108673=CARTESIAN_POINT('Ctrl Pts',(49.7261713119672,51.754299803068,0.));
#108674=CARTESIAN_POINT('Ctrl Pts',(49.7359010133741,51.7758152395857,0.));
#108675=CARTESIAN_POINT('Ctrl Pts',(49.7456273031555,51.7973796306826,0.));
#108676=CARTESIAN_POINT('Ctrl Pts',(49.7553500729563,51.8189928892841,0.));
#108677=CARTESIAN_POINT('Ctrl Pts',(49.7650692149464,51.8406549286177,0.));
#108678=CARTESIAN_POINT('Ctrl Pts',(49.7747846218177,51.8623656622092,0.));
#108679=CARTESIAN_POINT('Ctrl Pts',(49.78449618678,51.8841250038716,0.));
#108680=CARTESIAN_POINT('Ctrl Pts',(49.7942038035568,51.9059328677051,0.));
#108681=CARTESIAN_POINT('Ctrl Pts',(49.8039073663808,51.9277891681014,0.));
#108682=CARTESIAN_POINT('Ctrl Pts',(49.8136067699896,51.9496938197418,0.));
#108683=CARTESIAN_POINT('Ctrl Pts',(49.8233019096224,51.9716467375938,0.));
#108684=CARTESIAN_POINT('Ctrl Pts',(49.8329926810172,51.9936478369008,0.));
#108685=CARTESIAN_POINT('Ctrl Pts',(49.8426789804068,52.015697033182,0.));
#108686=CARTESIAN_POINT('Ctrl Pts',(49.8523607045146,52.0377942422373,0.));
#108687=CARTESIAN_POINT('Ctrl Pts',(49.8620377505498,52.059939380145,0.));
#108688=CARTESIAN_POINT('Ctrl Pts',(49.871710016205,52.0821323632588,0.));
#108689=CARTESIAN_POINT('Ctrl Pts',(49.8813773996523,52.1043731081968,0.));
#108690=CARTESIAN_POINT('Ctrl Pts',(49.8910397995404,52.1266615318414,0.));
#108691=CARTESIAN_POINT('Ctrl Pts',(49.90069711499,52.1489975513449,0.));
#108692=CARTESIAN_POINT('Ctrl Pts',(49.9103492455904,52.1713810841277,0.));
#108693=CARTESIAN_POINT('Ctrl Pts',(49.919996091396,52.1938120478752,0.));
#108694=CARTESIAN_POINT('Ctrl Pts',(49.9296375529241,52.2162903605272,0.));
#108695=CARTESIAN_POINT('Ctrl Pts',(49.9392735311507,52.238815940277,0.));
#108696=CARTESIAN_POINT('Ctrl Pts',(49.9489039275064,52.2613887055773,0.));
#108697=CARTESIAN_POINT('Ctrl Pts',(49.9585286438734,52.2840085751385,0.));
#108698=CARTESIAN_POINT('Ctrl Pts',(49.9681475825824,52.3066754679265,0.));
#108699=CARTESIAN_POINT('Ctrl Pts',(49.9777606464103,52.3293893031524,0.));
#108700=CARTESIAN_POINT('Ctrl Pts',(49.9873677385769,52.3521500002711,0.));
#108701=CARTESIAN_POINT('Ctrl Pts',(49.9969687627402,52.3749574789865,0.));
#108702=CARTESIAN_POINT('Ctrl Pts',(50.0065636229934,52.3978116592505,0.));
#108703=CARTESIAN_POINT('Ctrl Pts',(50.0161522238619,52.420712461261,0.));
#108704=CARTESIAN_POINT('Ctrl Pts',(50.0257344703008,52.4436598054523,0.));
#108705=CARTESIAN_POINT('Ctrl Pts',(50.0353102676933,52.4666536124926,0.));
#108706=CARTESIAN_POINT('Ctrl Pts',(50.0448795218453,52.4896938032896,0.));
#108707=CARTESIAN_POINT('Ctrl Pts',(50.0544421389824,52.5127802989903,0.));
#108708=CARTESIAN_POINT('Ctrl Pts',(50.0639980257477,52.5359130209789,0.));
#108709=CARTESIAN_POINT('Ctrl Pts',(50.0735470891996,52.5590918908691,0.));
#108710=CARTESIAN_POINT('Ctrl Pts',(50.0830892368095,52.5823168304981,0.));
#108711=CARTESIAN_POINT('Ctrl Pts',(50.0926243764569,52.6055877619338,0.));
#108712=CARTESIAN_POINT('Ctrl Pts',(50.1021524164261,52.6289046074743,0.));
#108713=CARTESIAN_POINT('Ctrl Pts',(50.1116732654041,52.6522672896462,0.));
#108714=CARTESIAN_POINT('Ctrl Pts',(50.1211868324781,52.6756757311979,0.));
#108715=CARTESIAN_POINT('Ctrl Pts',(50.1306930271343,52.6991298550928,0.));
#108716=CARTESIAN_POINT('Ctrl Pts',(50.1401917592532,52.7226295845156,0.));
#108717=CARTESIAN_POINT('Ctrl Pts',(50.1496829391068,52.7461748428733,0.));
#108718=CARTESIAN_POINT('Ctrl Pts',(50.1591664773561,52.769765553794,0.));
#108719=CARTESIAN_POINT('Ctrl Pts',(50.1686422850493,52.793401641121,0.));
#108720=CARTESIAN_POINT('Ctrl Pts',(50.1781102736215,52.8170830289052,0.));
#108721=CARTESIAN_POINT('Ctrl Pts',(50.1875703548893,52.8408096414101,0.));
#108722=CARTESIAN_POINT('Ctrl Pts',(50.1970224410476,52.8645814031137,0.));
#108723=CARTESIAN_POINT('Ctrl Pts',(50.2064664446663,52.8883982387068,0.));
#108724=CARTESIAN_POINT('Ctrl Pts',(50.2159022786876,52.9122600730882,0.));
#108725=CARTESIAN_POINT('Ctrl Pts',(50.2253298564237,52.9361668313539,0.));
#108726=CARTESIAN_POINT('Ctrl Pts',(50.2347490915553,52.9601184388027,0.));
#108727=CARTESIAN_POINT('Ctrl Pts',(50.2441598981286,52.9841148209404,0.));
#108728=CARTESIAN_POINT('Ctrl Pts',(50.2535621905553,53.0081559034802,0.));
#108729=CARTESIAN_POINT('Ctrl Pts',(50.262955883611,53.0322416123404,0.));
#108730=CARTESIAN_POINT('Ctrl Pts',(50.272340892437,53.0563718736361,0.));
#108731=CARTESIAN_POINT('Ctrl Pts',(50.2817171325354,53.0805466136791,0.));
#108732=CARTESIAN_POINT('Ctrl Pts',(50.2910845197615,53.1047657589806,0.));
#108733=CARTESIAN_POINT('Ctrl Pts',(50.3004429703188,53.1290292362482,0.));
#108734=CARTESIAN_POINT('Ctrl Pts',(50.3097924007535,53.153336972382,0.));
#108735=CARTESIAN_POINT('Ctrl Pts',(50.3191327279497,53.1776888944622,0.));
#108736=CARTESIAN_POINT('Ctrl Pts',(50.3284638691285,53.202084929748,0.));
#108737=CARTESIAN_POINT('Ctrl Pts',(50.3377857418522,53.2265250056896,0.));
#108738=CARTESIAN_POINT('Ctrl Pts',(50.3470982640293,53.2510090499341,0.));
#108739=CARTESIAN_POINT('Ctrl Pts',(50.3564013539198,53.2755369903291,0.));
#108740=CARTESIAN_POINT('Ctrl Pts',(50.3656949301423,53.3001087549222,0.));
#108741=CARTESIAN_POINT('Ctrl Pts',(50.3749789116777,53.3247242719575,0.));
#108742=CARTESIAN_POINT('Ctrl Pts',(50.384253217845,53.3493834698685,0.));
#108743=CARTESIAN_POINT('Ctrl Pts',(50.393517768283,53.3740862772673,0.));
#108744=CARTESIAN_POINT('Ctrl Pts',(50.4027724829296,53.3988326229308,0.));
#108745=CARTESIAN_POINT('Ctrl Pts',(50.4120172820054,53.4236224357846,0.));
#108746=CARTESIAN_POINT('Ctrl Pts',(50.4212520859924,53.4484556448787,0.));
#108747=CARTESIAN_POINT('Ctrl Pts',(50.4304768156677,53.4733321794199,0.));
#108748=CARTESIAN_POINT('Ctrl Pts',(50.4396913921389,53.4982519688032,0.));
#108749=CARTESIAN_POINT('Ctrl Pts',(50.4488957368841,53.5232149426415,0.));
#108750=CARTESIAN_POINT('Ctrl Pts',(50.4580897717835,53.5482210307864,0.));
#108751=CARTESIAN_POINT('Ctrl Pts',(50.4672734191749,53.5732701633603,0.));
#108752=CARTESIAN_POINT('Ctrl Pts',(50.4764466018064,53.5983622707231,0.));
#108753=CARTESIAN_POINT('Ctrl Pts',(50.4856092427309,53.6234972834055,0.));
#108754=CARTESIAN_POINT('Ctrl Pts',(50.4947612652147,53.6486751320434,0.));
#108755=CARTESIAN_POINT('Ctrl Pts',(50.5039025926531,53.6738957473158,0.));
#108756=CARTESIAN_POINT('Ctrl Pts',(50.5130331484563,53.6991590598551,0.));
#108757=CARTESIAN_POINT('Ctrl Pts',(50.5221528560427,53.7244650002382,0.));
#108758=CARTESIAN_POINT('Ctrl Pts',(50.5312616390789,53.7498134991714,0.));
#108759=CARTESIAN_POINT('Ctrl Pts',(50.5403594216706,53.7752044876313,0.));
#108760=CARTESIAN_POINT('Ctrl Pts',(50.5494461285762,53.8006378970198,0.));
#108761=CARTESIAN_POINT('Ctrl Pts',(50.5585216854082,53.8261136593064,0.));
#108762=CARTESIAN_POINT('Ctrl Pts',(50.567586018852,53.8516317071783,0.));
#108763=CARTESIAN_POINT('Ctrl Pts',(50.5766390561861,53.8771919737007,0.));
#108764=CARTESIAN_POINT('Ctrl Pts',(50.5856807248133,53.9027943919814,0.));
#108765=CARTESIAN_POINT('Ctrl Pts',(50.5947109517476,53.9284388947996,0.));
#108766=CARTESIAN_POINT('Ctrl Pts',(50.603729663215,53.9541254143131,0.));
#108767=CARTESIAN_POINT('Ctrl Pts',(50.6127367839738,53.9798538815561,0.));
#108768=CARTESIAN_POINT('Ctrl Pts',(50.6217322378686,54.0056242268443,0.));
#108769=CARTESIAN_POINT('Ctrl Pts',(50.630715949059,54.0314363806751,0.));
#108770=CARTESIAN_POINT('Ctrl Pts',(50.6396878430961,54.0572902745101,0.));
#108771=CARTESIAN_POINT('Ctrl Pts',(50.6486478479459,54.0831858415182,0.));
#108772=CARTESIAN_POINT('Ctrl Pts',(50.657595895318,54.1091230175319,0.));
#108773=CARTESIAN_POINT('Ctrl Pts',(50.6665319209798,54.1351017412722,0.));
#108774=CARTESIAN_POINT('Ctrl Pts',(50.6741814675382,54.1574061041882,0.));
#108775=CARTESIAN_POINT('Ctrl Pts',(50.6800396668659,54.1745287898577,0.));
#108776=CARTESIAN_POINT('Ctrl Pts',(50.6841118861803,54.1864514381924,0.));
#108777=CARTESIAN_POINT('Ctrl Pts',(50.6864016965603,54.1931619277295,0.));
#108778=CARTESIAN_POINT('Ctrl Pts',(50.6869108458688,54.1946543499978,0.));
#108779=CARTESIAN_POINT('',(48.8900464144686,50.0975384783634,12.));
#108780=CARTESIAN_POINT('',(48.8900464144686,50.0975384783634,0.));
#108781=CARTESIAN_POINT('Ctrl Pts',(50.6869108458688,54.1946543499978,12.));
#108782=CARTESIAN_POINT('Ctrl Pts',(50.6864016965603,54.1931619277295,12.));
#108783=CARTESIAN_POINT('Ctrl Pts',(50.6841118861803,54.1864514381924,12.));
#108784=CARTESIAN_POINT('Ctrl Pts',(50.6800396668659,54.1745287898577,12.));
#108785=CARTESIAN_POINT('Ctrl Pts',(50.6741814675382,54.1574061041882,12.));
#108786=CARTESIAN_POINT('Ctrl Pts',(50.6665319209798,54.1351017412722,12.));
#108787=CARTESIAN_POINT('Ctrl Pts',(50.657595895318,54.1091230175319,12.));
#108788=CARTESIAN_POINT('Ctrl Pts',(50.6486478479459,54.0831858415182,12.));
#108789=CARTESIAN_POINT('Ctrl Pts',(50.6396878430961,54.0572902745101,12.));
#108790=CARTESIAN_POINT('Ctrl Pts',(50.630715949059,54.0314363806751,12.));
#108791=CARTESIAN_POINT('Ctrl Pts',(50.6217322378686,54.0056242268443,12.));
#108792=CARTESIAN_POINT('Ctrl Pts',(50.6127367839738,53.9798538815561,12.));
#108793=CARTESIAN_POINT('Ctrl Pts',(50.603729663215,53.9541254143131,12.));
#108794=CARTESIAN_POINT('Ctrl Pts',(50.5947109517476,53.9284388947996,12.));
#108795=CARTESIAN_POINT('Ctrl Pts',(50.5856807248133,53.9027943919814,12.));
#108796=CARTESIAN_POINT('Ctrl Pts',(50.5766390561861,53.8771919737007,12.));
#108797=CARTESIAN_POINT('Ctrl Pts',(50.567586018852,53.8516317071783,12.));
#108798=CARTESIAN_POINT('Ctrl Pts',(50.5585216854082,53.8261136593064,12.));
#108799=CARTESIAN_POINT('Ctrl Pts',(50.5494461285762,53.8006378970198,12.));
#108800=CARTESIAN_POINT('Ctrl Pts',(50.5403594216706,53.7752044876313,12.));
#108801=CARTESIAN_POINT('Ctrl Pts',(50.5312616390789,53.7498134991714,12.));
#108802=CARTESIAN_POINT('Ctrl Pts',(50.5221528560427,53.7244650002382,12.));
#108803=CARTESIAN_POINT('Ctrl Pts',(50.5130331484563,53.6991590598551,12.));
#108804=CARTESIAN_POINT('Ctrl Pts',(50.5039025926531,53.6738957473158,12.));
#108805=CARTESIAN_POINT('Ctrl Pts',(50.4947612652147,53.6486751320434,12.));
#108806=CARTESIAN_POINT('Ctrl Pts',(50.4856092427309,53.6234972834055,12.));
#108807=CARTESIAN_POINT('Ctrl Pts',(50.4764466018064,53.5983622707231,12.));
#108808=CARTESIAN_POINT('Ctrl Pts',(50.4672734191749,53.5732701633603,12.));
#108809=CARTESIAN_POINT('Ctrl Pts',(50.4580897717835,53.5482210307864,12.));
#108810=CARTESIAN_POINT('Ctrl Pts',(50.4488957368841,53.5232149426415,12.));
#108811=CARTESIAN_POINT('Ctrl Pts',(50.4396913921389,53.4982519688032,12.));
#108812=CARTESIAN_POINT('Ctrl Pts',(50.4304768156677,53.4733321794199,12.));
#108813=CARTESIAN_POINT('Ctrl Pts',(50.4212520859924,53.4484556448787,12.));
#108814=CARTESIAN_POINT('Ctrl Pts',(50.4120172820054,53.4236224357846,12.));
#108815=CARTESIAN_POINT('Ctrl Pts',(50.4027724829296,53.3988326229308,12.));
#108816=CARTESIAN_POINT('Ctrl Pts',(50.393517768283,53.3740862772673,12.));
#108817=CARTESIAN_POINT('Ctrl Pts',(50.384253217845,53.3493834698685,12.));
#108818=CARTESIAN_POINT('Ctrl Pts',(50.3749789116777,53.3247242719575,12.));
#108819=CARTESIAN_POINT('Ctrl Pts',(50.3656949301423,53.3001087549222,12.));
#108820=CARTESIAN_POINT('Ctrl Pts',(50.3564013539198,53.2755369903291,12.));
#108821=CARTESIAN_POINT('Ctrl Pts',(50.3470982640293,53.2510090499341,12.));
#108822=CARTESIAN_POINT('Ctrl Pts',(50.3377857418522,53.2265250056896,12.));
#108823=CARTESIAN_POINT('Ctrl Pts',(50.3284638691285,53.202084929748,12.));
#108824=CARTESIAN_POINT('Ctrl Pts',(50.3191327279497,53.1776888944622,12.));
#108825=CARTESIAN_POINT('Ctrl Pts',(50.3097924007535,53.153336972382,12.));
#108826=CARTESIAN_POINT('Ctrl Pts',(50.3004429703188,53.1290292362482,12.));
#108827=CARTESIAN_POINT('Ctrl Pts',(50.2910845197615,53.1047657589806,12.));
#108828=CARTESIAN_POINT('Ctrl Pts',(50.2817171325354,53.0805466136791,12.));
#108829=CARTESIAN_POINT('Ctrl Pts',(50.272340892437,53.0563718736361,12.));
#108830=CARTESIAN_POINT('Ctrl Pts',(50.262955883611,53.0322416123404,12.));
#108831=CARTESIAN_POINT('Ctrl Pts',(50.2535621905553,53.0081559034802,12.));
#108832=CARTESIAN_POINT('Ctrl Pts',(50.2441598981286,52.9841148209404,12.));
#108833=CARTESIAN_POINT('Ctrl Pts',(50.2347490915553,52.9601184388027,12.));
#108834=CARTESIAN_POINT('Ctrl Pts',(50.2253298564237,52.9361668313539,12.));
#108835=CARTESIAN_POINT('Ctrl Pts',(50.2159022786876,52.9122600730882,12.));
#108836=CARTESIAN_POINT('Ctrl Pts',(50.2064664446663,52.8883982387068,12.));
#108837=CARTESIAN_POINT('Ctrl Pts',(50.1970224410476,52.8645814031137,12.));
#108838=CARTESIAN_POINT('Ctrl Pts',(50.1875703548893,52.8408096414101,12.));
#108839=CARTESIAN_POINT('Ctrl Pts',(50.1781102736215,52.8170830289052,12.));
#108840=CARTESIAN_POINT('Ctrl Pts',(50.1686422850493,52.793401641121,12.));
#108841=CARTESIAN_POINT('Ctrl Pts',(50.1591664773561,52.769765553794,12.));
#108842=CARTESIAN_POINT('Ctrl Pts',(50.1496829391068,52.7461748428733,12.));
#108843=CARTESIAN_POINT('Ctrl Pts',(50.1401917592532,52.7226295845156,12.));
#108844=CARTESIAN_POINT('Ctrl Pts',(50.1306930271343,52.6991298550928,12.));
#108845=CARTESIAN_POINT('Ctrl Pts',(50.1211868324781,52.6756757311979,12.));
#108846=CARTESIAN_POINT('Ctrl Pts',(50.1116732654041,52.6522672896462,12.));
#108847=CARTESIAN_POINT('Ctrl Pts',(50.1021524164261,52.6289046074743,12.));
#108848=CARTESIAN_POINT('Ctrl Pts',(50.0926243764569,52.6055877619338,12.));
#108849=CARTESIAN_POINT('Ctrl Pts',(50.0830892368095,52.5823168304981,12.));
#108850=CARTESIAN_POINT('Ctrl Pts',(50.0735470891996,52.5590918908691,12.));
#108851=CARTESIAN_POINT('Ctrl Pts',(50.0639980257477,52.5359130209789,12.));
#108852=CARTESIAN_POINT('Ctrl Pts',(50.0544421389824,52.5127802989903,12.));
#108853=CARTESIAN_POINT('Ctrl Pts',(50.0448795218453,52.4896938032896,12.));
#108854=CARTESIAN_POINT('Ctrl Pts',(50.0353102676933,52.4666536124926,12.));
#108855=CARTESIAN_POINT('Ctrl Pts',(50.0257344703008,52.4436598054523,12.));
#108856=CARTESIAN_POINT('Ctrl Pts',(50.0161522238619,52.420712461261,12.));
#108857=CARTESIAN_POINT('Ctrl Pts',(50.0065636229934,52.3978116592505,12.));
#108858=CARTESIAN_POINT('Ctrl Pts',(49.9969687627402,52.3749574789865,12.));
#108859=CARTESIAN_POINT('Ctrl Pts',(49.9873677385769,52.3521500002711,12.));
#108860=CARTESIAN_POINT('Ctrl Pts',(49.9777606464103,52.3293893031524,12.));
#108861=CARTESIAN_POINT('Ctrl Pts',(49.9681475825824,52.3066754679265,12.));
#108862=CARTESIAN_POINT('Ctrl Pts',(49.9585286438734,52.2840085751385,12.));
#108863=CARTESIAN_POINT('Ctrl Pts',(49.9489039275064,52.2613887055773,12.));
#108864=CARTESIAN_POINT('Ctrl Pts',(49.9392735311507,52.238815940277,12.));
#108865=CARTESIAN_POINT('Ctrl Pts',(49.9296375529241,52.2162903605272,12.));
#108866=CARTESIAN_POINT('Ctrl Pts',(49.919996091396,52.1938120478752,12.));
#108867=CARTESIAN_POINT('Ctrl Pts',(49.9103492455904,52.1713810841277,12.));
#108868=CARTESIAN_POINT('Ctrl Pts',(49.90069711499,52.1489975513449,12.));
#108869=CARTESIAN_POINT('Ctrl Pts',(49.8910397995404,52.1266615318414,12.));
#108870=CARTESIAN_POINT('Ctrl Pts',(49.8813773996523,52.1043731081968,12.));
#108871=CARTESIAN_POINT('Ctrl Pts',(49.871710016205,52.0821323632588,12.));
#108872=CARTESIAN_POINT('Ctrl Pts',(49.8620377505498,52.059939380145,12.));
#108873=CARTESIAN_POINT('Ctrl Pts',(49.8523607045146,52.0377942422373,12.));
#108874=CARTESIAN_POINT('Ctrl Pts',(49.8426789804068,52.015697033182,12.));
#108875=CARTESIAN_POINT('Ctrl Pts',(49.8329926810172,51.9936478369008,12.));
#108876=CARTESIAN_POINT('Ctrl Pts',(49.8233019096224,51.9716467375938,12.));
#108877=CARTESIAN_POINT('Ctrl Pts',(49.8136067699896,51.9496938197418,12.));
#108878=CARTESIAN_POINT('Ctrl Pts',(49.8039073663808,51.9277891681014,12.));
#108879=CARTESIAN_POINT('Ctrl Pts',(49.7942038035568,51.9059328677051,12.));
#108880=CARTESIAN_POINT('Ctrl Pts',(49.78449618678,51.8841250038716,12.));
#108881=CARTESIAN_POINT('Ctrl Pts',(49.7747846218177,51.8623656622092,12.));
#108882=CARTESIAN_POINT('Ctrl Pts',(49.7650692149464,51.8406549286177,12.));
#108883=CARTESIAN_POINT('Ctrl Pts',(49.7553500729563,51.8189928892841,12.));
#108884=CARTESIAN_POINT('Ctrl Pts',(49.7456273031555,51.7973796306826,12.));
#108885=CARTESIAN_POINT('Ctrl Pts',(49.7359010133741,51.7758152395857,12.));
#108886=CARTESIAN_POINT('Ctrl Pts',(49.7261713119672,51.754299803068,12.));
#108887=CARTESIAN_POINT('Ctrl Pts',(49.7164383078206,51.7328334085084,12.));
#108888=CARTESIAN_POINT('Ctrl Pts',(49.7067021103534,51.7114161435848,12.));
#108889=CARTESIAN_POINT('Ctrl Pts',(49.6969628295236,51.6900480962744,12.));
#108890=CARTESIAN_POINT('Ctrl Pts',(49.6872205758314,51.6687293548656,12.));
#108891=CARTESIAN_POINT('Ctrl Pts',(49.6774754603235,51.6474600079611,12.));
#108892=CARTESIAN_POINT('Ctrl Pts',(49.6677275945975,51.6262401444799,12.));
#108893=CARTESIAN_POINT('Ctrl Pts',(49.6579770908063,51.6050698536525,12.));
#108894=CARTESIAN_POINT('Ctrl Pts',(49.6482240616627,51.5839492250218,12.));
#108895=CARTESIAN_POINT('Ctrl Pts',(49.6384686204443,51.5628783484556,12.));
#108896=CARTESIAN_POINT('Ctrl Pts',(49.6287108809975,51.5418573141494,12.));
#108897=CARTESIAN_POINT('Ctrl Pts',(49.6189509577441,51.5208862126303,12.));
#108898=CARTESIAN_POINT('Ctrl Pts',(49.609188965684,51.4999651347496,12.));
#108899=CARTESIAN_POINT('Ctrl Pts',(49.5994250204003,51.4790941716859,12.));
#108900=CARTESIAN_POINT('Ctrl Pts',(49.5896592380634,51.4582734149562,12.));
#108901=CARTESIAN_POINT('Ctrl Pts',(49.579891735436,51.4375029564191,12.));
#108902=CARTESIAN_POINT('Ctrl Pts',(49.5701226298779,51.4167828882765,12.));
#108903=CARTESIAN_POINT('Ctrl Pts',(49.5603520393514,51.3961133030688,12.));
#108904=CARTESIAN_POINT('Ctrl Pts',(49.5505800824268,51.3754942936796,12.));
#108905=CARTESIAN_POINT('Ctrl Pts',(49.5408068782871,51.354925953347,12.));
#108906=CARTESIAN_POINT('Ctrl Pts',(49.5310325467334,51.3344083756659,12.));
#108907=CARTESIAN_POINT('Ctrl Pts',(49.5212572081901,51.3139416545903,12.));
#108908=CARTESIAN_POINT('Ctrl Pts',(49.5114809837111,51.2935258844278,12.));
#108909=CARTESIAN_POINT('Ctrl Pts',(49.5017039949841,51.2731611598465,12.));
#108910=CARTESIAN_POINT('Ctrl Pts',(49.4919263643357,51.2528475758841,12.));
#108911=CARTESIAN_POINT('Ctrl Pts',(49.4821482147357,51.2325852279507,12.));
#108912=CARTESIAN_POINT('Ctrl Pts',(49.4723696698022,51.2123742118288,12.));
#108913=CARTESIAN_POINT('Ctrl Pts',(49.4625908538076,51.1922146236686,12.));
#108914=CARTESIAN_POINT('Ctrl Pts',(49.4528118916833,51.1721065599972,12.));
#108915=CARTESIAN_POINT('Ctrl Pts',(49.4430329090288,51.1520501177291,12.));
#108916=CARTESIAN_POINT('Ctrl Pts',(49.4332540321178,51.1320453941702,12.));
#108917=CARTESIAN_POINT('Ctrl Pts',(49.4234753879071,51.1120924870196,12.));
#108918=CARTESIAN_POINT('Ctrl Pts',(49.4136971040428,51.0921914943663,12.));
#108919=CARTESIAN_POINT('Ctrl Pts',(49.4039193088635,51.0723425146987,12.));
#108920=CARTESIAN_POINT('Ctrl Pts',(49.3941421314014,51.0525456469072,12.));
#108921=CARTESIAN_POINT('Ctrl Pts',(49.3843657013851,51.0328009902857,12.));
#108922=CARTESIAN_POINT('Ctrl Pts',(49.3745901492428,51.0131086445268,12.));
#108923=CARTESIAN_POINT('Ctrl Pts',(49.3648156061049,50.9934687097179,12.));
#108924=CARTESIAN_POINT('Ctrl Pts',(49.3550422038221,50.9738812863636,12.));
#108925=CARTESIAN_POINT('Ctrl Pts',(49.3452700749804,50.9543464753974,12.));
#108926=CARTESIAN_POINT('Ctrl Pts',(49.3354993529163,50.9348643781928,12.));
#108927=CARTESIAN_POINT('Ctrl Pts',(49.325730171735,50.9154350965681,12.));
#108928=CARTESIAN_POINT('Ctrl Pts',(49.3159626663129,50.8960587327869,12.));
#108929=CARTESIAN_POINT('Ctrl Pts',(49.3061969722798,50.8767353895509,12.));
#108930=CARTESIAN_POINT('Ctrl Pts',(49.2964332260043,50.8574651699877,12.));
#108931=CARTESIAN_POINT('Ctrl Pts',(49.2866715645828,50.8382481776392,12.));
#108932=CARTESIAN_POINT('Ctrl Pts',(49.2769121258144,50.8190845164319,12.));
#108933=CARTESIAN_POINT('Ctrl Pts',(49.2671550482415,50.7999742907111,12.));
#108934=CARTESIAN_POINT('Ctrl Pts',(49.2574004712122,50.7809176052954,12.));
#108935=CARTESIAN_POINT('Ctrl Pts',(49.2476485349373,50.7619145655207,12.));
#108936=CARTESIAN_POINT('Ctrl Pts',(49.2378993805482,50.7429652772816,12.));
#108937=CARTESIAN_POINT('Ctrl Pts',(49.2281531501569,50.7240698470698,12.));
#108938=CARTESIAN_POINT('Ctrl Pts',(49.218409986748,50.7052283818941,12.));
#108939=CARTESIAN_POINT('Ctrl Pts',(49.2086700340625,50.6864409891905,12.));
#108940=CARTESIAN_POINT('Ctrl Pts',(49.1989334364991,50.6677077767427,12.));
#108941=CARTESIAN_POINT('Ctrl Pts',(49.1892003389743,50.6490288525639,12.));
#108942=CARTESIAN_POINT('Ctrl Pts',(49.1794708869074,50.6304043248796,12.));
#108943=CARTESIAN_POINT('Ctrl Pts',(49.1697452265473,50.6118343023937,12.));
#108944=CARTESIAN_POINT('Ctrl Pts',(49.1600235052613,50.593318894516,12.));
#108945=CARTESIAN_POINT('Ctrl Pts',(49.1503058717831,50.5748582115575,12.));
#108946=CARTESIAN_POINT('Ctrl Pts',(49.1405924766169,50.5564523650406,12.));
#108947=CARTESIAN_POINT('Ctrl Pts',(49.1308834717645,50.5381014674822,12.));
#108948=CARTESIAN_POINT('Ctrl Pts',(49.1211790099817,50.5198056318111,12.));
#108949=CARTESIAN_POINT('Ctrl Pts',(49.1114792441573,50.5015649708742,12.));
#108950=CARTESIAN_POINT('Ctrl Pts',(49.1017843266782,50.4833795969296,12.));
#108951=CARTESIAN_POINT('Ctrl Pts',(49.0920944086973,50.465249621057,12.));
#108952=CARTESIAN_POINT('Ctrl Pts',(49.0824096415339,50.4471751542717,12.));
#108953=CARTESIAN_POINT('Ctrl Pts',(49.0727301783477,50.4291563088528,12.));
#108954=CARTESIAN_POINT('Ctrl Pts',(49.0630561755082,50.4111931994264,12.));
#108955=CARTESIAN_POINT('Ctrl Pts',(49.0533877945771,50.393285944528,12.));
#108956=CARTESIAN_POINT('Ctrl Pts',(49.0437252024868,50.3754346667389,12.));
#108957=CARTESIAN_POINT('Ctrl Pts',(49.034068567401,50.3576394894136,12.));
#108958=CARTESIAN_POINT('Ctrl Pts',(49.0244180550759,50.3399005337967,12.));
#108959=CARTESIAN_POINT('Ctrl Pts',(49.0147738256925,50.3222179165102,12.));
#108960=CARTESIAN_POINT('Ctrl Pts',(49.0051360288002,50.3045917455383,12.));
#108961=CARTESIAN_POINT('Ctrl Pts',(48.9955048082028,50.2870221241003,12.));
#108962=CARTESIAN_POINT('Ctrl Pts',(48.9858803116649,50.2695091583473,12.));
#108963=CARTESIAN_POINT('Ctrl Pts',(48.9762626987227,50.252052963548,12.));
#108964=CARTESIAN_POINT('Ctrl Pts',(48.9666521500969,50.2346536715465,12.));
#108965=CARTESIAN_POINT('Ctrl Pts',(48.9570488741273,50.2173114358423,12.));
#108966=CARTESIAN_POINT('Ctrl Pts',(48.9474530868847,50.2000264157903,12.));
#108967=CARTESIAN_POINT('Ctrl Pts',(48.9378649933116,50.1827987615659,12.));
#108968=CARTESIAN_POINT('Ctrl Pts',(48.9282847698237,50.1656286003943,12.));
#108969=CARTESIAN_POINT('Ctrl Pts',(48.9187125417897,50.148516018447,12.));
#108970=CARTESIAN_POINT('Ctrl Pts',(48.9091483817797,50.1314610602286,12.));
#108971=CARTESIAN_POINT('Ctrl Pts',(48.9015035371772,50.1178632066821,12.));
#108972=CARTESIAN_POINT('Ctrl Pts',(48.8957735556681,50.1076907555303,12.));
#108973=CARTESIAN_POINT('Ctrl Pts',(48.8919551910299,50.1009206494209,12.));
#108974=CARTESIAN_POINT('Ctrl Pts',(48.8900464144686,50.0975384783634,12.));
#108975=CARTESIAN_POINT('Ctrl Pts',(49.5707719660639,55.2174072001495,-5.55111512312578E-16));
#108976=CARTESIAN_POINT('Ctrl Pts',(49.5707719660639,55.2174072001495,4.));
#108977=CARTESIAN_POINT('Ctrl Pts',(49.5707719660639,55.2174072001495,8.));
#108978=CARTESIAN_POINT('Ctrl Pts',(49.5707719660639,55.2174072001495,12.));
#108979=CARTESIAN_POINT('Ctrl Pts',(49.6712810246933,55.2618153697169,-5.55111512312578E-16));
#108980=CARTESIAN_POINT('Ctrl Pts',(49.6712810246933,55.2618153697169,4.));
#108981=CARTESIAN_POINT('Ctrl Pts',(49.6712810246933,55.2618153697169,8.));
#108982=CARTESIAN_POINT('Ctrl Pts',(49.6712810246933,55.2618153697169,12.));
#108983=CARTESIAN_POINT('Ctrl Pts',(49.8732090625342,55.2790667815473,-5.55111512312578E-16));
#108984=CARTESIAN_POINT('Ctrl Pts',(49.8732090625342,55.2790667815473,4.));
#108985=CARTESIAN_POINT('Ctrl Pts',(49.8732090625342,55.2790667815473,7.99999999999999));
#108986=CARTESIAN_POINT('Ctrl Pts',(49.8732090625342,55.2790667815473,12.));
#108987=CARTESIAN_POINT('Ctrl Pts',(50.0481613529516,55.1854902750885,-5.55111512312578E-16));
#108988=CARTESIAN_POINT('Ctrl Pts',(50.0481613529516,55.1854902750885,4.));
#108989=CARTESIAN_POINT('Ctrl Pts',(50.0481613529516,55.1854902750885,8.00000000000001));
#108990=CARTESIAN_POINT('Ctrl Pts',(50.0481613529516,55.1854902750885,12.));
#108991=CARTESIAN_POINT('Ctrl Pts',(50.1091461876225,55.1300595714123,-5.55111512312578E-16));
#108992=CARTESIAN_POINT('Ctrl Pts',(50.1091461876225,55.1300595714123,4.));
#108993=CARTESIAN_POINT('Ctrl Pts',(50.1091461876225,55.1300595714123,8.));
#108994=CARTESIAN_POINT('Ctrl Pts',(50.1091461876225,55.1300595714123,12.));
#108995=CARTESIAN_POINT('',(49.5707719660639,55.2174072001495,-2.77555756156289E-16));
#108996=CARTESIAN_POINT('',(50.1091461876225,55.1300595714124,2.77555756156289E-16));
#108997=CARTESIAN_POINT('Ctrl Pts',(49.5707719660639,55.2174072001495,-5.55111512312578E-16));
#108998=CARTESIAN_POINT('Ctrl Pts',(49.6712810246933,55.2618153697169,-5.55111512312578E-16));
#108999=CARTESIAN_POINT('Ctrl Pts',(49.7866684748881,55.2716733193343,-5.55111512312578E-16));
#109000=CARTESIAN_POINT('Ctrl Pts',(49.8932475177609,55.2453425609388,-5.55111512312578E-16));
#109001=CARTESIAN_POINT('Ctrl Pts',(49.9731817999155,55.2255944921423,-5.55111512312578E-16));
#109002=CARTESIAN_POINT('Ctrl Pts',(50.0481613529516,55.1854902750885,-5.55111512312578E-16));
#109003=CARTESIAN_POINT('Ctrl Pts',(50.1091461876225,55.1300595714123,-5.55111512312578E-16));
#109004=CARTESIAN_POINT('',(50.1091461876225,55.1300595714124,12.));
#109005=CARTESIAN_POINT('Ctrl Pts',(50.1091461876225,55.1300595714123,-5.55111512312578E-16));
#109006=CARTESIAN_POINT('Ctrl Pts',(50.1091461876225,55.1300595714123,4.));
#109007=CARTESIAN_POINT('Ctrl Pts',(50.1091461876225,55.1300595714123,8.));
#109008=CARTESIAN_POINT('Ctrl Pts',(50.1091461876225,55.1300595714123,12.));
#109009=CARTESIAN_POINT('',(49.5707719660639,55.2174072001495,12.));
#109010=CARTESIAN_POINT('Ctrl Pts',(50.1091461876225,55.1300595714123,12.));
#109011=CARTESIAN_POINT('Ctrl Pts',(50.0481613529516,55.1854902750885,12.));
#109012=CARTESIAN_POINT('Ctrl Pts',(49.9731817999155,55.2255944921423,12.));
#109013=CARTESIAN_POINT('Ctrl Pts',(49.8932475177609,55.2453425609388,12.));
#109014=CARTESIAN_POINT('Ctrl Pts',(49.7866684748881,55.2716733193343,12.));
#109015=CARTESIAN_POINT('Ctrl Pts',(49.6712810246933,55.2618153697169,12.));
#109016=CARTESIAN_POINT('Ctrl Pts',(49.5707719660639,55.2174072001495,12.));
#109017=CARTESIAN_POINT('Ctrl Pts',(49.5707719660639,55.2174072001495,12.));
#109018=CARTESIAN_POINT('Ctrl Pts',(49.5707719660639,55.2174072001495,8.));
#109019=CARTESIAN_POINT('Ctrl Pts',(49.5707719660639,55.2174072001495,4.));
#109020=CARTESIAN_POINT('Ctrl Pts',(49.5707719660639,55.2174072001495,-5.55111512312578E-16));
#109021=CARTESIAN_POINT('Origin',(2.53167595884892E-10,2.7643087079898E-10,
0.));
#109022=CARTESIAN_POINT('Origin',(2.53167595884892E-10,2.7643087079898E-10,
12.));
#109023=CARTESIAN_POINT('Origin',(2.53167595884892E-10,2.7643087079898E-10,
0.));
#109024=CARTESIAN_POINT('Ctrl Pts',(55.1300595714105,50.1091461876246,0.));
#109025=CARTESIAN_POINT('Ctrl Pts',(55.1300595714105,50.1091461876246,4.));
#109026=CARTESIAN_POINT('Ctrl Pts',(55.1300595714105,50.1091461876246,8.));
#109027=CARTESIAN_POINT('Ctrl Pts',(55.1300595714105,50.1091461876246,12.));
#109028=CARTESIAN_POINT('Ctrl Pts',(55.2039671763178,50.0278330747237,0.));
#109029=CARTESIAN_POINT('Ctrl Pts',(55.2039671763178,50.0278330747237,4.));
#109030=CARTESIAN_POINT('Ctrl Pts',(55.2039671763178,50.0278330747237,8.));
#109031=CARTESIAN_POINT('Ctrl Pts',(55.2039671763178,50.0278330747237,12.));
#109032=CARTESIAN_POINT('Ctrl Pts',(55.2841761056306,49.8417173275612,0.));
#109033=CARTESIAN_POINT('Ctrl Pts',(55.2841761056306,49.8417173275612,4.));
#109034=CARTESIAN_POINT('Ctrl Pts',(55.2841761056306,49.8417173275612,7.99999999999999));
#109035=CARTESIAN_POINT('Ctrl Pts',(55.2841761056306,49.8417173275612,12.));
#109036=CARTESIAN_POINT('Ctrl Pts',(55.2507133273147,49.6461537600002,0.));
#109037=CARTESIAN_POINT('Ctrl Pts',(55.2507133273147,49.6461537600002,4.));
#109038=CARTESIAN_POINT('Ctrl Pts',(55.2507133273147,49.6461537600002,8.00000000000001));
#109039=CARTESIAN_POINT('Ctrl Pts',(55.2507133273147,49.6461537600002,12.));
#109040=CARTESIAN_POINT('Ctrl Pts',(55.21740720013,49.5707719660253,0.));
#109041=CARTESIAN_POINT('Ctrl Pts',(55.21740720013,49.5707719660253,4.));
#109042=CARTESIAN_POINT('Ctrl Pts',(55.21740720013,49.5707719660253,8.));
#109043=CARTESIAN_POINT('Ctrl Pts',(55.21740720013,49.5707719660253,12.));
#109044=CARTESIAN_POINT('',(55.1300595714105,50.1091461876246,0.));
#109045=CARTESIAN_POINT('',(55.2174072001297,49.5707719660254,0.));
#109046=CARTESIAN_POINT('Ctrl Pts',(55.1300595714105,50.1091461876246,1.38777878078145E-16));
#109047=CARTESIAN_POINT('Ctrl Pts',(55.2039671763178,50.0278330747237,1.38777878078145E-16));
#109048=CARTESIAN_POINT('Ctrl Pts',(55.2498008502108,49.9214812192023,1.38777878078145E-16));
#109049=CARTESIAN_POINT('Ctrl Pts',(55.2585172318169,49.8120443611017,1.38777878078145E-16));
#109050=CARTESIAN_POINT('Ctrl Pts',(55.2650545180215,49.7299667175263,1.38777878078145E-16));
#109051=CARTESIAN_POINT('Ctrl Pts',(55.2507133273147,49.6461537600002,1.38777878078144E-16));
#109052=CARTESIAN_POINT('Ctrl Pts',(55.21740720013,49.5707719660253,1.38777878078145E-16));
#109053=CARTESIAN_POINT('',(55.2174072001297,49.5707719660254,12.));
#109054=CARTESIAN_POINT('Ctrl Pts',(55.21740720013,49.5707719660253,0.));
#109055=CARTESIAN_POINT('Ctrl Pts',(55.21740720013,49.5707719660253,4.));
#109056=CARTESIAN_POINT('Ctrl Pts',(55.21740720013,49.5707719660253,8.));
#109057=CARTESIAN_POINT('Ctrl Pts',(55.21740720013,49.5707719660253,12.));
#109058=CARTESIAN_POINT('',(55.1300595714105,50.1091461876246,12.));
#109059=CARTESIAN_POINT('Ctrl Pts',(55.21740720013,49.5707719660253,12.));
#109060=CARTESIAN_POINT('Ctrl Pts',(55.2507133273147,49.6461537600002,12.));
#109061=CARTESIAN_POINT('Ctrl Pts',(55.2650545180215,49.7299667175263,12.));
#109062=CARTESIAN_POINT('Ctrl Pts',(55.2585172318169,49.8120443611017,12.));
#109063=CARTESIAN_POINT('Ctrl Pts',(55.2498008502108,49.9214812192023,12.));
#109064=CARTESIAN_POINT('Ctrl Pts',(55.2039671763178,50.0278330747237,12.));
#109065=CARTESIAN_POINT('Ctrl Pts',(55.1300595714105,50.1091461876246,12.));
#109066=CARTESIAN_POINT('Ctrl Pts',(55.1300595714105,50.1091461876246,12.));
#109067=CARTESIAN_POINT('Ctrl Pts',(55.1300595714105,50.1091461876246,8.));
#109068=CARTESIAN_POINT('Ctrl Pts',(55.1300595714105,50.1091461876246,4.));
#109069=CARTESIAN_POINT('Ctrl Pts',(55.1300595714105,50.1091461876246,0.));
#109070=CARTESIAN_POINT('Ctrl Pts',(53.0702932034641,45.6458539113724,0.));
#109071=CARTESIAN_POINT('Ctrl Pts',(53.0702932034641,45.6458539113724,12.));
#109072=CARTESIAN_POINT('Ctrl Pts',(53.0724894921849,45.6490568514089,0.));
#109073=CARTESIAN_POINT('Ctrl Pts',(53.0724894921849,45.6490568514089,12.));
#109074=CARTESIAN_POINT('Ctrl Pts',(53.0768833804193,45.6554684028145,0.));
#109075=CARTESIAN_POINT('Ctrl Pts',(53.0768833804193,45.6554684028145,12.));
#109076=CARTESIAN_POINT('Ctrl Pts',(53.0834781451546,45.6651027439241,0.));
#109077=CARTESIAN_POINT('Ctrl Pts',(53.0834781451546,45.6651027439241,12.));
#109078=CARTESIAN_POINT('Ctrl Pts',(53.0922790298409,45.6779825614231,0.));
#109079=CARTESIAN_POINT('Ctrl Pts',(53.0922790298409,45.6779825614231,12.));
#109080=CARTESIAN_POINT('Ctrl Pts',(53.1032932328857,45.694139048907,0.));
#109081=CARTESIAN_POINT('Ctrl Pts',(53.1032932328857,45.694139048907,12.));
#109082=CARTESIAN_POINT('Ctrl Pts',(53.114320495492,45.7103522376696,0.));
#109083=CARTESIAN_POINT('Ctrl Pts',(53.114320495492,45.7103522376696,12.));
#109084=CARTESIAN_POINT('Ctrl Pts',(53.1253607414872,45.7266220897003,0.));
#109085=CARTESIAN_POINT('Ctrl Pts',(53.1253607414872,45.7266220897003,12.));
#109086=CARTESIAN_POINT('Ctrl Pts',(53.1364138384693,45.7429485300823,0.));
#109087=CARTESIAN_POINT('Ctrl Pts',(53.1364138384693,45.7429485300823,12.));
#109088=CARTESIAN_POINT('Ctrl Pts',(53.1474795996053,45.7593314474501,0.));
#109089=CARTESIAN_POINT('Ctrl Pts',(53.1474795996053,45.7593314474501,12.));
#109090=CARTESIAN_POINT('Ctrl Pts',(53.1585578076444,45.7757707100618,0.));
#109091=CARTESIAN_POINT('Ctrl Pts',(53.1585578076444,45.7757707100618,12.));
#109092=CARTESIAN_POINT('Ctrl Pts',(53.1696482334487,45.7922661780005,0.));
#109093=CARTESIAN_POINT('Ctrl Pts',(53.1696482334487,45.7922661780005,12.));
#109094=CARTESIAN_POINT('Ctrl Pts',(53.1807506560933,45.808817716509,0.));
#109095=CARTESIAN_POINT('Ctrl Pts',(53.1807506560933,45.808817716509,12.));
#109096=CARTESIAN_POINT('Ctrl Pts',(53.1918648840541,45.8254252099957,0.));
#109097=CARTESIAN_POINT('Ctrl Pts',(53.1918648840541,45.8254252099957,12.));
#109098=CARTESIAN_POINT('Ctrl Pts',(53.2029907483557,45.8420885575349,0.));
#109099=CARTESIAN_POINT('Ctrl Pts',(53.2029907483557,45.8420885575349,12.));
#109100=CARTESIAN_POINT('Ctrl Pts',(53.2141280925439,45.8588076662582,0.));
#109101=CARTESIAN_POINT('Ctrl Pts',(53.2141280925439,45.8588076662582,12.));
#109102=CARTESIAN_POINT('Ctrl Pts',(53.2252767643662,45.8755824458723,0.));
#109103=CARTESIAN_POINT('Ctrl Pts',(53.2252767643662,45.8755824458723,12.));
#109104=CARTESIAN_POINT('Ctrl Pts',(53.2364366054306,45.892412801838,0.));
#109105=CARTESIAN_POINT('Ctrl Pts',(53.2364366054306,45.892412801838,12.));
#109106=CARTESIAN_POINT('Ctrl Pts',(53.2476074460017,45.9092986319377,0.));
#109107=CARTESIAN_POINT('Ctrl Pts',(53.2476074460017,45.9092986319377,12.));
#109108=CARTESIAN_POINT('Ctrl Pts',(53.2587891103866,45.9262398298349,0.));
#109109=CARTESIAN_POINT('Ctrl Pts',(53.2587891103866,45.9262398298349,12.));
#109110=CARTESIAN_POINT('Ctrl Pts',(53.2699814203105,45.9432362873008,0.));
#109111=CARTESIAN_POINT('Ctrl Pts',(53.2699814203105,45.9432362873008,12.));
#109112=CARTESIAN_POINT('Ctrl Pts',(53.2811841987926,45.9602878967698,0.));
#109113=CARTESIAN_POINT('Ctrl Pts',(53.2811841987926,45.9602878967698,12.));
#109114=CARTESIAN_POINT('Ctrl Pts',(53.292397274555,45.9773945542384,0.));
#109115=CARTESIAN_POINT('Ctrl Pts',(53.292397274555,45.9773945542384,12.));
#109116=CARTESIAN_POINT('Ctrl Pts',(53.3036204818329,45.9945561591453,0.));
#109117=CARTESIAN_POINT('Ctrl Pts',(53.3036204818329,45.9945561591453,12.));
#109118=CARTESIAN_POINT('Ctrl Pts',(53.3148536582635,46.0117726129873,0.));
#109119=CARTESIAN_POINT('Ctrl Pts',(53.3148536582635,46.0117726129873,12.));
#109120=CARTESIAN_POINT('Ctrl Pts',(53.326096643428,46.02904381836,0.));
#109121=CARTESIAN_POINT('Ctrl Pts',(53.326096643428,46.02904381836,12.));
#109122=CARTESIAN_POINT('Ctrl Pts',(53.3373492770671,46.0463696777801,0.));
#109123=CARTESIAN_POINT('Ctrl Pts',(53.3373492770671,46.0463696777801,12.));
#109124=CARTESIAN_POINT('Ctrl Pts',(53.3486113975901,46.0637500926982,0.));
#109125=CARTESIAN_POINT('Ctrl Pts',(53.3486113975901,46.0637500926982,12.));
#109126=CARTESIAN_POINT('Ctrl Pts',(53.3598828428546,46.0811849640218,0.));
#109127=CARTESIAN_POINT('Ctrl Pts',(53.3598828428546,46.0811849640218,12.));
#109128=CARTESIAN_POINT('Ctrl Pts',(53.3711634508437,46.0986741925656,0.));
#109129=CARTESIAN_POINT('Ctrl Pts',(53.3711634508437,46.0986741925656,12.));
#109130=CARTESIAN_POINT('Ctrl Pts',(53.3824530603276,46.1162176794884,0.));
#109131=CARTESIAN_POINT('Ctrl Pts',(53.3824530603276,46.1162176794884,12.));
#109132=CARTESIAN_POINT('Ctrl Pts',(53.3937515116549,46.1338153268097,0.));
#109133=CARTESIAN_POINT('Ctrl Pts',(53.3937515116549,46.1338153268097,12.));
#109134=CARTESIAN_POINT('Ctrl Pts',(53.4050586470436,46.1514670376012,0.));
#109135=CARTESIAN_POINT('Ctrl Pts',(53.4050586470436,46.1514670376012,12.));
#109136=CARTESIAN_POINT('Ctrl Pts',(53.4163743101517,46.1691727157134,0.));
#109137=CARTESIAN_POINT('Ctrl Pts',(53.4163743101517,46.1691727157134,12.));
#109138=CARTESIAN_POINT('Ctrl Pts',(53.4276983458125,46.1869322656024,0.));
#109139=CARTESIAN_POINT('Ctrl Pts',(53.4276983458125,46.1869322656024,12.));
#109140=CARTESIAN_POINT('Ctrl Pts',(53.4390305997274,46.2047455921286,0.));
#109141=CARTESIAN_POINT('Ctrl Pts',(53.4390305997274,46.2047455921286,12.));
#109142=CARTESIAN_POINT('Ctrl Pts',(53.4503709181178,46.2226126003202,0.));
#109143=CARTESIAN_POINT('Ctrl Pts',(53.4503709181178,46.2226126003202,12.));
#109144=CARTESIAN_POINT('Ctrl Pts',(53.4617191477402,46.2405331953889,0.));
#109145=CARTESIAN_POINT('Ctrl Pts',(53.4617191477402,46.2405331953889,12.));
#109146=CARTESIAN_POINT('Ctrl Pts',(53.4730751360371,46.2585072828353,0.));
#109147=CARTESIAN_POINT('Ctrl Pts',(53.4730751360371,46.2585072828353,12.));
#109148=CARTESIAN_POINT('Ctrl Pts',(53.4844387312414,46.2765347685198,0.));
#109149=CARTESIAN_POINT('Ctrl Pts',(53.4844387312414,46.2765347685198,12.));
#109150=CARTESIAN_POINT('Ctrl Pts',(53.4958097825006,46.2946155587417,0.));
#109151=CARTESIAN_POINT('Ctrl Pts',(53.4958097825006,46.2946155587417,12.));
#109152=CARTESIAN_POINT('Ctrl Pts',(53.5071881399911,46.3127495603098,0.));
#109153=CARTESIAN_POINT('Ctrl Pts',(53.5071881399911,46.3127495603098,12.));
#109154=CARTESIAN_POINT('Ctrl Pts',(53.5185736548548,46.3309366805093,0.));
#109155=CARTESIAN_POINT('Ctrl Pts',(53.5185736548548,46.3309366805093,12.));
#109156=CARTESIAN_POINT('Ctrl Pts',(53.5299661791385,46.3491768270655,0.));
#109157=CARTESIAN_POINT('Ctrl Pts',(53.5299661791385,46.3491768270655,12.));
#109158=CARTESIAN_POINT('Ctrl Pts',(53.5413655657327,46.3674699081046,0.));
#109159=CARTESIAN_POINT('Ctrl Pts',(53.5413655657327,46.3674699081046,12.));
#109160=CARTESIAN_POINT('Ctrl Pts',(53.5527716683048,46.3858158321059,0.));
#109161=CARTESIAN_POINT('Ctrl Pts',(53.5527716683048,46.3858158321059,12.));
#109162=CARTESIAN_POINT('Ctrl Pts',(53.5641843412559,46.4042145078701,0.));
#109163=CARTESIAN_POINT('Ctrl Pts',(53.5641843412559,46.4042145078701,12.));
#109164=CARTESIAN_POINT('Ctrl Pts',(53.5756034397481,46.4226658445474,0.));
#109165=CARTESIAN_POINT('Ctrl Pts',(53.5756034397481,46.4226658445474,12.));
#109166=CARTESIAN_POINT('Ctrl Pts',(53.5870288197166,46.4411697516478,0.));
#109167=CARTESIAN_POINT('Ctrl Pts',(53.5870288197166,46.4411697516478,12.));
#109168=CARTESIAN_POINT('Ctrl Pts',(53.5984603378855,46.459726139052,0.));
#109169=CARTESIAN_POINT('Ctrl Pts',(53.5984603378855,46.459726139052,12.));
#109170=CARTESIAN_POINT('Ctrl Pts',(53.6098978517859,46.4783349170173,0.));
#109171=CARTESIAN_POINT('Ctrl Pts',(53.6098978517859,46.4783349170173,12.));
#109172=CARTESIAN_POINT('Ctrl Pts',(53.6213412197533,46.496995996177,0.));
#109173=CARTESIAN_POINT('Ctrl Pts',(53.6213412197533,46.496995996177,12.));
#109174=CARTESIAN_POINT('Ctrl Pts',(53.6327903009094,46.5157092875373,0.));
#109175=CARTESIAN_POINT('Ctrl Pts',(53.6327903009094,46.5157092875373,12.));
#109176=CARTESIAN_POINT('Ctrl Pts',(53.6442449551455,46.5344747024676,0.));
#109177=CARTESIAN_POINT('Ctrl Pts',(53.6442449551455,46.5344747024676,12.));
#109178=CARTESIAN_POINT('Ctrl Pts',(53.6557050431071,46.5532921526901,0.));
#109179=CARTESIAN_POINT('Ctrl Pts',(53.6557050431071,46.5532921526901,12.));
#109180=CARTESIAN_POINT('Ctrl Pts',(53.6671704261737,46.5721615502591,0.));
#109181=CARTESIAN_POINT('Ctrl Pts',(53.6671704261737,46.5721615502591,12.));
#109182=CARTESIAN_POINT('Ctrl Pts',(53.678640966456,46.5910828075653,0.));
#109183=CARTESIAN_POINT('Ctrl Pts',(53.678640966456,46.5910828075653,12.));
#109184=CARTESIAN_POINT('Ctrl Pts',(53.6901165267941,46.6100558373402,0.));
#109185=CARTESIAN_POINT('Ctrl Pts',(53.6901165267941,46.6100558373402,12.));
#109186=CARTESIAN_POINT('Ctrl Pts',(53.701596970754,46.6290805526559,0.));
#109187=CARTESIAN_POINT('Ctrl Pts',(53.701596970754,46.6290805526559,12.));
#109188=CARTESIAN_POINT('Ctrl Pts',(53.7130821626263,46.6481568669216,0.));
#109189=CARTESIAN_POINT('Ctrl Pts',(53.7130821626263,46.6481568669216,12.));
#109190=CARTESIAN_POINT('Ctrl Pts',(53.7245719674222,46.6672846938752,0.));
#109191=CARTESIAN_POINT('Ctrl Pts',(53.7245719674222,46.6672846938752,12.));
#109192=CARTESIAN_POINT('Ctrl Pts',(53.7360662508677,46.6864639475863,0.));
#109193=CARTESIAN_POINT('Ctrl Pts',(53.7360662508677,46.6864639475863,12.));
#109194=CARTESIAN_POINT('Ctrl Pts',(53.7475648793948,46.7056945424559,0.));
#109195=CARTESIAN_POINT('Ctrl Pts',(53.7475648793948,46.7056945424559,12.));
#109196=CARTESIAN_POINT('Ctrl Pts',(53.7590677201344,46.724976393213,0.));
#109197=CARTESIAN_POINT('Ctrl Pts',(53.7590677201344,46.724976393213,12.));
#109198=CARTESIAN_POINT('Ctrl Pts',(53.770574640907,46.7443094149041,0.));
#109199=CARTESIAN_POINT('Ctrl Pts',(53.770574640907,46.7443094149041,12.));
#109200=CARTESIAN_POINT('Ctrl Pts',(53.782085510217,46.7636935228851,0.));
#109201=CARTESIAN_POINT('Ctrl Pts',(53.782085510217,46.7636935228851,12.));
#109202=CARTESIAN_POINT('Ctrl Pts',(53.7936001972468,46.7831286328268,0.));
#109203=CARTESIAN_POINT('Ctrl Pts',(53.7936001972468,46.7831286328268,12.));
#109204=CARTESIAN_POINT('Ctrl Pts',(53.8051185718525,46.8026146607144,0.));
#109205=CARTESIAN_POINT('Ctrl Pts',(53.8051185718525,46.8026146607144,12.));
#109206=CARTESIAN_POINT('Ctrl Pts',(53.8166405045582,46.8221515228459,0.));
#109207=CARTESIAN_POINT('Ctrl Pts',(53.8166405045582,46.8221515228459,12.));
#109208=CARTESIAN_POINT('Ctrl Pts',(53.8281658665517,46.8417391358231,0.));
#109209=CARTESIAN_POINT('Ctrl Pts',(53.8281658665517,46.8417391358231,12.));
#109210=CARTESIAN_POINT('Ctrl Pts',(53.8396945296777,46.8613774165452,0.));
#109211=CARTESIAN_POINT('Ctrl Pts',(53.8396945296777,46.8613774165452,12.));
#109212=CARTESIAN_POINT('Ctrl Pts',(53.851226366434,46.8810662822147,0.));
#109213=CARTESIAN_POINT('Ctrl Pts',(53.851226366434,46.8810662822147,12.));
#109214=CARTESIAN_POINT('Ctrl Pts',(53.8627612499648,46.900805650336,0.));
#109215=CARTESIAN_POINT('Ctrl Pts',(53.8627612499648,46.900805650336,12.));
#109216=CARTESIAN_POINT('Ctrl Pts',(53.8742990540557,46.9205954387128,0.));
#109217=CARTESIAN_POINT('Ctrl Pts',(53.8742990540557,46.9205954387128,12.));
#109218=CARTESIAN_POINT('Ctrl Pts',(53.8858396531277,46.9404355654381,0.));
#109219=CARTESIAN_POINT('Ctrl Pts',(53.8858396531277,46.9404355654381,12.));
#109220=CARTESIAN_POINT('Ctrl Pts',(53.8973829222317,46.9603259488894,0.));
#109221=CARTESIAN_POINT('Ctrl Pts',(53.8973829222317,46.9603259488894,12.));
#109222=CARTESIAN_POINT('Ctrl Pts',(53.9089287370436,46.9802665077342,0.));
#109223=CARTESIAN_POINT('Ctrl Pts',(53.9089287370436,46.9802665077342,12.));
#109224=CARTESIAN_POINT('Ctrl Pts',(53.9204769738584,47.0002571609286,0.));
#109225=CARTESIAN_POINT('Ctrl Pts',(53.9204769738584,47.0002571609286,12.));
#109226=CARTESIAN_POINT('Ctrl Pts',(53.9320275095864,47.0202978277148,0.));
#109227=CARTESIAN_POINT('Ctrl Pts',(53.9320275095864,47.0202978277148,12.));
#109228=CARTESIAN_POINT('Ctrl Pts',(53.9435802217468,47.04038842761,0.));
#109229=CARTESIAN_POINT('Ctrl Pts',(53.9435802217468,47.04038842761,12.));
#109230=CARTESIAN_POINT('Ctrl Pts',(53.9551349884637,47.0605288804042,0.));
#109231=CARTESIAN_POINT('Ctrl Pts',(53.9551349884637,47.0605288804042,12.));
#109232=CARTESIAN_POINT('Ctrl Pts',(53.9666916884624,47.0807191061674,0.));
#109233=CARTESIAN_POINT('Ctrl Pts',(53.9666916884624,47.0807191061674,12.));
#109234=CARTESIAN_POINT('Ctrl Pts',(53.9782502010642,47.1009590252466,0.));
#109235=CARTESIAN_POINT('Ctrl Pts',(53.9782502010642,47.1009590252466,12.));
#109236=CARTESIAN_POINT('Ctrl Pts',(53.9898104061809,47.1212485582632,0.));
#109237=CARTESIAN_POINT('Ctrl Pts',(53.9898104061809,47.1212485582632,12.));
#109238=CARTESIAN_POINT('Ctrl Pts',(54.0013721843094,47.1415876261012,0.));
#109239=CARTESIAN_POINT('Ctrl Pts',(54.0013721843094,47.1415876261012,12.));
#109240=CARTESIAN_POINT('Ctrl Pts',(54.0129354165269,47.161976149906,0.));
#109241=CARTESIAN_POINT('Ctrl Pts',(54.0129354165269,47.161976149906,12.));
#109242=CARTESIAN_POINT('Ctrl Pts',(54.0244999844872,47.1824140510906,0.));
#109243=CARTESIAN_POINT('Ctrl Pts',(54.0244999844872,47.1824140510906,12.));
#109244=CARTESIAN_POINT('Ctrl Pts',(54.0360657704156,47.2029012513334,0.));
#109245=CARTESIAN_POINT('Ctrl Pts',(54.0360657704156,47.2029012513334,12.));
#109246=CARTESIAN_POINT('Ctrl Pts',(54.047632657105,47.2234376725752,0.));
#109247=CARTESIAN_POINT('Ctrl Pts',(54.047632657105,47.2234376725752,12.));
#109248=CARTESIAN_POINT('Ctrl Pts',(54.0592005279108,47.2440232370085,0.));
#109249=CARTESIAN_POINT('Ctrl Pts',(54.0592005279108,47.2440232370085,12.));
#109250=CARTESIAN_POINT('Ctrl Pts',(54.0707692667461,47.2646578670767,0.));
#109251=CARTESIAN_POINT('Ctrl Pts',(54.0707692667461,47.2646578670767,12.));
#109252=CARTESIAN_POINT('Ctrl Pts',(54.082338758079,47.2853414854805,0.));
#109253=CARTESIAN_POINT('Ctrl Pts',(54.082338758079,47.2853414854805,12.));
#109254=CARTESIAN_POINT('Ctrl Pts',(54.0939088869271,47.3060740151754,0.));
#109255=CARTESIAN_POINT('Ctrl Pts',(54.0939088869271,47.3060740151754,12.));
#109256=CARTESIAN_POINT('Ctrl Pts',(54.1054795388538,47.326855379369,0.));
#109257=CARTESIAN_POINT('Ctrl Pts',(54.1054795388538,47.326855379369,12.));
#109258=CARTESIAN_POINT('Ctrl Pts',(54.1170505999637,47.3476855015095,0.));
#109259=CARTESIAN_POINT('Ctrl Pts',(54.1170505999637,47.3476855015095,12.));
#109260=CARTESIAN_POINT('Ctrl Pts',(54.1286219568981,47.3685643052867,0.));
#109261=CARTESIAN_POINT('Ctrl Pts',(54.1286219568981,47.3685643052867,12.));
#109262=CARTESIAN_POINT('Ctrl Pts',(54.1401934968306,47.3894917146361,0.));
#109263=CARTESIAN_POINT('Ctrl Pts',(54.1401934968306,47.3894917146361,12.));
#109264=CARTESIAN_POINT('Ctrl Pts',(54.1517651074638,47.4104676537381,0.));
#109265=CARTESIAN_POINT('Ctrl Pts',(54.1517651074638,47.4104676537381,12.));
#109266=CARTESIAN_POINT('Ctrl Pts',(54.163336677024,47.4314920470142,0.));
#109267=CARTESIAN_POINT('Ctrl Pts',(54.163336677024,47.4314920470142,12.));
#109268=CARTESIAN_POINT('Ctrl Pts',(54.1749080942593,47.4525648191173,0.));
#109269=CARTESIAN_POINT('Ctrl Pts',(54.1749080942593,47.4525648191173,12.));
#109270=CARTESIAN_POINT('Ctrl Pts',(54.1864792484343,47.473685894932,0.));
#109271=CARTESIAN_POINT('Ctrl Pts',(54.1864792484343,47.473685894932,12.));
#109272=CARTESIAN_POINT('Ctrl Pts',(54.1980500293267,47.4948551995799,0.));
#109273=CARTESIAN_POINT('Ctrl Pts',(54.1980500293267,47.4948551995799,12.));
#109274=CARTESIAN_POINT('Ctrl Pts',(54.2096203272228,47.5160726584172,0.));
#109275=CARTESIAN_POINT('Ctrl Pts',(54.2096203272228,47.5160726584172,12.));
#109276=CARTESIAN_POINT('Ctrl Pts',(54.2211900329141,47.5373381970328,0.));
#109277=CARTESIAN_POINT('Ctrl Pts',(54.2211900329141,47.5373381970328,12.));
#109278=CARTESIAN_POINT('Ctrl Pts',(54.232759037693,47.5586517412368,0.));
#109279=CARTESIAN_POINT('Ctrl Pts',(54.232759037693,47.5586517412368,12.));
#109280=CARTESIAN_POINT('Ctrl Pts',(54.2443272333498,47.5800132170614,0.));
#109281=CARTESIAN_POINT('Ctrl Pts',(54.2443272333498,47.5800132170614,12.));
#109282=CARTESIAN_POINT('Ctrl Pts',(54.2558945121684,47.6014225507664,0.));
#109283=CARTESIAN_POINT('Ctrl Pts',(54.2558945121684,47.6014225507664,12.));
#109284=CARTESIAN_POINT('Ctrl Pts',(54.2674607669228,47.6228796688376,0.));
#109285=CARTESIAN_POINT('Ctrl Pts',(54.2674607669228,47.6228796688376,12.));
#109286=CARTESIAN_POINT('Ctrl Pts',(54.2790258908736,47.6443844979846,0.));
#109287=CARTESIAN_POINT('Ctrl Pts',(54.2790258908736,47.6443844979846,12.));
#109288=CARTESIAN_POINT('Ctrl Pts',(54.2905897777647,47.6659369651299,0.));
#109289=CARTESIAN_POINT('Ctrl Pts',(54.2905897777647,47.6659369651299,12.));
#109290=CARTESIAN_POINT('Ctrl Pts',(54.3021523218188,47.6875369974086,0.));
#109291=CARTESIAN_POINT('Ctrl Pts',(54.3021523218188,47.6875369974086,12.));
#109292=CARTESIAN_POINT('Ctrl Pts',(54.3137134177345,47.7091845221748,0.));
#109293=CARTESIAN_POINT('Ctrl Pts',(54.3137134177345,47.7091845221748,12.));
#109294=CARTESIAN_POINT('Ctrl Pts',(54.3252729606824,47.7308794669994,0.));
#109295=CARTESIAN_POINT('Ctrl Pts',(54.3252729606824,47.7308794669994,12.));
#109296=CARTESIAN_POINT('Ctrl Pts',(54.3368308463023,47.7526217596694,0.));
#109297=CARTESIAN_POINT('Ctrl Pts',(54.3368308463023,47.7526217596694,12.));
#109298=CARTESIAN_POINT('Ctrl Pts',(54.3483869706998,47.7744113281768,0.));
#109299=CARTESIAN_POINT('Ctrl Pts',(54.3483869706998,47.7744113281768,12.));
#109300=CARTESIAN_POINT('Ctrl Pts',(54.3599412304431,47.7962481007179,0.));
#109301=CARTESIAN_POINT('Ctrl Pts',(54.3599412304431,47.7962481007179,12.));
#109302=CARTESIAN_POINT('Ctrl Pts',(54.3714935225585,47.8181320056988,0.));
#109303=CARTESIAN_POINT('Ctrl Pts',(54.3714935225585,47.8181320056988,12.));
#109304=CARTESIAN_POINT('Ctrl Pts',(54.3830437445275,47.8400629717352,0.));
#109305=CARTESIAN_POINT('Ctrl Pts',(54.3830437445275,47.8400629717352,12.));
#109306=CARTESIAN_POINT('Ctrl Pts',(54.3945917942835,47.8620409276495,0.));
#109307=CARTESIAN_POINT('Ctrl Pts',(54.3945917942835,47.8620409276495,12.));
#109308=CARTESIAN_POINT('Ctrl Pts',(54.4061375702088,47.8840658024626,0.));
#109309=CARTESIAN_POINT('Ctrl Pts',(54.4061375702088,47.8840658024626,12.));
#109310=CARTESIAN_POINT('Ctrl Pts',(54.4176809711324,47.9061375253909,0.));
#109311=CARTESIAN_POINT('Ctrl Pts',(54.4176809711324,47.9061375253909,12.));
#109312=CARTESIAN_POINT('Ctrl Pts',(54.4292218963253,47.9282560258528,0.));
#109313=CARTESIAN_POINT('Ctrl Pts',(54.4292218963253,47.9282560258528,12.));
#109314=CARTESIAN_POINT('Ctrl Pts',(54.4407602454974,47.9504212334681,0.));
#109315=CARTESIAN_POINT('Ctrl Pts',(54.4407602454974,47.9504212334681,12.));
#109316=CARTESIAN_POINT('Ctrl Pts',(54.4522959187952,47.972633078057,0.));
#109317=CARTESIAN_POINT('Ctrl Pts',(54.4522959187952,47.972633078057,12.));
#109318=CARTESIAN_POINT('Ctrl Pts',(54.4638288167991,47.9948914896316,0.));
#109319=CARTESIAN_POINT('Ctrl Pts',(54.4638288167991,47.9948914896316,12.));
#109320=CARTESIAN_POINT('Ctrl Pts',(54.4753588405202,48.0171963983912,0.));
#109321=CARTESIAN_POINT('Ctrl Pts',(54.4753588405202,48.0171963983912,12.));
#109322=CARTESIAN_POINT('Ctrl Pts',(54.4868858913961,48.039547734729,0.));
#109323=CARTESIAN_POINT('Ctrl Pts',(54.4868858913961,48.039547734729,12.));
#109324=CARTESIAN_POINT('Ctrl Pts',(54.4984098712883,48.0619454292321,0.));
#109325=CARTESIAN_POINT('Ctrl Pts',(54.4984098712883,48.0619454292321,12.));
#109326=CARTESIAN_POINT('Ctrl Pts',(54.5099306824788,48.0843894126807,0.));
#109327=CARTESIAN_POINT('Ctrl Pts',(54.5099306824788,48.0843894126807,12.));
#109328=CARTESIAN_POINT('Ctrl Pts',(54.5214482276679,48.1068796160406,0.));
#109329=CARTESIAN_POINT('Ctrl Pts',(54.5214482276679,48.1068796160406,12.));
#109330=CARTESIAN_POINT('Ctrl Pts',(54.5329624099719,48.1294159704571,0.));
#109331=CARTESIAN_POINT('Ctrl Pts',(54.5329624099719,48.1294159704571,12.));
#109332=CARTESIAN_POINT('Ctrl Pts',(54.5444731329196,48.1519984072617,0.));
#109333=CARTESIAN_POINT('Ctrl Pts',(54.5444731329196,48.1519984072617,12.));
#109334=CARTESIAN_POINT('Ctrl Pts',(54.5559803004487,48.1746268579732,0.));
#109335=CARTESIAN_POINT('Ctrl Pts',(54.5559803004487,48.1746268579732,12.));
#109336=CARTESIAN_POINT('Ctrl Pts',(54.5674838169041,48.1973012542966,0.));
#109337=CARTESIAN_POINT('Ctrl Pts',(54.5674838169041,48.1973012542966,12.));
#109338=CARTESIAN_POINT('Ctrl Pts',(54.5789835870348,48.2200215281178,0.));
#109339=CARTESIAN_POINT('Ctrl Pts',(54.5789835870348,48.2200215281178,12.));
#109340=CARTESIAN_POINT('Ctrl Pts',(54.5904795159936,48.2427876114956,0.));
#109341=CARTESIAN_POINT('Ctrl Pts',(54.5904795159936,48.2427876114956,12.));
#109342=CARTESIAN_POINT('Ctrl Pts',(54.6019715093319,48.2655994366672,0.));
#109343=CARTESIAN_POINT('Ctrl Pts',(54.6019715093319,48.2655994366672,12.));
#109344=CARTESIAN_POINT('Ctrl Pts',(54.6134594729964,48.288456936051,0.));
#109345=CARTESIAN_POINT('Ctrl Pts',(54.6134594729964,48.288456936051,12.));
#109346=CARTESIAN_POINT('Ctrl Pts',(54.6249433133262,48.3113600422443,0.));
#109347=CARTESIAN_POINT('Ctrl Pts',(54.6249433133262,48.3113600422443,12.));
#109348=CARTESIAN_POINT('Ctrl Pts',(54.636422937049,48.3343086880192,0.));
#109349=CARTESIAN_POINT('Ctrl Pts',(54.636422937049,48.3343086880192,12.));
#109350=CARTESIAN_POINT('Ctrl Pts',(54.647898251279,48.3573028063122,0.));
#109351=CARTESIAN_POINT('Ctrl Pts',(54.647898251279,48.3573028063122,12.));
#109352=CARTESIAN_POINT('Ctrl Pts',(54.6593691635143,48.3803423302294,0.));
#109353=CARTESIAN_POINT('Ctrl Pts',(54.6593691635143,48.3803423302294,12.));
#109354=CARTESIAN_POINT('Ctrl Pts',(54.6708355816359,48.4034271930516,0.));
#109355=CARTESIAN_POINT('Ctrl Pts',(54.6708355816359,48.4034271930516,12.));
#109356=CARTESIAN_POINT('Ctrl Pts',(54.6822974139065,48.4265573282342,0.));
#109357=CARTESIAN_POINT('Ctrl Pts',(54.6822974139065,48.4265573282342,12.));
#109358=CARTESIAN_POINT('Ctrl Pts',(54.6937545689694,48.4497326694051,0.));
#109359=CARTESIAN_POINT('Ctrl Pts',(54.6937545689694,48.4497326694051,12.));
#109360=CARTESIAN_POINT('Ctrl Pts',(54.7052069558493,48.4729531503565,0.));
#109361=CARTESIAN_POINT('Ctrl Pts',(54.7052069558493,48.4729531503565,12.));
#109362=CARTESIAN_POINT('Ctrl Pts',(54.7166544839475,48.4962187050452,0.));
#109363=CARTESIAN_POINT('Ctrl Pts',(54.7166544839475,48.4962187050452,12.));
#109364=CARTESIAN_POINT('Ctrl Pts',(54.7280970630346,48.5195292675955,0.));
#109365=CARTESIAN_POINT('Ctrl Pts',(54.7280970630346,48.5195292675955,12.));
#109366=CARTESIAN_POINT('Ctrl Pts',(54.7395346032451,48.5428847722975,0.));
#109367=CARTESIAN_POINT('Ctrl Pts',(54.7395346032451,48.5428847722975,12.));
#109368=CARTESIAN_POINT('Ctrl Pts',(54.7509670150716,48.5662851536027,0.));
#109369=CARTESIAN_POINT('Ctrl Pts',(54.7509670150716,48.5662851536027,12.));
#109370=CARTESIAN_POINT('Ctrl Pts',(54.7623942093591,48.5897303461131,0.));
#109371=CARTESIAN_POINT('Ctrl Pts',(54.7623942093591,48.5897303461131,12.));
#109372=CARTESIAN_POINT('Ctrl Pts',(54.773816097304,48.6132202845792,0.));
#109373=CARTESIAN_POINT('Ctrl Pts',(54.773816097304,48.6132202845792,12.));
#109374=CARTESIAN_POINT('Ctrl Pts',(54.7852325904591,48.6367549039121,0.));
#109375=CARTESIAN_POINT('Ctrl Pts',(54.7852325904591,48.6367549039121,12.));
#109376=CARTESIAN_POINT('Ctrl Pts',(54.7966436007395,48.6603341391891,0.));
#109377=CARTESIAN_POINT('Ctrl Pts',(54.7966436007395,48.6603341391891,12.));
#109378=CARTESIAN_POINT('Ctrl Pts',(54.8080490404274,48.6839579256565,0.));
#109379=CARTESIAN_POINT('Ctrl Pts',(54.8080490404274,48.6839579256565,12.));
#109380=CARTESIAN_POINT('Ctrl Pts',(54.8194488221803,48.7076261987284,0.));
#109381=CARTESIAN_POINT('Ctrl Pts',(54.8194488221803,48.7076261987284,12.));
#109382=CARTESIAN_POINT('Ctrl Pts',(54.8308428590334,48.7313388939834,0.));
#109383=CARTESIAN_POINT('Ctrl Pts',(54.8308428590334,48.7313388939834,12.));
#109384=CARTESIAN_POINT('Ctrl Pts',(54.8422310643752,48.755095947159,0.));
#109385=CARTESIAN_POINT('Ctrl Pts',(54.8422310643752,48.755095947159,12.));
#109386=CARTESIAN_POINT('Ctrl Pts',(54.8536133519285,48.7788972941431,0.));
#109387=CARTESIAN_POINT('Ctrl Pts',(54.8536133519285,48.7788972941431,12.));
#109388=CARTESIAN_POINT('Ctrl Pts',(54.8649896357284,48.8027428709613,0.));
#109389=CARTESIAN_POINT('Ctrl Pts',(54.8649896357284,48.8027428709613,12.));
#109390=CARTESIAN_POINT('Ctrl Pts',(54.8763598301045,48.8266326137629,0.));
#109391=CARTESIAN_POINT('Ctrl Pts',(54.8763598301045,48.8266326137629,12.));
#109392=CARTESIAN_POINT('Ctrl Pts',(54.8877238496577,48.8505664587985,0.));
#109393=CARTESIAN_POINT('Ctrl Pts',(54.8877238496577,48.8505664587985,12.));
#109394=CARTESIAN_POINT('Ctrl Pts',(54.8990816092964,48.8745443424488,0.));
#109395=CARTESIAN_POINT('Ctrl Pts',(54.8990816092964,48.8745443424488,12.));
#109396=CARTESIAN_POINT('Ctrl Pts',(54.910433024275,48.8985662012535,0.));
#109397=CARTESIAN_POINT('Ctrl Pts',(54.910433024275,48.8985662012535,12.));
#109398=CARTESIAN_POINT('Ctrl Pts',(54.9217780102357,48.922631971937,0.));
#109399=CARTESIAN_POINT('Ctrl Pts',(54.9217780102357,48.922631971937,12.));
#109400=CARTESIAN_POINT('Ctrl Pts',(54.933116483242,48.9467415914266,0.));
#109401=CARTESIAN_POINT('Ctrl Pts',(54.933116483242,48.9467415914266,12.));
#109402=CARTESIAN_POINT('Ctrl Pts',(54.9444483598372,48.9708949968789,0.));
#109403=CARTESIAN_POINT('Ctrl Pts',(54.9444483598372,48.9708949968789,12.));
#109404=CARTESIAN_POINT('Ctrl Pts',(54.9557735569936,48.995092125652,0.));
#109405=CARTESIAN_POINT('Ctrl Pts',(54.9557735569936,48.995092125652,12.));
#109406=CARTESIAN_POINT('Ctrl Pts',(54.9670919920024,49.0193329152475,0.));
#109407=CARTESIAN_POINT('Ctrl Pts',(54.9670919920024,49.0193329152475,12.));
#109408=CARTESIAN_POINT('Ctrl Pts',(54.9784035823764,49.0436173032527,0.));
#109409=CARTESIAN_POINT('Ctrl Pts',(54.9784035823764,49.0436173032527,12.));
#109410=CARTESIAN_POINT('Ctrl Pts',(54.9897082457606,49.0679452272871,0.));
#109411=CARTESIAN_POINT('Ctrl Pts',(54.9897082457606,49.0679452272871,12.));
#109412=CARTESIAN_POINT('Ctrl Pts',(55.0010058998111,49.0923166249222,0.));
#109413=CARTESIAN_POINT('Ctrl Pts',(55.0010058998111,49.0923166249222,12.));
#109414=CARTESIAN_POINT('Ctrl Pts',(55.0122964621868,49.1167314336737,0.));
#109415=CARTESIAN_POINT('Ctrl Pts',(55.0122964621868,49.1167314336737,12.));
#109416=CARTESIAN_POINT('Ctrl Pts',(55.0235798508056,49.1411895911646,0.));
#109417=CARTESIAN_POINT('Ctrl Pts',(55.0235798508056,49.1411895911646,12.));
#109418=CARTESIAN_POINT('Ctrl Pts',(55.0348559840462,49.1656910352484,0.));
#109419=CARTESIAN_POINT('Ctrl Pts',(55.0348559840462,49.1656910352484,12.));
#109420=CARTESIAN_POINT('Ctrl Pts',(55.0461247809745,49.1902357041462,0.));
#109421=CARTESIAN_POINT('Ctrl Pts',(55.0461247809745,49.1902357041462,12.));
#109422=CARTESIAN_POINT('Ctrl Pts',(55.0573861615569,49.2148235365694,0.));
#109423=CARTESIAN_POINT('Ctrl Pts',(55.0573861615569,49.2148235365694,12.));
#109424=CARTESIAN_POINT('Ctrl Pts',(55.0686400468911,49.2394544718513,0.));
#109425=CARTESIAN_POINT('Ctrl Pts',(55.0686400468911,49.2394544718513,12.));
#109426=CARTESIAN_POINT('Ctrl Pts',(55.0798863586986,49.2641284496496,0.));
#109427=CARTESIAN_POINT('Ctrl Pts',(55.0798863586986,49.2641284496496,12.));
#109428=CARTESIAN_POINT('Ctrl Pts',(55.0911250188282,49.2888454096544,0.));
#109429=CARTESIAN_POINT('Ctrl Pts',(55.0911250188282,49.2888454096544,12.));
#109430=CARTESIAN_POINT('Ctrl Pts',(55.1023559487133,49.3136052912614,0.));
#109431=CARTESIAN_POINT('Ctrl Pts',(55.1023559487133,49.3136052912614,12.));
#109432=CARTESIAN_POINT('Ctrl Pts',(55.1135790689475,49.3384080333166,0.));
#109433=CARTESIAN_POINT('Ctrl Pts',(55.1135790689475,49.3384080333166,12.));
#109434=CARTESIAN_POINT('Ctrl Pts',(55.1247942985649,49.3632535736744,0.));
#109435=CARTESIAN_POINT('Ctrl Pts',(55.1247942985649,49.3632535736744,12.));
#109436=CARTESIAN_POINT('Ctrl Pts',(55.1360015556262,49.3881418495529,0.));
#109437=CARTESIAN_POINT('Ctrl Pts',(55.1360015556262,49.3881418495529,12.));
#109438=CARTESIAN_POINT('Ctrl Pts',(55.1472007585224,49.413072798324,0.));
#109439=CARTESIAN_POINT('Ctrl Pts',(55.1472007585224,49.413072798324,12.));
#109440=CARTESIAN_POINT('Ctrl Pts',(55.158391827114,49.4380463581989,0.));
#109441=CARTESIAN_POINT('Ctrl Pts',(55.158391827114,49.4380463581989,12.));
#109442=CARTESIAN_POINT('Ctrl Pts',(55.1695746838168,49.4630624688787,0.));
#109443=CARTESIAN_POINT('Ctrl Pts',(55.1695746838168,49.4630624688787,12.));
#109444=CARTESIAN_POINT('Ctrl Pts',(55.1807492550073,49.4881210723921,0.));
#109445=CARTESIAN_POINT('Ctrl Pts',(55.1807492550073,49.4881210723921,12.));
#109446=CARTESIAN_POINT('Ctrl Pts',(55.1919154713569,49.5132221132916,0.));
#109447=CARTESIAN_POINT('Ctrl Pts',(55.1919154713569,49.5132221132916,12.));
#109448=CARTESIAN_POINT('Ctrl Pts',(55.2030732647222,49.5383655367987,0.));
#109449=CARTESIAN_POINT('Ctrl Pts',(55.2030732647222,49.5383655367987,12.));
#109450=CARTESIAN_POINT('Ctrl Pts',(55.2142225656943,49.5635512873368,0.));
#109451=CARTESIAN_POINT('Ctrl Pts',(55.2142225656943,49.5635512873368,12.));
#109452=CARTESIAN_POINT('Ctrl Pts',(55.225363300765,49.5887793068337,0.));
#109453=CARTESIAN_POINT('Ctrl Pts',(55.225363300765,49.5887793068337,12.));
#109454=CARTESIAN_POINT('Ctrl Pts',(55.2364953899423,49.6140495332865,0.));
#109455=CARTESIAN_POINT('Ctrl Pts',(55.2364953899423,49.6140495332865,12.));
#109456=CARTESIAN_POINT('Ctrl Pts',(55.2476187434204,49.6393618987614,0.));
#109457=CARTESIAN_POINT('Ctrl Pts',(55.2476187434204,49.6393618987614,12.));
#109458=CARTESIAN_POINT('Ctrl Pts',(55.2587332663982,49.6647163322457,0.));
#109459=CARTESIAN_POINT('Ctrl Pts',(55.2587332663982,49.6647163322457,12.));
#109460=CARTESIAN_POINT('Ctrl Pts',(55.2698388650215,49.690112763181,0.));
#109461=CARTESIAN_POINT('Ctrl Pts',(55.2698388650215,49.690112763181,12.));
#109462=CARTESIAN_POINT('Ctrl Pts',(55.2809354521616,49.7155511248629,0.));
#109463=CARTESIAN_POINT('Ctrl Pts',(55.2809354521616,49.7155511248629,12.));
#109464=CARTESIAN_POINT('Ctrl Pts',(55.292022952748,49.7410313576444,0.));
#109465=CARTESIAN_POINT('Ctrl Pts',(55.292022952748,49.7410313576444,12.));
#109466=CARTESIAN_POINT('Ctrl Pts',(55.3031013105578,49.7665534128269,0.));
#109467=CARTESIAN_POINT('Ctrl Pts',(55.3031013105578,49.7665534128269,12.));
#109468=CARTESIAN_POINT('Ctrl Pts',(55.3141704897307,49.7921172540185,0.));
#109469=CARTESIAN_POINT('Ctrl Pts',(55.3141704897307,49.7921172540185,12.));
#109470=CARTESIAN_POINT('Ctrl Pts',(55.3252304694066,49.817722855186,0.));
#109471=CARTESIAN_POINT('Ctrl Pts',(55.3252304694066,49.817722855186,12.));
#109472=CARTESIAN_POINT('Ctrl Pts',(55.3340710859607,49.8382407306675,0.));
#109473=CARTESIAN_POINT('Ctrl Pts',(55.3340710859607,49.8382407306675,12.));
#109474=CARTESIAN_POINT('Ctrl Pts',(55.340697403233,49.8536479176573,0.));
#109475=CARTESIAN_POINT('Ctrl Pts',(55.340697403233,49.8536479176573,12.));
#109476=CARTESIAN_POINT('Ctrl Pts',(55.3451131058727,49.8639277221471,0.));
#109477=CARTESIAN_POINT('Ctrl Pts',(55.3451131058727,49.8639277221471,12.));
#109478=CARTESIAN_POINT('Ctrl Pts',(55.3473204966403,49.8690697110161,0.));
#109479=CARTESIAN_POINT('Ctrl Pts',(55.3473204966403,49.8690697110161,12.));
#109480=CARTESIAN_POINT('',(53.0702932034641,45.6458539113724,0.));
#109481=CARTESIAN_POINT('Ctrl Pts',(53.0702932034641,45.6458539113724,0.));
#109482=CARTESIAN_POINT('Ctrl Pts',(53.0724894921849,45.6490568514089,0.));
#109483=CARTESIAN_POINT('Ctrl Pts',(53.0768833804193,45.6554684028145,0.));
#109484=CARTESIAN_POINT('Ctrl Pts',(53.0834781451546,45.6651027439241,0.));
#109485=CARTESIAN_POINT('Ctrl Pts',(53.0922790298409,45.6779825614231,0.));
#109486=CARTESIAN_POINT('Ctrl Pts',(53.1032932328857,45.694139048907,0.));
#109487=CARTESIAN_POINT('Ctrl Pts',(53.114320495492,45.7103522376696,0.));
#109488=CARTESIAN_POINT('Ctrl Pts',(53.1253607414872,45.7266220897003,0.));
#109489=CARTESIAN_POINT('Ctrl Pts',(53.1364138384693,45.7429485300823,0.));
#109490=CARTESIAN_POINT('Ctrl Pts',(53.1474795996053,45.7593314474501,0.));
#109491=CARTESIAN_POINT('Ctrl Pts',(53.1585578076444,45.7757707100618,0.));
#109492=CARTESIAN_POINT('Ctrl Pts',(53.1696482334487,45.7922661780005,0.));
#109493=CARTESIAN_POINT('Ctrl Pts',(53.1807506560933,45.808817716509,0.));
#109494=CARTESIAN_POINT('Ctrl Pts',(53.1918648840541,45.8254252099957,0.));
#109495=CARTESIAN_POINT('Ctrl Pts',(53.2029907483557,45.8420885575349,0.));
#109496=CARTESIAN_POINT('Ctrl Pts',(53.2141280925439,45.8588076662582,0.));
#109497=CARTESIAN_POINT('Ctrl Pts',(53.2252767643662,45.8755824458723,0.));
#109498=CARTESIAN_POINT('Ctrl Pts',(53.2364366054306,45.892412801838,0.));
#109499=CARTESIAN_POINT('Ctrl Pts',(53.2476074460017,45.9092986319377,0.));
#109500=CARTESIAN_POINT('Ctrl Pts',(53.2587891103866,45.9262398298349,0.));
#109501=CARTESIAN_POINT('Ctrl Pts',(53.2699814203105,45.9432362873008,0.));
#109502=CARTESIAN_POINT('Ctrl Pts',(53.2811841987926,45.9602878967698,0.));
#109503=CARTESIAN_POINT('Ctrl Pts',(53.292397274555,45.9773945542384,0.));
#109504=CARTESIAN_POINT('Ctrl Pts',(53.3036204818329,45.9945561591453,0.));
#109505=CARTESIAN_POINT('Ctrl Pts',(53.3148536582635,46.0117726129873,0.));
#109506=CARTESIAN_POINT('Ctrl Pts',(53.326096643428,46.02904381836,0.));
#109507=CARTESIAN_POINT('Ctrl Pts',(53.3373492770671,46.0463696777801,0.));
#109508=CARTESIAN_POINT('Ctrl Pts',(53.3486113975901,46.0637500926982,0.));
#109509=CARTESIAN_POINT('Ctrl Pts',(53.3598828428546,46.0811849640218,0.));
#109510=CARTESIAN_POINT('Ctrl Pts',(53.3711634508437,46.0986741925656,0.));
#109511=CARTESIAN_POINT('Ctrl Pts',(53.3824530603276,46.1162176794884,0.));
#109512=CARTESIAN_POINT('Ctrl Pts',(53.3937515116549,46.1338153268097,0.));
#109513=CARTESIAN_POINT('Ctrl Pts',(53.4050586470436,46.1514670376012,0.));
#109514=CARTESIAN_POINT('Ctrl Pts',(53.4163743101517,46.1691727157134,0.));
#109515=CARTESIAN_POINT('Ctrl Pts',(53.4276983458125,46.1869322656024,0.));
#109516=CARTESIAN_POINT('Ctrl Pts',(53.4390305997274,46.2047455921286,0.));
#109517=CARTESIAN_POINT('Ctrl Pts',(53.4503709181178,46.2226126003202,0.));
#109518=CARTESIAN_POINT('Ctrl Pts',(53.4617191477402,46.2405331953889,0.));
#109519=CARTESIAN_POINT('Ctrl Pts',(53.4730751360371,46.2585072828353,0.));
#109520=CARTESIAN_POINT('Ctrl Pts',(53.4844387312414,46.2765347685198,0.));
#109521=CARTESIAN_POINT('Ctrl Pts',(53.4958097825006,46.2946155587417,0.));
#109522=CARTESIAN_POINT('Ctrl Pts',(53.5071881399911,46.3127495603098,0.));
#109523=CARTESIAN_POINT('Ctrl Pts',(53.5185736548548,46.3309366805093,0.));
#109524=CARTESIAN_POINT('Ctrl Pts',(53.5299661791385,46.3491768270655,0.));
#109525=CARTESIAN_POINT('Ctrl Pts',(53.5413655657327,46.3674699081046,0.));
#109526=CARTESIAN_POINT('Ctrl Pts',(53.5527716683048,46.3858158321059,0.));
#109527=CARTESIAN_POINT('Ctrl Pts',(53.5641843412559,46.4042145078701,0.));
#109528=CARTESIAN_POINT('Ctrl Pts',(53.5756034397481,46.4226658445474,0.));
#109529=CARTESIAN_POINT('Ctrl Pts',(53.5870288197166,46.4411697516478,0.));
#109530=CARTESIAN_POINT('Ctrl Pts',(53.5984603378855,46.459726139052,0.));
#109531=CARTESIAN_POINT('Ctrl Pts',(53.6098978517859,46.4783349170173,0.));
#109532=CARTESIAN_POINT('Ctrl Pts',(53.6213412197533,46.496995996177,0.));
#109533=CARTESIAN_POINT('Ctrl Pts',(53.6327903009094,46.5157092875373,0.));
#109534=CARTESIAN_POINT('Ctrl Pts',(53.6442449551455,46.5344747024676,0.));
#109535=CARTESIAN_POINT('Ctrl Pts',(53.6557050431071,46.5532921526901,0.));
#109536=CARTESIAN_POINT('Ctrl Pts',(53.6671704261737,46.5721615502591,0.));
#109537=CARTESIAN_POINT('Ctrl Pts',(53.678640966456,46.5910828075653,0.));
#109538=CARTESIAN_POINT('Ctrl Pts',(53.6901165267941,46.6100558373402,0.));
#109539=CARTESIAN_POINT('Ctrl Pts',(53.701596970754,46.6290805526559,0.));
#109540=CARTESIAN_POINT('Ctrl Pts',(53.7130821626263,46.6481568669216,0.));
#109541=CARTESIAN_POINT('Ctrl Pts',(53.7245719674222,46.6672846938752,0.));
#109542=CARTESIAN_POINT('Ctrl Pts',(53.7360662508677,46.6864639475863,0.));
#109543=CARTESIAN_POINT('Ctrl Pts',(53.7475648793948,46.7056945424559,0.));
#109544=CARTESIAN_POINT('Ctrl Pts',(53.7590677201344,46.724976393213,0.));
#109545=CARTESIAN_POINT('Ctrl Pts',(53.770574640907,46.7443094149041,0.));
#109546=CARTESIAN_POINT('Ctrl Pts',(53.782085510217,46.7636935228851,0.));
#109547=CARTESIAN_POINT('Ctrl Pts',(53.7936001972468,46.7831286328268,0.));
#109548=CARTESIAN_POINT('Ctrl Pts',(53.8051185718525,46.8026146607144,0.));
#109549=CARTESIAN_POINT('Ctrl Pts',(53.8166405045582,46.8221515228459,0.));
#109550=CARTESIAN_POINT('Ctrl Pts',(53.8281658665517,46.8417391358231,0.));
#109551=CARTESIAN_POINT('Ctrl Pts',(53.8396945296777,46.8613774165452,0.));
#109552=CARTESIAN_POINT('Ctrl Pts',(53.851226366434,46.8810662822147,0.));
#109553=CARTESIAN_POINT('Ctrl Pts',(53.8627612499648,46.900805650336,0.));
#109554=CARTESIAN_POINT('Ctrl Pts',(53.8742990540557,46.9205954387128,0.));
#109555=CARTESIAN_POINT('Ctrl Pts',(53.8858396531277,46.9404355654381,0.));
#109556=CARTESIAN_POINT('Ctrl Pts',(53.8973829222317,46.9603259488894,0.));
#109557=CARTESIAN_POINT('Ctrl Pts',(53.9089287370436,46.9802665077342,0.));
#109558=CARTESIAN_POINT('Ctrl Pts',(53.9204769738584,47.0002571609286,0.));
#109559=CARTESIAN_POINT('Ctrl Pts',(53.9320275095864,47.0202978277148,0.));
#109560=CARTESIAN_POINT('Ctrl Pts',(53.9435802217468,47.04038842761,0.));
#109561=CARTESIAN_POINT('Ctrl Pts',(53.9551349884637,47.0605288804042,0.));
#109562=CARTESIAN_POINT('Ctrl Pts',(53.9666916884624,47.0807191061674,0.));
#109563=CARTESIAN_POINT('Ctrl Pts',(53.9782502010642,47.1009590252466,0.));
#109564=CARTESIAN_POINT('Ctrl Pts',(53.9898104061809,47.1212485582632,0.));
#109565=CARTESIAN_POINT('Ctrl Pts',(54.0013721843094,47.1415876261012,0.));
#109566=CARTESIAN_POINT('Ctrl Pts',(54.0129354165269,47.161976149906,0.));
#109567=CARTESIAN_POINT('Ctrl Pts',(54.0244999844872,47.1824140510906,0.));
#109568=CARTESIAN_POINT('Ctrl Pts',(54.0360657704156,47.2029012513334,0.));
#109569=CARTESIAN_POINT('Ctrl Pts',(54.047632657105,47.2234376725752,0.));
#109570=CARTESIAN_POINT('Ctrl Pts',(54.0592005279108,47.2440232370085,0.));
#109571=CARTESIAN_POINT('Ctrl Pts',(54.0707692667461,47.2646578670767,0.));
#109572=CARTESIAN_POINT('Ctrl Pts',(54.082338758079,47.2853414854805,0.));
#109573=CARTESIAN_POINT('Ctrl Pts',(54.0939088869271,47.3060740151754,0.));
#109574=CARTESIAN_POINT('Ctrl Pts',(54.1054795388538,47.326855379369,0.));
#109575=CARTESIAN_POINT('Ctrl Pts',(54.1170505999637,47.3476855015095,0.));
#109576=CARTESIAN_POINT('Ctrl Pts',(54.1286219568981,47.3685643052867,0.));
#109577=CARTESIAN_POINT('Ctrl Pts',(54.1401934968306,47.3894917146361,0.));
#109578=CARTESIAN_POINT('Ctrl Pts',(54.1517651074638,47.4104676537381,0.));
#109579=CARTESIAN_POINT('Ctrl Pts',(54.163336677024,47.4314920470142,0.));
#109580=CARTESIAN_POINT('Ctrl Pts',(54.1749080942593,47.4525648191173,0.));
#109581=CARTESIAN_POINT('Ctrl Pts',(54.1864792484343,47.473685894932,0.));
#109582=CARTESIAN_POINT('Ctrl Pts',(54.1980500293267,47.4948551995799,0.));
#109583=CARTESIAN_POINT('Ctrl Pts',(54.2096203272228,47.5160726584172,0.));
#109584=CARTESIAN_POINT('Ctrl Pts',(54.2211900329141,47.5373381970328,0.));
#109585=CARTESIAN_POINT('Ctrl Pts',(54.232759037693,47.5586517412368,0.));
#109586=CARTESIAN_POINT('Ctrl Pts',(54.2443272333498,47.5800132170614,0.));
#109587=CARTESIAN_POINT('Ctrl Pts',(54.2558945121684,47.6014225507664,0.));
#109588=CARTESIAN_POINT('Ctrl Pts',(54.2674607669228,47.6228796688376,0.));
#109589=CARTESIAN_POINT('Ctrl Pts',(54.2790258908736,47.6443844979846,0.));
#109590=CARTESIAN_POINT('Ctrl Pts',(54.2905897777647,47.6659369651299,0.));
#109591=CARTESIAN_POINT('Ctrl Pts',(54.3021523218188,47.6875369974086,0.));
#109592=CARTESIAN_POINT('Ctrl Pts',(54.3137134177345,47.7091845221748,0.));
#109593=CARTESIAN_POINT('Ctrl Pts',(54.3252729606824,47.7308794669994,0.));
#109594=CARTESIAN_POINT('Ctrl Pts',(54.3368308463023,47.7526217596694,0.));
#109595=CARTESIAN_POINT('Ctrl Pts',(54.3483869706998,47.7744113281768,0.));
#109596=CARTESIAN_POINT('Ctrl Pts',(54.3599412304431,47.7962481007179,0.));
#109597=CARTESIAN_POINT('Ctrl Pts',(54.3714935225585,47.8181320056988,0.));
#109598=CARTESIAN_POINT('Ctrl Pts',(54.3830437445275,47.8400629717352,0.));
#109599=CARTESIAN_POINT('Ctrl Pts',(54.3945917942835,47.8620409276495,0.));
#109600=CARTESIAN_POINT('Ctrl Pts',(54.4061375702088,47.8840658024626,0.));
#109601=CARTESIAN_POINT('Ctrl Pts',(54.4176809711324,47.9061375253909,0.));
#109602=CARTESIAN_POINT('Ctrl Pts',(54.4292218963253,47.9282560258528,0.));
#109603=CARTESIAN_POINT('Ctrl Pts',(54.4407602454974,47.9504212334681,0.));
#109604=CARTESIAN_POINT('Ctrl Pts',(54.4522959187952,47.972633078057,0.));
#109605=CARTESIAN_POINT('Ctrl Pts',(54.4638288167991,47.9948914896316,0.));
#109606=CARTESIAN_POINT('Ctrl Pts',(54.4753588405202,48.0171963983912,0.));
#109607=CARTESIAN_POINT('Ctrl Pts',(54.4868858913961,48.039547734729,0.));
#109608=CARTESIAN_POINT('Ctrl Pts',(54.4984098712883,48.0619454292321,0.));
#109609=CARTESIAN_POINT('Ctrl Pts',(54.5099306824788,48.0843894126807,0.));
#109610=CARTESIAN_POINT('Ctrl Pts',(54.5214482276679,48.1068796160406,0.));
#109611=CARTESIAN_POINT('Ctrl Pts',(54.5329624099719,48.1294159704571,0.));
#109612=CARTESIAN_POINT('Ctrl Pts',(54.5444731329196,48.1519984072617,0.));
#109613=CARTESIAN_POINT('Ctrl Pts',(54.5559803004487,48.1746268579732,0.));
#109614=CARTESIAN_POINT('Ctrl Pts',(54.5674838169041,48.1973012542966,0.));
#109615=CARTESIAN_POINT('Ctrl Pts',(54.5789835870348,48.2200215281178,0.));
#109616=CARTESIAN_POINT('Ctrl Pts',(54.5904795159936,48.2427876114956,0.));
#109617=CARTESIAN_POINT('Ctrl Pts',(54.6019715093319,48.2655994366672,0.));
#109618=CARTESIAN_POINT('Ctrl Pts',(54.6134594729964,48.288456936051,0.));
#109619=CARTESIAN_POINT('Ctrl Pts',(54.6249433133262,48.3113600422443,0.));
#109620=CARTESIAN_POINT('Ctrl Pts',(54.636422937049,48.3343086880192,0.));
#109621=CARTESIAN_POINT('Ctrl Pts',(54.647898251279,48.3573028063122,0.));
#109622=CARTESIAN_POINT('Ctrl Pts',(54.6593691635143,48.3803423302294,0.));
#109623=CARTESIAN_POINT('Ctrl Pts',(54.6708355816359,48.4034271930516,0.));
#109624=CARTESIAN_POINT('Ctrl Pts',(54.6822974139065,48.4265573282342,0.));
#109625=CARTESIAN_POINT('Ctrl Pts',(54.6937545689694,48.4497326694051,0.));
#109626=CARTESIAN_POINT('Ctrl Pts',(54.7052069558493,48.4729531503565,0.));
#109627=CARTESIAN_POINT('Ctrl Pts',(54.7166544839475,48.4962187050452,0.));
#109628=CARTESIAN_POINT('Ctrl Pts',(54.7280970630346,48.5195292675955,0.));
#109629=CARTESIAN_POINT('Ctrl Pts',(54.7395346032451,48.5428847722975,0.));
#109630=CARTESIAN_POINT('Ctrl Pts',(54.7509670150716,48.5662851536027,0.));
#109631=CARTESIAN_POINT('Ctrl Pts',(54.7623942093591,48.5897303461131,0.));
#109632=CARTESIAN_POINT('Ctrl Pts',(54.773816097304,48.6132202845792,0.));
#109633=CARTESIAN_POINT('Ctrl Pts',(54.7852325904591,48.6367549039121,0.));
#109634=CARTESIAN_POINT('Ctrl Pts',(54.7966436007395,48.6603341391891,0.));
#109635=CARTESIAN_POINT('Ctrl Pts',(54.8080490404274,48.6839579256565,0.));
#109636=CARTESIAN_POINT('Ctrl Pts',(54.8194488221803,48.7076261987284,0.));
#109637=CARTESIAN_POINT('Ctrl Pts',(54.8308428590334,48.7313388939834,0.));
#109638=CARTESIAN_POINT('Ctrl Pts',(54.8422310643752,48.755095947159,0.));
#109639=CARTESIAN_POINT('Ctrl Pts',(54.8536133519285,48.7788972941431,0.));
#109640=CARTESIAN_POINT('Ctrl Pts',(54.8649896357284,48.8027428709613,0.));
#109641=CARTESIAN_POINT('Ctrl Pts',(54.8763598301045,48.8266326137629,0.));
#109642=CARTESIAN_POINT('Ctrl Pts',(54.8877238496577,48.8505664587985,0.));
#109643=CARTESIAN_POINT('Ctrl Pts',(54.8990816092964,48.8745443424488,0.));
#109644=CARTESIAN_POINT('Ctrl Pts',(54.910433024275,48.8985662012535,0.));
#109645=CARTESIAN_POINT('Ctrl Pts',(54.9217780102357,48.922631971937,0.));
#109646=CARTESIAN_POINT('Ctrl Pts',(54.933116483242,48.9467415914266,0.));
#109647=CARTESIAN_POINT('Ctrl Pts',(54.9444483598372,48.9708949968789,0.));
#109648=CARTESIAN_POINT('Ctrl Pts',(54.9557735569936,48.995092125652,0.));
#109649=CARTESIAN_POINT('Ctrl Pts',(54.9670919920024,49.0193329152475,0.));
#109650=CARTESIAN_POINT('Ctrl Pts',(54.9784035823764,49.0436173032527,0.));
#109651=CARTESIAN_POINT('Ctrl Pts',(54.9897082457606,49.0679452272871,0.));
#109652=CARTESIAN_POINT('Ctrl Pts',(55.0010058998111,49.0923166249222,0.));
#109653=CARTESIAN_POINT('Ctrl Pts',(55.0122964621868,49.1167314336737,0.));
#109654=CARTESIAN_POINT('Ctrl Pts',(55.0235798508056,49.1411895911646,0.));
#109655=CARTESIAN_POINT('Ctrl Pts',(55.0348559840462,49.1656910352484,0.));
#109656=CARTESIAN_POINT('Ctrl Pts',(55.0461247809745,49.1902357041462,0.));
#109657=CARTESIAN_POINT('Ctrl Pts',(55.0573861615569,49.2148235365694,0.));
#109658=CARTESIAN_POINT('Ctrl Pts',(55.0686400468911,49.2394544718513,0.));
#109659=CARTESIAN_POINT('Ctrl Pts',(55.0798863586986,49.2641284496496,0.));
#109660=CARTESIAN_POINT('Ctrl Pts',(55.0911250188282,49.2888454096544,0.));
#109661=CARTESIAN_POINT('Ctrl Pts',(55.1023559487133,49.3136052912614,0.));
#109662=CARTESIAN_POINT('Ctrl Pts',(55.1135790689475,49.3384080333166,0.));
#109663=CARTESIAN_POINT('Ctrl Pts',(55.1247942985649,49.3632535736744,0.));
#109664=CARTESIAN_POINT('Ctrl Pts',(55.1360015556262,49.3881418495529,0.));
#109665=CARTESIAN_POINT('Ctrl Pts',(55.1472007585224,49.413072798324,0.));
#109666=CARTESIAN_POINT('Ctrl Pts',(55.158391827114,49.4380463581989,0.));
#109667=CARTESIAN_POINT('Ctrl Pts',(55.1695746838168,49.4630624688787,0.));
#109668=CARTESIAN_POINT('Ctrl Pts',(55.1807492550073,49.4881210723921,0.));
#109669=CARTESIAN_POINT('Ctrl Pts',(55.1919154713569,49.5132221132916,0.));
#109670=CARTESIAN_POINT('Ctrl Pts',(55.2014798623975,49.5347748994607,0.));
#109671=CARTESIAN_POINT('Ctrl Pts',(55.2088081098955,49.5513218524279,0.));
#109672=CARTESIAN_POINT('Ctrl Pts',(55.2139039604569,49.5628442141869,0.));
#109673=CARTESIAN_POINT('Ctrl Pts',(55.2167699151168,49.5693295981608,0.));
#109674=CARTESIAN_POINT('Ctrl Pts',(55.2174072001297,49.5707719660254,0.));
#109675=CARTESIAN_POINT('',(53.0702932034641,45.6458539113724,12.));
#109676=CARTESIAN_POINT('',(53.0702932034641,45.6458539113724,0.));
#109677=CARTESIAN_POINT('Ctrl Pts',(55.2174072001297,49.5707719660254,12.));
#109678=CARTESIAN_POINT('Ctrl Pts',(55.2167699151168,49.5693295981608,12.));
#109679=CARTESIAN_POINT('Ctrl Pts',(55.2139039604569,49.5628442141869,12.));
#109680=CARTESIAN_POINT('Ctrl Pts',(55.2088081098955,49.5513218524279,12.));
#109681=CARTESIAN_POINT('Ctrl Pts',(55.2014798623975,49.5347748994607,12.));
#109682=CARTESIAN_POINT('Ctrl Pts',(55.1919154713569,49.5132221132916,12.));
#109683=CARTESIAN_POINT('Ctrl Pts',(55.1807492550073,49.4881210723921,12.));
#109684=CARTESIAN_POINT('Ctrl Pts',(55.1695746838168,49.4630624688787,12.));
#109685=CARTESIAN_POINT('Ctrl Pts',(55.158391827114,49.4380463581989,12.));
#109686=CARTESIAN_POINT('Ctrl Pts',(55.1472007585224,49.413072798324,12.));
#109687=CARTESIAN_POINT('Ctrl Pts',(55.1360015556262,49.3881418495529,12.));
#109688=CARTESIAN_POINT('Ctrl Pts',(55.1247942985649,49.3632535736744,12.));
#109689=CARTESIAN_POINT('Ctrl Pts',(55.1135790689475,49.3384080333166,12.));
#109690=CARTESIAN_POINT('Ctrl Pts',(55.1023559487133,49.3136052912614,12.));
#109691=CARTESIAN_POINT('Ctrl Pts',(55.0911250188282,49.2888454096544,12.));
#109692=CARTESIAN_POINT('Ctrl Pts',(55.0798863586986,49.2641284496496,12.));
#109693=CARTESIAN_POINT('Ctrl Pts',(55.0686400468911,49.2394544718513,12.));
#109694=CARTESIAN_POINT('Ctrl Pts',(55.0573861615569,49.2148235365694,12.));
#109695=CARTESIAN_POINT('Ctrl Pts',(55.0461247809745,49.1902357041462,12.));
#109696=CARTESIAN_POINT('Ctrl Pts',(55.0348559840462,49.1656910352484,12.));
#109697=CARTESIAN_POINT('Ctrl Pts',(55.0235798508056,49.1411895911646,12.));
#109698=CARTESIAN_POINT('Ctrl Pts',(55.0122964621868,49.1167314336737,12.));
#109699=CARTESIAN_POINT('Ctrl Pts',(55.0010058998111,49.0923166249222,12.));
#109700=CARTESIAN_POINT('Ctrl Pts',(54.9897082457606,49.0679452272871,12.));
#109701=CARTESIAN_POINT('Ctrl Pts',(54.9784035823764,49.0436173032527,12.));
#109702=CARTESIAN_POINT('Ctrl Pts',(54.9670919920024,49.0193329152475,12.));
#109703=CARTESIAN_POINT('Ctrl Pts',(54.9557735569936,48.995092125652,12.));
#109704=CARTESIAN_POINT('Ctrl Pts',(54.9444483598372,48.9708949968789,12.));
#109705=CARTESIAN_POINT('Ctrl Pts',(54.933116483242,48.9467415914266,12.));
#109706=CARTESIAN_POINT('Ctrl Pts',(54.9217780102357,48.922631971937,12.));
#109707=CARTESIAN_POINT('Ctrl Pts',(54.910433024275,48.8985662012535,12.));
#109708=CARTESIAN_POINT('Ctrl Pts',(54.8990816092964,48.8745443424488,12.));
#109709=CARTESIAN_POINT('Ctrl Pts',(54.8877238496577,48.8505664587985,12.));
#109710=CARTESIAN_POINT('Ctrl Pts',(54.8763598301045,48.8266326137629,12.));
#109711=CARTESIAN_POINT('Ctrl Pts',(54.8649896357284,48.8027428709613,12.));
#109712=CARTESIAN_POINT('Ctrl Pts',(54.8536133519285,48.7788972941431,12.));
#109713=CARTESIAN_POINT('Ctrl Pts',(54.8422310643752,48.755095947159,12.));
#109714=CARTESIAN_POINT('Ctrl Pts',(54.8308428590334,48.7313388939834,12.));
#109715=CARTESIAN_POINT('Ctrl Pts',(54.8194488221803,48.7076261987284,12.));
#109716=CARTESIAN_POINT('Ctrl Pts',(54.8080490404274,48.6839579256565,12.));
#109717=CARTESIAN_POINT('Ctrl Pts',(54.7966436007395,48.6603341391891,12.));
#109718=CARTESIAN_POINT('Ctrl Pts',(54.7852325904591,48.6367549039121,12.));
#109719=CARTESIAN_POINT('Ctrl Pts',(54.773816097304,48.6132202845792,12.));
#109720=CARTESIAN_POINT('Ctrl Pts',(54.7623942093591,48.5897303461131,12.));
#109721=CARTESIAN_POINT('Ctrl Pts',(54.7509670150716,48.5662851536027,12.));
#109722=CARTESIAN_POINT('Ctrl Pts',(54.7395346032451,48.5428847722975,12.));
#109723=CARTESIAN_POINT('Ctrl Pts',(54.7280970630346,48.5195292675955,12.));
#109724=CARTESIAN_POINT('Ctrl Pts',(54.7166544839475,48.4962187050452,12.));
#109725=CARTESIAN_POINT('Ctrl Pts',(54.7052069558493,48.4729531503565,12.));
#109726=CARTESIAN_POINT('Ctrl Pts',(54.6937545689694,48.4497326694051,12.));
#109727=CARTESIAN_POINT('Ctrl Pts',(54.6822974139065,48.4265573282342,12.));
#109728=CARTESIAN_POINT('Ctrl Pts',(54.6708355816359,48.4034271930516,12.));
#109729=CARTESIAN_POINT('Ctrl Pts',(54.6593691635143,48.3803423302294,12.));
#109730=CARTESIAN_POINT('Ctrl Pts',(54.647898251279,48.3573028063122,12.));
#109731=CARTESIAN_POINT('Ctrl Pts',(54.636422937049,48.3343086880192,12.));
#109732=CARTESIAN_POINT('Ctrl Pts',(54.6249433133262,48.3113600422443,12.));
#109733=CARTESIAN_POINT('Ctrl Pts',(54.6134594729964,48.288456936051,12.));
#109734=CARTESIAN_POINT('Ctrl Pts',(54.6019715093319,48.2655994366672,12.));
#109735=CARTESIAN_POINT('Ctrl Pts',(54.5904795159936,48.2427876114956,12.));
#109736=CARTESIAN_POINT('Ctrl Pts',(54.5789835870348,48.2200215281178,12.));
#109737=CARTESIAN_POINT('Ctrl Pts',(54.5674838169041,48.1973012542966,12.));
#109738=CARTESIAN_POINT('Ctrl Pts',(54.5559803004487,48.1746268579732,12.));
#109739=CARTESIAN_POINT('Ctrl Pts',(54.5444731329196,48.1519984072617,12.));
#109740=CARTESIAN_POINT('Ctrl Pts',(54.5329624099719,48.1294159704571,12.));
#109741=CARTESIAN_POINT('Ctrl Pts',(54.5214482276679,48.1068796160406,12.));
#109742=CARTESIAN_POINT('Ctrl Pts',(54.5099306824788,48.0843894126807,12.));
#109743=CARTESIAN_POINT('Ctrl Pts',(54.4984098712883,48.0619454292321,12.));
#109744=CARTESIAN_POINT('Ctrl Pts',(54.4868858913961,48.039547734729,12.));
#109745=CARTESIAN_POINT('Ctrl Pts',(54.4753588405202,48.0171963983912,12.));
#109746=CARTESIAN_POINT('Ctrl Pts',(54.4638288167991,47.9948914896316,12.));
#109747=CARTESIAN_POINT('Ctrl Pts',(54.4522959187952,47.972633078057,12.));
#109748=CARTESIAN_POINT('Ctrl Pts',(54.4407602454974,47.9504212334681,12.));
#109749=CARTESIAN_POINT('Ctrl Pts',(54.4292218963253,47.9282560258528,12.));
#109750=CARTESIAN_POINT('Ctrl Pts',(54.4176809711324,47.9061375253909,12.));
#109751=CARTESIAN_POINT('Ctrl Pts',(54.4061375702088,47.8840658024626,12.));
#109752=CARTESIAN_POINT('Ctrl Pts',(54.3945917942835,47.8620409276495,12.));
#109753=CARTESIAN_POINT('Ctrl Pts',(54.3830437445275,47.8400629717352,12.));
#109754=CARTESIAN_POINT('Ctrl Pts',(54.3714935225585,47.8181320056988,12.));
#109755=CARTESIAN_POINT('Ctrl Pts',(54.3599412304431,47.7962481007179,12.));
#109756=CARTESIAN_POINT('Ctrl Pts',(54.3483869706998,47.7744113281768,12.));
#109757=CARTESIAN_POINT('Ctrl Pts',(54.3368308463023,47.7526217596694,12.));
#109758=CARTESIAN_POINT('Ctrl Pts',(54.3252729606824,47.7308794669994,12.));
#109759=CARTESIAN_POINT('Ctrl Pts',(54.3137134177345,47.7091845221748,12.));
#109760=CARTESIAN_POINT('Ctrl Pts',(54.3021523218188,47.6875369974086,12.));
#109761=CARTESIAN_POINT('Ctrl Pts',(54.2905897777647,47.6659369651299,12.));
#109762=CARTESIAN_POINT('Ctrl Pts',(54.2790258908736,47.6443844979846,12.));
#109763=CARTESIAN_POINT('Ctrl Pts',(54.2674607669228,47.6228796688376,12.));
#109764=CARTESIAN_POINT('Ctrl Pts',(54.2558945121684,47.6014225507664,12.));
#109765=CARTESIAN_POINT('Ctrl Pts',(54.2443272333498,47.5800132170614,12.));
#109766=CARTESIAN_POINT('Ctrl Pts',(54.232759037693,47.5586517412368,12.));
#109767=CARTESIAN_POINT('Ctrl Pts',(54.2211900329141,47.5373381970328,12.));
#109768=CARTESIAN_POINT('Ctrl Pts',(54.2096203272228,47.5160726584172,12.));
#109769=CARTESIAN_POINT('Ctrl Pts',(54.1980500293267,47.4948551995799,12.));
#109770=CARTESIAN_POINT('Ctrl Pts',(54.1864792484343,47.473685894932,12.));
#109771=CARTESIAN_POINT('Ctrl Pts',(54.1749080942593,47.4525648191173,12.));
#109772=CARTESIAN_POINT('Ctrl Pts',(54.163336677024,47.4314920470142,12.));
#109773=CARTESIAN_POINT('Ctrl Pts',(54.1517651074638,47.4104676537381,12.));
#109774=CARTESIAN_POINT('Ctrl Pts',(54.1401934968306,47.3894917146361,12.));
#109775=CARTESIAN_POINT('Ctrl Pts',(54.1286219568981,47.3685643052867,12.));
#109776=CARTESIAN_POINT('Ctrl Pts',(54.1170505999637,47.3476855015095,12.));
#109777=CARTESIAN_POINT('Ctrl Pts',(54.1054795388538,47.326855379369,12.));
#109778=CARTESIAN_POINT('Ctrl Pts',(54.0939088869271,47.3060740151754,12.));
#109779=CARTESIAN_POINT('Ctrl Pts',(54.082338758079,47.2853414854805,12.));
#109780=CARTESIAN_POINT('Ctrl Pts',(54.0707692667461,47.2646578670767,12.));
#109781=CARTESIAN_POINT('Ctrl Pts',(54.0592005279108,47.2440232370085,12.));
#109782=CARTESIAN_POINT('Ctrl Pts',(54.047632657105,47.2234376725752,12.));
#109783=CARTESIAN_POINT('Ctrl Pts',(54.0360657704156,47.2029012513334,12.));
#109784=CARTESIAN_POINT('Ctrl Pts',(54.0244999844872,47.1824140510906,12.));
#109785=CARTESIAN_POINT('Ctrl Pts',(54.0129354165269,47.161976149906,12.));
#109786=CARTESIAN_POINT('Ctrl Pts',(54.0013721843094,47.1415876261012,12.));
#109787=CARTESIAN_POINT('Ctrl Pts',(53.9898104061809,47.1212485582632,12.));
#109788=CARTESIAN_POINT('Ctrl Pts',(53.9782502010642,47.1009590252466,12.));
#109789=CARTESIAN_POINT('Ctrl Pts',(53.9666916884624,47.0807191061674,12.));
#109790=CARTESIAN_POINT('Ctrl Pts',(53.9551349884637,47.0605288804042,12.));
#109791=CARTESIAN_POINT('Ctrl Pts',(53.9435802217468,47.04038842761,12.));
#109792=CARTESIAN_POINT('Ctrl Pts',(53.9320275095864,47.0202978277148,12.));
#109793=CARTESIAN_POINT('Ctrl Pts',(53.9204769738584,47.0002571609286,12.));
#109794=CARTESIAN_POINT('Ctrl Pts',(53.9089287370436,46.9802665077342,12.));
#109795=CARTESIAN_POINT('Ctrl Pts',(53.8973829222317,46.9603259488894,12.));
#109796=CARTESIAN_POINT('Ctrl Pts',(53.8858396531277,46.9404355654381,12.));
#109797=CARTESIAN_POINT('Ctrl Pts',(53.8742990540557,46.9205954387128,12.));
#109798=CARTESIAN_POINT('Ctrl Pts',(53.8627612499648,46.900805650336,12.));
#109799=CARTESIAN_POINT('Ctrl Pts',(53.851226366434,46.8810662822147,12.));
#109800=CARTESIAN_POINT('Ctrl Pts',(53.8396945296777,46.8613774165452,12.));
#109801=CARTESIAN_POINT('Ctrl Pts',(53.8281658665517,46.8417391358231,12.));
#109802=CARTESIAN_POINT('Ctrl Pts',(53.8166405045582,46.8221515228459,12.));
#109803=CARTESIAN_POINT('Ctrl Pts',(53.8051185718525,46.8026146607144,12.));
#109804=CARTESIAN_POINT('Ctrl Pts',(53.7936001972468,46.7831286328268,12.));
#109805=CARTESIAN_POINT('Ctrl Pts',(53.782085510217,46.7636935228851,12.));
#109806=CARTESIAN_POINT('Ctrl Pts',(53.770574640907,46.7443094149041,12.));
#109807=CARTESIAN_POINT('Ctrl Pts',(53.7590677201344,46.724976393213,12.));
#109808=CARTESIAN_POINT('Ctrl Pts',(53.7475648793948,46.7056945424559,12.));
#109809=CARTESIAN_POINT('Ctrl Pts',(53.7360662508677,46.6864639475863,12.));
#109810=CARTESIAN_POINT('Ctrl Pts',(53.7245719674222,46.6672846938752,12.));
#109811=CARTESIAN_POINT('Ctrl Pts',(53.7130821626263,46.6481568669216,12.));
#109812=CARTESIAN_POINT('Ctrl Pts',(53.701596970754,46.6290805526559,12.));
#109813=CARTESIAN_POINT('Ctrl Pts',(53.6901165267941,46.6100558373402,12.));
#109814=CARTESIAN_POINT('Ctrl Pts',(53.678640966456,46.5910828075653,12.));
#109815=CARTESIAN_POINT('Ctrl Pts',(53.6671704261737,46.5721615502591,12.));
#109816=CARTESIAN_POINT('Ctrl Pts',(53.6557050431071,46.5532921526901,12.));
#109817=CARTESIAN_POINT('Ctrl Pts',(53.6442449551455,46.5344747024676,12.));
#109818=CARTESIAN_POINT('Ctrl Pts',(53.6327903009094,46.5157092875373,12.));
#109819=CARTESIAN_POINT('Ctrl Pts',(53.6213412197533,46.496995996177,12.));
#109820=CARTESIAN_POINT('Ctrl Pts',(53.6098978517859,46.4783349170173,12.));
#109821=CARTESIAN_POINT('Ctrl Pts',(53.5984603378855,46.459726139052,12.));
#109822=CARTESIAN_POINT('Ctrl Pts',(53.5870288197166,46.4411697516478,12.));
#109823=CARTESIAN_POINT('Ctrl Pts',(53.5756034397481,46.4226658445474,12.));
#109824=CARTESIAN_POINT('Ctrl Pts',(53.5641843412559,46.4042145078701,12.));
#109825=CARTESIAN_POINT('Ctrl Pts',(53.5527716683048,46.3858158321059,12.));
#109826=CARTESIAN_POINT('Ctrl Pts',(53.5413655657327,46.3674699081046,12.));
#109827=CARTESIAN_POINT('Ctrl Pts',(53.5299661791385,46.3491768270655,12.));
#109828=CARTESIAN_POINT('Ctrl Pts',(53.5185736548548,46.3309366805093,12.));
#109829=CARTESIAN_POINT('Ctrl Pts',(53.5071881399911,46.3127495603098,12.));
#109830=CARTESIAN_POINT('Ctrl Pts',(53.4958097825006,46.2946155587417,12.));
#109831=CARTESIAN_POINT('Ctrl Pts',(53.4844387312414,46.2765347685198,12.));
#109832=CARTESIAN_POINT('Ctrl Pts',(53.4730751360371,46.2585072828353,12.));
#109833=CARTESIAN_POINT('Ctrl Pts',(53.4617191477402,46.2405331953889,12.));
#109834=CARTESIAN_POINT('Ctrl Pts',(53.4503709181178,46.2226126003202,12.));
#109835=CARTESIAN_POINT('Ctrl Pts',(53.4390305997274,46.2047455921286,12.));
#109836=CARTESIAN_POINT('Ctrl Pts',(53.4276983458125,46.1869322656024,12.));
#109837=CARTESIAN_POINT('Ctrl Pts',(53.4163743101517,46.1691727157134,12.));
#109838=CARTESIAN_POINT('Ctrl Pts',(53.4050586470436,46.1514670376012,12.));
#109839=CARTESIAN_POINT('Ctrl Pts',(53.3937515116549,46.1338153268097,12.));
#109840=CARTESIAN_POINT('Ctrl Pts',(53.3824530603276,46.1162176794884,12.));
#109841=CARTESIAN_POINT('Ctrl Pts',(53.3711634508437,46.0986741925656,12.));
#109842=CARTESIAN_POINT('Ctrl Pts',(53.3598828428546,46.0811849640218,12.));
#109843=CARTESIAN_POINT('Ctrl Pts',(53.3486113975901,46.0637500926982,12.));
#109844=CARTESIAN_POINT('Ctrl Pts',(53.3373492770671,46.0463696777801,12.));
#109845=CARTESIAN_POINT('Ctrl Pts',(53.326096643428,46.02904381836,12.));
#109846=CARTESIAN_POINT('Ctrl Pts',(53.3148536582635,46.0117726129873,12.));
#109847=CARTESIAN_POINT('Ctrl Pts',(53.3036204818329,45.9945561591453,12.));
#109848=CARTESIAN_POINT('Ctrl Pts',(53.292397274555,45.9773945542384,12.));
#109849=CARTESIAN_POINT('Ctrl Pts',(53.2811841987926,45.9602878967698,12.));
#109850=CARTESIAN_POINT('Ctrl Pts',(53.2699814203105,45.9432362873008,12.));
#109851=CARTESIAN_POINT('Ctrl Pts',(53.2587891103866,45.9262398298349,12.));
#109852=CARTESIAN_POINT('Ctrl Pts',(53.2476074460017,45.9092986319377,12.));
#109853=CARTESIAN_POINT('Ctrl Pts',(53.2364366054306,45.892412801838,12.));
#109854=CARTESIAN_POINT('Ctrl Pts',(53.2252767643662,45.8755824458723,12.));
#109855=CARTESIAN_POINT('Ctrl Pts',(53.2141280925439,45.8588076662582,12.));
#109856=CARTESIAN_POINT('Ctrl Pts',(53.2029907483557,45.8420885575349,12.));
#109857=CARTESIAN_POINT('Ctrl Pts',(53.1918648840541,45.8254252099957,12.));
#109858=CARTESIAN_POINT('Ctrl Pts',(53.1807506560933,45.808817716509,12.));
#109859=CARTESIAN_POINT('Ctrl Pts',(53.1696482334487,45.7922661780005,12.));
#109860=CARTESIAN_POINT('Ctrl Pts',(53.1585578076444,45.7757707100618,12.));
#109861=CARTESIAN_POINT('Ctrl Pts',(53.1474795996053,45.7593314474501,12.));
#109862=CARTESIAN_POINT('Ctrl Pts',(53.1364138384693,45.7429485300823,12.));
#109863=CARTESIAN_POINT('Ctrl Pts',(53.1253607414872,45.7266220897003,12.));
#109864=CARTESIAN_POINT('Ctrl Pts',(53.114320495492,45.7103522376696,12.));
#109865=CARTESIAN_POINT('Ctrl Pts',(53.1032932328857,45.694139048907,12.));
#109866=CARTESIAN_POINT('Ctrl Pts',(53.0922790298409,45.6779825614231,12.));
#109867=CARTESIAN_POINT('Ctrl Pts',(53.0834781451546,45.6651027439241,12.));
#109868=CARTESIAN_POINT('Ctrl Pts',(53.0768833804193,45.6554684028145,12.));
#109869=CARTESIAN_POINT('Ctrl Pts',(53.0724894921849,45.6490568514089,12.));
#109870=CARTESIAN_POINT('Ctrl Pts',(53.0702932034641,45.6458539113724,12.));
#109871=CARTESIAN_POINT('Ctrl Pts',(54.1946543500373,50.6869108458851,-1.11022302462516E-15));
#109872=CARTESIAN_POINT('Ctrl Pts',(54.1946543500373,50.6869108458851,4.));
#109873=CARTESIAN_POINT('Ctrl Pts',(54.1946543500373,50.6869108458851,8.));
#109874=CARTESIAN_POINT('Ctrl Pts',(54.1946543500373,50.6869108458851,12.));
#109875=CARTESIAN_POINT('Ctrl Pts',(54.2986513683568,50.7223900873023,-1.11022302462516E-15));
#109876=CARTESIAN_POINT('Ctrl Pts',(54.2986513683568,50.7223900873023,4.));
#109877=CARTESIAN_POINT('Ctrl Pts',(54.2986513683568,50.7223900873023,8.));
#109878=CARTESIAN_POINT('Ctrl Pts',(54.2986513683568,50.7223900873023,12.));
#109879=CARTESIAN_POINT('Ctrl Pts',(54.5013145669267,50.7219766588197,-1.03713937562159E-15));
#109880=CARTESIAN_POINT('Ctrl Pts',(54.5013145669267,50.7219766588197,4.));
#109881=CARTESIAN_POINT('Ctrl Pts',(54.5013145669267,50.7219766588197,7.99999999999999));
#109882=CARTESIAN_POINT('Ctrl Pts',(54.5013145669267,50.7219766588197,12.));
#109883=CARTESIAN_POINT('Ctrl Pts',(54.6674453828701,50.6135081477658,-8.63611844427818E-16));
#109884=CARTESIAN_POINT('Ctrl Pts',(54.6674453828701,50.6135081477658,4.));
#109885=CARTESIAN_POINT('Ctrl Pts',(54.6674453828701,50.6135081477658,8.));
#109886=CARTESIAN_POINT('Ctrl Pts',(54.6674453828701,50.6135081477658,12.));
#109887=CARTESIAN_POINT('Ctrl Pts',(54.7233670476834,50.55297319609,-7.79957864200068E-16));
#109888=CARTESIAN_POINT('Ctrl Pts',(54.7233670476834,50.55297319609,4.));
#109889=CARTESIAN_POINT('Ctrl Pts',(54.7233670476834,50.55297319609,8.));
#109890=CARTESIAN_POINT('Ctrl Pts',(54.7233670476834,50.55297319609,12.));
#109891=CARTESIAN_POINT('',(54.1946543500373,50.6869108458851,0.));
#109892=CARTESIAN_POINT('',(54.723367047683,50.5529731960897,0.));
#109893=CARTESIAN_POINT('Ctrl Pts',(54.1946543500373,50.6869108458851,8.74764948622162E-18));
#109894=CARTESIAN_POINT('Ctrl Pts',(54.2986513683568,50.7223900873023,8.74764948622131E-18));
#109895=CARTESIAN_POINT('Ctrl Pts',(54.4144589103968,50.7221538424551,5.05097346311187E-17));
#109896=CARTESIAN_POINT('Ctrl Pts',(54.5183375111709,50.6866343053397,1.25069822123835E-16));
#109897=CARTESIAN_POINT('Ctrl Pts',(54.5962464617515,50.6599946525032,1.80989887743373E-16));
#109898=CARTESIAN_POINT('Ctrl Pts',(54.6674453828701,50.6135081477658,2.55358829683559E-16));
#109899=CARTESIAN_POINT('Ctrl Pts',(54.7233670476834,50.55297319609,3.3901280991131E-16));
#109900=CARTESIAN_POINT('',(54.723367047683,50.5529731960897,12.));
#109901=CARTESIAN_POINT('Ctrl Pts',(54.7233670476834,50.55297319609,-7.79957864200068E-16));
#109902=CARTESIAN_POINT('Ctrl Pts',(54.7233670476834,50.55297319609,4.));
#109903=CARTESIAN_POINT('Ctrl Pts',(54.7233670476834,50.55297319609,8.));
#109904=CARTESIAN_POINT('Ctrl Pts',(54.7233670476834,50.55297319609,12.));
#109905=CARTESIAN_POINT('',(54.1946543500373,50.6869108458851,12.));
#109906=CARTESIAN_POINT('Ctrl Pts',(54.7233670476834,50.55297319609,12.));
#109907=CARTESIAN_POINT('Ctrl Pts',(54.6674453828701,50.6135081477658,12.));
#109908=CARTESIAN_POINT('Ctrl Pts',(54.5962464617515,50.6599946525032,12.));
#109909=CARTESIAN_POINT('Ctrl Pts',(54.5183375111709,50.6866343053397,12.));
#109910=CARTESIAN_POINT('Ctrl Pts',(54.4144589103968,50.7221538424551,12.));
#109911=CARTESIAN_POINT('Ctrl Pts',(54.2986513683568,50.7223900873023,12.));
#109912=CARTESIAN_POINT('Ctrl Pts',(54.1946543500373,50.6869108458851,12.));
#109913=CARTESIAN_POINT('Ctrl Pts',(54.1946543500373,50.6869108458851,12.));
#109914=CARTESIAN_POINT('Ctrl Pts',(54.1946543500373,50.6869108458851,8.));
#109915=CARTESIAN_POINT('Ctrl Pts',(54.1946543500373,50.6869108458851,4.));
#109916=CARTESIAN_POINT('Ctrl Pts',(54.1946543500373,50.6869108458851,-1.11022302462516E-15));
#109917=CARTESIAN_POINT('Origin',(2.7629675461203E-10,2.53313958019842E-10,
0.));
#109918=CARTESIAN_POINT('Origin',(2.7629675461203E-10,2.53313958019842E-10,
12.));
#109919=CARTESIAN_POINT('Origin',(2.7629675461203E-10,2.53313958019842E-10,
0.));
#109920=CARTESIAN_POINT('Ctrl Pts',(59.2875729049545,45.1135644683471,0.));
#109921=CARTESIAN_POINT('Ctrl Pts',(59.2875729049545,45.1135644683471,4.));
#109922=CARTESIAN_POINT('Ctrl Pts',(59.2875729049545,45.1135644683471,8.));
#109923=CARTESIAN_POINT('Ctrl Pts',(59.2875729049545,45.1135644683471,12.));
#109924=CARTESIAN_POINT('Ctrl Pts',(59.3541123643618,45.0261193041895,0.));
#109925=CARTESIAN_POINT('Ctrl Pts',(59.3541123643618,45.0261193041895,4.));
#109926=CARTESIAN_POINT('Ctrl Pts',(59.3541123643618,45.0261193041895,8.));
#109927=CARTESIAN_POINT('Ctrl Pts',(59.3541123643618,45.0261193041895,12.));
#109928=CARTESIAN_POINT('Ctrl Pts',(59.4177951463802,44.8337211159575,0.));
#109929=CARTESIAN_POINT('Ctrl Pts',(59.4177951463802,44.8337211159575,4.00000000000001));
#109930=CARTESIAN_POINT('Ctrl Pts',(59.4177951463802,44.8337211159575,8.));
#109931=CARTESIAN_POINT('Ctrl Pts',(59.4177951463802,44.8337211159575,12.));
#109932=CARTESIAN_POINT('Ctrl Pts',(59.3674150879748,44.6418181989799,0.));
#109933=CARTESIAN_POINT('Ctrl Pts',(59.3674150879748,44.6418181989799,4.));
#109934=CARTESIAN_POINT('Ctrl Pts',(59.3674150879747,44.6418181989798,8.00000000000001));
#109935=CARTESIAN_POINT('Ctrl Pts',(59.3674150879747,44.6418181989798,12.));
#109936=CARTESIAN_POINT('Ctrl Pts',(59.3276657444157,44.5696260757423,0.));
#109937=CARTESIAN_POINT('Ctrl Pts',(59.3276657444157,44.5696260757423,4.));
#109938=CARTESIAN_POINT('Ctrl Pts',(59.3276657444157,44.5696260757423,8.));
#109939=CARTESIAN_POINT('Ctrl Pts',(59.3276657444157,44.5696260757423,12.));
#109940=CARTESIAN_POINT('',(59.2875729049545,45.1135644683471,0.));
#109941=CARTESIAN_POINT('',(59.3276657444159,44.5696260757422,0.));
#109942=CARTESIAN_POINT('Ctrl Pts',(59.2875729049545,45.1135644683471,0.));
#109943=CARTESIAN_POINT('Ctrl Pts',(59.3541123643618,45.0261193041895,0.));
#109944=CARTESIAN_POINT('Ctrl Pts',(59.3905025255151,44.9161774823427,0.));
#109945=CARTESIAN_POINT('Ctrl Pts',(59.3896476775505,44.8063973817217,0.));
#109946=CARTESIAN_POINT('Ctrl Pts',(59.3890065415771,44.724062306256,0.));
#109947=CARTESIAN_POINT('Ctrl Pts',(59.3674150879748,44.6418181989799,0.));
#109948=CARTESIAN_POINT('Ctrl Pts',(59.3276657444157,44.5696260757423,0.));
#109949=CARTESIAN_POINT('',(59.3276657444159,44.5696260757422,12.));
#109950=CARTESIAN_POINT('Ctrl Pts',(59.3276657444157,44.5696260757423,0.));
#109951=CARTESIAN_POINT('Ctrl Pts',(59.3276657444157,44.5696260757423,4.));
#109952=CARTESIAN_POINT('Ctrl Pts',(59.3276657444157,44.5696260757423,8.));
#109953=CARTESIAN_POINT('Ctrl Pts',(59.3276657444157,44.5696260757423,12.));
#109954=CARTESIAN_POINT('',(59.2875729049545,45.1135644683471,12.));
#109955=CARTESIAN_POINT('Ctrl Pts',(59.3276657444157,44.5696260757423,12.));
#109956=CARTESIAN_POINT('Ctrl Pts',(59.3674150879747,44.6418181989798,12.));
#109957=CARTESIAN_POINT('Ctrl Pts',(59.3890065415771,44.724062306256,12.));
#109958=CARTESIAN_POINT('Ctrl Pts',(59.3896476775505,44.8063973817217,12.));
#109959=CARTESIAN_POINT('Ctrl Pts',(59.3905025255151,44.9161774823427,12.));
#109960=CARTESIAN_POINT('Ctrl Pts',(59.3541123643618,45.0261193041895,12.));
#109961=CARTESIAN_POINT('Ctrl Pts',(59.2875729049545,45.1135644683471,12.));
#109962=CARTESIAN_POINT('Ctrl Pts',(59.2875729049545,45.1135644683471,12.));
#109963=CARTESIAN_POINT('Ctrl Pts',(59.2875729049545,45.1135644683471,8.));
#109964=CARTESIAN_POINT('Ctrl Pts',(59.2875729049545,45.1135644683471,4.));
#109965=CARTESIAN_POINT('Ctrl Pts',(59.2875729049545,45.1135644683471,0.));
#109966=CARTESIAN_POINT('Ctrl Pts',(56.8466430164621,40.8467768343956,0.));
#109967=CARTESIAN_POINT('Ctrl Pts',(56.8466430164621,40.8467768343956,12.));
#109968=CARTESIAN_POINT('Ctrl Pts',(56.8491101022591,40.8497761671036,0.));
#109969=CARTESIAN_POINT('Ctrl Pts',(56.8491101022591,40.8497761671036,12.));
#109970=CARTESIAN_POINT('Ctrl Pts',(56.8540460739472,40.8557803680278,0.));
#109971=CARTESIAN_POINT('Ctrl Pts',(56.8540460739472,40.8557803680278,12.));
#109972=CARTESIAN_POINT('Ctrl Pts',(56.8614554317668,40.864803275942,0.));
#109973=CARTESIAN_POINT('Ctrl Pts',(56.8614554317668,40.864803275942,12.));
#109974=CARTESIAN_POINT('Ctrl Pts',(56.8713453764905,40.8768670342052,0.));
#109975=CARTESIAN_POINT('Ctrl Pts',(56.8713453764905,40.8768670342052,12.));
#109976=CARTESIAN_POINT('Ctrl Pts',(56.8837257978343,40.8920020903293,0.));
#109977=CARTESIAN_POINT('Ctrl Pts',(56.8837257978343,40.8920020903293,12.));
#109978=CARTESIAN_POINT('Ctrl Pts',(56.8961241708861,40.9071924937508,0.));
#109979=CARTESIAN_POINT('Ctrl Pts',(56.8961241708861,40.9071924937508,12.));
#109980=CARTESIAN_POINT('Ctrl Pts',(56.9085404164502,40.9224382132427,0.));
#109981=CARTESIAN_POINT('Ctrl Pts',(56.9085404164502,40.9224382132427,12.));
#109982=CARTESIAN_POINT('Ctrl Pts',(56.9209743960992,40.9377391857129,0.));
#109983=CARTESIAN_POINT('Ctrl Pts',(56.9209743960992,40.9377391857129,12.));
#109984=CARTESIAN_POINT('Ctrl Pts',(56.9334259140049,40.9530953165031,0.));
#109985=CARTESIAN_POINT('Ctrl Pts',(56.9334259140049,40.9530953165031,12.));
#109986=CARTESIAN_POINT('Ctrl Pts',(56.9458947422608,40.9685064933074,0.));
#109987=CARTESIAN_POINT('Ctrl Pts',(56.9458947422608,40.9685064933074,12.));
#109988=CARTESIAN_POINT('Ctrl Pts',(56.9583806404069,40.9839725967121,0.));
#109989=CARTESIAN_POINT('Ctrl Pts',(56.9583806404069,40.9839725967121,12.));
#109990=CARTESIAN_POINT('Ctrl Pts',(56.9708833766137,40.9994935117276,0.));
#109991=CARTESIAN_POINT('Ctrl Pts',(56.9708833766137,40.9994935117276,12.));
#109992=CARTESIAN_POINT('Ctrl Pts',(56.9834027500117,41.0150691398947,0.));
#109993=CARTESIAN_POINT('Ctrl Pts',(56.9834027500117,41.0150691398947,12.));
#109994=CARTESIAN_POINT('Ctrl Pts',(56.995938583472,41.0306993953989,0.));
#109995=CARTESIAN_POINT('Ctrl Pts',(56.995938583472,41.0306993953989,12.));
#109996=CARTESIAN_POINT('Ctrl Pts',(57.008490713042,41.0463841993608,0.));
#109997=CARTESIAN_POINT('Ctrl Pts',(57.008490713042,41.0463841993608,12.));
#109998=CARTESIAN_POINT('Ctrl Pts',(57.0210589791788,41.0621234751007,0.));
#109999=CARTESIAN_POINT('Ctrl Pts',(57.0210589791788,41.0621234751007,12.));
#110000=CARTESIAN_POINT('Ctrl Pts',(57.0336432158536,41.0779171422438,0.));
#110001=CARTESIAN_POINT('Ctrl Pts',(57.0336432158536,41.0779171422438,12.));
#110002=CARTESIAN_POINT('Ctrl Pts',(57.046243245068,41.0937651137549,0.));
#110003=CARTESIAN_POINT('Ctrl Pts',(57.046243245068,41.0937651137549,12.));
#110004=CARTESIAN_POINT('Ctrl Pts',(57.0588588825298,41.1096672990148,0.));
#110005=CARTESIAN_POINT('Ctrl Pts',(57.0588588825298,41.1096672990148,12.));
#110006=CARTESIAN_POINT('Ctrl Pts',(57.0714899412099,41.1256236057443,0.));
#110007=CARTESIAN_POINT('Ctrl Pts',(57.0714899412099,41.1256236057443,12.));
#110008=CARTESIAN_POINT('Ctrl Pts',(57.084136235426,41.1416339422117,0.));
#110009=CARTESIAN_POINT('Ctrl Pts',(57.084136235426,41.1416339422117,12.));
#110010=CARTESIAN_POINT('Ctrl Pts',(57.0967975854874,41.1576982197375,0.));
#110011=CARTESIAN_POINT('Ctrl Pts',(57.0967975854874,41.1576982197375,12.));
#110012=CARTESIAN_POINT('Ctrl Pts',(57.1094738174957,41.1738163525902,0.));
#110013=CARTESIAN_POINT('Ctrl Pts',(57.1094738174957,41.1738163525902,12.));
#110014=CARTESIAN_POINT('Ctrl Pts',(57.1221647611207,41.1899882567923,0.));
#110015=CARTESIAN_POINT('Ctrl Pts',(57.1221647611207,41.1899882567923,12.));
#110016=CARTESIAN_POINT('Ctrl Pts',(57.1348702480647,41.2062138492915,0.));
#110017=CARTESIAN_POINT('Ctrl Pts',(57.1348702480647,41.2062138492915,12.));
#110018=CARTESIAN_POINT('Ctrl Pts',(57.147590110182,41.222493046943,0.));
#110019=CARTESIAN_POINT('Ctrl Pts',(57.147590110182,41.222493046943,12.));
#110020=CARTESIAN_POINT('Ctrl Pts',(57.1603241779077,41.2388257656559,0.));
#110021=CARTESIAN_POINT('Ctrl Pts',(57.1603241779077,41.2388257656559,12.));
#110022=CARTESIAN_POINT('Ctrl Pts',(57.17307228108,41.2552119208466,0.));
#110023=CARTESIAN_POINT('Ctrl Pts',(57.17307228108,41.2552119208466,12.));
#110024=CARTESIAN_POINT('Ctrl Pts',(57.1858342496538,41.2716514278276,0.));
#110025=CARTESIAN_POINT('Ctrl Pts',(57.1858342496538,41.2716514278276,12.));
#110026=CARTESIAN_POINT('Ctrl Pts',(57.1986099143983,41.2881442021863,0.));
#110027=CARTESIAN_POINT('Ctrl Pts',(57.1986099143983,41.2881442021863,12.));
#110028=CARTESIAN_POINT('Ctrl Pts',(57.2113991077302,41.3046901602293,0.));
#110029=CARTESIAN_POINT('Ctrl Pts',(57.2113991077302,41.3046901602293,12.));
#110030=CARTESIAN_POINT('Ctrl Pts',(57.2242016640198,41.321289219149,0.));
#110031=CARTESIAN_POINT('Ctrl Pts',(57.2242016640198,41.321289219149,12.));
#110032=CARTESIAN_POINT('Ctrl Pts',(57.2370174191401,41.3379412967875,0.));
#110033=CARTESIAN_POINT('Ctrl Pts',(57.2370174191401,41.3379412967875,12.));
#110034=CARTESIAN_POINT('Ctrl Pts',(57.2498462101879,41.3546463114885,0.));
#110035=CARTESIAN_POINT('Ctrl Pts',(57.2498462101879,41.3546463114885,12.));
#110036=CARTESIAN_POINT('Ctrl Pts',(57.2626878751596,41.3714041819224,0.));
#110037=CARTESIAN_POINT('Ctrl Pts',(57.2626878751596,41.3714041819224,12.));
#110038=CARTESIAN_POINT('Ctrl Pts',(57.2755422525844,41.3882148268814,0.));
#110039=CARTESIAN_POINT('Ctrl Pts',(57.2755422525844,41.3882148268814,12.));
#110040=CARTESIAN_POINT('Ctrl Pts',(57.2884091815406,41.4050781652938,0.));
#110041=CARTESIAN_POINT('Ctrl Pts',(57.2884091815406,41.4050781652938,12.));
#110042=CARTESIAN_POINT('Ctrl Pts',(57.3012885018151,41.4219941163163,0.));
#110043=CARTESIAN_POINT('Ctrl Pts',(57.3012885018151,41.4219941163163,12.));
#110044=CARTESIAN_POINT('Ctrl Pts',(57.3141800540137,41.4389625993948,0.));
#110045=CARTESIAN_POINT('Ctrl Pts',(57.3141800540137,41.4389625993948,12.));
#110046=CARTESIAN_POINT('Ctrl Pts',(57.3270836796911,41.4559835343328,0.));
#110047=CARTESIAN_POINT('Ctrl Pts',(57.3270836796911,41.4559835343328,12.));
#110048=CARTESIAN_POINT('Ctrl Pts',(57.3399992214717,41.4730568413518,0.));
#110049=CARTESIAN_POINT('Ctrl Pts',(57.3399992214717,41.4730568413518,12.));
#110050=CARTESIAN_POINT('Ctrl Pts',(57.3529265229835,41.4901824410637,0.));
#110051=CARTESIAN_POINT('Ctrl Pts',(57.3529265229835,41.4901824410637,12.));
#110052=CARTESIAN_POINT('Ctrl Pts',(57.3658654287937,41.5073602544396,0.));
#110053=CARTESIAN_POINT('Ctrl Pts',(57.3658654287937,41.5073602544396,12.));
#110054=CARTESIAN_POINT('Ctrl Pts',(57.3788157843454,41.5245902027771,0.));
#110055=CARTESIAN_POINT('Ctrl Pts',(57.3788157843454,41.5245902027771,12.));
#110056=CARTESIAN_POINT('Ctrl Pts',(57.3917774358863,41.5418722076572,0.));
#110057=CARTESIAN_POINT('Ctrl Pts',(57.3917774358863,41.5418722076572,12.));
#110058=CARTESIAN_POINT('Ctrl Pts',(57.4047502304231,41.5592061909176,0.));
#110059=CARTESIAN_POINT('Ctrl Pts',(57.4047502304231,41.5592061909176,12.));
#110060=CARTESIAN_POINT('Ctrl Pts',(57.4177340157508,41.5765920746777,0.));
#110061=CARTESIAN_POINT('Ctrl Pts',(57.4177340157508,41.5765920746777,12.));
#110062=CARTESIAN_POINT('Ctrl Pts',(57.4307286404662,41.5940297813477,0.));
#110063=CARTESIAN_POINT('Ctrl Pts',(57.4307286404662,41.5940297813477,12.));
#110064=CARTESIAN_POINT('Ctrl Pts',(57.4437339539841,41.6115192336388,0.));
#110065=CARTESIAN_POINT('Ctrl Pts',(57.4437339539841,41.6115192336388,12.));
#110066=CARTESIAN_POINT('Ctrl Pts',(57.4567498065562,41.6290603545666,0.));
#110067=CARTESIAN_POINT('Ctrl Pts',(57.4567498065562,41.6290603545666,12.));
#110068=CARTESIAN_POINT('Ctrl Pts',(57.4697760492683,41.6466530674515,0.));
#110069=CARTESIAN_POINT('Ctrl Pts',(57.4697760492683,41.6466530674515,12.));
#110070=CARTESIAN_POINT('Ctrl Pts',(57.4828125340218,41.6642972959165,0.));
#110071=CARTESIAN_POINT('Ctrl Pts',(57.4828125340218,41.6642972959165,12.));
#110072=CARTESIAN_POINT('Ctrl Pts',(57.4958591135165,41.6819929638797,0.));
#110073=CARTESIAN_POINT('Ctrl Pts',(57.4958591135165,41.6819929638797,12.));
#110074=CARTESIAN_POINT('Ctrl Pts',(57.5089156412343,41.6997399955447,0.));
#110075=CARTESIAN_POINT('Ctrl Pts',(57.5089156412343,41.6997399955447,12.));
#110076=CARTESIAN_POINT('Ctrl Pts',(57.5219819714171,41.7175383153821,0.));
#110077=CARTESIAN_POINT('Ctrl Pts',(57.5219819714171,41.7175383153821,12.));
#110078=CARTESIAN_POINT('Ctrl Pts',(57.5350579590649,41.7353878481337,0.));
#110079=CARTESIAN_POINT('Ctrl Pts',(57.5350579590649,41.7353878481337,12.));
#110080=CARTESIAN_POINT('Ctrl Pts',(57.5481434599335,41.7532885188175,0.));
#110081=CARTESIAN_POINT('Ctrl Pts',(57.5481434599335,41.7532885188175,12.));
#110082=CARTESIAN_POINT('Ctrl Pts',(57.561238330532,41.7712402527273,0.));
#110083=CARTESIAN_POINT('Ctrl Pts',(57.561238330532,41.7712402527273,12.));
#110084=CARTESIAN_POINT('Ctrl Pts',(57.5743424281204,41.7892429754297,0.));
#110085=CARTESIAN_POINT('Ctrl Pts',(57.5743424281204,41.7892429754297,12.));
#110086=CARTESIAN_POINT('Ctrl Pts',(57.5874556107056,41.8072966127558,0.));
#110087=CARTESIAN_POINT('Ctrl Pts',(57.5874556107056,41.8072966127558,12.));
#110088=CARTESIAN_POINT('Ctrl Pts',(57.6005777370349,41.8254010908051,0.));
#110089=CARTESIAN_POINT('Ctrl Pts',(57.6005777370349,41.8254010908051,12.));
#110090=CARTESIAN_POINT('Ctrl Pts',(57.6137086665882,41.8435563359456,0.));
#110091=CARTESIAN_POINT('Ctrl Pts',(57.6137086665882,41.8435563359456,12.));
#110092=CARTESIAN_POINT('Ctrl Pts',(57.6268482595702,41.8617622748108,0.));
#110093=CARTESIAN_POINT('Ctrl Pts',(57.6268482595702,41.8617622748108,12.));
#110094=CARTESIAN_POINT('Ctrl Pts',(57.6399963769003,41.8800188342909,0.));
#110095=CARTESIAN_POINT('Ctrl Pts',(57.6399963769003,41.8800188342909,12.));
#110096=CARTESIAN_POINT('Ctrl Pts',(57.6531528802059,41.8983259415245,0.));
#110097=CARTESIAN_POINT('Ctrl Pts',(57.6531528802059,41.8983259415245,12.));
#110098=CARTESIAN_POINT('Ctrl Pts',(57.6663176318176,41.9166835239046,0.));
#110099=CARTESIAN_POINT('Ctrl Pts',(57.6663176318176,41.9166835239046,12.));
#110100=CARTESIAN_POINT('Ctrl Pts',(57.6794904947641,41.9350915090791,0.));
#110101=CARTESIAN_POINT('Ctrl Pts',(57.6794904947641,41.9350915090791,12.));
#110102=CARTESIAN_POINT('Ctrl Pts',(57.6926713327674,41.9535498249489,0.));
#110103=CARTESIAN_POINT('Ctrl Pts',(57.6926713327674,41.9535498249489,12.));
#110104=CARTESIAN_POINT('Ctrl Pts',(57.7058600102365,41.9720583996601,0.));
#110105=CARTESIAN_POINT('Ctrl Pts',(57.7058600102365,41.9720583996601,12.));
#110106=CARTESIAN_POINT('Ctrl Pts',(57.7190563922614,41.9906171615975,0.));
#110107=CARTESIAN_POINT('Ctrl Pts',(57.7190563922614,41.9906171615975,12.));
#110108=CARTESIAN_POINT('Ctrl Pts',(57.7322603446086,42.0092260393911,0.));
#110109=CARTESIAN_POINT('Ctrl Pts',(57.7322603446086,42.0092260393911,12.));
#110110=CARTESIAN_POINT('Ctrl Pts',(57.7454717337151,42.0278849619156,0.));
#110111=CARTESIAN_POINT('Ctrl Pts',(57.7454717337151,42.0278849619156,12.));
#110112=CARTESIAN_POINT('Ctrl Pts',(57.7586904266828,42.0465938582878,0.));
#110113=CARTESIAN_POINT('Ctrl Pts',(57.7586904266828,42.0465938582878,12.));
#110114=CARTESIAN_POINT('Ctrl Pts',(57.7719162912721,42.0653526578571,0.));
#110115=CARTESIAN_POINT('Ctrl Pts',(57.7719162912721,42.0653526578571,12.));
#110116=CARTESIAN_POINT('Ctrl Pts',(57.7851491958954,42.0841612902018,0.));
#110117=CARTESIAN_POINT('Ctrl Pts',(57.7851491958954,42.0841612902018,12.));
#110118=CARTESIAN_POINT('Ctrl Pts',(57.798389009613,42.1030196851344,0.));
#110119=CARTESIAN_POINT('Ctrl Pts',(57.798389009613,42.1030196851344,12.));
#110120=CARTESIAN_POINT('Ctrl Pts',(57.8116356021274,42.121927772701,0.));
#110121=CARTESIAN_POINT('Ctrl Pts',(57.8116356021274,42.121927772701,12.));
#110122=CARTESIAN_POINT('Ctrl Pts',(57.8248888437787,42.1408854831792,0.));
#110123=CARTESIAN_POINT('Ctrl Pts',(57.8248888437787,42.1408854831792,12.));
#110124=CARTESIAN_POINT('Ctrl Pts',(57.8381486055376,42.1598927470671,0.));
#110125=CARTESIAN_POINT('Ctrl Pts',(57.8381486055376,42.1598927470671,12.));
#110126=CARTESIAN_POINT('Ctrl Pts',(57.8514147590012,42.1789494950824,0.));
#110127=CARTESIAN_POINT('Ctrl Pts',(57.8514147590012,42.1789494950824,12.));
#110128=CARTESIAN_POINT('Ctrl Pts',(57.86468717639,42.1980556581689,0.));
#110129=CARTESIAN_POINT('Ctrl Pts',(57.86468717639,42.1980556581689,12.));
#110130=CARTESIAN_POINT('Ctrl Pts',(57.8779657305422,42.2172111674946,0.));
#110131=CARTESIAN_POINT('Ctrl Pts',(57.8779657305422,42.2172111674946,12.));
#110132=CARTESIAN_POINT('Ctrl Pts',(57.8912502949084,42.2364159544492,0.));
#110133=CARTESIAN_POINT('Ctrl Pts',(57.8912502949084,42.2364159544492,12.));
#110134=CARTESIAN_POINT('Ctrl Pts',(57.9045407435447,42.2556699506332,0.));
#110135=CARTESIAN_POINT('Ctrl Pts',(57.9045407435447,42.2556699506332,12.));
#110136=CARTESIAN_POINT('Ctrl Pts',(57.9178369511084,42.274973087857,0.));
#110137=CARTESIAN_POINT('Ctrl Pts',(57.9178369511084,42.274973087857,12.));
#110138=CARTESIAN_POINT('Ctrl Pts',(57.9311387928541,42.2943252981471,0.));
#110139=CARTESIAN_POINT('Ctrl Pts',(57.9311387928541,42.2943252981471,12.));
#110140=CARTESIAN_POINT('Ctrl Pts',(57.9444461446292,42.3137265137446,0.));
#110141=CARTESIAN_POINT('Ctrl Pts',(57.9444461446292,42.3137265137446,12.));
#110142=CARTESIAN_POINT('Ctrl Pts',(57.9577588828693,42.3331766671028,0.));
#110143=CARTESIAN_POINT('Ctrl Pts',(57.9577588828693,42.3331766671028,12.));
#110144=CARTESIAN_POINT('Ctrl Pts',(57.9710768845923,42.3526756908764,0.));
#110145=CARTESIAN_POINT('Ctrl Pts',(57.9710768845923,42.3526756908764,12.));
#110146=CARTESIAN_POINT('Ctrl Pts',(57.9844000273936,42.3722235179216,0.));
#110147=CARTESIAN_POINT('Ctrl Pts',(57.9844000273936,42.3722235179216,12.));
#110148=CARTESIAN_POINT('Ctrl Pts',(57.9977281894437,42.3918200813025,0.));
#110149=CARTESIAN_POINT('Ctrl Pts',(57.9977281894437,42.3918200813025,12.));
#110150=CARTESIAN_POINT('Ctrl Pts',(58.011061249483,42.4114653142891,0.));
#110151=CARTESIAN_POINT('Ctrl Pts',(58.011061249483,42.4114653142891,12.));
#110152=CARTESIAN_POINT('Ctrl Pts',(58.0243990868175,42.4311591503551,0.));
#110153=CARTESIAN_POINT('Ctrl Pts',(58.0243990868175,42.4311591503551,12.));
#110154=CARTESIAN_POINT('Ctrl Pts',(58.0377415813132,42.4509015231668,0.));
#110155=CARTESIAN_POINT('Ctrl Pts',(58.0377415813132,42.4509015231668,12.));
#110156=CARTESIAN_POINT('Ctrl Pts',(58.0510886133917,42.4706923665838,0.));
#110157=CARTESIAN_POINT('Ctrl Pts',(58.0510886133917,42.4706923665838,12.));
#110158=CARTESIAN_POINT('Ctrl Pts',(58.064440064027,42.490531614665,0.));
#110159=CARTESIAN_POINT('Ctrl Pts',(58.064440064027,42.490531614665,12.));
#110160=CARTESIAN_POINT('Ctrl Pts',(58.0777958147404,42.5104192016664,0.));
#110161=CARTESIAN_POINT('Ctrl Pts',(58.0777958147404,42.5104192016664,12.));
#110162=CARTESIAN_POINT('Ctrl Pts',(58.0911557475967,42.5303550620388,0.));
#110163=CARTESIAN_POINT('Ctrl Pts',(58.0911557475967,42.5303550620388,12.));
#110164=CARTESIAN_POINT('Ctrl Pts',(58.1045197452003,42.5503391304183,0.));
#110165=CARTESIAN_POINT('Ctrl Pts',(58.1045197452003,42.5503391304183,12.));
#110166=CARTESIAN_POINT('Ctrl Pts',(58.1178876906905,42.5703713416263,0.));
#110167=CARTESIAN_POINT('Ctrl Pts',(58.1178876906905,42.5703713416263,12.));
#110168=CARTESIAN_POINT('Ctrl Pts',(58.1312594677383,42.5904516306759,0.));
#110169=CARTESIAN_POINT('Ctrl Pts',(58.1312594677383,42.5904516306759,12.));
#110170=CARTESIAN_POINT('Ctrl Pts',(58.1446349605419,42.6105799327697,0.));
#110171=CARTESIAN_POINT('Ctrl Pts',(58.1446349605419,42.6105799327697,12.));
#110172=CARTESIAN_POINT('Ctrl Pts',(58.158014053823,42.6307561832978,0.));
#110173=CARTESIAN_POINT('Ctrl Pts',(58.158014053823,42.6307561832978,12.));
#110174=CARTESIAN_POINT('Ctrl Pts',(58.1713966328217,42.650980317827,0.));
#110175=CARTESIAN_POINT('Ctrl Pts',(58.1713966328217,42.650980317827,12.));
#110176=CARTESIAN_POINT('Ctrl Pts',(58.1847825832932,42.6712522721021,0.));
#110177=CARTESIAN_POINT('Ctrl Pts',(58.1847825832932,42.6712522721021,12.));
#110178=CARTESIAN_POINT('Ctrl Pts',(58.1981717915043,42.6915719820517,0.));
#110179=CARTESIAN_POINT('Ctrl Pts',(58.1981717915043,42.6915719820517,12.));
#110180=CARTESIAN_POINT('Ctrl Pts',(58.2115641442302,42.7119393837867,0.));
#110181=CARTESIAN_POINT('Ctrl Pts',(58.2115641442302,42.7119393837867,12.));
#110182=CARTESIAN_POINT('Ctrl Pts',(58.2249595287497,42.7323544135983,0.));
#110183=CARTESIAN_POINT('Ctrl Pts',(58.2249595287497,42.7323544135983,12.));
#110184=CARTESIAN_POINT('Ctrl Pts',(58.238357832842,42.7528170079482,0.));
#110185=CARTESIAN_POINT('Ctrl Pts',(58.238357832842,42.7528170079482,12.));
#110186=CARTESIAN_POINT('Ctrl Pts',(58.2517589447818,42.7733271034679,0.));
#110187=CARTESIAN_POINT('Ctrl Pts',(58.2517589447818,42.7733271034679,12.));
#110188=CARTESIAN_POINT('Ctrl Pts',(58.2651627533368,42.7938846369651,0.));
#110189=CARTESIAN_POINT('Ctrl Pts',(58.2651627533368,42.7938846369651,12.));
#110190=CARTESIAN_POINT('Ctrl Pts',(58.278569147764,42.8144895454234,0.));
#110191=CARTESIAN_POINT('Ctrl Pts',(58.278569147764,42.8144895454234,12.));
#110192=CARTESIAN_POINT('Ctrl Pts',(58.2919780178063,42.8351417659998,0.));
#110193=CARTESIAN_POINT('Ctrl Pts',(58.2919780178063,42.8351417659998,12.));
#110194=CARTESIAN_POINT('Ctrl Pts',(58.305389253689,42.8558412360154,0.));
#110195=CARTESIAN_POINT('Ctrl Pts',(58.305389253689,42.8558412360154,12.));
#110196=CARTESIAN_POINT('Ctrl Pts',(58.3188027461157,42.8765878929545,0.));
#110197=CARTESIAN_POINT('Ctrl Pts',(58.3188027461157,42.8765878929545,12.));
#110198=CARTESIAN_POINT('Ctrl Pts',(58.3322183862647,42.8973816744703,0.));
#110199=CARTESIAN_POINT('Ctrl Pts',(58.3322183862647,42.8973816744703,12.));
#110200=CARTESIAN_POINT('Ctrl Pts',(58.3456360657861,42.9182225183851,0.));
#110201=CARTESIAN_POINT('Ctrl Pts',(58.3456360657861,42.9182225183851,12.));
#110202=CARTESIAN_POINT('Ctrl Pts',(58.3590556767981,42.9391103626881,0.));
#110203=CARTESIAN_POINT('Ctrl Pts',(58.3590556767981,42.9391103626881,12.));
#110204=CARTESIAN_POINT('Ctrl Pts',(58.3724771118835,42.9600451455267,0.));
#110205=CARTESIAN_POINT('Ctrl Pts',(58.3724771118835,42.9600451455267,12.));
#110206=CARTESIAN_POINT('Ctrl Pts',(58.3859002640871,42.9810268052043,0.));
#110207=CARTESIAN_POINT('Ctrl Pts',(58.3859002640871,42.9810268052043,12.));
#110208=CARTESIAN_POINT('Ctrl Pts',(58.3993250269115,43.002055280187,0.));
#110209=CARTESIAN_POINT('Ctrl Pts',(58.3993250269115,43.002055280187,12.));
#110210=CARTESIAN_POINT('Ctrl Pts',(58.4127512943144,43.0231305091033,0.));
#110211=CARTESIAN_POINT('Ctrl Pts',(58.4127512943144,43.0231305091033,12.));
#110212=CARTESIAN_POINT('Ctrl Pts',(58.4261789607055,43.0442524307432,0.));
#110213=CARTESIAN_POINT('Ctrl Pts',(58.4261789607055,43.0442524307432,12.));
#110214=CARTESIAN_POINT('Ctrl Pts',(58.4396079209438,43.0654209840502,0.));
#110215=CARTESIAN_POINT('Ctrl Pts',(58.4396079209438,43.0654209840502,12.));
#110216=CARTESIAN_POINT('Ctrl Pts',(58.4530380703335,43.0866361081166,0.));
#110217=CARTESIAN_POINT('Ctrl Pts',(58.4530380703335,43.0866361081166,12.));
#110218=CARTESIAN_POINT('Ctrl Pts',(58.4664693046206,43.1078977421908,0.));
#110219=CARTESIAN_POINT('Ctrl Pts',(58.4664693046206,43.1078977421908,12.));
#110220=CARTESIAN_POINT('Ctrl Pts',(58.4799015199904,43.1292058256774,0.));
#110221=CARTESIAN_POINT('Ctrl Pts',(58.4799015199904,43.1292058256774,12.));
#110222=CARTESIAN_POINT('Ctrl Pts',(58.4933346130638,43.1505602981366,0.));
#110223=CARTESIAN_POINT('Ctrl Pts',(58.4933346130638,43.1505602981366,12.));
#110224=CARTESIAN_POINT('Ctrl Pts',(58.5067684808946,43.1719610992772,0.));
#110225=CARTESIAN_POINT('Ctrl Pts',(58.5067684808946,43.1719610992772,12.));
#110226=CARTESIAN_POINT('Ctrl Pts',(58.5202030209667,43.1934081689504,0.));
#110227=CARTESIAN_POINT('Ctrl Pts',(58.5202030209667,43.1934081689504,12.));
#110228=CARTESIAN_POINT('Ctrl Pts',(58.5336381311911,43.214901447157,0.));
#110229=CARTESIAN_POINT('Ctrl Pts',(58.5336381311911,43.214901447157,12.));
#110230=CARTESIAN_POINT('Ctrl Pts',(58.5470737099027,43.2364408740489,0.));
#110231=CARTESIAN_POINT('Ctrl Pts',(58.5470737099027,43.2364408740489,12.));
#110232=CARTESIAN_POINT('Ctrl Pts',(58.5605096558578,43.2580263899278,0.));
#110233=CARTESIAN_POINT('Ctrl Pts',(58.5605096558578,43.2580263899278,12.));
#110234=CARTESIAN_POINT('Ctrl Pts',(58.5739458682317,43.2796579352405,0.));
#110235=CARTESIAN_POINT('Ctrl Pts',(58.5739458682317,43.2796579352405,12.));
#110236=CARTESIAN_POINT('Ctrl Pts',(58.5873822466163,43.3013354505708,0.));
#110237=CARTESIAN_POINT('Ctrl Pts',(58.5873822466163,43.3013354505708,12.));
#110238=CARTESIAN_POINT('Ctrl Pts',(58.6008186910166,43.3230588766456,0.));
#110239=CARTESIAN_POINT('Ctrl Pts',(58.6008186910166,43.3230588766456,12.));
#110240=CARTESIAN_POINT('Ctrl Pts',(58.6142551018473,43.3448281543375,0.));
#110241=CARTESIAN_POINT('Ctrl Pts',(58.6142551018473,43.3448281543375,12.));
#110242=CARTESIAN_POINT('Ctrl Pts',(58.627691379929,43.3666432246635,0.));
#110243=CARTESIAN_POINT('Ctrl Pts',(58.627691379929,43.3666432246635,12.));
#110244=CARTESIAN_POINT('Ctrl Pts',(58.6411274264854,43.3885040287808,0.));
#110245=CARTESIAN_POINT('Ctrl Pts',(58.6411274264854,43.3885040287808,12.));
#110246=CARTESIAN_POINT('Ctrl Pts',(58.6545631431388,43.4104105079766,0.));
#110247=CARTESIAN_POINT('Ctrl Pts',(58.6545631431388,43.4104105079766,12.));
#110248=CARTESIAN_POINT('Ctrl Pts',(58.6679984319095,43.4323626036736,0.));
#110249=CARTESIAN_POINT('Ctrl Pts',(58.6679984319095,43.4323626036736,12.));
#110250=CARTESIAN_POINT('Ctrl Pts',(58.6814331952138,43.4543602574352,0.));
#110251=CARTESIAN_POINT('Ctrl Pts',(58.6814331952138,43.4543602574352,12.));
#110252=CARTESIAN_POINT('Ctrl Pts',(58.6948673358639,43.4764034109655,0.));
#110253=CARTESIAN_POINT('Ctrl Pts',(58.6948673358639,43.4764034109655,12.));
#110254=CARTESIAN_POINT('Ctrl Pts',(58.708300757066,43.4984920061071,0.));
#110255=CARTESIAN_POINT('Ctrl Pts',(58.708300757066,43.4984920061071,12.));
#110256=CARTESIAN_POINT('Ctrl Pts',(58.7217333624206,43.5206259848333,0.));
#110257=CARTESIAN_POINT('Ctrl Pts',(58.7217333624206,43.5206259848333,12.));
#110258=CARTESIAN_POINT('Ctrl Pts',(58.7351650559176,43.5428052892483,0.));
#110259=CARTESIAN_POINT('Ctrl Pts',(58.7351650559176,43.5428052892483,12.));
#110260=CARTESIAN_POINT('Ctrl Pts',(58.7485957419296,43.5650298615912,0.));
#110261=CARTESIAN_POINT('Ctrl Pts',(58.7485957419296,43.5650298615912,12.));
#110262=CARTESIAN_POINT('Ctrl Pts',(58.7620253252059,43.5872996442343,0.));
#110263=CARTESIAN_POINT('Ctrl Pts',(58.7620253252059,43.5872996442343,12.));
#110264=CARTESIAN_POINT('Ctrl Pts',(58.7754537108672,43.6096145796798,0.));
#110265=CARTESIAN_POINT('Ctrl Pts',(58.7754537108672,43.6096145796798,12.));
#110266=CARTESIAN_POINT('Ctrl Pts',(58.7888808043976,43.6319746105488,0.));
#110267=CARTESIAN_POINT('Ctrl Pts',(58.7888808043976,43.6319746105488,12.));
#110268=CARTESIAN_POINT('Ctrl Pts',(58.8023065116446,43.6543796795797,0.));
#110269=CARTESIAN_POINT('Ctrl Pts',(58.8023065116446,43.6543796795797,12.));
#110270=CARTESIAN_POINT('Ctrl Pts',(58.8157307388247,43.6768297296403,0.));
#110271=CARTESIAN_POINT('Ctrl Pts',(58.8157307388247,43.6768297296403,12.));
#110272=CARTESIAN_POINT('Ctrl Pts',(58.8291533925299,43.6993247037318,0.));
#110273=CARTESIAN_POINT('Ctrl Pts',(58.8291533925299,43.6993247037318,12.));
#110274=CARTESIAN_POINT('Ctrl Pts',(58.8425743797325,43.7218645449921,0.));
#110275=CARTESIAN_POINT('Ctrl Pts',(58.8425743797325,43.7218645449921,12.));
#110276=CARTESIAN_POINT('Ctrl Pts',(58.8559936077933,43.7444491966935,0.));
#110277=CARTESIAN_POINT('Ctrl Pts',(58.8559936077933,43.7444491966935,12.));
#110278=CARTESIAN_POINT('Ctrl Pts',(58.8694109844636,43.7670786022392,0.));
#110279=CARTESIAN_POINT('Ctrl Pts',(58.8694109844636,43.7670786022392,12.));
#110280=CARTESIAN_POINT('Ctrl Pts',(58.882826417861,43.7897527051599,0.));
#110281=CARTESIAN_POINT('Ctrl Pts',(58.882826417861,43.7897527051599,12.));
#110282=CARTESIAN_POINT('Ctrl Pts',(58.8962398164486,43.812471449107,0.));
#110283=CARTESIAN_POINT('Ctrl Pts',(58.8962398164486,43.812471449107,12.));
#110284=CARTESIAN_POINT('Ctrl Pts',(58.9096510890128,43.8352347778419,0.));
#110285=CARTESIAN_POINT('Ctrl Pts',(58.9096510890128,43.8352347778419,12.));
#110286=CARTESIAN_POINT('Ctrl Pts',(58.9230601446445,43.8580426352236,0.));
#110287=CARTESIAN_POINT('Ctrl Pts',(58.9230601446445,43.8580426352236,12.));
#110288=CARTESIAN_POINT('Ctrl Pts',(58.9364668927132,43.8808949651882,0.));
#110289=CARTESIAN_POINT('Ctrl Pts',(58.9364668927132,43.8808949651882,12.));
#110290=CARTESIAN_POINT('Ctrl Pts',(58.9498712429066,43.9037917117749,0.));
#110291=CARTESIAN_POINT('Ctrl Pts',(58.9498712429066,43.9037917117749,12.));
#110292=CARTESIAN_POINT('Ctrl Pts',(58.9632731052704,43.9267328191508,0.));
#110293=CARTESIAN_POINT('Ctrl Pts',(58.9632731052704,43.9267328191508,12.));
#110294=CARTESIAN_POINT('Ctrl Pts',(58.9766723902531,43.9497182316333,0.));
#110295=CARTESIAN_POINT('Ctrl Pts',(58.9766723902531,43.9497182316333,12.));
#110296=CARTESIAN_POINT('Ctrl Pts',(58.9900690087404,43.9727478937053,0.));
#110297=CARTESIAN_POINT('Ctrl Pts',(58.9900690087404,43.9727478937053,12.));
#110298=CARTESIAN_POINT('Ctrl Pts',(59.0034628721161,43.9958217500364,0.));
#110299=CARTESIAN_POINT('Ctrl Pts',(59.0034628721161,43.9958217500364,12.));
#110300=CARTESIAN_POINT('Ctrl Pts',(59.0168538922087,44.0189397454593,0.));
#110301=CARTESIAN_POINT('Ctrl Pts',(59.0168538922087,44.0189397454593,12.));
#110302=CARTESIAN_POINT('Ctrl Pts',(59.0302419811772,44.0421018249219,0.));
#110303=CARTESIAN_POINT('Ctrl Pts',(59.0302419811772,44.0421018249219,12.));
#110304=CARTESIAN_POINT('Ctrl Pts',(59.0436270514085,44.0653079334384,0.));
#110305=CARTESIAN_POINT('Ctrl Pts',(59.0436270514085,44.0653079334384,12.));
#110306=CARTESIAN_POINT('Ctrl Pts',(59.0570090154243,44.0885580160433,0.));
#110307=CARTESIAN_POINT('Ctrl Pts',(59.0570090154243,44.0885580160433,12.));
#110308=CARTESIAN_POINT('Ctrl Pts',(59.0703877857529,44.1118520177224,0.));
#110309=CARTESIAN_POINT('Ctrl Pts',(59.0703877857529,44.1118520177224,12.));
#110310=CARTESIAN_POINT('Ctrl Pts',(59.0837632749209,44.1351898834057,0.));
#110311=CARTESIAN_POINT('Ctrl Pts',(59.0837632749209,44.1351898834057,12.));
#110312=CARTESIAN_POINT('Ctrl Pts',(59.0971353957218,44.1585715581074,0.));
#110313=CARTESIAN_POINT('Ctrl Pts',(59.0971353957218,44.1585715581074,12.));
#110314=CARTESIAN_POINT('Ctrl Pts',(59.1105040614285,44.1819969870314,0.));
#110315=CARTESIAN_POINT('Ctrl Pts',(59.1105040614285,44.1819969870314,12.));
#110316=CARTESIAN_POINT('Ctrl Pts',(59.1238691860307,44.2054661156876,0.));
#110317=CARTESIAN_POINT('Ctrl Pts',(59.1238691860307,44.2054661156876,12.));
#110318=CARTESIAN_POINT('Ctrl Pts',(59.1372306844575,44.2289788899962,0.));
#110319=CARTESIAN_POINT('Ctrl Pts',(59.1372306844575,44.2289788899962,12.));
#110320=CARTESIAN_POINT('Ctrl Pts',(59.1505884728194,44.2525352563979,0.));
#110321=CARTESIAN_POINT('Ctrl Pts',(59.1505884728194,44.2525352563979,12.));
#110322=CARTESIAN_POINT('Ctrl Pts',(59.1639424678766,44.2761351616027,0.));
#110323=CARTESIAN_POINT('Ctrl Pts',(59.1639424678766,44.2761351616027,12.));
#110324=CARTESIAN_POINT('Ctrl Pts',(59.1772925865191,44.2997785523413,0.));
#110325=CARTESIAN_POINT('Ctrl Pts',(59.1772925865191,44.2997785523413,12.));
#110326=CARTESIAN_POINT('Ctrl Pts',(59.1906387451971,44.3234653750877,0.));
#110327=CARTESIAN_POINT('Ctrl Pts',(59.1906387451971,44.3234653750877,12.));
#110328=CARTESIAN_POINT('Ctrl Pts',(59.2039808594765,44.3471955758412,0.));
#110329=CARTESIAN_POINT('Ctrl Pts',(59.2039808594765,44.3471955758412,12.));
#110330=CARTESIAN_POINT('Ctrl Pts',(59.217318843283,44.3709690997495,0.));
#110331=CARTESIAN_POINT('Ctrl Pts',(59.217318843283,44.3709690997495,12.));
#110332=CARTESIAN_POINT('Ctrl Pts',(59.2306526095175,44.394785891411,0.));
#110333=CARTESIAN_POINT('Ctrl Pts',(59.2306526095175,44.394785891411,12.));
#110334=CARTESIAN_POINT('Ctrl Pts',(59.2439820714231,44.4186458955486,0.));
#110335=CARTESIAN_POINT('Ctrl Pts',(59.2439820714231,44.4186458955486,12.));
#110336=CARTESIAN_POINT('Ctrl Pts',(59.2573071437801,44.4425490575932,0.));
#110337=CARTESIAN_POINT('Ctrl Pts',(59.2573071437801,44.4425490575932,12.));
#110338=CARTESIAN_POINT('Ctrl Pts',(59.2706277440438,44.4664953242373,0.));
#110339=CARTESIAN_POINT('Ctrl Pts',(59.2706277440438,44.4664953242373,12.));
#110340=CARTESIAN_POINT('Ctrl Pts',(59.2839437938187,44.490484644147,0.));
#110341=CARTESIAN_POINT('Ctrl Pts',(59.2839437938187,44.490484644147,12.));
#110342=CARTESIAN_POINT('Ctrl Pts',(59.2972552192072,44.514516968128,0.));
#110343=CARTESIAN_POINT('Ctrl Pts',(59.2972552192072,44.514516968128,12.));
#110344=CARTESIAN_POINT('Ctrl Pts',(59.3105619475512,44.5385922475494,0.));
#110345=CARTESIAN_POINT('Ctrl Pts',(59.3105619475512,44.5385922475494,12.));
#110346=CARTESIAN_POINT('Ctrl Pts',(59.3238639048618,44.5627104330956,0.));
#110347=CARTESIAN_POINT('Ctrl Pts',(59.3238639048618,44.5627104330956,12.));
#110348=CARTESIAN_POINT('Ctrl Pts',(59.3371610128494,44.586871473322,0.));
#110349=CARTESIAN_POINT('Ctrl Pts',(59.3371610128494,44.586871473322,12.));
#110350=CARTESIAN_POINT('Ctrl Pts',(59.3504531864223,44.6110753134333,0.));
#110351=CARTESIAN_POINT('Ctrl Pts',(59.3504531864223,44.6110753134333,12.));
#110352=CARTESIAN_POINT('Ctrl Pts',(59.3637403301959,44.6353218935813,0.));
#110353=CARTESIAN_POINT('Ctrl Pts',(59.3637403301959,44.6353218935813,12.));
#110354=CARTESIAN_POINT('Ctrl Pts',(59.3770223435405,44.6596111512861,0.));
#110355=CARTESIAN_POINT('Ctrl Pts',(59.3770223435405,44.6596111512861,12.));
#110356=CARTESIAN_POINT('Ctrl Pts',(59.3902991268094,44.6839430244376,0.));
#110357=CARTESIAN_POINT('Ctrl Pts',(59.3902991268094,44.6839430244376,12.));
#110358=CARTESIAN_POINT('Ctrl Pts',(59.403570587392,44.708317454179,0.));
#110359=CARTESIAN_POINT('Ctrl Pts',(59.403570587392,44.708317454179,12.));
#110360=CARTESIAN_POINT('Ctrl Pts',(59.4168366453047,44.7327343876333,0.));
#110361=CARTESIAN_POINT('Ctrl Pts',(59.4168366453047,44.7327343876333,12.));
#110362=CARTESIAN_POINT('Ctrl Pts',(59.4300972402943,44.7571937811872,0.));
#110363=CARTESIAN_POINT('Ctrl Pts',(59.4300972402943,44.7571937811872,12.));
#110364=CARTESIAN_POINT('Ctrl Pts',(59.4433523334651,44.7816956017127,0.));
#110365=CARTESIAN_POINT('Ctrl Pts',(59.4433523334651,44.7816956017127,12.));
#110366=CARTESIAN_POINT('Ctrl Pts',(59.4566019017674,44.8062398250937,0.));
#110367=CARTESIAN_POINT('Ctrl Pts',(59.4566019017674,44.8062398250937,12.));
#110368=CARTESIAN_POINT('Ctrl Pts',(59.4671971277837,44.8259091133624,0.));
#110369=CARTESIAN_POINT('Ctrl Pts',(59.4671971277837,44.8259091133624,12.));
#110370=CARTESIAN_POINT('Ctrl Pts',(59.475141054744,44.8406801497506,0.));
#110371=CARTESIAN_POINT('Ctrl Pts',(59.475141054744,44.8406801497506,12.));
#110372=CARTESIAN_POINT('Ctrl Pts',(59.4804358982977,44.8505359826374,0.));
#110373=CARTESIAN_POINT('Ctrl Pts',(59.4804358982977,44.8505359826374,12.));
#110374=CARTESIAN_POINT('Ctrl Pts',(59.483083043136,44.8554660179045,0.));
#110375=CARTESIAN_POINT('Ctrl Pts',(59.483083043136,44.8554660179045,12.));
#110376=CARTESIAN_POINT('',(56.8466430164621,40.8467768343956,0.));
#110377=CARTESIAN_POINT('Ctrl Pts',(56.8466430164621,40.8467768343956,0.));
#110378=CARTESIAN_POINT('Ctrl Pts',(56.8491101022591,40.8497761671036,0.));
#110379=CARTESIAN_POINT('Ctrl Pts',(56.8540460739472,40.8557803680278,0.));
#110380=CARTESIAN_POINT('Ctrl Pts',(56.8614554317668,40.864803275942,0.));
#110381=CARTESIAN_POINT('Ctrl Pts',(56.8713453764905,40.8768670342052,0.));
#110382=CARTESIAN_POINT('Ctrl Pts',(56.8837257978343,40.8920020903293,0.));
#110383=CARTESIAN_POINT('Ctrl Pts',(56.8961241708861,40.9071924937508,0.));
#110384=CARTESIAN_POINT('Ctrl Pts',(56.9085404164502,40.9224382132427,0.));
#110385=CARTESIAN_POINT('Ctrl Pts',(56.9209743960992,40.9377391857129,0.));
#110386=CARTESIAN_POINT('Ctrl Pts',(56.9334259140049,40.9530953165031,0.));
#110387=CARTESIAN_POINT('Ctrl Pts',(56.9458947422608,40.9685064933074,0.));
#110388=CARTESIAN_POINT('Ctrl Pts',(56.9583806404069,40.9839725967121,0.));
#110389=CARTESIAN_POINT('Ctrl Pts',(56.9708833766137,40.9994935117276,0.));
#110390=CARTESIAN_POINT('Ctrl Pts',(56.9834027500117,41.0150691398947,0.));
#110391=CARTESIAN_POINT('Ctrl Pts',(56.995938583472,41.0306993953989,0.));
#110392=CARTESIAN_POINT('Ctrl Pts',(57.008490713042,41.0463841993608,0.));
#110393=CARTESIAN_POINT('Ctrl Pts',(57.0210589791788,41.0621234751007,0.));
#110394=CARTESIAN_POINT('Ctrl Pts',(57.0336432158536,41.0779171422438,0.));
#110395=CARTESIAN_POINT('Ctrl Pts',(57.046243245068,41.0937651137549,0.));
#110396=CARTESIAN_POINT('Ctrl Pts',(57.0588588825298,41.1096672990148,0.));
#110397=CARTESIAN_POINT('Ctrl Pts',(57.0714899412099,41.1256236057443,0.));
#110398=CARTESIAN_POINT('Ctrl Pts',(57.084136235426,41.1416339422117,0.));
#110399=CARTESIAN_POINT('Ctrl Pts',(57.0967975854874,41.1576982197375,0.));
#110400=CARTESIAN_POINT('Ctrl Pts',(57.1094738174957,41.1738163525902,0.));
#110401=CARTESIAN_POINT('Ctrl Pts',(57.1221647611207,41.1899882567923,0.));
#110402=CARTESIAN_POINT('Ctrl Pts',(57.1348702480647,41.2062138492915,0.));
#110403=CARTESIAN_POINT('Ctrl Pts',(57.147590110182,41.222493046943,0.));
#110404=CARTESIAN_POINT('Ctrl Pts',(57.1603241779077,41.2388257656559,0.));
#110405=CARTESIAN_POINT('Ctrl Pts',(57.17307228108,41.2552119208466,0.));
#110406=CARTESIAN_POINT('Ctrl Pts',(57.1858342496538,41.2716514278276,0.));
#110407=CARTESIAN_POINT('Ctrl Pts',(57.1986099143983,41.2881442021863,0.));
#110408=CARTESIAN_POINT('Ctrl Pts',(57.2113991077302,41.3046901602293,0.));
#110409=CARTESIAN_POINT('Ctrl Pts',(57.2242016640198,41.321289219149,0.));
#110410=CARTESIAN_POINT('Ctrl Pts',(57.2370174191401,41.3379412967875,0.));
#110411=CARTESIAN_POINT('Ctrl Pts',(57.2498462101879,41.3546463114885,0.));
#110412=CARTESIAN_POINT('Ctrl Pts',(57.2626878751596,41.3714041819224,0.));
#110413=CARTESIAN_POINT('Ctrl Pts',(57.2755422525844,41.3882148268814,0.));
#110414=CARTESIAN_POINT('Ctrl Pts',(57.2884091815406,41.4050781652938,0.));
#110415=CARTESIAN_POINT('Ctrl Pts',(57.3012885018151,41.4219941163163,0.));
#110416=CARTESIAN_POINT('Ctrl Pts',(57.3141800540137,41.4389625993948,0.));
#110417=CARTESIAN_POINT('Ctrl Pts',(57.3270836796911,41.4559835343328,0.));
#110418=CARTESIAN_POINT('Ctrl Pts',(57.3399992214717,41.4730568413518,0.));
#110419=CARTESIAN_POINT('Ctrl Pts',(57.3529265229835,41.4901824410637,0.));
#110420=CARTESIAN_POINT('Ctrl Pts',(57.3658654287937,41.5073602544396,0.));
#110421=CARTESIAN_POINT('Ctrl Pts',(57.3788157843454,41.5245902027771,0.));
#110422=CARTESIAN_POINT('Ctrl Pts',(57.3917774358863,41.5418722076572,0.));
#110423=CARTESIAN_POINT('Ctrl Pts',(57.4047502304231,41.5592061909176,0.));
#110424=CARTESIAN_POINT('Ctrl Pts',(57.4177340157508,41.5765920746777,0.));
#110425=CARTESIAN_POINT('Ctrl Pts',(57.4307286404662,41.5940297813477,0.));
#110426=CARTESIAN_POINT('Ctrl Pts',(57.4437339539841,41.6115192336388,0.));
#110427=CARTESIAN_POINT('Ctrl Pts',(57.4567498065562,41.6290603545666,0.));
#110428=CARTESIAN_POINT('Ctrl Pts',(57.4697760492683,41.6466530674515,0.));
#110429=CARTESIAN_POINT('Ctrl Pts',(57.4828125340218,41.6642972959165,0.));
#110430=CARTESIAN_POINT('Ctrl Pts',(57.4958591135165,41.6819929638797,0.));
#110431=CARTESIAN_POINT('Ctrl Pts',(57.5089156412343,41.6997399955447,0.));
#110432=CARTESIAN_POINT('Ctrl Pts',(57.5219819714171,41.7175383153821,0.));
#110433=CARTESIAN_POINT('Ctrl Pts',(57.5350579590649,41.7353878481337,0.));
#110434=CARTESIAN_POINT('Ctrl Pts',(57.5481434599335,41.7532885188175,0.));
#110435=CARTESIAN_POINT('Ctrl Pts',(57.561238330532,41.7712402527273,0.));
#110436=CARTESIAN_POINT('Ctrl Pts',(57.5743424281204,41.7892429754297,0.));
#110437=CARTESIAN_POINT('Ctrl Pts',(57.5874556107056,41.8072966127558,0.));
#110438=CARTESIAN_POINT('Ctrl Pts',(57.6005777370349,41.8254010908051,0.));
#110439=CARTESIAN_POINT('Ctrl Pts',(57.6137086665882,41.8435563359456,0.));
#110440=CARTESIAN_POINT('Ctrl Pts',(57.6268482595702,41.8617622748108,0.));
#110441=CARTESIAN_POINT('Ctrl Pts',(57.6399963769003,41.8800188342909,0.));
#110442=CARTESIAN_POINT('Ctrl Pts',(57.6531528802059,41.8983259415245,0.));
#110443=CARTESIAN_POINT('Ctrl Pts',(57.6663176318176,41.9166835239046,0.));
#110444=CARTESIAN_POINT('Ctrl Pts',(57.6794904947641,41.9350915090791,0.));
#110445=CARTESIAN_POINT('Ctrl Pts',(57.6926713327674,41.9535498249489,0.));
#110446=CARTESIAN_POINT('Ctrl Pts',(57.7058600102365,41.9720583996601,0.));
#110447=CARTESIAN_POINT('Ctrl Pts',(57.7190563922614,41.9906171615975,0.));
#110448=CARTESIAN_POINT('Ctrl Pts',(57.7322603446086,42.0092260393911,0.));
#110449=CARTESIAN_POINT('Ctrl Pts',(57.7454717337151,42.0278849619156,0.));
#110450=CARTESIAN_POINT('Ctrl Pts',(57.7586904266828,42.0465938582878,0.));
#110451=CARTESIAN_POINT('Ctrl Pts',(57.7719162912721,42.0653526578571,0.));
#110452=CARTESIAN_POINT('Ctrl Pts',(57.7851491958954,42.0841612902018,0.));
#110453=CARTESIAN_POINT('Ctrl Pts',(57.798389009613,42.1030196851344,0.));
#110454=CARTESIAN_POINT('Ctrl Pts',(57.8116356021274,42.121927772701,0.));
#110455=CARTESIAN_POINT('Ctrl Pts',(57.8248888437787,42.1408854831792,0.));
#110456=CARTESIAN_POINT('Ctrl Pts',(57.8381486055376,42.1598927470671,0.));
#110457=CARTESIAN_POINT('Ctrl Pts',(57.8514147590012,42.1789494950824,0.));
#110458=CARTESIAN_POINT('Ctrl Pts',(57.86468717639,42.1980556581689,0.));
#110459=CARTESIAN_POINT('Ctrl Pts',(57.8779657305422,42.2172111674946,0.));
#110460=CARTESIAN_POINT('Ctrl Pts',(57.8912502949084,42.2364159544492,0.));
#110461=CARTESIAN_POINT('Ctrl Pts',(57.9045407435447,42.2556699506332,0.));
#110462=CARTESIAN_POINT('Ctrl Pts',(57.9178369511084,42.274973087857,0.));
#110463=CARTESIAN_POINT('Ctrl Pts',(57.9311387928541,42.2943252981471,0.));
#110464=CARTESIAN_POINT('Ctrl Pts',(57.9444461446292,42.3137265137446,0.));
#110465=CARTESIAN_POINT('Ctrl Pts',(57.9577588828693,42.3331766671028,0.));
#110466=CARTESIAN_POINT('Ctrl Pts',(57.9710768845923,42.3526756908764,0.));
#110467=CARTESIAN_POINT('Ctrl Pts',(57.9844000273936,42.3722235179216,0.));
#110468=CARTESIAN_POINT('Ctrl Pts',(57.9977281894437,42.3918200813025,0.));
#110469=CARTESIAN_POINT('Ctrl Pts',(58.011061249483,42.4114653142891,0.));
#110470=CARTESIAN_POINT('Ctrl Pts',(58.0243990868175,42.4311591503551,0.));
#110471=CARTESIAN_POINT('Ctrl Pts',(58.0377415813132,42.4509015231668,0.));
#110472=CARTESIAN_POINT('Ctrl Pts',(58.0510886133917,42.4706923665838,0.));
#110473=CARTESIAN_POINT('Ctrl Pts',(58.064440064027,42.490531614665,0.));
#110474=CARTESIAN_POINT('Ctrl Pts',(58.0777958147404,42.5104192016664,0.));
#110475=CARTESIAN_POINT('Ctrl Pts',(58.0911557475967,42.5303550620388,0.));
#110476=CARTESIAN_POINT('Ctrl Pts',(58.1045197452003,42.5503391304183,0.));
#110477=CARTESIAN_POINT('Ctrl Pts',(58.1178876906905,42.5703713416263,0.));
#110478=CARTESIAN_POINT('Ctrl Pts',(58.1312594677383,42.5904516306759,0.));
#110479=CARTESIAN_POINT('Ctrl Pts',(58.1446349605419,42.6105799327697,0.));
#110480=CARTESIAN_POINT('Ctrl Pts',(58.158014053823,42.6307561832978,0.));
#110481=CARTESIAN_POINT('Ctrl Pts',(58.1713966328217,42.650980317827,0.));
#110482=CARTESIAN_POINT('Ctrl Pts',(58.1847825832932,42.6712522721021,0.));
#110483=CARTESIAN_POINT('Ctrl Pts',(58.1981717915043,42.6915719820517,0.));
#110484=CARTESIAN_POINT('Ctrl Pts',(58.2115641442302,42.7119393837867,0.));
#110485=CARTESIAN_POINT('Ctrl Pts',(58.2249595287497,42.7323544135983,0.));
#110486=CARTESIAN_POINT('Ctrl Pts',(58.238357832842,42.7528170079482,0.));
#110487=CARTESIAN_POINT('Ctrl Pts',(58.2517589447818,42.7733271034679,0.));
#110488=CARTESIAN_POINT('Ctrl Pts',(58.2651627533368,42.7938846369651,0.));
#110489=CARTESIAN_POINT('Ctrl Pts',(58.278569147764,42.8144895454234,0.));
#110490=CARTESIAN_POINT('Ctrl Pts',(58.2919780178063,42.8351417659998,0.));
#110491=CARTESIAN_POINT('Ctrl Pts',(58.305389253689,42.8558412360154,0.));
#110492=CARTESIAN_POINT('Ctrl Pts',(58.3188027461157,42.8765878929545,0.));
#110493=CARTESIAN_POINT('Ctrl Pts',(58.3322183862647,42.8973816744703,0.));
#110494=CARTESIAN_POINT('Ctrl Pts',(58.3456360657861,42.9182225183851,0.));
#110495=CARTESIAN_POINT('Ctrl Pts',(58.3590556767981,42.9391103626881,0.));
#110496=CARTESIAN_POINT('Ctrl Pts',(58.3724771118835,42.9600451455267,0.));
#110497=CARTESIAN_POINT('Ctrl Pts',(58.3859002640871,42.9810268052043,0.));
#110498=CARTESIAN_POINT('Ctrl Pts',(58.3993250269115,43.002055280187,0.));
#110499=CARTESIAN_POINT('Ctrl Pts',(58.4127512943144,43.0231305091033,0.));
#110500=CARTESIAN_POINT('Ctrl Pts',(58.4261789607055,43.0442524307432,0.));
#110501=CARTESIAN_POINT('Ctrl Pts',(58.4396079209438,43.0654209840502,0.));
#110502=CARTESIAN_POINT('Ctrl Pts',(58.4530380703335,43.0866361081166,0.));
#110503=CARTESIAN_POINT('Ctrl Pts',(58.4664693046206,43.1078977421908,0.));
#110504=CARTESIAN_POINT('Ctrl Pts',(58.4799015199904,43.1292058256774,0.));
#110505=CARTESIAN_POINT('Ctrl Pts',(58.4933346130638,43.1505602981366,0.));
#110506=CARTESIAN_POINT('Ctrl Pts',(58.5067684808946,43.1719610992772,0.));
#110507=CARTESIAN_POINT('Ctrl Pts',(58.5202030209667,43.1934081689504,0.));
#110508=CARTESIAN_POINT('Ctrl Pts',(58.5336381311911,43.214901447157,0.));
#110509=CARTESIAN_POINT('Ctrl Pts',(58.5470737099027,43.2364408740489,0.));
#110510=CARTESIAN_POINT('Ctrl Pts',(58.5605096558578,43.2580263899278,0.));
#110511=CARTESIAN_POINT('Ctrl Pts',(58.5739458682317,43.2796579352405,0.));
#110512=CARTESIAN_POINT('Ctrl Pts',(58.5873822466163,43.3013354505708,0.));
#110513=CARTESIAN_POINT('Ctrl Pts',(58.6008186910166,43.3230588766456,0.));
#110514=CARTESIAN_POINT('Ctrl Pts',(58.6142551018473,43.3448281543375,0.));
#110515=CARTESIAN_POINT('Ctrl Pts',(58.627691379929,43.3666432246635,0.));
#110516=CARTESIAN_POINT('Ctrl Pts',(58.6411274264854,43.3885040287808,0.));
#110517=CARTESIAN_POINT('Ctrl Pts',(58.6545631431388,43.4104105079766,0.));
#110518=CARTESIAN_POINT('Ctrl Pts',(58.6679984319095,43.4323626036736,0.));
#110519=CARTESIAN_POINT('Ctrl Pts',(58.6814331952138,43.4543602574352,0.));
#110520=CARTESIAN_POINT('Ctrl Pts',(58.6948673358639,43.4764034109655,0.));
#110521=CARTESIAN_POINT('Ctrl Pts',(58.708300757066,43.4984920061071,0.));
#110522=CARTESIAN_POINT('Ctrl Pts',(58.7217333624206,43.5206259848333,0.));
#110523=CARTESIAN_POINT('Ctrl Pts',(58.7351650559176,43.5428052892483,0.));
#110524=CARTESIAN_POINT('Ctrl Pts',(58.7485957419296,43.5650298615912,0.));
#110525=CARTESIAN_POINT('Ctrl Pts',(58.7620253252059,43.5872996442343,0.));
#110526=CARTESIAN_POINT('Ctrl Pts',(58.7754537108672,43.6096145796798,0.));
#110527=CARTESIAN_POINT('Ctrl Pts',(58.7888808043976,43.6319746105488,0.));
#110528=CARTESIAN_POINT('Ctrl Pts',(58.8023065116446,43.6543796795797,0.));
#110529=CARTESIAN_POINT('Ctrl Pts',(58.8157307388247,43.6768297296403,0.));
#110530=CARTESIAN_POINT('Ctrl Pts',(58.8291533925299,43.6993247037318,0.));
#110531=CARTESIAN_POINT('Ctrl Pts',(58.8425743797325,43.7218645449921,0.));
#110532=CARTESIAN_POINT('Ctrl Pts',(58.8559936077933,43.7444491966935,0.));
#110533=CARTESIAN_POINT('Ctrl Pts',(58.8694109844636,43.7670786022392,0.));
#110534=CARTESIAN_POINT('Ctrl Pts',(58.882826417861,43.7897527051599,0.));
#110535=CARTESIAN_POINT('Ctrl Pts',(58.8962398164486,43.812471449107,0.));
#110536=CARTESIAN_POINT('Ctrl Pts',(58.9096510890128,43.8352347778419,0.));
#110537=CARTESIAN_POINT('Ctrl Pts',(58.9230601446445,43.8580426352236,0.));
#110538=CARTESIAN_POINT('Ctrl Pts',(58.9364668927132,43.8808949651882,0.));
#110539=CARTESIAN_POINT('Ctrl Pts',(58.9498712429066,43.9037917117749,0.));
#110540=CARTESIAN_POINT('Ctrl Pts',(58.9632731052704,43.9267328191508,0.));
#110541=CARTESIAN_POINT('Ctrl Pts',(58.9766723902531,43.9497182316333,0.));
#110542=CARTESIAN_POINT('Ctrl Pts',(58.9900690087404,43.9727478937053,0.));
#110543=CARTESIAN_POINT('Ctrl Pts',(59.0034628721161,43.9958217500364,0.));
#110544=CARTESIAN_POINT('Ctrl Pts',(59.0168538922087,44.0189397454593,0.));
#110545=CARTESIAN_POINT('Ctrl Pts',(59.0302419811772,44.0421018249219,0.));
#110546=CARTESIAN_POINT('Ctrl Pts',(59.0436270514085,44.0653079334384,0.));
#110547=CARTESIAN_POINT('Ctrl Pts',(59.0570090154243,44.0885580160433,0.));
#110548=CARTESIAN_POINT('Ctrl Pts',(59.0703877857529,44.1118520177224,0.));
#110549=CARTESIAN_POINT('Ctrl Pts',(59.0837632749209,44.1351898834057,0.));
#110550=CARTESIAN_POINT('Ctrl Pts',(59.0971353957218,44.1585715581074,0.));
#110551=CARTESIAN_POINT('Ctrl Pts',(59.1105040614285,44.1819969870314,0.));
#110552=CARTESIAN_POINT('Ctrl Pts',(59.1238691860307,44.2054661156876,0.));
#110553=CARTESIAN_POINT('Ctrl Pts',(59.1372306844575,44.2289788899962,0.));
#110554=CARTESIAN_POINT('Ctrl Pts',(59.1505884728194,44.2525352563979,0.));
#110555=CARTESIAN_POINT('Ctrl Pts',(59.1639424678766,44.2761351616027,0.));
#110556=CARTESIAN_POINT('Ctrl Pts',(59.1772925865191,44.2997785523413,0.));
#110557=CARTESIAN_POINT('Ctrl Pts',(59.1906387451971,44.3234653750877,0.));
#110558=CARTESIAN_POINT('Ctrl Pts',(59.2039808594765,44.3471955758412,0.));
#110559=CARTESIAN_POINT('Ctrl Pts',(59.217318843283,44.3709690997495,0.));
#110560=CARTESIAN_POINT('Ctrl Pts',(59.2306526095175,44.394785891411,0.));
#110561=CARTESIAN_POINT('Ctrl Pts',(59.2439820714231,44.4186458955486,0.));
#110562=CARTESIAN_POINT('Ctrl Pts',(59.2573071437801,44.4425490575932,0.));
#110563=CARTESIAN_POINT('Ctrl Pts',(59.2706277440438,44.4664953242373,0.));
#110564=CARTESIAN_POINT('Ctrl Pts',(59.2839437938187,44.490484644147,0.));
#110565=CARTESIAN_POINT('Ctrl Pts',(59.2972552192072,44.514516968128,0.));
#110566=CARTESIAN_POINT('Ctrl Pts',(59.3086616639392,44.5351541478336,0.));
#110567=CARTESIAN_POINT('Ctrl Pts',(59.317404187219,44.5509994357954,0.));
#110568=CARTESIAN_POINT('Ctrl Pts',(59.3234848865279,44.5620338188487,0.));
#110569=CARTESIAN_POINT('Ctrl Pts',(59.3269051738223,44.5682447395714,0.));
#110570=CARTESIAN_POINT('Ctrl Pts',(59.3276657444159,44.5696260757422,0.));
#110571=CARTESIAN_POINT('',(56.8466430164621,40.8467768343956,12.));
#110572=CARTESIAN_POINT('',(56.8466430164621,40.8467768343956,0.));
#110573=CARTESIAN_POINT('Ctrl Pts',(59.3276657444159,44.5696260757422,12.));
#110574=CARTESIAN_POINT('Ctrl Pts',(59.3269051738223,44.5682447395714,12.));
#110575=CARTESIAN_POINT('Ctrl Pts',(59.3234848865279,44.5620338188486,12.));
#110576=CARTESIAN_POINT('Ctrl Pts',(59.317404187219,44.5509994357954,12.));
#110577=CARTESIAN_POINT('Ctrl Pts',(59.3086616639392,44.5351541478336,12.));
#110578=CARTESIAN_POINT('Ctrl Pts',(59.2972552192072,44.514516968128,12.));
#110579=CARTESIAN_POINT('Ctrl Pts',(59.2839437938187,44.490484644147,12.));
#110580=CARTESIAN_POINT('Ctrl Pts',(59.2706277440438,44.4664953242373,12.));
#110581=CARTESIAN_POINT('Ctrl Pts',(59.2573071437801,44.4425490575932,12.));
#110582=CARTESIAN_POINT('Ctrl Pts',(59.2439820714231,44.4186458955486,12.));
#110583=CARTESIAN_POINT('Ctrl Pts',(59.2306526095175,44.394785891411,12.));
#110584=CARTESIAN_POINT('Ctrl Pts',(59.217318843283,44.3709690997495,12.));
#110585=CARTESIAN_POINT('Ctrl Pts',(59.2039808594765,44.3471955758412,12.));
#110586=CARTESIAN_POINT('Ctrl Pts',(59.1906387451971,44.3234653750877,12.));
#110587=CARTESIAN_POINT('Ctrl Pts',(59.1772925865191,44.2997785523413,12.));
#110588=CARTESIAN_POINT('Ctrl Pts',(59.1639424678766,44.2761351616027,12.));
#110589=CARTESIAN_POINT('Ctrl Pts',(59.1505884728194,44.2525352563979,12.));
#110590=CARTESIAN_POINT('Ctrl Pts',(59.1372306844575,44.2289788899962,12.));
#110591=CARTESIAN_POINT('Ctrl Pts',(59.1238691860307,44.2054661156876,12.));
#110592=CARTESIAN_POINT('Ctrl Pts',(59.1105040614285,44.1819969870314,12.));
#110593=CARTESIAN_POINT('Ctrl Pts',(59.0971353957218,44.1585715581074,12.));
#110594=CARTESIAN_POINT('Ctrl Pts',(59.0837632749209,44.1351898834057,12.));
#110595=CARTESIAN_POINT('Ctrl Pts',(59.0703877857529,44.1118520177224,12.));
#110596=CARTESIAN_POINT('Ctrl Pts',(59.0570090154243,44.0885580160433,12.));
#110597=CARTESIAN_POINT('Ctrl Pts',(59.0436270514085,44.0653079334384,12.));
#110598=CARTESIAN_POINT('Ctrl Pts',(59.0302419811772,44.0421018249219,12.));
#110599=CARTESIAN_POINT('Ctrl Pts',(59.0168538922087,44.0189397454593,12.));
#110600=CARTESIAN_POINT('Ctrl Pts',(59.0034628721161,43.9958217500364,12.));
#110601=CARTESIAN_POINT('Ctrl Pts',(58.9900690087404,43.9727478937053,12.));
#110602=CARTESIAN_POINT('Ctrl Pts',(58.9766723902531,43.9497182316333,12.));
#110603=CARTESIAN_POINT('Ctrl Pts',(58.9632731052704,43.9267328191508,12.));
#110604=CARTESIAN_POINT('Ctrl Pts',(58.9498712429066,43.9037917117749,12.));
#110605=CARTESIAN_POINT('Ctrl Pts',(58.9364668927132,43.8808949651882,12.));
#110606=CARTESIAN_POINT('Ctrl Pts',(58.9230601446445,43.8580426352236,12.));
#110607=CARTESIAN_POINT('Ctrl Pts',(58.9096510890128,43.8352347778419,12.));
#110608=CARTESIAN_POINT('Ctrl Pts',(58.8962398164486,43.812471449107,12.));
#110609=CARTESIAN_POINT('Ctrl Pts',(58.882826417861,43.7897527051599,12.));
#110610=CARTESIAN_POINT('Ctrl Pts',(58.8694109844636,43.7670786022392,12.));
#110611=CARTESIAN_POINT('Ctrl Pts',(58.8559936077933,43.7444491966935,12.));
#110612=CARTESIAN_POINT('Ctrl Pts',(58.8425743797325,43.7218645449921,12.));
#110613=CARTESIAN_POINT('Ctrl Pts',(58.8291533925299,43.6993247037318,12.));
#110614=CARTESIAN_POINT('Ctrl Pts',(58.8157307388247,43.6768297296403,12.));
#110615=CARTESIAN_POINT('Ctrl Pts',(58.8023065116446,43.6543796795797,12.));
#110616=CARTESIAN_POINT('Ctrl Pts',(58.7888808043976,43.6319746105488,12.));
#110617=CARTESIAN_POINT('Ctrl Pts',(58.7754537108672,43.6096145796798,12.));
#110618=CARTESIAN_POINT('Ctrl Pts',(58.7620253252059,43.5872996442343,12.));
#110619=CARTESIAN_POINT('Ctrl Pts',(58.7485957419296,43.5650298615912,12.));
#110620=CARTESIAN_POINT('Ctrl Pts',(58.7351650559176,43.5428052892483,12.));
#110621=CARTESIAN_POINT('Ctrl Pts',(58.7217333624206,43.5206259848333,12.));
#110622=CARTESIAN_POINT('Ctrl Pts',(58.708300757066,43.4984920061071,12.));
#110623=CARTESIAN_POINT('Ctrl Pts',(58.6948673358639,43.4764034109655,12.));
#110624=CARTESIAN_POINT('Ctrl Pts',(58.6814331952138,43.4543602574352,12.));
#110625=CARTESIAN_POINT('Ctrl Pts',(58.6679984319095,43.4323626036736,12.));
#110626=CARTESIAN_POINT('Ctrl Pts',(58.6545631431388,43.4104105079766,12.));
#110627=CARTESIAN_POINT('Ctrl Pts',(58.6411274264854,43.3885040287808,12.));
#110628=CARTESIAN_POINT('Ctrl Pts',(58.627691379929,43.3666432246635,12.));
#110629=CARTESIAN_POINT('Ctrl Pts',(58.6142551018473,43.3448281543375,12.));
#110630=CARTESIAN_POINT('Ctrl Pts',(58.6008186910166,43.3230588766456,12.));
#110631=CARTESIAN_POINT('Ctrl Pts',(58.5873822466163,43.3013354505708,12.));
#110632=CARTESIAN_POINT('Ctrl Pts',(58.5739458682317,43.2796579352405,12.));
#110633=CARTESIAN_POINT('Ctrl Pts',(58.5605096558578,43.2580263899278,12.));
#110634=CARTESIAN_POINT('Ctrl Pts',(58.5470737099027,43.2364408740489,12.));
#110635=CARTESIAN_POINT('Ctrl Pts',(58.5336381311911,43.214901447157,12.));
#110636=CARTESIAN_POINT('Ctrl Pts',(58.5202030209667,43.1934081689504,12.));
#110637=CARTESIAN_POINT('Ctrl Pts',(58.5067684808946,43.1719610992772,12.));
#110638=CARTESIAN_POINT('Ctrl Pts',(58.4933346130638,43.1505602981366,12.));
#110639=CARTESIAN_POINT('Ctrl Pts',(58.4799015199904,43.1292058256774,12.));
#110640=CARTESIAN_POINT('Ctrl Pts',(58.4664693046206,43.1078977421908,12.));
#110641=CARTESIAN_POINT('Ctrl Pts',(58.4530380703335,43.0866361081166,12.));
#110642=CARTESIAN_POINT('Ctrl Pts',(58.4396079209438,43.0654209840502,12.));
#110643=CARTESIAN_POINT('Ctrl Pts',(58.4261789607055,43.0442524307432,12.));
#110644=CARTESIAN_POINT('Ctrl Pts',(58.4127512943144,43.0231305091033,12.));
#110645=CARTESIAN_POINT('Ctrl Pts',(58.3993250269115,43.002055280187,12.));
#110646=CARTESIAN_POINT('Ctrl Pts',(58.3859002640871,42.9810268052043,12.));
#110647=CARTESIAN_POINT('Ctrl Pts',(58.3724771118835,42.9600451455267,12.));
#110648=CARTESIAN_POINT('Ctrl Pts',(58.3590556767981,42.9391103626881,12.));
#110649=CARTESIAN_POINT('Ctrl Pts',(58.3456360657861,42.9182225183851,12.));
#110650=CARTESIAN_POINT('Ctrl Pts',(58.3322183862647,42.8973816744703,12.));
#110651=CARTESIAN_POINT('Ctrl Pts',(58.3188027461157,42.8765878929545,12.));
#110652=CARTESIAN_POINT('Ctrl Pts',(58.305389253689,42.8558412360154,12.));
#110653=CARTESIAN_POINT('Ctrl Pts',(58.2919780178063,42.8351417659998,12.));
#110654=CARTESIAN_POINT('Ctrl Pts',(58.278569147764,42.8144895454234,12.));
#110655=CARTESIAN_POINT('Ctrl Pts',(58.2651627533368,42.7938846369651,12.));
#110656=CARTESIAN_POINT('Ctrl Pts',(58.2517589447818,42.7733271034679,12.));
#110657=CARTESIAN_POINT('Ctrl Pts',(58.238357832842,42.7528170079482,12.));
#110658=CARTESIAN_POINT('Ctrl Pts',(58.2249595287497,42.7323544135983,12.));
#110659=CARTESIAN_POINT('Ctrl Pts',(58.2115641442302,42.7119393837867,12.));
#110660=CARTESIAN_POINT('Ctrl Pts',(58.1981717915043,42.6915719820517,12.));
#110661=CARTESIAN_POINT('Ctrl Pts',(58.1847825832932,42.6712522721021,12.));
#110662=CARTESIAN_POINT('Ctrl Pts',(58.1713966328217,42.650980317827,12.));
#110663=CARTESIAN_POINT('Ctrl Pts',(58.158014053823,42.6307561832978,12.));
#110664=CARTESIAN_POINT('Ctrl Pts',(58.1446349605419,42.6105799327697,12.));
#110665=CARTESIAN_POINT('Ctrl Pts',(58.1312594677383,42.5904516306759,12.));
#110666=CARTESIAN_POINT('Ctrl Pts',(58.1178876906905,42.5703713416263,12.));
#110667=CARTESIAN_POINT('Ctrl Pts',(58.1045197452003,42.5503391304183,12.));
#110668=CARTESIAN_POINT('Ctrl Pts',(58.0911557475967,42.5303550620388,12.));
#110669=CARTESIAN_POINT('Ctrl Pts',(58.0777958147404,42.5104192016664,12.));
#110670=CARTESIAN_POINT('Ctrl Pts',(58.064440064027,42.490531614665,12.));
#110671=CARTESIAN_POINT('Ctrl Pts',(58.0510886133917,42.4706923665838,12.));
#110672=CARTESIAN_POINT('Ctrl Pts',(58.0377415813132,42.4509015231668,12.));
#110673=CARTESIAN_POINT('Ctrl Pts',(58.0243990868175,42.4311591503551,12.));
#110674=CARTESIAN_POINT('Ctrl Pts',(58.011061249483,42.4114653142891,12.));
#110675=CARTESIAN_POINT('Ctrl Pts',(57.9977281894437,42.3918200813025,12.));
#110676=CARTESIAN_POINT('Ctrl Pts',(57.9844000273936,42.3722235179216,12.));
#110677=CARTESIAN_POINT('Ctrl Pts',(57.9710768845923,42.3526756908764,12.));
#110678=CARTESIAN_POINT('Ctrl Pts',(57.9577588828693,42.3331766671028,12.));
#110679=CARTESIAN_POINT('Ctrl Pts',(57.9444461446292,42.3137265137446,12.));
#110680=CARTESIAN_POINT('Ctrl Pts',(57.9311387928541,42.2943252981471,12.));
#110681=CARTESIAN_POINT('Ctrl Pts',(57.9178369511084,42.274973087857,12.));
#110682=CARTESIAN_POINT('Ctrl Pts',(57.9045407435447,42.2556699506332,12.));
#110683=CARTESIAN_POINT('Ctrl Pts',(57.8912502949084,42.2364159544492,12.));
#110684=CARTESIAN_POINT('Ctrl Pts',(57.8779657305422,42.2172111674946,12.));
#110685=CARTESIAN_POINT('Ctrl Pts',(57.86468717639,42.1980556581689,12.));
#110686=CARTESIAN_POINT('Ctrl Pts',(57.8514147590012,42.1789494950824,12.));
#110687=CARTESIAN_POINT('Ctrl Pts',(57.8381486055376,42.1598927470671,12.));
#110688=CARTESIAN_POINT('Ctrl Pts',(57.8248888437787,42.1408854831792,12.));
#110689=CARTESIAN_POINT('Ctrl Pts',(57.8116356021274,42.121927772701,12.));
#110690=CARTESIAN_POINT('Ctrl Pts',(57.798389009613,42.1030196851344,12.));
#110691=CARTESIAN_POINT('Ctrl Pts',(57.7851491958954,42.0841612902018,12.));
#110692=CARTESIAN_POINT('Ctrl Pts',(57.7719162912721,42.0653526578571,12.));
#110693=CARTESIAN_POINT('Ctrl Pts',(57.7586904266828,42.0465938582878,12.));
#110694=CARTESIAN_POINT('Ctrl Pts',(57.7454717337151,42.0278849619156,12.));
#110695=CARTESIAN_POINT('Ctrl Pts',(57.7322603446086,42.0092260393911,12.));
#110696=CARTESIAN_POINT('Ctrl Pts',(57.7190563922614,41.9906171615975,12.));
#110697=CARTESIAN_POINT('Ctrl Pts',(57.7058600102365,41.9720583996601,12.));
#110698=CARTESIAN_POINT('Ctrl Pts',(57.6926713327674,41.9535498249489,12.));
#110699=CARTESIAN_POINT('Ctrl Pts',(57.6794904947641,41.9350915090791,12.));
#110700=CARTESIAN_POINT('Ctrl Pts',(57.6663176318176,41.9166835239046,12.));
#110701=CARTESIAN_POINT('Ctrl Pts',(57.6531528802059,41.8983259415245,12.));
#110702=CARTESIAN_POINT('Ctrl Pts',(57.6399963769003,41.8800188342909,12.));
#110703=CARTESIAN_POINT('Ctrl Pts',(57.6268482595702,41.8617622748108,12.));
#110704=CARTESIAN_POINT('Ctrl Pts',(57.6137086665882,41.8435563359456,12.));
#110705=CARTESIAN_POINT('Ctrl Pts',(57.6005777370349,41.8254010908051,12.));
#110706=CARTESIAN_POINT('Ctrl Pts',(57.5874556107056,41.8072966127558,12.));
#110707=CARTESIAN_POINT('Ctrl Pts',(57.5743424281204,41.7892429754297,12.));
#110708=CARTESIAN_POINT('Ctrl Pts',(57.561238330532,41.7712402527273,12.));
#110709=CARTESIAN_POINT('Ctrl Pts',(57.5481434599335,41.7532885188175,12.));
#110710=CARTESIAN_POINT('Ctrl Pts',(57.5350579590649,41.7353878481337,12.));
#110711=CARTESIAN_POINT('Ctrl Pts',(57.5219819714171,41.7175383153821,12.));
#110712=CARTESIAN_POINT('Ctrl Pts',(57.5089156412343,41.6997399955447,12.));
#110713=CARTESIAN_POINT('Ctrl Pts',(57.4958591135165,41.6819929638797,12.));
#110714=CARTESIAN_POINT('Ctrl Pts',(57.4828125340218,41.6642972959165,12.));
#110715=CARTESIAN_POINT('Ctrl Pts',(57.4697760492683,41.6466530674515,12.));
#110716=CARTESIAN_POINT('Ctrl Pts',(57.4567498065562,41.6290603545666,12.));
#110717=CARTESIAN_POINT('Ctrl Pts',(57.4437339539841,41.6115192336388,12.));
#110718=CARTESIAN_POINT('Ctrl Pts',(57.4307286404662,41.5940297813477,12.));
#110719=CARTESIAN_POINT('Ctrl Pts',(57.4177340157508,41.5765920746777,12.));
#110720=CARTESIAN_POINT('Ctrl Pts',(57.4047502304231,41.5592061909176,12.));
#110721=CARTESIAN_POINT('Ctrl Pts',(57.3917774358863,41.5418722076572,12.));
#110722=CARTESIAN_POINT('Ctrl Pts',(57.3788157843454,41.5245902027771,12.));
#110723=CARTESIAN_POINT('Ctrl Pts',(57.3658654287937,41.5073602544396,12.));
#110724=CARTESIAN_POINT('Ctrl Pts',(57.3529265229835,41.4901824410637,12.));
#110725=CARTESIAN_POINT('Ctrl Pts',(57.3399992214717,41.4730568413518,12.));
#110726=CARTESIAN_POINT('Ctrl Pts',(57.3270836796911,41.4559835343328,12.));
#110727=CARTESIAN_POINT('Ctrl Pts',(57.3141800540137,41.4389625993948,12.));
#110728=CARTESIAN_POINT('Ctrl Pts',(57.3012885018151,41.4219941163163,12.));
#110729=CARTESIAN_POINT('Ctrl Pts',(57.2884091815406,41.4050781652938,12.));
#110730=CARTESIAN_POINT('Ctrl Pts',(57.2755422525844,41.3882148268814,12.));
#110731=CARTESIAN_POINT('Ctrl Pts',(57.2626878751596,41.3714041819224,12.));
#110732=CARTESIAN_POINT('Ctrl Pts',(57.2498462101879,41.3546463114885,12.));
#110733=CARTESIAN_POINT('Ctrl Pts',(57.2370174191401,41.3379412967875,12.));
#110734=CARTESIAN_POINT('Ctrl Pts',(57.2242016640198,41.321289219149,12.));
#110735=CARTESIAN_POINT('Ctrl Pts',(57.2113991077302,41.3046901602293,12.));
#110736=CARTESIAN_POINT('Ctrl Pts',(57.1986099143983,41.2881442021863,12.));
#110737=CARTESIAN_POINT('Ctrl Pts',(57.1858342496538,41.2716514278276,12.));
#110738=CARTESIAN_POINT('Ctrl Pts',(57.17307228108,41.2552119208466,12.));
#110739=CARTESIAN_POINT('Ctrl Pts',(57.1603241779077,41.2388257656559,12.));
#110740=CARTESIAN_POINT('Ctrl Pts',(57.147590110182,41.222493046943,12.));
#110741=CARTESIAN_POINT('Ctrl Pts',(57.1348702480647,41.2062138492915,12.));
#110742=CARTESIAN_POINT('Ctrl Pts',(57.1221647611207,41.1899882567923,12.));
#110743=CARTESIAN_POINT('Ctrl Pts',(57.1094738174957,41.1738163525902,12.));
#110744=CARTESIAN_POINT('Ctrl Pts',(57.0967975854874,41.1576982197375,12.));
#110745=CARTESIAN_POINT('Ctrl Pts',(57.084136235426,41.1416339422117,12.));
#110746=CARTESIAN_POINT('Ctrl Pts',(57.0714899412099,41.1256236057443,12.));
#110747=CARTESIAN_POINT('Ctrl Pts',(57.0588588825298,41.1096672990148,12.));
#110748=CARTESIAN_POINT('Ctrl Pts',(57.046243245068,41.0937651137549,12.));
#110749=CARTESIAN_POINT('Ctrl Pts',(57.0336432158536,41.0779171422438,12.));
#110750=CARTESIAN_POINT('Ctrl Pts',(57.0210589791788,41.0621234751007,12.));
#110751=CARTESIAN_POINT('Ctrl Pts',(57.008490713042,41.0463841993608,12.));
#110752=CARTESIAN_POINT('Ctrl Pts',(56.995938583472,41.0306993953989,12.));
#110753=CARTESIAN_POINT('Ctrl Pts',(56.9834027500117,41.0150691398947,12.));
#110754=CARTESIAN_POINT('Ctrl Pts',(56.9708833766137,40.9994935117276,12.));
#110755=CARTESIAN_POINT('Ctrl Pts',(56.9583806404069,40.9839725967121,12.));
#110756=CARTESIAN_POINT('Ctrl Pts',(56.9458947422608,40.9685064933074,12.));
#110757=CARTESIAN_POINT('Ctrl Pts',(56.9334259140049,40.9530953165031,12.));
#110758=CARTESIAN_POINT('Ctrl Pts',(56.9209743960992,40.9377391857129,12.));
#110759=CARTESIAN_POINT('Ctrl Pts',(56.9085404164502,40.9224382132427,12.));
#110760=CARTESIAN_POINT('Ctrl Pts',(56.8961241708861,40.9071924937508,12.));
#110761=CARTESIAN_POINT('Ctrl Pts',(56.8837257978343,40.8920020903293,12.));
#110762=CARTESIAN_POINT('Ctrl Pts',(56.8713453764905,40.8768670342052,12.));
#110763=CARTESIAN_POINT('Ctrl Pts',(56.8614554317668,40.864803275942,12.));
#110764=CARTESIAN_POINT('Ctrl Pts',(56.8540460739472,40.8557803680278,12.));
#110765=CARTESIAN_POINT('Ctrl Pts',(56.8491101022591,40.8497761671036,12.));
#110766=CARTESIAN_POINT('Ctrl Pts',(56.8466430164621,40.8467768343956,12.));
#110767=CARTESIAN_POINT('Ctrl Pts',(58.4060826907792,45.7706564944895,-5.55111512312578E-16));
#110768=CARTESIAN_POINT('Ctrl Pts',(58.4060826907792,45.7706564944895,4.));
#110769=CARTESIAN_POINT('Ctrl Pts',(58.4060826907792,45.7706564944895,8.));
#110770=CARTESIAN_POINT('Ctrl Pts',(58.4060826907792,45.7706564944895,12.));
#110771=CARTESIAN_POINT('Ctrl Pts',(58.5127761886842,45.7969367893064,-5.55111512312578E-16));
#110772=CARTESIAN_POINT('Ctrl Pts',(58.5127761886842,45.7969367893064,4.));
#110773=CARTESIAN_POINT('Ctrl Pts',(58.5127761886843,45.7969367893065,8.00000000000001));
#110774=CARTESIAN_POINT('Ctrl Pts',(58.5127761886843,45.7969367893065,12.));
#110775=CARTESIAN_POINT('Ctrl Pts',(58.7146322050558,45.7788617791412,-5.55111512312578E-16));
#110776=CARTESIAN_POINT('Ctrl Pts',(58.7146322050558,45.7788617791412,4.));
#110777=CARTESIAN_POINT('Ctrl Pts',(58.7146322050559,45.7788617791413,7.99999999999999));
#110778=CARTESIAN_POINT('Ctrl Pts',(58.7146322050559,45.7788617791413,12.));
#110779=CARTESIAN_POINT('Ctrl Pts',(58.870677144318,45.6563266621664,-5.55111512312578E-16));
#110780=CARTESIAN_POINT('Ctrl Pts',(58.870677144318,45.6563266621664,4.));
#110781=CARTESIAN_POINT('Ctrl Pts',(58.870677144318,45.6563266621664,8.00000000000001));
#110782=CARTESIAN_POINT('Ctrl Pts',(58.870677144318,45.6563266621664,12.));
#110783=CARTESIAN_POINT('Ctrl Pts',(58.9211100416379,45.5911481700253,-5.55111512312578E-16));
#110784=CARTESIAN_POINT('Ctrl Pts',(58.9211100416379,45.5911481700253,4.));
#110785=CARTESIAN_POINT('Ctrl Pts',(58.9211100416379,45.5911481700253,8.));
#110786=CARTESIAN_POINT('Ctrl Pts',(58.9211100416379,45.5911481700253,12.));
#110787=CARTESIAN_POINT('',(58.4060826907792,45.7706564944895,2.77555756156289E-16));
#110788=CARTESIAN_POINT('',(58.9211100416379,45.5911481700253,0.));
#110789=CARTESIAN_POINT('Ctrl Pts',(58.4060826907792,45.7706564944895,-1.38777878078145E-16));
#110790=CARTESIAN_POINT('Ctrl Pts',(58.5127761886842,45.7969367893064,-1.38777878078145E-16));
#110791=CARTESIAN_POINT('Ctrl Pts',(58.6281224837537,45.7866082120692,-1.38777878078144E-16));
#110792=CARTESIAN_POINT('Ctrl Pts',(58.7285100597671,45.7421702122002,-1.38777878078145E-16));
#110793=CARTESIAN_POINT('Ctrl Pts',(58.8038007417771,45.7088417122985,-1.38777878078145E-16));
#110794=CARTESIAN_POINT('Ctrl Pts',(58.870677144318,45.6563266621664,-1.38777878078145E-16));
#110795=CARTESIAN_POINT('Ctrl Pts',(58.9211100416379,45.5911481700253,-1.38777878078145E-16));
#110796=CARTESIAN_POINT('',(58.9211100416379,45.5911481700253,12.));
#110797=CARTESIAN_POINT('Ctrl Pts',(58.9211100416379,45.5911481700253,-5.55111512312578E-16));
#110798=CARTESIAN_POINT('Ctrl Pts',(58.9211100416379,45.5911481700253,4.));
#110799=CARTESIAN_POINT('Ctrl Pts',(58.9211100416379,45.5911481700253,8.));
#110800=CARTESIAN_POINT('Ctrl Pts',(58.9211100416379,45.5911481700253,12.));
#110801=CARTESIAN_POINT('',(58.4060826907792,45.7706564944895,12.));
#110802=CARTESIAN_POINT('Ctrl Pts',(58.9211100416379,45.5911481700253,12.));
#110803=CARTESIAN_POINT('Ctrl Pts',(58.870677144318,45.6563266621664,12.));
#110804=CARTESIAN_POINT('Ctrl Pts',(58.8038007417771,45.7088417122985,12.));
#110805=CARTESIAN_POINT('Ctrl Pts',(58.7285100597671,45.7421702122002,12.));
#110806=CARTESIAN_POINT('Ctrl Pts',(58.6281224837538,45.7866082120692,12.));
#110807=CARTESIAN_POINT('Ctrl Pts',(58.5127761886843,45.7969367893065,12.));
#110808=CARTESIAN_POINT('Ctrl Pts',(58.4060826907792,45.7706564944895,12.));
#110809=CARTESIAN_POINT('Ctrl Pts',(58.4060826907792,45.7706564944895,12.));
#110810=CARTESIAN_POINT('Ctrl Pts',(58.4060826907792,45.7706564944895,8.));
#110811=CARTESIAN_POINT('Ctrl Pts',(58.4060826907792,45.7706564944895,4.));
#110812=CARTESIAN_POINT('Ctrl Pts',(58.4060826907792,45.7706564944895,-5.55111512312578E-16));
#110813=CARTESIAN_POINT('Origin',(2.97323128204029E-10,2.28269173065022E-10,
0.));
#110814=CARTESIAN_POINT('Origin',(2.97323128204029E-10,2.28269173065022E-10,
12.));
#110815=CARTESIAN_POINT('Origin',(2.97323128204029E-10,2.28269173065022E-10,
0.));
#110816=CARTESIAN_POINT('Ctrl Pts',(62.9938720098768,39.77464128315,0.));
#110817=CARTESIAN_POINT('Ctrl Pts',(62.9938720098768,39.77464128315,4.));
#110818=CARTESIAN_POINT('Ctrl Pts',(62.9938720098768,39.77464128315,8.));
#110819=CARTESIAN_POINT('Ctrl Pts',(62.9938720098768,39.77464128315,12.));
#110820=CARTESIAN_POINT('Ctrl Pts',(63.0525369183203,39.681729578236,0.));
#110821=CARTESIAN_POINT('Ctrl Pts',(63.0525369183203,39.681729578236,4.));
#110822=CARTESIAN_POINT('Ctrl Pts',(63.0525369183204,39.6817295782359,8.00000000000001));
#110823=CARTESIAN_POINT('Ctrl Pts',(63.0525369183204,39.6817295782359,12.));
#110824=CARTESIAN_POINT('Ctrl Pts',(63.099209014761,39.484513183097,0.));
#110825=CARTESIAN_POINT('Ctrl Pts',(63.099209014761,39.484513183097,4.));
#110826=CARTESIAN_POINT('Ctrl Pts',(63.099209014761,39.484513183097,7.99999999999999));
#110827=CARTESIAN_POINT('Ctrl Pts',(63.099209014761,39.484513183097,12.));
#110828=CARTESIAN_POINT('Ctrl Pts',(63.032294972791,39.2977314459986,0.));
#110829=CARTESIAN_POINT('Ctrl Pts',(63.032294972791,39.2977314459986,4.));
#110830=CARTESIAN_POINT('Ctrl Pts',(63.0322949727911,39.2977314459985,8.00000000000001));
#110831=CARTESIAN_POINT('Ctrl Pts',(63.0322949727911,39.2977314459985,12.));
#110832=CARTESIAN_POINT('Ctrl Pts',(62.9864049293638,39.2292784191469,0.));
#110833=CARTESIAN_POINT('Ctrl Pts',(62.9864049293638,39.2292784191469,4.));
#110834=CARTESIAN_POINT('Ctrl Pts',(62.986404929364,39.2292784191468,8.));
#110835=CARTESIAN_POINT('Ctrl Pts',(62.986404929364,39.2292784191468,12.));
#110836=CARTESIAN_POINT('',(62.9938720098768,39.77464128315,0.));
#110837=CARTESIAN_POINT('',(62.9864049293634,39.2292784191472,0.));
#110838=CARTESIAN_POINT('Ctrl Pts',(62.9938720098768,39.77464128315,2.77555756156289E-16));
#110839=CARTESIAN_POINT('Ctrl Pts',(63.0525369183203,39.681729578236,2.77555756156289E-16));
#110840=CARTESIAN_POINT('Ctrl Pts',(63.079206687715,39.5690344952994,2.77555756156289E-16));
#110841=CARTESIAN_POINT('Ctrl Pts',(63.0687871057919,39.4597466476414,2.77555756156289E-16));
#110842=CARTESIAN_POINT('Ctrl Pts',(63.0609724193496,39.3777807618979,2.77555756156289E-16));
#110843=CARTESIAN_POINT('Ctrl Pts',(63.032294972791,39.2977314459986,2.77555756156289E-16));
#110844=CARTESIAN_POINT('Ctrl Pts',(62.9864049293638,39.2292784191469,2.77555756156289E-16));
#110845=CARTESIAN_POINT('',(62.9864049293634,39.2292784191472,12.));
#110846=CARTESIAN_POINT('Ctrl Pts',(62.9864049293638,39.2292784191469,0.));
#110847=CARTESIAN_POINT('Ctrl Pts',(62.9864049293638,39.2292784191469,4.));
#110848=CARTESIAN_POINT('Ctrl Pts',(62.986404929364,39.2292784191468,8.));
#110849=CARTESIAN_POINT('Ctrl Pts',(62.986404929364,39.2292784191468,12.));
#110850=CARTESIAN_POINT('',(62.9938720098768,39.77464128315,12.));
#110851=CARTESIAN_POINT('Ctrl Pts',(62.986404929364,39.2292784191468,12.));
#110852=CARTESIAN_POINT('Ctrl Pts',(63.0322949727911,39.2977314459985,12.));
#110853=CARTESIAN_POINT('Ctrl Pts',(63.0609724193497,39.3777807618979,12.));
#110854=CARTESIAN_POINT('Ctrl Pts',(63.068787105792,39.4597466476414,12.));
#110855=CARTESIAN_POINT('Ctrl Pts',(63.079206687715,39.5690344952994,12.));
#110856=CARTESIAN_POINT('Ctrl Pts',(63.0525369183204,39.6817295782359,12.));
#110857=CARTESIAN_POINT('Ctrl Pts',(62.9938720098768,39.77464128315,12.));
#110858=CARTESIAN_POINT('Ctrl Pts',(62.9938720098768,39.77464128315,12.));
#110859=CARTESIAN_POINT('Ctrl Pts',(62.9938720098768,39.77464128315,8.));
#110860=CARTESIAN_POINT('Ctrl Pts',(62.9938720098768,39.77464128315,4.));
#110861=CARTESIAN_POINT('Ctrl Pts',(62.9938720098768,39.77464128315,0.));
#110862=CARTESIAN_POINT('Ctrl Pts',(60.1903555511633,35.7368311217509,0.));
#110863=CARTESIAN_POINT('Ctrl Pts',(60.1903555511633,35.7368311217509,12.));
#110864=CARTESIAN_POINT('Ctrl Pts',(60.1930746580239,35.7396040203973,0.));
#110865=CARTESIAN_POINT('Ctrl Pts',(60.1930746580239,35.7396040203973,12.));
#110866=CARTESIAN_POINT('Ctrl Pts',(60.1985151474406,35.7451551752456,0.));
#110867=CARTESIAN_POINT('Ctrl Pts',(60.1985151474406,35.7451551752456,12.));
#110868=CARTESIAN_POINT('Ctrl Pts',(60.2066827086579,35.7534979801871,0.));
#110869=CARTESIAN_POINT('Ctrl Pts',(60.2066827086579,35.7534979801871,12.));
#110870=CARTESIAN_POINT('Ctrl Pts',(60.2175864449678,35.7646538667299,0.));
#110871=CARTESIAN_POINT('Ctrl Pts',(60.2175864449678,35.7646538667299,12.));
#110872=CARTESIAN_POINT('Ctrl Pts',(60.2312388621286,35.7786523045782,0.));
#110873=CARTESIAN_POINT('Ctrl Pts',(60.2312388621286,35.7786523045782,12.));
#110874=CARTESIAN_POINT('Ctrl Pts',(60.2449139865206,35.7927043145165,0.));
#110875=CARTESIAN_POINT('Ctrl Pts',(60.2449139865206,35.7927043145165,12.));
#110876=CARTESIAN_POINT('Ctrl Pts',(60.2586117365278,35.8068098723386,0.));
#110877=CARTESIAN_POINT('Ctrl Pts',(60.2586117365278,35.8068098723386,12.));
#110878=CARTESIAN_POINT('Ctrl Pts',(60.2723319687507,35.8209689272574,0.));
#110879=CARTESIAN_POINT('Ctrl Pts',(60.2723319687507,35.8209689272574,12.));
#110880=CARTESIAN_POINT('Ctrl Pts',(60.2860744798563,35.8351814020424,0.));
#110881=CARTESIAN_POINT('Ctrl Pts',(60.2860744798563,35.8351814020424,12.));
#110882=CARTESIAN_POINT('Ctrl Pts',(60.2998390330173,35.8494472046784,0.));
#110883=CARTESIAN_POINT('Ctrl Pts',(60.2998390330173,35.8494472046784,12.));
#110884=CARTESIAN_POINT('Ctrl Pts',(60.313625378281,35.8637662371635,0.));
#110885=CARTESIAN_POINT('Ctrl Pts',(60.313625378281,35.8637662371635,12.));
#110886=CARTESIAN_POINT('Ctrl Pts',(60.3274332746782,35.878138405151,0.));
#110887=CARTESIAN_POINT('Ctrl Pts',(60.3274332746782,35.878138405151,12.));
#110888=CARTESIAN_POINT('Ctrl Pts',(60.3412625135223,35.8925636280632,0.));
#110889=CARTESIAN_POINT('Ctrl Pts',(60.3412625135223,35.8925636280632,12.));
#110890=CARTESIAN_POINT('Ctrl Pts',(60.3551129108794,35.9070418358501,0.));
#110891=CARTESIAN_POINT('Ctrl Pts',(60.3551129108794,35.9070418358501,12.));
#110892=CARTESIAN_POINT('Ctrl Pts',(60.368984296546,35.9215729642219,0.));
#110893=CARTESIAN_POINT('Ctrl Pts',(60.368984296546,35.9215729642219,12.));
#110894=CARTESIAN_POINT('Ctrl Pts',(60.3828765049031,35.9361569506955,0.));
#110895=CARTESIAN_POINT('Ctrl Pts',(60.3828765049031,35.9361569506955,12.));
#110896=CARTESIAN_POINT('Ctrl Pts',(60.3967893635487,35.9507937296726,0.));
#110897=CARTESIAN_POINT('Ctrl Pts',(60.3967893635487,35.9507937296726,12.));
#110898=CARTESIAN_POINT('Ctrl Pts',(60.4107226875759,35.9654832299627,0.));
#110899=CARTESIAN_POINT('Ctrl Pts',(60.4107226875759,35.9654832299627,12.));
#110900=CARTESIAN_POINT('Ctrl Pts',(60.4246762854961,35.9802253773534,0.));
#110901=CARTESIAN_POINT('Ctrl Pts',(60.4246762854961,35.9802253773534,12.));
#110902=CARTESIAN_POINT('Ctrl Pts',(60.438649962949,35.9950200962175,0.));
#110903=CARTESIAN_POINT('Ctrl Pts',(60.438649962949,35.9950200962175,12.));
#110904=CARTESIAN_POINT('Ctrl Pts',(60.452643526964,36.0098673113557,0.));
#110905=CARTESIAN_POINT('Ctrl Pts',(60.452643526964,36.0098673113557,12.));
#110906=CARTESIAN_POINT('Ctrl Pts',(60.4666567908053,36.0247669500867,0.));
#110907=CARTESIAN_POINT('Ctrl Pts',(60.4666567908053,36.0247669500867,12.));
#110908=CARTESIAN_POINT('Ctrl Pts',(60.4806895737643,36.0397189421617,0.));
#110909=CARTESIAN_POINT('Ctrl Pts',(60.4806895737643,36.0397189421617,12.));
#110910=CARTESIAN_POINT('Ctrl Pts',(60.4947416988396,36.0547232187681,0.));
#110911=CARTESIAN_POINT('Ctrl Pts',(60.4947416988396,36.0547232187681,12.));
#110912=CARTESIAN_POINT('Ctrl Pts',(60.5088129911357,36.0697797118377,0.));
#110913=CARTESIAN_POINT('Ctrl Pts',(60.5088129911357,36.0697797118377,12.));
#110914=CARTESIAN_POINT('Ctrl Pts',(60.5229032759001,36.0848883531969,0.));
#110915=CARTESIAN_POINT('Ctrl Pts',(60.5229032759001,36.0848883531969,12.));
#110916=CARTESIAN_POINT('Ctrl Pts',(60.5370123768841,36.1000490738532,0.));
#110917=CARTESIAN_POINT('Ctrl Pts',(60.5370123768841,36.1000490738532,12.));
#110918=CARTESIAN_POINT('Ctrl Pts',(60.5511401172014,36.1152618043756,0.));
#110919=CARTESIAN_POINT('Ctrl Pts',(60.5511401172014,36.1152618043756,12.));
#110920=CARTESIAN_POINT('Ctrl Pts',(60.5652863200732,36.1305264752195,0.));
#110921=CARTESIAN_POINT('Ctrl Pts',(60.5652863200732,36.1305264752195,12.));
#110922=CARTESIAN_POINT('Ctrl Pts',(60.5794508095555,36.1458430170425,0.));
#110923=CARTESIAN_POINT('Ctrl Pts',(60.5794508095555,36.1458430170425,12.));
#110924=CARTESIAN_POINT('Ctrl Pts',(60.5936334114082,36.1612113610758,0.));
#110925=CARTESIAN_POINT('Ctrl Pts',(60.5936334114082,36.1612113610758,12.));
#110926=CARTESIAN_POINT('Ctrl Pts',(60.6078339534151,36.1766314392624,0.));
#110927=CARTESIAN_POINT('Ctrl Pts',(60.6078339534151,36.1766314392624,12.));
#110928=CARTESIAN_POINT('Ctrl Pts',(60.6220522649129,36.1921031840618,0.));
#110929=CARTESIAN_POINT('Ctrl Pts',(60.6220522649129,36.1921031840618,12.));
#110930=CARTESIAN_POINT('Ctrl Pts',(60.6362881765014,36.2076265283261,0.));
#110931=CARTESIAN_POINT('Ctrl Pts',(60.6362881765014,36.2076265283261,12.));
#110932=CARTESIAN_POINT('Ctrl Pts',(60.6505415197055,36.2232014051549,0.));
#110933=CARTESIAN_POINT('Ctrl Pts',(60.6505415197055,36.2232014051549,12.));
#110934=CARTESIAN_POINT('Ctrl Pts',(60.6648121265908,36.2388277477225,0.));
#110935=CARTESIAN_POINT('Ctrl Pts',(60.6648121265908,36.2388277477225,12.));
#110936=CARTESIAN_POINT('Ctrl Pts',(60.6790998297823,36.2545054892911,0.));
#110937=CARTESIAN_POINT('Ctrl Pts',(60.6790998297823,36.2545054892911,12.));
#110938=CARTESIAN_POINT('Ctrl Pts',(60.6934044626304,36.2702345632883,0.));
#110939=CARTESIAN_POINT('Ctrl Pts',(60.6934044626304,36.2702345632883,12.));
#110940=CARTESIAN_POINT('Ctrl Pts',(60.7077258593268,36.2860149033586,0.));
#110941=CARTESIAN_POINT('Ctrl Pts',(60.7077258593268,36.2860149033586,12.));
#110942=CARTESIAN_POINT('Ctrl Pts',(60.7220638550396,36.3018464434204,0.));
#110943=CARTESIAN_POINT('Ctrl Pts',(60.7220638550396,36.3018464434204,12.));
#110944=CARTESIAN_POINT('Ctrl Pts',(60.7364182860388,36.3177291177148,0.));
#110945=CARTESIAN_POINT('Ctrl Pts',(60.7364182860388,36.3177291177148,12.));
#110946=CARTESIAN_POINT('Ctrl Pts',(60.7507889896283,36.3336628607844,0.));
#110947=CARTESIAN_POINT('Ctrl Pts',(60.7507889896283,36.3336628607844,12.));
#110948=CARTESIAN_POINT('Ctrl Pts',(60.7651758040791,36.349647607448,0.));
#110949=CARTESIAN_POINT('Ctrl Pts',(60.7651758040791,36.349647607448,12.));
#110950=CARTESIAN_POINT('Ctrl Pts',(60.779578568563,36.3656832927733,0.));
#110951=CARTESIAN_POINT('Ctrl Pts',(60.779578568563,36.3656832927733,12.));
#110952=CARTESIAN_POINT('Ctrl Pts',(60.7939971230781,36.38176985204,0.));
#110953=CARTESIAN_POINT('Ctrl Pts',(60.7939971230781,36.38176985204,12.));
#110954=CARTESIAN_POINT('Ctrl Pts',(60.8084313084009,36.3979072207174,0.));
#110955=CARTESIAN_POINT('Ctrl Pts',(60.8084313084009,36.3979072207174,12.));
#110956=CARTESIAN_POINT('Ctrl Pts',(60.8228809661179,36.414095334487,0.));
#110957=CARTESIAN_POINT('Ctrl Pts',(60.8228809661179,36.414095334487,12.));
#110958=CARTESIAN_POINT('Ctrl Pts',(60.8373459386397,36.4303341292497,0.));
#110959=CARTESIAN_POINT('Ctrl Pts',(60.8373459386397,36.4303341292497,12.));
#110960=CARTESIAN_POINT('Ctrl Pts',(60.851826069218,36.4466235411353,0.));
#110961=CARTESIAN_POINT('Ctrl Pts',(60.851826069218,36.4466235411353,12.));
#110962=CARTESIAN_POINT('Ctrl Pts',(60.8663212019646,36.4629635065037,0.));
#110963=CARTESIAN_POINT('Ctrl Pts',(60.8663212019646,36.4629635065037,12.));
#110964=CARTESIAN_POINT('Ctrl Pts',(60.8808311818489,36.4793539619459,0.));
#110965=CARTESIAN_POINT('Ctrl Pts',(60.8808311818489,36.4793539619459,12.));
#110966=CARTESIAN_POINT('Ctrl Pts',(60.8953558546791,36.4957948442832,0.));
#110967=CARTESIAN_POINT('Ctrl Pts',(60.8953558546791,36.4957948442832,12.));
#110968=CARTESIAN_POINT('Ctrl Pts',(60.9098950670847,36.5122860905611,0.));
#110969=CARTESIAN_POINT('Ctrl Pts',(60.9098950670847,36.5122860905611,12.));
#110970=CARTESIAN_POINT('Ctrl Pts',(60.924448666499,36.5288276380417,0.));
#110971=CARTESIAN_POINT('Ctrl Pts',(60.924448666499,36.5288276380417,12.));
#110972=CARTESIAN_POINT('Ctrl Pts',(60.9390165011357,36.5454194241866,0.));
#110973=CARTESIAN_POINT('Ctrl Pts',(60.9390165011357,36.5454194241866,12.));
#110974=CARTESIAN_POINT('Ctrl Pts',(60.9535984199874,36.5620613866616,0.));
#110975=CARTESIAN_POINT('Ctrl Pts',(60.9535984199874,36.5620613866616,12.));
#110976=CARTESIAN_POINT('Ctrl Pts',(60.9681942728237,36.5787534633416,0.));
#110977=CARTESIAN_POINT('Ctrl Pts',(60.9681942728237,36.5787534633416,12.));
#110978=CARTESIAN_POINT('Ctrl Pts',(60.9828039101887,36.5954955923109,0.));
#110979=CARTESIAN_POINT('Ctrl Pts',(60.9828039101887,36.5954955923109,12.));
#110980=CARTESIAN_POINT('Ctrl Pts',(60.9974271833982,36.6122877118599,0.));
#110981=CARTESIAN_POINT('Ctrl Pts',(60.9974271833982,36.6122877118599,12.));
#110982=CARTESIAN_POINT('Ctrl Pts',(61.012063944535,36.6291297604775,0.));
#110983=CARTESIAN_POINT('Ctrl Pts',(61.012063944535,36.6291297604775,12.));
#110984=CARTESIAN_POINT('Ctrl Pts',(61.0267140464434,36.6460216768553,0.));
#110985=CARTESIAN_POINT('Ctrl Pts',(61.0267140464434,36.6460216768553,12.));
#110986=CARTESIAN_POINT('Ctrl Pts',(61.0413773427204,36.6629633998886,0.));
#110987=CARTESIAN_POINT('Ctrl Pts',(61.0413773427204,36.6629633998886,12.));
#110988=CARTESIAN_POINT('Ctrl Pts',(61.0560536877084,36.6799548686741,0.));
#110989=CARTESIAN_POINT('Ctrl Pts',(61.0560536877084,36.6799548686741,12.));
#110990=CARTESIAN_POINT('Ctrl Pts',(61.0707429364841,36.6969960225019,0.));
#110991=CARTESIAN_POINT('Ctrl Pts',(61.0707429364841,36.6969960225019,12.));
#110992=CARTESIAN_POINT('Ctrl Pts',(61.085444944851,36.7140868008479,0.));
#110993=CARTESIAN_POINT('Ctrl Pts',(61.085444944851,36.7140868008479,12.));
#110994=CARTESIAN_POINT('Ctrl Pts',(61.1001595693357,36.7312271433799,0.));
#110995=CARTESIAN_POINT('Ctrl Pts',(61.1001595693357,36.7312271433799,12.));
#110996=CARTESIAN_POINT('Ctrl Pts',(61.1148866671821,36.7484169899591,0.));
#110997=CARTESIAN_POINT('Ctrl Pts',(61.1148866671821,36.7484169899591,12.));
#110998=CARTESIAN_POINT('Ctrl Pts',(61.1296260963468,36.7656562806381,0.));
#110999=CARTESIAN_POINT('Ctrl Pts',(61.1296260963468,36.7656562806381,12.));
#111000=CARTESIAN_POINT('Ctrl Pts',(61.1443777154926,36.782944955654,0.));
#111001=CARTESIAN_POINT('Ctrl Pts',(61.1443777154926,36.782944955654,12.));
#111002=CARTESIAN_POINT('Ctrl Pts',(61.1591413839809,36.8002829554221,0.));
#111003=CARTESIAN_POINT('Ctrl Pts',(61.1591413839809,36.8002829554221,12.));
#111004=CARTESIAN_POINT('Ctrl Pts',(61.1739169618688,36.8176702205436,0.));
#111005=CARTESIAN_POINT('Ctrl Pts',(61.1739169618688,36.8176702205436,12.));
#111006=CARTESIAN_POINT('Ctrl Pts',(61.1887043099026,36.8351066918043,0.));
#111007=CARTESIAN_POINT('Ctrl Pts',(61.1887043099026,36.8351066918043,12.));
#111008=CARTESIAN_POINT('Ctrl Pts',(61.2035032895121,36.8525923101736,0.));
#111009=CARTESIAN_POINT('Ctrl Pts',(61.2035032895121,36.8525923101736,12.));
#111010=CARTESIAN_POINT('Ctrl Pts',(61.2183137628031,36.8701270167954,0.));
#111011=CARTESIAN_POINT('Ctrl Pts',(61.2183137628031,36.8701270167954,12.));
#111012=CARTESIAN_POINT('Ctrl Pts',(61.2331355925513,36.8877107529844,0.));
#111013=CARTESIAN_POINT('Ctrl Pts',(61.2331355925513,36.8877107529844,12.));
#111014=CARTESIAN_POINT('Ctrl Pts',(61.2479686421979,36.9053434602324,0.));
#111015=CARTESIAN_POINT('Ctrl Pts',(61.2479686421979,36.9053434602324,12.));
#111016=CARTESIAN_POINT('Ctrl Pts',(61.2628127758443,36.9230250802079,0.));
#111017=CARTESIAN_POINT('Ctrl Pts',(61.2628127758443,36.9230250802079,12.));
#111018=CARTESIAN_POINT('Ctrl Pts',(61.2776678582474,36.9407555547542,0.));
#111019=CARTESIAN_POINT('Ctrl Pts',(61.2776678582474,36.9407555547542,12.));
#111020=CARTESIAN_POINT('Ctrl Pts',(61.2925337548113,36.9585348258798,0.));
#111021=CARTESIAN_POINT('Ctrl Pts',(61.2925337548113,36.9585348258798,12.));
#111022=CARTESIAN_POINT('Ctrl Pts',(61.3074103315834,36.976362835757,0.));
#111023=CARTESIAN_POINT('Ctrl Pts',(61.3074103315834,36.976362835757,12.));
#111024=CARTESIAN_POINT('Ctrl Pts',(61.3222974552519,36.994239526729,0.));
#111025=CARTESIAN_POINT('Ctrl Pts',(61.3222974552519,36.994239526729,12.));
#111026=CARTESIAN_POINT('Ctrl Pts',(61.3371949931396,37.0121648413088,0.));
#111027=CARTESIAN_POINT('Ctrl Pts',(61.3371949931396,37.0121648413088,12.));
#111028=CARTESIAN_POINT('Ctrl Pts',(61.352102813199,37.0301387221766,0.));
#111029=CARTESIAN_POINT('Ctrl Pts',(61.352102813199,37.0301387221766,12.));
#111030=CARTESIAN_POINT('Ctrl Pts',(61.3670207840041,37.0481611121698,0.));
#111031=CARTESIAN_POINT('Ctrl Pts',(61.3670207840041,37.0481611121698,12.));
#111032=CARTESIAN_POINT('Ctrl Pts',(61.3819487747458,37.0662319542827,0.));
#111033=CARTESIAN_POINT('Ctrl Pts',(61.3819487747458,37.0662319542827,12.));
#111034=CARTESIAN_POINT('Ctrl Pts',(61.3968866552294,37.0843511916729,0.));
#111035=CARTESIAN_POINT('Ctrl Pts',(61.3968866552294,37.0843511916729,12.));
#111036=CARTESIAN_POINT('Ctrl Pts',(61.411834295869,37.1025187676597,0.));
#111037=CARTESIAN_POINT('Ctrl Pts',(61.411834295869,37.1025187676597,12.));
#111038=CARTESIAN_POINT('Ctrl Pts',(61.4267915676834,37.1207346257229,0.));
#111039=CARTESIAN_POINT('Ctrl Pts',(61.4267915676834,37.1207346257229,12.));
#111040=CARTESIAN_POINT('Ctrl Pts',(61.4417583422888,37.138998709492,0.));
#111041=CARTESIAN_POINT('Ctrl Pts',(61.4417583422888,37.138998709492,12.));
#111042=CARTESIAN_POINT('Ctrl Pts',(61.4567344918946,37.157310962747,0.));
#111043=CARTESIAN_POINT('Ctrl Pts',(61.4567344918946,37.157310962747,12.));
#111044=CARTESIAN_POINT('Ctrl Pts',(61.471719889301,37.1756713294249,0.));
#111045=CARTESIAN_POINT('Ctrl Pts',(61.471719889301,37.1756713294249,12.));
#111046=CARTESIAN_POINT('Ctrl Pts',(61.4867144078939,37.1940797536182,0.));
#111047=CARTESIAN_POINT('Ctrl Pts',(61.4867144078939,37.1940797536182,12.));
#111048=CARTESIAN_POINT('Ctrl Pts',(61.5017179216404,37.2125361795727,0.));
#111049=CARTESIAN_POINT('Ctrl Pts',(61.5017179216404,37.2125361795727,12.));
#111050=CARTESIAN_POINT('Ctrl Pts',(61.5167303050823,37.2310405516775,0.));
#111051=CARTESIAN_POINT('Ctrl Pts',(61.5167303050823,37.2310405516775,12.));
#111052=CARTESIAN_POINT('Ctrl Pts',(61.5317514333319,37.2495928144661,0.));
#111053=CARTESIAN_POINT('Ctrl Pts',(61.5317514333319,37.2495928144661,12.));
#111054=CARTESIAN_POINT('Ctrl Pts',(61.5467811820686,37.2681929126218,0.));
#111055=CARTESIAN_POINT('Ctrl Pts',(61.5467811820686,37.2681929126218,12.));
#111056=CARTESIAN_POINT('Ctrl Pts',(61.5618194275349,37.286840790977,0.));
#111057=CARTESIAN_POINT('Ctrl Pts',(61.5618194275349,37.286840790977,12.));
#111058=CARTESIAN_POINT('Ctrl Pts',(61.5768660465313,37.3055363945108,0.));
#111059=CARTESIAN_POINT('Ctrl Pts',(61.5768660465313,37.3055363945108,12.));
#111060=CARTESIAN_POINT('Ctrl Pts',(61.591920916412,37.3242796683395,0.));
#111061=CARTESIAN_POINT('Ctrl Pts',(61.591920916412,37.3242796683395,12.));
#111062=CARTESIAN_POINT('Ctrl Pts',(61.6069839150804,37.3430705577178,0.));
#111063=CARTESIAN_POINT('Ctrl Pts',(61.6069839150804,37.3430705577178,12.));
#111064=CARTESIAN_POINT('Ctrl Pts',(61.6220549209862,37.3619090080447,0.));
#111065=CARTESIAN_POINT('Ctrl Pts',(61.6220549209862,37.3619090080447,12.));
#111066=CARTESIAN_POINT('Ctrl Pts',(61.6371338131208,37.3807949648622,0.));
#111067=CARTESIAN_POINT('Ctrl Pts',(61.6371338131208,37.3807949648622,12.));
#111068=CARTESIAN_POINT('Ctrl Pts',(61.6522204710133,37.3997283738534,0.));
#111069=CARTESIAN_POINT('Ctrl Pts',(61.6522204710133,37.3997283738534,12.));
#111070=CARTESIAN_POINT('Ctrl Pts',(61.6673147747249,37.4187091808324,0.));
#111071=CARTESIAN_POINT('Ctrl Pts',(61.6673147747249,37.4187091808324,12.));
#111072=CARTESIAN_POINT('Ctrl Pts',(61.6824166048453,37.4377373317456,0.));
#111073=CARTESIAN_POINT('Ctrl Pts',(61.6824166048453,37.4377373317456,12.));
#111074=CARTESIAN_POINT('Ctrl Pts',(61.69752584249,37.4568127726776,0.));
#111075=CARTESIAN_POINT('Ctrl Pts',(61.69752584249,37.4568127726776,12.));
#111076=CARTESIAN_POINT('Ctrl Pts',(61.7126423692965,37.4759354498509,0.));
#111077=CARTESIAN_POINT('Ctrl Pts',(61.7126423692965,37.4759354498509,12.));
#111078=CARTESIAN_POINT('Ctrl Pts',(61.7277660674203,37.4951053096235,0.));
#111079=CARTESIAN_POINT('Ctrl Pts',(61.7277660674203,37.4951053096235,12.));
#111080=CARTESIAN_POINT('Ctrl Pts',(61.7428968195296,37.5143222984794,0.));
#111081=CARTESIAN_POINT('Ctrl Pts',(61.7428968195296,37.5143222984794,12.));
#111082=CARTESIAN_POINT('Ctrl Pts',(61.7580345088014,37.5335863630286,0.));
#111083=CARTESIAN_POINT('Ctrl Pts',(61.7580345088014,37.5335863630286,12.));
#111084=CARTESIAN_POINT('Ctrl Pts',(61.7731790189191,37.5528974500142,0.));
#111085=CARTESIAN_POINT('Ctrl Pts',(61.7731790189191,37.5528974500142,12.));
#111086=CARTESIAN_POINT('Ctrl Pts',(61.7883302340689,37.5722555063112,0.));
#111087=CARTESIAN_POINT('Ctrl Pts',(61.7883302340689,37.5722555063112,12.));
#111088=CARTESIAN_POINT('Ctrl Pts',(61.8034880389362,37.5916604789252,0.));
#111089=CARTESIAN_POINT('Ctrl Pts',(61.8034880389362,37.5916604789252,12.));
#111090=CARTESIAN_POINT('Ctrl Pts',(61.8186523187011,37.6111123149836,0.));
#111091=CARTESIAN_POINT('Ctrl Pts',(61.8186523187011,37.6111123149836,12.));
#111092=CARTESIAN_POINT('Ctrl Pts',(61.8338229590345,37.6306109617341,0.));
#111093=CARTESIAN_POINT('Ctrl Pts',(61.8338229590345,37.6306109617341,12.));
#111094=CARTESIAN_POINT('Ctrl Pts',(61.848999846095,37.6501563665518,0.));
#111095=CARTESIAN_POINT('Ctrl Pts',(61.848999846095,37.6501563665518,12.));
#111096=CARTESIAN_POINT('Ctrl Pts',(61.8641828665257,37.6697484769389,0.));
#111097=CARTESIAN_POINT('Ctrl Pts',(61.8641828665257,37.6697484769389,12.));
#111098=CARTESIAN_POINT('Ctrl Pts',(61.879371907451,37.689387240523,0.));
#111099=CARTESIAN_POINT('Ctrl Pts',(61.879371907451,37.689387240523,12.));
#111100=CARTESIAN_POINT('Ctrl Pts',(61.8945668564714,37.7090726050488,0.));
#111101=CARTESIAN_POINT('Ctrl Pts',(61.8945668564714,37.7090726050488,12.));
#111102=CARTESIAN_POINT('Ctrl Pts',(61.9097676016616,37.7288045183765,0.));
#111103=CARTESIAN_POINT('Ctrl Pts',(61.9097676016616,37.7288045183765,12.));
#111104=CARTESIAN_POINT('Ctrl Pts',(61.9249740315664,37.748582928488,0.));
#111105=CARTESIAN_POINT('Ctrl Pts',(61.9249740315664,37.748582928488,12.));
#111106=CARTESIAN_POINT('Ctrl Pts',(61.940186035198,37.7684077834877,0.));
#111107=CARTESIAN_POINT('Ctrl Pts',(61.940186035198,37.7684077834877,12.));
#111108=CARTESIAN_POINT('Ctrl Pts',(61.9554035020335,37.7882790316012,0.));
#111109=CARTESIAN_POINT('Ctrl Pts',(61.9554035020335,37.7882790316012,12.));
#111110=CARTESIAN_POINT('Ctrl Pts',(61.9706263220101,37.808196621168,0.));
#111111=CARTESIAN_POINT('Ctrl Pts',(61.9706263220101,37.808196621168,12.));
#111112=CARTESIAN_POINT('Ctrl Pts',(61.9858543855221,37.8281605006371,0.));
#111113=CARTESIAN_POINT('Ctrl Pts',(61.9858543855221,37.8281605006371,12.));
#111114=CARTESIAN_POINT('Ctrl Pts',(62.0010875834176,37.8481706185742,0.));
#111115=CARTESIAN_POINT('Ctrl Pts',(62.0010875834176,37.8481706185742,12.));
#111116=CARTESIAN_POINT('Ctrl Pts',(62.0163258069954,37.8682269236628,0.));
#111117=CARTESIAN_POINT('Ctrl Pts',(62.0163258069954,37.8682269236628,12.));
#111118=CARTESIAN_POINT('Ctrl Pts',(62.0315689480022,37.888329364703,0.));
#111119=CARTESIAN_POINT('Ctrl Pts',(62.0315689480022,37.888329364703,12.));
#111120=CARTESIAN_POINT('Ctrl Pts',(62.0468168986289,37.9084778906053,0.));
#111121=CARTESIAN_POINT('Ctrl Pts',(62.0468168986289,37.9084778906053,12.));
#111122=CARTESIAN_POINT('Ctrl Pts',(62.0620695515072,37.9286724503849,0.));
#111123=CARTESIAN_POINT('Ctrl Pts',(62.0620695515072,37.9286724503849,12.));
#111124=CARTESIAN_POINT('Ctrl Pts',(62.0773267997072,37.9489129931685,0.));
#111125=CARTESIAN_POINT('Ctrl Pts',(62.0773267997072,37.9489129931685,12.));
#111126=CARTESIAN_POINT('Ctrl Pts',(62.0925885367346,37.9691994681962,0.));
#111127=CARTESIAN_POINT('Ctrl Pts',(62.0925885367346,37.9691994681962,12.));
#111128=CARTESIAN_POINT('Ctrl Pts',(62.107854656528,37.9895318248212,0.));
#111129=CARTESIAN_POINT('Ctrl Pts',(62.107854656528,37.9895318248212,12.));
#111130=CARTESIAN_POINT('Ctrl Pts',(62.1231250534558,38.0099100125041,0.));
#111131=CARTESIAN_POINT('Ctrl Pts',(62.1231250534558,38.0099100125041,12.));
#111132=CARTESIAN_POINT('Ctrl Pts',(62.1383996223136,38.0303339808059,0.));
#111133=CARTESIAN_POINT('Ctrl Pts',(62.1383996223136,38.0303339808059,12.));
#111134=CARTESIAN_POINT('Ctrl Pts',(62.153678258321,38.0508036793944,0.));
#111135=CARTESIAN_POINT('Ctrl Pts',(62.153678258321,38.0508036793944,12.));
#111136=CARTESIAN_POINT('Ctrl Pts',(62.1689608571182,38.0713190580466,0.));
#111137=CARTESIAN_POINT('Ctrl Pts',(62.1689608571182,38.0713190580466,12.));
#111138=CARTESIAN_POINT('Ctrl Pts',(62.1842473147627,38.0918800666479,0.));
#111139=CARTESIAN_POINT('Ctrl Pts',(62.1842473147627,38.0918800666479,12.));
#111140=CARTESIAN_POINT('Ctrl Pts',(62.1995375277253,38.1124866551884,0.));
#111141=CARTESIAN_POINT('Ctrl Pts',(62.1995375277253,38.1124866551884,12.));
#111142=CARTESIAN_POINT('Ctrl Pts',(62.2148313928859,38.1331387737528,0.));
#111143=CARTESIAN_POINT('Ctrl Pts',(62.2148313928859,38.1331387737528,12.));
#111144=CARTESIAN_POINT('Ctrl Pts',(62.2301288075319,38.1538363725263,0.));
#111145=CARTESIAN_POINT('Ctrl Pts',(62.2301288075319,38.1538363725263,12.));
#111146=CARTESIAN_POINT('Ctrl Pts',(62.2454296693581,38.1745794017997,0.));
#111147=CARTESIAN_POINT('Ctrl Pts',(62.2454296693581,38.1745794017997,12.));
#111148=CARTESIAN_POINT('Ctrl Pts',(62.2607338764655,38.1953678119692,0.));
#111149=CARTESIAN_POINT('Ctrl Pts',(62.2607338764655,38.1953678119692,12.));
#111150=CARTESIAN_POINT('Ctrl Pts',(62.2760413273601,38.2162015535351,0.));
#111151=CARTESIAN_POINT('Ctrl Pts',(62.2760413273601,38.2162015535351,12.));
#111152=CARTESIAN_POINT('Ctrl Pts',(62.2913519209517,38.2370805770931,0.));
#111153=CARTESIAN_POINT('Ctrl Pts',(62.2913519209517,38.2370805770931,12.));
#111154=CARTESIAN_POINT('Ctrl Pts',(62.3066655565497,38.2580048333356,0.));
#111155=CARTESIAN_POINT('Ctrl Pts',(62.3066655565497,38.2580048333356,12.));
#111156=CARTESIAN_POINT('Ctrl Pts',(62.3219821338564,38.2789742730559,0.));
#111157=CARTESIAN_POINT('Ctrl Pts',(62.3219821338564,38.2789742730559,12.));
#111158=CARTESIAN_POINT('Ctrl Pts',(62.337301552961,38.2999888471474,0.));
#111159=CARTESIAN_POINT('Ctrl Pts',(62.337301552961,38.2999888471474,12.));
#111160=CARTESIAN_POINT('Ctrl Pts',(62.3526237143338,38.3210485066003,0.));
#111161=CARTESIAN_POINT('Ctrl Pts',(62.3526237143338,38.3210485066003,12.));
#111162=CARTESIAN_POINT('Ctrl Pts',(62.3679485188178,38.3421532024915,0.));
#111163=CARTESIAN_POINT('Ctrl Pts',(62.3679485188178,38.3421532024915,12.));
#111164=CARTESIAN_POINT('Ctrl Pts',(62.3832758676281,38.3633028859835,0.));
#111165=CARTESIAN_POINT('Ctrl Pts',(62.3832758676281,38.3633028859835,12.));
#111166=CARTESIAN_POINT('Ctrl Pts',(62.3986056623587,38.384497508335,0.));
#111167=CARTESIAN_POINT('Ctrl Pts',(62.3986056623587,38.384497508335,12.));
#111168=CARTESIAN_POINT('Ctrl Pts',(62.4139378049891,38.4057370209054,0.));
#111169=CARTESIAN_POINT('Ctrl Pts',(62.4139378049891,38.4057370209054,12.));
#111170=CARTESIAN_POINT('Ctrl Pts',(62.42927219789,38.4270213751567,0.));
#111171=CARTESIAN_POINT('Ctrl Pts',(62.42927219789,38.4270213751567,12.));
#111172=CARTESIAN_POINT('Ctrl Pts',(62.4446087438304,38.4483505226511,0.));
#111173=CARTESIAN_POINT('Ctrl Pts',(62.4446087438304,38.4483505226511,12.));
#111174=CARTESIAN_POINT('Ctrl Pts',(62.4599473459799,38.4697244150473,0.));
#111175=CARTESIAN_POINT('Ctrl Pts',(62.4599473459799,38.4697244150473,12.));
#111176=CARTESIAN_POINT('Ctrl Pts',(62.4752879078842,38.4911430040988,0.));
#111177=CARTESIAN_POINT('Ctrl Pts',(62.4752879078842,38.4911430040988,12.));
#111178=CARTESIAN_POINT('Ctrl Pts',(62.4906303334435,38.5126062416496,0.));
#111179=CARTESIAN_POINT('Ctrl Pts',(62.4906303334435,38.5126062416496,12.));
#111180=CARTESIAN_POINT('Ctrl Pts',(62.50597452689,38.5341140796247,0.));
#111181=CARTESIAN_POINT('Ctrl Pts',(62.50597452689,38.5341140796247,12.));
#111182=CARTESIAN_POINT('Ctrl Pts',(62.5213203927672,38.5556664700201,0.));
#111183=CARTESIAN_POINT('Ctrl Pts',(62.5213203927672,38.5556664700201,12.));
#111184=CARTESIAN_POINT('Ctrl Pts',(62.5366678359036,38.5772633648841,0.));
#111185=CARTESIAN_POINT('Ctrl Pts',(62.5366678359036,38.5772633648841,12.));
#111186=CARTESIAN_POINT('Ctrl Pts',(62.5520167614529,38.5989047163401,0.));
#111187=CARTESIAN_POINT('Ctrl Pts',(62.5520167614529,38.5989047163401,12.));
#111188=CARTESIAN_POINT('Ctrl Pts',(62.567367074937,38.6205904766078,0.));
#111189=CARTESIAN_POINT('Ctrl Pts',(62.567367074937,38.6205904766078,12.));
#111190=CARTESIAN_POINT('Ctrl Pts',(62.5827186822923,38.6423205980214,0.));
#111191=CARTESIAN_POINT('Ctrl Pts',(62.5827186822923,38.6423205980214,12.));
#111192=CARTESIAN_POINT('Ctrl Pts',(62.5980714899048,38.6640950330418,0.));
#111193=CARTESIAN_POINT('Ctrl Pts',(62.5980714899048,38.6640950330418,12.));
#111194=CARTESIAN_POINT('Ctrl Pts',(62.6134254046732,38.6859137342726,0.));
#111195=CARTESIAN_POINT('Ctrl Pts',(62.6134254046732,38.6859137342726,12.));
#111196=CARTESIAN_POINT('Ctrl Pts',(62.6287803339534,38.7077766544411,0.));
#111197=CARTESIAN_POINT('Ctrl Pts',(62.6287803339534,38.7077766544411,12.));
#111198=CARTESIAN_POINT('Ctrl Pts',(62.6441361854406,38.7296837463605,0.));
#111199=CARTESIAN_POINT('Ctrl Pts',(62.6441361854406,38.7296837463605,12.));
#111200=CARTESIAN_POINT('Ctrl Pts',(62.6594928670626,38.7516349628902,0.));
#111201=CARTESIAN_POINT('Ctrl Pts',(62.6594928670626,38.7516349628902,12.));
#111202=CARTESIAN_POINT('Ctrl Pts',(62.6748502868836,38.7736302568982,0.));
#111203=CARTESIAN_POINT('Ctrl Pts',(62.6748502868836,38.7736302568982,12.));
#111204=CARTESIAN_POINT('Ctrl Pts',(62.6902083529698,38.7956695812032,0.));
#111205=CARTESIAN_POINT('Ctrl Pts',(62.6902083529698,38.7956695812032,12.));
#111206=CARTESIAN_POINT('Ctrl Pts',(62.7055669733811,38.8177528885687,0.));
#111207=CARTESIAN_POINT('Ctrl Pts',(62.7055669733811,38.8177528885687,12.));
#111208=CARTESIAN_POINT('Ctrl Pts',(62.7209260564506,38.8398801318184,0.));
#111209=CARTESIAN_POINT('Ctrl Pts',(62.7209260564506,38.8398801318184,12.));
#111210=CARTESIAN_POINT('Ctrl Pts',(62.7362855110052,38.8620512639239,0.));
#111211=CARTESIAN_POINT('Ctrl Pts',(62.7362855110052,38.8620512639239,12.));
#111212=CARTESIAN_POINT('Ctrl Pts',(62.7516452466129,38.8842662380984,0.));
#111213=CARTESIAN_POINT('Ctrl Pts',(62.7516452466129,38.8842662380984,12.));
#111214=CARTESIAN_POINT('Ctrl Pts',(62.7670051738132,38.9065250078824,0.));
#111215=CARTESIAN_POINT('Ctrl Pts',(62.7670051738132,38.9065250078824,12.));
#111216=CARTESIAN_POINT('Ctrl Pts',(62.7823652043677,38.928827527232,0.));
#111217=CARTESIAN_POINT('Ctrl Pts',(62.7823652043677,38.928827527232,12.));
#111218=CARTESIAN_POINT('Ctrl Pts',(62.797725250709,38.9511737503146,0.));
#111219=CARTESIAN_POINT('Ctrl Pts',(62.797725250709,38.9511737503146,12.));
#111220=CARTESIAN_POINT('Ctrl Pts',(62.8130852254004,38.9735636313073,0.));
#111221=CARTESIAN_POINT('Ctrl Pts',(62.8130852254004,38.9735636313073,12.));
#111222=CARTESIAN_POINT('Ctrl Pts',(62.8284450405451,38.9959971241695,0.));
#111223=CARTESIAN_POINT('Ctrl Pts',(62.8284450405451,38.9959971241695,12.));
#111224=CARTESIAN_POINT('Ctrl Pts',(62.8438046073237,39.0184741824649,0.));
#111225=CARTESIAN_POINT('Ctrl Pts',(62.8438046073237,39.0184741824649,12.));
#111226=CARTESIAN_POINT('Ctrl Pts',(62.859163835209,39.0409947590519,0.));
#111227=CARTESIAN_POINT('Ctrl Pts',(62.859163835209,39.0409947590519,12.));
#111228=CARTESIAN_POINT('Ctrl Pts',(62.8745226326046,39.0635588063309,0.));
#111229=CARTESIAN_POINT('Ctrl Pts',(62.8745226326046,39.0635588063309,12.));
#111230=CARTESIAN_POINT('Ctrl Pts',(62.8898809082659,39.0861662767964,0.));
#111231=CARTESIAN_POINT('Ctrl Pts',(62.8898809082659,39.0861662767964,12.));
#111232=CARTESIAN_POINT('Ctrl Pts',(62.9052385725416,39.1088171235144,0.));
#111233=CARTESIAN_POINT('Ctrl Pts',(62.9052385725416,39.1088171235144,12.));
#111234=CARTESIAN_POINT('Ctrl Pts',(62.9205955385551,39.1315113005745,0.));
#111235=CARTESIAN_POINT('Ctrl Pts',(62.9205955385551,39.1315113005745,12.));
#111236=CARTESIAN_POINT('Ctrl Pts',(62.9359517237352,39.1542487636708,0.));
#111237=CARTESIAN_POINT('Ctrl Pts',(62.9359517237352,39.1542487636708,12.));
#111238=CARTESIAN_POINT('Ctrl Pts',(62.9513070501777,39.1770294702367,0.));
#111239=CARTESIAN_POINT('Ctrl Pts',(62.9513070501777,39.1770294702367,12.));
#111240=CARTESIAN_POINT('Ctrl Pts',(62.9666614412627,39.199853378159,0.));
#111241=CARTESIAN_POINT('Ctrl Pts',(62.9666614412627,39.199853378159,12.));
#111242=CARTESIAN_POINT('Ctrl Pts',(62.9820148189849,39.2227204447583,0.));
#111243=CARTESIAN_POINT('Ctrl Pts',(62.9820148189849,39.2227204447583,12.));
#111244=CARTESIAN_POINT('Ctrl Pts',(62.9973671008685,39.2456306256092,0.));
#111245=CARTESIAN_POINT('Ctrl Pts',(62.9973671008685,39.2456306256092,12.));
#111246=CARTESIAN_POINT('Ctrl Pts',(63.0127181973702,39.268583873541,0.));
#111247=CARTESIAN_POINT('Ctrl Pts',(63.0127181973702,39.268583873541,12.));
#111248=CARTESIAN_POINT('Ctrl Pts',(63.0280680082522,39.2915801372468,0.));
#111249=CARTESIAN_POINT('Ctrl Pts',(63.0280680082522,39.2915801372468,12.));
#111250=CARTESIAN_POINT('Ctrl Pts',(63.0434164278221,39.3146193632546,0.));
#111251=CARTESIAN_POINT('Ctrl Pts',(63.0434164278221,39.3146193632546,12.));
#111252=CARTESIAN_POINT('Ctrl Pts',(63.0587633513993,39.3377014983757,0.));
#111253=CARTESIAN_POINT('Ctrl Pts',(63.0587633513993,39.3377014983757,12.));
#111254=CARTESIAN_POINT('Ctrl Pts',(63.0741086815957,39.3608264920487,0.));
#111255=CARTESIAN_POINT('Ctrl Pts',(63.0741086815957,39.3608264920487,12.));
#111256=CARTESIAN_POINT('Ctrl Pts',(63.0894523341238,39.3839942985688,0.));
#111257=CARTESIAN_POINT('Ctrl Pts',(63.0894523341238,39.3839942985688,12.));
#111258=CARTESIAN_POINT('Ctrl Pts',(63.1047942451583,39.4072048797401,0.));
#111259=CARTESIAN_POINT('Ctrl Pts',(63.1047942451583,39.4072048797401,12.));
#111260=CARTESIAN_POINT('Ctrl Pts',(63.1201343730643,39.4304582059507,0.));
#111261=CARTESIAN_POINT('Ctrl Pts',(63.1201343730643,39.4304582059507,12.));
#111262=CARTESIAN_POINT('Ctrl Pts',(63.1354726927781,39.4537542551852,0.));
#111263=CARTESIAN_POINT('Ctrl Pts',(63.1354726927781,39.4537542551852,12.));
#111264=CARTESIAN_POINT('Ctrl Pts',(63.147741892189,39.4724252610807,0.));
#111265=CARTESIAN_POINT('Ctrl Pts',(63.147741892189,39.4724252610807,12.));
#111266=CARTESIAN_POINT('Ctrl Pts',(63.1569429707564,39.4864477303613,0.));
#111267=CARTESIAN_POINT('Ctrl Pts',(63.1569429707564,39.4864477303613,12.));
#111268=CARTESIAN_POINT('Ctrl Pts',(63.1630766582674,39.4958045828059,0.));
#111269=CARTESIAN_POINT('Ctrl Pts',(63.1630766582674,39.4958045828059,12.));
#111270=CARTESIAN_POINT('Ctrl Pts',(63.1661434108059,39.5004851439258,0.));
#111271=CARTESIAN_POINT('Ctrl Pts',(63.1661434108059,39.5004851439258,12.));
#111272=CARTESIAN_POINT('',(60.1903555511633,35.7368311217509,0.));
#111273=CARTESIAN_POINT('Ctrl Pts',(60.1903555511633,35.7368311217509,0.));
#111274=CARTESIAN_POINT('Ctrl Pts',(60.1930746580239,35.7396040203973,0.));
#111275=CARTESIAN_POINT('Ctrl Pts',(60.1985151474406,35.7451551752456,0.));
#111276=CARTESIAN_POINT('Ctrl Pts',(60.2066827086579,35.7534979801871,0.));
#111277=CARTESIAN_POINT('Ctrl Pts',(60.2175864449678,35.7646538667299,0.));
#111278=CARTESIAN_POINT('Ctrl Pts',(60.2312388621286,35.7786523045782,0.));
#111279=CARTESIAN_POINT('Ctrl Pts',(60.2449139865206,35.7927043145165,0.));
#111280=CARTESIAN_POINT('Ctrl Pts',(60.2586117365278,35.8068098723386,0.));
#111281=CARTESIAN_POINT('Ctrl Pts',(60.2723319687507,35.8209689272574,0.));
#111282=CARTESIAN_POINT('Ctrl Pts',(60.2860744798563,35.8351814020424,0.));
#111283=CARTESIAN_POINT('Ctrl Pts',(60.2998390330173,35.8494472046784,0.));
#111284=CARTESIAN_POINT('Ctrl Pts',(60.313625378281,35.8637662371635,0.));
#111285=CARTESIAN_POINT('Ctrl Pts',(60.3274332746782,35.878138405151,0.));
#111286=CARTESIAN_POINT('Ctrl Pts',(60.3412625135223,35.8925636280632,0.));
#111287=CARTESIAN_POINT('Ctrl Pts',(60.3551129108794,35.9070418358501,0.));
#111288=CARTESIAN_POINT('Ctrl Pts',(60.368984296546,35.9215729642219,0.));
#111289=CARTESIAN_POINT('Ctrl Pts',(60.3828765049031,35.9361569506955,0.));
#111290=CARTESIAN_POINT('Ctrl Pts',(60.3967893635487,35.9507937296726,0.));
#111291=CARTESIAN_POINT('Ctrl Pts',(60.4107226875759,35.9654832299627,0.));
#111292=CARTESIAN_POINT('Ctrl Pts',(60.4246762854961,35.9802253773534,0.));
#111293=CARTESIAN_POINT('Ctrl Pts',(60.438649962949,35.9950200962175,0.));
#111294=CARTESIAN_POINT('Ctrl Pts',(60.452643526964,36.0098673113557,0.));
#111295=CARTESIAN_POINT('Ctrl Pts',(60.4666567908053,36.0247669500867,0.));
#111296=CARTESIAN_POINT('Ctrl Pts',(60.4806895737643,36.0397189421617,0.));
#111297=CARTESIAN_POINT('Ctrl Pts',(60.4947416988396,36.0547232187681,0.));
#111298=CARTESIAN_POINT('Ctrl Pts',(60.5088129911357,36.0697797118377,0.));
#111299=CARTESIAN_POINT('Ctrl Pts',(60.5229032759001,36.0848883531969,0.));
#111300=CARTESIAN_POINT('Ctrl Pts',(60.5370123768841,36.1000490738532,0.));
#111301=CARTESIAN_POINT('Ctrl Pts',(60.5511401172014,36.1152618043756,0.));
#111302=CARTESIAN_POINT('Ctrl Pts',(60.5652863200732,36.1305264752195,0.));
#111303=CARTESIAN_POINT('Ctrl Pts',(60.5794508095555,36.1458430170425,0.));
#111304=CARTESIAN_POINT('Ctrl Pts',(60.5936334114082,36.1612113610758,0.));
#111305=CARTESIAN_POINT('Ctrl Pts',(60.6078339534151,36.1766314392624,0.));
#111306=CARTESIAN_POINT('Ctrl Pts',(60.6220522649129,36.1921031840618,0.));
#111307=CARTESIAN_POINT('Ctrl Pts',(60.6362881765014,36.2076265283261,0.));
#111308=CARTESIAN_POINT('Ctrl Pts',(60.6505415197055,36.2232014051549,0.));
#111309=CARTESIAN_POINT('Ctrl Pts',(60.6648121265908,36.2388277477225,0.));
#111310=CARTESIAN_POINT('Ctrl Pts',(60.6790998297823,36.2545054892911,0.));
#111311=CARTESIAN_POINT('Ctrl Pts',(60.6934044626304,36.2702345632883,0.));
#111312=CARTESIAN_POINT('Ctrl Pts',(60.7077258593268,36.2860149033586,0.));
#111313=CARTESIAN_POINT('Ctrl Pts',(60.7220638550396,36.3018464434204,0.));
#111314=CARTESIAN_POINT('Ctrl Pts',(60.7364182860388,36.3177291177148,0.));
#111315=CARTESIAN_POINT('Ctrl Pts',(60.7507889896283,36.3336628607844,0.));
#111316=CARTESIAN_POINT('Ctrl Pts',(60.7651758040791,36.349647607448,0.));
#111317=CARTESIAN_POINT('Ctrl Pts',(60.779578568563,36.3656832927733,0.));
#111318=CARTESIAN_POINT('Ctrl Pts',(60.7939971230781,36.38176985204,0.));
#111319=CARTESIAN_POINT('Ctrl Pts',(60.8084313084009,36.3979072207174,0.));
#111320=CARTESIAN_POINT('Ctrl Pts',(60.8228809661179,36.414095334487,0.));
#111321=CARTESIAN_POINT('Ctrl Pts',(60.8373459386397,36.4303341292497,0.));
#111322=CARTESIAN_POINT('Ctrl Pts',(60.851826069218,36.4466235411353,0.));
#111323=CARTESIAN_POINT('Ctrl Pts',(60.8663212019646,36.4629635065037,0.));
#111324=CARTESIAN_POINT('Ctrl Pts',(60.8808311818489,36.4793539619459,0.));
#111325=CARTESIAN_POINT('Ctrl Pts',(60.8953558546791,36.4957948442832,0.));
#111326=CARTESIAN_POINT('Ctrl Pts',(60.9098950670847,36.5122860905611,0.));
#111327=CARTESIAN_POINT('Ctrl Pts',(60.924448666499,36.5288276380417,0.));
#111328=CARTESIAN_POINT('Ctrl Pts',(60.9390165011357,36.5454194241866,0.));
#111329=CARTESIAN_POINT('Ctrl Pts',(60.9535984199874,36.5620613866616,0.));
#111330=CARTESIAN_POINT('Ctrl Pts',(60.9681942728237,36.5787534633416,0.));
#111331=CARTESIAN_POINT('Ctrl Pts',(60.9828039101887,36.5954955923109,0.));
#111332=CARTESIAN_POINT('Ctrl Pts',(60.9974271833982,36.6122877118599,0.));
#111333=CARTESIAN_POINT('Ctrl Pts',(61.012063944535,36.6291297604775,0.));
#111334=CARTESIAN_POINT('Ctrl Pts',(61.0267140464434,36.6460216768553,0.));
#111335=CARTESIAN_POINT('Ctrl Pts',(61.0413773427204,36.6629633998886,0.));
#111336=CARTESIAN_POINT('Ctrl Pts',(61.0560536877084,36.6799548686741,0.));
#111337=CARTESIAN_POINT('Ctrl Pts',(61.0707429364841,36.6969960225019,0.));
#111338=CARTESIAN_POINT('Ctrl Pts',(61.085444944851,36.7140868008479,0.));
#111339=CARTESIAN_POINT('Ctrl Pts',(61.1001595693357,36.7312271433799,0.));
#111340=CARTESIAN_POINT('Ctrl Pts',(61.1148866671821,36.7484169899591,0.));
#111341=CARTESIAN_POINT('Ctrl Pts',(61.1296260963468,36.7656562806381,0.));
#111342=CARTESIAN_POINT('Ctrl Pts',(61.1443777154926,36.782944955654,0.));
#111343=CARTESIAN_POINT('Ctrl Pts',(61.1591413839809,36.8002829554221,0.));
#111344=CARTESIAN_POINT('Ctrl Pts',(61.1739169618688,36.8176702205436,0.));
#111345=CARTESIAN_POINT('Ctrl Pts',(61.1887043099026,36.8351066918043,0.));
#111346=CARTESIAN_POINT('Ctrl Pts',(61.2035032895121,36.8525923101736,0.));
#111347=CARTESIAN_POINT('Ctrl Pts',(61.2183137628031,36.8701270167954,0.));
#111348=CARTESIAN_POINT('Ctrl Pts',(61.2331355925513,36.8877107529844,0.));
#111349=CARTESIAN_POINT('Ctrl Pts',(61.2479686421979,36.9053434602324,0.));
#111350=CARTESIAN_POINT('Ctrl Pts',(61.2628127758443,36.9230250802079,0.));
#111351=CARTESIAN_POINT('Ctrl Pts',(61.2776678582474,36.9407555547542,0.));
#111352=CARTESIAN_POINT('Ctrl Pts',(61.2925337548113,36.9585348258798,0.));
#111353=CARTESIAN_POINT('Ctrl Pts',(61.3074103315834,36.976362835757,0.));
#111354=CARTESIAN_POINT('Ctrl Pts',(61.3222974552519,36.994239526729,0.));
#111355=CARTESIAN_POINT('Ctrl Pts',(61.3371949931396,37.0121648413088,0.));
#111356=CARTESIAN_POINT('Ctrl Pts',(61.352102813199,37.0301387221766,0.));
#111357=CARTESIAN_POINT('Ctrl Pts',(61.3670207840041,37.0481611121698,0.));
#111358=CARTESIAN_POINT('Ctrl Pts',(61.3819487747458,37.0662319542827,0.));
#111359=CARTESIAN_POINT('Ctrl Pts',(61.3968866552294,37.0843511916729,0.));
#111360=CARTESIAN_POINT('Ctrl Pts',(61.411834295869,37.1025187676597,0.));
#111361=CARTESIAN_POINT('Ctrl Pts',(61.4267915676834,37.1207346257229,0.));
#111362=CARTESIAN_POINT('Ctrl Pts',(61.4417583422888,37.138998709492,0.));
#111363=CARTESIAN_POINT('Ctrl Pts',(61.4567344918946,37.157310962747,0.));
#111364=CARTESIAN_POINT('Ctrl Pts',(61.471719889301,37.1756713294249,0.));
#111365=CARTESIAN_POINT('Ctrl Pts',(61.4867144078939,37.1940797536182,0.));
#111366=CARTESIAN_POINT('Ctrl Pts',(61.5017179216404,37.2125361795727,0.));
#111367=CARTESIAN_POINT('Ctrl Pts',(61.5167303050823,37.2310405516775,0.));
#111368=CARTESIAN_POINT('Ctrl Pts',(61.5317514333319,37.2495928144661,0.));
#111369=CARTESIAN_POINT('Ctrl Pts',(61.5467811820686,37.2681929126218,0.));
#111370=CARTESIAN_POINT('Ctrl Pts',(61.5618194275349,37.286840790977,0.));
#111371=CARTESIAN_POINT('Ctrl Pts',(61.5768660465313,37.3055363945108,0.));
#111372=CARTESIAN_POINT('Ctrl Pts',(61.591920916412,37.3242796683395,0.));
#111373=CARTESIAN_POINT('Ctrl Pts',(61.6069839150804,37.3430705577178,0.));
#111374=CARTESIAN_POINT('Ctrl Pts',(61.6220549209862,37.3619090080447,0.));
#111375=CARTESIAN_POINT('Ctrl Pts',(61.6371338131208,37.3807949648622,0.));
#111376=CARTESIAN_POINT('Ctrl Pts',(61.6522204710133,37.3997283738534,0.));
#111377=CARTESIAN_POINT('Ctrl Pts',(61.6673147747249,37.4187091808324,0.));
#111378=CARTESIAN_POINT('Ctrl Pts',(61.6824166048453,37.4377373317456,0.));
#111379=CARTESIAN_POINT('Ctrl Pts',(61.69752584249,37.4568127726776,0.));
#111380=CARTESIAN_POINT('Ctrl Pts',(61.7126423692965,37.4759354498509,0.));
#111381=CARTESIAN_POINT('Ctrl Pts',(61.7277660674203,37.4951053096235,0.));
#111382=CARTESIAN_POINT('Ctrl Pts',(61.7428968195296,37.5143222984794,0.));
#111383=CARTESIAN_POINT('Ctrl Pts',(61.7580345088014,37.5335863630286,0.));
#111384=CARTESIAN_POINT('Ctrl Pts',(61.7731790189191,37.5528974500142,0.));
#111385=CARTESIAN_POINT('Ctrl Pts',(61.7883302340689,37.5722555063112,0.));
#111386=CARTESIAN_POINT('Ctrl Pts',(61.8034880389362,37.5916604789252,0.));
#111387=CARTESIAN_POINT('Ctrl Pts',(61.8186523187011,37.6111123149836,0.));
#111388=CARTESIAN_POINT('Ctrl Pts',(61.8338229590345,37.6306109617341,0.));
#111389=CARTESIAN_POINT('Ctrl Pts',(61.848999846095,37.6501563665518,0.));
#111390=CARTESIAN_POINT('Ctrl Pts',(61.8641828665257,37.6697484769389,0.));
#111391=CARTESIAN_POINT('Ctrl Pts',(61.879371907451,37.689387240523,0.));
#111392=CARTESIAN_POINT('Ctrl Pts',(61.8945668564714,37.7090726050488,0.));
#111393=CARTESIAN_POINT('Ctrl Pts',(61.9097676016616,37.7288045183765,0.));
#111394=CARTESIAN_POINT('Ctrl Pts',(61.9249740315664,37.748582928488,0.));
#111395=CARTESIAN_POINT('Ctrl Pts',(61.940186035198,37.7684077834877,0.));
#111396=CARTESIAN_POINT('Ctrl Pts',(61.9554035020335,37.7882790316012,0.));
#111397=CARTESIAN_POINT('Ctrl Pts',(61.9706263220101,37.808196621168,0.));
#111398=CARTESIAN_POINT('Ctrl Pts',(61.9858543855221,37.8281605006371,0.));
#111399=CARTESIAN_POINT('Ctrl Pts',(62.0010875834176,37.8481706185742,0.));
#111400=CARTESIAN_POINT('Ctrl Pts',(62.0163258069954,37.8682269236628,0.));
#111401=CARTESIAN_POINT('Ctrl Pts',(62.0315689480022,37.888329364703,0.));
#111402=CARTESIAN_POINT('Ctrl Pts',(62.0468168986289,37.9084778906053,0.));
#111403=CARTESIAN_POINT('Ctrl Pts',(62.0620695515072,37.9286724503849,0.));
#111404=CARTESIAN_POINT('Ctrl Pts',(62.0773267997072,37.9489129931685,0.));
#111405=CARTESIAN_POINT('Ctrl Pts',(62.0925885367346,37.9691994681962,0.));
#111406=CARTESIAN_POINT('Ctrl Pts',(62.107854656528,37.9895318248212,0.));
#111407=CARTESIAN_POINT('Ctrl Pts',(62.1231250534558,38.0099100125041,0.));
#111408=CARTESIAN_POINT('Ctrl Pts',(62.1383996223136,38.0303339808059,0.));
#111409=CARTESIAN_POINT('Ctrl Pts',(62.153678258321,38.0508036793944,0.));
#111410=CARTESIAN_POINT('Ctrl Pts',(62.1689608571182,38.0713190580466,0.));
#111411=CARTESIAN_POINT('Ctrl Pts',(62.1842473147627,38.0918800666479,0.));
#111412=CARTESIAN_POINT('Ctrl Pts',(62.1995375277253,38.1124866551884,0.));
#111413=CARTESIAN_POINT('Ctrl Pts',(62.2148313928859,38.1331387737528,0.));
#111414=CARTESIAN_POINT('Ctrl Pts',(62.2301288075319,38.1538363725263,0.));
#111415=CARTESIAN_POINT('Ctrl Pts',(62.2454296693581,38.1745794017997,0.));
#111416=CARTESIAN_POINT('Ctrl Pts',(62.2607338764655,38.1953678119692,0.));
#111417=CARTESIAN_POINT('Ctrl Pts',(62.2760413273601,38.2162015535351,0.));
#111418=CARTESIAN_POINT('Ctrl Pts',(62.2913519209517,38.2370805770931,0.));
#111419=CARTESIAN_POINT('Ctrl Pts',(62.3066655565497,38.2580048333356,0.));
#111420=CARTESIAN_POINT('Ctrl Pts',(62.3219821338564,38.2789742730559,0.));
#111421=CARTESIAN_POINT('Ctrl Pts',(62.337301552961,38.2999888471474,0.));
#111422=CARTESIAN_POINT('Ctrl Pts',(62.3526237143338,38.3210485066003,0.));
#111423=CARTESIAN_POINT('Ctrl Pts',(62.3679485188178,38.3421532024915,0.));
#111424=CARTESIAN_POINT('Ctrl Pts',(62.3832758676281,38.3633028859835,0.));
#111425=CARTESIAN_POINT('Ctrl Pts',(62.3986056623587,38.384497508335,0.));
#111426=CARTESIAN_POINT('Ctrl Pts',(62.4139378049891,38.4057370209054,0.));
#111427=CARTESIAN_POINT('Ctrl Pts',(62.42927219789,38.4270213751567,0.));
#111428=CARTESIAN_POINT('Ctrl Pts',(62.4446087438304,38.4483505226511,0.));
#111429=CARTESIAN_POINT('Ctrl Pts',(62.4599473459799,38.4697244150473,0.));
#111430=CARTESIAN_POINT('Ctrl Pts',(62.4752879078842,38.4911430040988,0.));
#111431=CARTESIAN_POINT('Ctrl Pts',(62.4906303334435,38.5126062416496,0.));
#111432=CARTESIAN_POINT('Ctrl Pts',(62.50597452689,38.5341140796247,0.));
#111433=CARTESIAN_POINT('Ctrl Pts',(62.5213203927672,38.5556664700201,0.));
#111434=CARTESIAN_POINT('Ctrl Pts',(62.5366678359036,38.5772633648841,0.));
#111435=CARTESIAN_POINT('Ctrl Pts',(62.5520167614529,38.5989047163401,0.));
#111436=CARTESIAN_POINT('Ctrl Pts',(62.567367074937,38.6205904766078,0.));
#111437=CARTESIAN_POINT('Ctrl Pts',(62.5827186822923,38.6423205980214,0.));
#111438=CARTESIAN_POINT('Ctrl Pts',(62.5980714899048,38.6640950330418,0.));
#111439=CARTESIAN_POINT('Ctrl Pts',(62.6134254046732,38.6859137342726,0.));
#111440=CARTESIAN_POINT('Ctrl Pts',(62.6287803339534,38.7077766544411,0.));
#111441=CARTESIAN_POINT('Ctrl Pts',(62.6441361854406,38.7296837463605,0.));
#111442=CARTESIAN_POINT('Ctrl Pts',(62.6594928670626,38.7516349628902,0.));
#111443=CARTESIAN_POINT('Ctrl Pts',(62.6748502868836,38.7736302568982,0.));
#111444=CARTESIAN_POINT('Ctrl Pts',(62.6902083529698,38.7956695812032,0.));
#111445=CARTESIAN_POINT('Ctrl Pts',(62.7055669733811,38.8177528885687,0.));
#111446=CARTESIAN_POINT('Ctrl Pts',(62.7209260564506,38.8398801318184,0.));
#111447=CARTESIAN_POINT('Ctrl Pts',(62.7362855110052,38.8620512639239,0.));
#111448=CARTESIAN_POINT('Ctrl Pts',(62.7516452466129,38.8842662380984,0.));
#111449=CARTESIAN_POINT('Ctrl Pts',(62.7670051738132,38.9065250078824,0.));
#111450=CARTESIAN_POINT('Ctrl Pts',(62.7823652043677,38.928827527232,0.));
#111451=CARTESIAN_POINT('Ctrl Pts',(62.797725250709,38.9511737503146,0.));
#111452=CARTESIAN_POINT('Ctrl Pts',(62.8130852254004,38.9735636313073,0.));
#111453=CARTESIAN_POINT('Ctrl Pts',(62.8284450405451,38.9959971241695,0.));
#111454=CARTESIAN_POINT('Ctrl Pts',(62.8438046073237,39.0184741824649,0.));
#111455=CARTESIAN_POINT('Ctrl Pts',(62.859163835209,39.0409947590519,0.));
#111456=CARTESIAN_POINT('Ctrl Pts',(62.8745226326046,39.0635588063309,0.));
#111457=CARTESIAN_POINT('Ctrl Pts',(62.8898809082659,39.0861662767964,0.));
#111458=CARTESIAN_POINT('Ctrl Pts',(62.9052385725416,39.1088171235144,0.));
#111459=CARTESIAN_POINT('Ctrl Pts',(62.9205955385551,39.1315113005745,0.));
#111460=CARTESIAN_POINT('Ctrl Pts',(62.9359517237352,39.1542487636708,0.));
#111461=CARTESIAN_POINT('Ctrl Pts',(62.9513070501777,39.1770294702367,0.));
#111462=CARTESIAN_POINT('Ctrl Pts',(62.9644687386694,39.1965939820804,0.));
#111463=CARTESIAN_POINT('Ctrl Pts',(62.9745590018501,39.2116170128279,0.));
#111464=CARTESIAN_POINT('Ctrl Pts',(62.9815782721131,39.2220794388576,0.));
#111465=CARTESIAN_POINT('Ctrl Pts',(62.9855268615905,39.2279686274724,0.));
#111466=CARTESIAN_POINT('Ctrl Pts',(62.9864049293634,39.2292784191472,0.));
#111467=CARTESIAN_POINT('',(60.1903555511633,35.7368311217509,12.));
#111468=CARTESIAN_POINT('',(60.1903555511633,35.7368311217509,0.));
#111469=CARTESIAN_POINT('Ctrl Pts',(62.9864049293634,39.2292784191472,12.));
#111470=CARTESIAN_POINT('Ctrl Pts',(62.9855268615905,39.2279686274724,12.));
#111471=CARTESIAN_POINT('Ctrl Pts',(62.9815782721131,39.2220794388576,12.));
#111472=CARTESIAN_POINT('Ctrl Pts',(62.9745590018501,39.2116170128279,12.));
#111473=CARTESIAN_POINT('Ctrl Pts',(62.9644687386694,39.1965939820804,12.));
#111474=CARTESIAN_POINT('Ctrl Pts',(62.9513070501777,39.1770294702367,12.));
#111475=CARTESIAN_POINT('Ctrl Pts',(62.9359517237352,39.1542487636708,12.));
#111476=CARTESIAN_POINT('Ctrl Pts',(62.9205955385551,39.1315113005745,12.));
#111477=CARTESIAN_POINT('Ctrl Pts',(62.9052385725416,39.1088171235144,12.));
#111478=CARTESIAN_POINT('Ctrl Pts',(62.8898809082659,39.0861662767964,12.));
#111479=CARTESIAN_POINT('Ctrl Pts',(62.8745226326046,39.0635588063309,12.));
#111480=CARTESIAN_POINT('Ctrl Pts',(62.859163835209,39.0409947590519,12.));
#111481=CARTESIAN_POINT('Ctrl Pts',(62.8438046073237,39.0184741824649,12.));
#111482=CARTESIAN_POINT('Ctrl Pts',(62.8284450405451,38.9959971241695,12.));
#111483=CARTESIAN_POINT('Ctrl Pts',(62.8130852254004,38.9735636313073,12.));
#111484=CARTESIAN_POINT('Ctrl Pts',(62.797725250709,38.9511737503146,12.));
#111485=CARTESIAN_POINT('Ctrl Pts',(62.7823652043677,38.928827527232,12.));
#111486=CARTESIAN_POINT('Ctrl Pts',(62.7670051738132,38.9065250078824,12.));
#111487=CARTESIAN_POINT('Ctrl Pts',(62.7516452466129,38.8842662380984,12.));
#111488=CARTESIAN_POINT('Ctrl Pts',(62.7362855110052,38.8620512639239,12.));
#111489=CARTESIAN_POINT('Ctrl Pts',(62.7209260564506,38.8398801318184,12.));
#111490=CARTESIAN_POINT('Ctrl Pts',(62.7055669733811,38.8177528885687,12.));
#111491=CARTESIAN_POINT('Ctrl Pts',(62.6902083529698,38.7956695812032,12.));
#111492=CARTESIAN_POINT('Ctrl Pts',(62.6748502868836,38.7736302568982,12.));
#111493=CARTESIAN_POINT('Ctrl Pts',(62.6594928670626,38.7516349628902,12.));
#111494=CARTESIAN_POINT('Ctrl Pts',(62.6441361854406,38.7296837463605,12.));
#111495=CARTESIAN_POINT('Ctrl Pts',(62.6287803339534,38.7077766544411,12.));
#111496=CARTESIAN_POINT('Ctrl Pts',(62.6134254046732,38.6859137342726,12.));
#111497=CARTESIAN_POINT('Ctrl Pts',(62.5980714899048,38.6640950330418,12.));
#111498=CARTESIAN_POINT('Ctrl Pts',(62.5827186822923,38.6423205980214,12.));
#111499=CARTESIAN_POINT('Ctrl Pts',(62.567367074937,38.6205904766078,12.));
#111500=CARTESIAN_POINT('Ctrl Pts',(62.5520167614529,38.5989047163401,12.));
#111501=CARTESIAN_POINT('Ctrl Pts',(62.5366678359036,38.5772633648841,12.));
#111502=CARTESIAN_POINT('Ctrl Pts',(62.5213203927672,38.5556664700201,12.));
#111503=CARTESIAN_POINT('Ctrl Pts',(62.50597452689,38.5341140796247,12.));
#111504=CARTESIAN_POINT('Ctrl Pts',(62.4906303334435,38.5126062416496,12.));
#111505=CARTESIAN_POINT('Ctrl Pts',(62.4752879078842,38.4911430040988,12.));
#111506=CARTESIAN_POINT('Ctrl Pts',(62.4599473459799,38.4697244150473,12.));
#111507=CARTESIAN_POINT('Ctrl Pts',(62.4446087438304,38.4483505226511,12.));
#111508=CARTESIAN_POINT('Ctrl Pts',(62.42927219789,38.4270213751567,12.));
#111509=CARTESIAN_POINT('Ctrl Pts',(62.4139378049891,38.4057370209054,12.));
#111510=CARTESIAN_POINT('Ctrl Pts',(62.3986056623587,38.384497508335,12.));
#111511=CARTESIAN_POINT('Ctrl Pts',(62.3832758676281,38.3633028859835,12.));
#111512=CARTESIAN_POINT('Ctrl Pts',(62.3679485188178,38.3421532024915,12.));
#111513=CARTESIAN_POINT('Ctrl Pts',(62.3526237143338,38.3210485066003,12.));
#111514=CARTESIAN_POINT('Ctrl Pts',(62.337301552961,38.2999888471474,12.));
#111515=CARTESIAN_POINT('Ctrl Pts',(62.3219821338564,38.2789742730559,12.));
#111516=CARTESIAN_POINT('Ctrl Pts',(62.3066655565497,38.2580048333356,12.));
#111517=CARTESIAN_POINT('Ctrl Pts',(62.2913519209517,38.2370805770931,12.));
#111518=CARTESIAN_POINT('Ctrl Pts',(62.2760413273601,38.2162015535351,12.));
#111519=CARTESIAN_POINT('Ctrl Pts',(62.2607338764655,38.1953678119692,12.));
#111520=CARTESIAN_POINT('Ctrl Pts',(62.2454296693581,38.1745794017997,12.));
#111521=CARTESIAN_POINT('Ctrl Pts',(62.2301288075319,38.1538363725263,12.));
#111522=CARTESIAN_POINT('Ctrl Pts',(62.2148313928859,38.1331387737528,12.));
#111523=CARTESIAN_POINT('Ctrl Pts',(62.1995375277253,38.1124866551884,12.));
#111524=CARTESIAN_POINT('Ctrl Pts',(62.1842473147627,38.0918800666479,12.));
#111525=CARTESIAN_POINT('Ctrl Pts',(62.1689608571182,38.0713190580466,12.));
#111526=CARTESIAN_POINT('Ctrl Pts',(62.153678258321,38.0508036793944,12.));
#111527=CARTESIAN_POINT('Ctrl Pts',(62.1383996223136,38.0303339808059,12.));
#111528=CARTESIAN_POINT('Ctrl Pts',(62.1231250534558,38.0099100125041,12.));
#111529=CARTESIAN_POINT('Ctrl Pts',(62.107854656528,37.9895318248212,12.));
#111530=CARTESIAN_POINT('Ctrl Pts',(62.0925885367346,37.9691994681962,12.));
#111531=CARTESIAN_POINT('Ctrl Pts',(62.0773267997072,37.9489129931685,12.));
#111532=CARTESIAN_POINT('Ctrl Pts',(62.0620695515072,37.9286724503849,12.));
#111533=CARTESIAN_POINT('Ctrl Pts',(62.0468168986289,37.9084778906053,12.));
#111534=CARTESIAN_POINT('Ctrl Pts',(62.0315689480022,37.888329364703,12.));
#111535=CARTESIAN_POINT('Ctrl Pts',(62.0163258069954,37.8682269236628,12.));
#111536=CARTESIAN_POINT('Ctrl Pts',(62.0010875834176,37.8481706185742,12.));
#111537=CARTESIAN_POINT('Ctrl Pts',(61.9858543855221,37.8281605006371,12.));
#111538=CARTESIAN_POINT('Ctrl Pts',(61.9706263220101,37.808196621168,12.));
#111539=CARTESIAN_POINT('Ctrl Pts',(61.9554035020335,37.7882790316012,12.));
#111540=CARTESIAN_POINT('Ctrl Pts',(61.940186035198,37.7684077834877,12.));
#111541=CARTESIAN_POINT('Ctrl Pts',(61.9249740315664,37.748582928488,12.));
#111542=CARTESIAN_POINT('Ctrl Pts',(61.9097676016616,37.7288045183765,12.));
#111543=CARTESIAN_POINT('Ctrl Pts',(61.8945668564714,37.7090726050488,12.));
#111544=CARTESIAN_POINT('Ctrl Pts',(61.879371907451,37.689387240523,12.));
#111545=CARTESIAN_POINT('Ctrl Pts',(61.8641828665257,37.6697484769389,12.));
#111546=CARTESIAN_POINT('Ctrl Pts',(61.848999846095,37.6501563665518,12.));
#111547=CARTESIAN_POINT('Ctrl Pts',(61.8338229590345,37.6306109617341,12.));
#111548=CARTESIAN_POINT('Ctrl Pts',(61.8186523187011,37.6111123149836,12.));
#111549=CARTESIAN_POINT('Ctrl Pts',(61.8034880389362,37.5916604789252,12.));
#111550=CARTESIAN_POINT('Ctrl Pts',(61.7883302340689,37.5722555063112,12.));
#111551=CARTESIAN_POINT('Ctrl Pts',(61.7731790189191,37.5528974500142,12.));
#111552=CARTESIAN_POINT('Ctrl Pts',(61.7580345088014,37.5335863630286,12.));
#111553=CARTESIAN_POINT('Ctrl Pts',(61.7428968195296,37.5143222984794,12.));
#111554=CARTESIAN_POINT('Ctrl Pts',(61.7277660674203,37.4951053096235,12.));
#111555=CARTESIAN_POINT('Ctrl Pts',(61.7126423692965,37.4759354498509,12.));
#111556=CARTESIAN_POINT('Ctrl Pts',(61.69752584249,37.4568127726776,12.));
#111557=CARTESIAN_POINT('Ctrl Pts',(61.6824166048453,37.4377373317456,12.));
#111558=CARTESIAN_POINT('Ctrl Pts',(61.6673147747249,37.4187091808324,12.));
#111559=CARTESIAN_POINT('Ctrl Pts',(61.6522204710133,37.3997283738534,12.));
#111560=CARTESIAN_POINT('Ctrl Pts',(61.6371338131208,37.3807949648622,12.));
#111561=CARTESIAN_POINT('Ctrl Pts',(61.6220549209862,37.3619090080447,12.));
#111562=CARTESIAN_POINT('Ctrl Pts',(61.6069839150804,37.3430705577178,12.));
#111563=CARTESIAN_POINT('Ctrl Pts',(61.591920916412,37.3242796683395,12.));
#111564=CARTESIAN_POINT('Ctrl Pts',(61.5768660465313,37.3055363945108,12.));
#111565=CARTESIAN_POINT('Ctrl Pts',(61.5618194275349,37.286840790977,12.));
#111566=CARTESIAN_POINT('Ctrl Pts',(61.5467811820686,37.2681929126218,12.));
#111567=CARTESIAN_POINT('Ctrl Pts',(61.5317514333319,37.2495928144661,12.));
#111568=CARTESIAN_POINT('Ctrl Pts',(61.5167303050823,37.2310405516775,12.));
#111569=CARTESIAN_POINT('Ctrl Pts',(61.5017179216404,37.2125361795727,12.));
#111570=CARTESIAN_POINT('Ctrl Pts',(61.4867144078939,37.1940797536182,12.));
#111571=CARTESIAN_POINT('Ctrl Pts',(61.471719889301,37.1756713294249,12.));
#111572=CARTESIAN_POINT('Ctrl Pts',(61.4567344918946,37.157310962747,12.));
#111573=CARTESIAN_POINT('Ctrl Pts',(61.4417583422888,37.138998709492,12.));
#111574=CARTESIAN_POINT('Ctrl Pts',(61.4267915676834,37.1207346257229,12.));
#111575=CARTESIAN_POINT('Ctrl Pts',(61.411834295869,37.1025187676597,12.));
#111576=CARTESIAN_POINT('Ctrl Pts',(61.3968866552294,37.0843511916729,12.));
#111577=CARTESIAN_POINT('Ctrl Pts',(61.3819487747458,37.0662319542827,12.));
#111578=CARTESIAN_POINT('Ctrl Pts',(61.3670207840041,37.0481611121698,12.));
#111579=CARTESIAN_POINT('Ctrl Pts',(61.352102813199,37.0301387221766,12.));
#111580=CARTESIAN_POINT('Ctrl Pts',(61.3371949931396,37.0121648413088,12.));
#111581=CARTESIAN_POINT('Ctrl Pts',(61.3222974552519,36.994239526729,12.));
#111582=CARTESIAN_POINT('Ctrl Pts',(61.3074103315834,36.976362835757,12.));
#111583=CARTESIAN_POINT('Ctrl Pts',(61.2925337548113,36.9585348258798,12.));
#111584=CARTESIAN_POINT('Ctrl Pts',(61.2776678582474,36.9407555547542,12.));
#111585=CARTESIAN_POINT('Ctrl Pts',(61.2628127758443,36.9230250802079,12.));
#111586=CARTESIAN_POINT('Ctrl Pts',(61.2479686421979,36.9053434602324,12.));
#111587=CARTESIAN_POINT('Ctrl Pts',(61.2331355925513,36.8877107529844,12.));
#111588=CARTESIAN_POINT('Ctrl Pts',(61.2183137628031,36.8701270167954,12.));
#111589=CARTESIAN_POINT('Ctrl Pts',(61.2035032895121,36.8525923101736,12.));
#111590=CARTESIAN_POINT('Ctrl Pts',(61.1887043099026,36.8351066918043,12.));
#111591=CARTESIAN_POINT('Ctrl Pts',(61.1739169618688,36.8176702205436,12.));
#111592=CARTESIAN_POINT('Ctrl Pts',(61.1591413839809,36.8002829554221,12.));
#111593=CARTESIAN_POINT('Ctrl Pts',(61.1443777154926,36.782944955654,12.));
#111594=CARTESIAN_POINT('Ctrl Pts',(61.1296260963468,36.7656562806381,12.));
#111595=CARTESIAN_POINT('Ctrl Pts',(61.1148866671821,36.7484169899591,12.));
#111596=CARTESIAN_POINT('Ctrl Pts',(61.1001595693357,36.7312271433799,12.));
#111597=CARTESIAN_POINT('Ctrl Pts',(61.085444944851,36.7140868008479,12.));
#111598=CARTESIAN_POINT('Ctrl Pts',(61.0707429364841,36.6969960225019,12.));
#111599=CARTESIAN_POINT('Ctrl Pts',(61.0560536877084,36.6799548686741,12.));
#111600=CARTESIAN_POINT('Ctrl Pts',(61.0413773427204,36.6629633998886,12.));
#111601=CARTESIAN_POINT('Ctrl Pts',(61.0267140464434,36.6460216768553,12.));
#111602=CARTESIAN_POINT('Ctrl Pts',(61.012063944535,36.6291297604775,12.));
#111603=CARTESIAN_POINT('Ctrl Pts',(60.9974271833982,36.6122877118599,12.));
#111604=CARTESIAN_POINT('Ctrl Pts',(60.9828039101887,36.5954955923109,12.));
#111605=CARTESIAN_POINT('Ctrl Pts',(60.9681942728237,36.5787534633416,12.));
#111606=CARTESIAN_POINT('Ctrl Pts',(60.9535984199874,36.5620613866616,12.));
#111607=CARTESIAN_POINT('Ctrl Pts',(60.9390165011357,36.5454194241866,12.));
#111608=CARTESIAN_POINT('Ctrl Pts',(60.924448666499,36.5288276380417,12.));
#111609=CARTESIAN_POINT('Ctrl Pts',(60.9098950670847,36.5122860905611,12.));
#111610=CARTESIAN_POINT('Ctrl Pts',(60.8953558546791,36.4957948442832,12.));
#111611=CARTESIAN_POINT('Ctrl Pts',(60.8808311818489,36.4793539619459,12.));
#111612=CARTESIAN_POINT('Ctrl Pts',(60.8663212019646,36.4629635065037,12.));
#111613=CARTESIAN_POINT('Ctrl Pts',(60.851826069218,36.4466235411353,12.));
#111614=CARTESIAN_POINT('Ctrl Pts',(60.8373459386397,36.4303341292497,12.));
#111615=CARTESIAN_POINT('Ctrl Pts',(60.8228809661179,36.414095334487,12.));
#111616=CARTESIAN_POINT('Ctrl Pts',(60.8084313084009,36.3979072207174,12.));
#111617=CARTESIAN_POINT('Ctrl Pts',(60.7939971230781,36.38176985204,12.));
#111618=CARTESIAN_POINT('Ctrl Pts',(60.779578568563,36.3656832927733,12.));
#111619=CARTESIAN_POINT('Ctrl Pts',(60.7651758040791,36.349647607448,12.));
#111620=CARTESIAN_POINT('Ctrl Pts',(60.7507889896283,36.3336628607844,12.));
#111621=CARTESIAN_POINT('Ctrl Pts',(60.7364182860388,36.3177291177148,12.));
#111622=CARTESIAN_POINT('Ctrl Pts',(60.7220638550396,36.3018464434204,12.));
#111623=CARTESIAN_POINT('Ctrl Pts',(60.7077258593268,36.2860149033586,12.));
#111624=CARTESIAN_POINT('Ctrl Pts',(60.6934044626304,36.2702345632883,12.));
#111625=CARTESIAN_POINT('Ctrl Pts',(60.6790998297823,36.2545054892911,12.));
#111626=CARTESIAN_POINT('Ctrl Pts',(60.6648121265908,36.2388277477225,12.));
#111627=CARTESIAN_POINT('Ctrl Pts',(60.6505415197055,36.2232014051549,12.));
#111628=CARTESIAN_POINT('Ctrl Pts',(60.6362881765014,36.2076265283261,12.));
#111629=CARTESIAN_POINT('Ctrl Pts',(60.6220522649129,36.1921031840618,12.));
#111630=CARTESIAN_POINT('Ctrl Pts',(60.6078339534151,36.1766314392624,12.));
#111631=CARTESIAN_POINT('Ctrl Pts',(60.5936334114082,36.1612113610758,12.));
#111632=CARTESIAN_POINT('Ctrl Pts',(60.5794508095555,36.1458430170425,12.));
#111633=CARTESIAN_POINT('Ctrl Pts',(60.5652863200732,36.1305264752195,12.));
#111634=CARTESIAN_POINT('Ctrl Pts',(60.5511401172014,36.1152618043756,12.));
#111635=CARTESIAN_POINT('Ctrl Pts',(60.5370123768841,36.1000490738532,12.));
#111636=CARTESIAN_POINT('Ctrl Pts',(60.5229032759001,36.0848883531969,12.));
#111637=CARTESIAN_POINT('Ctrl Pts',(60.5088129911357,36.0697797118377,12.));
#111638=CARTESIAN_POINT('Ctrl Pts',(60.4947416988396,36.0547232187681,12.));
#111639=CARTESIAN_POINT('Ctrl Pts',(60.4806895737643,36.0397189421617,12.));
#111640=CARTESIAN_POINT('Ctrl Pts',(60.4666567908053,36.0247669500867,12.));
#111641=CARTESIAN_POINT('Ctrl Pts',(60.452643526964,36.0098673113557,12.));
#111642=CARTESIAN_POINT('Ctrl Pts',(60.438649962949,35.9950200962175,12.));
#111643=CARTESIAN_POINT('Ctrl Pts',(60.4246762854961,35.9802253773534,12.));
#111644=CARTESIAN_POINT('Ctrl Pts',(60.4107226875759,35.9654832299627,12.));
#111645=CARTESIAN_POINT('Ctrl Pts',(60.3967893635487,35.9507937296726,12.));
#111646=CARTESIAN_POINT('Ctrl Pts',(60.3828765049031,35.9361569506955,12.));
#111647=CARTESIAN_POINT('Ctrl Pts',(60.368984296546,35.9215729642219,12.));
#111648=CARTESIAN_POINT('Ctrl Pts',(60.3551129108794,35.9070418358501,12.));
#111649=CARTESIAN_POINT('Ctrl Pts',(60.3412625135223,35.8925636280632,12.));
#111650=CARTESIAN_POINT('Ctrl Pts',(60.3274332746782,35.878138405151,12.));
#111651=CARTESIAN_POINT('Ctrl Pts',(60.313625378281,35.8637662371635,12.));
#111652=CARTESIAN_POINT('Ctrl Pts',(60.2998390330173,35.8494472046784,12.));
#111653=CARTESIAN_POINT('Ctrl Pts',(60.2860744798563,35.8351814020424,12.));
#111654=CARTESIAN_POINT('Ctrl Pts',(60.2723319687507,35.8209689272574,12.));
#111655=CARTESIAN_POINT('Ctrl Pts',(60.2586117365278,35.8068098723386,12.));
#111656=CARTESIAN_POINT('Ctrl Pts',(60.2449139865206,35.7927043145165,12.));
#111657=CARTESIAN_POINT('Ctrl Pts',(60.2312388621286,35.7786523045782,12.));
#111658=CARTESIAN_POINT('Ctrl Pts',(60.2175864449678,35.7646538667299,12.));
#111659=CARTESIAN_POINT('Ctrl Pts',(60.2066827086579,35.7534979801871,12.));
#111660=CARTESIAN_POINT('Ctrl Pts',(60.1985151474406,35.7451551752456,12.));
#111661=CARTESIAN_POINT('Ctrl Pts',(60.1930746580239,35.7396040203973,12.));
#111662=CARTESIAN_POINT('Ctrl Pts',(60.1903555511633,35.7368311217509,12.));
#111663=CARTESIAN_POINT('Ctrl Pts',(62.1730054756871,40.5060598100929,-1.11022302462516E-15));
#111664=CARTESIAN_POINT('Ctrl Pts',(62.1730054756871,40.5060598100929,4.));
#111665=CARTESIAN_POINT('Ctrl Pts',(62.1730054756872,40.5060598100929,8.));
#111666=CARTESIAN_POINT('Ctrl Pts',(62.1730054756872,40.5060598100929,12.));
#111667=CARTESIAN_POINT('Ctrl Pts',(62.2815834512355,40.5229411493977,-1.11022302462516E-15));
#111668=CARTESIAN_POINT('Ctrl Pts',(62.2815834512355,40.5229411493977,4.));
#111669=CARTESIAN_POINT('Ctrl Pts',(62.2815834512355,40.5229411493977,8.00000000000001));
#111670=CARTESIAN_POINT('Ctrl Pts',(62.2815834512355,40.5229411493977,12.));
#111671=CARTESIAN_POINT('Ctrl Pts',(62.4810961163745,40.4873422218648,-1.11022302462516E-15));
#111672=CARTESIAN_POINT('Ctrl Pts',(62.4810961163745,40.4873422218648,4.));
#111673=CARTESIAN_POINT('Ctrl Pts',(62.4810961163746,40.4873422218649,7.99999999999999));
#111674=CARTESIAN_POINT('Ctrl Pts',(62.4810961163746,40.4873422218649,12.));
#111675=CARTESIAN_POINT('Ctrl Pts',(62.6258675056116,40.3516729626244,-1.11022302462516E-15));
#111676=CARTESIAN_POINT('Ctrl Pts',(62.6258675056116,40.3516729626244,4.));
#111677=CARTESIAN_POINT('Ctrl Pts',(62.6258675056117,40.3516729626244,8.00000000000001));
#111678=CARTESIAN_POINT('Ctrl Pts',(62.6258675056117,40.3516729626244,12.));
#111679=CARTESIAN_POINT('Ctrl Pts',(62.6704278106374,40.282346977699,-1.11022302462516E-15));
#111680=CARTESIAN_POINT('Ctrl Pts',(62.6704278106374,40.282346977699,4.));
#111681=CARTESIAN_POINT('Ctrl Pts',(62.6704278106375,40.282346977699,8.));
#111682=CARTESIAN_POINT('Ctrl Pts',(62.6704278106375,40.282346977699,12.));
#111683=CARTESIAN_POINT('',(62.1730054756871,40.5060598100929,0.));
#111684=CARTESIAN_POINT('',(62.6704278106372,40.2823469776988,0.));
#111685=CARTESIAN_POINT('Ctrl Pts',(62.1730054756871,40.5060598100929,-2.77555756156289E-16));
#111686=CARTESIAN_POINT('Ctrl Pts',(62.2815834512355,40.5229411493977,-2.77555756156289E-16));
#111687=CARTESIAN_POINT('Ctrl Pts',(62.3955906884578,40.5025989050932,-2.77555756156289E-16));
#111688=CARTESIAN_POINT('Ctrl Pts',(62.4917232233448,40.4495806341087,-2.77555756156289E-16));
#111689=CARTESIAN_POINT('Ctrl Pts',(62.56382262451,40.4098169308703,-2.77555756156289E-16));
#111690=CARTESIAN_POINT('Ctrl Pts',(62.6258675056116,40.3516729626244,-2.7755575615629E-16));
#111691=CARTESIAN_POINT('Ctrl Pts',(62.6704278106374,40.282346977699,-2.77555756156289E-16));
#111692=CARTESIAN_POINT('',(62.6704278106372,40.2823469776988,12.));
#111693=CARTESIAN_POINT('Ctrl Pts',(62.6704278106374,40.282346977699,-1.11022302462516E-15));
#111694=CARTESIAN_POINT('Ctrl Pts',(62.6704278106374,40.282346977699,4.));
#111695=CARTESIAN_POINT('Ctrl Pts',(62.6704278106375,40.282346977699,8.));
#111696=CARTESIAN_POINT('Ctrl Pts',(62.6704278106375,40.282346977699,12.));
#111697=CARTESIAN_POINT('',(62.1730054756872,40.5060598100929,12.));
#111698=CARTESIAN_POINT('Ctrl Pts',(62.6704278106375,40.282346977699,12.));
#111699=CARTESIAN_POINT('Ctrl Pts',(62.6258675056117,40.3516729626244,12.));
#111700=CARTESIAN_POINT('Ctrl Pts',(62.5638226245101,40.4098169308703,12.));
#111701=CARTESIAN_POINT('Ctrl Pts',(62.4917232233448,40.4495806341087,12.));
#111702=CARTESIAN_POINT('Ctrl Pts',(62.3955906884578,40.5025989050932,12.));
#111703=CARTESIAN_POINT('Ctrl Pts',(62.2815834512355,40.5229411493977,12.));
#111704=CARTESIAN_POINT('Ctrl Pts',(62.1730054756872,40.5060598100929,12.));
#111705=CARTESIAN_POINT('Ctrl Pts',(62.1730054756872,40.5060598100929,12.));
#111706=CARTESIAN_POINT('Ctrl Pts',(62.1730054756872,40.5060598100929,8.));
#111707=CARTESIAN_POINT('Ctrl Pts',(62.1730054756871,40.5060598100929,4.));
#111708=CARTESIAN_POINT('Ctrl Pts',(62.1730054756871,40.5060598100929,-1.11022302462516E-15));
#111709=CARTESIAN_POINT('Origin',(3.16086693261782E-10,2.01487121870483E-10,
0.));
#111710=CARTESIAN_POINT('Origin',(3.16086693261782E-10,2.01487121870483E-10,
12.));
#111711=CARTESIAN_POINT('Origin',(3.16086693261782E-10,2.01487121870483E-10,
0.));
#111712=CARTESIAN_POINT('Ctrl Pts',(66.2207497120638,34.1330090612036,-1.11022302462516E-15));
#111713=CARTESIAN_POINT('Ctrl Pts',(66.2207497120638,34.1330090612036,4.));
#111714=CARTESIAN_POINT('Ctrl Pts',(66.2207497120638,34.1330090612036,8.));
#111715=CARTESIAN_POINT('Ctrl Pts',(66.2207497120638,34.1330090612036,12.));
#111716=CARTESIAN_POINT('Ctrl Pts',(66.2710935941675,34.035337929709,-1.11022302462516E-15));
#111717=CARTESIAN_POINT('Ctrl Pts',(66.2710935941675,34.035337929709,3.99999999999999));
#111718=CARTESIAN_POINT('Ctrl Pts',(66.2710935941675,34.035337929709,8.));
#111719=CARTESIAN_POINT('Ctrl Pts',(66.2710935941675,34.035337929709,12.));
#111720=CARTESIAN_POINT('Ctrl Pts',(66.3003999311009,33.8348041971636,-1.03714006649092E-15));
#111721=CARTESIAN_POINT('Ctrl Pts',(66.3003999311009,33.8348041971636,4.00000000000001));
#111722=CARTESIAN_POINT('Ctrl Pts',(66.3003999311009,33.8348041971637,8.));
#111723=CARTESIAN_POINT('Ctrl Pts',(66.3003999311009,33.8348041971637,12.));
#111724=CARTESIAN_POINT('Ctrl Pts',(66.2174610329232,33.6545652280944,-8.63611844392939E-16));
#111725=CARTESIAN_POINT('Ctrl Pts',(66.2174610329232,33.6545652280944,3.99999999999999));
#111726=CARTESIAN_POINT('Ctrl Pts',(66.2174610329232,33.6545652280945,8.));
#111727=CARTESIAN_POINT('Ctrl Pts',(66.2174610329232,33.6545652280945,12.));
#111728=CARTESIAN_POINT('Ctrl Pts',(66.1657795405672,33.5903722664961,-7.79957864155586E-16));
#111729=CARTESIAN_POINT('Ctrl Pts',(66.1657795405672,33.5903722664961,4.));
#111730=CARTESIAN_POINT('Ctrl Pts',(66.1657795405672,33.5903722664962,8.));
#111731=CARTESIAN_POINT('Ctrl Pts',(66.1657795405672,33.5903722664962,12.));
#111732=CARTESIAN_POINT('',(66.2207497120638,34.1330090612036,0.));
#111733=CARTESIAN_POINT('',(66.1657795405672,33.5903722664961,0.));
#111734=CARTESIAN_POINT('Ctrl Pts',(66.2207497120638,34.1330090612036,1.47525527571556E-16));
#111735=CARTESIAN_POINT('Ctrl Pts',(66.2710935941675,34.035337929709,1.47525527571554E-16));
#111736=CARTESIAN_POINT('Ctrl Pts',(66.2878400724152,33.9207472253973,1.8928721793398E-16));
#111737=CARTESIAN_POINT('Ctrl Pts',(66.2679350453204,33.8127833826289,2.63847361835582E-16));
#111738=CARTESIAN_POINT('Ctrl Pts',(66.2530062749993,33.7318105005526,3.19767469761783E-16));
#111739=CARTESIAN_POINT('Ctrl Pts',(66.2174610329232,33.6545652280944,3.94136707803771E-16));
#111740=CARTESIAN_POINT('Ctrl Pts',(66.1657795405672,33.5903722664961,4.77790688041126E-16));
#111741=CARTESIAN_POINT('',(66.1657795405673,33.5903722664962,12.));
#111742=CARTESIAN_POINT('Ctrl Pts',(66.1657795405672,33.5903722664961,-7.79957864155586E-16));
#111743=CARTESIAN_POINT('Ctrl Pts',(66.1657795405672,33.5903722664961,4.));
#111744=CARTESIAN_POINT('Ctrl Pts',(66.1657795405672,33.5903722664962,8.));
#111745=CARTESIAN_POINT('Ctrl Pts',(66.1657795405672,33.5903722664962,12.));
#111746=CARTESIAN_POINT('',(66.2207497120638,34.1330090612036,12.));
#111747=CARTESIAN_POINT('Ctrl Pts',(66.1657795405672,33.5903722664962,12.));
#111748=CARTESIAN_POINT('Ctrl Pts',(66.2174610329232,33.6545652280945,12.));
#111749=CARTESIAN_POINT('Ctrl Pts',(66.2530062749993,33.7318105005527,12.));
#111750=CARTESIAN_POINT('Ctrl Pts',(66.2679350453204,33.812783382629,12.));
#111751=CARTESIAN_POINT('Ctrl Pts',(66.2878400724151,33.9207472253974,12.));
#111752=CARTESIAN_POINT('Ctrl Pts',(66.2710935941675,34.035337929709,12.));
#111753=CARTESIAN_POINT('Ctrl Pts',(66.2207497120638,34.1330090612036,12.));
#111754=CARTESIAN_POINT('Ctrl Pts',(66.2207497120638,34.1330090612036,12.));
#111755=CARTESIAN_POINT('Ctrl Pts',(66.2207497120638,34.1330090612036,8.));
#111756=CARTESIAN_POINT('Ctrl Pts',(66.2207497120638,34.1330090612036,4.));
#111757=CARTESIAN_POINT('Ctrl Pts',(66.2207497120638,34.1330090612036,-1.11022302462516E-15));
#111758=CARTESIAN_POINT('Ctrl Pts',(63.0759831361898,30.3549065457811,0.));
#111759=CARTESIAN_POINT('Ctrl Pts',(63.0759831361898,30.3549065457811,12.));
#111760=CARTESIAN_POINT('Ctrl Pts',(63.078933570069,30.357431906933,0.));
#111761=CARTESIAN_POINT('Ctrl Pts',(63.078933570069,30.357431906933,12.));
#111762=CARTESIAN_POINT('Ctrl Pts',(63.0848371718048,30.3624877680651,0.));
#111763=CARTESIAN_POINT('Ctrl Pts',(63.0848371718048,30.3624877680651,12.));
#111764=CARTESIAN_POINT('Ctrl Pts',(63.0937007763471,30.3700869762507,0.));
#111765=CARTESIAN_POINT('Ctrl Pts',(63.0937007763471,30.3700869762507,12.));
#111766=CARTESIAN_POINT('Ctrl Pts',(63.105535320226,30.3802500880403,0.));
#111767=CARTESIAN_POINT('Ctrl Pts',(63.105535320226,30.3802500880403,12.));
#111768=CARTESIAN_POINT('Ctrl Pts',(63.1203558300657,30.3930053710484,0.));
#111769=CARTESIAN_POINT('Ctrl Pts',(63.1203558300657,30.3930053710484,12.));
#111770=CARTESIAN_POINT('Ctrl Pts',(63.135203629844,30.4058120432229,0.));
#111771=CARTESIAN_POINT('Ctrl Pts',(63.135203629844,30.4058120432229,12.));
#111772=CARTESIAN_POINT('Ctrl Pts',(63.1500786361459,30.418670087563,0.));
#111773=CARTESIAN_POINT('Ctrl Pts',(63.1500786361459,30.418670087563,12.));
#111774=CARTESIAN_POINT('Ctrl Pts',(63.164980701691,30.4315794659731,0.));
#111775=CARTESIAN_POINT('Ctrl Pts',(63.164980701691,30.4315794659731,12.));
#111776=CARTESIAN_POINT('Ctrl Pts',(63.179909617189,30.4445401192381,0.));
#111777=CARTESIAN_POINT('Ctrl Pts',(63.179909617189,30.4445401192381,12.));
#111778=CARTESIAN_POINT('Ctrl Pts',(63.1948651386942,30.4575519763337,0.));
#111779=CARTESIAN_POINT('Ctrl Pts',(63.1948651386942,30.4575519763337,12.));
#111780=CARTESIAN_POINT('Ctrl Pts',(63.2098470086636,30.470614961416,0.));
#111781=CARTESIAN_POINT('Ctrl Pts',(63.2098470086636,30.470614961416,12.));
#111782=CARTESIAN_POINT('Ctrl Pts',(63.2248549788221,30.4837290014989,0.));
#111783=CARTESIAN_POINT('Ctrl Pts',(63.2248549788221,30.4837290014989,12.));
#111784=CARTESIAN_POINT('Ctrl Pts',(63.2398888342545,30.4968940344998,0.));
#111785=CARTESIAN_POINT('Ctrl Pts',(63.2398888342545,30.4968940344998,12.));
#111786=CARTESIAN_POINT('Ctrl Pts',(63.2549483856215,30.5101100066659,0.));
#111787=CARTESIAN_POINT('Ctrl Pts',(63.2549483856215,30.5101100066659,12.));
#111788=CARTESIAN_POINT('Ctrl Pts',(63.2700334577639,30.5233768687865,0.));
#111789=CARTESIAN_POINT('Ctrl Pts',(63.2700334577639,30.5233768687865,12.));
#111790=CARTESIAN_POINT('Ctrl Pts',(63.2851438802473,30.5366945730508,0.));
#111791=CARTESIAN_POINT('Ctrl Pts',(63.2851438802473,30.5366945730508,12.));
#111792=CARTESIAN_POINT('Ctrl Pts',(63.3002794756086,30.5500630691359,0.));
#111793=CARTESIAN_POINT('Ctrl Pts',(63.3002794756086,30.5500630691359,12.));
#111794=CARTESIAN_POINT('Ctrl Pts',(63.3154400534397,30.563482302238,0.));
#111795=CARTESIAN_POINT('Ctrl Pts',(63.3154400534397,30.563482302238,12.));
#111796=CARTESIAN_POINT('Ctrl Pts',(63.3306254165126,30.5769522151164,0.));
#111797=CARTESIAN_POINT('Ctrl Pts',(63.3306254165126,30.5769522151164,12.));
#111798=CARTESIAN_POINT('Ctrl Pts',(63.3458353646154,30.5904727493712,0.));
#111799=CARTESIAN_POINT('Ctrl Pts',(63.3458353646154,30.5904727493712,12.));
#111800=CARTESIAN_POINT('Ctrl Pts',(63.3610696989577,30.6040438469078,0.));
#111801=CARTESIAN_POINT('Ctrl Pts',(63.3610696989577,30.6040438469078,12.));
#111802=CARTESIAN_POINT('Ctrl Pts',(63.3763282271796,30.6176654515967,0.));
#111803=CARTESIAN_POINT('Ctrl Pts',(63.3763282271796,30.6176654515967,12.));
#111804=CARTESIAN_POINT('Ctrl Pts',(63.3916107631376,30.6313375092062,0.));
#111805=CARTESIAN_POINT('Ctrl Pts',(63.3916107631376,30.6313375092062,12.));
#111806=CARTESIAN_POINT('Ctrl Pts',(63.4069171245066,30.6450599666121,0.));
#111807=CARTESIAN_POINT('Ctrl Pts',(63.4069171245066,30.6450599666121,12.));
#111808=CARTESIAN_POINT('Ctrl Pts',(63.4222471311239,30.6588327712484,0.));
#111809=CARTESIAN_POINT('Ctrl Pts',(63.4222471311239,30.6588327712484,12.));
#111810=CARTESIAN_POINT('Ctrl Pts',(63.4376006029604,30.6726558704315,0.));
#111811=CARTESIAN_POINT('Ctrl Pts',(63.4376006029604,30.6726558704315,12.));
#111812=CARTESIAN_POINT('Ctrl Pts',(63.4529773584249,30.6865292107929,0.));
#111813=CARTESIAN_POINT('Ctrl Pts',(63.4529773584249,30.6865292107929,12.));
#111814=CARTESIAN_POINT('Ctrl Pts',(63.4683772152529,30.7004527385821,0.));
#111815=CARTESIAN_POINT('Ctrl Pts',(63.4683772152529,30.7004527385821,12.));
#111816=CARTESIAN_POINT('Ctrl Pts',(63.4837999912771,30.7144263999265,0.));
#111817=CARTESIAN_POINT('Ctrl Pts',(63.4837999912771,30.7144263999265,12.));
#111818=CARTESIAN_POINT('Ctrl Pts',(63.4992455051795,30.7284501410822,0.));
#111819=CARTESIAN_POINT('Ctrl Pts',(63.4992455051795,30.7284501410822,12.));
#111820=CARTESIAN_POINT('Ctrl Pts',(63.5147135773894,30.7425239087281,0.));
#111821=CARTESIAN_POINT('Ctrl Pts',(63.5147135773894,30.7425239087281,12.));
#111822=CARTESIAN_POINT('Ctrl Pts',(63.5302040304142,30.7566476500757,0.));
#111823=CARTESIAN_POINT('Ctrl Pts',(63.5302040304142,30.7566476500757,12.));
#111824=CARTESIAN_POINT('Ctrl Pts',(63.5457166883537,30.7708213127159,0.));
#111825=CARTESIAN_POINT('Ctrl Pts',(63.5457166883537,30.7708213127159,12.));
#111826=CARTESIAN_POINT('Ctrl Pts',(63.5612513766,30.7850448445205,0.));
#111827=CARTESIAN_POINT('Ctrl Pts',(63.5612513766,30.7850448445205,12.));
#111828=CARTESIAN_POINT('Ctrl Pts',(63.5768079214881,30.7993181935271,0.));
#111829=CARTESIAN_POINT('Ctrl Pts',(63.5768079214881,30.7993181935271,12.));
#111830=CARTESIAN_POINT('Ctrl Pts',(63.5923861498987,30.813641307801,0.));
#111831=CARTESIAN_POINT('Ctrl Pts',(63.5923861498987,30.813641307801,12.));
#111832=CARTESIAN_POINT('Ctrl Pts',(63.6079858892771,30.8280141354459,0.));
#111833=CARTESIAN_POINT('Ctrl Pts',(63.6079858892771,30.8280141354459,12.));
#111834=CARTESIAN_POINT('Ctrl Pts',(63.6236069678055,30.8424366246672,0.));
#111835=CARTESIAN_POINT('Ctrl Pts',(63.6236069678055,30.8424366246672,12.));
#111836=CARTESIAN_POINT('Ctrl Pts',(63.6392492145233,30.8569087238131,0.));
#111837=CARTESIAN_POINT('Ctrl Pts',(63.6392492145233,30.8569087238131,12.));
#111838=CARTESIAN_POINT('Ctrl Pts',(63.6549124594666,30.8714303814194,0.));
#111839=CARTESIAN_POINT('Ctrl Pts',(63.6549124594666,30.8714303814194,12.));
#111840=CARTESIAN_POINT('Ctrl Pts',(63.6705965337971,30.8860015462475,0.));
#111841=CARTESIAN_POINT('Ctrl Pts',(63.6705965337971,30.8860015462475,12.));
#111842=CARTESIAN_POINT('Ctrl Pts',(63.6863012697328,30.900622167269,0.));
#111843=CARTESIAN_POINT('Ctrl Pts',(63.6863012697328,30.900622167269,12.));
#111844=CARTESIAN_POINT('Ctrl Pts',(63.7020265004792,30.9152921936465,0.));
#111845=CARTESIAN_POINT('Ctrl Pts',(63.7020265004792,30.9152921936465,12.));
#111846=CARTESIAN_POINT('Ctrl Pts',(63.7177720601609,30.9300115747116,0.));
#111847=CARTESIAN_POINT('Ctrl Pts',(63.7177720601609,30.9300115747116,12.));
#111848=CARTESIAN_POINT('Ctrl Pts',(63.7335377837441,30.9447802599355,0.));
#111849=CARTESIAN_POINT('Ctrl Pts',(63.7335377837441,30.9447802599355,12.));
#111850=CARTESIAN_POINT('Ctrl Pts',(63.749323506987,30.9595981989104,0.));
#111851=CARTESIAN_POINT('Ctrl Pts',(63.749323506987,30.9595981989104,12.));
#111852=CARTESIAN_POINT('Ctrl Pts',(63.7651290664733,30.9744653413689,0.));
#111853=CARTESIAN_POINT('Ctrl Pts',(63.7651290664733,30.9744653413689,12.));
#111854=CARTESIAN_POINT('Ctrl Pts',(63.7809542996264,30.989381637191,0.));
#111855=CARTESIAN_POINT('Ctrl Pts',(63.7809542996264,30.989381637191,12.));
#111856=CARTESIAN_POINT('Ctrl Pts',(63.796799044728,31.0043470364108,0.));
#111857=CARTESIAN_POINT('Ctrl Pts',(63.796799044728,31.0043470364108,12.));
#111858=CARTESIAN_POINT('Ctrl Pts',(63.8126631409364,31.0193614892171,0.));
#111859=CARTESIAN_POINT('Ctrl Pts',(63.8126631409364,31.0193614892171,12.));
#111860=CARTESIAN_POINT('Ctrl Pts',(63.8285464282846,31.0344249459538,0.));
#111861=CARTESIAN_POINT('Ctrl Pts',(63.8285464282846,31.0344249459538,12.));
#111862=CARTESIAN_POINT('Ctrl Pts',(63.8444487476611,31.0495373571215,0.));
#111863=CARTESIAN_POINT('Ctrl Pts',(63.8444487476611,31.0495373571215,12.));
#111864=CARTESIAN_POINT('Ctrl Pts',(63.8603699407922,31.0646986733723,0.));
#111865=CARTESIAN_POINT('Ctrl Pts',(63.8603699407922,31.0646986733723,12.));
#111866=CARTESIAN_POINT('Ctrl Pts',(63.8763098502237,31.0799088455041,0.));
#111867=CARTESIAN_POINT('Ctrl Pts',(63.8763098502237,31.0799088455041,12.));
#111868=CARTESIAN_POINT('Ctrl Pts',(63.8922683192964,31.0951678244455,0.));
#111869=CARTESIAN_POINT('Ctrl Pts',(63.8922683192964,31.0951678244455,12.));
#111870=CARTESIAN_POINT('Ctrl Pts',(63.9082451921448,31.1104755612607,0.));
#111871=CARTESIAN_POINT('Ctrl Pts',(63.9082451921448,31.1104755612607,12.));
#111872=CARTESIAN_POINT('Ctrl Pts',(63.9242403136955,31.1258320071545,0.));
#111873=CARTESIAN_POINT('Ctrl Pts',(63.9242403136955,31.1258320071545,12.));
#111874=CARTESIAN_POINT('Ctrl Pts',(63.940253529665,31.1412371134727,0.));
#111875=CARTESIAN_POINT('Ctrl Pts',(63.940253529665,31.1412371134727,12.));
#111876=CARTESIAN_POINT('Ctrl Pts',(63.9562846865567,31.1566908316992,0.));
#111877=CARTESIAN_POINT('Ctrl Pts',(63.9562846865567,31.1566908316992,12.));
#111878=CARTESIAN_POINT('Ctrl Pts',(63.9723336316551,31.1721931134487,0.));
#111879=CARTESIAN_POINT('Ctrl Pts',(63.9723336316551,31.1721931134487,12.));
#111880=CARTESIAN_POINT('Ctrl Pts',(63.9884002130211,31.1877439104717,0.));
#111881=CARTESIAN_POINT('Ctrl Pts',(63.9884002130211,31.1877439104717,12.));
#111882=CARTESIAN_POINT('Ctrl Pts',(64.0044842794831,31.2033431746558,0.));
#111883=CARTESIAN_POINT('Ctrl Pts',(64.0044842794831,31.2033431746558,12.));
#111884=CARTESIAN_POINT('Ctrl Pts',(64.02058568063,31.2189908580245,0.));
#111885=CARTESIAN_POINT('Ctrl Pts',(64.02058568063,31.2189908580245,12.));
#111886=CARTESIAN_POINT('Ctrl Pts',(64.0367042667984,31.2346869127297,0.));
#111887=CARTESIAN_POINT('Ctrl Pts',(64.0367042667984,31.2346869127297,12.));
#111888=CARTESIAN_POINT('Ctrl Pts',(64.0528398890657,31.2504312910451,0.));
#111889=CARTESIAN_POINT('Ctrl Pts',(64.0528398890657,31.2504312910451,12.));
#111890=CARTESIAN_POINT('Ctrl Pts',(64.0689923992461,31.2662239453728,0.));
#111891=CARTESIAN_POINT('Ctrl Pts',(64.0689923992461,31.2662239453728,12.));
#111892=CARTESIAN_POINT('Ctrl Pts',(64.0851616498852,31.2820648282447,0.));
#111893=CARTESIAN_POINT('Ctrl Pts',(64.0851616498852,31.2820648282447,12.));
#111894=CARTESIAN_POINT('Ctrl Pts',(64.1013474942556,31.2979538923214,0.));
#111895=CARTESIAN_POINT('Ctrl Pts',(64.1013474942556,31.2979538923214,12.));
#111896=CARTESIAN_POINT('Ctrl Pts',(64.117549786349,31.3138910903859,0.));
#111897=CARTESIAN_POINT('Ctrl Pts',(64.117549786349,31.3138910903859,12.));
#111898=CARTESIAN_POINT('Ctrl Pts',(64.133768380869,31.3298763753377,0.));
#111899=CARTESIAN_POINT('Ctrl Pts',(64.133768380869,31.3298763753377,12.));
#111900=CARTESIAN_POINT('Ctrl Pts',(64.1500031332282,31.3459097002006,0.));
#111901=CARTESIAN_POINT('Ctrl Pts',(64.1500031332282,31.3459097002006,12.));
#111902=CARTESIAN_POINT('Ctrl Pts',(64.166253899542,31.3619910181228,0.));
#111903=CARTESIAN_POINT('Ctrl Pts',(64.166253899542,31.3619910181228,12.));
#111904=CARTESIAN_POINT('Ctrl Pts',(64.1825205366224,31.3781202823754,0.));
#111905=CARTESIAN_POINT('Ctrl Pts',(64.1825205366224,31.3781202823754,12.));
#111906=CARTESIAN_POINT('Ctrl Pts',(64.1988029019707,31.3942974463446,0.));
#111907=CARTESIAN_POINT('Ctrl Pts',(64.1988029019707,31.3942974463446,12.));
#111908=CARTESIAN_POINT('Ctrl Pts',(64.2151008537697,31.410522463528,0.));
#111909=CARTESIAN_POINT('Ctrl Pts',(64.2151008537697,31.410522463528,12.));
#111910=CARTESIAN_POINT('Ctrl Pts',(64.231414250881,31.4267952875423,0.));
#111911=CARTESIAN_POINT('Ctrl Pts',(64.231414250881,31.4267952875423,12.));
#111912=CARTESIAN_POINT('Ctrl Pts',(64.2477429528393,31.4431158721222,0.));
#111913=CARTESIAN_POINT('Ctrl Pts',(64.2477429528393,31.4431158721222,12.));
#111914=CARTESIAN_POINT('Ctrl Pts',(64.2640868198473,31.4594841711195,0.));
#111915=CARTESIAN_POINT('Ctrl Pts',(64.2640868198473,31.4594841711195,12.));
#111916=CARTESIAN_POINT('Ctrl Pts',(64.2804457127671,31.4759001384941,0.));
#111917=CARTESIAN_POINT('Ctrl Pts',(64.2804457127671,31.4759001384941,12.));
#111918=CARTESIAN_POINT('Ctrl Pts',(64.2968194931158,31.4923637283132,0.));
#111919=CARTESIAN_POINT('Ctrl Pts',(64.2968194931158,31.4923637283132,12.));
#111920=CARTESIAN_POINT('Ctrl Pts',(64.3132080230637,31.5088748947582,0.));
#111921=CARTESIAN_POINT('Ctrl Pts',(64.3132080230637,31.5088748947582,12.));
#111922=CARTESIAN_POINT('Ctrl Pts',(64.3296111654283,31.5254335921245,0.));
#111923=CARTESIAN_POINT('Ctrl Pts',(64.3296111654283,31.5254335921245,12.));
#111924=CARTESIAN_POINT('Ctrl Pts',(64.3460287836687,31.5420397748191,0.));
#111925=CARTESIAN_POINT('Ctrl Pts',(64.3460287836687,31.5420397748191,12.));
#111926=CARTESIAN_POINT('Ctrl Pts',(64.3624607418768,31.5586933973515,0.));
#111927=CARTESIAN_POINT('Ctrl Pts',(64.3624607418768,31.5586933973515,12.));
#111928=CARTESIAN_POINT('Ctrl Pts',(64.3789069047733,31.5753944143336,0.));
#111929=CARTESIAN_POINT('Ctrl Pts',(64.3789069047733,31.5753944143336,12.));
#111930=CARTESIAN_POINT('Ctrl Pts',(64.3953671377046,31.5921427804865,0.));
#111931=CARTESIAN_POINT('Ctrl Pts',(64.3953671377046,31.5921427804865,12.));
#111932=CARTESIAN_POINT('Ctrl Pts',(64.4118413066378,31.6089384506395,0.));
#111933=CARTESIAN_POINT('Ctrl Pts',(64.4118413066378,31.6089384506395,12.));
#111934=CARTESIAN_POINT('Ctrl Pts',(64.4283292781565,31.6257813797288,0.));
#111935=CARTESIAN_POINT('Ctrl Pts',(64.4283292781565,31.6257813797288,12.));
#111936=CARTESIAN_POINT('Ctrl Pts',(64.4448309194525,31.6426715227878,0.));
#111937=CARTESIAN_POINT('Ctrl Pts',(64.4448309194525,31.6426715227878,12.));
#111938=CARTESIAN_POINT('Ctrl Pts',(64.4613460983214,31.6596088349482,0.));
#111939=CARTESIAN_POINT('Ctrl Pts',(64.4613460983214,31.6596088349482,12.));
#111940=CARTESIAN_POINT('Ctrl Pts',(64.4778746831614,31.6765932714464,0.));
#111941=CARTESIAN_POINT('Ctrl Pts',(64.4778746831614,31.6765932714464,12.));
#111942=CARTESIAN_POINT('Ctrl Pts',(64.4944165429674,31.6936247876229,0.));
#111943=CARTESIAN_POINT('Ctrl Pts',(64.4944165429674,31.6936247876229,12.));
#111944=CARTESIAN_POINT('Ctrl Pts',(64.510971547327,31.7107033389201,0.));
#111945=CARTESIAN_POINT('Ctrl Pts',(64.510971547327,31.7107033389201,12.));
#111946=CARTESIAN_POINT('Ctrl Pts',(64.5275395664124,31.7278288808731,0.));
#111947=CARTESIAN_POINT('Ctrl Pts',(64.5275395664124,31.7278288808731,12.));
#111948=CARTESIAN_POINT('Ctrl Pts',(64.544120470977,31.7450013691112,0.));
#111949=CARTESIAN_POINT('Ctrl Pts',(64.544120470977,31.7450013691112,12.));
#111950=CARTESIAN_POINT('Ctrl Pts',(64.5607141323521,31.7622207593634,0.));
#111951=CARTESIAN_POINT('Ctrl Pts',(64.5607141323521,31.7622207593634,12.));
#111952=CARTESIAN_POINT('Ctrl Pts',(64.5773204224429,31.7794870074583,0.));
#111953=CARTESIAN_POINT('Ctrl Pts',(64.5773204224429,31.7794870074583,12.));
#111954=CARTESIAN_POINT('Ctrl Pts',(64.5939392137235,31.7968000693218,0.));
#111955=CARTESIAN_POINT('Ctrl Pts',(64.5939392137235,31.7968000693218,12.));
#111956=CARTESIAN_POINT('Ctrl Pts',(64.6105703792312,31.8141599009684,0.));
#111957=CARTESIAN_POINT('Ctrl Pts',(64.6105703792312,31.8141599009684,12.));
#111958=CARTESIAN_POINT('Ctrl Pts',(64.6272137925627,31.8315664585026,0.));
#111959=CARTESIAN_POINT('Ctrl Pts',(64.6272137925627,31.8315664585026,12.));
#111960=CARTESIAN_POINT('Ctrl Pts',(64.6438693278714,31.8490196981248,0.));
#111961=CARTESIAN_POINT('Ctrl Pts',(64.6438693278714,31.8490196981248,12.));
#111962=CARTESIAN_POINT('Ctrl Pts',(64.6605368598629,31.8665195761311,0.));
#111963=CARTESIAN_POINT('Ctrl Pts',(64.6605368598629,31.8665195761311,12.));
#111964=CARTESIAN_POINT('Ctrl Pts',(64.6772162637907,31.8840660489107,0.));
#111965=CARTESIAN_POINT('Ctrl Pts',(64.6772162637907,31.8840660489107,12.));
#111966=CARTESIAN_POINT('Ctrl Pts',(64.6939074154498,31.9016590729374,0.));
#111967=CARTESIAN_POINT('Ctrl Pts',(64.6939074154498,31.9016590729374,12.));
#111968=CARTESIAN_POINT('Ctrl Pts',(64.7106101911732,31.9192986047706,0.));
#111969=CARTESIAN_POINT('Ctrl Pts',(64.7106101911732,31.9192986047706,12.));
#111970=CARTESIAN_POINT('Ctrl Pts',(64.7273244678297,31.9369846010616,0.));
#111971=CARTESIAN_POINT('Ctrl Pts',(64.7273244678297,31.9369846010616,12.));
#111972=CARTESIAN_POINT('Ctrl Pts',(64.7440501228202,31.9547170185534,0.));
#111973=CARTESIAN_POINT('Ctrl Pts',(64.7440501228202,31.9547170185534,12.));
#111974=CARTESIAN_POINT('Ctrl Pts',(64.7607870340735,31.9724958140789,0.));
#111975=CARTESIAN_POINT('Ctrl Pts',(64.7607870340735,31.9724958140789,12.));
#111976=CARTESIAN_POINT('Ctrl Pts',(64.77753508004,31.990320944552,0.));
#111977=CARTESIAN_POINT('Ctrl Pts',(64.77753508004,31.990320944552,12.));
#111978=CARTESIAN_POINT('Ctrl Pts',(64.7942941396881,32.0081923669677,0.));
#111979=CARTESIAN_POINT('Ctrl Pts',(64.7942941396881,32.0081923669677,12.));
#111980=CARTESIAN_POINT('Ctrl Pts',(64.8110640925021,32.0261100384092,0.));
#111981=CARTESIAN_POINT('Ctrl Pts',(64.8110640925021,32.0261100384092,12.));
#111982=CARTESIAN_POINT('Ctrl Pts',(64.8278448184786,32.0440739160477,0.));
#111983=CARTESIAN_POINT('Ctrl Pts',(64.8278448184786,32.0440739160477,12.));
#111984=CARTESIAN_POINT('Ctrl Pts',(64.8446361981234,32.0620839571408,0.));
#111985=CARTESIAN_POINT('Ctrl Pts',(64.8446361981234,32.0620839571408,12.));
#111986=CARTESIAN_POINT('Ctrl Pts',(64.861438112445,32.0801401190241,0.));
#111987=CARTESIAN_POINT('Ctrl Pts',(64.861438112445,32.0801401190241,12.));
#111988=CARTESIAN_POINT('Ctrl Pts',(64.878250442952,32.0982423591108,0.));
#111989=CARTESIAN_POINT('Ctrl Pts',(64.878250442952,32.0982423591108,12.));
#111990=CARTESIAN_POINT('Ctrl Pts',(64.8950730716493,32.1163906348979,0.));
#111991=CARTESIAN_POINT('Ctrl Pts',(64.8950730716493,32.1163906348979,12.));
#111992=CARTESIAN_POINT('Ctrl Pts',(64.9119058810362,32.1345849039671,0.));
#111993=CARTESIAN_POINT('Ctrl Pts',(64.9119058810362,32.1345849039671,12.));
#111994=CARTESIAN_POINT('Ctrl Pts',(64.9287487541018,32.1528251239832,0.));
#111995=CARTESIAN_POINT('Ctrl Pts',(64.9287487541018,32.1528251239832,12.));
#111996=CARTESIAN_POINT('Ctrl Pts',(64.9456015743203,32.171111252686,0.));
#111997=CARTESIAN_POINT('Ctrl Pts',(64.9456015743203,32.171111252686,12.));
#111998=CARTESIAN_POINT('Ctrl Pts',(64.9624642256477,32.1894432478889,0.));
#111999=CARTESIAN_POINT('Ctrl Pts',(64.9624642256477,32.1894432478889,12.));
#112000=CARTESIAN_POINT('Ctrl Pts',(64.9793365925194,32.2078210674858,0.));
#112001=CARTESIAN_POINT('Ctrl Pts',(64.9793365925194,32.2078210674858,12.));
#112002=CARTESIAN_POINT('Ctrl Pts',(64.996218559847,32.2262446694516,0.));
#112003=CARTESIAN_POINT('Ctrl Pts',(64.996218559847,32.2262446694516,12.));
#112004=CARTESIAN_POINT('Ctrl Pts',(65.0131100130155,32.244714011842,0.));
#112005=CARTESIAN_POINT('Ctrl Pts',(65.0131100130155,32.244714011842,12.));
#112006=CARTESIAN_POINT('Ctrl Pts',(65.0300108378786,32.2632290527855,0.));
#112007=CARTESIAN_POINT('Ctrl Pts',(65.0300108378786,32.2632290527855,12.));
#112008=CARTESIAN_POINT('Ctrl Pts',(65.0469209207548,32.2817897504799,0.));
#112009=CARTESIAN_POINT('Ctrl Pts',(65.0469209207548,32.2817897504799,12.));
#112010=CARTESIAN_POINT('Ctrl Pts',(65.0638401484245,32.3003960632001,0.));
#112011=CARTESIAN_POINT('Ctrl Pts',(65.0638401484245,32.3003960632001,12.));
#112012=CARTESIAN_POINT('Ctrl Pts',(65.0807684081278,32.3190479492985,0.));
#112013=CARTESIAN_POINT('Ctrl Pts',(65.0807684081278,32.3190479492985,12.));
#112014=CARTESIAN_POINT('Ctrl Pts',(65.097705587561,32.3377453672052,0.));
#112015=CARTESIAN_POINT('Ctrl Pts',(65.097705587561,32.3377453672052,12.));
#112016=CARTESIAN_POINT('Ctrl Pts',(65.1146515748723,32.3564882754213,0.));
#112017=CARTESIAN_POINT('Ctrl Pts',(65.1146515748723,32.3564882754213,12.));
#112018=CARTESIAN_POINT('Ctrl Pts',(65.1316062586586,32.3752766325135,0.));
#112019=CARTESIAN_POINT('Ctrl Pts',(65.1316062586586,32.3752766325135,12.));
#112020=CARTESIAN_POINT('Ctrl Pts',(65.1485695279628,32.3941103971218,0.));
#112021=CARTESIAN_POINT('Ctrl Pts',(65.1485695279628,32.3941103971218,12.));
#112022=CARTESIAN_POINT('Ctrl Pts',(65.165541272272,32.4129895279612,0.));
#112023=CARTESIAN_POINT('Ctrl Pts',(65.165541272272,32.4129895279612,12.));
#112024=CARTESIAN_POINT('Ctrl Pts',(65.182521381514,32.4319139838212,0.));
#112025=CARTESIAN_POINT('Ctrl Pts',(65.182521381514,32.4319139838212,12.));
#112026=CARTESIAN_POINT('Ctrl Pts',(65.1995097460545,32.4508837235613,0.));
#112027=CARTESIAN_POINT('Ctrl Pts',(65.1995097460545,32.4508837235613,12.));
#112028=CARTESIAN_POINT('Ctrl Pts',(65.2165062566936,32.4698987061037,0.));
#112029=CARTESIAN_POINT('Ctrl Pts',(65.2165062566936,32.4698987061037,12.));
#112030=CARTESIAN_POINT('Ctrl Pts',(65.2335108046625,32.4889588904397,0.));
#112031=CARTESIAN_POINT('Ctrl Pts',(65.2335108046625,32.4889588904397,12.));
#112032=CARTESIAN_POINT('Ctrl Pts',(65.2505232816215,32.508064235633,0.));
#112033=CARTESIAN_POINT('Ctrl Pts',(65.2505232816215,32.508064235633,12.));
#112034=CARTESIAN_POINT('Ctrl Pts',(65.2675435796558,32.5272147008191,0.));
#112035=CARTESIAN_POINT('Ctrl Pts',(65.2675435796558,32.5272147008191,12.));
#112036=CARTESIAN_POINT('Ctrl Pts',(65.2845715912717,32.5464102452013,0.));
#112037=CARTESIAN_POINT('Ctrl Pts',(65.2845715912717,32.5464102452013,12.));
#112038=CARTESIAN_POINT('Ctrl Pts',(65.3016072093907,32.565650828042,0.));
#112039=CARTESIAN_POINT('Ctrl Pts',(65.3016072093907,32.565650828042,12.));
#112040=CARTESIAN_POINT('Ctrl Pts',(65.3186503273498,32.5849364086679,0.));
#112041=CARTESIAN_POINT('Ctrl Pts',(65.3186503273498,32.5849364086679,12.));
#112042=CARTESIAN_POINT('Ctrl Pts',(65.3357008389004,32.6042669464752,0.));
#112043=CARTESIAN_POINT('Ctrl Pts',(65.3357008389004,32.6042669464752,12.));
#112044=CARTESIAN_POINT('Ctrl Pts',(65.3527586382082,32.6236424009302,0.));
#112045=CARTESIAN_POINT('Ctrl Pts',(65.3527586382082,32.6236424009302,12.));
#112046=CARTESIAN_POINT('Ctrl Pts',(65.3698236198511,32.6430627315673,0.));
#112047=CARTESIAN_POINT('Ctrl Pts',(65.3698236198511,32.6430627315673,12.));
#112048=CARTESIAN_POINT('Ctrl Pts',(65.3868956788178,32.6625278979807,0.));
#112049=CARTESIAN_POINT('Ctrl Pts',(65.3868956788178,32.6625278979807,12.));
#112050=CARTESIAN_POINT('Ctrl Pts',(65.4039747105033,32.6820378598263,0.));
#112051=CARTESIAN_POINT('Ctrl Pts',(65.4039747105033,32.6820378598263,12.));
#112052=CARTESIAN_POINT('Ctrl Pts',(65.4210606107029,32.7015925768261,0.));
#112053=CARTESIAN_POINT('Ctrl Pts',(65.4210606107029,32.7015925768261,12.));
#112054=CARTESIAN_POINT('Ctrl Pts',(65.4381532756062,32.7211920087682,0.));
#112055=CARTESIAN_POINT('Ctrl Pts',(65.4381532756062,32.7211920087682,12.));
#112056=CARTESIAN_POINT('Ctrl Pts',(65.4552526017907,32.7408361155038,0.));
#112057=CARTESIAN_POINT('Ctrl Pts',(65.4552526017907,32.7408361155038,12.));
#112058=CARTESIAN_POINT('Ctrl Pts',(65.4723584862129,32.7605248569382,0.));
#112059=CARTESIAN_POINT('Ctrl Pts',(65.4723584862129,32.7605248569382,12.));
#112060=CARTESIAN_POINT('Ctrl Pts',(65.4894708262071,32.7802581930294,0.));
#112061=CARTESIAN_POINT('Ctrl Pts',(65.4894708262071,32.7802581930294,12.));
#112062=CARTESIAN_POINT('Ctrl Pts',(65.5065895194938,32.8000360837981,0.));
#112063=CARTESIAN_POINT('Ctrl Pts',(65.5065895194938,32.8000360837981,12.));
#112064=CARTESIAN_POINT('Ctrl Pts',(65.5237144641864,32.8198584893319,0.));
#112065=CARTESIAN_POINT('Ctrl Pts',(65.5237144641864,32.8198584893319,12.));
#112066=CARTESIAN_POINT('Ctrl Pts',(65.5408455587963,32.8397253697865,0.));
#112067=CARTESIAN_POINT('Ctrl Pts',(65.5408455587963,32.8397253697865,12.));
#112068=CARTESIAN_POINT('Ctrl Pts',(65.5579827022412,32.8596366853826,0.));
#112069=CARTESIAN_POINT('Ctrl Pts',(65.5579827022412,32.8596366853826,12.));
#112070=CARTESIAN_POINT('Ctrl Pts',(65.575125793846,32.8795923964022,0.));
#112071=CARTESIAN_POINT('Ctrl Pts',(65.575125793846,32.8795923964022,12.));
#112072=CARTESIAN_POINT('Ctrl Pts',(65.5922747333181,32.899592463189,0.));
#112073=CARTESIAN_POINT('Ctrl Pts',(65.5922747333181,32.899592463189,12.));
#112074=CARTESIAN_POINT('Ctrl Pts',(65.6094294207267,32.9196368461457,0.));
#112075=CARTESIAN_POINT('Ctrl Pts',(65.6094294207267,32.9196368461457,12.));
#112076=CARTESIAN_POINT('Ctrl Pts',(65.6265897564782,32.9397255057273,0.));
#112077=CARTESIAN_POINT('Ctrl Pts',(65.6265897564782,32.9397255057273,12.));
#112078=CARTESIAN_POINT('Ctrl Pts',(65.6437556412956,32.9598584024318,0.));
#112079=CARTESIAN_POINT('Ctrl Pts',(65.6437556412956,32.9598584024318,12.));
#112080=CARTESIAN_POINT('Ctrl Pts',(65.6609269761902,32.9800354967847,0.));
#112081=CARTESIAN_POINT('Ctrl Pts',(65.6609269761902,32.9800354967847,12.));
#112082=CARTESIAN_POINT('Ctrl Pts',(65.6781036625041,33.0002567493581,0.));
#112083=CARTESIAN_POINT('Ctrl Pts',(65.6781036625041,33.0002567493581,12.));
#112084=CARTESIAN_POINT('Ctrl Pts',(65.6952856019542,33.0205221207877,0.));
#112085=CARTESIAN_POINT('Ctrl Pts',(65.6952856019542,33.0205221207877,12.));
#112086=CARTESIAN_POINT('Ctrl Pts',(65.7124726966805,33.0408315717874,0.));
#112087=CARTESIAN_POINT('Ctrl Pts',(65.7124726966805,33.0408315717874,12.));
#112088=CARTESIAN_POINT('Ctrl Pts',(65.729664849282,33.061185063158,0.));
#112089=CARTESIAN_POINT('Ctrl Pts',(65.729664849282,33.061185063158,12.));
#112090=CARTESIAN_POINT('Ctrl Pts',(65.7468619628808,33.0815825557976,0.));
#112091=CARTESIAN_POINT('Ctrl Pts',(65.7468619628808,33.0815825557976,12.));
#112092=CARTESIAN_POINT('Ctrl Pts',(65.7640639410653,33.102024010688,0.));
#112093=CARTESIAN_POINT('Ctrl Pts',(65.7640639410653,33.102024010688,12.));
#112094=CARTESIAN_POINT('Ctrl Pts',(65.7812706877691,33.1225093888669,0.));
#112095=CARTESIAN_POINT('Ctrl Pts',(65.7812706877691,33.1225093888669,12.));
#112096=CARTESIAN_POINT('Ctrl Pts',(65.7984821071621,33.1430386513975,0.));
#112097=CARTESIAN_POINT('Ctrl Pts',(65.7984821071621,33.1430386513975,12.));
#112098=CARTESIAN_POINT('Ctrl Pts',(65.8156981035504,33.16361175934,0.));
#112099=CARTESIAN_POINT('Ctrl Pts',(65.8156981035504,33.16361175934,12.));
#112100=CARTESIAN_POINT('Ctrl Pts',(65.8329185812379,33.1842286737053,0.));
#112101=CARTESIAN_POINT('Ctrl Pts',(65.8329185812379,33.1842286737053,12.));
#112102=CARTESIAN_POINT('Ctrl Pts',(65.8501434445174,33.2048893554496,0.));
#112103=CARTESIAN_POINT('Ctrl Pts',(65.8501434445174,33.2048893554496,12.));
#112104=CARTESIAN_POINT('Ctrl Pts',(65.8673725979591,33.2255937655656,0.));
#112105=CARTESIAN_POINT('Ctrl Pts',(65.8673725979591,33.2255937655656,12.));
#112106=CARTESIAN_POINT('Ctrl Pts',(65.8846059466382,33.2463418651498,0.));
#112107=CARTESIAN_POINT('Ctrl Pts',(65.8846059466382,33.2463418651498,12.));
#112108=CARTESIAN_POINT('Ctrl Pts',(65.901843396389,33.2671336154754,0.));
#112109=CARTESIAN_POINT('Ctrl Pts',(65.901843396389,33.2671336154754,12.));
#112110=CARTESIAN_POINT('Ctrl Pts',(65.9190848540422,33.2879689780566,0.));
#112111=CARTESIAN_POINT('Ctrl Pts',(65.9190848540422,33.2879689780566,12.));
#112112=CARTESIAN_POINT('Ctrl Pts',(65.9363302276822,33.3088479147151,0.));
#112113=CARTESIAN_POINT('Ctrl Pts',(65.9363302276822,33.3088479147151,12.));
#112114=CARTESIAN_POINT('Ctrl Pts',(65.9535794260802,33.3297703874249,0.));
#112115=CARTESIAN_POINT('Ctrl Pts',(65.9535794260802,33.3297703874249,12.));
#112116=CARTESIAN_POINT('Ctrl Pts',(65.9708323581385,33.3507363581579,0.));
#112117=CARTESIAN_POINT('Ctrl Pts',(65.9708323581385,33.3507363581579,12.));
#112118=CARTESIAN_POINT('Ctrl Pts',(65.9880889322822,33.3717457887095,0.));
#112119=CARTESIAN_POINT('Ctrl Pts',(65.9880889322822,33.3717457887095,12.));
#112120=CARTESIAN_POINT('Ctrl Pts',(66.0053490559826,33.3927986405612,0.));
#112121=CARTESIAN_POINT('Ctrl Pts',(66.0053490559826,33.3927986405612,12.));
#112122=CARTESIAN_POINT('Ctrl Pts',(66.0226126349482,33.4138948746408,0.));
#112123=CARTESIAN_POINT('Ctrl Pts',(66.0226126349482,33.4138948746408,12.));
#112124=CARTESIAN_POINT('Ctrl Pts',(66.0398795737827,33.4350344515128,0.));
#112125=CARTESIAN_POINT('Ctrl Pts',(66.0398795737827,33.4350344515128,12.));
#112126=CARTESIAN_POINT('Ctrl Pts',(66.0571497774484,33.4562173318053,0.));
#112127=CARTESIAN_POINT('Ctrl Pts',(66.0571497774484,33.4562173318053,12.));
#112128=CARTESIAN_POINT('Ctrl Pts',(66.0744231525445,33.4774434765762,0.));
#112129=CARTESIAN_POINT('Ctrl Pts',(66.0744231525445,33.4774434765762,12.));
#112130=CARTESIAN_POINT('Ctrl Pts',(66.0916996085237,33.4987128476618,0.));
#112131=CARTESIAN_POINT('Ctrl Pts',(66.0916996085237,33.4987128476618,12.));
#112132=CARTESIAN_POINT('Ctrl Pts',(66.1089790592673,33.5200254081212,0.));
#112133=CARTESIAN_POINT('Ctrl Pts',(66.1089790592673,33.5200254081212,12.));
#112134=CARTESIAN_POINT('Ctrl Pts',(66.1262614234579,33.5413811223398,0.));
#112135=CARTESIAN_POINT('Ctrl Pts',(66.1262614234579,33.5413811223398,12.));
#112136=CARTESIAN_POINT('Ctrl Pts',(66.1435466210966,33.5627799550423,0.));
#112137=CARTESIAN_POINT('Ctrl Pts',(66.1435466210966,33.5627799550423,12.));
#112138=CARTESIAN_POINT('Ctrl Pts',(66.1608345707551,33.5842218705103,0.));
#112139=CARTESIAN_POINT('Ctrl Pts',(66.1608345707551,33.5842218705103,12.));
#112140=CARTESIAN_POINT('Ctrl Pts',(66.1781251863998,33.6057068316758,0.));
#112141=CARTESIAN_POINT('Ctrl Pts',(66.1781251863998,33.6057068316758,12.));
#112142=CARTESIAN_POINT('Ctrl Pts',(66.1954183747167,33.6272347993519,0.));
#112143=CARTESIAN_POINT('Ctrl Pts',(66.1954183747167,33.6272347993519,12.));
#112144=CARTESIAN_POINT('Ctrl Pts',(66.2127140313777,33.648805731163,0.));
#112145=CARTESIAN_POINT('Ctrl Pts',(66.2127140313777,33.648805731163,12.));
#112146=CARTESIAN_POINT('Ctrl Pts',(66.2300120464323,33.6704195830526,0.));
#112147=CARTESIAN_POINT('Ctrl Pts',(66.2300120464323,33.6704195830526,12.));
#112148=CARTESIAN_POINT('Ctrl Pts',(66.2473123109626,33.6920763111575,0.));
#112149=CARTESIAN_POINT('Ctrl Pts',(66.2473123109626,33.6920763111575,12.));
#112150=CARTESIAN_POINT('Ctrl Pts',(66.2646147235444,33.713775873597,0.));
#112151=CARTESIAN_POINT('Ctrl Pts',(66.2646147235444,33.713775873597,12.));
#112152=CARTESIAN_POINT('Ctrl Pts',(66.2819191962273,33.7355182321862,0.));
#112153=CARTESIAN_POINT('Ctrl Pts',(66.2819191962273,33.7355182321862,12.));
#112154=CARTESIAN_POINT('Ctrl Pts',(66.2992256621001,33.7573033544374,0.));
#112155=CARTESIAN_POINT('Ctrl Pts',(66.2992256621001,33.7573033544374,12.));
#112156=CARTESIAN_POINT('Ctrl Pts',(66.3165340771053,33.7791312144798,0.));
#112157=CARTESIAN_POINT('Ctrl Pts',(66.3165340771053,33.7791312144798,12.));
#112158=CARTESIAN_POINT('Ctrl Pts',(66.3338444143559,33.8010017925666,0.));
#112159=CARTESIAN_POINT('Ctrl Pts',(66.3338444143559,33.8010017925666,12.));
#112160=CARTESIAN_POINT('Ctrl Pts',(66.3476942111456,33.8185324184602,0.));
#112161=CARTESIAN_POINT('Ctrl Pts',(66.3476942111456,33.8185324184602,12.));
#112162=CARTESIAN_POINT('Ctrl Pts',(66.3580824155565,33.8316996011751,0.));
#112163=CARTESIAN_POINT('Ctrl Pts',(66.3580824155565,33.8316996011751,12.));
#112164=CARTESIAN_POINT('Ctrl Pts',(66.3650082659593,33.8404862618803,0.));
#112165=CARTESIAN_POINT('Ctrl Pts',(66.3650082659593,33.8404862618803,12.));
#112166=CARTESIAN_POINT('Ctrl Pts',(66.3684712863594,33.8448817269567,0.));
#112167=CARTESIAN_POINT('Ctrl Pts',(66.3684712863594,33.8448817269567,12.));
#112168=CARTESIAN_POINT('',(63.0759831361898,30.3549065457811,0.));
#112169=CARTESIAN_POINT('Ctrl Pts',(63.0759831361898,30.3549065457811,0.));
#112170=CARTESIAN_POINT('Ctrl Pts',(63.078933570069,30.357431906933,0.));
#112171=CARTESIAN_POINT('Ctrl Pts',(63.0848371718048,30.3624877680651,0.));
#112172=CARTESIAN_POINT('Ctrl Pts',(63.0937007763471,30.3700869762507,0.));
#112173=CARTESIAN_POINT('Ctrl Pts',(63.105535320226,30.3802500880403,0.));
#112174=CARTESIAN_POINT('Ctrl Pts',(63.1203558300657,30.3930053710484,0.));
#112175=CARTESIAN_POINT('Ctrl Pts',(63.135203629844,30.4058120432229,0.));
#112176=CARTESIAN_POINT('Ctrl Pts',(63.1500786361459,30.418670087563,0.));
#112177=CARTESIAN_POINT('Ctrl Pts',(63.164980701691,30.4315794659731,0.));
#112178=CARTESIAN_POINT('Ctrl Pts',(63.179909617189,30.4445401192381,0.));
#112179=CARTESIAN_POINT('Ctrl Pts',(63.1948651386942,30.4575519763337,0.));
#112180=CARTESIAN_POINT('Ctrl Pts',(63.2098470086636,30.470614961416,0.));
#112181=CARTESIAN_POINT('Ctrl Pts',(63.2248549788221,30.4837290014989,0.));
#112182=CARTESIAN_POINT('Ctrl Pts',(63.2398888342545,30.4968940344998,0.));
#112183=CARTESIAN_POINT('Ctrl Pts',(63.2549483856215,30.5101100066659,0.));
#112184=CARTESIAN_POINT('Ctrl Pts',(63.2700334577639,30.5233768687865,0.));
#112185=CARTESIAN_POINT('Ctrl Pts',(63.2851438802473,30.5366945730508,0.));
#112186=CARTESIAN_POINT('Ctrl Pts',(63.3002794756086,30.5500630691359,0.));
#112187=CARTESIAN_POINT('Ctrl Pts',(63.3154400534397,30.563482302238,0.));
#112188=CARTESIAN_POINT('Ctrl Pts',(63.3306254165126,30.5769522151164,0.));
#112189=CARTESIAN_POINT('Ctrl Pts',(63.3458353646154,30.5904727493712,0.));
#112190=CARTESIAN_POINT('Ctrl Pts',(63.3610696989577,30.6040438469078,0.));
#112191=CARTESIAN_POINT('Ctrl Pts',(63.3763282271796,30.6176654515967,0.));
#112192=CARTESIAN_POINT('Ctrl Pts',(63.3916107631376,30.6313375092062,0.));
#112193=CARTESIAN_POINT('Ctrl Pts',(63.4069171245066,30.6450599666121,0.));
#112194=CARTESIAN_POINT('Ctrl Pts',(63.4222471311239,30.6588327712484,0.));
#112195=CARTESIAN_POINT('Ctrl Pts',(63.4376006029604,30.6726558704315,0.));
#112196=CARTESIAN_POINT('Ctrl Pts',(63.4529773584249,30.6865292107929,0.));
#112197=CARTESIAN_POINT('Ctrl Pts',(63.4683772152529,30.7004527385821,0.));
#112198=CARTESIAN_POINT('Ctrl Pts',(63.4837999912771,30.7144263999265,0.));
#112199=CARTESIAN_POINT('Ctrl Pts',(63.4992455051795,30.7284501410822,0.));
#112200=CARTESIAN_POINT('Ctrl Pts',(63.5147135773894,30.7425239087281,0.));
#112201=CARTESIAN_POINT('Ctrl Pts',(63.5302040304142,30.7566476500757,0.));
#112202=CARTESIAN_POINT('Ctrl Pts',(63.5457166883537,30.7708213127159,0.));
#112203=CARTESIAN_POINT('Ctrl Pts',(63.5612513766,30.7850448445205,0.));
#112204=CARTESIAN_POINT('Ctrl Pts',(63.5768079214881,30.7993181935271,0.));
#112205=CARTESIAN_POINT('Ctrl Pts',(63.5923861498987,30.813641307801,0.));
#112206=CARTESIAN_POINT('Ctrl Pts',(63.6079858892771,30.8280141354459,0.));
#112207=CARTESIAN_POINT('Ctrl Pts',(63.6236069678055,30.8424366246672,0.));
#112208=CARTESIAN_POINT('Ctrl Pts',(63.6392492145233,30.8569087238131,0.));
#112209=CARTESIAN_POINT('Ctrl Pts',(63.6549124594666,30.8714303814194,0.));
#112210=CARTESIAN_POINT('Ctrl Pts',(63.6705965337971,30.8860015462475,0.));
#112211=CARTESIAN_POINT('Ctrl Pts',(63.6863012697328,30.900622167269,0.));
#112212=CARTESIAN_POINT('Ctrl Pts',(63.7020265004792,30.9152921936465,0.));
#112213=CARTESIAN_POINT('Ctrl Pts',(63.7177720601609,30.9300115747116,0.));
#112214=CARTESIAN_POINT('Ctrl Pts',(63.7335377837441,30.9447802599355,0.));
#112215=CARTESIAN_POINT('Ctrl Pts',(63.749323506987,30.9595981989104,0.));
#112216=CARTESIAN_POINT('Ctrl Pts',(63.7651290664733,30.9744653413689,0.));
#112217=CARTESIAN_POINT('Ctrl Pts',(63.7809542996264,30.989381637191,0.));
#112218=CARTESIAN_POINT('Ctrl Pts',(63.796799044728,31.0043470364108,0.));
#112219=CARTESIAN_POINT('Ctrl Pts',(63.8126631409364,31.0193614892171,0.));
#112220=CARTESIAN_POINT('Ctrl Pts',(63.8285464282846,31.0344249459538,0.));
#112221=CARTESIAN_POINT('Ctrl Pts',(63.8444487476611,31.0495373571215,0.));
#112222=CARTESIAN_POINT('Ctrl Pts',(63.8603699407922,31.0646986733723,0.));
#112223=CARTESIAN_POINT('Ctrl Pts',(63.8763098502237,31.0799088455041,0.));
#112224=CARTESIAN_POINT('Ctrl Pts',(63.8922683192964,31.0951678244455,0.));
#112225=CARTESIAN_POINT('Ctrl Pts',(63.9082451921448,31.1104755612607,0.));
#112226=CARTESIAN_POINT('Ctrl Pts',(63.9242403136955,31.1258320071545,0.));
#112227=CARTESIAN_POINT('Ctrl Pts',(63.940253529665,31.1412371134727,0.));
#112228=CARTESIAN_POINT('Ctrl Pts',(63.9562846865567,31.1566908316992,0.));
#112229=CARTESIAN_POINT('Ctrl Pts',(63.9723336316551,31.1721931134487,0.));
#112230=CARTESIAN_POINT('Ctrl Pts',(63.9884002130211,31.1877439104717,0.));
#112231=CARTESIAN_POINT('Ctrl Pts',(64.0044842794831,31.2033431746558,0.));
#112232=CARTESIAN_POINT('Ctrl Pts',(64.02058568063,31.2189908580245,0.));
#112233=CARTESIAN_POINT('Ctrl Pts',(64.0367042667984,31.2346869127297,0.));
#112234=CARTESIAN_POINT('Ctrl Pts',(64.0528398890657,31.2504312910451,0.));
#112235=CARTESIAN_POINT('Ctrl Pts',(64.0689923992461,31.2662239453728,0.));
#112236=CARTESIAN_POINT('Ctrl Pts',(64.0851616498852,31.2820648282447,0.));
#112237=CARTESIAN_POINT('Ctrl Pts',(64.1013474942556,31.2979538923214,0.));
#112238=CARTESIAN_POINT('Ctrl Pts',(64.117549786349,31.3138910903859,0.));
#112239=CARTESIAN_POINT('Ctrl Pts',(64.133768380869,31.3298763753377,0.));
#112240=CARTESIAN_POINT('Ctrl Pts',(64.1500031332282,31.3459097002006,0.));
#112241=CARTESIAN_POINT('Ctrl Pts',(64.166253899542,31.3619910181228,0.));
#112242=CARTESIAN_POINT('Ctrl Pts',(64.1825205366224,31.3781202823754,0.));
#112243=CARTESIAN_POINT('Ctrl Pts',(64.1988029019707,31.3942974463446,0.));
#112244=CARTESIAN_POINT('Ctrl Pts',(64.2151008537697,31.410522463528,0.));
#112245=CARTESIAN_POINT('Ctrl Pts',(64.231414250881,31.4267952875423,0.));
#112246=CARTESIAN_POINT('Ctrl Pts',(64.2477429528393,31.4431158721222,0.));
#112247=CARTESIAN_POINT('Ctrl Pts',(64.2640868198473,31.4594841711195,0.));
#112248=CARTESIAN_POINT('Ctrl Pts',(64.2804457127671,31.4759001384941,0.));
#112249=CARTESIAN_POINT('Ctrl Pts',(64.2968194931158,31.4923637283132,0.));
#112250=CARTESIAN_POINT('Ctrl Pts',(64.3132080230637,31.5088748947582,0.));
#112251=CARTESIAN_POINT('Ctrl Pts',(64.3296111654283,31.5254335921245,0.));
#112252=CARTESIAN_POINT('Ctrl Pts',(64.3460287836687,31.5420397748191,0.));
#112253=CARTESIAN_POINT('Ctrl Pts',(64.3624607418768,31.5586933973515,0.));
#112254=CARTESIAN_POINT('Ctrl Pts',(64.3789069047733,31.5753944143336,0.));
#112255=CARTESIAN_POINT('Ctrl Pts',(64.3953671377046,31.5921427804865,0.));
#112256=CARTESIAN_POINT('Ctrl Pts',(64.4118413066378,31.6089384506395,0.));
#112257=CARTESIAN_POINT('Ctrl Pts',(64.4283292781565,31.6257813797288,0.));
#112258=CARTESIAN_POINT('Ctrl Pts',(64.4448309194525,31.6426715227878,0.));
#112259=CARTESIAN_POINT('Ctrl Pts',(64.4613460983214,31.6596088349482,0.));
#112260=CARTESIAN_POINT('Ctrl Pts',(64.4778746831614,31.6765932714464,0.));
#112261=CARTESIAN_POINT('Ctrl Pts',(64.4944165429674,31.6936247876229,0.));
#112262=CARTESIAN_POINT('Ctrl Pts',(64.510971547327,31.7107033389201,0.));
#112263=CARTESIAN_POINT('Ctrl Pts',(64.5275395664124,31.7278288808731,0.));
#112264=CARTESIAN_POINT('Ctrl Pts',(64.544120470977,31.7450013691112,0.));
#112265=CARTESIAN_POINT('Ctrl Pts',(64.5607141323521,31.7622207593634,0.));
#112266=CARTESIAN_POINT('Ctrl Pts',(64.5773204224429,31.7794870074583,0.));
#112267=CARTESIAN_POINT('Ctrl Pts',(64.5939392137235,31.7968000693218,0.));
#112268=CARTESIAN_POINT('Ctrl Pts',(64.6105703792312,31.8141599009684,0.));
#112269=CARTESIAN_POINT('Ctrl Pts',(64.6272137925627,31.8315664585026,0.));
#112270=CARTESIAN_POINT('Ctrl Pts',(64.6438693278714,31.8490196981248,0.));
#112271=CARTESIAN_POINT('Ctrl Pts',(64.6605368598629,31.8665195761311,0.));
#112272=CARTESIAN_POINT('Ctrl Pts',(64.6772162637907,31.8840660489107,0.));
#112273=CARTESIAN_POINT('Ctrl Pts',(64.6939074154498,31.9016590729374,0.));
#112274=CARTESIAN_POINT('Ctrl Pts',(64.7106101911732,31.9192986047706,0.));
#112275=CARTESIAN_POINT('Ctrl Pts',(64.7273244678297,31.9369846010616,0.));
#112276=CARTESIAN_POINT('Ctrl Pts',(64.7440501228202,31.9547170185534,0.));
#112277=CARTESIAN_POINT('Ctrl Pts',(64.7607870340735,31.9724958140789,0.));
#112278=CARTESIAN_POINT('Ctrl Pts',(64.77753508004,31.990320944552,0.));
#112279=CARTESIAN_POINT('Ctrl Pts',(64.7942941396881,32.0081923669677,0.));
#112280=CARTESIAN_POINT('Ctrl Pts',(64.8110640925021,32.0261100384092,0.));
#112281=CARTESIAN_POINT('Ctrl Pts',(64.8278448184786,32.0440739160477,0.));
#112282=CARTESIAN_POINT('Ctrl Pts',(64.8446361981234,32.0620839571408,0.));
#112283=CARTESIAN_POINT('Ctrl Pts',(64.861438112445,32.0801401190241,0.));
#112284=CARTESIAN_POINT('Ctrl Pts',(64.878250442952,32.0982423591108,0.));
#112285=CARTESIAN_POINT('Ctrl Pts',(64.8950730716493,32.1163906348979,0.));
#112286=CARTESIAN_POINT('Ctrl Pts',(64.9119058810362,32.1345849039671,0.));
#112287=CARTESIAN_POINT('Ctrl Pts',(64.9287487541018,32.1528251239832,0.));
#112288=CARTESIAN_POINT('Ctrl Pts',(64.9456015743203,32.171111252686,0.));
#112289=CARTESIAN_POINT('Ctrl Pts',(64.9624642256477,32.1894432478889,0.));
#112290=CARTESIAN_POINT('Ctrl Pts',(64.9793365925194,32.2078210674858,0.));
#112291=CARTESIAN_POINT('Ctrl Pts',(64.996218559847,32.2262446694516,0.));
#112292=CARTESIAN_POINT('Ctrl Pts',(65.0131100130155,32.244714011842,0.));
#112293=CARTESIAN_POINT('Ctrl Pts',(65.0300108378786,32.2632290527855,0.));
#112294=CARTESIAN_POINT('Ctrl Pts',(65.0469209207548,32.2817897504799,0.));
#112295=CARTESIAN_POINT('Ctrl Pts',(65.0638401484245,32.3003960632001,0.));
#112296=CARTESIAN_POINT('Ctrl Pts',(65.0807684081278,32.3190479492985,0.));
#112297=CARTESIAN_POINT('Ctrl Pts',(65.097705587561,32.3377453672052,0.));
#112298=CARTESIAN_POINT('Ctrl Pts',(65.1146515748723,32.3564882754213,0.));
#112299=CARTESIAN_POINT('Ctrl Pts',(65.1316062586586,32.3752766325135,0.));
#112300=CARTESIAN_POINT('Ctrl Pts',(65.1485695279628,32.3941103971218,0.));
#112301=CARTESIAN_POINT('Ctrl Pts',(65.165541272272,32.4129895279612,0.));
#112302=CARTESIAN_POINT('Ctrl Pts',(65.182521381514,32.4319139838212,0.));
#112303=CARTESIAN_POINT('Ctrl Pts',(65.1995097460545,32.4508837235613,0.));
#112304=CARTESIAN_POINT('Ctrl Pts',(65.2165062566936,32.4698987061037,0.));
#112305=CARTESIAN_POINT('Ctrl Pts',(65.2335108046625,32.4889588904397,0.));
#112306=CARTESIAN_POINT('Ctrl Pts',(65.2505232816215,32.508064235633,0.));
#112307=CARTESIAN_POINT('Ctrl Pts',(65.2675435796558,32.5272147008191,0.));
#112308=CARTESIAN_POINT('Ctrl Pts',(65.2845715912717,32.5464102452013,0.));
#112309=CARTESIAN_POINT('Ctrl Pts',(65.3016072093907,32.565650828042,0.));
#112310=CARTESIAN_POINT('Ctrl Pts',(65.3186503273498,32.5849364086679,0.));
#112311=CARTESIAN_POINT('Ctrl Pts',(65.3357008389004,32.6042669464752,0.));
#112312=CARTESIAN_POINT('Ctrl Pts',(65.3527586382082,32.6236424009302,0.));
#112313=CARTESIAN_POINT('Ctrl Pts',(65.3698236198511,32.6430627315673,0.));
#112314=CARTESIAN_POINT('Ctrl Pts',(65.3868956788178,32.6625278979807,0.));
#112315=CARTESIAN_POINT('Ctrl Pts',(65.4039747105033,32.6820378598263,0.));
#112316=CARTESIAN_POINT('Ctrl Pts',(65.4210606107029,32.7015925768261,0.));
#112317=CARTESIAN_POINT('Ctrl Pts',(65.4381532756062,32.7211920087682,0.));
#112318=CARTESIAN_POINT('Ctrl Pts',(65.4552526017907,32.7408361155038,0.));
#112319=CARTESIAN_POINT('Ctrl Pts',(65.4723584862129,32.7605248569382,0.));
#112320=CARTESIAN_POINT('Ctrl Pts',(65.4894708262071,32.7802581930294,0.));
#112321=CARTESIAN_POINT('Ctrl Pts',(65.5065895194938,32.8000360837981,0.));
#112322=CARTESIAN_POINT('Ctrl Pts',(65.5237144641864,32.8198584893319,0.));
#112323=CARTESIAN_POINT('Ctrl Pts',(65.5408455587963,32.8397253697865,0.));
#112324=CARTESIAN_POINT('Ctrl Pts',(65.5579827022412,32.8596366853826,0.));
#112325=CARTESIAN_POINT('Ctrl Pts',(65.575125793846,32.8795923964022,0.));
#112326=CARTESIAN_POINT('Ctrl Pts',(65.5922747333181,32.899592463189,0.));
#112327=CARTESIAN_POINT('Ctrl Pts',(65.6094294207267,32.9196368461457,0.));
#112328=CARTESIAN_POINT('Ctrl Pts',(65.6265897564782,32.9397255057273,0.));
#112329=CARTESIAN_POINT('Ctrl Pts',(65.6437556412956,32.9598584024318,0.));
#112330=CARTESIAN_POINT('Ctrl Pts',(65.6609269761902,32.9800354967847,0.));
#112331=CARTESIAN_POINT('Ctrl Pts',(65.6781036625041,33.0002567493581,0.));
#112332=CARTESIAN_POINT('Ctrl Pts',(65.6952856019542,33.0205221207877,0.));
#112333=CARTESIAN_POINT('Ctrl Pts',(65.7124726966805,33.0408315717874,0.));
#112334=CARTESIAN_POINT('Ctrl Pts',(65.729664849282,33.061185063158,0.));
#112335=CARTESIAN_POINT('Ctrl Pts',(65.7468619628808,33.0815825557976,0.));
#112336=CARTESIAN_POINT('Ctrl Pts',(65.7640639410653,33.102024010688,0.));
#112337=CARTESIAN_POINT('Ctrl Pts',(65.7812706877691,33.1225093888669,0.));
#112338=CARTESIAN_POINT('Ctrl Pts',(65.7984821071621,33.1430386513975,0.));
#112339=CARTESIAN_POINT('Ctrl Pts',(65.8156981035504,33.16361175934,0.));
#112340=CARTESIAN_POINT('Ctrl Pts',(65.8329185812379,33.1842286737053,0.));
#112341=CARTESIAN_POINT('Ctrl Pts',(65.8501434445174,33.2048893554496,0.));
#112342=CARTESIAN_POINT('Ctrl Pts',(65.8673725979591,33.2255937655656,0.));
#112343=CARTESIAN_POINT('Ctrl Pts',(65.8846059466382,33.2463418651498,0.));
#112344=CARTESIAN_POINT('Ctrl Pts',(65.901843396389,33.2671336154754,0.));
#112345=CARTESIAN_POINT('Ctrl Pts',(65.9190848540422,33.2879689780566,0.));
#112346=CARTESIAN_POINT('Ctrl Pts',(65.9363302276822,33.3088479147151,0.));
#112347=CARTESIAN_POINT('Ctrl Pts',(65.9535794260802,33.3297703874249,0.));
#112348=CARTESIAN_POINT('Ctrl Pts',(65.9708323581385,33.3507363581579,0.));
#112349=CARTESIAN_POINT('Ctrl Pts',(65.9880889322822,33.3717457887095,0.));
#112350=CARTESIAN_POINT('Ctrl Pts',(66.0053490559826,33.3927986405612,0.));
#112351=CARTESIAN_POINT('Ctrl Pts',(66.0226126349482,33.4138948746408,0.));
#112352=CARTESIAN_POINT('Ctrl Pts',(66.0398795737827,33.4350344515128,0.));
#112353=CARTESIAN_POINT('Ctrl Pts',(66.0571497774484,33.4562173318053,0.));
#112354=CARTESIAN_POINT('Ctrl Pts',(66.0744231525445,33.4774434765762,0.));
#112355=CARTESIAN_POINT('Ctrl Pts',(66.0916996085237,33.4987128476618,0.));
#112356=CARTESIAN_POINT('Ctrl Pts',(66.1089790592673,33.5200254081212,0.));
#112357=CARTESIAN_POINT('Ctrl Pts',(66.1262614234579,33.5413811223398,0.));
#112358=CARTESIAN_POINT('Ctrl Pts',(66.1410781873125,33.5597240685729,0.));
#112359=CARTESIAN_POINT('Ctrl Pts',(66.1524393973986,33.5738105077708,0.));
#112360=CARTESIAN_POINT('Ctrl Pts',(66.1603438177307,33.5836213513975,0.));
#112361=CARTESIAN_POINT('Ctrl Pts',(66.164790658241,33.589143987623,0.));
#112362=CARTESIAN_POINT('Ctrl Pts',(66.1657795405672,33.590372266496,0.));
#112363=CARTESIAN_POINT('',(63.0759831361898,30.3549065457811,12.));
#112364=CARTESIAN_POINT('',(63.0759831361898,30.3549065457811,0.));
#112365=CARTESIAN_POINT('Ctrl Pts',(66.1657795405673,33.5903722664962,12.));
#112366=CARTESIAN_POINT('Ctrl Pts',(66.1647906582411,33.5891439876231,12.));
#112367=CARTESIAN_POINT('Ctrl Pts',(66.1603438177307,33.5836213513976,12.));
#112368=CARTESIAN_POINT('Ctrl Pts',(66.1524393973986,33.5738105077708,12.));
#112369=CARTESIAN_POINT('Ctrl Pts',(66.1410781873125,33.5597240685729,12.));
#112370=CARTESIAN_POINT('Ctrl Pts',(66.1262614234579,33.5413811223398,12.));
#112371=CARTESIAN_POINT('Ctrl Pts',(66.1089790592673,33.5200254081212,12.));
#112372=CARTESIAN_POINT('Ctrl Pts',(66.0916996085237,33.4987128476618,12.));
#112373=CARTESIAN_POINT('Ctrl Pts',(66.0744231525445,33.4774434765762,12.));
#112374=CARTESIAN_POINT('Ctrl Pts',(66.0571497774484,33.4562173318053,12.));
#112375=CARTESIAN_POINT('Ctrl Pts',(66.0398795737827,33.4350344515128,12.));
#112376=CARTESIAN_POINT('Ctrl Pts',(66.0226126349482,33.4138948746408,12.));
#112377=CARTESIAN_POINT('Ctrl Pts',(66.0053490559826,33.3927986405612,12.));
#112378=CARTESIAN_POINT('Ctrl Pts',(65.9880889322822,33.3717457887095,12.));
#112379=CARTESIAN_POINT('Ctrl Pts',(65.9708323581385,33.3507363581579,12.));
#112380=CARTESIAN_POINT('Ctrl Pts',(65.9535794260802,33.3297703874249,12.));
#112381=CARTESIAN_POINT('Ctrl Pts',(65.9363302276822,33.3088479147151,12.));
#112382=CARTESIAN_POINT('Ctrl Pts',(65.9190848540422,33.2879689780566,12.));
#112383=CARTESIAN_POINT('Ctrl Pts',(65.901843396389,33.2671336154754,12.));
#112384=CARTESIAN_POINT('Ctrl Pts',(65.8846059466382,33.2463418651498,12.));
#112385=CARTESIAN_POINT('Ctrl Pts',(65.8673725979591,33.2255937655656,12.));
#112386=CARTESIAN_POINT('Ctrl Pts',(65.8501434445174,33.2048893554496,12.));
#112387=CARTESIAN_POINT('Ctrl Pts',(65.8329185812379,33.1842286737053,12.));
#112388=CARTESIAN_POINT('Ctrl Pts',(65.8156981035504,33.16361175934,12.));
#112389=CARTESIAN_POINT('Ctrl Pts',(65.7984821071621,33.1430386513975,12.));
#112390=CARTESIAN_POINT('Ctrl Pts',(65.7812706877691,33.1225093888669,12.));
#112391=CARTESIAN_POINT('Ctrl Pts',(65.7640639410653,33.102024010688,12.));
#112392=CARTESIAN_POINT('Ctrl Pts',(65.7468619628808,33.0815825557976,12.));
#112393=CARTESIAN_POINT('Ctrl Pts',(65.729664849282,33.061185063158,12.));
#112394=CARTESIAN_POINT('Ctrl Pts',(65.7124726966805,33.0408315717874,12.));
#112395=CARTESIAN_POINT('Ctrl Pts',(65.6952856019542,33.0205221207877,12.));
#112396=CARTESIAN_POINT('Ctrl Pts',(65.6781036625041,33.0002567493581,12.));
#112397=CARTESIAN_POINT('Ctrl Pts',(65.6609269761902,32.9800354967847,12.));
#112398=CARTESIAN_POINT('Ctrl Pts',(65.6437556412956,32.9598584024318,12.));
#112399=CARTESIAN_POINT('Ctrl Pts',(65.6265897564782,32.9397255057273,12.));
#112400=CARTESIAN_POINT('Ctrl Pts',(65.6094294207267,32.9196368461457,12.));
#112401=CARTESIAN_POINT('Ctrl Pts',(65.5922747333181,32.899592463189,12.));
#112402=CARTESIAN_POINT('Ctrl Pts',(65.575125793846,32.8795923964022,12.));
#112403=CARTESIAN_POINT('Ctrl Pts',(65.5579827022412,32.8596366853826,12.));
#112404=CARTESIAN_POINT('Ctrl Pts',(65.5408455587963,32.8397253697865,12.));
#112405=CARTESIAN_POINT('Ctrl Pts',(65.5237144641864,32.8198584893319,12.));
#112406=CARTESIAN_POINT('Ctrl Pts',(65.5065895194938,32.8000360837981,12.));
#112407=CARTESIAN_POINT('Ctrl Pts',(65.4894708262071,32.7802581930294,12.));
#112408=CARTESIAN_POINT('Ctrl Pts',(65.4723584862129,32.7605248569382,12.));
#112409=CARTESIAN_POINT('Ctrl Pts',(65.4552526017907,32.7408361155038,12.));
#112410=CARTESIAN_POINT('Ctrl Pts',(65.4381532756062,32.7211920087682,12.));
#112411=CARTESIAN_POINT('Ctrl Pts',(65.4210606107029,32.7015925768261,12.));
#112412=CARTESIAN_POINT('Ctrl Pts',(65.4039747105033,32.6820378598263,12.));
#112413=CARTESIAN_POINT('Ctrl Pts',(65.3868956788178,32.6625278979807,12.));
#112414=CARTESIAN_POINT('Ctrl Pts',(65.3698236198511,32.6430627315673,12.));
#112415=CARTESIAN_POINT('Ctrl Pts',(65.3527586382082,32.6236424009302,12.));
#112416=CARTESIAN_POINT('Ctrl Pts',(65.3357008389004,32.6042669464752,12.));
#112417=CARTESIAN_POINT('Ctrl Pts',(65.3186503273498,32.5849364086679,12.));
#112418=CARTESIAN_POINT('Ctrl Pts',(65.3016072093907,32.565650828042,12.));
#112419=CARTESIAN_POINT('Ctrl Pts',(65.2845715912717,32.5464102452013,12.));
#112420=CARTESIAN_POINT('Ctrl Pts',(65.2675435796558,32.5272147008191,12.));
#112421=CARTESIAN_POINT('Ctrl Pts',(65.2505232816215,32.508064235633,12.));
#112422=CARTESIAN_POINT('Ctrl Pts',(65.2335108046625,32.4889588904397,12.));
#112423=CARTESIAN_POINT('Ctrl Pts',(65.2165062566936,32.4698987061037,12.));
#112424=CARTESIAN_POINT('Ctrl Pts',(65.1995097460545,32.4508837235613,12.));
#112425=CARTESIAN_POINT('Ctrl Pts',(65.182521381514,32.4319139838212,12.));
#112426=CARTESIAN_POINT('Ctrl Pts',(65.165541272272,32.4129895279612,12.));
#112427=CARTESIAN_POINT('Ctrl Pts',(65.1485695279628,32.3941103971218,12.));
#112428=CARTESIAN_POINT('Ctrl Pts',(65.1316062586586,32.3752766325135,12.));
#112429=CARTESIAN_POINT('Ctrl Pts',(65.1146515748723,32.3564882754213,12.));
#112430=CARTESIAN_POINT('Ctrl Pts',(65.097705587561,32.3377453672052,12.));
#112431=CARTESIAN_POINT('Ctrl Pts',(65.0807684081278,32.3190479492985,12.));
#112432=CARTESIAN_POINT('Ctrl Pts',(65.0638401484245,32.3003960632001,12.));
#112433=CARTESIAN_POINT('Ctrl Pts',(65.0469209207548,32.2817897504799,12.));
#112434=CARTESIAN_POINT('Ctrl Pts',(65.0300108378786,32.2632290527855,12.));
#112435=CARTESIAN_POINT('Ctrl Pts',(65.0131100130155,32.244714011842,12.));
#112436=CARTESIAN_POINT('Ctrl Pts',(64.996218559847,32.2262446694516,12.));
#112437=CARTESIAN_POINT('Ctrl Pts',(64.9793365925194,32.2078210674858,12.));
#112438=CARTESIAN_POINT('Ctrl Pts',(64.9624642256477,32.1894432478889,12.));
#112439=CARTESIAN_POINT('Ctrl Pts',(64.9456015743203,32.171111252686,12.));
#112440=CARTESIAN_POINT('Ctrl Pts',(64.9287487541018,32.1528251239832,12.));
#112441=CARTESIAN_POINT('Ctrl Pts',(64.9119058810362,32.1345849039671,12.));
#112442=CARTESIAN_POINT('Ctrl Pts',(64.8950730716493,32.1163906348979,12.));
#112443=CARTESIAN_POINT('Ctrl Pts',(64.878250442952,32.0982423591108,12.));
#112444=CARTESIAN_POINT('Ctrl Pts',(64.861438112445,32.0801401190241,12.));
#112445=CARTESIAN_POINT('Ctrl Pts',(64.8446361981234,32.0620839571408,12.));
#112446=CARTESIAN_POINT('Ctrl Pts',(64.8278448184786,32.0440739160477,12.));
#112447=CARTESIAN_POINT('Ctrl Pts',(64.8110640925021,32.0261100384092,12.));
#112448=CARTESIAN_POINT('Ctrl Pts',(64.7942941396881,32.0081923669677,12.));
#112449=CARTESIAN_POINT('Ctrl Pts',(64.77753508004,31.990320944552,12.));
#112450=CARTESIAN_POINT('Ctrl Pts',(64.7607870340735,31.9724958140789,12.));
#112451=CARTESIAN_POINT('Ctrl Pts',(64.7440501228202,31.9547170185534,12.));
#112452=CARTESIAN_POINT('Ctrl Pts',(64.7273244678297,31.9369846010616,12.));
#112453=CARTESIAN_POINT('Ctrl Pts',(64.7106101911732,31.9192986047706,12.));
#112454=CARTESIAN_POINT('Ctrl Pts',(64.6939074154498,31.9016590729374,12.));
#112455=CARTESIAN_POINT('Ctrl Pts',(64.6772162637907,31.8840660489107,12.));
#112456=CARTESIAN_POINT('Ctrl Pts',(64.6605368598629,31.8665195761311,12.));
#112457=CARTESIAN_POINT('Ctrl Pts',(64.6438693278714,31.8490196981248,12.));
#112458=CARTESIAN_POINT('Ctrl Pts',(64.6272137925627,31.8315664585026,12.));
#112459=CARTESIAN_POINT('Ctrl Pts',(64.6105703792312,31.8141599009684,12.));
#112460=CARTESIAN_POINT('Ctrl Pts',(64.5939392137235,31.7968000693218,12.));
#112461=CARTESIAN_POINT('Ctrl Pts',(64.5773204224429,31.7794870074583,12.));
#112462=CARTESIAN_POINT('Ctrl Pts',(64.5607141323521,31.7622207593634,12.));
#112463=CARTESIAN_POINT('Ctrl Pts',(64.544120470977,31.7450013691112,12.));
#112464=CARTESIAN_POINT('Ctrl Pts',(64.5275395664124,31.7278288808731,12.));
#112465=CARTESIAN_POINT('Ctrl Pts',(64.510971547327,31.7107033389201,12.));
#112466=CARTESIAN_POINT('Ctrl Pts',(64.4944165429674,31.6936247876229,12.));
#112467=CARTESIAN_POINT('Ctrl Pts',(64.4778746831614,31.6765932714464,12.));
#112468=CARTESIAN_POINT('Ctrl Pts',(64.4613460983214,31.6596088349482,12.));
#112469=CARTESIAN_POINT('Ctrl Pts',(64.4448309194525,31.6426715227878,12.));
#112470=CARTESIAN_POINT('Ctrl Pts',(64.4283292781565,31.6257813797288,12.));
#112471=CARTESIAN_POINT('Ctrl Pts',(64.4118413066378,31.6089384506395,12.));
#112472=CARTESIAN_POINT('Ctrl Pts',(64.3953671377046,31.5921427804865,12.));
#112473=CARTESIAN_POINT('Ctrl Pts',(64.3789069047733,31.5753944143336,12.));
#112474=CARTESIAN_POINT('Ctrl Pts',(64.3624607418768,31.5586933973515,12.));
#112475=CARTESIAN_POINT('Ctrl Pts',(64.3460287836687,31.5420397748191,12.));
#112476=CARTESIAN_POINT('Ctrl Pts',(64.3296111654283,31.5254335921245,12.));
#112477=CARTESIAN_POINT('Ctrl Pts',(64.3132080230637,31.5088748947582,12.));
#112478=CARTESIAN_POINT('Ctrl Pts',(64.2968194931158,31.4923637283132,12.));
#112479=CARTESIAN_POINT('Ctrl Pts',(64.2804457127671,31.4759001384941,12.));
#112480=CARTESIAN_POINT('Ctrl Pts',(64.2640868198473,31.4594841711195,12.));
#112481=CARTESIAN_POINT('Ctrl Pts',(64.2477429528393,31.4431158721222,12.));
#112482=CARTESIAN_POINT('Ctrl Pts',(64.231414250881,31.4267952875423,12.));
#112483=CARTESIAN_POINT('Ctrl Pts',(64.2151008537697,31.410522463528,12.));
#112484=CARTESIAN_POINT('Ctrl Pts',(64.1988029019707,31.3942974463446,12.));
#112485=CARTESIAN_POINT('Ctrl Pts',(64.1825205366224,31.3781202823754,12.));
#112486=CARTESIAN_POINT('Ctrl Pts',(64.166253899542,31.3619910181228,12.));
#112487=CARTESIAN_POINT('Ctrl Pts',(64.1500031332282,31.3459097002006,12.));
#112488=CARTESIAN_POINT('Ctrl Pts',(64.133768380869,31.3298763753377,12.));
#112489=CARTESIAN_POINT('Ctrl Pts',(64.117549786349,31.3138910903859,12.));
#112490=CARTESIAN_POINT('Ctrl Pts',(64.1013474942556,31.2979538923214,12.));
#112491=CARTESIAN_POINT('Ctrl Pts',(64.0851616498852,31.2820648282447,12.));
#112492=CARTESIAN_POINT('Ctrl Pts',(64.0689923992461,31.2662239453728,12.));
#112493=CARTESIAN_POINT('Ctrl Pts',(64.0528398890657,31.2504312910451,12.));
#112494=CARTESIAN_POINT('Ctrl Pts',(64.0367042667984,31.2346869127297,12.));
#112495=CARTESIAN_POINT('Ctrl Pts',(64.02058568063,31.2189908580245,12.));
#112496=CARTESIAN_POINT('Ctrl Pts',(64.0044842794831,31.2033431746558,12.));
#112497=CARTESIAN_POINT('Ctrl Pts',(63.9884002130211,31.1877439104717,12.));
#112498=CARTESIAN_POINT('Ctrl Pts',(63.9723336316551,31.1721931134487,12.));
#112499=CARTESIAN_POINT('Ctrl Pts',(63.9562846865567,31.1566908316992,12.));
#112500=CARTESIAN_POINT('Ctrl Pts',(63.940253529665,31.1412371134727,12.));
#112501=CARTESIAN_POINT('Ctrl Pts',(63.9242403136955,31.1258320071545,12.));
#112502=CARTESIAN_POINT('Ctrl Pts',(63.9082451921448,31.1104755612607,12.));
#112503=CARTESIAN_POINT('Ctrl Pts',(63.8922683192964,31.0951678244455,12.));
#112504=CARTESIAN_POINT('Ctrl Pts',(63.8763098502237,31.0799088455041,12.));
#112505=CARTESIAN_POINT('Ctrl Pts',(63.8603699407922,31.0646986733723,12.));
#112506=CARTESIAN_POINT('Ctrl Pts',(63.8444487476611,31.0495373571215,12.));
#112507=CARTESIAN_POINT('Ctrl Pts',(63.8285464282846,31.0344249459538,12.));
#112508=CARTESIAN_POINT('Ctrl Pts',(63.8126631409364,31.0193614892171,12.));
#112509=CARTESIAN_POINT('Ctrl Pts',(63.796799044728,31.0043470364108,12.));
#112510=CARTESIAN_POINT('Ctrl Pts',(63.7809542996264,30.989381637191,12.));
#112511=CARTESIAN_POINT('Ctrl Pts',(63.7651290664733,30.9744653413689,12.));
#112512=CARTESIAN_POINT('Ctrl Pts',(63.749323506987,30.9595981989104,12.));
#112513=CARTESIAN_POINT('Ctrl Pts',(63.7335377837441,30.9447802599355,12.));
#112514=CARTESIAN_POINT('Ctrl Pts',(63.7177720601609,30.9300115747116,12.));
#112515=CARTESIAN_POINT('Ctrl Pts',(63.7020265004792,30.9152921936465,12.));
#112516=CARTESIAN_POINT('Ctrl Pts',(63.6863012697328,30.900622167269,12.));
#112517=CARTESIAN_POINT('Ctrl Pts',(63.6705965337971,30.8860015462475,12.));
#112518=CARTESIAN_POINT('Ctrl Pts',(63.6549124594666,30.8714303814194,12.));
#112519=CARTESIAN_POINT('Ctrl Pts',(63.6392492145233,30.8569087238131,12.));
#112520=CARTESIAN_POINT('Ctrl Pts',(63.6236069678055,30.8424366246672,12.));
#112521=CARTESIAN_POINT('Ctrl Pts',(63.6079858892771,30.8280141354459,12.));
#112522=CARTESIAN_POINT('Ctrl Pts',(63.5923861498987,30.813641307801,12.));
#112523=CARTESIAN_POINT('Ctrl Pts',(63.5768079214881,30.7993181935271,12.));
#112524=CARTESIAN_POINT('Ctrl Pts',(63.5612513766,30.7850448445205,12.));
#112525=CARTESIAN_POINT('Ctrl Pts',(63.5457166883537,30.7708213127159,12.));
#112526=CARTESIAN_POINT('Ctrl Pts',(63.5302040304142,30.7566476500757,12.));
#112527=CARTESIAN_POINT('Ctrl Pts',(63.5147135773894,30.7425239087281,12.));
#112528=CARTESIAN_POINT('Ctrl Pts',(63.4992455051795,30.7284501410822,12.));
#112529=CARTESIAN_POINT('Ctrl Pts',(63.4837999912771,30.7144263999265,12.));
#112530=CARTESIAN_POINT('Ctrl Pts',(63.4683772152529,30.7004527385821,12.));
#112531=CARTESIAN_POINT('Ctrl Pts',(63.4529773584249,30.6865292107929,12.));
#112532=CARTESIAN_POINT('Ctrl Pts',(63.4376006029604,30.6726558704315,12.));
#112533=CARTESIAN_POINT('Ctrl Pts',(63.4222471311239,30.6588327712484,12.));
#112534=CARTESIAN_POINT('Ctrl Pts',(63.4069171245066,30.6450599666121,12.));
#112535=CARTESIAN_POINT('Ctrl Pts',(63.3916107631376,30.6313375092062,12.));
#112536=CARTESIAN_POINT('Ctrl Pts',(63.3763282271796,30.6176654515967,12.));
#112537=CARTESIAN_POINT('Ctrl Pts',(63.3610696989577,30.6040438469078,12.));
#112538=CARTESIAN_POINT('Ctrl Pts',(63.3458353646154,30.5904727493712,12.));
#112539=CARTESIAN_POINT('Ctrl Pts',(63.3306254165126,30.5769522151164,12.));
#112540=CARTESIAN_POINT('Ctrl Pts',(63.3154400534397,30.563482302238,12.));
#112541=CARTESIAN_POINT('Ctrl Pts',(63.3002794756086,30.5500630691359,12.));
#112542=CARTESIAN_POINT('Ctrl Pts',(63.2851438802473,30.5366945730508,12.));
#112543=CARTESIAN_POINT('Ctrl Pts',(63.2700334577639,30.5233768687865,12.));
#112544=CARTESIAN_POINT('Ctrl Pts',(63.2549483856215,30.5101100066659,12.));
#112545=CARTESIAN_POINT('Ctrl Pts',(63.2398888342545,30.4968940344998,12.));
#112546=CARTESIAN_POINT('Ctrl Pts',(63.2248549788221,30.4837290014989,12.));
#112547=CARTESIAN_POINT('Ctrl Pts',(63.2098470086636,30.470614961416,12.));
#112548=CARTESIAN_POINT('Ctrl Pts',(63.1948651386942,30.4575519763337,12.));
#112549=CARTESIAN_POINT('Ctrl Pts',(63.179909617189,30.4445401192381,12.));
#112550=CARTESIAN_POINT('Ctrl Pts',(63.164980701691,30.4315794659731,12.));
#112551=CARTESIAN_POINT('Ctrl Pts',(63.1500786361459,30.418670087563,12.));
#112552=CARTESIAN_POINT('Ctrl Pts',(63.135203629844,30.4058120432229,12.));
#112553=CARTESIAN_POINT('Ctrl Pts',(63.1203558300657,30.3930053710484,12.));
#112554=CARTESIAN_POINT('Ctrl Pts',(63.105535320226,30.3802500880403,12.));
#112555=CARTESIAN_POINT('Ctrl Pts',(63.0937007763471,30.3700869762507,12.));
#112556=CARTESIAN_POINT('Ctrl Pts',(63.0848371718048,30.3624877680651,12.));
#112557=CARTESIAN_POINT('Ctrl Pts',(63.078933570069,30.357431906933,12.));
#112558=CARTESIAN_POINT('Ctrl Pts',(63.0759831361898,30.3549065457811,12.));
#112559=CARTESIAN_POINT('Ctrl Pts',(65.4667541478388,34.933187552314,0.));
#112560=CARTESIAN_POINT('Ctrl Pts',(65.4667541478388,34.933187552314,4.));
#112561=CARTESIAN_POINT('Ctrl Pts',(65.4667541478387,34.933187552314,8.));
#112562=CARTESIAN_POINT('Ctrl Pts',(65.4667541478387,34.933187552314,12.));
#112563=CARTESIAN_POINT('Ctrl Pts',(65.5763902570752,34.940541458921,0.));
#112564=CARTESIAN_POINT('Ctrl Pts',(65.5763902570752,34.940541458921,4.));
#112565=CARTESIAN_POINT('Ctrl Pts',(65.576390257075,34.940541458921,8.));
#112566=CARTESIAN_POINT('Ctrl Pts',(65.576390257075,34.940541458921,12.));
#112567=CARTESIAN_POINT('Ctrl Pts',(65.772041268059,34.8876896346299,0.));
#112568=CARTESIAN_POINT('Ctrl Pts',(65.772041268059,34.8876896346299,4.));
#112569=CARTESIAN_POINT('Ctrl Pts',(65.7720412680589,34.8876896346299,7.99999999999999));
#112570=CARTESIAN_POINT('Ctrl Pts',(65.7720412680589,34.8876896346299,12.));
#112571=CARTESIAN_POINT('Ctrl Pts',(65.9044372006544,34.7399186668304,0.));
#112572=CARTESIAN_POINT('Ctrl Pts',(65.9044372006544,34.7399186668304,4.));
#112573=CARTESIAN_POINT('Ctrl Pts',(65.9044372006543,34.7399186668304,8.00000000000001));
#112574=CARTESIAN_POINT('Ctrl Pts',(65.9044372006543,34.7399186668304,12.));
#112575=CARTESIAN_POINT('Ctrl Pts',(65.9427857825585,34.6669728017261,0.));
#112576=CARTESIAN_POINT('Ctrl Pts',(65.9427857825585,34.6669728017261,4.));
#112577=CARTESIAN_POINT('Ctrl Pts',(65.9427857825584,34.6669728017261,8.));
#112578=CARTESIAN_POINT('Ctrl Pts',(65.9427857825584,34.6669728017261,12.));
#112579=CARTESIAN_POINT('',(65.4667541478388,34.933187552314,0.));
#112580=CARTESIAN_POINT('',(65.9427857825584,34.6669728017261,0.));
#112581=CARTESIAN_POINT('Ctrl Pts',(65.4667541478388,34.933187552314,3.76195697576961E-35));
#112582=CARTESIAN_POINT('Ctrl Pts',(65.5763902570752,34.940541458921,3.76195697576961E-35));
#112583=CARTESIAN_POINT('Ctrl Pts',(65.6881908347802,34.9103404164689,3.76195697576962E-35));
#112584=CARTESIAN_POINT('Ctrl Pts',(65.7793366930115,34.8491453679733,3.76195697576961E-35));
#112585=CARTESIAN_POINT('Ctrl Pts',(65.8476960866849,34.8032490816016,3.76195697576961E-35));
#112586=CARTESIAN_POINT('Ctrl Pts',(65.9044372006544,34.7399186668304,3.76195697576961E-35));
#112587=CARTESIAN_POINT('Ctrl Pts',(65.9427857825585,34.6669728017261,3.76195697576961E-35));
#112588=CARTESIAN_POINT('',(65.9427857825584,34.6669728017261,12.));
#112589=CARTESIAN_POINT('Ctrl Pts',(65.9427857825585,34.6669728017261,0.));
#112590=CARTESIAN_POINT('Ctrl Pts',(65.9427857825585,34.6669728017261,4.));
#112591=CARTESIAN_POINT('Ctrl Pts',(65.9427857825584,34.6669728017261,8.));
#112592=CARTESIAN_POINT('Ctrl Pts',(65.9427857825584,34.6669728017261,12.));
#112593=CARTESIAN_POINT('',(65.4667541478387,34.933187552314,12.));
#112594=CARTESIAN_POINT('Ctrl Pts',(65.9427857825584,34.6669728017261,12.));
#112595=CARTESIAN_POINT('Ctrl Pts',(65.9044372006543,34.7399186668304,12.));
#112596=CARTESIAN_POINT('Ctrl Pts',(65.8476960866848,34.8032490816016,12.));
#112597=CARTESIAN_POINT('Ctrl Pts',(65.7793366930113,34.8491453679733,12.));
#112598=CARTESIAN_POINT('Ctrl Pts',(65.6881908347801,34.9103404164689,12.));
#112599=CARTESIAN_POINT('Ctrl Pts',(65.576390257075,34.940541458921,12.));
#112600=CARTESIAN_POINT('Ctrl Pts',(65.4667541478387,34.933187552314,12.));
#112601=CARTESIAN_POINT('Ctrl Pts',(65.4667541478387,34.933187552314,12.));
#112602=CARTESIAN_POINT('Ctrl Pts',(65.4667541478387,34.933187552314,8.));
#112603=CARTESIAN_POINT('Ctrl Pts',(65.4667541478388,34.933187552314,4.));
#112604=CARTESIAN_POINT('Ctrl Pts',(65.4667541478388,34.933187552314,0.));
#112605=CARTESIAN_POINT('Origin',(3.32444647725448E-10,1.73171632017259E-10,
0.));
#112606=CARTESIAN_POINT('Origin',(3.32444647725448E-10,1.73171632017259E-10,
12.));
#112607=CARTESIAN_POINT('Origin',(3.32444647725448E-10,1.73171632017259E-10,
0.));
#112608=CARTESIAN_POINT('Ctrl Pts',(68.9436475237602,28.2316040302268,-5.55111512312578E-16));
#112609=CARTESIAN_POINT('Ctrl Pts',(68.9436475237602,28.2316040302268,4.));
#112610=CARTESIAN_POINT('Ctrl Pts',(68.9436475237602,28.2316040302269,8.));
#112611=CARTESIAN_POINT('Ctrl Pts',(68.9436475237602,28.2316040302269,12.));
#112612=CARTESIAN_POINT('Ctrl Pts',(68.9852872321828,28.1299168084378,-5.55111512312578E-16));
#112613=CARTESIAN_POINT('Ctrl Pts',(68.9852872321828,28.1299168084378,4.));
#112614=CARTESIAN_POINT('Ctrl Pts',(68.9852872321828,28.1299168084378,8.00000000000001));
#112615=CARTESIAN_POINT('Ctrl Pts',(68.9852872321828,28.1299168084378,12.));
#112616=CARTESIAN_POINT('Ctrl Pts',(68.9970049015576,27.9275918177432,-5.55111512312578E-16));
#112617=CARTESIAN_POINT('Ctrl Pts',(68.9970049015576,27.9275918177432,4.));
#112618=CARTESIAN_POINT('Ctrl Pts',(68.9970049015576,27.9275918177433,7.99999999999999));
#112619=CARTESIAN_POINT('Ctrl Pts',(68.9970049015576,27.9275918177433,12.));
#112620=CARTESIAN_POINT('Ctrl Pts',(68.8986722313991,27.7552674476222,-5.55111512312578E-16));
#112621=CARTESIAN_POINT('Ctrl Pts',(68.8986722313991,27.7552674476222,4.));
#112622=CARTESIAN_POINT('Ctrl Pts',(68.8986722313991,27.7552674476223,8.00000000000001));
#112623=CARTESIAN_POINT('Ctrl Pts',(68.8986722313991,27.7552674476223,12.));
#112624=CARTESIAN_POINT('Ctrl Pts',(68.8415926174774,27.6958230984758,-5.55111512312578E-16));
#112625=CARTESIAN_POINT('Ctrl Pts',(68.8415926174774,27.6958230984758,4.));
#112626=CARTESIAN_POINT('Ctrl Pts',(68.8415926174774,27.6958230984758,8.));
#112627=CARTESIAN_POINT('Ctrl Pts',(68.8415926174774,27.6958230984758,12.));
#112628=CARTESIAN_POINT('',(68.9436475237602,28.2316040302268,0.));
#112629=CARTESIAN_POINT('',(68.8415926174774,27.6958230984757,2.77555756156289E-16));
#112630=CARTESIAN_POINT('Ctrl Pts',(68.9436475237602,28.2316040302268,-5.55111512312578E-16));
#112631=CARTESIAN_POINT('Ctrl Pts',(68.9852872321828,28.1299168084378,-5.55111512312578E-16));
#112632=CARTESIAN_POINT('Ctrl Pts',(68.9919830432541,28.0143025280409,-5.55111512312578E-16));
#112633=CARTESIAN_POINT('Ctrl Pts',(68.9627440495799,27.9084843686476,-5.55111512312578E-16));
#112634=CARTESIAN_POINT('Ctrl Pts',(68.9408148043242,27.8291207491026,-5.55111512312578E-16));
#112635=CARTESIAN_POINT('Ctrl Pts',(68.8986722313991,27.7552674476222,-5.55111512312578E-16));
#112636=CARTESIAN_POINT('Ctrl Pts',(68.8415926174774,27.6958230984758,-5.55111512312578E-16));
#112637=CARTESIAN_POINT('',(68.8415926174774,27.6958230984758,12.));
#112638=CARTESIAN_POINT('Ctrl Pts',(68.8415926174774,27.6958230984758,-5.55111512312578E-16));
#112639=CARTESIAN_POINT('Ctrl Pts',(68.8415926174774,27.6958230984758,4.));
#112640=CARTESIAN_POINT('Ctrl Pts',(68.8415926174774,27.6958230984758,8.));
#112641=CARTESIAN_POINT('Ctrl Pts',(68.8415926174774,27.6958230984758,12.));
#112642=CARTESIAN_POINT('',(68.9436475237602,28.2316040302269,12.));
#112643=CARTESIAN_POINT('Ctrl Pts',(68.8415926174774,27.6958230984758,12.));
#112644=CARTESIAN_POINT('Ctrl Pts',(68.8986722313991,27.7552674476223,12.));
#112645=CARTESIAN_POINT('Ctrl Pts',(68.9408148043242,27.8291207491027,12.));
#112646=CARTESIAN_POINT('Ctrl Pts',(68.9627440495799,27.9084843686477,12.));
#112647=CARTESIAN_POINT('Ctrl Pts',(68.9919830432541,28.0143025280409,12.));
#112648=CARTESIAN_POINT('Ctrl Pts',(68.9852872321828,28.1299168084378,12.));
#112649=CARTESIAN_POINT('Ctrl Pts',(68.9436475237602,28.2316040302269,12.));
#112650=CARTESIAN_POINT('Ctrl Pts',(68.9436475237602,28.2316040302269,12.));
#112651=CARTESIAN_POINT('Ctrl Pts',(68.9436475237602,28.2316040302269,8.));
#112652=CARTESIAN_POINT('Ctrl Pts',(68.9436475237602,28.2316040302268,4.));
#112653=CARTESIAN_POINT('Ctrl Pts',(68.9436475237602,28.2316040302268,-5.55111512312578E-16));
#112654=CARTESIAN_POINT('Ctrl Pts',(65.4815644032299,24.7419628022042,0.));
#112655=CARTESIAN_POINT('Ctrl Pts',(65.4815644032299,24.7419628022042,12.));
#112656=CARTESIAN_POINT('Ctrl Pts',(65.4847237095443,24.7442214063382,0.));
#112657=CARTESIAN_POINT('Ctrl Pts',(65.4847237095443,24.7442214063382,12.));
#112658=CARTESIAN_POINT('Ctrl Pts',(65.4910454936254,24.7487434955982,0.));
#112659=CARTESIAN_POINT('Ctrl Pts',(65.4910454936254,24.7487434955982,12.));
#112660=CARTESIAN_POINT('Ctrl Pts',(65.5005376841101,24.7555412724651,0.));
#112661=CARTESIAN_POINT('Ctrl Pts',(65.5005376841101,24.7555412724651,12.));
#112662=CARTESIAN_POINT('Ctrl Pts',(65.5132129675333,24.7646342620841,0.));
#112663=CARTESIAN_POINT('Ctrl Pts',(65.5132129675333,24.7646342620841,12.));
#112664=CARTESIAN_POINT('Ctrl Pts',(65.5290887770232,24.7760493148465,0.));
#112665=CARTESIAN_POINT('Ctrl Pts',(65.5290887770232,24.7760493148465,12.));
#112666=CARTESIAN_POINT('Ctrl Pts',(65.5449962514661,24.7875131827491,0.));
#112667=CARTESIAN_POINT('Ctrl Pts',(65.5449962514661,24.7875131827491,12.));
#112668=CARTESIAN_POINT('Ctrl Pts',(65.5609353062829,24.799025856126,0.));
#112669=CARTESIAN_POINT('Ctrl Pts',(65.5609353062829,24.799025856126,12.));
#112670=CARTESIAN_POINT('Ctrl Pts',(65.5769057914333,24.8105873098626,0.));
#112671=CARTESIAN_POINT('Ctrl Pts',(65.5769057914333,24.8105873098626,12.));
#112672=CARTESIAN_POINT('Ctrl Pts',(65.5929074932624,24.8221975032104,0.));
#112673=CARTESIAN_POINT('Ctrl Pts',(65.5929074932624,24.8221975032104,12.));
#112674=CARTESIAN_POINT('Ctrl Pts',(65.6089401625628,24.8338563866764,0.));
#112675=CARTESIAN_POINT('Ctrl Pts',(65.6089401625628,24.8338563866764,12.));
#112676=CARTESIAN_POINT('Ctrl Pts',(65.6250035361612,24.8455639071517,0.));
#112677=CARTESIAN_POINT('Ctrl Pts',(65.6250035361612,24.8455639071517,12.));
#112678=CARTESIAN_POINT('Ctrl Pts',(65.6410973603661,24.8573200135666,0.));
#112679=CARTESIAN_POINT('Ctrl Pts',(65.6410973603661,24.8573200135666,12.));
#112680=CARTESIAN_POINT('Ctrl Pts',(65.6572214156692,24.8691246628057,0.));
#112681=CARTESIAN_POINT('Ctrl Pts',(65.6572214156692,24.8691246628057,12.));
#112682=CARTESIAN_POINT('Ctrl Pts',(65.6733755087669,24.8809778178229,0.));
#112683=CARTESIAN_POINT('Ctrl Pts',(65.6733755087669,24.8809778178229,12.));
#112684=CARTESIAN_POINT('Ctrl Pts',(65.6895594608775,24.8928794448607,0.));
#112685=CARTESIAN_POINT('Ctrl Pts',(65.6895594608775,24.8928794448607,12.));
#112686=CARTESIAN_POINT('Ctrl Pts',(65.7057730980483,24.9048295111448,0.));
#112687=CARTESIAN_POINT('Ctrl Pts',(65.7057730980483,24.9048295111448,12.));
#112688=CARTESIAN_POINT('Ctrl Pts',(65.7220162391053,24.9168279820106,0.));
#112689=CARTESIAN_POINT('Ctrl Pts',(65.7220162391053,24.9168279820106,12.));
#112690=CARTESIAN_POINT('Ctrl Pts',(65.7382886895888,24.928874819458,0.));
#112691=CARTESIAN_POINT('Ctrl Pts',(65.7382886895888,24.928874819458,12.));
#112692=CARTESIAN_POINT('Ctrl Pts',(65.7545902480323,24.9409699836537,0.));
#112693=CARTESIAN_POINT('Ctrl Pts',(65.7545902480323,24.9409699836537,12.));
#112694=CARTESIAN_POINT('Ctrl Pts',(65.7709207098959,24.9531134338696,0.));
#112695=CARTESIAN_POINT('Ctrl Pts',(65.7709207098959,24.9531134338696,12.));
#112696=CARTESIAN_POINT('Ctrl Pts',(65.7872798720823,24.9653051295581,0.));
#112697=CARTESIAN_POINT('Ctrl Pts',(65.7872798720823,24.9653051295581,12.));
#112698=CARTESIAN_POINT('Ctrl Pts',(65.8036675380718,24.9775450315683,0.));
#112699=CARTESIAN_POINT('Ctrl Pts',(65.8036675380718,24.9775450315683,12.));
#112700=CARTESIAN_POINT('Ctrl Pts',(65.8200835177024,24.9898331020983,0.));
#112701=CARTESIAN_POINT('Ctrl Pts',(65.8200835177024,24.9898331020983,12.));
#112702=CARTESIAN_POINT('Ctrl Pts',(65.8365276247128,25.002169304117,0.));
#112703=CARTESIAN_POINT('Ctrl Pts',(65.8365276247128,25.002169304117,12.));
#112704=CARTESIAN_POINT('Ctrl Pts',(65.8529996750445,25.0145536009604,0.));
#112705=CARTESIAN_POINT('Ctrl Pts',(65.8529996750445,25.0145536009604,12.));
#112706=CARTESIAN_POINT('Ctrl Pts',(65.8694994847616,25.0269859558363,0.));
#112707=CARTESIAN_POINT('Ctrl Pts',(65.8694994847616,25.0269859558363,12.));
#112708=CARTESIAN_POINT('Ctrl Pts',(65.8860268683128,25.0394663314055,0.));
#112709=CARTESIAN_POINT('Ctrl Pts',(65.8860268683128,25.0394663314055,12.));
#112710=CARTESIAN_POINT('Ctrl Pts',(65.9025816394424,25.0519946900078,0.));
#112711=CARTESIAN_POINT('Ctrl Pts',(65.9025816394424,25.0519946900078,12.));
#112712=CARTESIAN_POINT('Ctrl Pts',(65.919163611981,25.0645709938524,0.));
#112713=CARTESIAN_POINT('Ctrl Pts',(65.919163611981,25.0645709938524,12.));
#112714=CARTESIAN_POINT('Ctrl Pts',(65.9357726006163,25.0771952052028,0.));
#112715=CARTESIAN_POINT('Ctrl Pts',(65.9357726006163,25.0771952052028,12.));
#112716=CARTESIAN_POINT('Ctrl Pts',(65.9524084218139,25.0898672865915,0.));
#112717=CARTESIAN_POINT('Ctrl Pts',(65.9524084218139,25.0898672865915,12.));
#112718=CARTESIAN_POINT('Ctrl Pts',(65.9690708941558,25.1025872009004,0.));
#112719=CARTESIAN_POINT('Ctrl Pts',(65.9690708941558,25.1025872009004,12.));
#112720=CARTESIAN_POINT('Ctrl Pts',(65.9857598378433,25.1153549112503,0.));
#112721=CARTESIAN_POINT('Ctrl Pts',(65.9857598378433,25.1153549112503,12.));
#112722=CARTESIAN_POINT('Ctrl Pts',(66.0024750743897,25.1281703809297,0.));
#112723=CARTESIAN_POINT('Ctrl Pts',(66.0024750743897,25.1281703809297,12.));
#112724=CARTESIAN_POINT('Ctrl Pts',(66.0192164262621,25.1410335733099,0.));
#112725=CARTESIAN_POINT('Ctrl Pts',(66.0192164262621,25.1410335733099,12.));
#112726=CARTESIAN_POINT('Ctrl Pts',(66.0359837164734,25.1539444517419,0.));
#112727=CARTESIAN_POINT('Ctrl Pts',(66.0359837164734,25.1539444517419,12.));
#112728=CARTESIAN_POINT('Ctrl Pts',(66.0527767686025,25.1669029795661,0.));
#112729=CARTESIAN_POINT('Ctrl Pts',(66.0527767686025,25.1669029795661,12.));
#112730=CARTESIAN_POINT('Ctrl Pts',(66.0695954069713,25.1799091201599,0.));
#112731=CARTESIAN_POINT('Ctrl Pts',(66.0695954069713,25.1799091201599,12.));
#112732=CARTESIAN_POINT('Ctrl Pts',(66.086439456768,25.1929628369685,0.));
#112733=CARTESIAN_POINT('Ctrl Pts',(66.086439456768,25.1929628369685,12.));
#112734=CARTESIAN_POINT('Ctrl Pts',(66.10330874419,25.2060640935365,0.));
#112735=CARTESIAN_POINT('Ctrl Pts',(66.10330874419,25.2060640935365,12.));
#112736=CARTESIAN_POINT('Ctrl Pts',(66.1202030965758,25.2192128535357,0.));
#112737=CARTESIAN_POINT('Ctrl Pts',(66.1202030965758,25.2192128535357,12.));
#112738=CARTESIAN_POINT('Ctrl Pts',(66.1371223423345,25.232409080755,0.));
#112739=CARTESIAN_POINT('Ctrl Pts',(66.1371223423345,25.232409080755,12.));
#112740=CARTESIAN_POINT('Ctrl Pts',(66.1540663108754,25.2456527390875,0.));
#112741=CARTESIAN_POINT('Ctrl Pts',(66.1540663108754,25.2456527390875,12.));
#112742=CARTESIAN_POINT('Ctrl Pts',(66.1710348325384,25.2589437925147,0.));
#112743=CARTESIAN_POINT('Ctrl Pts',(66.1710348325384,25.2589437925147,12.));
#112744=CARTESIAN_POINT('Ctrl Pts',(66.1880277385136,25.2722822050837,0.));
#112745=CARTESIAN_POINT('Ctrl Pts',(66.1880277385136,25.2722822050837,12.));
#112746=CARTESIAN_POINT('Ctrl Pts',(66.2050448607911,25.285667940893,0.));
#112747=CARTESIAN_POINT('Ctrl Pts',(66.2050448607911,25.285667940893,12.));
#112748=CARTESIAN_POINT('Ctrl Pts',(66.2220860321952,25.2991009641094,0.));
#112749=CARTESIAN_POINT('Ctrl Pts',(66.2220860321952,25.2991009641094,12.));
#112750=CARTESIAN_POINT('Ctrl Pts',(66.2391510863998,25.312581238973,0.));
#112751=CARTESIAN_POINT('Ctrl Pts',(66.2391510863998,25.312581238973,12.));
#112752=CARTESIAN_POINT('Ctrl Pts',(66.2562398579471,25.3261087298026,0.));
#112753=CARTESIAN_POINT('Ctrl Pts',(66.2562398579471,25.3261087298026,12.));
#112754=CARTESIAN_POINT('Ctrl Pts',(66.2733521822662,25.3396834009949,0.));
#112755=CARTESIAN_POINT('Ctrl Pts',(66.2733521822662,25.3396834009949,12.));
#112756=CARTESIAN_POINT('Ctrl Pts',(66.290487895671,25.3533052170249,0.));
#112757=CARTESIAN_POINT('Ctrl Pts',(66.290487895671,25.3533052170249,12.));
#112758=CARTESIAN_POINT('Ctrl Pts',(66.3076468353412,25.3669741424488,0.));
#112759=CARTESIAN_POINT('Ctrl Pts',(66.3076468353412,25.3669741424488,12.));
#112760=CARTESIAN_POINT('Ctrl Pts',(66.3248288393046,25.3806901419012,0.));
#112761=CARTESIAN_POINT('Ctrl Pts',(66.3248288393046,25.3806901419012,12.));
#112762=CARTESIAN_POINT('Ctrl Pts',(66.3420337464178,25.3944531800901,0.));
#112763=CARTESIAN_POINT('Ctrl Pts',(66.3420337464178,25.3944531800901,12.));
#112764=CARTESIAN_POINT('Ctrl Pts',(66.359261396341,25.4082632217847,0.));
#112765=CARTESIAN_POINT('Ctrl Pts',(66.359261396341,25.4082632217847,12.));
#112766=CARTESIAN_POINT('Ctrl Pts',(66.3765116295364,25.4221202318199,0.));
#112767=CARTESIAN_POINT('Ctrl Pts',(66.3765116295364,25.4221202318199,12.));
#112768=CARTESIAN_POINT('Ctrl Pts',(66.3937842872685,25.4360241751018,0.));
#112769=CARTESIAN_POINT('Ctrl Pts',(66.3937842872685,25.4360241751018,12.));
#112770=CARTESIAN_POINT('Ctrl Pts',(66.4110792116,25.4499750166079,0.));
#112771=CARTESIAN_POINT('Ctrl Pts',(66.4110792116,25.4499750166079,12.));
#112772=CARTESIAN_POINT('Ctrl Pts',(66.4283962453899,25.4639727213849,0.));
#112773=CARTESIAN_POINT('Ctrl Pts',(66.4283962453899,25.4639727213849,12.));
#112774=CARTESIAN_POINT('Ctrl Pts',(66.4457352322871,25.4780172545417,0.));
#112775=CARTESIAN_POINT('Ctrl Pts',(66.4457352322871,25.4780172545417,12.));
#112776=CARTESIAN_POINT('Ctrl Pts',(66.4630960167252,25.4921085812548,0.));
#112777=CARTESIAN_POINT('Ctrl Pts',(66.4630960167252,25.4921085812548,12.));
#112778=CARTESIAN_POINT('Ctrl Pts',(66.4804784439148,25.5062466667702,0.));
#112779=CARTESIAN_POINT('Ctrl Pts',(66.4804784439148,25.5062466667702,12.));
#112780=CARTESIAN_POINT('Ctrl Pts',(66.4978823598354,25.5204314764033,0.));
#112781=CARTESIAN_POINT('Ctrl Pts',(66.4978823598354,25.5204314764033,12.));
#112782=CARTESIAN_POINT('Ctrl Pts',(66.5153076112231,25.534662975532,0.));
#112783=CARTESIAN_POINT('Ctrl Pts',(66.5153076112231,25.534662975532,12.));
#112784=CARTESIAN_POINT('Ctrl Pts',(66.5327540455624,25.5489411295912,0.));
#112785=CARTESIAN_POINT('Ctrl Pts',(66.5327540455624,25.5489411295912,12.));
#112786=CARTESIAN_POINT('Ctrl Pts',(66.5502215110829,25.5632659040792,0.));
#112787=CARTESIAN_POINT('Ctrl Pts',(66.5502215110829,25.5632659040792,12.));
#112788=CARTESIAN_POINT('Ctrl Pts',(66.5677098567542,25.5776372645601,0.));
#112789=CARTESIAN_POINT('Ctrl Pts',(66.5677098567542,25.5776372645601,12.));
#112790=CARTESIAN_POINT('Ctrl Pts',(66.5852189322813,25.5920551766629,0.));
#112791=CARTESIAN_POINT('Ctrl Pts',(66.5852189322813,25.5920551766629,12.));
#112792=CARTESIAN_POINT('Ctrl Pts',(66.6027485880963,25.6065196060756,0.));
#112793=CARTESIAN_POINT('Ctrl Pts',(66.6027485880963,25.6065196060756,12.));
#112794=CARTESIAN_POINT('Ctrl Pts',(66.6202986753506,25.6210305185403,0.));
#112795=CARTESIAN_POINT('Ctrl Pts',(66.6202986753506,25.6210305185403,12.));
#112796=CARTESIAN_POINT('Ctrl Pts',(66.6378690459129,25.6355878798614,0.));
#112797=CARTESIAN_POINT('Ctrl Pts',(66.6378690459129,25.6355878798614,12.));
#112798=CARTESIAN_POINT('Ctrl Pts',(66.6554595523624,25.6501916559055,0.));
#112799=CARTESIAN_POINT('Ctrl Pts',(66.6554595523624,25.6501916559055,12.));
#112800=CARTESIAN_POINT('Ctrl Pts',(66.6730700479837,25.6648418126013,0.));
#112801=CARTESIAN_POINT('Ctrl Pts',(66.6730700479837,25.6648418126013,12.));
#112802=CARTESIAN_POINT('Ctrl Pts',(66.6907003867572,25.6795383159319,0.));
#112803=CARTESIAN_POINT('Ctrl Pts',(66.6907003867572,25.6795383159319,12.));
#112804=CARTESIAN_POINT('Ctrl Pts',(66.7083504233529,25.6942811319322,0.));
#112805=CARTESIAN_POINT('Ctrl Pts',(66.7083504233529,25.6942811319322,12.));
#112806=CARTESIAN_POINT('Ctrl Pts',(66.7260200131266,25.7090702266963,0.));
#112807=CARTESIAN_POINT('Ctrl Pts',(66.7260200131266,25.7090702266963,12.));
#112808=CARTESIAN_POINT('Ctrl Pts',(66.7437090121153,25.7239055663772,0.));
#112809=CARTESIAN_POINT('Ctrl Pts',(66.7437090121153,25.7239055663772,12.));
#112810=CARTESIAN_POINT('Ctrl Pts',(66.7614172770316,25.7387871171866,0.));
#112811=CARTESIAN_POINT('Ctrl Pts',(66.7614172770316,25.7387871171866,12.));
#112812=CARTESIAN_POINT('Ctrl Pts',(66.7791446652545,25.7537148453864,0.));
#112813=CARTESIAN_POINT('Ctrl Pts',(66.7791446652545,25.7537148453864,12.));
#112814=CARTESIAN_POINT('Ctrl Pts',(66.7968910348245,25.7686887172878,0.));
#112815=CARTESIAN_POINT('Ctrl Pts',(66.7968910348245,25.7686887172878,12.));
#112816=CARTESIAN_POINT('Ctrl Pts',(66.8146562444433,25.7837086992595,0.));
#112817=CARTESIAN_POINT('Ctrl Pts',(66.8146562444433,25.7837086992595,12.));
#112818=CARTESIAN_POINT('Ctrl Pts',(66.8324401534668,25.7987747577269,0.));
#112819=CARTESIAN_POINT('Ctrl Pts',(66.8324401534668,25.7987747577269,12.));
#112820=CARTESIAN_POINT('Ctrl Pts',(66.8502426219001,25.8138868591709,0.));
#112821=CARTESIAN_POINT('Ctrl Pts',(66.8502426219001,25.8138868591709,12.));
#112822=CARTESIAN_POINT('Ctrl Pts',(66.8680635103876,25.8290449701193,0.));
#112823=CARTESIAN_POINT('Ctrl Pts',(66.8680635103876,25.8290449701193,12.));
#112824=CARTESIAN_POINT('Ctrl Pts',(66.8859026802088,25.844249057147,0.));
#112825=CARTESIAN_POINT('Ctrl Pts',(66.8859026802088,25.844249057147,12.));
#112826=CARTESIAN_POINT('Ctrl Pts',(66.9037599932761,25.8594990868833,0.));
#112827=CARTESIAN_POINT('Ctrl Pts',(66.9037599932761,25.8594990868833,12.));
#112828=CARTESIAN_POINT('Ctrl Pts',(66.92163531213,25.8747950260111,0.));
#112829=CARTESIAN_POINT('Ctrl Pts',(66.92163531213,25.8747950260111,12.));
#112830=CARTESIAN_POINT('Ctrl Pts',(66.939528499934,25.890136841266,0.));
#112831=CARTESIAN_POINT('Ctrl Pts',(66.939528499934,25.890136841266,12.));
#112832=CARTESIAN_POINT('Ctrl Pts',(66.9574394204663,25.9055244994277,0.));
#112833=CARTESIAN_POINT('Ctrl Pts',(66.9574394204663,25.9055244994277,12.));
#112834=CARTESIAN_POINT('Ctrl Pts',(66.975367938115,25.9209579673209,0.));
#112835=CARTESIAN_POINT('Ctrl Pts',(66.975367938115,25.9209579673209,12.));
#112836=CARTESIAN_POINT('Ctrl Pts',(66.9933139178778,25.9364372118222,0.));
#112837=CARTESIAN_POINT('Ctrl Pts',(66.9933139178778,25.9364372118222,12.));
#112838=CARTESIAN_POINT('Ctrl Pts',(67.0112772253556,25.9519621998598,0.));
#112839=CARTESIAN_POINT('Ctrl Pts',(67.0112772253556,25.9519621998598,12.));
#112840=CARTESIAN_POINT('Ctrl Pts',(67.0292577267489,25.9675328984121,0.));
#112841=CARTESIAN_POINT('Ctrl Pts',(67.0292577267489,25.9675328984121,12.));
#112842=CARTESIAN_POINT('Ctrl Pts',(67.0472552888485,25.9831492744984,0.));
#112843=CARTESIAN_POINT('Ctrl Pts',(67.0472552888485,25.9831492744984,12.));
#112844=CARTESIAN_POINT('Ctrl Pts',(67.0652697790325,25.9988112951814,0.));
#112845=CARTESIAN_POINT('Ctrl Pts',(67.0652697790325,25.9988112951814,12.));
#112846=CARTESIAN_POINT('Ctrl Pts',(67.0833010652634,26.014518927573,0.));
#112847=CARTESIAN_POINT('Ctrl Pts',(67.0833010652634,26.014518927573,12.));
#112848=CARTESIAN_POINT('Ctrl Pts',(67.101349016084,26.030272138834,0.));
#112849=CARTESIAN_POINT('Ctrl Pts',(67.101349016084,26.030272138834,12.));
#112850=CARTESIAN_POINT('Ctrl Pts',(67.1194135006124,26.0460708961725,0.));
#112851=CARTESIAN_POINT('Ctrl Pts',(67.1194135006124,26.0460708961725,12.));
#112852=CARTESIAN_POINT('Ctrl Pts',(67.1374943885354,26.061915166836,0.));
#112853=CARTESIAN_POINT('Ctrl Pts',(67.1374943885354,26.061915166836,12.));
#112854=CARTESIAN_POINT('Ctrl Pts',(67.1555915501049,26.0778049181128,0.));
#112855=CARTESIAN_POINT('Ctrl Pts',(67.1555915501049,26.0778049181128,12.));
#112856=CARTESIAN_POINT('Ctrl Pts',(67.173704856136,26.0937401173383,0.));
#112857=CARTESIAN_POINT('Ctrl Pts',(67.173704856136,26.0937401173383,12.));
#112858=CARTESIAN_POINT('Ctrl Pts',(67.1918341780018,26.1097207318949,0.));
#112859=CARTESIAN_POINT('Ctrl Pts',(67.1918341780018,26.1097207318949,12.));
#112860=CARTESIAN_POINT('Ctrl Pts',(67.2099793876297,26.1257467292102,0.));
#112861=CARTESIAN_POINT('Ctrl Pts',(67.2099793876297,26.1257467292102,12.));
#112862=CARTESIAN_POINT('Ctrl Pts',(67.2281403574938,26.1418180767489,0.));
#112863=CARTESIAN_POINT('Ctrl Pts',(67.2281403574938,26.1418180767489,12.));
#112864=CARTESIAN_POINT('Ctrl Pts',(67.2463169606115,26.1579347420138,0.));
#112865=CARTESIAN_POINT('Ctrl Pts',(67.2463169606115,26.1579347420138,12.));
#112866=CARTESIAN_POINT('Ctrl Pts',(67.2645090705421,26.1740966925529,0.));
#112867=CARTESIAN_POINT('Ctrl Pts',(67.2645090705421,26.1740966925529,12.));
#112868=CARTESIAN_POINT('Ctrl Pts',(67.282716561383,26.1903038959589,0.));
#112869=CARTESIAN_POINT('Ctrl Pts',(67.282716561383,26.1903038959589,12.));
#112870=CARTESIAN_POINT('Ctrl Pts',(67.3009393077651,26.2065563198683,0.));
#112871=CARTESIAN_POINT('Ctrl Pts',(67.3009393077651,26.2065563198683,12.));
#112872=CARTESIAN_POINT('Ctrl Pts',(67.3191771848463,26.2228539319526,0.));
#112873=CARTESIAN_POINT('Ctrl Pts',(67.3191771848463,26.2228539319526,12.));
#112874=CARTESIAN_POINT('Ctrl Pts',(67.3374300683073,26.2391966999191,0.));
#112875=CARTESIAN_POINT('Ctrl Pts',(67.3374300683073,26.2391966999191,12.));
#112876=CARTESIAN_POINT('Ctrl Pts',(67.3556978343507,26.255584591518,0.));
#112877=CARTESIAN_POINT('Ctrl Pts',(67.3556978343507,26.255584591518,12.));
#112878=CARTESIAN_POINT('Ctrl Pts',(67.3739803596969,26.2720175745423,0.));
#112879=CARTESIAN_POINT('Ctrl Pts',(67.3739803596969,26.2720175745423,12.));
#112880=CARTESIAN_POINT('Ctrl Pts',(67.392277521581,26.288495616827,0.));
#112881=CARTESIAN_POINT('Ctrl Pts',(67.392277521581,26.288495616827,12.));
#112882=CARTESIAN_POINT('Ctrl Pts',(67.4105891977461,26.3050186862407,0.));
#112883=CARTESIAN_POINT('Ctrl Pts',(67.4105891977461,26.3050186862407,12.));
#112884=CARTESIAN_POINT('Ctrl Pts',(67.4289152664398,26.321586750686,0.));
#112885=CARTESIAN_POINT('Ctrl Pts',(67.4289152664398,26.321586750686,12.));
#112886=CARTESIAN_POINT('Ctrl Pts',(67.4472556064119,26.3381997781055,0.));
#112887=CARTESIAN_POINT('Ctrl Pts',(67.4472556064119,26.3381997781055,12.));
#112888=CARTESIAN_POINT('Ctrl Pts',(67.4656100969116,26.3548577364833,0.));
#112889=CARTESIAN_POINT('Ctrl Pts',(67.4656100969116,26.3548577364833,12.));
#112890=CARTESIAN_POINT('Ctrl Pts',(67.4839786176836,26.3715605938433,0.));
#112891=CARTESIAN_POINT('Ctrl Pts',(67.4839786176836,26.3715605938433,12.));
#112892=CARTESIAN_POINT('Ctrl Pts',(67.5023610489622,26.3883083182421,0.));
#112893=CARTESIAN_POINT('Ctrl Pts',(67.5023610489622,26.3883083182421,12.));
#112894=CARTESIAN_POINT('Ctrl Pts',(67.5207572714683,26.4051008777675,0.));
#112895=CARTESIAN_POINT('Ctrl Pts',(67.5207572714683,26.4051008777675,12.));
#112896=CARTESIAN_POINT('Ctrl Pts',(67.5391671664072,26.4219382405458,0.));
#112897=CARTESIAN_POINT('Ctrl Pts',(67.5391671664072,26.4219382405458,12.));
#112898=CARTESIAN_POINT('Ctrl Pts',(67.5575906154657,26.4388203747425,0.));
#112899=CARTESIAN_POINT('Ctrl Pts',(67.5575906154657,26.4388203747425,12.));
#112900=CARTESIAN_POINT('Ctrl Pts',(67.5760275008093,26.4557472485621,0.));
#112901=CARTESIAN_POINT('Ctrl Pts',(67.5760275008093,26.4557472485621,12.));
#112902=CARTESIAN_POINT('Ctrl Pts',(67.5944777050768,26.4727188302409,0.));
#112903=CARTESIAN_POINT('Ctrl Pts',(67.5944777050768,26.4727188302409,12.));
#112904=CARTESIAN_POINT('Ctrl Pts',(67.6129411113757,26.489735088044,0.));
#112905=CARTESIAN_POINT('Ctrl Pts',(67.6129411113757,26.489735088044,12.));
#112906=CARTESIAN_POINT('Ctrl Pts',(67.6314176032811,26.5067959902725,0.));
#112907=CARTESIAN_POINT('Ctrl Pts',(67.6314176032811,26.5067959902725,12.));
#112908=CARTESIAN_POINT('Ctrl Pts',(67.649907064832,26.5239015052654,0.));
#112909=CARTESIAN_POINT('Ctrl Pts',(67.649907064832,26.5239015052654,12.));
#112910=CARTESIAN_POINT('Ctrl Pts',(67.6684093805291,26.5410516013985,0.));
#112911=CARTESIAN_POINT('Ctrl Pts',(67.6684093805291,26.5410516013985,12.));
#112912=CARTESIAN_POINT('Ctrl Pts',(67.6869244353294,26.5582462470794,0.));
#112913=CARTESIAN_POINT('Ctrl Pts',(67.6869244353294,26.5582462470794,12.));
#112914=CARTESIAN_POINT('Ctrl Pts',(67.7054521146424,26.5754854107421,0.));
#112915=CARTESIAN_POINT('Ctrl Pts',(67.7054521146424,26.5754854107421,12.));
#112916=CARTESIAN_POINT('Ctrl Pts',(67.7239923043288,26.5927690608544,0.));
#112917=CARTESIAN_POINT('Ctrl Pts',(67.7239923043288,26.5927690608544,12.));
#112918=CARTESIAN_POINT('Ctrl Pts',(67.7425448906977,26.6100971659202,0.));
#112919=CARTESIAN_POINT('Ctrl Pts',(67.7425448906977,26.6100971659202,12.));
#112920=CARTESIAN_POINT('Ctrl Pts',(67.7611097605042,26.6274696944793,0.));
#112921=CARTESIAN_POINT('Ctrl Pts',(67.7611097605042,26.6274696944793,12.));
#112922=CARTESIAN_POINT('Ctrl Pts',(67.7796868009455,26.6448866151029,0.));
#112923=CARTESIAN_POINT('Ctrl Pts',(67.7796868009455,26.6448866151029,12.));
#112924=CARTESIAN_POINT('Ctrl Pts',(67.798275899657,26.6623478963871,0.));
#112925=CARTESIAN_POINT('Ctrl Pts',(67.798275899657,26.6623478963871,12.));
#112926=CARTESIAN_POINT('Ctrl Pts',(67.8168769447098,26.6798535069589,0.));
#112927=CARTESIAN_POINT('Ctrl Pts',(67.8168769447098,26.6798535069589,12.));
#112928=CARTESIAN_POINT('Ctrl Pts',(67.8354898246086,26.6974034154804,0.));
#112929=CARTESIAN_POINT('Ctrl Pts',(67.8354898246086,26.6974034154804,12.));
#112930=CARTESIAN_POINT('Ctrl Pts',(67.8541144282875,26.7149975906478,0.));
#112931=CARTESIAN_POINT('Ctrl Pts',(67.8541144282875,26.7149975906478,12.));
#112932=CARTESIAN_POINT('Ctrl Pts',(67.8727506451063,26.7326360011885,0.));
#112933=CARTESIAN_POINT('Ctrl Pts',(67.8727506451063,26.7326360011885,12.));
#112934=CARTESIAN_POINT('Ctrl Pts',(67.8913983648436,26.7503186158522,0.));
#112935=CARTESIAN_POINT('Ctrl Pts',(67.8913983648436,26.7503186158522,12.));
#112936=CARTESIAN_POINT('Ctrl Pts',(67.9100574776972,26.7680454034169,0.));
#112937=CARTESIAN_POINT('Ctrl Pts',(67.9100574776972,26.7680454034169,12.));
#112938=CARTESIAN_POINT('Ctrl Pts',(67.928727874284,26.7858163326934,0.));
#112939=CARTESIAN_POINT('Ctrl Pts',(67.928727874284,26.7858163326934,12.));
#112940=CARTESIAN_POINT('Ctrl Pts',(67.9474094456396,26.8036313725262,0.));
#112941=CARTESIAN_POINT('Ctrl Pts',(67.9474094456396,26.8036313725262,12.));
#112942=CARTESIAN_POINT('Ctrl Pts',(67.9661020832164,26.821490491792,0.));
#112943=CARTESIAN_POINT('Ctrl Pts',(67.9661020832164,26.821490491792,12.));
#112944=CARTESIAN_POINT('Ctrl Pts',(67.9848056788809,26.8393936593911,0.));
#112945=CARTESIAN_POINT('Ctrl Pts',(67.9848056788809,26.8393936593911,12.));
#112946=CARTESIAN_POINT('Ctrl Pts',(68.0035201249102,26.8573408442496,0.));
#112947=CARTESIAN_POINT('Ctrl Pts',(68.0035201249102,26.8573408442496,12.));
#112948=CARTESIAN_POINT('Ctrl Pts',(68.0222453139856,26.8753320153252,0.));
#112949=CARTESIAN_POINT('Ctrl Pts',(68.0222453139856,26.8753320153252,12.));
#112950=CARTESIAN_POINT('Ctrl Pts',(68.0409811391869,26.8933671416063,0.));
#112951=CARTESIAN_POINT('Ctrl Pts',(68.0409811391869,26.8933671416063,12.));
#112952=CARTESIAN_POINT('Ctrl Pts',(68.0597274939859,26.911446192111,0.));
#112953=CARTESIAN_POINT('Ctrl Pts',(68.0597274939859,26.911446192111,12.));
#112954=CARTESIAN_POINT('Ctrl Pts',(68.0784842722369,26.9295691358779,0.));
#112955=CARTESIAN_POINT('Ctrl Pts',(68.0784842722369,26.9295691358779,12.));
#112956=CARTESIAN_POINT('Ctrl Pts',(68.0972513681751,26.9477359419652,0.));
#112957=CARTESIAN_POINT('Ctrl Pts',(68.0972513681751,26.9477359419652,12.));
#112958=CARTESIAN_POINT('Ctrl Pts',(68.1160286764255,26.9659465794601,0.));
#112959=CARTESIAN_POINT('Ctrl Pts',(68.1160286764255,26.9659465794601,12.));
#112960=CARTESIAN_POINT('Ctrl Pts',(68.1348160920106,26.9842010174822,0.));
#112961=CARTESIAN_POINT('Ctrl Pts',(68.1348160920106,26.9842010174822,12.));
#112962=CARTESIAN_POINT('Ctrl Pts',(68.1536135103557,27.0024992251838,0.));
#112963=CARTESIAN_POINT('Ctrl Pts',(68.1536135103557,27.0024992251838,12.));
#112964=CARTESIAN_POINT('Ctrl Pts',(68.1724208272958,27.0208411717472,0.));
#112965=CARTESIAN_POINT('Ctrl Pts',(68.1724208272958,27.0208411717472,12.));
#112966=CARTESIAN_POINT('Ctrl Pts',(68.1912379390773,27.0392268263798,0.));
#112967=CARTESIAN_POINT('Ctrl Pts',(68.1912379390773,27.0392268263798,12.));
#112968=CARTESIAN_POINT('Ctrl Pts',(68.2100647423332,27.0576561583172,0.));
#112969=CARTESIAN_POINT('Ctrl Pts',(68.2100647423332,27.0576561583172,12.));
#112970=CARTESIAN_POINT('Ctrl Pts',(68.2289011340615,27.0761291368226,0.));
#112971=CARTESIAN_POINT('Ctrl Pts',(68.2289011340615,27.0761291368226,12.));
#112972=CARTESIAN_POINT('Ctrl Pts',(68.2477470116012,27.0946457311813,0.));
#112973=CARTESIAN_POINT('Ctrl Pts',(68.2477470116012,27.0946457311813,12.));
#112974=CARTESIAN_POINT('Ctrl Pts',(68.2666022726104,27.1132059106943,0.));
#112975=CARTESIAN_POINT('Ctrl Pts',(68.2666022726104,27.1132059106943,12.));
#112976=CARTESIAN_POINT('Ctrl Pts',(68.2854668150364,27.1318096446649,0.));
#112977=CARTESIAN_POINT('Ctrl Pts',(68.2854668150364,27.1318096446649,12.));
#112978=CARTESIAN_POINT('Ctrl Pts',(68.3043405371603,27.1504569024136,0.));
#112979=CARTESIAN_POINT('Ctrl Pts',(68.3043405371603,27.1504569024136,12.));
#112980=CARTESIAN_POINT('Ctrl Pts',(68.3232233376425,27.1691476532921,0.));
#112981=CARTESIAN_POINT('Ctrl Pts',(68.3232233376425,27.1691476532921,12.));
#112982=CARTESIAN_POINT('Ctrl Pts',(68.3421151155711,27.1878818666926,0.));
#112983=CARTESIAN_POINT('Ctrl Pts',(68.3421151155711,27.1878818666926,12.));
#112984=CARTESIAN_POINT('Ctrl Pts',(68.3610157704994,27.2066595120542,0.));
#112985=CARTESIAN_POINT('Ctrl Pts',(68.3610157704994,27.2066595120542,12.));
#112986=CARTESIAN_POINT('Ctrl Pts',(68.3799252025102,27.2254805588673,0.));
#112987=CARTESIAN_POINT('Ctrl Pts',(68.3799252025102,27.2254805588673,12.));
#112988=CARTESIAN_POINT('Ctrl Pts',(68.3988433121581,27.244344976665,0.));
#112989=CARTESIAN_POINT('Ctrl Pts',(68.3988433121581,27.244344976665,12.));
#112990=CARTESIAN_POINT('Ctrl Pts',(68.4177700003465,27.263252735006,0.));
#112991=CARTESIAN_POINT('Ctrl Pts',(68.4177700003465,27.263252735006,12.));
#112992=CARTESIAN_POINT('Ctrl Pts',(68.4367051682164,27.2822038034538,0.));
#112993=CARTESIAN_POINT('Ctrl Pts',(68.4367051682164,27.2822038034538,12.));
#112994=CARTESIAN_POINT('Ctrl Pts',(68.4556487170441,27.301198151557,0.));
#112995=CARTESIAN_POINT('Ctrl Pts',(68.4556487170441,27.301198151557,12.));
#112996=CARTESIAN_POINT('Ctrl Pts',(68.4746005480997,27.3202357488154,0.));
#112997=CARTESIAN_POINT('Ctrl Pts',(68.4746005480997,27.3202357488154,12.));
#112998=CARTESIAN_POINT('Ctrl Pts',(68.4935605626372,27.3393165646752,0.));
#112999=CARTESIAN_POINT('Ctrl Pts',(68.4935605626372,27.3393165646752,12.));
#113000=CARTESIAN_POINT('Ctrl Pts',(68.5125286621902,27.3584405685947,0.));
#113001=CARTESIAN_POINT('Ctrl Pts',(68.5125286621902,27.3584405685947,12.));
#113002=CARTESIAN_POINT('Ctrl Pts',(68.5315047488046,27.3776077300918,0.));
#113003=CARTESIAN_POINT('Ctrl Pts',(68.5315047488046,27.3776077300918,12.));
#113004=CARTESIAN_POINT('Ctrl Pts',(68.5504887252976,27.3968180187941,0.));
#113005=CARTESIAN_POINT('Ctrl Pts',(68.5504887252976,27.3968180187941,12.));
#113006=CARTESIAN_POINT('Ctrl Pts',(68.5694804955002,27.4160714044825,0.));
#113007=CARTESIAN_POINT('Ctrl Pts',(68.5694804955002,27.4160714044825,12.));
#113008=CARTESIAN_POINT('Ctrl Pts',(68.5884799645193,27.4353678571349,0.));
#113009=CARTESIAN_POINT('Ctrl Pts',(68.5884799645193,27.4353678571349,12.));
#113010=CARTESIAN_POINT('Ctrl Pts',(68.6074870381588,27.4547073468213,0.));
#113011=CARTESIAN_POINT('Ctrl Pts',(68.6074870381588,27.4547073468213,12.));
#113012=CARTESIAN_POINT('Ctrl Pts',(68.6265016223536,27.4740898435977,0.));
#113013=CARTESIAN_POINT('Ctrl Pts',(68.6265016223536,27.4740898435977,12.));
#113014=CARTESIAN_POINT('Ctrl Pts',(68.6455236225471,27.4935153173863,0.));
#113015=CARTESIAN_POINT('Ctrl Pts',(68.6455236225471,27.4935153173863,12.));
#113016=CARTESIAN_POINT('Ctrl Pts',(68.6645529432059,27.5129837378798,0.));
#113017=CARTESIAN_POINT('Ctrl Pts',(68.6645529432059,27.5129837378798,12.));
#113018=CARTESIAN_POINT('Ctrl Pts',(68.683589486992,27.5324950743723,0.));
#113019=CARTESIAN_POINT('Ctrl Pts',(68.683589486992,27.5324950743723,12.));
#113020=CARTESIAN_POINT('Ctrl Pts',(68.7026331554348,27.552049295893,0.));
#113021=CARTESIAN_POINT('Ctrl Pts',(68.7026331554348,27.552049295893,12.));
#113022=CARTESIAN_POINT('Ctrl Pts',(68.721683850427,27.5716463715027,0.));
#113023=CARTESIAN_POINT('Ctrl Pts',(68.721683850427,27.5716463715027,12.));
#113024=CARTESIAN_POINT('Ctrl Pts',(68.7407414755291,27.5912862705482,0.));
#113025=CARTESIAN_POINT('Ctrl Pts',(68.7407414755291,27.5912862705482,12.));
#113026=CARTESIAN_POINT('Ctrl Pts',(68.7598059372121,27.6109689629025,0.));
#113027=CARTESIAN_POINT('Ctrl Pts',(68.7598059372121,27.6109689629025,12.));
#113028=CARTESIAN_POINT('Ctrl Pts',(68.7788771464655,27.6306944192711,0.));
#113029=CARTESIAN_POINT('Ctrl Pts',(68.7788771464655,27.6306944192711,12.));
#113030=CARTESIAN_POINT('Ctrl Pts',(68.7979550191773,27.6504626112621,0.));
#113031=CARTESIAN_POINT('Ctrl Pts',(68.7979550191773,27.6504626112621,12.));
#113032=CARTESIAN_POINT('Ctrl Pts',(68.8170394725786,27.670273510707,0.));
#113033=CARTESIAN_POINT('Ctrl Pts',(68.8170394725786,27.670273510707,12.));
#113034=CARTESIAN_POINT('Ctrl Pts',(68.8361304224378,27.6901270891201,0.));
#113035=CARTESIAN_POINT('Ctrl Pts',(68.8361304224378,27.6901270891201,12.));
#113036=CARTESIAN_POINT('Ctrl Pts',(68.855227779818,27.7100233170728,0.));
#113037=CARTESIAN_POINT('Ctrl Pts',(68.855227779818,27.7100233170728,12.));
#113038=CARTESIAN_POINT('Ctrl Pts',(68.8743314483451,27.7299621636602,0.));
#113039=CARTESIAN_POINT('Ctrl Pts',(68.8743314483451,27.7299621636602,12.));
#113040=CARTESIAN_POINT('Ctrl Pts',(68.8934413203945,27.7499435957608,0.));
#113041=CARTESIAN_POINT('Ctrl Pts',(68.8934413203945,27.7499435957608,12.));
#113042=CARTESIAN_POINT('Ctrl Pts',(68.9125572825946,27.7699675790683,0.));
#113043=CARTESIAN_POINT('Ctrl Pts',(68.9125572825946,27.7699675790683,12.));
#113044=CARTESIAN_POINT('Ctrl Pts',(68.9316792226187,27.7900340793796,0.));
#113045=CARTESIAN_POINT('Ctrl Pts',(68.9316792226187,27.7900340793796,12.));
#113046=CARTESIAN_POINT('Ctrl Pts',(68.9508070357786,27.8101430638128,0.));
#113047=CARTESIAN_POINT('Ctrl Pts',(68.9508070357786,27.8101430638128,12.));
#113048=CARTESIAN_POINT('Ctrl Pts',(68.9699406311305,27.8302945019939,0.));
#113049=CARTESIAN_POINT('Ctrl Pts',(68.9699406311305,27.8302945019939,12.));
#113050=CARTESIAN_POINT('Ctrl Pts',(68.9890799391863,27.8504883673903,0.));
#113051=CARTESIAN_POINT('Ctrl Pts',(68.9890799391863,27.8504883673903,12.));
#113052=CARTESIAN_POINT('Ctrl Pts',(69.0082249138015,27.8707246380697,0.));
#113053=CARTESIAN_POINT('Ctrl Pts',(69.0082249138015,27.8707246380697,12.));
#113054=CARTESIAN_POINT('Ctrl Pts',(69.0273755264702,27.8910032967037,0.));
#113055=CARTESIAN_POINT('Ctrl Pts',(69.0273755264702,27.8910032967037,12.));
#113056=CARTESIAN_POINT('Ctrl Pts',(69.0427005153223,27.9072601239469,0.));
#113057=CARTESIAN_POINT('Ctrl Pts',(69.0427005153223,27.9072601239469,12.));
#113058=CARTESIAN_POINT('Ctrl Pts',(69.0541967850685,27.9194718098851,0.));
#113059=CARTESIAN_POINT('Ctrl Pts',(69.0541967850685,27.9194718098851,12.));
#113060=CARTESIAN_POINT('Ctrl Pts',(69.0618620884596,27.9276214070576,0.));
#113061=CARTESIAN_POINT('Ctrl Pts',(69.0618620884596,27.9276214070576,12.));
#113062=CARTESIAN_POINT('Ctrl Pts',(69.065695021045,27.9316983239472,0.));
#113063=CARTESIAN_POINT('Ctrl Pts',(69.065695021045,27.9316983239472,12.));
#113064=CARTESIAN_POINT('',(65.4815644032299,24.7419628022042,0.));
#113065=CARTESIAN_POINT('Ctrl Pts',(65.4815644032299,24.7419628022042,0.));
#113066=CARTESIAN_POINT('Ctrl Pts',(65.4847237095443,24.7442214063382,0.));
#113067=CARTESIAN_POINT('Ctrl Pts',(65.4910454936254,24.7487434955982,0.));
#113068=CARTESIAN_POINT('Ctrl Pts',(65.5005376841101,24.7555412724651,0.));
#113069=CARTESIAN_POINT('Ctrl Pts',(65.5132129675333,24.7646342620841,0.));
#113070=CARTESIAN_POINT('Ctrl Pts',(65.5290887770232,24.7760493148465,0.));
#113071=CARTESIAN_POINT('Ctrl Pts',(65.5449962514661,24.7875131827491,0.));
#113072=CARTESIAN_POINT('Ctrl Pts',(65.5609353062829,24.799025856126,0.));
#113073=CARTESIAN_POINT('Ctrl Pts',(65.5769057914333,24.8105873098626,0.));
#113074=CARTESIAN_POINT('Ctrl Pts',(65.5929074932624,24.8221975032104,0.));
#113075=CARTESIAN_POINT('Ctrl Pts',(65.6089401625628,24.8338563866764,0.));
#113076=CARTESIAN_POINT('Ctrl Pts',(65.6250035361612,24.8455639071517,0.));
#113077=CARTESIAN_POINT('Ctrl Pts',(65.6410973603661,24.8573200135666,0.));
#113078=CARTESIAN_POINT('Ctrl Pts',(65.6572214156692,24.8691246628057,0.));
#113079=CARTESIAN_POINT('Ctrl Pts',(65.6733755087669,24.8809778178229,0.));
#113080=CARTESIAN_POINT('Ctrl Pts',(65.6895594608775,24.8928794448607,0.));
#113081=CARTESIAN_POINT('Ctrl Pts',(65.7057730980483,24.9048295111448,0.));
#113082=CARTESIAN_POINT('Ctrl Pts',(65.7220162391053,24.9168279820106,0.));
#113083=CARTESIAN_POINT('Ctrl Pts',(65.7382886895888,24.928874819458,0.));
#113084=CARTESIAN_POINT('Ctrl Pts',(65.7545902480323,24.9409699836537,0.));
#113085=CARTESIAN_POINT('Ctrl Pts',(65.7709207098959,24.9531134338696,0.));
#113086=CARTESIAN_POINT('Ctrl Pts',(65.7872798720823,24.9653051295581,0.));
#113087=CARTESIAN_POINT('Ctrl Pts',(65.8036675380718,24.9775450315683,0.));
#113088=CARTESIAN_POINT('Ctrl Pts',(65.8200835177024,24.9898331020983,0.));
#113089=CARTESIAN_POINT('Ctrl Pts',(65.8365276247128,25.002169304117,0.));
#113090=CARTESIAN_POINT('Ctrl Pts',(65.8529996750445,25.0145536009604,0.));
#113091=CARTESIAN_POINT('Ctrl Pts',(65.8694994847616,25.0269859558363,0.));
#113092=CARTESIAN_POINT('Ctrl Pts',(65.8860268683128,25.0394663314055,0.));
#113093=CARTESIAN_POINT('Ctrl Pts',(65.9025816394424,25.0519946900078,0.));
#113094=CARTESIAN_POINT('Ctrl Pts',(65.919163611981,25.0645709938524,0.));
#113095=CARTESIAN_POINT('Ctrl Pts',(65.9357726006163,25.0771952052028,0.));
#113096=CARTESIAN_POINT('Ctrl Pts',(65.9524084218139,25.0898672865915,0.));
#113097=CARTESIAN_POINT('Ctrl Pts',(65.9690708941558,25.1025872009004,0.));
#113098=CARTESIAN_POINT('Ctrl Pts',(65.9857598378433,25.1153549112503,0.));
#113099=CARTESIAN_POINT('Ctrl Pts',(66.0024750743897,25.1281703809297,0.));
#113100=CARTESIAN_POINT('Ctrl Pts',(66.0192164262621,25.1410335733099,0.));
#113101=CARTESIAN_POINT('Ctrl Pts',(66.0359837164734,25.1539444517419,0.));
#113102=CARTESIAN_POINT('Ctrl Pts',(66.0527767686025,25.1669029795661,0.));
#113103=CARTESIAN_POINT('Ctrl Pts',(66.0695954069713,25.1799091201599,0.));
#113104=CARTESIAN_POINT('Ctrl Pts',(66.086439456768,25.1929628369685,0.));
#113105=CARTESIAN_POINT('Ctrl Pts',(66.10330874419,25.2060640935365,0.));
#113106=CARTESIAN_POINT('Ctrl Pts',(66.1202030965758,25.2192128535357,0.));
#113107=CARTESIAN_POINT('Ctrl Pts',(66.1371223423345,25.232409080755,0.));
#113108=CARTESIAN_POINT('Ctrl Pts',(66.1540663108754,25.2456527390875,0.));
#113109=CARTESIAN_POINT('Ctrl Pts',(66.1710348325384,25.2589437925147,0.));
#113110=CARTESIAN_POINT('Ctrl Pts',(66.1880277385136,25.2722822050837,0.));
#113111=CARTESIAN_POINT('Ctrl Pts',(66.2050448607911,25.285667940893,0.));
#113112=CARTESIAN_POINT('Ctrl Pts',(66.2220860321952,25.2991009641094,0.));
#113113=CARTESIAN_POINT('Ctrl Pts',(66.2391510863998,25.312581238973,0.));
#113114=CARTESIAN_POINT('Ctrl Pts',(66.2562398579471,25.3261087298026,0.));
#113115=CARTESIAN_POINT('Ctrl Pts',(66.2733521822662,25.3396834009949,0.));
#113116=CARTESIAN_POINT('Ctrl Pts',(66.290487895671,25.3533052170249,0.));
#113117=CARTESIAN_POINT('Ctrl Pts',(66.3076468353412,25.3669741424488,0.));
#113118=CARTESIAN_POINT('Ctrl Pts',(66.3248288393046,25.3806901419012,0.));
#113119=CARTESIAN_POINT('Ctrl Pts',(66.3420337464178,25.3944531800901,0.));
#113120=CARTESIAN_POINT('Ctrl Pts',(66.359261396341,25.4082632217847,0.));
#113121=CARTESIAN_POINT('Ctrl Pts',(66.3765116295364,25.4221202318199,0.));
#113122=CARTESIAN_POINT('Ctrl Pts',(66.3937842872685,25.4360241751018,0.));
#113123=CARTESIAN_POINT('Ctrl Pts',(66.4110792116,25.4499750166079,0.));
#113124=CARTESIAN_POINT('Ctrl Pts',(66.4283962453899,25.4639727213849,0.));
#113125=CARTESIAN_POINT('Ctrl Pts',(66.4457352322871,25.4780172545417,0.));
#113126=CARTESIAN_POINT('Ctrl Pts',(66.4630960167252,25.4921085812548,0.));
#113127=CARTESIAN_POINT('Ctrl Pts',(66.4804784439148,25.5062466667702,0.));
#113128=CARTESIAN_POINT('Ctrl Pts',(66.4978823598354,25.5204314764033,0.));
#113129=CARTESIAN_POINT('Ctrl Pts',(66.5153076112231,25.534662975532,0.));
#113130=CARTESIAN_POINT('Ctrl Pts',(66.5327540455624,25.5489411295912,0.));
#113131=CARTESIAN_POINT('Ctrl Pts',(66.5502215110829,25.5632659040792,0.));
#113132=CARTESIAN_POINT('Ctrl Pts',(66.5677098567542,25.5776372645601,0.));
#113133=CARTESIAN_POINT('Ctrl Pts',(66.5852189322813,25.5920551766629,0.));
#113134=CARTESIAN_POINT('Ctrl Pts',(66.6027485880963,25.6065196060756,0.));
#113135=CARTESIAN_POINT('Ctrl Pts',(66.6202986753506,25.6210305185403,0.));
#113136=CARTESIAN_POINT('Ctrl Pts',(66.6378690459129,25.6355878798614,0.));
#113137=CARTESIAN_POINT('Ctrl Pts',(66.6554595523624,25.6501916559055,0.));
#113138=CARTESIAN_POINT('Ctrl Pts',(66.6730700479837,25.6648418126013,0.));
#113139=CARTESIAN_POINT('Ctrl Pts',(66.6907003867572,25.6795383159319,0.));
#113140=CARTESIAN_POINT('Ctrl Pts',(66.7083504233529,25.6942811319322,0.));
#113141=CARTESIAN_POINT('Ctrl Pts',(66.7260200131266,25.7090702266963,0.));
#113142=CARTESIAN_POINT('Ctrl Pts',(66.7437090121153,25.7239055663772,0.));
#113143=CARTESIAN_POINT('Ctrl Pts',(66.7614172770316,25.7387871171866,0.));
#113144=CARTESIAN_POINT('Ctrl Pts',(66.7791446652545,25.7537148453864,0.));
#113145=CARTESIAN_POINT('Ctrl Pts',(66.7968910348245,25.7686887172878,0.));
#113146=CARTESIAN_POINT('Ctrl Pts',(66.8146562444433,25.7837086992595,0.));
#113147=CARTESIAN_POINT('Ctrl Pts',(66.8324401534668,25.7987747577269,0.));
#113148=CARTESIAN_POINT('Ctrl Pts',(66.8502426219001,25.8138868591709,0.));
#113149=CARTESIAN_POINT('Ctrl Pts',(66.8680635103876,25.8290449701193,0.));
#113150=CARTESIAN_POINT('Ctrl Pts',(66.8859026802088,25.844249057147,0.));
#113151=CARTESIAN_POINT('Ctrl Pts',(66.9037599932761,25.8594990868833,0.));
#113152=CARTESIAN_POINT('Ctrl Pts',(66.92163531213,25.8747950260111,0.));
#113153=CARTESIAN_POINT('Ctrl Pts',(66.939528499934,25.890136841266,0.));
#113154=CARTESIAN_POINT('Ctrl Pts',(66.9574394204663,25.9055244994277,0.));
#113155=CARTESIAN_POINT('Ctrl Pts',(66.975367938115,25.9209579673209,0.));
#113156=CARTESIAN_POINT('Ctrl Pts',(66.9933139178778,25.9364372118222,0.));
#113157=CARTESIAN_POINT('Ctrl Pts',(67.0112772253556,25.9519621998598,0.));
#113158=CARTESIAN_POINT('Ctrl Pts',(67.0292577267489,25.9675328984121,0.));
#113159=CARTESIAN_POINT('Ctrl Pts',(67.0472552888485,25.9831492744984,0.));
#113160=CARTESIAN_POINT('Ctrl Pts',(67.0652697790325,25.9988112951814,0.));
#113161=CARTESIAN_POINT('Ctrl Pts',(67.0833010652634,26.014518927573,0.));
#113162=CARTESIAN_POINT('Ctrl Pts',(67.101349016084,26.030272138834,0.));
#113163=CARTESIAN_POINT('Ctrl Pts',(67.1194135006124,26.0460708961725,0.));
#113164=CARTESIAN_POINT('Ctrl Pts',(67.1374943885354,26.061915166836,0.));
#113165=CARTESIAN_POINT('Ctrl Pts',(67.1555915501049,26.0778049181128,0.));
#113166=CARTESIAN_POINT('Ctrl Pts',(67.173704856136,26.0937401173383,0.));
#113167=CARTESIAN_POINT('Ctrl Pts',(67.1918341780018,26.1097207318949,0.));
#113168=CARTESIAN_POINT('Ctrl Pts',(67.2099793876297,26.1257467292102,0.));
#113169=CARTESIAN_POINT('Ctrl Pts',(67.2281403574938,26.1418180767489,0.));
#113170=CARTESIAN_POINT('Ctrl Pts',(67.2463169606115,26.1579347420138,0.));
#113171=CARTESIAN_POINT('Ctrl Pts',(67.2645090705421,26.1740966925529,0.));
#113172=CARTESIAN_POINT('Ctrl Pts',(67.282716561383,26.1903038959589,0.));
#113173=CARTESIAN_POINT('Ctrl Pts',(67.3009393077651,26.2065563198683,0.));
#113174=CARTESIAN_POINT('Ctrl Pts',(67.3191771848463,26.2228539319526,0.));
#113175=CARTESIAN_POINT('Ctrl Pts',(67.3374300683073,26.2391966999191,0.));
#113176=CARTESIAN_POINT('Ctrl Pts',(67.3556978343507,26.255584591518,0.));
#113177=CARTESIAN_POINT('Ctrl Pts',(67.3739803596969,26.2720175745423,0.));
#113178=CARTESIAN_POINT('Ctrl Pts',(67.392277521581,26.288495616827,0.));
#113179=CARTESIAN_POINT('Ctrl Pts',(67.4105891977461,26.3050186862407,0.));
#113180=CARTESIAN_POINT('Ctrl Pts',(67.4289152664398,26.321586750686,0.));
#113181=CARTESIAN_POINT('Ctrl Pts',(67.4472556064119,26.3381997781055,0.));
#113182=CARTESIAN_POINT('Ctrl Pts',(67.4656100969116,26.3548577364833,0.));
#113183=CARTESIAN_POINT('Ctrl Pts',(67.4839786176836,26.3715605938433,0.));
#113184=CARTESIAN_POINT('Ctrl Pts',(67.5023610489622,26.3883083182421,0.));
#113185=CARTESIAN_POINT('Ctrl Pts',(67.5207572714683,26.4051008777675,0.));
#113186=CARTESIAN_POINT('Ctrl Pts',(67.5391671664072,26.4219382405458,0.));
#113187=CARTESIAN_POINT('Ctrl Pts',(67.5575906154657,26.4388203747425,0.));
#113188=CARTESIAN_POINT('Ctrl Pts',(67.5760275008093,26.4557472485621,0.));
#113189=CARTESIAN_POINT('Ctrl Pts',(67.5944777050768,26.4727188302409,0.));
#113190=CARTESIAN_POINT('Ctrl Pts',(67.6129411113757,26.489735088044,0.));
#113191=CARTESIAN_POINT('Ctrl Pts',(67.6314176032811,26.5067959902725,0.));
#113192=CARTESIAN_POINT('Ctrl Pts',(67.649907064832,26.5239015052654,0.));
#113193=CARTESIAN_POINT('Ctrl Pts',(67.6684093805291,26.5410516013985,0.));
#113194=CARTESIAN_POINT('Ctrl Pts',(67.6869244353294,26.5582462470794,0.));
#113195=CARTESIAN_POINT('Ctrl Pts',(67.7054521146424,26.5754854107421,0.));
#113196=CARTESIAN_POINT('Ctrl Pts',(67.7239923043288,26.5927690608544,0.));
#113197=CARTESIAN_POINT('Ctrl Pts',(67.7425448906977,26.6100971659202,0.));
#113198=CARTESIAN_POINT('Ctrl Pts',(67.7611097605042,26.6274696944793,0.));
#113199=CARTESIAN_POINT('Ctrl Pts',(67.7796868009455,26.6448866151029,0.));
#113200=CARTESIAN_POINT('Ctrl Pts',(67.798275899657,26.6623478963871,0.));
#113201=CARTESIAN_POINT('Ctrl Pts',(67.8168769447098,26.6798535069589,0.));
#113202=CARTESIAN_POINT('Ctrl Pts',(67.8354898246086,26.6974034154804,0.));
#113203=CARTESIAN_POINT('Ctrl Pts',(67.8541144282875,26.7149975906478,0.));
#113204=CARTESIAN_POINT('Ctrl Pts',(67.8727506451063,26.7326360011885,0.));
#113205=CARTESIAN_POINT('Ctrl Pts',(67.8913983648436,26.7503186158522,0.));
#113206=CARTESIAN_POINT('Ctrl Pts',(67.9100574776972,26.7680454034169,0.));
#113207=CARTESIAN_POINT('Ctrl Pts',(67.928727874284,26.7858163326934,0.));
#113208=CARTESIAN_POINT('Ctrl Pts',(67.9474094456396,26.8036313725262,0.));
#113209=CARTESIAN_POINT('Ctrl Pts',(67.9661020832164,26.821490491792,0.));
#113210=CARTESIAN_POINT('Ctrl Pts',(67.9848056788809,26.8393936593911,0.));
#113211=CARTESIAN_POINT('Ctrl Pts',(68.0035201249102,26.8573408442496,0.));
#113212=CARTESIAN_POINT('Ctrl Pts',(68.0222453139856,26.8753320153252,0.));
#113213=CARTESIAN_POINT('Ctrl Pts',(68.0409811391869,26.8933671416063,0.));
#113214=CARTESIAN_POINT('Ctrl Pts',(68.0597274939859,26.911446192111,0.));
#113215=CARTESIAN_POINT('Ctrl Pts',(68.0784842722369,26.9295691358779,0.));
#113216=CARTESIAN_POINT('Ctrl Pts',(68.0972513681751,26.9477359419652,0.));
#113217=CARTESIAN_POINT('Ctrl Pts',(68.1160286764255,26.9659465794601,0.));
#113218=CARTESIAN_POINT('Ctrl Pts',(68.1348160920106,26.9842010174822,0.));
#113219=CARTESIAN_POINT('Ctrl Pts',(68.1536135103557,27.0024992251838,0.));
#113220=CARTESIAN_POINT('Ctrl Pts',(68.1724208272958,27.0208411717472,0.));
#113221=CARTESIAN_POINT('Ctrl Pts',(68.1912379390773,27.0392268263798,0.));
#113222=CARTESIAN_POINT('Ctrl Pts',(68.2100647423332,27.0576561583172,0.));
#113223=CARTESIAN_POINT('Ctrl Pts',(68.2289011340615,27.0761291368226,0.));
#113224=CARTESIAN_POINT('Ctrl Pts',(68.2477470116012,27.0946457311813,0.));
#113225=CARTESIAN_POINT('Ctrl Pts',(68.2666022726104,27.1132059106943,0.));
#113226=CARTESIAN_POINT('Ctrl Pts',(68.2854668150364,27.1318096446649,0.));
#113227=CARTESIAN_POINT('Ctrl Pts',(68.3043405371603,27.1504569024136,0.));
#113228=CARTESIAN_POINT('Ctrl Pts',(68.3232233376425,27.1691476532921,0.));
#113229=CARTESIAN_POINT('Ctrl Pts',(68.3421151155711,27.1878818666926,0.));
#113230=CARTESIAN_POINT('Ctrl Pts',(68.3610157704994,27.2066595120542,0.));
#113231=CARTESIAN_POINT('Ctrl Pts',(68.3799252025102,27.2254805588673,0.));
#113232=CARTESIAN_POINT('Ctrl Pts',(68.3988433121581,27.244344976665,0.));
#113233=CARTESIAN_POINT('Ctrl Pts',(68.4177700003465,27.263252735006,0.));
#113234=CARTESIAN_POINT('Ctrl Pts',(68.4367051682164,27.2822038034538,0.));
#113235=CARTESIAN_POINT('Ctrl Pts',(68.4556487170441,27.301198151557,0.));
#113236=CARTESIAN_POINT('Ctrl Pts',(68.4746005480997,27.3202357488154,0.));
#113237=CARTESIAN_POINT('Ctrl Pts',(68.4935605626372,27.3393165646752,0.));
#113238=CARTESIAN_POINT('Ctrl Pts',(68.5125286621902,27.3584405685947,0.));
#113239=CARTESIAN_POINT('Ctrl Pts',(68.5315047488046,27.3776077300918,0.));
#113240=CARTESIAN_POINT('Ctrl Pts',(68.5504887252976,27.3968180187941,0.));
#113241=CARTESIAN_POINT('Ctrl Pts',(68.5694804955002,27.4160714044825,0.));
#113242=CARTESIAN_POINT('Ctrl Pts',(68.5884799645193,27.4353678571349,0.));
#113243=CARTESIAN_POINT('Ctrl Pts',(68.6074870381588,27.4547073468213,0.));
#113244=CARTESIAN_POINT('Ctrl Pts',(68.6265016223536,27.4740898435977,0.));
#113245=CARTESIAN_POINT('Ctrl Pts',(68.6455236225471,27.4935153173863,0.));
#113246=CARTESIAN_POINT('Ctrl Pts',(68.6645529432059,27.5129837378798,0.));
#113247=CARTESIAN_POINT('Ctrl Pts',(68.683589486992,27.5324950743723,0.));
#113248=CARTESIAN_POINT('Ctrl Pts',(68.7026331554348,27.552049295893,0.));
#113249=CARTESIAN_POINT('Ctrl Pts',(68.721683850427,27.5716463715027,0.));
#113250=CARTESIAN_POINT('Ctrl Pts',(68.7407414755291,27.5912862705482,0.));
#113251=CARTESIAN_POINT('Ctrl Pts',(68.7598059372121,27.6109689629025,0.));
#113252=CARTESIAN_POINT('Ctrl Pts',(68.7788771464655,27.6306944192711,0.));
#113253=CARTESIAN_POINT('Ctrl Pts',(68.7979550191773,27.6504626112621,0.));
#113254=CARTESIAN_POINT('Ctrl Pts',(68.8143140938753,27.6674443909882,0.));
#113255=CARTESIAN_POINT('Ctrl Pts',(68.826859785198,27.6804870323286,0.));
#113256=CARTESIAN_POINT('Ctrl Pts',(68.8355891981877,27.6895716271084,0.));
#113257=CARTESIAN_POINT('Ctrl Pts',(68.8405004465895,27.6946856803482,0.));
#113258=CARTESIAN_POINT('Ctrl Pts',(68.8415926174774,27.6958230984757,0.));
#113259=CARTESIAN_POINT('',(65.4815644032299,24.7419628022042,12.));
#113260=CARTESIAN_POINT('',(65.4815644032299,24.7419628022042,0.));
#113261=CARTESIAN_POINT('Ctrl Pts',(68.8415926174774,27.6958230984758,12.));
#113262=CARTESIAN_POINT('Ctrl Pts',(68.8405004465895,27.6946856803482,12.));
#113263=CARTESIAN_POINT('Ctrl Pts',(68.8355891981877,27.6895716271084,12.));
#113264=CARTESIAN_POINT('Ctrl Pts',(68.826859785198,27.6804870323286,12.));
#113265=CARTESIAN_POINT('Ctrl Pts',(68.8143140938753,27.6674443909882,12.));
#113266=CARTESIAN_POINT('Ctrl Pts',(68.7979550191773,27.6504626112621,12.));
#113267=CARTESIAN_POINT('Ctrl Pts',(68.7788771464655,27.6306944192711,12.));
#113268=CARTESIAN_POINT('Ctrl Pts',(68.7598059372121,27.6109689629025,12.));
#113269=CARTESIAN_POINT('Ctrl Pts',(68.7407414755291,27.5912862705482,12.));
#113270=CARTESIAN_POINT('Ctrl Pts',(68.721683850427,27.5716463715027,12.));
#113271=CARTESIAN_POINT('Ctrl Pts',(68.7026331554348,27.552049295893,12.));
#113272=CARTESIAN_POINT('Ctrl Pts',(68.683589486992,27.5324950743723,12.));
#113273=CARTESIAN_POINT('Ctrl Pts',(68.6645529432059,27.5129837378798,12.));
#113274=CARTESIAN_POINT('Ctrl Pts',(68.6455236225471,27.4935153173863,12.));
#113275=CARTESIAN_POINT('Ctrl Pts',(68.6265016223536,27.4740898435977,12.));
#113276=CARTESIAN_POINT('Ctrl Pts',(68.6074870381588,27.4547073468213,12.));
#113277=CARTESIAN_POINT('Ctrl Pts',(68.5884799645193,27.4353678571349,12.));
#113278=CARTESIAN_POINT('Ctrl Pts',(68.5694804955002,27.4160714044825,12.));
#113279=CARTESIAN_POINT('Ctrl Pts',(68.5504887252976,27.3968180187941,12.));
#113280=CARTESIAN_POINT('Ctrl Pts',(68.5315047488046,27.3776077300918,12.));
#113281=CARTESIAN_POINT('Ctrl Pts',(68.5125286621902,27.3584405685947,12.));
#113282=CARTESIAN_POINT('Ctrl Pts',(68.4935605626372,27.3393165646752,12.));
#113283=CARTESIAN_POINT('Ctrl Pts',(68.4746005480997,27.3202357488154,12.));
#113284=CARTESIAN_POINT('Ctrl Pts',(68.4556487170441,27.301198151557,12.));
#113285=CARTESIAN_POINT('Ctrl Pts',(68.4367051682164,27.2822038034538,12.));
#113286=CARTESIAN_POINT('Ctrl Pts',(68.4177700003465,27.263252735006,12.));
#113287=CARTESIAN_POINT('Ctrl Pts',(68.3988433121581,27.244344976665,12.));
#113288=CARTESIAN_POINT('Ctrl Pts',(68.3799252025102,27.2254805588673,12.));
#113289=CARTESIAN_POINT('Ctrl Pts',(68.3610157704994,27.2066595120542,12.));
#113290=CARTESIAN_POINT('Ctrl Pts',(68.3421151155711,27.1878818666926,12.));
#113291=CARTESIAN_POINT('Ctrl Pts',(68.3232233376425,27.1691476532921,12.));
#113292=CARTESIAN_POINT('Ctrl Pts',(68.3043405371603,27.1504569024136,12.));
#113293=CARTESIAN_POINT('Ctrl Pts',(68.2854668150364,27.1318096446649,12.));
#113294=CARTESIAN_POINT('Ctrl Pts',(68.2666022726104,27.1132059106943,12.));
#113295=CARTESIAN_POINT('Ctrl Pts',(68.2477470116012,27.0946457311813,12.));
#113296=CARTESIAN_POINT('Ctrl Pts',(68.2289011340615,27.0761291368226,12.));
#113297=CARTESIAN_POINT('Ctrl Pts',(68.2100647423332,27.0576561583172,12.));
#113298=CARTESIAN_POINT('Ctrl Pts',(68.1912379390773,27.0392268263798,12.));
#113299=CARTESIAN_POINT('Ctrl Pts',(68.1724208272958,27.0208411717472,12.));
#113300=CARTESIAN_POINT('Ctrl Pts',(68.1536135103557,27.0024992251838,12.));
#113301=CARTESIAN_POINT('Ctrl Pts',(68.1348160920106,26.9842010174822,12.));
#113302=CARTESIAN_POINT('Ctrl Pts',(68.1160286764255,26.9659465794601,12.));
#113303=CARTESIAN_POINT('Ctrl Pts',(68.0972513681751,26.9477359419652,12.));
#113304=CARTESIAN_POINT('Ctrl Pts',(68.0784842722369,26.9295691358779,12.));
#113305=CARTESIAN_POINT('Ctrl Pts',(68.0597274939859,26.911446192111,12.));
#113306=CARTESIAN_POINT('Ctrl Pts',(68.0409811391869,26.8933671416063,12.));
#113307=CARTESIAN_POINT('Ctrl Pts',(68.0222453139856,26.8753320153252,12.));
#113308=CARTESIAN_POINT('Ctrl Pts',(68.0035201249102,26.8573408442496,12.));
#113309=CARTESIAN_POINT('Ctrl Pts',(67.9848056788809,26.8393936593911,12.));
#113310=CARTESIAN_POINT('Ctrl Pts',(67.9661020832164,26.821490491792,12.));
#113311=CARTESIAN_POINT('Ctrl Pts',(67.9474094456396,26.8036313725262,12.));
#113312=CARTESIAN_POINT('Ctrl Pts',(67.928727874284,26.7858163326934,12.));
#113313=CARTESIAN_POINT('Ctrl Pts',(67.9100574776972,26.7680454034169,12.));
#113314=CARTESIAN_POINT('Ctrl Pts',(67.8913983648436,26.7503186158522,12.));
#113315=CARTESIAN_POINT('Ctrl Pts',(67.8727506451063,26.7326360011885,12.));
#113316=CARTESIAN_POINT('Ctrl Pts',(67.8541144282875,26.7149975906478,12.));
#113317=CARTESIAN_POINT('Ctrl Pts',(67.8354898246086,26.6974034154804,12.));
#113318=CARTESIAN_POINT('Ctrl Pts',(67.8168769447098,26.6798535069589,12.));
#113319=CARTESIAN_POINT('Ctrl Pts',(67.798275899657,26.6623478963871,12.));
#113320=CARTESIAN_POINT('Ctrl Pts',(67.7796868009455,26.6448866151029,12.));
#113321=CARTESIAN_POINT('Ctrl Pts',(67.7611097605042,26.6274696944793,12.));
#113322=CARTESIAN_POINT('Ctrl Pts',(67.7425448906977,26.6100971659202,12.));
#113323=CARTESIAN_POINT('Ctrl Pts',(67.7239923043288,26.5927690608544,12.));
#113324=CARTESIAN_POINT('Ctrl Pts',(67.7054521146424,26.5754854107421,12.));
#113325=CARTESIAN_POINT('Ctrl Pts',(67.6869244353294,26.5582462470794,12.));
#113326=CARTESIAN_POINT('Ctrl Pts',(67.6684093805291,26.5410516013985,12.));
#113327=CARTESIAN_POINT('Ctrl Pts',(67.649907064832,26.5239015052654,12.));
#113328=CARTESIAN_POINT('Ctrl Pts',(67.6314176032811,26.5067959902725,12.));
#113329=CARTESIAN_POINT('Ctrl Pts',(67.6129411113757,26.489735088044,12.));
#113330=CARTESIAN_POINT('Ctrl Pts',(67.5944777050768,26.4727188302409,12.));
#113331=CARTESIAN_POINT('Ctrl Pts',(67.5760275008093,26.4557472485621,12.));
#113332=CARTESIAN_POINT('Ctrl Pts',(67.5575906154657,26.4388203747425,12.));
#113333=CARTESIAN_POINT('Ctrl Pts',(67.5391671664072,26.4219382405458,12.));
#113334=CARTESIAN_POINT('Ctrl Pts',(67.5207572714683,26.4051008777675,12.));
#113335=CARTESIAN_POINT('Ctrl Pts',(67.5023610489622,26.3883083182421,12.));
#113336=CARTESIAN_POINT('Ctrl Pts',(67.4839786176836,26.3715605938433,12.));
#113337=CARTESIAN_POINT('Ctrl Pts',(67.4656100969116,26.3548577364833,12.));
#113338=CARTESIAN_POINT('Ctrl Pts',(67.4472556064119,26.3381997781055,12.));
#113339=CARTESIAN_POINT('Ctrl Pts',(67.4289152664398,26.321586750686,12.));
#113340=CARTESIAN_POINT('Ctrl Pts',(67.4105891977461,26.3050186862407,12.));
#113341=CARTESIAN_POINT('Ctrl Pts',(67.392277521581,26.288495616827,12.));
#113342=CARTESIAN_POINT('Ctrl Pts',(67.3739803596969,26.2720175745423,12.));
#113343=CARTESIAN_POINT('Ctrl Pts',(67.3556978343507,26.255584591518,12.));
#113344=CARTESIAN_POINT('Ctrl Pts',(67.3374300683073,26.2391966999191,12.));
#113345=CARTESIAN_POINT('Ctrl Pts',(67.3191771848463,26.2228539319526,12.));
#113346=CARTESIAN_POINT('Ctrl Pts',(67.3009393077651,26.2065563198683,12.));
#113347=CARTESIAN_POINT('Ctrl Pts',(67.282716561383,26.1903038959589,12.));
#113348=CARTESIAN_POINT('Ctrl Pts',(67.2645090705421,26.1740966925529,12.));
#113349=CARTESIAN_POINT('Ctrl Pts',(67.2463169606115,26.1579347420138,12.));
#113350=CARTESIAN_POINT('Ctrl Pts',(67.2281403574938,26.1418180767489,12.));
#113351=CARTESIAN_POINT('Ctrl Pts',(67.2099793876297,26.1257467292102,12.));
#113352=CARTESIAN_POINT('Ctrl Pts',(67.1918341780018,26.1097207318949,12.));
#113353=CARTESIAN_POINT('Ctrl Pts',(67.173704856136,26.0937401173383,12.));
#113354=CARTESIAN_POINT('Ctrl Pts',(67.1555915501049,26.0778049181128,12.));
#113355=CARTESIAN_POINT('Ctrl Pts',(67.1374943885354,26.061915166836,12.));
#113356=CARTESIAN_POINT('Ctrl Pts',(67.1194135006124,26.0460708961725,12.));
#113357=CARTESIAN_POINT('Ctrl Pts',(67.101349016084,26.030272138834,12.));
#113358=CARTESIAN_POINT('Ctrl Pts',(67.0833010652634,26.014518927573,12.));
#113359=CARTESIAN_POINT('Ctrl Pts',(67.0652697790325,25.9988112951814,12.));
#113360=CARTESIAN_POINT('Ctrl Pts',(67.0472552888485,25.9831492744984,12.));
#113361=CARTESIAN_POINT('Ctrl Pts',(67.0292577267489,25.9675328984121,12.));
#113362=CARTESIAN_POINT('Ctrl Pts',(67.0112772253556,25.9519621998598,12.));
#113363=CARTESIAN_POINT('Ctrl Pts',(66.9933139178778,25.9364372118222,12.));
#113364=CARTESIAN_POINT('Ctrl Pts',(66.975367938115,25.9209579673209,12.));
#113365=CARTESIAN_POINT('Ctrl Pts',(66.9574394204663,25.9055244994277,12.));
#113366=CARTESIAN_POINT('Ctrl Pts',(66.939528499934,25.890136841266,12.));
#113367=CARTESIAN_POINT('Ctrl Pts',(66.92163531213,25.8747950260111,12.));
#113368=CARTESIAN_POINT('Ctrl Pts',(66.9037599932761,25.8594990868833,12.));
#113369=CARTESIAN_POINT('Ctrl Pts',(66.8859026802088,25.844249057147,12.));
#113370=CARTESIAN_POINT('Ctrl Pts',(66.8680635103876,25.8290449701193,12.));
#113371=CARTESIAN_POINT('Ctrl Pts',(66.8502426219001,25.8138868591709,12.));
#113372=CARTESIAN_POINT('Ctrl Pts',(66.8324401534668,25.7987747577269,12.));
#113373=CARTESIAN_POINT('Ctrl Pts',(66.8146562444433,25.7837086992595,12.));
#113374=CARTESIAN_POINT('Ctrl Pts',(66.7968910348245,25.7686887172878,12.));
#113375=CARTESIAN_POINT('Ctrl Pts',(66.7791446652545,25.7537148453864,12.));
#113376=CARTESIAN_POINT('Ctrl Pts',(66.7614172770316,25.7387871171866,12.));
#113377=CARTESIAN_POINT('Ctrl Pts',(66.7437090121153,25.7239055663772,12.));
#113378=CARTESIAN_POINT('Ctrl Pts',(66.7260200131266,25.7090702266963,12.));
#113379=CARTESIAN_POINT('Ctrl Pts',(66.7083504233529,25.6942811319322,12.));
#113380=CARTESIAN_POINT('Ctrl Pts',(66.6907003867572,25.6795383159319,12.));
#113381=CARTESIAN_POINT('Ctrl Pts',(66.6730700479837,25.6648418126013,12.));
#113382=CARTESIAN_POINT('Ctrl Pts',(66.6554595523624,25.6501916559055,12.));
#113383=CARTESIAN_POINT('Ctrl Pts',(66.6378690459129,25.6355878798614,12.));
#113384=CARTESIAN_POINT('Ctrl Pts',(66.6202986753506,25.6210305185403,12.));
#113385=CARTESIAN_POINT('Ctrl Pts',(66.6027485880963,25.6065196060756,12.));
#113386=CARTESIAN_POINT('Ctrl Pts',(66.5852189322813,25.5920551766629,12.));
#113387=CARTESIAN_POINT('Ctrl Pts',(66.5677098567542,25.5776372645601,12.));
#113388=CARTESIAN_POINT('Ctrl Pts',(66.5502215110829,25.5632659040792,12.));
#113389=CARTESIAN_POINT('Ctrl Pts',(66.5327540455624,25.5489411295912,12.));
#113390=CARTESIAN_POINT('Ctrl Pts',(66.5153076112231,25.534662975532,12.));
#113391=CARTESIAN_POINT('Ctrl Pts',(66.4978823598354,25.5204314764033,12.));
#113392=CARTESIAN_POINT('Ctrl Pts',(66.4804784439148,25.5062466667702,12.));
#113393=CARTESIAN_POINT('Ctrl Pts',(66.4630960167252,25.4921085812548,12.));
#113394=CARTESIAN_POINT('Ctrl Pts',(66.4457352322871,25.4780172545417,12.));
#113395=CARTESIAN_POINT('Ctrl Pts',(66.4283962453899,25.4639727213849,12.));
#113396=CARTESIAN_POINT('Ctrl Pts',(66.4110792116,25.4499750166079,12.));
#113397=CARTESIAN_POINT('Ctrl Pts',(66.3937842872685,25.4360241751018,12.));
#113398=CARTESIAN_POINT('Ctrl Pts',(66.3765116295364,25.4221202318199,12.));
#113399=CARTESIAN_POINT('Ctrl Pts',(66.359261396341,25.4082632217847,12.));
#113400=CARTESIAN_POINT('Ctrl Pts',(66.3420337464178,25.3944531800901,12.));
#113401=CARTESIAN_POINT('Ctrl Pts',(66.3248288393046,25.3806901419012,12.));
#113402=CARTESIAN_POINT('Ctrl Pts',(66.3076468353412,25.3669741424488,12.));
#113403=CARTESIAN_POINT('Ctrl Pts',(66.290487895671,25.3533052170249,12.));
#113404=CARTESIAN_POINT('Ctrl Pts',(66.2733521822662,25.3396834009949,12.));
#113405=CARTESIAN_POINT('Ctrl Pts',(66.2562398579471,25.3261087298026,12.));
#113406=CARTESIAN_POINT('Ctrl Pts',(66.2391510863998,25.312581238973,12.));
#113407=CARTESIAN_POINT('Ctrl Pts',(66.2220860321952,25.2991009641094,12.));
#113408=CARTESIAN_POINT('Ctrl Pts',(66.2050448607911,25.285667940893,12.));
#113409=CARTESIAN_POINT('Ctrl Pts',(66.1880277385136,25.2722822050837,12.));
#113410=CARTESIAN_POINT('Ctrl Pts',(66.1710348325384,25.2589437925147,12.));
#113411=CARTESIAN_POINT('Ctrl Pts',(66.1540663108754,25.2456527390875,12.));
#113412=CARTESIAN_POINT('Ctrl Pts',(66.1371223423345,25.232409080755,12.));
#113413=CARTESIAN_POINT('Ctrl Pts',(66.1202030965758,25.2192128535357,12.));
#113414=CARTESIAN_POINT('Ctrl Pts',(66.10330874419,25.2060640935365,12.));
#113415=CARTESIAN_POINT('Ctrl Pts',(66.086439456768,25.1929628369685,12.));
#113416=CARTESIAN_POINT('Ctrl Pts',(66.0695954069713,25.1799091201599,12.));
#113417=CARTESIAN_POINT('Ctrl Pts',(66.0527767686025,25.1669029795661,12.));
#113418=CARTESIAN_POINT('Ctrl Pts',(66.0359837164734,25.1539444517419,12.));
#113419=CARTESIAN_POINT('Ctrl Pts',(66.0192164262621,25.1410335733099,12.));
#113420=CARTESIAN_POINT('Ctrl Pts',(66.0024750743897,25.1281703809297,12.));
#113421=CARTESIAN_POINT('Ctrl Pts',(65.9857598378433,25.1153549112503,12.));
#113422=CARTESIAN_POINT('Ctrl Pts',(65.9690708941558,25.1025872009004,12.));
#113423=CARTESIAN_POINT('Ctrl Pts',(65.9524084218139,25.0898672865915,12.));
#113424=CARTESIAN_POINT('Ctrl Pts',(65.9357726006163,25.0771952052028,12.));
#113425=CARTESIAN_POINT('Ctrl Pts',(65.919163611981,25.0645709938524,12.));
#113426=CARTESIAN_POINT('Ctrl Pts',(65.9025816394424,25.0519946900078,12.));
#113427=CARTESIAN_POINT('Ctrl Pts',(65.8860268683128,25.0394663314055,12.));
#113428=CARTESIAN_POINT('Ctrl Pts',(65.8694994847616,25.0269859558363,12.));
#113429=CARTESIAN_POINT('Ctrl Pts',(65.8529996750445,25.0145536009604,12.));
#113430=CARTESIAN_POINT('Ctrl Pts',(65.8365276247128,25.002169304117,12.));
#113431=CARTESIAN_POINT('Ctrl Pts',(65.8200835177024,24.9898331020983,12.));
#113432=CARTESIAN_POINT('Ctrl Pts',(65.8036675380718,24.9775450315683,12.));
#113433=CARTESIAN_POINT('Ctrl Pts',(65.7872798720823,24.9653051295581,12.));
#113434=CARTESIAN_POINT('Ctrl Pts',(65.7709207098959,24.9531134338696,12.));
#113435=CARTESIAN_POINT('Ctrl Pts',(65.7545902480323,24.9409699836537,12.));
#113436=CARTESIAN_POINT('Ctrl Pts',(65.7382886895888,24.928874819458,12.));
#113437=CARTESIAN_POINT('Ctrl Pts',(65.7220162391053,24.9168279820106,12.));
#113438=CARTESIAN_POINT('Ctrl Pts',(65.7057730980483,24.9048295111448,12.));
#113439=CARTESIAN_POINT('Ctrl Pts',(65.6895594608775,24.8928794448607,12.));
#113440=CARTESIAN_POINT('Ctrl Pts',(65.6733755087669,24.8809778178229,12.));
#113441=CARTESIAN_POINT('Ctrl Pts',(65.6572214156692,24.8691246628057,12.));
#113442=CARTESIAN_POINT('Ctrl Pts',(65.6410973603661,24.8573200135666,12.));
#113443=CARTESIAN_POINT('Ctrl Pts',(65.6250035361612,24.8455639071517,12.));
#113444=CARTESIAN_POINT('Ctrl Pts',(65.6089401625628,24.8338563866764,12.));
#113445=CARTESIAN_POINT('Ctrl Pts',(65.5929074932624,24.8221975032104,12.));
#113446=CARTESIAN_POINT('Ctrl Pts',(65.5769057914333,24.8105873098626,12.));
#113447=CARTESIAN_POINT('Ctrl Pts',(65.5609353062829,24.799025856126,12.));
#113448=CARTESIAN_POINT('Ctrl Pts',(65.5449962514661,24.7875131827491,12.));
#113449=CARTESIAN_POINT('Ctrl Pts',(65.5290887770232,24.7760493148465,12.));
#113450=CARTESIAN_POINT('Ctrl Pts',(65.5132129675333,24.7646342620841,12.));
#113451=CARTESIAN_POINT('Ctrl Pts',(65.5005376841101,24.7555412724651,12.));
#113452=CARTESIAN_POINT('Ctrl Pts',(65.4910454936254,24.7487434955982,12.));
#113453=CARTESIAN_POINT('Ctrl Pts',(65.4847237095443,24.7442214063382,12.));
#113454=CARTESIAN_POINT('Ctrl Pts',(65.4815644032299,24.7419628022042,12.));
#113455=CARTESIAN_POINT('Ctrl Pts',(68.2622612910177,29.0944526440266,0.));
#113456=CARTESIAN_POINT('Ctrl Pts',(68.2622612910177,29.0944526440266,4.));
#113457=CARTESIAN_POINT('Ctrl Pts',(68.2622612910177,29.0944526440266,8.));
#113458=CARTESIAN_POINT('Ctrl Pts',(68.2622612910177,29.0944526440266,12.));
#113459=CARTESIAN_POINT('Ctrl Pts',(68.3721211369508,29.0922231502663,0.));
#113460=CARTESIAN_POINT('Ctrl Pts',(68.3721211369508,29.0922231502663,4.));
#113461=CARTESIAN_POINT('Ctrl Pts',(68.3721211369509,29.0922231502664,8.00000000000001));
#113462=CARTESIAN_POINT('Ctrl Pts',(68.3721211369509,29.0922231502664,12.));
#113463=CARTESIAN_POINT('Ctrl Pts',(68.5624216146675,29.0225207419381,0.));
#113464=CARTESIAN_POINT('Ctrl Pts',(68.5624216146675,29.0225207419381,4.00000000000001));
#113465=CARTESIAN_POINT('Ctrl Pts',(68.5624216146676,29.0225207419382,7.99999999999999));
#113466=CARTESIAN_POINT('Ctrl Pts',(68.5624216146676,29.0225207419382,12.));
#113467=CARTESIAN_POINT('Ctrl Pts',(68.6814343344131,28.8637726134455,0.));
#113468=CARTESIAN_POINT('Ctrl Pts',(68.6814343344131,28.8637726134455,3.99999999999999));
#113469=CARTESIAN_POINT('Ctrl Pts',(68.6814343344132,28.8637726134455,8.00000000000001));
#113470=CARTESIAN_POINT('Ctrl Pts',(68.6814343344132,28.8637726134455,12.));
#113471=CARTESIAN_POINT('Ctrl Pts',(68.7132793373318,28.7877620302417,0.));
#113472=CARTESIAN_POINT('Ctrl Pts',(68.7132793373318,28.7877620302417,4.));
#113473=CARTESIAN_POINT('Ctrl Pts',(68.7132793373319,28.7877620302417,8.));
#113474=CARTESIAN_POINT('Ctrl Pts',(68.7132793373319,28.7877620302417,12.));
#113475=CARTESIAN_POINT('',(68.2622612910177,29.0944526440266,0.));
#113476=CARTESIAN_POINT('',(68.7132793373317,28.7877620302417,0.));
#113477=CARTESIAN_POINT('Ctrl Pts',(68.2622612910177,29.0944526440266,0.));
#113478=CARTESIAN_POINT('Ctrl Pts',(68.3721211369508,29.0922231502663,0.));
#113479=CARTESIAN_POINT('Ctrl Pts',(68.4808642670747,29.0523932026502,0.));
#113480=CARTESIAN_POINT('Ctrl Pts',(68.5663297619426,28.983487101511,0.));
#113481=CARTESIAN_POINT('Ctrl Pts',(68.6304288830936,28.9318075256566,0.));
#113482=CARTESIAN_POINT('Ctrl Pts',(68.6814343344131,28.8637726134455,0.));
#113483=CARTESIAN_POINT('Ctrl Pts',(68.7132793373318,28.7877620302417,0.));
#113484=CARTESIAN_POINT('',(68.7132793373317,28.7877620302417,12.));
#113485=CARTESIAN_POINT('Ctrl Pts',(68.7132793373318,28.7877620302417,0.));
#113486=CARTESIAN_POINT('Ctrl Pts',(68.7132793373318,28.7877620302417,4.));
#113487=CARTESIAN_POINT('Ctrl Pts',(68.7132793373319,28.7877620302417,8.));
#113488=CARTESIAN_POINT('Ctrl Pts',(68.7132793373319,28.7877620302417,12.));
#113489=CARTESIAN_POINT('',(68.2622612910177,29.0944526440266,12.));
#113490=CARTESIAN_POINT('Ctrl Pts',(68.7132793373319,28.7877620302417,12.));
#113491=CARTESIAN_POINT('Ctrl Pts',(68.6814343344132,28.8637726134455,12.));
#113492=CARTESIAN_POINT('Ctrl Pts',(68.6304288830936,28.9318075256567,12.));
#113493=CARTESIAN_POINT('Ctrl Pts',(68.5663297619426,28.9834871015111,12.));
#113494=CARTESIAN_POINT('Ctrl Pts',(68.4808642670747,29.0523932026503,12.));
#113495=CARTESIAN_POINT('Ctrl Pts',(68.3721211369509,29.0922231502664,12.));
#113496=CARTESIAN_POINT('Ctrl Pts',(68.2622612910177,29.0944526440266,12.));
#113497=CARTESIAN_POINT('Ctrl Pts',(68.2622612910177,29.0944526440266,12.));
#113498=CARTESIAN_POINT('Ctrl Pts',(68.2622612910177,29.0944526440266,8.));
#113499=CARTESIAN_POINT('Ctrl Pts',(68.2622612910177,29.0944526440266,4.));
#113500=CARTESIAN_POINT('Ctrl Pts',(68.2622612910177,29.0944526440266,0.));
#113501=CARTESIAN_POINT('Origin',(3.46272497684358E-10,1.43538201480493E-10,
0.));
#113502=CARTESIAN_POINT('Origin',(3.46272497684358E-10,1.43538201480493E-10,
12.));
#113503=CARTESIAN_POINT('Origin',(3.46272497684358E-10,1.43538201480493E-10,
0.));
#113504=CARTESIAN_POINT('Ctrl Pts',(71.1418425484881,22.1153394458717,0.));
#113505=CARTESIAN_POINT('Ctrl Pts',(71.1418425484881,22.1153394458717,4.));
#113506=CARTESIAN_POINT('Ctrl Pts',(71.1418425484881,22.1153394458717,8.));
#113507=CARTESIAN_POINT('Ctrl Pts',(71.1418425484881,22.1153394458717,12.));
#113508=CARTESIAN_POINT('Ctrl Pts',(71.1744611799059,22.0104100349462,0.));
#113509=CARTESIAN_POINT('Ctrl Pts',(71.1744611799059,22.0104100349462,4.));
#113510=CARTESIAN_POINT('Ctrl Pts',(71.1744611799059,22.0104100349462,8.));
#113511=CARTESIAN_POINT('Ctrl Pts',(71.1744611799059,22.0104100349462,12.));
#113512=CARTESIAN_POINT('Ctrl Pts',(71.1685011351939,21.8078334561031,0.));
#113513=CARTESIAN_POINT('Ctrl Pts',(71.1685011351939,21.8078334561031,4.));
#113514=CARTESIAN_POINT('Ctrl Pts',(71.168501135194,21.8078334561031,8.));
#113515=CARTESIAN_POINT('Ctrl Pts',(71.168501135194,21.8078334561031,12.));
#113516=CARTESIAN_POINT('Ctrl Pts',(71.0555229320375,21.6447353227844,0.));
#113517=CARTESIAN_POINT('Ctrl Pts',(71.0555229320375,21.6447353227844,4.));
#113518=CARTESIAN_POINT('Ctrl Pts',(71.0555229320376,21.6447353227844,8.00000000000001));
#113519=CARTESIAN_POINT('Ctrl Pts',(71.0555229320376,21.6447353227844,12.));
#113520=CARTESIAN_POINT('Ctrl Pts',(70.9934796068774,21.5904919934804,0.));
#113521=CARTESIAN_POINT('Ctrl Pts',(70.9934796068774,21.5904919934804,4.));
#113522=CARTESIAN_POINT('Ctrl Pts',(70.9934796068774,21.5904919934804,8.));
#113523=CARTESIAN_POINT('Ctrl Pts',(70.9934796068774,21.5904919934804,12.));
#113524=CARTESIAN_POINT('',(71.1418425484881,22.1153394458717,0.));
#113525=CARTESIAN_POINT('',(70.9934796068777,21.59049199348,0.));
#113526=CARTESIAN_POINT('Ctrl Pts',(71.1418425484881,22.1153394458717,0.));
#113527=CARTESIAN_POINT('Ctrl Pts',(71.1744611799059,22.0104100349462,0.));
#113528=CARTESIAN_POINT('Ctrl Pts',(71.1710554400705,21.894651989893,0.));
#113529=CARTESIAN_POINT('Ctrl Pts',(71.1327049954369,21.7917848658274,0.));
#113530=CARTESIAN_POINT('Ctrl Pts',(71.1039421619617,21.7146345227781,0.));
#113531=CARTESIAN_POINT('Ctrl Pts',(71.0555229320375,21.6447353227844,0.));
#113532=CARTESIAN_POINT('Ctrl Pts',(70.9934796068774,21.5904919934804,0.));
#113533=CARTESIAN_POINT('',(70.9934796068777,21.5904919934801,12.));
#113534=CARTESIAN_POINT('Ctrl Pts',(70.9934796068774,21.5904919934804,0.));
#113535=CARTESIAN_POINT('Ctrl Pts',(70.9934796068774,21.5904919934804,4.));
#113536=CARTESIAN_POINT('Ctrl Pts',(70.9934796068774,21.5904919934804,8.));
#113537=CARTESIAN_POINT('Ctrl Pts',(70.9934796068774,21.5904919934804,12.));
#113538=CARTESIAN_POINT('',(71.1418425484881,22.1153394458717,12.));
#113539=CARTESIAN_POINT('Ctrl Pts',(70.9934796068774,21.5904919934804,12.));
#113540=CARTESIAN_POINT('Ctrl Pts',(71.0555229320376,21.6447353227844,12.));
#113541=CARTESIAN_POINT('Ctrl Pts',(71.1039421619617,21.7146345227781,12.));
#113542=CARTESIAN_POINT('Ctrl Pts',(71.1327049954369,21.7917848658274,12.));
#113543=CARTESIAN_POINT('Ctrl Pts',(71.1710554400705,21.894651989893,12.));
#113544=CARTESIAN_POINT('Ctrl Pts',(71.1744611799059,22.0104100349462,12.));
#113545=CARTESIAN_POINT('Ctrl Pts',(71.1418425484881,22.1153394458717,12.));
#113546=CARTESIAN_POINT('Ctrl Pts',(71.1418425484881,22.1153394458717,12.));
#113547=CARTESIAN_POINT('Ctrl Pts',(71.1418425484881,22.1153394458717,8.));
#113548=CARTESIAN_POINT('Ctrl Pts',(71.1418425484881,22.1153394458717,4.));
#113549=CARTESIAN_POINT('Ctrl Pts',(71.1418425484881,22.1153394458717,0.));
#113550=CARTESIAN_POINT('Ctrl Pts',(67.3887914263118,18.9407177820969,0.));
#113551=CARTESIAN_POINT('Ctrl Pts',(67.3887914263118,18.9407177820969,12.));
#113552=CARTESIAN_POINT('Ctrl Pts',(67.3921355608328,18.9426924398719,0.));
#113553=CARTESIAN_POINT('Ctrl Pts',(67.3921355608328,18.9426924398719,12.));
#113554=CARTESIAN_POINT('Ctrl Pts',(67.3988274146651,18.9466463414299,0.));
#113555=CARTESIAN_POINT('Ctrl Pts',(67.3988274146651,18.9466463414299,12.));
#113556=CARTESIAN_POINT('Ctrl Pts',(67.4088759497911,18.9525909517915,0.));
#113557=CARTESIAN_POINT('Ctrl Pts',(67.4088759497911,18.9525909517915,12.));
#113558=CARTESIAN_POINT('Ctrl Pts',(67.4222955061981,18.9605446160985,0.));
#113559=CARTESIAN_POINT('Ctrl Pts',(67.4222955061981,18.9605446160985,12.));
#113560=CARTESIAN_POINT('Ctrl Pts',(67.4391057908418,18.9705325631711,0.));
#113561=CARTESIAN_POINT('Ctrl Pts',(67.4391057908418,18.9705325631711,12.));
#113562=CARTESIAN_POINT('Ctrl Pts',(67.4559518744638,18.9805663798449,0.));
#113563=CARTESIAN_POINT('Ctrl Pts',(67.4559518744638,18.9805663798449,12.));
#113564=CARTESIAN_POINT('Ctrl Pts',(67.472833671964,18.9906460638625,0.));
#113565=CARTESIAN_POINT('Ctrl Pts',(67.472833671964,18.9906460638625,12.));
#113566=CARTESIAN_POINT('Ctrl Pts',(67.4897510316844,19.0007716032819,0.));
#113567=CARTESIAN_POINT('Ctrl Pts',(67.4897510316844,19.0007716032819,12.));
#113568=CARTESIAN_POINT('Ctrl Pts',(67.5067037372317,19.0109429761306,0.));
#113569=CARTESIAN_POINT('Ctrl Pts',(67.5067037372317,19.0109429761306,12.));
#113570=CARTESIAN_POINT('Ctrl Pts',(67.5236915360331,19.021160154824,0.));
#113571=CARTESIAN_POINT('Ctrl Pts',(67.5236915360331,19.021160154824,12.));
#113572=CARTESIAN_POINT('Ctrl Pts',(67.540714161288,19.0314231093923,0.));
#113573=CARTESIAN_POINT('Ctrl Pts',(67.540714161288,19.0314231093923,12.));
#113574=CARTESIAN_POINT('Ctrl Pts',(67.5577713558194,19.0417318110708,0.));
#113575=CARTESIAN_POINT('Ctrl Pts',(67.5577713558194,19.0417318110708,12.));
#113576=CARTESIAN_POINT('Ctrl Pts',(67.5748628971964,19.0520862360396,0.));
#113577=CARTESIAN_POINT('Ctrl Pts',(67.5748628971964,19.0520862360396,12.));
#113578=CARTESIAN_POINT('Ctrl Pts',(67.5919885896222,19.062486364241,0.));
#113579=CARTESIAN_POINT('Ctrl Pts',(67.5919885896222,19.062486364241,12.));
#113580=CARTESIAN_POINT('Ctrl Pts',(67.6091482520534,19.072932177628,0.));
#113581=CARTESIAN_POINT('Ctrl Pts',(67.6091482520534,19.072932177628,12.));
#113582=CARTESIAN_POINT('Ctrl Pts',(67.6263417083426,19.0834236587118,0.));
#113583=CARTESIAN_POINT('Ctrl Pts',(67.6263417083426,19.0834236587118,12.));
#113584=CARTESIAN_POINT('Ctrl Pts',(67.6435687749841,19.0939607887502,0.));
#113585=CARTESIAN_POINT('Ctrl Pts',(67.6435687749841,19.0939607887502,12.));
#113586=CARTESIAN_POINT('Ctrl Pts',(67.6608292549462,19.1045435468358,0.));
#113587=CARTESIAN_POINT('Ctrl Pts',(67.6608292549462,19.1045435468358,12.));
#113588=CARTESIAN_POINT('Ctrl Pts',(67.6781229440573,19.115171910846,0.));
#113589=CARTESIAN_POINT('Ctrl Pts',(67.6781229440573,19.115171910846,12.));
#113590=CARTESIAN_POINT('Ctrl Pts',(67.6954496350063,19.1258458580345,0.));
#113591=CARTESIAN_POINT('Ctrl Pts',(67.6954496350063,19.1258458580345,12.));
#113592=CARTESIAN_POINT('Ctrl Pts',(67.7128091219348,19.136565365709,0.));
#113593=CARTESIAN_POINT('Ctrl Pts',(67.7128091219348,19.136565365709,12.));
#113594=CARTESIAN_POINT('Ctrl Pts',(67.7302012056584,19.1473304119955,0.));
#113595=CARTESIAN_POINT('Ctrl Pts',(67.7302012056584,19.1473304119955,12.));
#113596=CARTESIAN_POINT('Ctrl Pts',(67.7476256934444,19.1581409758097,0.));
#113597=CARTESIAN_POINT('Ctrl Pts',(67.7476256934444,19.1581409758097,12.));
#113598=CARTESIAN_POINT('Ctrl Pts',(67.7650823965127,19.168997036495,0.));
#113599=CARTESIAN_POINT('Ctrl Pts',(67.7650823965127,19.168997036495,12.));
#113600=CARTESIAN_POINT('Ctrl Pts',(67.7825711283096,19.1798985735688,0.));
#113601=CARTESIAN_POINT('Ctrl Pts',(67.7825711283096,19.1798985735688,12.));
#113602=CARTESIAN_POINT('Ctrl Pts',(67.8000917023926,19.1908455664098,0.));
#113603=CARTESIAN_POINT('Ctrl Pts',(67.8000917023926,19.1908455664098,12.));
#113604=CARTESIAN_POINT('Ctrl Pts',(67.8176439306621,19.201837993993,0.));
#113605=CARTESIAN_POINT('Ctrl Pts',(67.8176439306621,19.201837993993,12.));
#113606=CARTESIAN_POINT('Ctrl Pts',(67.835227624289,19.2128758350346,0.));
#113607=CARTESIAN_POINT('Ctrl Pts',(67.835227624289,19.2128758350346,12.));
#113608=CARTESIAN_POINT('Ctrl Pts',(67.8528425945184,19.2239590681133,0.));
#113609=CARTESIAN_POINT('Ctrl Pts',(67.8528425945184,19.2239590681133,12.));
#113610=CARTESIAN_POINT('Ctrl Pts',(67.8704886534544,19.2350876717874,0.));
#113611=CARTESIAN_POINT('Ctrl Pts',(67.8704886534544,19.2350876717874,12.));
#113612=CARTESIAN_POINT('Ctrl Pts',(67.8881656149955,19.2462616247279,0.));
#113613=CARTESIAN_POINT('Ctrl Pts',(67.8881656149955,19.2462616247279,12.));
#113614=CARTESIAN_POINT('Ctrl Pts',(67.9058732951788,19.2574809057696,0.));
#113615=CARTESIAN_POINT('Ctrl Pts',(67.9058732951788,19.2574809057696,12.));
#113616=CARTESIAN_POINT('Ctrl Pts',(67.9236115116758,19.2687454938442,0.));
#113617=CARTESIAN_POINT('Ctrl Pts',(67.9236115116758,19.2687454938442,12.));
#113618=CARTESIAN_POINT('Ctrl Pts',(67.9413800834793,19.280055367936,0.));
#113619=CARTESIAN_POINT('Ctrl Pts',(67.9413800834793,19.280055367936,12.));
#113620=CARTESIAN_POINT('Ctrl Pts',(67.9591788305394,19.2914105070286,0.));
#113621=CARTESIAN_POINT('Ctrl Pts',(67.9591788305394,19.2914105070286,12.));
#113622=CARTESIAN_POINT('Ctrl Pts',(67.9770075733485,19.302810890038,0.));
#113623=CARTESIAN_POINT('Ctrl Pts',(67.9770075733485,19.302810890038,12.));
#113624=CARTESIAN_POINT('Ctrl Pts',(67.9948661329617,19.3142564958203,0.));
#113625=CARTESIAN_POINT('Ctrl Pts',(67.9948661329617,19.3142564958203,12.));
#113626=CARTESIAN_POINT('Ctrl Pts',(68.0127543311776,19.3257473032035,0.));
#113627=CARTESIAN_POINT('Ctrl Pts',(68.0127543311776,19.3257473032035,12.));
#113628=CARTESIAN_POINT('Ctrl Pts',(68.0306719906636,19.3372832910076,0.));
#113629=CARTESIAN_POINT('Ctrl Pts',(68.0306719906636,19.3372832910076,12.));
#113630=CARTESIAN_POINT('Ctrl Pts',(68.0486189351011,19.3488644380641,0.));
#113631=CARTESIAN_POINT('Ctrl Pts',(68.0486189351011,19.3488644380641,12.));
#113632=CARTESIAN_POINT('Ctrl Pts',(68.0665949893195,19.3604907232314,0.));
#113633=CARTESIAN_POINT('Ctrl Pts',(68.0665949893195,19.3604907232314,12.));
#113634=CARTESIAN_POINT('Ctrl Pts',(68.0845999792247,19.3721621253912,0.));
#113635=CARTESIAN_POINT('Ctrl Pts',(68.0845999792247,19.3721621253912,12.));
#113636=CARTESIAN_POINT('Ctrl Pts',(68.1026337317285,19.3838786234421,0.));
#113637=CARTESIAN_POINT('Ctrl Pts',(68.1026337317285,19.3838786234421,12.));
#113638=CARTESIAN_POINT('Ctrl Pts',(68.1206960746769,19.3956401962895,0.));
#113639=CARTESIAN_POINT('Ctrl Pts',(68.1206960746769,19.3956401962895,12.));
#113640=CARTESIAN_POINT('Ctrl Pts',(68.1387868367691,19.40744682283,0.));
#113641=CARTESIAN_POINT('Ctrl Pts',(68.1387868367691,19.40744682283,12.));
#113642=CARTESIAN_POINT('Ctrl Pts',(68.1569058475054,19.4192984819418,0.));
#113643=CARTESIAN_POINT('Ctrl Pts',(68.1569058475054,19.4192984819418,12.));
#113644=CARTESIAN_POINT('Ctrl Pts',(68.1750529372232,19.4311951524983,0.));
#113645=CARTESIAN_POINT('Ctrl Pts',(68.1750529372232,19.4311951524983,12.));
#113646=CARTESIAN_POINT('Ctrl Pts',(68.1932279371127,19.4431368133719,0.));
#113647=CARTESIAN_POINT('Ctrl Pts',(68.1932279371127,19.4431368133719,12.));
#113648=CARTESIAN_POINT('Ctrl Pts',(68.2114306792358,19.4551234434381,0.));
#113649=CARTESIAN_POINT('Ctrl Pts',(68.2114306792358,19.4551234434381,12.));
#113650=CARTESIAN_POINT('Ctrl Pts',(68.2296609965448,19.467155021572,0.));
#113651=CARTESIAN_POINT('Ctrl Pts',(68.2296609965448,19.467155021572,12.));
#113652=CARTESIAN_POINT('Ctrl Pts',(68.2479187228803,19.4792315266501,0.));
#113653=CARTESIAN_POINT('Ctrl Pts',(68.2479187228803,19.4792315266501,12.));
#113654=CARTESIAN_POINT('Ctrl Pts',(68.2662036929526,19.4913529375543,0.));
#113655=CARTESIAN_POINT('Ctrl Pts',(68.2662036929526,19.4913529375543,12.));
#113656=CARTESIAN_POINT('Ctrl Pts',(68.2845157423233,19.5035192331705,0.));
#113657=CARTESIAN_POINT('Ctrl Pts',(68.2845157423233,19.5035192331705,12.));
#113658=CARTESIAN_POINT('Ctrl Pts',(68.3028547073864,19.5157303923856,0.));
#113659=CARTESIAN_POINT('Ctrl Pts',(68.3028547073864,19.5157303923856,12.));
#113660=CARTESIAN_POINT('Ctrl Pts',(68.3212204253417,19.5279863940773,0.));
#113661=CARTESIAN_POINT('Ctrl Pts',(68.3212204253417,19.5279863940773,12.));
#113662=CARTESIAN_POINT('Ctrl Pts',(68.3396127341938,19.5402872171191,0.));
#113663=CARTESIAN_POINT('Ctrl Pts',(68.3396127341938,19.5402872171191,12.));
#113664=CARTESIAN_POINT('Ctrl Pts',(68.3580314727523,19.5526328403852,0.));
#113665=CARTESIAN_POINT('Ctrl Pts',(68.3580314727523,19.5526328403852,12.));
#113666=CARTESIAN_POINT('Ctrl Pts',(68.3764764806287,19.5650232427516,0.));
#113667=CARTESIAN_POINT('Ctrl Pts',(68.3764764806287,19.5650232427516,12.));
#113668=CARTESIAN_POINT('Ctrl Pts',(68.3949475982335,19.5774584030938,0.));
#113669=CARTESIAN_POINT('Ctrl Pts',(68.3949475982335,19.5774584030938,12.));
#113670=CARTESIAN_POINT('Ctrl Pts',(68.4134446667696,19.5899383002803,0.));
#113671=CARTESIAN_POINT('Ctrl Pts',(68.4134446667696,19.5899383002803,12.));
#113672=CARTESIAN_POINT('Ctrl Pts',(68.4319675282275,19.6024629131785,0.));
#113673=CARTESIAN_POINT('Ctrl Pts',(68.4319675282275,19.6024629131785,12.));
#113674=CARTESIAN_POINT('Ctrl Pts',(68.4505160253778,19.6150322206577,0.));
#113675=CARTESIAN_POINT('Ctrl Pts',(68.4505160253778,19.6150322206577,12.));
#113676=CARTESIAN_POINT('Ctrl Pts',(68.4690900017632,19.6276462015888,0.));
#113677=CARTESIAN_POINT('Ctrl Pts',(68.4690900017632,19.6276462015888,12.));
#113678=CARTESIAN_POINT('Ctrl Pts',(68.4876893016856,19.6403048348395,0.));
#113679=CARTESIAN_POINT('Ctrl Pts',(68.4876893016856,19.6403048348395,12.));
#113680=CARTESIAN_POINT('Ctrl Pts',(68.5063137701971,19.6530080992686,0.));
#113681=CARTESIAN_POINT('Ctrl Pts',(68.5063137701971,19.6530080992686,12.));
#113682=CARTESIAN_POINT('Ctrl Pts',(68.5249632530979,19.6657559737336,0.));
#113683=CARTESIAN_POINT('Ctrl Pts',(68.5249632530979,19.6657559737336,12.));
#113684=CARTESIAN_POINT('Ctrl Pts',(68.5436375969311,19.6785484370927,0.));
#113685=CARTESIAN_POINT('Ctrl Pts',(68.5436375969311,19.6785484370927,12.));
#113686=CARTESIAN_POINT('Ctrl Pts',(68.5623366489779,19.6913854682046,0.));
#113687=CARTESIAN_POINT('Ctrl Pts',(68.5623366489779,19.6913854682046,12.));
#113688=CARTESIAN_POINT('Ctrl Pts',(68.581060257249,19.7042670459237,0.));
#113689=CARTESIAN_POINT('Ctrl Pts',(68.581060257249,19.7042670459237,12.));
#113690=CARTESIAN_POINT('Ctrl Pts',(68.5998082704766,19.7171931490956,0.));
#113691=CARTESIAN_POINT('Ctrl Pts',(68.5998082704766,19.7171931490956,12.));
#113692=CARTESIAN_POINT('Ctrl Pts',(68.6185805381126,19.7301637565652,0.));
#113693=CARTESIAN_POINT('Ctrl Pts',(68.6185805381126,19.7301637565652,12.));
#113694=CARTESIAN_POINT('Ctrl Pts',(68.6373769103224,19.7431788471776,0.));
#113695=CARTESIAN_POINT('Ctrl Pts',(68.6373769103224,19.7431788471776,12.));
#113696=CARTESIAN_POINT('Ctrl Pts',(68.6561972379793,19.7562383997781,0.));
#113697=CARTESIAN_POINT('Ctrl Pts',(68.6561972379793,19.7562383997781,12.));
#113698=CARTESIAN_POINT('Ctrl Pts',(68.6750413726547,19.7693423932058,0.));
#113699=CARTESIAN_POINT('Ctrl Pts',(68.6750413726547,19.7693423932058,12.));
#113700=CARTESIAN_POINT('Ctrl Pts',(68.6939091666111,19.7824908062913,0.));
#113701=CARTESIAN_POINT('Ctrl Pts',(68.6939091666111,19.7824908062913,12.));
#113702=CARTESIAN_POINT('Ctrl Pts',(68.7128004727998,19.795683617864,0.));
#113703=CARTESIAN_POINT('Ctrl Pts',(68.7128004727998,19.795683617864,12.));
#113704=CARTESIAN_POINT('Ctrl Pts',(68.7317151448557,19.8089208067532,0.));
#113705=CARTESIAN_POINT('Ctrl Pts',(68.7317151448557,19.8089208067532,12.));
#113706=CARTESIAN_POINT('Ctrl Pts',(68.7506530370918,19.8222023517874,0.));
#113707=CARTESIAN_POINT('Ctrl Pts',(68.7506530370918,19.8222023517874,12.));
#113708=CARTESIAN_POINT('Ctrl Pts',(68.7696140044892,19.835528231787,0.));
#113709=CARTESIAN_POINT('Ctrl Pts',(68.7696140044892,19.835528231787,12.));
#113710=CARTESIAN_POINT('Ctrl Pts',(68.7885979026927,19.8488984255641,0.));
#113711=CARTESIAN_POINT('Ctrl Pts',(68.7885979026927,19.8488984255641,12.));
#113712=CARTESIAN_POINT('Ctrl Pts',(68.8076045880102,19.8623129119304,0.));
#113713=CARTESIAN_POINT('Ctrl Pts',(68.8076045880102,19.8623129119304,12.));
#113714=CARTESIAN_POINT('Ctrl Pts',(68.8266339174068,19.8757716696969,0.));
#113715=CARTESIAN_POINT('Ctrl Pts',(68.8266339174068,19.8757716696969,12.));
#113716=CARTESIAN_POINT('Ctrl Pts',(68.8456857484988,19.8892746776734,0.));
#113717=CARTESIAN_POINT('Ctrl Pts',(68.8456857484988,19.8892746776734,12.));
#113718=CARTESIAN_POINT('Ctrl Pts',(68.8647599395437,19.9028219146607,0.));
#113719=CARTESIAN_POINT('Ctrl Pts',(68.8647599395437,19.9028219146607,12.));
#113720=CARTESIAN_POINT('Ctrl Pts',(68.8838563494356,19.9164133594513,0.));
#113721=CARTESIAN_POINT('Ctrl Pts',(68.8838563494356,19.9164133594513,12.));
#113722=CARTESIAN_POINT('Ctrl Pts',(68.902974837704,19.9300489908364,0.));
#113723=CARTESIAN_POINT('Ctrl Pts',(68.902974837704,19.9300489908364,12.));
#113724=CARTESIAN_POINT('Ctrl Pts',(68.9221152645086,19.9437287876063,0.));
#113725=CARTESIAN_POINT('Ctrl Pts',(68.9221152645086,19.9437287876063,12.));
#113726=CARTESIAN_POINT('Ctrl Pts',(68.9412774906346,19.9574527285492,0.));
#113727=CARTESIAN_POINT('Ctrl Pts',(68.9412774906346,19.9574527285492,12.));
#113728=CARTESIAN_POINT('Ctrl Pts',(68.960461377483,19.9712207924437,0.));
#113729=CARTESIAN_POINT('Ctrl Pts',(68.960461377483,19.9712207924437,12.));
#113730=CARTESIAN_POINT('Ctrl Pts',(68.9796667870667,19.98503295806,0.));
#113731=CARTESIAN_POINT('Ctrl Pts',(68.9796667870667,19.98503295806,12.));
#113732=CARTESIAN_POINT('Ctrl Pts',(68.9988935820101,19.9988892041671,0.));
#113733=CARTESIAN_POINT('Ctrl Pts',(68.9988935820101,19.9988892041671,12.));
#113734=CARTESIAN_POINT('Ctrl Pts',(69.0181416255433,20.0127895095327,0.));
#113735=CARTESIAN_POINT('Ctrl Pts',(69.0181416255433,20.0127895095327,12.));
#113736=CARTESIAN_POINT('Ctrl Pts',(69.0374107814977,20.0267338529221,0.));
#113737=CARTESIAN_POINT('Ctrl Pts',(69.0374107814977,20.0267338529221,12.));
#113738=CARTESIAN_POINT('Ctrl Pts',(69.0567009142968,20.0407222130902,0.));
#113739=CARTESIAN_POINT('Ctrl Pts',(69.0567009142968,20.0407222130902,12.));
#113740=CARTESIAN_POINT('Ctrl Pts',(69.0760118889525,20.0547545687839,0.));
#113741=CARTESIAN_POINT('Ctrl Pts',(69.0760118889525,20.0547545687839,12.));
#113742=CARTESIAN_POINT('Ctrl Pts',(69.0953435710634,20.0688308987478,0.));
#113743=CARTESIAN_POINT('Ctrl Pts',(69.0953435710634,20.0688308987478,12.));
#113744=CARTESIAN_POINT('Ctrl Pts',(69.1146958268104,20.0829511817251,0.));
#113745=CARTESIAN_POINT('Ctrl Pts',(69.1146958268104,20.0829511817251,12.));
#113746=CARTESIAN_POINT('Ctrl Pts',(69.1340685229516,20.0971153964557,0.));
#113747=CARTESIAN_POINT('Ctrl Pts',(69.1340685229516,20.0971153964557,12.));
#113748=CARTESIAN_POINT('Ctrl Pts',(69.1534615268153,20.1113235216694,0.));
#113749=CARTESIAN_POINT('Ctrl Pts',(69.1534615268153,20.1113235216694,12.));
#113750=CARTESIAN_POINT('Ctrl Pts',(69.172874706296,20.1255755360871,0.));
#113751=CARTESIAN_POINT('Ctrl Pts',(69.172874706296,20.1255755360871,12.));
#113752=CARTESIAN_POINT('Ctrl Pts',(69.1923079298534,20.1398714184278,0.));
#113753=CARTESIAN_POINT('Ctrl Pts',(69.1923079298534,20.1398714184278,12.));
#113754=CARTESIAN_POINT('Ctrl Pts',(69.2117610665073,20.1542111474086,0.));
#113755=CARTESIAN_POINT('Ctrl Pts',(69.2117610665073,20.1542111474086,12.));
#113756=CARTESIAN_POINT('Ctrl Pts',(69.2312339858337,20.1685947017433,0.));
#113757=CARTESIAN_POINT('Ctrl Pts',(69.2312339858337,20.1685947017433,12.));
#113758=CARTESIAN_POINT('Ctrl Pts',(69.2507265579562,20.183022060135,0.));
#113759=CARTESIAN_POINT('Ctrl Pts',(69.2507265579562,20.183022060135,12.));
#113760=CARTESIAN_POINT('Ctrl Pts',(69.2702386535432,20.1974932012775,0.));
#113761=CARTESIAN_POINT('Ctrl Pts',(69.2702386535432,20.1974932012775,12.));
#113762=CARTESIAN_POINT('Ctrl Pts',(69.2897701438066,20.2120081038622,0.));
#113763=CARTESIAN_POINT('Ctrl Pts',(69.2897701438066,20.2120081038622,12.));
#113764=CARTESIAN_POINT('Ctrl Pts',(69.3093209004986,20.2265667465784,0.));
#113765=CARTESIAN_POINT('Ctrl Pts',(69.3093209004986,20.2265667465784,12.));
#113766=CARTESIAN_POINT('Ctrl Pts',(69.3288907959065,20.2411691081122,0.));
#113767=CARTESIAN_POINT('Ctrl Pts',(69.3288907959065,20.2411691081122,12.));
#113768=CARTESIAN_POINT('Ctrl Pts',(69.3484797028454,20.255815167139,0.));
#113769=CARTESIAN_POINT('Ctrl Pts',(69.3484797028454,20.255815167139,12.));
#113770=CARTESIAN_POINT('Ctrl Pts',(69.3680874946548,20.2705049023241,0.));
#113771=CARTESIAN_POINT('Ctrl Pts',(69.3680874946548,20.2705049023241,12.));
#113772=CARTESIAN_POINT('Ctrl Pts',(69.3877140451975,20.2852382923299,0.));
#113773=CARTESIAN_POINT('Ctrl Pts',(69.3877140451975,20.2852382923299,12.));
#113774=CARTESIAN_POINT('Ctrl Pts',(69.4073592288562,20.3000153158167,0.));
#113775=CARTESIAN_POINT('Ctrl Pts',(69.4073592288562,20.3000153158167,12.));
#113776=CARTESIAN_POINT('Ctrl Pts',(69.4270229205296,20.3148359514414,0.));
#113777=CARTESIAN_POINT('Ctrl Pts',(69.4270229205296,20.3148359514414,12.));
#113778=CARTESIAN_POINT('Ctrl Pts',(69.4467049956257,20.3297001778505,0.));
#113779=CARTESIAN_POINT('Ctrl Pts',(69.4467049956257,20.3297001778505,12.));
#113780=CARTESIAN_POINT('Ctrl Pts',(69.4664053300579,20.3446079736799,0.));
#113781=CARTESIAN_POINT('Ctrl Pts',(69.4664053300579,20.3446079736799,12.));
#113782=CARTESIAN_POINT('Ctrl Pts',(69.4861238002433,20.359559317562,0.));
#113783=CARTESIAN_POINT('Ctrl Pts',(69.4861238002433,20.359559317562,12.));
#113784=CARTESIAN_POINT('Ctrl Pts',(69.5058602831004,20.3745541881267,0.));
#113785=CARTESIAN_POINT('Ctrl Pts',(69.5058602831004,20.3745541881267,12.));
#113786=CARTESIAN_POINT('Ctrl Pts',(69.5256146560444,20.3895925640006,0.));
#113787=CARTESIAN_POINT('Ctrl Pts',(69.5256146560444,20.3895925640006,12.));
#113788=CARTESIAN_POINT('Ctrl Pts',(69.5453867969815,20.4046744238002,0.));
#113789=CARTESIAN_POINT('Ctrl Pts',(69.5453867969815,20.4046744238002,12.));
#113790=CARTESIAN_POINT('Ctrl Pts',(69.565176584305,20.4197997461306,0.));
#113791=CARTESIAN_POINT('Ctrl Pts',(69.565176584305,20.4197997461306,12.));
#113792=CARTESIAN_POINT('Ctrl Pts',(69.5849838968944,20.4349685095928,0.));
#113793=CARTESIAN_POINT('Ctrl Pts',(69.5849838968944,20.4349685095928,12.));
#113794=CARTESIAN_POINT('Ctrl Pts',(69.6048086141122,20.4501806927854,0.));
#113795=CARTESIAN_POINT('Ctrl Pts',(69.6048086141122,20.4501806927854,12.));
#113796=CARTESIAN_POINT('Ctrl Pts',(69.6246506158009,20.4654362743036,0.));
#113797=CARTESIAN_POINT('Ctrl Pts',(69.6246506158009,20.4654362743036,12.));
#113798=CARTESIAN_POINT('Ctrl Pts',(69.6445097822778,20.4807352327335,0.));
#113799=CARTESIAN_POINT('Ctrl Pts',(69.6445097822778,20.4807352327335,12.));
#113800=CARTESIAN_POINT('Ctrl Pts',(69.6643859943291,20.4960775466487,0.));
#113801=CARTESIAN_POINT('Ctrl Pts',(69.6643859943291,20.4960775466487,12.));
#113802=CARTESIAN_POINT('Ctrl Pts',(69.6842791332102,20.511463194618,0.));
#113803=CARTESIAN_POINT('Ctrl Pts',(69.6842791332102,20.511463194618,12.));
#113804=CARTESIAN_POINT('Ctrl Pts',(69.7041890806421,20.5268921552076,0.));
#113805=CARTESIAN_POINT('Ctrl Pts',(69.7041890806421,20.5268921552076,12.));
#113806=CARTESIAN_POINT('Ctrl Pts',(69.7241157188086,20.54236440698,0.));
#113807=CARTESIAN_POINT('Ctrl Pts',(69.7241157188086,20.54236440698,12.));
#113808=CARTESIAN_POINT('Ctrl Pts',(69.7440589303511,20.5578799284898,0.));
#113809=CARTESIAN_POINT('Ctrl Pts',(69.7440589303511,20.5578799284898,12.));
#113810=CARTESIAN_POINT('Ctrl Pts',(69.7640185983641,20.5734386982782,0.));
#113811=CARTESIAN_POINT('Ctrl Pts',(69.7640185983641,20.5734386982782,12.));
#113812=CARTESIAN_POINT('Ctrl Pts',(69.7839946063942,20.5890406948809,0.));
#113813=CARTESIAN_POINT('Ctrl Pts',(69.7839946063942,20.5890406948809,12.));
#113814=CARTESIAN_POINT('Ctrl Pts',(69.8039868384382,20.6046858968305,0.));
#113815=CARTESIAN_POINT('Ctrl Pts',(69.8039868384382,20.6046858968305,12.));
#113816=CARTESIAN_POINT('Ctrl Pts',(69.8239951789402,20.6203742826566,0.));
#113817=CARTESIAN_POINT('Ctrl Pts',(69.8239951789402,20.6203742826566,12.));
#113818=CARTESIAN_POINT('Ctrl Pts',(69.8440195127874,20.6361058308812,0.));
#113819=CARTESIAN_POINT('Ctrl Pts',(69.8440195127874,20.6361058308812,12.));
#113820=CARTESIAN_POINT('Ctrl Pts',(69.8640597253058,20.6518805200132,0.));
#113821=CARTESIAN_POINT('Ctrl Pts',(69.8640597253058,20.6518805200132,12.));
#113822=CARTESIAN_POINT('Ctrl Pts',(69.884115702258,20.6676983285542,0.));
#113823=CARTESIAN_POINT('Ctrl Pts',(69.884115702258,20.6676983285542,12.));
#113824=CARTESIAN_POINT('Ctrl Pts',(69.9041873298416,20.6835592350031,0.));
#113825=CARTESIAN_POINT('Ctrl Pts',(69.9041873298416,20.6835592350031,12.));
#113826=CARTESIAN_POINT('Ctrl Pts',(69.9242744946854,20.6994632178551,0.));
#113827=CARTESIAN_POINT('Ctrl Pts',(69.9242744946854,20.6994632178551,12.));
#113828=CARTESIAN_POINT('Ctrl Pts',(69.9443770838444,20.7154102555996,0.));
#113829=CARTESIAN_POINT('Ctrl Pts',(69.9443770838444,20.7154102555996,12.));
#113830=CARTESIAN_POINT('Ctrl Pts',(69.9644949847929,20.7314003267118,0.));
#113831=CARTESIAN_POINT('Ctrl Pts',(69.9644949847929,20.7314003267118,12.));
#113832=CARTESIAN_POINT('Ctrl Pts',(69.9846280854254,20.7474334096582,0.));
#113833=CARTESIAN_POINT('Ctrl Pts',(69.9846280854254,20.7474334096582,12.));
#113834=CARTESIAN_POINT('Ctrl Pts',(70.0047762740569,20.7635094829016,0.));
#113835=CARTESIAN_POINT('Ctrl Pts',(70.0047762740569,20.7635094829016,12.));
#113836=CARTESIAN_POINT('Ctrl Pts',(70.0249394394221,20.7796285249023,0.));
#113837=CARTESIAN_POINT('Ctrl Pts',(70.0249394394221,20.7796285249023,12.));
#113838=CARTESIAN_POINT('Ctrl Pts',(70.0451174706739,20.7957905141155,0.));
#113839=CARTESIAN_POINT('Ctrl Pts',(70.0451174706739,20.7957905141155,12.));
#113840=CARTESIAN_POINT('Ctrl Pts',(70.0653102573798,20.8119954289846,0.));
#113841=CARTESIAN_POINT('Ctrl Pts',(70.0653102573798,20.8119954289846,12.));
#113842=CARTESIAN_POINT('Ctrl Pts',(70.0855176895185,20.8282432479425,0.));
#113843=CARTESIAN_POINT('Ctrl Pts',(70.0855176895185,20.8282432479425,12.));
#113844=CARTESIAN_POINT('Ctrl Pts',(70.1057396574741,20.8445339494184,0.));
#113845=CARTESIAN_POINT('Ctrl Pts',(70.1057396574741,20.8445339494184,12.));
#113846=CARTESIAN_POINT('Ctrl Pts',(70.1259760520306,20.8608675118377,0.));
#113847=CARTESIAN_POINT('Ctrl Pts',(70.1259760520306,20.8608675118377,12.));
#113848=CARTESIAN_POINT('Ctrl Pts',(70.1462267643649,20.8772439136207,0.));
#113849=CARTESIAN_POINT('Ctrl Pts',(70.1462267643649,20.8772439136207,12.));
#113850=CARTESIAN_POINT('Ctrl Pts',(70.1664916860366,20.8936631331751,0.));
#113851=CARTESIAN_POINT('Ctrl Pts',(70.1664916860366,20.8936631331751,12.));
#113852=CARTESIAN_POINT('Ctrl Pts',(70.1867707089866,20.9101251488948,0.));
#113853=CARTESIAN_POINT('Ctrl Pts',(70.1867707089866,20.9101251488948,12.));
#113854=CARTESIAN_POINT('Ctrl Pts',(70.2070637255469,20.9266299391688,0.));
#113855=CARTESIAN_POINT('Ctrl Pts',(70.2070637255469,20.9266299391688,12.));
#113856=CARTESIAN_POINT('Ctrl Pts',(70.2273706284479,20.9431774823833,0.));
#113857=CARTESIAN_POINT('Ctrl Pts',(70.2273706284479,20.9431774823833,12.));
#113858=CARTESIAN_POINT('Ctrl Pts',(70.2476913108242,20.9597677569227,0.));
#113859=CARTESIAN_POINT('Ctrl Pts',(70.2476913108242,20.9597677569227,12.));
#113860=CARTESIAN_POINT('Ctrl Pts',(70.2680256662215,20.9764007411649,0.));
#113861=CARTESIAN_POINT('Ctrl Pts',(70.2680256662215,20.9764007411649,12.));
#113862=CARTESIAN_POINT('Ctrl Pts',(70.288373588597,20.993076413477,0.));
#113863=CARTESIAN_POINT('Ctrl Pts',(70.288373588597,20.993076413477,12.));
#113864=CARTESIAN_POINT('Ctrl Pts',(70.3087349722959,21.0097947522212,0.));
#113865=CARTESIAN_POINT('Ctrl Pts',(70.3087349722959,21.0097947522212,12.));
#113866=CARTESIAN_POINT('Ctrl Pts',(70.3291097120293,21.0265557357544,0.));
#113867=CARTESIAN_POINT('Ctrl Pts',(70.3291097120293,21.0265557357544,12.));
#113868=CARTESIAN_POINT('Ctrl Pts',(70.3494977028497,21.0433593424266,0.));
#113869=CARTESIAN_POINT('Ctrl Pts',(70.3494977028497,21.0433593424266,12.));
#113870=CARTESIAN_POINT('Ctrl Pts',(70.3698988401291,21.0602055505751,0.));
#113871=CARTESIAN_POINT('Ctrl Pts',(70.3698988401291,21.0602055505751,12.));
#113872=CARTESIAN_POINT('Ctrl Pts',(70.3903130195279,21.0770943385146,0.));
#113873=CARTESIAN_POINT('Ctrl Pts',(70.3903130195279,21.0770943385146,12.));
#113874=CARTESIAN_POINT('Ctrl Pts',(70.4107401370403,21.0940256845477,0.));
#113875=CARTESIAN_POINT('Ctrl Pts',(70.4107401370403,21.0940256845477,12.));
#113876=CARTESIAN_POINT('Ctrl Pts',(70.4311800890411,21.110999566975,0.));
#113877=CARTESIAN_POINT('Ctrl Pts',(70.4311800890411,21.110999566975,12.));
#113878=CARTESIAN_POINT('Ctrl Pts',(70.4516327723349,21.1280159641003,0.));
#113879=CARTESIAN_POINT('Ctrl Pts',(70.4516327723349,21.1280159641003,12.));
#113880=CARTESIAN_POINT('Ctrl Pts',(70.4720980841934,21.1450748542335,0.));
#113881=CARTESIAN_POINT('Ctrl Pts',(70.4720980841934,21.1450748542335,12.));
#113882=CARTESIAN_POINT('Ctrl Pts',(70.4925759224208,21.1621762156894,0.));
#113883=CARTESIAN_POINT('Ctrl Pts',(70.4925759224208,21.1621762156894,12.));
#113884=CARTESIAN_POINT('Ctrl Pts',(70.5130661852946,21.1793200267843,0.));
#113885=CARTESIAN_POINT('Ctrl Pts',(70.5130661852946,21.1793200267843,12.));
#113886=CARTESIAN_POINT('Ctrl Pts',(70.5335687714422,21.1965062658296,0.));
#113887=CARTESIAN_POINT('Ctrl Pts',(70.5335687714422,21.1965062658296,12.));
#113888=CARTESIAN_POINT('Ctrl Pts',(70.5540835797281,21.2137349111207,0.));
#113889=CARTESIAN_POINT('Ctrl Pts',(70.5540835797281,21.2137349111207,12.));
#113890=CARTESIAN_POINT('Ctrl Pts',(70.5746105091503,21.2310059409265,0.));
#113891=CARTESIAN_POINT('Ctrl Pts',(70.5746105091503,21.2310059409265,12.));
#113892=CARTESIAN_POINT('Ctrl Pts',(70.5951494586961,21.2483193334677,0.));
#113893=CARTESIAN_POINT('Ctrl Pts',(70.5951494586961,21.2483193334677,12.));
#113894=CARTESIAN_POINT('Ctrl Pts',(70.6157003273326,21.2656750669129,0.));
#113895=CARTESIAN_POINT('Ctrl Pts',(70.6157003273326,21.2656750669129,12.));
#113896=CARTESIAN_POINT('Ctrl Pts',(70.6362630143062,21.2830731194188,0.));
#113897=CARTESIAN_POINT('Ctrl Pts',(70.6362630143062,21.2830731194188,12.));
#113898=CARTESIAN_POINT('Ctrl Pts',(70.6568374193786,21.3005134691563,0.));
#113899=CARTESIAN_POINT('Ctrl Pts',(70.6568374193786,21.3005134691563,12.));
#113900=CARTESIAN_POINT('Ctrl Pts',(70.6774234430899,21.3179960943389,0.));
#113901=CARTESIAN_POINT('Ctrl Pts',(70.6774234430899,21.3179960943389,12.));
#113902=CARTESIAN_POINT('Ctrl Pts',(70.6980209870032,21.3355209732438,0.));
#113903=CARTESIAN_POINT('Ctrl Pts',(70.6980209870032,21.3355209732438,12.));
#113904=CARTESIAN_POINT('Ctrl Pts',(70.7186299539698,21.353088084234,0.));
#113905=CARTESIAN_POINT('Ctrl Pts',(70.7186299539698,21.353088084234,12.));
#113906=CARTESIAN_POINT('Ctrl Pts',(70.7392502475437,21.3706974057028,0.));
#113907=CARTESIAN_POINT('Ctrl Pts',(70.7392502475437,21.3706974057028,12.));
#113908=CARTESIAN_POINT('Ctrl Pts',(70.7598817714078,21.3883489160187,0.));
#113909=CARTESIAN_POINT('Ctrl Pts',(70.7598817714078,21.3883489160187,12.));
#113910=CARTESIAN_POINT('Ctrl Pts',(70.780524428744,21.4060425934595,0.));
#113911=CARTESIAN_POINT('Ctrl Pts',(70.780524428744,21.4060425934595,12.));
#113912=CARTESIAN_POINT('Ctrl Pts',(70.8011781217409,21.4237784161592,0.));
#113913=CARTESIAN_POINT('Ctrl Pts',(70.8011781217409,21.4237784161592,12.));
#113914=CARTESIAN_POINT('Ctrl Pts',(70.8218427507545,21.4415563620127,0.));
#113915=CARTESIAN_POINT('Ctrl Pts',(70.8218427507545,21.4415563620127,12.));
#113916=CARTESIAN_POINT('Ctrl Pts',(70.84251821499,21.4593764087492,0.));
#113917=CARTESIAN_POINT('Ctrl Pts',(70.84251821499,21.4593764087492,12.));
#113918=CARTESIAN_POINT('Ctrl Pts',(70.8632044140166,21.4772385340978,0.));
#113919=CARTESIAN_POINT('Ctrl Pts',(70.8632044140166,21.4772385340978,12.));
#113920=CARTESIAN_POINT('Ctrl Pts',(70.8839012490903,21.4951427159272,0.));
#113921=CARTESIAN_POINT('Ctrl Pts',(70.8839012490903,21.4951427159272,12.));
#113922=CARTESIAN_POINT('Ctrl Pts',(70.9046086244123,21.5130889323767,0.));
#113923=CARTESIAN_POINT('Ctrl Pts',(70.9046086244123,21.5130889323767,12.));
#113924=CARTESIAN_POINT('Ctrl Pts',(70.9253264487576,21.5310771620209,0.));
#113925=CARTESIAN_POINT('Ctrl Pts',(70.9253264487576,21.5310771620209,12.));
#113926=CARTESIAN_POINT('Ctrl Pts',(70.9460546358597,21.549107383907,0.));
#113927=CARTESIAN_POINT('Ctrl Pts',(70.9460546358597,21.549107383907,12.));
#113928=CARTESIAN_POINT('Ctrl Pts',(70.9667931008097,21.5671795771873,0.));
#113929=CARTESIAN_POINT('Ctrl Pts',(70.9667931008097,21.5671795771873,12.));
#113930=CARTESIAN_POINT('Ctrl Pts',(70.9875417572138,21.5852937208258,0.));
#113931=CARTESIAN_POINT('Ctrl Pts',(70.9875417572138,21.5852937208258,12.));
#113932=CARTESIAN_POINT('Ctrl Pts',(71.0083005139086,21.6034497932574,0.));
#113933=CARTESIAN_POINT('Ctrl Pts',(71.0083005139086,21.6034497932574,12.));
#113934=CARTESIAN_POINT('Ctrl Pts',(71.0290692721932,21.6216477720941,0.));
#113935=CARTESIAN_POINT('Ctrl Pts',(71.0290692721932,21.6216477720941,12.));
#113936=CARTESIAN_POINT('Ctrl Pts',(71.0498479219659,21.6398876337207,0.));
#113937=CARTESIAN_POINT('Ctrl Pts',(71.0498479219659,21.6398876337207,12.));
#113938=CARTESIAN_POINT('Ctrl Pts',(71.0706363472965,21.6581693538424,0.));
#113939=CARTESIAN_POINT('Ctrl Pts',(71.0706363472965,21.6581693538424,12.));
#113940=CARTESIAN_POINT('Ctrl Pts',(71.0914344333048,21.6764929081762,0.));
#113941=CARTESIAN_POINT('Ctrl Pts',(71.0914344333048,21.6764929081762,12.));
#113942=CARTESIAN_POINT('Ctrl Pts',(71.1122420728349,21.6948582730895,0.));
#113943=CARTESIAN_POINT('Ctrl Pts',(71.1122420728349,21.6948582730895,12.));
#113944=CARTESIAN_POINT('Ctrl Pts',(71.133059172642,21.7132654262501,0.));
#113945=CARTESIAN_POINT('Ctrl Pts',(71.133059172642,21.7132654262501,12.));
#113946=CARTESIAN_POINT('Ctrl Pts',(71.1538856611899,21.7317143472827,0.));
#113947=CARTESIAN_POINT('Ctrl Pts',(71.1538856611899,21.7317143472827,12.));
#113948=CARTESIAN_POINT('Ctrl Pts',(71.1747214905981,21.7502050183602,0.));
#113949=CARTESIAN_POINT('Ctrl Pts',(71.1747214905981,21.7502050183602,12.));
#113950=CARTESIAN_POINT('Ctrl Pts',(71.1955666309591,21.7687374247046,0.));
#113951=CARTESIAN_POINT('Ctrl Pts',(71.1955666309591,21.7687374247046,12.));
#113952=CARTESIAN_POINT('Ctrl Pts',(71.212250179455,21.7835967290261,0.));
#113953=CARTESIAN_POINT('Ctrl Pts',(71.212250179455,21.7835967290261,12.));
#113954=CARTESIAN_POINT('Ctrl Pts',(71.2247670209821,21.7947599798839,0.));
#113955=CARTESIAN_POINT('Ctrl Pts',(71.2247670209821,21.7947599798839,12.));
#113956=CARTESIAN_POINT('Ctrl Pts',(71.2331134397743,21.8022104901682,0.));
#113957=CARTESIAN_POINT('Ctrl Pts',(71.2331134397743,21.8022104901682,12.));
#113958=CARTESIAN_POINT('Ctrl Pts',(71.2372871136137,21.8059378310719,0.));
#113959=CARTESIAN_POINT('Ctrl Pts',(71.2372871136137,21.8059378310719,12.));
#113960=CARTESIAN_POINT('',(67.3887914263118,18.9407177820969,0.));
#113961=CARTESIAN_POINT('Ctrl Pts',(67.3887914263118,18.9407177820969,0.));
#113962=CARTESIAN_POINT('Ctrl Pts',(67.3921355608328,18.9426924398719,0.));
#113963=CARTESIAN_POINT('Ctrl Pts',(67.3988274146651,18.9466463414299,0.));
#113964=CARTESIAN_POINT('Ctrl Pts',(67.4088759497911,18.9525909517915,0.));
#113965=CARTESIAN_POINT('Ctrl Pts',(67.4222955061981,18.9605446160985,0.));
#113966=CARTESIAN_POINT('Ctrl Pts',(67.4391057908418,18.9705325631711,0.));
#113967=CARTESIAN_POINT('Ctrl Pts',(67.4559518744638,18.9805663798449,0.));
#113968=CARTESIAN_POINT('Ctrl Pts',(67.472833671964,18.9906460638625,0.));
#113969=CARTESIAN_POINT('Ctrl Pts',(67.4897510316844,19.0007716032819,0.));
#113970=CARTESIAN_POINT('Ctrl Pts',(67.5067037372317,19.0109429761306,0.));
#113971=CARTESIAN_POINT('Ctrl Pts',(67.5236915360331,19.021160154824,0.));
#113972=CARTESIAN_POINT('Ctrl Pts',(67.540714161288,19.0314231093923,0.));
#113973=CARTESIAN_POINT('Ctrl Pts',(67.5577713558194,19.0417318110708,0.));
#113974=CARTESIAN_POINT('Ctrl Pts',(67.5748628971964,19.0520862360396,0.));
#113975=CARTESIAN_POINT('Ctrl Pts',(67.5919885896222,19.062486364241,0.));
#113976=CARTESIAN_POINT('Ctrl Pts',(67.6091482520534,19.072932177628,0.));
#113977=CARTESIAN_POINT('Ctrl Pts',(67.6263417083426,19.0834236587118,0.));
#113978=CARTESIAN_POINT('Ctrl Pts',(67.6435687749841,19.0939607887502,0.));
#113979=CARTESIAN_POINT('Ctrl Pts',(67.6608292549462,19.1045435468358,0.));
#113980=CARTESIAN_POINT('Ctrl Pts',(67.6781229440573,19.115171910846,0.));
#113981=CARTESIAN_POINT('Ctrl Pts',(67.6954496350063,19.1258458580345,0.));
#113982=CARTESIAN_POINT('Ctrl Pts',(67.7128091219348,19.136565365709,0.));
#113983=CARTESIAN_POINT('Ctrl Pts',(67.7302012056584,19.1473304119955,0.));
#113984=CARTESIAN_POINT('Ctrl Pts',(67.7476256934444,19.1581409758097,0.));
#113985=CARTESIAN_POINT('Ctrl Pts',(67.7650823965127,19.168997036495,0.));
#113986=CARTESIAN_POINT('Ctrl Pts',(67.7825711283096,19.1798985735688,0.));
#113987=CARTESIAN_POINT('Ctrl Pts',(67.8000917023926,19.1908455664098,0.));
#113988=CARTESIAN_POINT('Ctrl Pts',(67.8176439306621,19.201837993993,0.));
#113989=CARTESIAN_POINT('Ctrl Pts',(67.835227624289,19.2128758350346,0.));
#113990=CARTESIAN_POINT('Ctrl Pts',(67.8528425945184,19.2239590681133,0.));
#113991=CARTESIAN_POINT('Ctrl Pts',(67.8704886534544,19.2350876717874,0.));
#113992=CARTESIAN_POINT('Ctrl Pts',(67.8881656149955,19.2462616247279,0.));
#113993=CARTESIAN_POINT('Ctrl Pts',(67.9058732951788,19.2574809057696,0.));
#113994=CARTESIAN_POINT('Ctrl Pts',(67.9236115116758,19.2687454938442,0.));
#113995=CARTESIAN_POINT('Ctrl Pts',(67.9413800834793,19.280055367936,0.));
#113996=CARTESIAN_POINT('Ctrl Pts',(67.9591788305394,19.2914105070286,0.));
#113997=CARTESIAN_POINT('Ctrl Pts',(67.9770075733485,19.302810890038,0.));
#113998=CARTESIAN_POINT('Ctrl Pts',(67.9948661329617,19.3142564958203,0.));
#113999=CARTESIAN_POINT('Ctrl Pts',(68.0127543311776,19.3257473032035,0.));
#114000=CARTESIAN_POINT('Ctrl Pts',(68.0306719906636,19.3372832910076,0.));
#114001=CARTESIAN_POINT('Ctrl Pts',(68.0486189351011,19.3488644380641,0.));
#114002=CARTESIAN_POINT('Ctrl Pts',(68.0665949893195,19.3604907232314,0.));
#114003=CARTESIAN_POINT('Ctrl Pts',(68.0845999792247,19.3721621253912,0.));
#114004=CARTESIAN_POINT('Ctrl Pts',(68.1026337317285,19.3838786234421,0.));
#114005=CARTESIAN_POINT('Ctrl Pts',(68.1206960746769,19.3956401962895,0.));
#114006=CARTESIAN_POINT('Ctrl Pts',(68.1387868367691,19.40744682283,0.));
#114007=CARTESIAN_POINT('Ctrl Pts',(68.1569058475054,19.4192984819418,0.));
#114008=CARTESIAN_POINT('Ctrl Pts',(68.1750529372232,19.4311951524983,0.));
#114009=CARTESIAN_POINT('Ctrl Pts',(68.1932279371127,19.4431368133719,0.));
#114010=CARTESIAN_POINT('Ctrl Pts',(68.2114306792358,19.4551234434381,0.));
#114011=CARTESIAN_POINT('Ctrl Pts',(68.2296609965448,19.467155021572,0.));
#114012=CARTESIAN_POINT('Ctrl Pts',(68.2479187228803,19.4792315266501,0.));
#114013=CARTESIAN_POINT('Ctrl Pts',(68.2662036929526,19.4913529375543,0.));
#114014=CARTESIAN_POINT('Ctrl Pts',(68.2845157423233,19.5035192331705,0.));
#114015=CARTESIAN_POINT('Ctrl Pts',(68.3028547073864,19.5157303923856,0.));
#114016=CARTESIAN_POINT('Ctrl Pts',(68.3212204253417,19.5279863940773,0.));
#114017=CARTESIAN_POINT('Ctrl Pts',(68.3396127341938,19.5402872171191,0.));
#114018=CARTESIAN_POINT('Ctrl Pts',(68.3580314727523,19.5526328403852,0.));
#114019=CARTESIAN_POINT('Ctrl Pts',(68.3764764806287,19.5650232427516,0.));
#114020=CARTESIAN_POINT('Ctrl Pts',(68.3949475982335,19.5774584030938,0.));
#114021=CARTESIAN_POINT('Ctrl Pts',(68.4134446667696,19.5899383002803,0.));
#114022=CARTESIAN_POINT('Ctrl Pts',(68.4319675282275,19.6024629131785,0.));
#114023=CARTESIAN_POINT('Ctrl Pts',(68.4505160253778,19.6150322206577,0.));
#114024=CARTESIAN_POINT('Ctrl Pts',(68.4690900017632,19.6276462015888,0.));
#114025=CARTESIAN_POINT('Ctrl Pts',(68.4876893016856,19.6403048348395,0.));
#114026=CARTESIAN_POINT('Ctrl Pts',(68.5063137701971,19.6530080992686,0.));
#114027=CARTESIAN_POINT('Ctrl Pts',(68.5249632530979,19.6657559737336,0.));
#114028=CARTESIAN_POINT('Ctrl Pts',(68.5436375969311,19.6785484370927,0.));
#114029=CARTESIAN_POINT('Ctrl Pts',(68.5623366489779,19.6913854682046,0.));
#114030=CARTESIAN_POINT('Ctrl Pts',(68.581060257249,19.7042670459237,0.));
#114031=CARTESIAN_POINT('Ctrl Pts',(68.5998082704766,19.7171931490956,0.));
#114032=CARTESIAN_POINT('Ctrl Pts',(68.6185805381126,19.7301637565652,0.));
#114033=CARTESIAN_POINT('Ctrl Pts',(68.6373769103224,19.7431788471776,0.));
#114034=CARTESIAN_POINT('Ctrl Pts',(68.6561972379793,19.7562383997781,0.));
#114035=CARTESIAN_POINT('Ctrl Pts',(68.6750413726547,19.7693423932058,0.));
#114036=CARTESIAN_POINT('Ctrl Pts',(68.6939091666111,19.7824908062913,0.));
#114037=CARTESIAN_POINT('Ctrl Pts',(68.7128004727998,19.795683617864,0.));
#114038=CARTESIAN_POINT('Ctrl Pts',(68.7317151448557,19.8089208067532,0.));
#114039=CARTESIAN_POINT('Ctrl Pts',(68.7506530370918,19.8222023517874,0.));
#114040=CARTESIAN_POINT('Ctrl Pts',(68.7696140044892,19.835528231787,0.));
#114041=CARTESIAN_POINT('Ctrl Pts',(68.7885979026927,19.8488984255641,0.));
#114042=CARTESIAN_POINT('Ctrl Pts',(68.8076045880102,19.8623129119304,0.));
#114043=CARTESIAN_POINT('Ctrl Pts',(68.8266339174068,19.8757716696969,0.));
#114044=CARTESIAN_POINT('Ctrl Pts',(68.8456857484988,19.8892746776734,0.));
#114045=CARTESIAN_POINT('Ctrl Pts',(68.8647599395437,19.9028219146607,0.));
#114046=CARTESIAN_POINT('Ctrl Pts',(68.8838563494356,19.9164133594513,0.));
#114047=CARTESIAN_POINT('Ctrl Pts',(68.902974837704,19.9300489908364,0.));
#114048=CARTESIAN_POINT('Ctrl Pts',(68.9221152645086,19.9437287876063,0.));
#114049=CARTESIAN_POINT('Ctrl Pts',(68.9412774906346,19.9574527285492,0.));
#114050=CARTESIAN_POINT('Ctrl Pts',(68.960461377483,19.9712207924437,0.));
#114051=CARTESIAN_POINT('Ctrl Pts',(68.9796667870667,19.98503295806,0.));
#114052=CARTESIAN_POINT('Ctrl Pts',(68.9988935820101,19.9988892041671,0.));
#114053=CARTESIAN_POINT('Ctrl Pts',(69.0181416255433,20.0127895095327,0.));
#114054=CARTESIAN_POINT('Ctrl Pts',(69.0374107814977,20.0267338529221,0.));
#114055=CARTESIAN_POINT('Ctrl Pts',(69.0567009142968,20.0407222130902,0.));
#114056=CARTESIAN_POINT('Ctrl Pts',(69.0760118889525,20.0547545687839,0.));
#114057=CARTESIAN_POINT('Ctrl Pts',(69.0953435710634,20.0688308987478,0.));
#114058=CARTESIAN_POINT('Ctrl Pts',(69.1146958268104,20.0829511817251,0.));
#114059=CARTESIAN_POINT('Ctrl Pts',(69.1340685229516,20.0971153964557,0.));
#114060=CARTESIAN_POINT('Ctrl Pts',(69.1534615268153,20.1113235216694,0.));
#114061=CARTESIAN_POINT('Ctrl Pts',(69.172874706296,20.1255755360871,0.));
#114062=CARTESIAN_POINT('Ctrl Pts',(69.1923079298534,20.1398714184278,0.));
#114063=CARTESIAN_POINT('Ctrl Pts',(69.2117610665073,20.1542111474086,0.));
#114064=CARTESIAN_POINT('Ctrl Pts',(69.2312339858337,20.1685947017433,0.));
#114065=CARTESIAN_POINT('Ctrl Pts',(69.2507265579562,20.183022060135,0.));
#114066=CARTESIAN_POINT('Ctrl Pts',(69.2702386535432,20.1974932012775,0.));
#114067=CARTESIAN_POINT('Ctrl Pts',(69.2897701438066,20.2120081038622,0.));
#114068=CARTESIAN_POINT('Ctrl Pts',(69.3093209004986,20.2265667465784,0.));
#114069=CARTESIAN_POINT('Ctrl Pts',(69.3288907959065,20.2411691081122,0.));
#114070=CARTESIAN_POINT('Ctrl Pts',(69.3484797028454,20.255815167139,0.));
#114071=CARTESIAN_POINT('Ctrl Pts',(69.3680874946548,20.2705049023241,0.));
#114072=CARTESIAN_POINT('Ctrl Pts',(69.3877140451975,20.2852382923299,0.));
#114073=CARTESIAN_POINT('Ctrl Pts',(69.4073592288562,20.3000153158167,0.));
#114074=CARTESIAN_POINT('Ctrl Pts',(69.4270229205296,20.3148359514414,0.));
#114075=CARTESIAN_POINT('Ctrl Pts',(69.4467049956257,20.3297001778505,0.));
#114076=CARTESIAN_POINT('Ctrl Pts',(69.4664053300579,20.3446079736799,0.));
#114077=CARTESIAN_POINT('Ctrl Pts',(69.4861238002433,20.359559317562,0.));
#114078=CARTESIAN_POINT('Ctrl Pts',(69.5058602831004,20.3745541881267,0.));
#114079=CARTESIAN_POINT('Ctrl Pts',(69.5256146560444,20.3895925640006,0.));
#114080=CARTESIAN_POINT('Ctrl Pts',(69.5453867969815,20.4046744238002,0.));
#114081=CARTESIAN_POINT('Ctrl Pts',(69.565176584305,20.4197997461306,0.));
#114082=CARTESIAN_POINT('Ctrl Pts',(69.5849838968944,20.4349685095928,0.));
#114083=CARTESIAN_POINT('Ctrl Pts',(69.6048086141122,20.4501806927854,0.));
#114084=CARTESIAN_POINT('Ctrl Pts',(69.6246506158009,20.4654362743036,0.));
#114085=CARTESIAN_POINT('Ctrl Pts',(69.6445097822778,20.4807352327335,0.));
#114086=CARTESIAN_POINT('Ctrl Pts',(69.6643859943291,20.4960775466487,0.));
#114087=CARTESIAN_POINT('Ctrl Pts',(69.6842791332102,20.511463194618,0.));
#114088=CARTESIAN_POINT('Ctrl Pts',(69.7041890806421,20.5268921552076,0.));
#114089=CARTESIAN_POINT('Ctrl Pts',(69.7241157188086,20.54236440698,0.));
#114090=CARTESIAN_POINT('Ctrl Pts',(69.7440589303511,20.5578799284898,0.));
#114091=CARTESIAN_POINT('Ctrl Pts',(69.7640185983641,20.5734386982782,0.));
#114092=CARTESIAN_POINT('Ctrl Pts',(69.7839946063942,20.5890406948809,0.));
#114093=CARTESIAN_POINT('Ctrl Pts',(69.8039868384382,20.6046858968305,0.));
#114094=CARTESIAN_POINT('Ctrl Pts',(69.8239951789402,20.6203742826566,0.));
#114095=CARTESIAN_POINT('Ctrl Pts',(69.8440195127874,20.6361058308812,0.));
#114096=CARTESIAN_POINT('Ctrl Pts',(69.8640597253058,20.6518805200132,0.));
#114097=CARTESIAN_POINT('Ctrl Pts',(69.884115702258,20.6676983285542,0.));
#114098=CARTESIAN_POINT('Ctrl Pts',(69.9041873298416,20.6835592350031,0.));
#114099=CARTESIAN_POINT('Ctrl Pts',(69.9242744946854,20.6994632178551,0.));
#114100=CARTESIAN_POINT('Ctrl Pts',(69.9443770838444,20.7154102555996,0.));
#114101=CARTESIAN_POINT('Ctrl Pts',(69.9644949847929,20.7314003267118,0.));
#114102=CARTESIAN_POINT('Ctrl Pts',(69.9846280854254,20.7474334096582,0.));
#114103=CARTESIAN_POINT('Ctrl Pts',(70.0047762740569,20.7635094829016,0.));
#114104=CARTESIAN_POINT('Ctrl Pts',(70.0249394394221,20.7796285249023,0.));
#114105=CARTESIAN_POINT('Ctrl Pts',(70.0451174706739,20.7957905141155,0.));
#114106=CARTESIAN_POINT('Ctrl Pts',(70.0653102573798,20.8119954289846,0.));
#114107=CARTESIAN_POINT('Ctrl Pts',(70.0855176895185,20.8282432479425,0.));
#114108=CARTESIAN_POINT('Ctrl Pts',(70.1057396574741,20.8445339494184,0.));
#114109=CARTESIAN_POINT('Ctrl Pts',(70.1259760520306,20.8608675118377,0.));
#114110=CARTESIAN_POINT('Ctrl Pts',(70.1462267643649,20.8772439136207,0.));
#114111=CARTESIAN_POINT('Ctrl Pts',(70.1664916860366,20.8936631331751,0.));
#114112=CARTESIAN_POINT('Ctrl Pts',(70.1867707089866,20.9101251488948,0.));
#114113=CARTESIAN_POINT('Ctrl Pts',(70.2070637255469,20.9266299391688,0.));
#114114=CARTESIAN_POINT('Ctrl Pts',(70.2273706284479,20.9431774823833,0.));
#114115=CARTESIAN_POINT('Ctrl Pts',(70.2476913108242,20.9597677569227,0.));
#114116=CARTESIAN_POINT('Ctrl Pts',(70.2680256662215,20.9764007411649,0.));
#114117=CARTESIAN_POINT('Ctrl Pts',(70.288373588597,20.993076413477,0.));
#114118=CARTESIAN_POINT('Ctrl Pts',(70.3087349722959,21.0097947522212,0.));
#114119=CARTESIAN_POINT('Ctrl Pts',(70.3291097120293,21.0265557357544,0.));
#114120=CARTESIAN_POINT('Ctrl Pts',(70.3494977028497,21.0433593424266,0.));
#114121=CARTESIAN_POINT('Ctrl Pts',(70.3698988401291,21.0602055505751,0.));
#114122=CARTESIAN_POINT('Ctrl Pts',(70.3903130195279,21.0770943385146,0.));
#114123=CARTESIAN_POINT('Ctrl Pts',(70.4107401370403,21.0940256845477,0.));
#114124=CARTESIAN_POINT('Ctrl Pts',(70.4311800890411,21.110999566975,0.));
#114125=CARTESIAN_POINT('Ctrl Pts',(70.4516327723349,21.1280159641003,0.));
#114126=CARTESIAN_POINT('Ctrl Pts',(70.4720980841934,21.1450748542335,0.));
#114127=CARTESIAN_POINT('Ctrl Pts',(70.4925759224208,21.1621762156894,0.));
#114128=CARTESIAN_POINT('Ctrl Pts',(70.5130661852946,21.1793200267843,0.));
#114129=CARTESIAN_POINT('Ctrl Pts',(70.5335687714422,21.1965062658296,0.));
#114130=CARTESIAN_POINT('Ctrl Pts',(70.5540835797281,21.2137349111207,0.));
#114131=CARTESIAN_POINT('Ctrl Pts',(70.5746105091503,21.2310059409265,0.));
#114132=CARTESIAN_POINT('Ctrl Pts',(70.5951494586961,21.2483193334677,0.));
#114133=CARTESIAN_POINT('Ctrl Pts',(70.6157003273326,21.2656750669129,0.));
#114134=CARTESIAN_POINT('Ctrl Pts',(70.6362630143062,21.2830731194188,0.));
#114135=CARTESIAN_POINT('Ctrl Pts',(70.6568374193786,21.3005134691563,0.));
#114136=CARTESIAN_POINT('Ctrl Pts',(70.6774234430899,21.3179960943389,0.));
#114137=CARTESIAN_POINT('Ctrl Pts',(70.6980209870032,21.3355209732438,0.));
#114138=CARTESIAN_POINT('Ctrl Pts',(70.7186299539698,21.353088084234,0.));
#114139=CARTESIAN_POINT('Ctrl Pts',(70.7392502475437,21.3706974057028,0.));
#114140=CARTESIAN_POINT('Ctrl Pts',(70.7598817714078,21.3883489160187,0.));
#114141=CARTESIAN_POINT('Ctrl Pts',(70.780524428744,21.4060425934595,0.));
#114142=CARTESIAN_POINT('Ctrl Pts',(70.8011781217409,21.4237784161592,0.));
#114143=CARTESIAN_POINT('Ctrl Pts',(70.8218427507545,21.4415563620127,0.));
#114144=CARTESIAN_POINT('Ctrl Pts',(70.84251821499,21.4593764087492,0.));
#114145=CARTESIAN_POINT('Ctrl Pts',(70.8632044140166,21.4772385340978,0.));
#114146=CARTESIAN_POINT('Ctrl Pts',(70.8839012490903,21.4951427159272,0.));
#114147=CARTESIAN_POINT('Ctrl Pts',(70.9046086244123,21.5130889323767,0.));
#114148=CARTESIAN_POINT('Ctrl Pts',(70.9253264487576,21.5310771620209,0.));
#114149=CARTESIAN_POINT('Ctrl Pts',(70.9460546358597,21.549107383907,0.));
#114150=CARTESIAN_POINT('Ctrl Pts',(70.9638315189647,21.5645987555282,0.));
#114151=CARTESIAN_POINT('Ctrl Pts',(70.9774662112376,21.576498336635,0.));
#114152=CARTESIAN_POINT('Ctrl Pts',(70.9869541807808,21.584787543316,0.));
#114153=CARTESIAN_POINT('Ctrl Pts',(70.9922924595081,21.5894540925369,0.));
#114154=CARTESIAN_POINT('Ctrl Pts',(70.9934796068777,21.59049199348,0.));
#114155=CARTESIAN_POINT('',(67.3887914263118,18.9407177820969,12.));
#114156=CARTESIAN_POINT('',(67.3887914263118,18.9407177820969,0.));
#114157=CARTESIAN_POINT('Ctrl Pts',(70.9934796068777,21.59049199348,12.));
#114158=CARTESIAN_POINT('Ctrl Pts',(70.9922924595081,21.5894540925369,12.));
#114159=CARTESIAN_POINT('Ctrl Pts',(70.9869541807808,21.584787543316,12.));
#114160=CARTESIAN_POINT('Ctrl Pts',(70.9774662112376,21.576498336635,12.));
#114161=CARTESIAN_POINT('Ctrl Pts',(70.9638315189647,21.5645987555282,12.));
#114162=CARTESIAN_POINT('Ctrl Pts',(70.9460546358597,21.549107383907,12.));
#114163=CARTESIAN_POINT('Ctrl Pts',(70.9253264487576,21.5310771620209,12.));
#114164=CARTESIAN_POINT('Ctrl Pts',(70.9046086244123,21.5130889323767,12.));
#114165=CARTESIAN_POINT('Ctrl Pts',(70.8839012490903,21.4951427159272,12.));
#114166=CARTESIAN_POINT('Ctrl Pts',(70.8632044140166,21.4772385340978,12.));
#114167=CARTESIAN_POINT('Ctrl Pts',(70.84251821499,21.4593764087492,12.));
#114168=CARTESIAN_POINT('Ctrl Pts',(70.8218427507545,21.4415563620127,12.));
#114169=CARTESIAN_POINT('Ctrl Pts',(70.8011781217409,21.4237784161592,12.));
#114170=CARTESIAN_POINT('Ctrl Pts',(70.780524428744,21.4060425934595,12.));
#114171=CARTESIAN_POINT('Ctrl Pts',(70.7598817714078,21.3883489160187,12.));
#114172=CARTESIAN_POINT('Ctrl Pts',(70.7392502475437,21.3706974057028,12.));
#114173=CARTESIAN_POINT('Ctrl Pts',(70.7186299539698,21.353088084234,12.));
#114174=CARTESIAN_POINT('Ctrl Pts',(70.6980209870032,21.3355209732438,12.));
#114175=CARTESIAN_POINT('Ctrl Pts',(70.6774234430899,21.3179960943389,12.));
#114176=CARTESIAN_POINT('Ctrl Pts',(70.6568374193786,21.3005134691563,12.));
#114177=CARTESIAN_POINT('Ctrl Pts',(70.6362630143062,21.2830731194188,12.));
#114178=CARTESIAN_POINT('Ctrl Pts',(70.6157003273326,21.2656750669129,12.));
#114179=CARTESIAN_POINT('Ctrl Pts',(70.5951494586961,21.2483193334677,12.));
#114180=CARTESIAN_POINT('Ctrl Pts',(70.5746105091503,21.2310059409265,12.));
#114181=CARTESIAN_POINT('Ctrl Pts',(70.5540835797281,21.2137349111207,12.));
#114182=CARTESIAN_POINT('Ctrl Pts',(70.5335687714422,21.1965062658296,12.));
#114183=CARTESIAN_POINT('Ctrl Pts',(70.5130661852946,21.1793200267843,12.));
#114184=CARTESIAN_POINT('Ctrl Pts',(70.4925759224208,21.1621762156894,12.));
#114185=CARTESIAN_POINT('Ctrl Pts',(70.4720980841934,21.1450748542335,12.));
#114186=CARTESIAN_POINT('Ctrl Pts',(70.4516327723349,21.1280159641003,12.));
#114187=CARTESIAN_POINT('Ctrl Pts',(70.4311800890411,21.110999566975,12.));
#114188=CARTESIAN_POINT('Ctrl Pts',(70.4107401370403,21.0940256845477,12.));
#114189=CARTESIAN_POINT('Ctrl Pts',(70.3903130195279,21.0770943385146,12.));
#114190=CARTESIAN_POINT('Ctrl Pts',(70.3698988401291,21.0602055505751,12.));
#114191=CARTESIAN_POINT('Ctrl Pts',(70.3494977028497,21.0433593424266,12.));
#114192=CARTESIAN_POINT('Ctrl Pts',(70.3291097120293,21.0265557357544,12.));
#114193=CARTESIAN_POINT('Ctrl Pts',(70.3087349722959,21.0097947522212,12.));
#114194=CARTESIAN_POINT('Ctrl Pts',(70.288373588597,20.993076413477,12.));
#114195=CARTESIAN_POINT('Ctrl Pts',(70.2680256662215,20.9764007411649,12.));
#114196=CARTESIAN_POINT('Ctrl Pts',(70.2476913108242,20.9597677569227,12.));
#114197=CARTESIAN_POINT('Ctrl Pts',(70.2273706284479,20.9431774823833,12.));
#114198=CARTESIAN_POINT('Ctrl Pts',(70.2070637255469,20.9266299391688,12.));
#114199=CARTESIAN_POINT('Ctrl Pts',(70.1867707089866,20.9101251488948,12.));
#114200=CARTESIAN_POINT('Ctrl Pts',(70.1664916860366,20.8936631331751,12.));
#114201=CARTESIAN_POINT('Ctrl Pts',(70.1462267643649,20.8772439136207,12.));
#114202=CARTESIAN_POINT('Ctrl Pts',(70.1259760520306,20.8608675118377,12.));
#114203=CARTESIAN_POINT('Ctrl Pts',(70.1057396574741,20.8445339494184,12.));
#114204=CARTESIAN_POINT('Ctrl Pts',(70.0855176895185,20.8282432479425,12.));
#114205=CARTESIAN_POINT('Ctrl Pts',(70.0653102573798,20.8119954289846,12.));
#114206=CARTESIAN_POINT('Ctrl Pts',(70.0451174706739,20.7957905141155,12.));
#114207=CARTESIAN_POINT('Ctrl Pts',(70.0249394394221,20.7796285249023,12.));
#114208=CARTESIAN_POINT('Ctrl Pts',(70.0047762740569,20.7635094829016,12.));
#114209=CARTESIAN_POINT('Ctrl Pts',(69.9846280854254,20.7474334096582,12.));
#114210=CARTESIAN_POINT('Ctrl Pts',(69.9644949847929,20.7314003267118,12.));
#114211=CARTESIAN_POINT('Ctrl Pts',(69.9443770838444,20.7154102555996,12.));
#114212=CARTESIAN_POINT('Ctrl Pts',(69.9242744946854,20.6994632178551,12.));
#114213=CARTESIAN_POINT('Ctrl Pts',(69.9041873298416,20.6835592350031,12.));
#114214=CARTESIAN_POINT('Ctrl Pts',(69.884115702258,20.6676983285542,12.));
#114215=CARTESIAN_POINT('Ctrl Pts',(69.8640597253058,20.6518805200132,12.));
#114216=CARTESIAN_POINT('Ctrl Pts',(69.8440195127874,20.6361058308812,12.));
#114217=CARTESIAN_POINT('Ctrl Pts',(69.8239951789402,20.6203742826566,12.));
#114218=CARTESIAN_POINT('Ctrl Pts',(69.8039868384382,20.6046858968305,12.));
#114219=CARTESIAN_POINT('Ctrl Pts',(69.7839946063942,20.5890406948809,12.));
#114220=CARTESIAN_POINT('Ctrl Pts',(69.7640185983641,20.5734386982782,12.));
#114221=CARTESIAN_POINT('Ctrl Pts',(69.7440589303511,20.5578799284898,12.));
#114222=CARTESIAN_POINT('Ctrl Pts',(69.7241157188086,20.54236440698,12.));
#114223=CARTESIAN_POINT('Ctrl Pts',(69.7041890806421,20.5268921552076,12.));
#114224=CARTESIAN_POINT('Ctrl Pts',(69.6842791332102,20.511463194618,12.));
#114225=CARTESIAN_POINT('Ctrl Pts',(69.6643859943291,20.4960775466487,12.));
#114226=CARTESIAN_POINT('Ctrl Pts',(69.6445097822778,20.4807352327335,12.));
#114227=CARTESIAN_POINT('Ctrl Pts',(69.6246506158009,20.4654362743036,12.));
#114228=CARTESIAN_POINT('Ctrl Pts',(69.6048086141122,20.4501806927854,12.));
#114229=CARTESIAN_POINT('Ctrl Pts',(69.5849838968944,20.4349685095928,12.));
#114230=CARTESIAN_POINT('Ctrl Pts',(69.565176584305,20.4197997461306,12.));
#114231=CARTESIAN_POINT('Ctrl Pts',(69.5453867969815,20.4046744238002,12.));
#114232=CARTESIAN_POINT('Ctrl Pts',(69.5256146560444,20.3895925640006,12.));
#114233=CARTESIAN_POINT('Ctrl Pts',(69.5058602831004,20.3745541881267,12.));
#114234=CARTESIAN_POINT('Ctrl Pts',(69.4861238002433,20.359559317562,12.));
#114235=CARTESIAN_POINT('Ctrl Pts',(69.4664053300579,20.3446079736799,12.));
#114236=CARTESIAN_POINT('Ctrl Pts',(69.4467049956257,20.3297001778505,12.));
#114237=CARTESIAN_POINT('Ctrl Pts',(69.4270229205296,20.3148359514414,12.));
#114238=CARTESIAN_POINT('Ctrl Pts',(69.4073592288562,20.3000153158167,12.));
#114239=CARTESIAN_POINT('Ctrl Pts',(69.3877140451975,20.2852382923299,12.));
#114240=CARTESIAN_POINT('Ctrl Pts',(69.3680874946548,20.2705049023241,12.));
#114241=CARTESIAN_POINT('Ctrl Pts',(69.3484797028454,20.255815167139,12.));
#114242=CARTESIAN_POINT('Ctrl Pts',(69.3288907959065,20.2411691081122,12.));
#114243=CARTESIAN_POINT('Ctrl Pts',(69.3093209004986,20.2265667465784,12.));
#114244=CARTESIAN_POINT('Ctrl Pts',(69.2897701438066,20.2120081038622,12.));
#114245=CARTESIAN_POINT('Ctrl Pts',(69.2702386535432,20.1974932012775,12.));
#114246=CARTESIAN_POINT('Ctrl Pts',(69.2507265579562,20.183022060135,12.));
#114247=CARTESIAN_POINT('Ctrl Pts',(69.2312339858337,20.1685947017433,12.));
#114248=CARTESIAN_POINT('Ctrl Pts',(69.2117610665073,20.1542111474086,12.));
#114249=CARTESIAN_POINT('Ctrl Pts',(69.1923079298534,20.1398714184278,12.));
#114250=CARTESIAN_POINT('Ctrl Pts',(69.172874706296,20.1255755360871,12.));
#114251=CARTESIAN_POINT('Ctrl Pts',(69.1534615268153,20.1113235216694,12.));
#114252=CARTESIAN_POINT('Ctrl Pts',(69.1340685229516,20.0971153964557,12.));
#114253=CARTESIAN_POINT('Ctrl Pts',(69.1146958268104,20.0829511817251,12.));
#114254=CARTESIAN_POINT('Ctrl Pts',(69.0953435710634,20.0688308987478,12.));
#114255=CARTESIAN_POINT('Ctrl Pts',(69.0760118889525,20.0547545687839,12.));
#114256=CARTESIAN_POINT('Ctrl Pts',(69.0567009142968,20.0407222130902,12.));
#114257=CARTESIAN_POINT('Ctrl Pts',(69.0374107814977,20.0267338529221,12.));
#114258=CARTESIAN_POINT('Ctrl Pts',(69.0181416255433,20.0127895095327,12.));
#114259=CARTESIAN_POINT('Ctrl Pts',(68.9988935820101,19.9988892041671,12.));
#114260=CARTESIAN_POINT('Ctrl Pts',(68.9796667870667,19.98503295806,12.));
#114261=CARTESIAN_POINT('Ctrl Pts',(68.960461377483,19.9712207924437,12.));
#114262=CARTESIAN_POINT('Ctrl Pts',(68.9412774906346,19.9574527285492,12.));
#114263=CARTESIAN_POINT('Ctrl Pts',(68.9221152645086,19.9437287876063,12.));
#114264=CARTESIAN_POINT('Ctrl Pts',(68.902974837704,19.9300489908364,12.));
#114265=CARTESIAN_POINT('Ctrl Pts',(68.8838563494356,19.9164133594513,12.));
#114266=CARTESIAN_POINT('Ctrl Pts',(68.8647599395437,19.9028219146607,12.));
#114267=CARTESIAN_POINT('Ctrl Pts',(68.8456857484988,19.8892746776734,12.));
#114268=CARTESIAN_POINT('Ctrl Pts',(68.8266339174068,19.8757716696969,12.));
#114269=CARTESIAN_POINT('Ctrl Pts',(68.8076045880102,19.8623129119304,12.));
#114270=CARTESIAN_POINT('Ctrl Pts',(68.7885979026927,19.8488984255641,12.));
#114271=CARTESIAN_POINT('Ctrl Pts',(68.7696140044892,19.835528231787,12.));
#114272=CARTESIAN_POINT('Ctrl Pts',(68.7506530370918,19.8222023517874,12.));
#114273=CARTESIAN_POINT('Ctrl Pts',(68.7317151448557,19.8089208067532,12.));
#114274=CARTESIAN_POINT('Ctrl Pts',(68.7128004727998,19.795683617864,12.));
#114275=CARTESIAN_POINT('Ctrl Pts',(68.6939091666111,19.7824908062913,12.));
#114276=CARTESIAN_POINT('Ctrl Pts',(68.6750413726547,19.7693423932058,12.));
#114277=CARTESIAN_POINT('Ctrl Pts',(68.6561972379793,19.7562383997781,12.));
#114278=CARTESIAN_POINT('Ctrl Pts',(68.6373769103224,19.7431788471776,12.));
#114279=CARTESIAN_POINT('Ctrl Pts',(68.6185805381126,19.7301637565652,12.));
#114280=CARTESIAN_POINT('Ctrl Pts',(68.5998082704766,19.7171931490956,12.));
#114281=CARTESIAN_POINT('Ctrl Pts',(68.581060257249,19.7042670459237,12.));
#114282=CARTESIAN_POINT('Ctrl Pts',(68.5623366489779,19.6913854682046,12.));
#114283=CARTESIAN_POINT('Ctrl Pts',(68.5436375969311,19.6785484370927,12.));
#114284=CARTESIAN_POINT('Ctrl Pts',(68.5249632530979,19.6657559737336,12.));
#114285=CARTESIAN_POINT('Ctrl Pts',(68.5063137701971,19.6530080992686,12.));
#114286=CARTESIAN_POINT('Ctrl Pts',(68.4876893016856,19.6403048348395,12.));
#114287=CARTESIAN_POINT('Ctrl Pts',(68.4690900017632,19.6276462015888,12.));
#114288=CARTESIAN_POINT('Ctrl Pts',(68.4505160253778,19.6150322206577,12.));
#114289=CARTESIAN_POINT('Ctrl Pts',(68.4319675282275,19.6024629131785,12.));
#114290=CARTESIAN_POINT('Ctrl Pts',(68.4134446667696,19.5899383002803,12.));
#114291=CARTESIAN_POINT('Ctrl Pts',(68.3949475982335,19.5774584030938,12.));
#114292=CARTESIAN_POINT('Ctrl Pts',(68.3764764806287,19.5650232427516,12.));
#114293=CARTESIAN_POINT('Ctrl Pts',(68.3580314727523,19.5526328403852,12.));
#114294=CARTESIAN_POINT('Ctrl Pts',(68.3396127341938,19.5402872171191,12.));
#114295=CARTESIAN_POINT('Ctrl Pts',(68.3212204253417,19.5279863940773,12.));
#114296=CARTESIAN_POINT('Ctrl Pts',(68.3028547073864,19.5157303923856,12.));
#114297=CARTESIAN_POINT('Ctrl Pts',(68.2845157423233,19.5035192331705,12.));
#114298=CARTESIAN_POINT('Ctrl Pts',(68.2662036929526,19.4913529375543,12.));
#114299=CARTESIAN_POINT('Ctrl Pts',(68.2479187228803,19.4792315266501,12.));
#114300=CARTESIAN_POINT('Ctrl Pts',(68.2296609965448,19.467155021572,12.));
#114301=CARTESIAN_POINT('Ctrl Pts',(68.2114306792358,19.4551234434381,12.));
#114302=CARTESIAN_POINT('Ctrl Pts',(68.1932279371127,19.4431368133719,12.));
#114303=CARTESIAN_POINT('Ctrl Pts',(68.1750529372232,19.4311951524983,12.));
#114304=CARTESIAN_POINT('Ctrl Pts',(68.1569058475054,19.4192984819418,12.));
#114305=CARTESIAN_POINT('Ctrl Pts',(68.1387868367691,19.40744682283,12.));
#114306=CARTESIAN_POINT('Ctrl Pts',(68.1206960746769,19.3956401962895,12.));
#114307=CARTESIAN_POINT('Ctrl Pts',(68.1026337317285,19.3838786234421,12.));
#114308=CARTESIAN_POINT('Ctrl Pts',(68.0845999792247,19.3721621253912,12.));
#114309=CARTESIAN_POINT('Ctrl Pts',(68.0665949893195,19.3604907232314,12.));
#114310=CARTESIAN_POINT('Ctrl Pts',(68.0486189351011,19.3488644380641,12.));
#114311=CARTESIAN_POINT('Ctrl Pts',(68.0306719906636,19.3372832910076,12.));
#114312=CARTESIAN_POINT('Ctrl Pts',(68.0127543311776,19.3257473032035,12.));
#114313=CARTESIAN_POINT('Ctrl Pts',(67.9948661329617,19.3142564958203,12.));
#114314=CARTESIAN_POINT('Ctrl Pts',(67.9770075733485,19.302810890038,12.));
#114315=CARTESIAN_POINT('Ctrl Pts',(67.9591788305394,19.2914105070286,12.));
#114316=CARTESIAN_POINT('Ctrl Pts',(67.9413800834793,19.280055367936,12.));
#114317=CARTESIAN_POINT('Ctrl Pts',(67.9236115116758,19.2687454938442,12.));
#114318=CARTESIAN_POINT('Ctrl Pts',(67.9058732951788,19.2574809057696,12.));
#114319=CARTESIAN_POINT('Ctrl Pts',(67.8881656149955,19.2462616247279,12.));
#114320=CARTESIAN_POINT('Ctrl Pts',(67.8704886534544,19.2350876717874,12.));
#114321=CARTESIAN_POINT('Ctrl Pts',(67.8528425945184,19.2239590681133,12.));
#114322=CARTESIAN_POINT('Ctrl Pts',(67.835227624289,19.2128758350346,12.));
#114323=CARTESIAN_POINT('Ctrl Pts',(67.8176439306621,19.201837993993,12.));
#114324=CARTESIAN_POINT('Ctrl Pts',(67.8000917023926,19.1908455664098,12.));
#114325=CARTESIAN_POINT('Ctrl Pts',(67.7825711283096,19.1798985735688,12.));
#114326=CARTESIAN_POINT('Ctrl Pts',(67.7650823965127,19.168997036495,12.));
#114327=CARTESIAN_POINT('Ctrl Pts',(67.7476256934444,19.1581409758097,12.));
#114328=CARTESIAN_POINT('Ctrl Pts',(67.7302012056584,19.1473304119955,12.));
#114329=CARTESIAN_POINT('Ctrl Pts',(67.7128091219348,19.136565365709,12.));
#114330=CARTESIAN_POINT('Ctrl Pts',(67.6954496350063,19.1258458580345,12.));
#114331=CARTESIAN_POINT('Ctrl Pts',(67.6781229440573,19.115171910846,12.));
#114332=CARTESIAN_POINT('Ctrl Pts',(67.6608292549462,19.1045435468358,12.));
#114333=CARTESIAN_POINT('Ctrl Pts',(67.6435687749841,19.0939607887502,12.));
#114334=CARTESIAN_POINT('Ctrl Pts',(67.6263417083426,19.0834236587118,12.));
#114335=CARTESIAN_POINT('Ctrl Pts',(67.6091482520534,19.072932177628,12.));
#114336=CARTESIAN_POINT('Ctrl Pts',(67.5919885896222,19.062486364241,12.));
#114337=CARTESIAN_POINT('Ctrl Pts',(67.5748628971964,19.0520862360396,12.));
#114338=CARTESIAN_POINT('Ctrl Pts',(67.5577713558194,19.0417318110708,12.));
#114339=CARTESIAN_POINT('Ctrl Pts',(67.540714161288,19.0314231093923,12.));
#114340=CARTESIAN_POINT('Ctrl Pts',(67.5236915360331,19.021160154824,12.));
#114341=CARTESIAN_POINT('Ctrl Pts',(67.5067037372317,19.0109429761306,12.));
#114342=CARTESIAN_POINT('Ctrl Pts',(67.4897510316844,19.0007716032819,12.));
#114343=CARTESIAN_POINT('Ctrl Pts',(67.472833671964,18.9906460638625,12.));
#114344=CARTESIAN_POINT('Ctrl Pts',(67.4559518744638,18.9805663798449,12.));
#114345=CARTESIAN_POINT('Ctrl Pts',(67.4391057908418,18.9705325631711,12.));
#114346=CARTESIAN_POINT('Ctrl Pts',(67.4222955061981,18.9605446160985,12.));
#114347=CARTESIAN_POINT('Ctrl Pts',(67.4088759497911,18.9525909517915,12.));
#114348=CARTESIAN_POINT('Ctrl Pts',(67.3988274146651,18.9466463414299,12.));
#114349=CARTESIAN_POINT('Ctrl Pts',(67.3921355608328,18.9426924398719,12.));
#114350=CARTESIAN_POINT('Ctrl Pts',(67.3887914263118,18.9407177820969,12.));
#114351=CARTESIAN_POINT('Ctrl Pts',(70.538251407892,23.0342913834073,0.));
#114352=CARTESIAN_POINT('Ctrl Pts',(70.538251407892,23.0342913834073,4.));
#114353=CARTESIAN_POINT('Ctrl Pts',(70.538251407892,23.0342913834073,8.));
#114354=CARTESIAN_POINT('Ctrl Pts',(70.538251407892,23.0342913834073,12.));
#114355=CARTESIAN_POINT('Ctrl Pts',(70.6474988907591,23.0224954570734,0.));
#114356=CARTESIAN_POINT('Ctrl Pts',(70.6474988907591,23.0224954570734,4.));
#114357=CARTESIAN_POINT('Ctrl Pts',(70.6474988907591,23.0224954570734,8.));
#114358=CARTESIAN_POINT('Ctrl Pts',(70.6474988907591,23.0224954570734,12.));
#114359=CARTESIAN_POINT('Ctrl Pts',(70.83100071469,22.9364730048789,7.30819363922311E-17));
#114360=CARTESIAN_POINT('Ctrl Pts',(70.83100071469,22.9364730048789,4.00000000000001));
#114361=CARTESIAN_POINT('Ctrl Pts',(70.83100071469,22.9364730048789,7.99999999999999));
#114362=CARTESIAN_POINT('Ctrl Pts',(70.83100071469,22.9364730048789,12.));
#114363=CARTESIAN_POINT('Ctrl Pts',(70.9357242819029,22.7679558220498,2.46611180197085E-16));
#114364=CARTESIAN_POINT('Ctrl Pts',(70.9357242819029,22.7679558220498,4.));
#114365=CARTESIAN_POINT('Ctrl Pts',(70.9357242819029,22.7679558220498,8.00000000000001));
#114366=CARTESIAN_POINT('Ctrl Pts',(70.9357242819029,22.7679558220498,12.));
#114367=CARTESIAN_POINT('Ctrl Pts',(70.9608233461354,22.6894590071812,3.30265160424765E-16));
#114368=CARTESIAN_POINT('Ctrl Pts',(70.9608233461354,22.6894590071812,4.));
#114369=CARTESIAN_POINT('Ctrl Pts',(70.9608233461354,22.6894590071812,8.));
#114370=CARTESIAN_POINT('Ctrl Pts',(70.9608233461354,22.6894590071812,12.));
#114371=CARTESIAN_POINT('',(70.538251407892,23.0342913834073,0.));
#114372=CARTESIAN_POINT('',(70.9608233461355,22.6894590071812,0.));
#114373=CARTESIAN_POINT('Ctrl Pts',(70.538251407892,23.0342913834073,1.8765334327149E-16));
#114374=CARTESIAN_POINT('Ctrl Pts',(70.6474988907591,23.0224954570734,1.8765334327149E-16));
#114375=CARTESIAN_POINT('Ctrl Pts',(70.7523570758625,22.9733397701051,2.29414449781337E-16));
#114376=CARTESIAN_POINT('Ctrl Pts',(70.8314917485681,22.8972470282358,3.03974677078978E-16));
#114377=CARTESIAN_POINT('Ctrl Pts',(70.8908427530974,22.8401774718338,3.59894847552209E-16));
#114378=CARTESIAN_POINT('Ctrl Pts',(70.9357242819029,22.7679558220498,4.34264523468575E-16));
#114379=CARTESIAN_POINT('Ctrl Pts',(70.9608233461354,22.6894590071812,5.17918503696256E-16));
#114380=CARTESIAN_POINT('',(70.9608233461355,22.6894590071812,12.));
#114381=CARTESIAN_POINT('Ctrl Pts',(70.9608233461354,22.6894590071812,3.30265160424765E-16));
#114382=CARTESIAN_POINT('Ctrl Pts',(70.9608233461354,22.6894590071812,4.));
#114383=CARTESIAN_POINT('Ctrl Pts',(70.9608233461354,22.6894590071812,8.));
#114384=CARTESIAN_POINT('Ctrl Pts',(70.9608233461354,22.6894590071812,12.));
#114385=CARTESIAN_POINT('',(70.538251407892,23.0342913834073,12.));
#114386=CARTESIAN_POINT('Ctrl Pts',(70.9608233461354,22.6894590071812,12.));
#114387=CARTESIAN_POINT('Ctrl Pts',(70.9357242819029,22.7679558220498,12.));
#114388=CARTESIAN_POINT('Ctrl Pts',(70.8908427530974,22.8401774718337,12.));
#114389=CARTESIAN_POINT('Ctrl Pts',(70.8314917485681,22.8972470282358,12.));
#114390=CARTESIAN_POINT('Ctrl Pts',(70.7523570758625,22.9733397701051,12.));
#114391=CARTESIAN_POINT('Ctrl Pts',(70.6474988907591,23.0224954570734,12.));
#114392=CARTESIAN_POINT('Ctrl Pts',(70.538251407892,23.0342913834073,12.));
#114393=CARTESIAN_POINT('Ctrl Pts',(70.538251407892,23.0342913834073,12.));
#114394=CARTESIAN_POINT('Ctrl Pts',(70.538251407892,23.0342913834073,8.));
#114395=CARTESIAN_POINT('Ctrl Pts',(70.538251407892,23.0342913834073,4.));
#114396=CARTESIAN_POINT('Ctrl Pts',(70.538251407892,23.0342913834073,0.));
#114397=CARTESIAN_POINT('Origin',(3.57465004850839E-10,1.12812358559725E-10,
0.));
#114398=CARTESIAN_POINT('Origin',(3.57465004850839E-10,1.12812358559725E-10,
12.));
#114399=CARTESIAN_POINT('Origin',(3.57465004850839E-10,1.12812358559725E-10,
0.));
#114400=CARTESIAN_POINT('Ctrl Pts',(72.7986051948032,15.830763774726,-5.55111512312578E-16));
#114401=CARTESIAN_POINT('Ctrl Pts',(72.7986051948032,15.830763774726,4.));
#114402=CARTESIAN_POINT('Ctrl Pts',(72.7986051948032,15.830763774726,8.));
#114403=CARTESIAN_POINT('Ctrl Pts',(72.7986051948032,15.830763774726,12.));
#114404=CARTESIAN_POINT('Ctrl Pts',(72.8219545017353,15.7233907508395,-5.55111512312578E-16));
#114405=CARTESIAN_POINT('Ctrl Pts',(72.8219545017353,15.7233907508395,4.));
#114406=CARTESIAN_POINT('Ctrl Pts',(72.8219545017353,15.7233907508395,8.));
#114407=CARTESIAN_POINT('Ctrl Pts',(72.8219545017353,15.7233907508395,12.));
#114408=CARTESIAN_POINT('Ctrl Pts',(72.7983622347336,15.522104120072,-5.55111512312578E-16));
#114409=CARTESIAN_POINT('Ctrl Pts',(72.7983622347336,15.522104120072,4.00000000000001));
#114410=CARTESIAN_POINT('Ctrl Pts',(72.7983622347336,15.522104120072,8.));
#114411=CARTESIAN_POINT('Ctrl Pts',(72.7983622347336,15.522104120072,12.));
#114412=CARTESIAN_POINT('Ctrl Pts',(72.6715981986661,15.3694736926917,-5.55111512312578E-16));
#114413=CARTESIAN_POINT('Ctrl Pts',(72.6715981986661,15.3694736926917,4.));
#114414=CARTESIAN_POINT('Ctrl Pts',(72.6715981986661,15.3694736926917,8.));
#114415=CARTESIAN_POINT('Ctrl Pts',(72.6715981986661,15.3694736926917,12.));
#114416=CARTESIAN_POINT('Ctrl Pts',(72.605063349435,15.320844207719,-5.55111512312578E-16));
#114417=CARTESIAN_POINT('Ctrl Pts',(72.605063349435,15.320844207719,4.));
#114418=CARTESIAN_POINT('Ctrl Pts',(72.6050633494351,15.3208442077189,8.));
#114419=CARTESIAN_POINT('Ctrl Pts',(72.6050633494351,15.3208442077189,12.));
#114420=CARTESIAN_POINT('',(72.7986051948032,15.830763774726,0.));
#114421=CARTESIAN_POINT('',(72.6050633494351,15.3208442077189,0.));
#114422=CARTESIAN_POINT('Ctrl Pts',(72.7986051948032,15.830763774726,1.38777878078144E-16));
#114423=CARTESIAN_POINT('Ctrl Pts',(72.8219545017353,15.7233907508395,1.38777878078144E-16));
#114424=CARTESIAN_POINT('Ctrl Pts',(72.8084732063058,15.6083698189724,1.38777878078145E-16));
#114425=CARTESIAN_POINT('Ctrl Pts',(72.7613031699568,15.5092366269867,1.38777878078145E-16));
#114426=CARTESIAN_POINT('Ctrl Pts',(72.725925642695,15.4348867329975,1.38777878078145E-16));
#114427=CARTESIAN_POINT('Ctrl Pts',(72.6715981986661,15.3694736926917,1.38777878078144E-16));
#114428=CARTESIAN_POINT('Ctrl Pts',(72.605063349435,15.320844207719,1.38777878078145E-16));
#114429=CARTESIAN_POINT('',(72.6050633494351,15.3208442077189,12.));
#114430=CARTESIAN_POINT('Ctrl Pts',(72.605063349435,15.320844207719,-5.55111512312578E-16));
#114431=CARTESIAN_POINT('Ctrl Pts',(72.605063349435,15.320844207719,4.));
#114432=CARTESIAN_POINT('Ctrl Pts',(72.6050633494351,15.3208442077189,8.));
#114433=CARTESIAN_POINT('Ctrl Pts',(72.6050633494351,15.3208442077189,12.));
#114434=CARTESIAN_POINT('',(72.7986051948032,15.830763774726,12.));
#114435=CARTESIAN_POINT('Ctrl Pts',(72.6050633494351,15.3208442077189,12.));
#114436=CARTESIAN_POINT('Ctrl Pts',(72.6715981986661,15.3694736926917,12.));
#114437=CARTESIAN_POINT('Ctrl Pts',(72.7259256426951,15.4348867329975,12.));
#114438=CARTESIAN_POINT('Ctrl Pts',(72.7613031699568,15.5092366269867,12.));
#114439=CARTESIAN_POINT('Ctrl Pts',(72.8084732063058,15.6083698189724,12.));
#114440=CARTESIAN_POINT('Ctrl Pts',(72.8219545017353,15.7233907508395,12.));
#114441=CARTESIAN_POINT('Ctrl Pts',(72.7986051948032,15.830763774726,12.));
#114442=CARTESIAN_POINT('Ctrl Pts',(72.7986051948032,15.830763774726,12.));
#114443=CARTESIAN_POINT('Ctrl Pts',(72.7986051948032,15.830763774726,8.));
#114444=CARTESIAN_POINT('Ctrl Pts',(72.7986051948032,15.830763774726,4.));
#114445=CARTESIAN_POINT('Ctrl Pts',(72.7986051948032,15.830763774726,-5.55111512312578E-16));
#114446=CARTESIAN_POINT('Ctrl Pts',(68.7831490561748,12.9953224629497,0.));
#114447=CARTESIAN_POINT('Ctrl Pts',(68.7831490561748,12.9953224629497,12.));
#114448=CARTESIAN_POINT('Ctrl Pts',(68.7866525680193,12.9969981460277,0.));
#114449=CARTESIAN_POINT('Ctrl Pts',(68.7866525680193,12.9969981460277,12.));
#114450=CARTESIAN_POINT('Ctrl Pts',(68.7936635625545,13.0003537683055,0.));
#114451=CARTESIAN_POINT('Ctrl Pts',(68.7936635625545,13.0003537683055,12.));
#114452=CARTESIAN_POINT('Ctrl Pts',(68.804191966902,13.0053999700875,0.));
#114453=CARTESIAN_POINT('Ctrl Pts',(68.804191966902,13.0053999700875,12.));
#114454=CARTESIAN_POINT('Ctrl Pts',(68.8182536653656,13.0121537768946,0.));
#114455=CARTESIAN_POINT('Ctrl Pts',(68.8182536653656,13.0121537768946,12.));
#114456=CARTESIAN_POINT('Ctrl Pts',(68.8358704887468,13.0206386039691,0.));
#114457=CARTESIAN_POINT('Ctrl Pts',(68.8358704887468,13.0206386039691,12.));
#114458=CARTESIAN_POINT('Ctrl Pts',(68.8535269726793,13.0291660060107,0.));
#114459=CARTESIAN_POINT('Ctrl Pts',(68.8535269726793,13.0291660060107,12.));
#114460=CARTESIAN_POINT('Ctrl Pts',(68.8712230321906,13.0377359881875,0.));
#114461=CARTESIAN_POINT('Ctrl Pts',(68.8712230321906,13.0377359881875,12.));
#114462=CARTESIAN_POINT('Ctrl Pts',(68.8889585151585,13.0463485518207,0.));
#114463=CARTESIAN_POINT('Ctrl Pts',(68.8889585151585,13.0463485518207,12.));
#114464=CARTESIAN_POINT('Ctrl Pts',(68.9067332040985,13.0550036938813,0.));
#114465=CARTESIAN_POINT('Ctrl Pts',(68.9067332040985,13.0550036938813,12.));
#114466=CARTESIAN_POINT('Ctrl Pts',(68.9245468449945,13.0637014089029,0.));
#114467=CARTESIAN_POINT('Ctrl Pts',(68.9245468449945,13.0637014089029,12.));
#114468=CARTESIAN_POINT('Ctrl Pts',(68.9423991694492,13.072441690283,0.));
#114469=CARTESIAN_POINT('Ctrl Pts',(68.9423991694492,13.072441690283,12.));
#114470=CARTESIAN_POINT('Ctrl Pts',(68.9602899187573,13.0812245317808,0.));
#114471=CARTESIAN_POINT('Ctrl Pts',(68.9602899187573,13.0812245317808,12.));
#114472=CARTESIAN_POINT('Ctrl Pts',(68.9782188692581,13.090049929053,0.));
#114473=CARTESIAN_POINT('Ctrl Pts',(68.9782188692581,13.090049929053,12.));
#114474=CARTESIAN_POINT('Ctrl Pts',(68.9961858241519,13.0989178791834,0.));
#114475=CARTESIAN_POINT('Ctrl Pts',(68.9961858241519,13.0989178791834,12.));
#114476=CARTESIAN_POINT('Ctrl Pts',(69.0141906015113,13.1078283799722,0.));
#114477=CARTESIAN_POINT('Ctrl Pts',(69.0141906015113,13.1078283799722,12.));
#114478=CARTESIAN_POINT('Ctrl Pts',(69.0322330243348,13.1167814293497,0.));
#114479=CARTESIAN_POINT('Ctrl Pts',(69.0322330243348,13.1167814293497,12.));
#114480=CARTESIAN_POINT('Ctrl Pts',(69.0503129081817,13.1257770246386,0.));
#114481=CARTESIAN_POINT('Ctrl Pts',(69.0503129081817,13.1257770246386,12.));
#114482=CARTESIAN_POINT('Ctrl Pts',(69.0684300549477,13.1348151621834,0.));
#114483=CARTESIAN_POINT('Ctrl Pts',(69.0684300549477,13.1348151621834,12.));
#114484=CARTESIAN_POINT('Ctrl Pts',(69.0865842593102,13.1438958377404,0.));
#114485=CARTESIAN_POINT('Ctrl Pts',(69.0865842593102,13.1438958377404,12.));
#114486=CARTESIAN_POINT('Ctrl Pts',(69.1047753127643,13.1530190467183,0.));
#114487=CARTESIAN_POINT('Ctrl Pts',(69.1047753127643,13.1530190467183,12.));
#114488=CARTESIAN_POINT('Ctrl Pts',(69.1230030082573,13.1621847844528,0.));
#114489=CARTESIAN_POINT('Ctrl Pts',(69.1230030082573,13.1621847844528,12.));
#114490=CARTESIAN_POINT('Ctrl Pts',(69.1412671454564,13.1713930465133,0.));
#114491=CARTESIAN_POINT('Ctrl Pts',(69.1412671454564,13.1713930465133,12.));
#114492=CARTESIAN_POINT('Ctrl Pts',(69.1595675305245,13.1806438286934,0.));
#114493=CARTESIAN_POINT('Ctrl Pts',(69.1595675305245,13.1806438286934,12.));
#114494=CARTESIAN_POINT('Ctrl Pts',(69.1779039735996,13.1899371268683,0.));
#114495=CARTESIAN_POINT('Ctrl Pts',(69.1779039735996,13.1899371268683,12.));
#114496=CARTESIAN_POINT('Ctrl Pts',(69.1962762870527,13.1992729368929,0.));
#114497=CARTESIAN_POINT('Ctrl Pts',(69.1962762870527,13.1992729368929,12.));
#114498=CARTESIAN_POINT('Ctrl Pts',(69.2146842833537,13.2086512544735,0.));
#114499=CARTESIAN_POINT('Ctrl Pts',(69.2146842833537,13.2086512544735,12.));
#114500=CARTESIAN_POINT('Ctrl Pts',(69.2331277732861,13.2180720750594,0.));
#114501=CARTESIAN_POINT('Ctrl Pts',(69.2331277732861,13.2180720750594,12.));
#114502=CARTESIAN_POINT('Ctrl Pts',(69.2516065668844,13.2275353939051,0.));
#114503=CARTESIAN_POINT('Ctrl Pts',(69.2516065668844,13.2275353939051,12.));
#114504=CARTESIAN_POINT('Ctrl Pts',(69.270120474245,13.237041206122,0.));
#114505=CARTESIAN_POINT('Ctrl Pts',(69.270120474245,13.237041206122,12.));
#114506=CARTESIAN_POINT('Ctrl Pts',(69.2886693063182,13.2465895067262,0.));
#114507=CARTESIAN_POINT('Ctrl Pts',(69.2886693063182,13.2465895067262,12.));
#114508=CARTESIAN_POINT('Ctrl Pts',(69.3072528758518,13.2561802906896,0.));
#114509=CARTESIAN_POINT('Ctrl Pts',(69.3072528758518,13.2561802906896,12.));
#114510=CARTESIAN_POINT('Ctrl Pts',(69.3258709977382,13.265813552961,0.));
#114511=CARTESIAN_POINT('Ctrl Pts',(69.3258709977382,13.265813552961,12.));
#114512=CARTESIAN_POINT('Ctrl Pts',(69.3445234885065,13.2754892884433,0.));
#114513=CARTESIAN_POINT('Ctrl Pts',(69.3445234885065,13.2754892884433,12.));
#114514=CARTESIAN_POINT('Ctrl Pts',(69.3632101660066,13.2852074919766,0.));
#114515=CARTESIAN_POINT('Ctrl Pts',(69.3632101660066,13.2852074919766,12.));
#114516=CARTESIAN_POINT('Ctrl Pts',(69.3819308490422,13.2949681583167,0.));
#114517=CARTESIAN_POINT('Ctrl Pts',(69.3819308490422,13.2949681583167,12.));
#114518=CARTESIAN_POINT('Ctrl Pts',(69.4006853569511,13.3047712821051,0.));
#114519=CARTESIAN_POINT('Ctrl Pts',(69.4006853569511,13.3047712821051,12.));
#114520=CARTESIAN_POINT('Ctrl Pts',(69.4194735096265,13.3146168578743,0.));
#114521=CARTESIAN_POINT('Ctrl Pts',(69.4194735096265,13.3146168578743,12.));
#114522=CARTESIAN_POINT('Ctrl Pts',(69.4382951276998,13.3245048800643,0.));
#114523=CARTESIAN_POINT('Ctrl Pts',(69.4382951276998,13.3245048800643,12.));
#114524=CARTESIAN_POINT('Ctrl Pts',(69.4571500326673,13.3344353430313,0.));
#114525=CARTESIAN_POINT('Ctrl Pts',(69.4571500326673,13.3344353430313,12.));
#114526=CARTESIAN_POINT('Ctrl Pts',(69.4760380470365,13.3444082410543,0.));
#114527=CARTESIAN_POINT('Ctrl Pts',(69.4760380470365,13.3444082410543,12.));
#114528=CARTESIAN_POINT('Ctrl Pts',(69.4949589944606,13.3544235683394,0.));
#114529=CARTESIAN_POINT('Ctrl Pts',(69.4949589944606,13.3544235683394,12.));
#114530=CARTESIAN_POINT('Ctrl Pts',(69.5139126996675,13.3644813190219,0.));
#114531=CARTESIAN_POINT('Ctrl Pts',(69.5139126996675,13.3644813190219,12.));
#114532=CARTESIAN_POINT('Ctrl Pts',(69.5328989883885,13.3745814871665,0.));
#114533=CARTESIAN_POINT('Ctrl Pts',(69.5328989883885,13.3745814871665,12.));
#114534=CARTESIAN_POINT('Ctrl Pts',(69.5519176872862,13.3847240667628,0.));
#114535=CARTESIAN_POINT('Ctrl Pts',(69.5519176872862,13.3847240667628,12.));
#114536=CARTESIAN_POINT('Ctrl Pts',(69.5709686238724,13.3949090517177,0.));
#114537=CARTESIAN_POINT('Ctrl Pts',(69.5709686238724,13.3949090517177,12.));
#114538=CARTESIAN_POINT('Ctrl Pts',(69.5900516264553,13.40513643585,0.));
#114539=CARTESIAN_POINT('Ctrl Pts',(69.5900516264553,13.40513643585,12.));
#114540=CARTESIAN_POINT('Ctrl Pts',(69.6091665241765,13.4154062129002,0.));
#114541=CARTESIAN_POINT('Ctrl Pts',(69.6091665241765,13.4154062129002,12.));
#114542=CARTESIAN_POINT('Ctrl Pts',(69.6283131470273,13.4257183765341,0.));
#114543=CARTESIAN_POINT('Ctrl Pts',(69.6283131470273,13.4257183765341,12.));
#114544=CARTESIAN_POINT('Ctrl Pts',(69.6474913258675,13.4360729203442,0.));
#114545=CARTESIAN_POINT('Ctrl Pts',(69.6474913258675,13.4360729203442,12.));
#114546=CARTESIAN_POINT('Ctrl Pts',(69.666700892444,13.4464698378453,0.));
#114547=CARTESIAN_POINT('Ctrl Pts',(69.666700892444,13.4464698378453,12.));
#114548=CARTESIAN_POINT('Ctrl Pts',(69.6859416793885,13.456909122476,0.));
#114549=CARTESIAN_POINT('Ctrl Pts',(69.6859416793885,13.456909122476,12.));
#114550=CARTESIAN_POINT('Ctrl Pts',(69.7052135201998,13.4673907676044,0.));
#114551=CARTESIAN_POINT('Ctrl Pts',(69.7052135201998,13.4673907676044,12.));
#114552=CARTESIAN_POINT('Ctrl Pts',(69.724516249225,13.4779147665285,0.));
#114553=CARTESIAN_POINT('Ctrl Pts',(69.724516249225,13.4779147665285,12.));
#114554=CARTESIAN_POINT('Ctrl Pts',(69.7438497016406,13.4884811124748,0.));
#114555=CARTESIAN_POINT('Ctrl Pts',(69.7438497016406,13.4884811124748,12.));
#114556=CARTESIAN_POINT('Ctrl Pts',(69.7632137134249,13.4990897985905,0.));
#114557=CARTESIAN_POINT('Ctrl Pts',(69.7632137134249,13.4990897985905,12.));
#114558=CARTESIAN_POINT('Ctrl Pts',(69.7826081213576,13.5097408179479,0.));
#114559=CARTESIAN_POINT('Ctrl Pts',(69.7826081213576,13.5097408179479,12.));
#114560=CARTESIAN_POINT('Ctrl Pts',(69.8020327630205,13.5204341635507,0.));
#114561=CARTESIAN_POINT('Ctrl Pts',(69.8020327630205,13.5204341635507,12.));
#114562=CARTESIAN_POINT('Ctrl Pts',(69.8214874767944,13.5311698283339,0.));
#114563=CARTESIAN_POINT('Ctrl Pts',(69.8214874767944,13.5311698283339,12.));
#114564=CARTESIAN_POINT('Ctrl Pts',(69.840972101856,13.5419478051625,0.));
#114565=CARTESIAN_POINT('Ctrl Pts',(69.840972101856,13.5419478051625,12.));
#114566=CARTESIAN_POINT('Ctrl Pts',(69.8604864781706,13.5527680868255,0.));
#114567=CARTESIAN_POINT('Ctrl Pts',(69.8604864781706,13.5527680868255,12.));
#114568=CARTESIAN_POINT('Ctrl Pts',(69.8800304464882,13.5636306660422,0.));
#114569=CARTESIAN_POINT('Ctrl Pts',(69.8800304464882,13.5636306660422,12.));
#114570=CARTESIAN_POINT('Ctrl Pts',(69.8996038483361,13.5745355354657,0.));
#114571=CARTESIAN_POINT('Ctrl Pts',(69.8996038483361,13.5745355354657,12.));
#114572=CARTESIAN_POINT('Ctrl Pts',(69.9192065260108,13.5854826876835,0.));
#114573=CARTESIAN_POINT('Ctrl Pts',(69.9192065260108,13.5854826876835,12.));
#114574=CARTESIAN_POINT('Ctrl Pts',(69.9388383225648,13.5964721152135,0.));
#114575=CARTESIAN_POINT('Ctrl Pts',(69.9388383225648,13.5964721152135,12.));
#114576=CARTESIAN_POINT('Ctrl Pts',(69.9584990817974,13.6075038104999,0.));
#114577=CARTESIAN_POINT('Ctrl Pts',(69.9584990817974,13.6075038104999,12.));
#114578=CARTESIAN_POINT('Ctrl Pts',(69.9781886482528,13.6185777659198,0.));
#114579=CARTESIAN_POINT('Ctrl Pts',(69.9781886482528,13.6185777659198,12.));
#114580=CARTESIAN_POINT('Ctrl Pts',(69.9979068672153,13.6296939737865,0.));
#114581=CARTESIAN_POINT('Ctrl Pts',(69.9979068672153,13.6296939737865,12.));
#114582=CARTESIAN_POINT('Ctrl Pts',(70.0176535847049,13.6408524263496,0.));
#114583=CARTESIAN_POINT('Ctrl Pts',(70.0176535847049,13.6408524263496,12.));
#114584=CARTESIAN_POINT('Ctrl Pts',(70.0374286474677,13.6520531157907,0.));
#114585=CARTESIAN_POINT('Ctrl Pts',(70.0374286474677,13.6520531157907,12.));
#114586=CARTESIAN_POINT('Ctrl Pts',(70.0572319029676,13.6632960342196,0.));
#114587=CARTESIAN_POINT('Ctrl Pts',(70.0572319029676,13.6632960342196,12.));
#114588=CARTESIAN_POINT('Ctrl Pts',(70.0770631993856,13.674581173683,0.));
#114589=CARTESIAN_POINT('Ctrl Pts',(70.0770631993856,13.674581173683,12.));
#114590=CARTESIAN_POINT('Ctrl Pts',(70.0969223856136,13.6859085261653,0.));
#114591=CARTESIAN_POINT('Ctrl Pts',(70.0969223856136,13.6859085261653,12.));
#114592=CARTESIAN_POINT('Ctrl Pts',(70.1168093112486,13.6972780835897,0.));
#114593=CARTESIAN_POINT('Ctrl Pts',(70.1168093112486,13.6972780835897,12.));
#114594=CARTESIAN_POINT('Ctrl Pts',(70.1367238265825,13.7086898378122,0.));
#114595=CARTESIAN_POINT('Ctrl Pts',(70.1367238265825,13.7086898378122,12.));
#114596=CARTESIAN_POINT('Ctrl Pts',(70.156665782595,13.7201437806199,0.));
#114597=CARTESIAN_POINT('Ctrl Pts',(70.156665782595,13.7201437806199,12.));
#114598=CARTESIAN_POINT('Ctrl Pts',(70.1766350309518,13.7316399037393,0.));
#114599=CARTESIAN_POINT('Ctrl Pts',(70.1766350309518,13.7316399037393,12.));
#114600=CARTESIAN_POINT('Ctrl Pts',(70.1966314239995,13.7431781988365,0.));
#114601=CARTESIAN_POINT('Ctrl Pts',(70.1966314239995,13.7431781988365,12.));
#114602=CARTESIAN_POINT('Ctrl Pts',(70.2166548147604,13.7547586575181,0.));
#114603=CARTESIAN_POINT('Ctrl Pts',(70.2166548147604,13.7547586575181,12.));
#114604=CARTESIAN_POINT('Ctrl Pts',(70.2367050569216,13.7663812713243,0.));
#114605=CARTESIAN_POINT('Ctrl Pts',(70.2367050569216,13.7663812713243,12.));
#114606=CARTESIAN_POINT('Ctrl Pts',(70.2567820048303,13.7780460317294,0.));
#114607=CARTESIAN_POINT('Ctrl Pts',(70.2567820048303,13.7780460317294,12.));
#114608=CARTESIAN_POINT('Ctrl Pts',(70.2768855134947,13.7897529301491,0.));
#114609=CARTESIAN_POINT('Ctrl Pts',(70.2768855134947,13.7897529301491,12.));
#114610=CARTESIAN_POINT('Ctrl Pts',(70.2970154385774,13.8015019579414,0.));
#114611=CARTESIAN_POINT('Ctrl Pts',(70.2970154385774,13.8015019579414,12.));
#114612=CARTESIAN_POINT('Ctrl Pts',(70.3171716363897,13.8132931064064,0.));
#114613=CARTESIAN_POINT('Ctrl Pts',(70.3171716363897,13.8132931064064,12.));
#114614=CARTESIAN_POINT('Ctrl Pts',(70.3373539638809,13.8251263667791,0.));
#114615=CARTESIAN_POINT('Ctrl Pts',(70.3373539638809,13.8251263667791,12.));
#114616=CARTESIAN_POINT('Ctrl Pts',(70.3575622786335,13.8370017302309,0.));
#114617=CARTESIAN_POINT('Ctrl Pts',(70.3575622786335,13.8370017302309,12.));
#114618=CARTESIAN_POINT('Ctrl Pts',(70.3777964388632,13.8489191878767,0.));
#114619=CARTESIAN_POINT('Ctrl Pts',(70.3777964388632,13.8489191878767,12.));
#114620=CARTESIAN_POINT('Ctrl Pts',(70.3980563034133,13.8608787307752,0.));
#114621=CARTESIAN_POINT('Ctrl Pts',(70.3980563034133,13.8608787307752,12.));
#114622=CARTESIAN_POINT('Ctrl Pts',(70.41834173175,13.8728803499287,0.));
#114623=CARTESIAN_POINT('Ctrl Pts',(70.41834173175,13.8728803499287,12.));
#114624=CARTESIAN_POINT('Ctrl Pts',(70.4386525839521,13.8849240362763,0.));
#114625=CARTESIAN_POINT('Ctrl Pts',(70.4386525839521,13.8849240362763,12.));
#114626=CARTESIAN_POINT('Ctrl Pts',(70.4589887207073,13.8970097806954,0.));
#114627=CARTESIAN_POINT('Ctrl Pts',(70.4589887207073,13.8970097806954,12.));
#114628=CARTESIAN_POINT('Ctrl Pts',(70.4793500033124,13.9091375740088,0.));
#114629=CARTESIAN_POINT('Ctrl Pts',(70.4793500033124,13.9091375740088,12.));
#114630=CARTESIAN_POINT('Ctrl Pts',(70.4997362936673,13.9213074069853,0.));
#114631=CARTESIAN_POINT('Ctrl Pts',(70.4997362936673,13.9213074069853,12.));
#114632=CARTESIAN_POINT('Ctrl Pts',(70.520147454271,13.9335192703388,0.));
#114633=CARTESIAN_POINT('Ctrl Pts',(70.520147454271,13.9335192703388,12.));
#114634=CARTESIAN_POINT('Ctrl Pts',(70.5405833482112,13.9457731547215,0.));
#114635=CARTESIAN_POINT('Ctrl Pts',(70.5405833482112,13.9457731547215,12.));
#114636=CARTESIAN_POINT('Ctrl Pts',(70.5610438391612,13.958069050726,0.));
#114637=CARTESIAN_POINT('Ctrl Pts',(70.5610438391612,13.958069050726,12.));
#114638=CARTESIAN_POINT('Ctrl Pts',(70.5815287913784,13.9704069488917,0.));
#114639=CARTESIAN_POINT('Ctrl Pts',(70.5815287913784,13.9704069488917,12.));
#114640=CARTESIAN_POINT('Ctrl Pts',(70.6020380697005,13.9827868397057,0.));
#114641=CARTESIAN_POINT('Ctrl Pts',(70.6020380697005,13.9827868397057,12.));
#114642=CARTESIAN_POINT('Ctrl Pts',(70.6225715395394,13.9952087136018,0.));
#114643=CARTESIAN_POINT('Ctrl Pts',(70.6225715395394,13.9952087136018,12.));
#114644=CARTESIAN_POINT('Ctrl Pts',(70.6431290668745,14.0076725609537,0.));
#114645=CARTESIAN_POINT('Ctrl Pts',(70.6431290668745,14.0076725609537,12.));
#114646=CARTESIAN_POINT('Ctrl Pts',(70.6637105182484,14.020178372077,0.));
#114647=CARTESIAN_POINT('Ctrl Pts',(70.6637105182484,14.020178372077,12.));
#114648=CARTESIAN_POINT('Ctrl Pts',(70.6843157607668,14.0327261372362,0.));
#114649=CARTESIAN_POINT('Ctrl Pts',(70.6843157607668,14.0327261372362,12.));
#114650=CARTESIAN_POINT('Ctrl Pts',(70.7049446620928,14.0453158466451,0.));
#114651=CARTESIAN_POINT('Ctrl Pts',(70.7049446620928,14.0453158466451,12.));
#114652=CARTESIAN_POINT('Ctrl Pts',(70.7255970904436,14.0579474904657,0.));
#114653=CARTESIAN_POINT('Ctrl Pts',(70.7255970904436,14.0579474904657,12.));
#114654=CARTESIAN_POINT('Ctrl Pts',(70.7462729145807,14.0706210588016,0.));
#114655=CARTESIAN_POINT('Ctrl Pts',(70.7462729145807,14.0706210588016,12.));
#114656=CARTESIAN_POINT('Ctrl Pts',(70.7669720038077,14.0833365416996,0.));
#114657=CARTESIAN_POINT('Ctrl Pts',(70.7669720038077,14.0833365416996,12.));
#114658=CARTESIAN_POINT('Ctrl Pts',(70.7876942279697,14.0960939291569,0.));
#114659=CARTESIAN_POINT('Ctrl Pts',(70.7876942279697,14.0960939291569,12.));
#114660=CARTESIAN_POINT('Ctrl Pts',(70.8084394574493,14.1088932111214,0.));
#114661=CARTESIAN_POINT('Ctrl Pts',(70.8084394574493,14.1088932111214,12.));
#114662=CARTESIAN_POINT('Ctrl Pts',(70.8292075631621,14.1217343774913,0.));
#114663=CARTESIAN_POINT('Ctrl Pts',(70.8292075631621,14.1217343774913,12.));
#114664=CARTESIAN_POINT('Ctrl Pts',(70.8499984165489,14.1346174181079,0.));
#114665=CARTESIAN_POINT('Ctrl Pts',(70.8499984165489,14.1346174181079,12.));
#114666=CARTESIAN_POINT('Ctrl Pts',(70.8708118895715,14.1475423227568,0.));
#114667=CARTESIAN_POINT('Ctrl Pts',(70.8708118895715,14.1475423227568,12.));
#114668=CARTESIAN_POINT('Ctrl Pts',(70.8916478547132,14.1605090811754,0.));
#114669=CARTESIAN_POINT('Ctrl Pts',(70.8916478547132,14.1605090811754,12.));
#114670=CARTESIAN_POINT('Ctrl Pts',(70.9125061849745,14.1735176830533,0.));
#114671=CARTESIAN_POINT('Ctrl Pts',(70.9125061849745,14.1735176830533,12.));
#114672=CARTESIAN_POINT('Ctrl Pts',(70.9333867538704,14.1865681180321,0.));
#114673=CARTESIAN_POINT('Ctrl Pts',(70.9333867538704,14.1865681180321,12.));
#114674=CARTESIAN_POINT('Ctrl Pts',(70.9542894354216,14.1996603756982,0.));
#114675=CARTESIAN_POINT('Ctrl Pts',(70.9542894354216,14.1996603756982,12.));
#114676=CARTESIAN_POINT('Ctrl Pts',(70.9752141041518,14.2127944455839,0.));
#114677=CARTESIAN_POINT('Ctrl Pts',(70.9752141041518,14.2127944455839,12.));
#114678=CARTESIAN_POINT('Ctrl Pts',(70.9961606350861,14.2259703171737,0.));
#114679=CARTESIAN_POINT('Ctrl Pts',(70.9961606350861,14.2259703171737,12.));
#114680=CARTESIAN_POINT('Ctrl Pts',(71.0171289037488,14.2391879799062,0.));
#114681=CARTESIAN_POINT('Ctrl Pts',(71.0171289037488,14.2391879799062,12.));
#114682=CARTESIAN_POINT('Ctrl Pts',(71.0381187861588,14.2524474231733,0.));
#114683=CARTESIAN_POINT('Ctrl Pts',(71.0381187861588,14.2524474231733,12.));
#114684=CARTESIAN_POINT('Ctrl Pts',(71.0591301588231,14.2657486363139,0.));
#114685=CARTESIAN_POINT('Ctrl Pts',(71.0591301588231,14.2657486363139,12.));
#114686=CARTESIAN_POINT('Ctrl Pts',(71.0801628987332,14.2790916086133,0.));
#114687=CARTESIAN_POINT('Ctrl Pts',(71.0801628987332,14.2790916086133,12.));
#114688=CARTESIAN_POINT('Ctrl Pts',(71.1012168833643,14.2924763293105,0.));
#114689=CARTESIAN_POINT('Ctrl Pts',(71.1012168833643,14.2924763293105,12.));
#114690=CARTESIAN_POINT('Ctrl Pts',(71.1222919906727,14.3059027875994,0.));
#114691=CARTESIAN_POINT('Ctrl Pts',(71.1222919906727,14.3059027875994,12.));
#114692=CARTESIAN_POINT('Ctrl Pts',(71.1433880990929,14.3193709726294,0.));
#114693=CARTESIAN_POINT('Ctrl Pts',(71.1433880990929,14.3193709726294,12.));
#114694=CARTESIAN_POINT('Ctrl Pts',(71.1645050875308,14.332880873499,0.));
#114695=CARTESIAN_POINT('Ctrl Pts',(71.1645050875308,14.332880873499,12.));
#114696=CARTESIAN_POINT('Ctrl Pts',(71.1856428353593,14.3464324792534,0.));
#114697=CARTESIAN_POINT('Ctrl Pts',(71.1856428353593,14.3464324792534,12.));
#114698=CARTESIAN_POINT('Ctrl Pts',(71.2068012224174,14.3600257788924,0.));
#114699=CARTESIAN_POINT('Ctrl Pts',(71.2068012224174,14.3600257788924,12.));
#114700=CARTESIAN_POINT('Ctrl Pts',(71.2279801290084,14.3736607613722,0.));
#114701=CARTESIAN_POINT('Ctrl Pts',(71.2279801290084,14.3736607613722,12.));
#114702=CARTESIAN_POINT('Ctrl Pts',(71.2491794358958,14.3873374156056,0.));
#114703=CARTESIAN_POINT('Ctrl Pts',(71.2491794358958,14.3873374156056,12.));
#114704=CARTESIAN_POINT('Ctrl Pts',(71.2703990242988,14.401055730457,0.));
#114705=CARTESIAN_POINT('Ctrl Pts',(71.2703990242988,14.401055730457,12.));
#114706=CARTESIAN_POINT('Ctrl Pts',(71.2916387758861,14.4148156947384,0.));
#114707=CARTESIAN_POINT('Ctrl Pts',(71.2916387758861,14.4148156947384,12.));
#114708=CARTESIAN_POINT('Ctrl Pts',(71.312898572777,14.4286172972167,0.));
#114709=CARTESIAN_POINT('Ctrl Pts',(71.312898572777,14.4286172972167,12.));
#114710=CARTESIAN_POINT('Ctrl Pts',(71.3341782975386,14.4424605266165,0.));
#114711=CARTESIAN_POINT('Ctrl Pts',(71.3341782975386,14.4424605266165,12.));
#114712=CARTESIAN_POINT('Ctrl Pts',(71.3554778331835,14.4563453716204,0.));
#114713=CARTESIAN_POINT('Ctrl Pts',(71.3554778331835,14.4563453716204,12.));
#114714=CARTESIAN_POINT('Ctrl Pts',(71.376797063165,14.4702718208651,0.));
#114715=CARTESIAN_POINT('Ctrl Pts',(71.376797063165,14.4702718208651,12.));
#114716=CARTESIAN_POINT('Ctrl Pts',(71.3981358713723,14.4842398629355,0.));
#114717=CARTESIAN_POINT('Ctrl Pts',(71.3981358713723,14.4842398629355,12.));
#114718=CARTESIAN_POINT('Ctrl Pts',(71.4194941421292,14.4982494863718,0.));
#114719=CARTESIAN_POINT('Ctrl Pts',(71.4194941421292,14.4982494863718,12.));
#114720=CARTESIAN_POINT('Ctrl Pts',(71.4408717601923,14.5123006796728,0.));
#114721=CARTESIAN_POINT('Ctrl Pts',(71.4408717601923,14.5123006796728,12.));
#114722=CARTESIAN_POINT('Ctrl Pts',(71.4622686107475,14.5263934312969,0.));
#114723=CARTESIAN_POINT('Ctrl Pts',(71.4622686107475,14.5263934312969,12.));
#114724=CARTESIAN_POINT('Ctrl Pts',(71.4836845794048,14.540527729659,0.));
#114725=CARTESIAN_POINT('Ctrl Pts',(71.4836845794048,14.540527729659,12.));
#114726=CARTESIAN_POINT('Ctrl Pts',(71.5051195521909,14.5547035631234,0.));
#114727=CARTESIAN_POINT('Ctrl Pts',(71.5051195521909,14.5547035631234,12.));
#114728=CARTESIAN_POINT('Ctrl Pts',(71.5265734155498,14.5689209200091,0.));
#114729=CARTESIAN_POINT('Ctrl Pts',(71.5265734155498,14.5689209200091,12.));
#114730=CARTESIAN_POINT('Ctrl Pts',(71.5480460563447,14.5831797885952,0.));
#114731=CARTESIAN_POINT('Ctrl Pts',(71.5480460563447,14.5831797885952,12.));
#114732=CARTESIAN_POINT('Ctrl Pts',(71.5695373618562,14.597480157121,0.));
#114733=CARTESIAN_POINT('Ctrl Pts',(71.5695373618562,14.597480157121,12.));
#114734=CARTESIAN_POINT('Ctrl Pts',(71.5910472197813,14.6118220137849,0.));
#114735=CARTESIAN_POINT('Ctrl Pts',(71.5910472197813,14.6118220137849,12.));
#114736=CARTESIAN_POINT('Ctrl Pts',(71.612575518229,14.626205346737,0.));
#114737=CARTESIAN_POINT('Ctrl Pts',(71.612575518229,14.626205346737,12.));
#114738=CARTESIAN_POINT('Ctrl Pts',(71.6341221457169,14.6406301440814,0.));
#114739=CARTESIAN_POINT('Ctrl Pts',(71.6341221457169,14.6406301440814,12.));
#114740=CARTESIAN_POINT('Ctrl Pts',(71.6556869911662,14.6550963938829,0.));
#114741=CARTESIAN_POINT('Ctrl Pts',(71.6556869911662,14.6550963938829,12.));
#114742=CARTESIAN_POINT('Ctrl Pts',(71.6772699438963,14.6696040841678,0.));
#114743=CARTESIAN_POINT('Ctrl Pts',(71.6772699438963,14.6696040841678,12.));
#114744=CARTESIAN_POINT('Ctrl Pts',(71.6988708936172,14.6841532029232,0.));
#114745=CARTESIAN_POINT('Ctrl Pts',(71.6988708936172,14.6841532029232,12.));
#114746=CARTESIAN_POINT('Ctrl Pts',(71.7204897304194,14.6987437380901,0.));
#114747=CARTESIAN_POINT('Ctrl Pts',(71.7204897304194,14.6987437380901,12.));
#114748=CARTESIAN_POINT('Ctrl Pts',(71.7421263447719,14.7133756775626,0.));
#114749=CARTESIAN_POINT('Ctrl Pts',(71.7421263447719,14.7133756775626,12.));
#114750=CARTESIAN_POINT('Ctrl Pts',(71.7637806275328,14.7280490091957,0.));
#114751=CARTESIAN_POINT('Ctrl Pts',(71.7637806275328,14.7280490091957,12.));
#114752=CARTESIAN_POINT('Ctrl Pts',(71.7854524699569,14.7427637208073,0.));
#114753=CARTESIAN_POINT('Ctrl Pts',(71.7854524699569,14.7427637208073,12.));
#114754=CARTESIAN_POINT('Ctrl Pts',(71.8071417637017,14.7575198001776,0.));
#114755=CARTESIAN_POINT('Ctrl Pts',(71.8071417637017,14.7575198001776,12.));
#114756=CARTESIAN_POINT('Ctrl Pts',(71.8288484008333,14.7723172350451,0.));
#114757=CARTESIAN_POINT('Ctrl Pts',(71.8288484008333,14.7723172350451,12.));
#114758=CARTESIAN_POINT('Ctrl Pts',(71.8505722738272,14.7871560131017,0.));
#114759=CARTESIAN_POINT('Ctrl Pts',(71.8505722738272,14.7871560131017,12.));
#114760=CARTESIAN_POINT('Ctrl Pts',(71.8723132755446,14.8020361219998,0.));
#114761=CARTESIAN_POINT('Ctrl Pts',(71.8723132755446,14.8020361219998,12.));
#114762=CARTESIAN_POINT('Ctrl Pts',(71.8940712992109,14.8169575493557,0.));
#114763=CARTESIAN_POINT('Ctrl Pts',(71.8940712992109,14.8169575493557,12.));
#114764=CARTESIAN_POINT('Ctrl Pts',(71.9158462383914,14.8319202827482,0.));
#114765=CARTESIAN_POINT('Ctrl Pts',(71.9158462383914,14.8319202827482,12.));
#114766=CARTESIAN_POINT('Ctrl Pts',(71.9376379869678,14.8469243097163,0.));
#114767=CARTESIAN_POINT('Ctrl Pts',(71.9376379869678,14.8469243097163,12.));
#114768=CARTESIAN_POINT('Ctrl Pts',(71.9594464391078,14.8619696177507,0.));
#114769=CARTESIAN_POINT('Ctrl Pts',(71.9594464391078,14.8619696177507,12.));
#114770=CARTESIAN_POINT('Ctrl Pts',(71.9812714893102,14.8770561943014,0.));
#114771=CARTESIAN_POINT('Ctrl Pts',(71.9812714893102,14.8770561943014,12.));
#114772=CARTESIAN_POINT('Ctrl Pts',(72.0031130324529,14.8921840267832,0.));
#114773=CARTESIAN_POINT('Ctrl Pts',(72.0031130324529,14.8921840267832,12.));
#114774=CARTESIAN_POINT('Ctrl Pts',(72.0249709638422,14.9073531025764,0.));
#114775=CARTESIAN_POINT('Ctrl Pts',(72.0249709638422,14.9073531025764,12.));
#114776=CARTESIAN_POINT('Ctrl Pts',(72.0468451792505,14.9225634090268,0.));
#114777=CARTESIAN_POINT('Ctrl Pts',(72.0468451792505,14.9225634090268,12.));
#114778=CARTESIAN_POINT('Ctrl Pts',(72.0687355749807,14.9378149334388,0.));
#114779=CARTESIAN_POINT('Ctrl Pts',(72.0687355749807,14.9378149334388,12.));
#114780=CARTESIAN_POINT('Ctrl Pts',(72.0906420478076,14.9531076630768,0.));
#114781=CARTESIAN_POINT('Ctrl Pts',(72.0906420478076,14.9531076630768,12.));
#114782=CARTESIAN_POINT('Ctrl Pts',(72.112564494854,14.9684415851698,0.));
#114783=CARTESIAN_POINT('Ctrl Pts',(72.112564494854,14.9684415851698,12.));
#114784=CARTESIAN_POINT('Ctrl Pts',(72.1345028134777,14.9838166869107,0.));
#114785=CARTESIAN_POINT('Ctrl Pts',(72.1345028134777,14.9838166869107,12.));
#114786=CARTESIAN_POINT('Ctrl Pts',(72.1564569011669,14.9992329554537,0.));
#114787=CARTESIAN_POINT('Ctrl Pts',(72.1564569011669,14.9992329554537,12.));
#114788=CARTESIAN_POINT('Ctrl Pts',(72.1784266553953,15.0146903779062,0.));
#114789=CARTESIAN_POINT('Ctrl Pts',(72.1784266553953,15.0146903779062,12.));
#114790=CARTESIAN_POINT('Ctrl Pts',(72.2004119736115,15.0301889413257,0.));
#114791=CARTESIAN_POINT('Ctrl Pts',(72.2004119736115,15.0301889413257,12.));
#114792=CARTESIAN_POINT('Ctrl Pts',(72.2224127535415,15.0457286327331,0.));
#114793=CARTESIAN_POINT('Ctrl Pts',(72.2224127535415,15.0457286327331,12.));
#114794=CARTESIAN_POINT('Ctrl Pts',(72.2444288934262,15.0613094391189,0.));
#114795=CARTESIAN_POINT('Ctrl Pts',(72.2444288934262,15.0613094391189,12.));
#114796=CARTESIAN_POINT('Ctrl Pts',(72.2664602922852,15.0769313474477,0.));
#114797=CARTESIAN_POINT('Ctrl Pts',(72.2664602922852,15.0769313474477,12.));
#114798=CARTESIAN_POINT('Ctrl Pts',(72.2885068501628,15.092594344659,0.));
#114799=CARTESIAN_POINT('Ctrl Pts',(72.2885068501628,15.092594344659,12.));
#114800=CARTESIAN_POINT('Ctrl Pts',(72.3105684683944,15.1082984176649,0.));
#114801=CARTESIAN_POINT('Ctrl Pts',(72.3105684683944,15.1082984176649,12.));
#114802=CARTESIAN_POINT('Ctrl Pts',(72.3326450490177,15.124043553347,0.));
#114803=CARTESIAN_POINT('Ctrl Pts',(72.3326450490177,15.124043553347,12.));
#114804=CARTESIAN_POINT('Ctrl Pts',(72.3547364941969,15.1398297385506,0.));
#114805=CARTESIAN_POINT('Ctrl Pts',(72.3547364941969,15.1398297385506,12.));
#114806=CARTESIAN_POINT('Ctrl Pts',(72.376842705589,15.1556569600745,0.));
#114807=CARTESIAN_POINT('Ctrl Pts',(72.376842705589,15.1556569600745,12.));
#114808=CARTESIAN_POINT('Ctrl Pts',(72.3989635838492,15.1715252046606,0.));
#114809=CARTESIAN_POINT('Ctrl Pts',(72.3989635838492,15.1715252046606,12.));
#114810=CARTESIAN_POINT('Ctrl Pts',(72.421099027786,15.1874344589726,0.));
#114811=CARTESIAN_POINT('Ctrl Pts',(72.421099027786,15.1874344589726,12.));
#114812=CARTESIAN_POINT('Ctrl Pts',(72.4432489350471,15.2033847096091,0.));
#114813=CARTESIAN_POINT('Ctrl Pts',(72.4432489350471,15.2033847096091,12.));
#114814=CARTESIAN_POINT('Ctrl Pts',(72.4654132036428,15.2193759431373,0.));
#114815=CARTESIAN_POINT('Ctrl Pts',(72.4654132036428,15.2193759431373,12.));
#114816=CARTESIAN_POINT('Ctrl Pts',(72.4875917332762,15.235408146116,0.));
#114817=CARTESIAN_POINT('Ctrl Pts',(72.4875917332762,15.235408146116,12.));
#114818=CARTESIAN_POINT('Ctrl Pts',(72.5097844266075,15.2514813051172,0.));
#114819=CARTESIAN_POINT('Ctrl Pts',(72.5097844266075,15.2514813051172,12.));
#114820=CARTESIAN_POINT('Ctrl Pts',(72.5319911908917,15.2675954067479,0.));
#114821=CARTESIAN_POINT('Ctrl Pts',(72.5319911908917,15.2675954067479,12.));
#114822=CARTESIAN_POINT('Ctrl Pts',(72.5542119383642,15.2837504376536,0.));
#114823=CARTESIAN_POINT('Ctrl Pts',(72.5542119383642,15.2837504376536,12.));
#114824=CARTESIAN_POINT('Ctrl Pts',(72.5764465826224,15.2999463844661,0.));
#114825=CARTESIAN_POINT('Ctrl Pts',(72.5764465826224,15.2999463844661,12.));
#114826=CARTESIAN_POINT('Ctrl Pts',(72.5986950357677,15.3161832337594,0.));
#114827=CARTESIAN_POINT('Ctrl Pts',(72.5986950357677,15.3161832337594,12.));
#114828=CARTESIAN_POINT('Ctrl Pts',(72.6209572051042,15.3324609719956,0.));
#114829=CARTESIAN_POINT('Ctrl Pts',(72.6209572051042,15.3324609719956,12.));
#114830=CARTESIAN_POINT('Ctrl Pts',(72.6432329903553,15.3487795854745,0.));
#114831=CARTESIAN_POINT('Ctrl Pts',(72.6432329903553,15.3487795854745,12.));
#114832=CARTESIAN_POINT('Ctrl Pts',(72.6655222797801,15.3651390602666,0.));
#114833=CARTESIAN_POINT('Ctrl Pts',(72.6655222797801,15.3651390602666,12.));
#114834=CARTESIAN_POINT('Ctrl Pts',(72.687824955772,15.3815393822736,0.));
#114835=CARTESIAN_POINT('Ctrl Pts',(72.687824955772,15.3815393822736,12.));
#114836=CARTESIAN_POINT('Ctrl Pts',(72.7101409017716,15.3979805373174,0.));
#114837=CARTESIAN_POINT('Ctrl Pts',(72.7101409017716,15.3979805373174,12.));
#114838=CARTESIAN_POINT('Ctrl Pts',(72.7324700089712,15.4144625111944,0.));
#114839=CARTESIAN_POINT('Ctrl Pts',(72.7324700089712,15.4144625111944,12.));
#114840=CARTESIAN_POINT('Ctrl Pts',(72.7548121825342,15.4309852897844,0.));
#114841=CARTESIAN_POINT('Ctrl Pts',(72.7548121825342,15.4309852897844,12.));
#114842=CARTESIAN_POINT('Ctrl Pts',(72.777167349421,15.4475488590244,0.));
#114843=CARTESIAN_POINT('Ctrl Pts',(72.777167349421,15.4475488590244,12.));
#114844=CARTESIAN_POINT('Ctrl Pts',(72.7995354603795,15.4641532053281,0.));
#114845=CARTESIAN_POINT('Ctrl Pts',(72.7995354603795,15.4641532053281,12.));
#114846=CARTESIAN_POINT('Ctrl Pts',(72.8219164843279,15.4807983165804,0.));
#114847=CARTESIAN_POINT('Ctrl Pts',(72.8219164843279,15.4807983165804,12.));
#114848=CARTESIAN_POINT('Ctrl Pts',(72.8398316205897,15.494147009702,0.));
#114849=CARTESIAN_POINT('Ctrl Pts',(72.8398316205897,15.494147009702,12.));
#114850=CARTESIAN_POINT('Ctrl Pts',(72.8532737731759,15.5041768663999,0.));
#114851=CARTESIAN_POINT('Ctrl Pts',(72.8532737731759,15.5041768663999,12.));
#114852=CARTESIAN_POINT('Ctrl Pts',(72.8622377860824,15.5108715869141,0.));
#114853=CARTESIAN_POINT('Ctrl Pts',(72.8622377860824,15.5108715869141,12.));
#114854=CARTESIAN_POINT('Ctrl Pts',(72.8667204369977,15.5142209845168,0.));
#114855=CARTESIAN_POINT('Ctrl Pts',(72.8667204369977,15.5142209845168,12.));
#114856=CARTESIAN_POINT('',(68.7831490561748,12.9953224629497,0.));
#114857=CARTESIAN_POINT('Ctrl Pts',(68.7831490561748,12.9953224629497,0.));
#114858=CARTESIAN_POINT('Ctrl Pts',(68.7866525680193,12.9969981460277,0.));
#114859=CARTESIAN_POINT('Ctrl Pts',(68.7936635625545,13.0003537683055,0.));
#114860=CARTESIAN_POINT('Ctrl Pts',(68.804191966902,13.0053999700875,0.));
#114861=CARTESIAN_POINT('Ctrl Pts',(68.8182536653656,13.0121537768946,0.));
#114862=CARTESIAN_POINT('Ctrl Pts',(68.8358704887468,13.0206386039691,0.));
#114863=CARTESIAN_POINT('Ctrl Pts',(68.8535269726793,13.0291660060107,0.));
#114864=CARTESIAN_POINT('Ctrl Pts',(68.8712230321906,13.0377359881875,0.));
#114865=CARTESIAN_POINT('Ctrl Pts',(68.8889585151585,13.0463485518207,0.));
#114866=CARTESIAN_POINT('Ctrl Pts',(68.9067332040985,13.0550036938813,0.));
#114867=CARTESIAN_POINT('Ctrl Pts',(68.9245468449945,13.0637014089029,0.));
#114868=CARTESIAN_POINT('Ctrl Pts',(68.9423991694492,13.072441690283,0.));
#114869=CARTESIAN_POINT('Ctrl Pts',(68.9602899187573,13.0812245317808,0.));
#114870=CARTESIAN_POINT('Ctrl Pts',(68.9782188692581,13.090049929053,0.));
#114871=CARTESIAN_POINT('Ctrl Pts',(68.9961858241519,13.0989178791834,0.));
#114872=CARTESIAN_POINT('Ctrl Pts',(69.0141906015113,13.1078283799722,0.));
#114873=CARTESIAN_POINT('Ctrl Pts',(69.0322330243348,13.1167814293497,0.));
#114874=CARTESIAN_POINT('Ctrl Pts',(69.0503129081817,13.1257770246386,0.));
#114875=CARTESIAN_POINT('Ctrl Pts',(69.0684300549477,13.1348151621834,0.));
#114876=CARTESIAN_POINT('Ctrl Pts',(69.0865842593102,13.1438958377404,0.));
#114877=CARTESIAN_POINT('Ctrl Pts',(69.1047753127643,13.1530190467183,0.));
#114878=CARTESIAN_POINT('Ctrl Pts',(69.1230030082573,13.1621847844528,0.));
#114879=CARTESIAN_POINT('Ctrl Pts',(69.1412671454564,13.1713930465133,0.));
#114880=CARTESIAN_POINT('Ctrl Pts',(69.1595675305245,13.1806438286934,0.));
#114881=CARTESIAN_POINT('Ctrl Pts',(69.1779039735996,13.1899371268683,0.));
#114882=CARTESIAN_POINT('Ctrl Pts',(69.1962762870527,13.1992729368929,0.));
#114883=CARTESIAN_POINT('Ctrl Pts',(69.2146842833537,13.2086512544735,0.));
#114884=CARTESIAN_POINT('Ctrl Pts',(69.2331277732861,13.2180720750594,0.));
#114885=CARTESIAN_POINT('Ctrl Pts',(69.2516065668844,13.2275353939051,0.));
#114886=CARTESIAN_POINT('Ctrl Pts',(69.270120474245,13.237041206122,0.));
#114887=CARTESIAN_POINT('Ctrl Pts',(69.2886693063182,13.2465895067262,0.));
#114888=CARTESIAN_POINT('Ctrl Pts',(69.3072528758518,13.2561802906896,0.));
#114889=CARTESIAN_POINT('Ctrl Pts',(69.3258709977382,13.265813552961,0.));
#114890=CARTESIAN_POINT('Ctrl Pts',(69.3445234885065,13.2754892884433,0.));
#114891=CARTESIAN_POINT('Ctrl Pts',(69.3632101660066,13.2852074919766,0.));
#114892=CARTESIAN_POINT('Ctrl Pts',(69.3819308490422,13.2949681583167,0.));
#114893=CARTESIAN_POINT('Ctrl Pts',(69.4006853569511,13.3047712821051,0.));
#114894=CARTESIAN_POINT('Ctrl Pts',(69.4194735096265,13.3146168578743,0.));
#114895=CARTESIAN_POINT('Ctrl Pts',(69.4382951276998,13.3245048800643,0.));
#114896=CARTESIAN_POINT('Ctrl Pts',(69.4571500326673,13.3344353430313,0.));
#114897=CARTESIAN_POINT('Ctrl Pts',(69.4760380470365,13.3444082410543,0.));
#114898=CARTESIAN_POINT('Ctrl Pts',(69.4949589944606,13.3544235683394,0.));
#114899=CARTESIAN_POINT('Ctrl Pts',(69.5139126996675,13.3644813190219,0.));
#114900=CARTESIAN_POINT('Ctrl Pts',(69.5328989883885,13.3745814871665,0.));
#114901=CARTESIAN_POINT('Ctrl Pts',(69.5519176872862,13.3847240667628,0.));
#114902=CARTESIAN_POINT('Ctrl Pts',(69.5709686238724,13.3949090517177,0.));
#114903=CARTESIAN_POINT('Ctrl Pts',(69.5900516264553,13.40513643585,0.));
#114904=CARTESIAN_POINT('Ctrl Pts',(69.6091665241765,13.4154062129002,0.));
#114905=CARTESIAN_POINT('Ctrl Pts',(69.6283131470273,13.4257183765341,0.));
#114906=CARTESIAN_POINT('Ctrl Pts',(69.6474913258675,13.4360729203442,0.));
#114907=CARTESIAN_POINT('Ctrl Pts',(69.666700892444,13.4464698378453,0.));
#114908=CARTESIAN_POINT('Ctrl Pts',(69.6859416793885,13.456909122476,0.));
#114909=CARTESIAN_POINT('Ctrl Pts',(69.7052135201998,13.4673907676044,0.));
#114910=CARTESIAN_POINT('Ctrl Pts',(69.724516249225,13.4779147665285,0.));
#114911=CARTESIAN_POINT('Ctrl Pts',(69.7438497016406,13.4884811124748,0.));
#114912=CARTESIAN_POINT('Ctrl Pts',(69.7632137134249,13.4990897985905,0.));
#114913=CARTESIAN_POINT('Ctrl Pts',(69.7826081213576,13.5097408179479,0.));
#114914=CARTESIAN_POINT('Ctrl Pts',(69.8020327630205,13.5204341635507,0.));
#114915=CARTESIAN_POINT('Ctrl Pts',(69.8214874767944,13.5311698283339,0.));
#114916=CARTESIAN_POINT('Ctrl Pts',(69.840972101856,13.5419478051625,0.));
#114917=CARTESIAN_POINT('Ctrl Pts',(69.8604864781706,13.5527680868255,0.));
#114918=CARTESIAN_POINT('Ctrl Pts',(69.8800304464882,13.5636306660422,0.));
#114919=CARTESIAN_POINT('Ctrl Pts',(69.8996038483361,13.5745355354657,0.));
#114920=CARTESIAN_POINT('Ctrl Pts',(69.9192065260108,13.5854826876835,0.));
#114921=CARTESIAN_POINT('Ctrl Pts',(69.9388383225648,13.5964721152135,0.));
#114922=CARTESIAN_POINT('Ctrl Pts',(69.9584990817974,13.6075038104999,0.));
#114923=CARTESIAN_POINT('Ctrl Pts',(69.9781886482528,13.6185777659198,0.));
#114924=CARTESIAN_POINT('Ctrl Pts',(69.9979068672153,13.6296939737865,0.));
#114925=CARTESIAN_POINT('Ctrl Pts',(70.0176535847049,13.6408524263496,0.));
#114926=CARTESIAN_POINT('Ctrl Pts',(70.0374286474677,13.6520531157907,0.));
#114927=CARTESIAN_POINT('Ctrl Pts',(70.0572319029676,13.6632960342196,0.));
#114928=CARTESIAN_POINT('Ctrl Pts',(70.0770631993856,13.674581173683,0.));
#114929=CARTESIAN_POINT('Ctrl Pts',(70.0969223856136,13.6859085261653,0.));
#114930=CARTESIAN_POINT('Ctrl Pts',(70.1168093112486,13.6972780835897,0.));
#114931=CARTESIAN_POINT('Ctrl Pts',(70.1367238265825,13.7086898378122,0.));
#114932=CARTESIAN_POINT('Ctrl Pts',(70.156665782595,13.7201437806199,0.));
#114933=CARTESIAN_POINT('Ctrl Pts',(70.1766350309518,13.7316399037393,0.));
#114934=CARTESIAN_POINT('Ctrl Pts',(70.1966314239995,13.7431781988365,0.));
#114935=CARTESIAN_POINT('Ctrl Pts',(70.2166548147604,13.7547586575181,0.));
#114936=CARTESIAN_POINT('Ctrl Pts',(70.2367050569216,13.7663812713243,0.));
#114937=CARTESIAN_POINT('Ctrl Pts',(70.2567820048303,13.7780460317294,0.));
#114938=CARTESIAN_POINT('Ctrl Pts',(70.2768855134947,13.7897529301491,0.));
#114939=CARTESIAN_POINT('Ctrl Pts',(70.2970154385774,13.8015019579414,0.));
#114940=CARTESIAN_POINT('Ctrl Pts',(70.3171716363897,13.8132931064064,0.));
#114941=CARTESIAN_POINT('Ctrl Pts',(70.3373539638809,13.8251263667791,0.));
#114942=CARTESIAN_POINT('Ctrl Pts',(70.3575622786335,13.8370017302309,0.));
#114943=CARTESIAN_POINT('Ctrl Pts',(70.3777964388632,13.8489191878767,0.));
#114944=CARTESIAN_POINT('Ctrl Pts',(70.3980563034133,13.8608787307752,0.));
#114945=CARTESIAN_POINT('Ctrl Pts',(70.41834173175,13.8728803499287,0.));
#114946=CARTESIAN_POINT('Ctrl Pts',(70.4386525839521,13.8849240362763,0.));
#114947=CARTESIAN_POINT('Ctrl Pts',(70.4589887207073,13.8970097806954,0.));
#114948=CARTESIAN_POINT('Ctrl Pts',(70.4793500033124,13.9091375740088,0.));
#114949=CARTESIAN_POINT('Ctrl Pts',(70.4997362936673,13.9213074069853,0.));
#114950=CARTESIAN_POINT('Ctrl Pts',(70.520147454271,13.9335192703388,0.));
#114951=CARTESIAN_POINT('Ctrl Pts',(70.5405833482112,13.9457731547215,0.));
#114952=CARTESIAN_POINT('Ctrl Pts',(70.5610438391612,13.958069050726,0.));
#114953=CARTESIAN_POINT('Ctrl Pts',(70.5815287913784,13.9704069488917,0.));
#114954=CARTESIAN_POINT('Ctrl Pts',(70.6020380697005,13.9827868397057,0.));
#114955=CARTESIAN_POINT('Ctrl Pts',(70.6225715395394,13.9952087136018,0.));
#114956=CARTESIAN_POINT('Ctrl Pts',(70.6431290668745,14.0076725609537,0.));
#114957=CARTESIAN_POINT('Ctrl Pts',(70.6637105182484,14.020178372077,0.));
#114958=CARTESIAN_POINT('Ctrl Pts',(70.6843157607668,14.0327261372362,0.));
#114959=CARTESIAN_POINT('Ctrl Pts',(70.7049446620928,14.0453158466451,0.));
#114960=CARTESIAN_POINT('Ctrl Pts',(70.7255970904436,14.0579474904657,0.));
#114961=CARTESIAN_POINT('Ctrl Pts',(70.7462729145807,14.0706210588016,0.));
#114962=CARTESIAN_POINT('Ctrl Pts',(70.7669720038077,14.0833365416996,0.));
#114963=CARTESIAN_POINT('Ctrl Pts',(70.7876942279697,14.0960939291569,0.));
#114964=CARTESIAN_POINT('Ctrl Pts',(70.8084394574493,14.1088932111214,0.));
#114965=CARTESIAN_POINT('Ctrl Pts',(70.8292075631621,14.1217343774913,0.));
#114966=CARTESIAN_POINT('Ctrl Pts',(70.8499984165489,14.1346174181079,0.));
#114967=CARTESIAN_POINT('Ctrl Pts',(70.8708118895715,14.1475423227568,0.));
#114968=CARTESIAN_POINT('Ctrl Pts',(70.8916478547132,14.1605090811754,0.));
#114969=CARTESIAN_POINT('Ctrl Pts',(70.9125061849745,14.1735176830533,0.));
#114970=CARTESIAN_POINT('Ctrl Pts',(70.9333867538704,14.1865681180321,0.));
#114971=CARTESIAN_POINT('Ctrl Pts',(70.9542894354216,14.1996603756982,0.));
#114972=CARTESIAN_POINT('Ctrl Pts',(70.9752141041518,14.2127944455839,0.));
#114973=CARTESIAN_POINT('Ctrl Pts',(70.9961606350861,14.2259703171737,0.));
#114974=CARTESIAN_POINT('Ctrl Pts',(71.0171289037488,14.2391879799062,0.));
#114975=CARTESIAN_POINT('Ctrl Pts',(71.0381187861588,14.2524474231733,0.));
#114976=CARTESIAN_POINT('Ctrl Pts',(71.0591301588231,14.2657486363139,0.));
#114977=CARTESIAN_POINT('Ctrl Pts',(71.0801628987332,14.2790916086133,0.));
#114978=CARTESIAN_POINT('Ctrl Pts',(71.1012168833643,14.2924763293105,0.));
#114979=CARTESIAN_POINT('Ctrl Pts',(71.1222919906727,14.3059027875994,0.));
#114980=CARTESIAN_POINT('Ctrl Pts',(71.1433880990929,14.3193709726294,0.));
#114981=CARTESIAN_POINT('Ctrl Pts',(71.1645050875308,14.332880873499,0.));
#114982=CARTESIAN_POINT('Ctrl Pts',(71.1856428353593,14.3464324792534,0.));
#114983=CARTESIAN_POINT('Ctrl Pts',(71.2068012224174,14.3600257788924,0.));
#114984=CARTESIAN_POINT('Ctrl Pts',(71.2279801290084,14.3736607613722,0.));
#114985=CARTESIAN_POINT('Ctrl Pts',(71.2491794358958,14.3873374156056,0.));
#114986=CARTESIAN_POINT('Ctrl Pts',(71.2703990242988,14.401055730457,0.));
#114987=CARTESIAN_POINT('Ctrl Pts',(71.2916387758861,14.4148156947384,0.));
#114988=CARTESIAN_POINT('Ctrl Pts',(71.312898572777,14.4286172972167,0.));
#114989=CARTESIAN_POINT('Ctrl Pts',(71.3341782975386,14.4424605266165,0.));
#114990=CARTESIAN_POINT('Ctrl Pts',(71.3554778331835,14.4563453716204,0.));
#114991=CARTESIAN_POINT('Ctrl Pts',(71.376797063165,14.4702718208651,0.));
#114992=CARTESIAN_POINT('Ctrl Pts',(71.3981358713723,14.4842398629355,0.));
#114993=CARTESIAN_POINT('Ctrl Pts',(71.4194941421292,14.4982494863718,0.));
#114994=CARTESIAN_POINT('Ctrl Pts',(71.4408717601923,14.5123006796728,0.));
#114995=CARTESIAN_POINT('Ctrl Pts',(71.4622686107475,14.5263934312969,0.));
#114996=CARTESIAN_POINT('Ctrl Pts',(71.4836845794048,14.540527729659,0.));
#114997=CARTESIAN_POINT('Ctrl Pts',(71.5051195521909,14.5547035631234,0.));
#114998=CARTESIAN_POINT('Ctrl Pts',(71.5265734155498,14.5689209200091,0.));
#114999=CARTESIAN_POINT('Ctrl Pts',(71.5480460563447,14.5831797885952,0.));
#115000=CARTESIAN_POINT('Ctrl Pts',(71.5695373618562,14.597480157121,0.));
#115001=CARTESIAN_POINT('Ctrl Pts',(71.5910472197813,14.6118220137849,0.));
#115002=CARTESIAN_POINT('Ctrl Pts',(71.612575518229,14.626205346737,0.));
#115003=CARTESIAN_POINT('Ctrl Pts',(71.6341221457169,14.6406301440814,0.));
#115004=CARTESIAN_POINT('Ctrl Pts',(71.6556869911662,14.6550963938829,0.));
#115005=CARTESIAN_POINT('Ctrl Pts',(71.6772699438963,14.6696040841678,0.));
#115006=CARTESIAN_POINT('Ctrl Pts',(71.6988708936172,14.6841532029232,0.));
#115007=CARTESIAN_POINT('Ctrl Pts',(71.7204897304194,14.6987437380901,0.));
#115008=CARTESIAN_POINT('Ctrl Pts',(71.7421263447719,14.7133756775626,0.));
#115009=CARTESIAN_POINT('Ctrl Pts',(71.7637806275328,14.7280490091957,0.));
#115010=CARTESIAN_POINT('Ctrl Pts',(71.7854524699569,14.7427637208073,0.));
#115011=CARTESIAN_POINT('Ctrl Pts',(71.8071417637017,14.7575198001776,0.));
#115012=CARTESIAN_POINT('Ctrl Pts',(71.8288484008333,14.7723172350451,0.));
#115013=CARTESIAN_POINT('Ctrl Pts',(71.8505722738272,14.7871560131017,0.));
#115014=CARTESIAN_POINT('Ctrl Pts',(71.8723132755446,14.8020361219998,0.));
#115015=CARTESIAN_POINT('Ctrl Pts',(71.8940712992109,14.8169575493557,0.));
#115016=CARTESIAN_POINT('Ctrl Pts',(71.9158462383914,14.8319202827482,0.));
#115017=CARTESIAN_POINT('Ctrl Pts',(71.9376379869678,14.8469243097163,0.));
#115018=CARTESIAN_POINT('Ctrl Pts',(71.9594464391078,14.8619696177507,0.));
#115019=CARTESIAN_POINT('Ctrl Pts',(71.9812714893102,14.8770561943014,0.));
#115020=CARTESIAN_POINT('Ctrl Pts',(72.0031130324529,14.8921840267832,0.));
#115021=CARTESIAN_POINT('Ctrl Pts',(72.0249709638422,14.9073531025764,0.));
#115022=CARTESIAN_POINT('Ctrl Pts',(72.0468451792505,14.9225634090268,0.));
#115023=CARTESIAN_POINT('Ctrl Pts',(72.0687355749807,14.9378149334388,0.));
#115024=CARTESIAN_POINT('Ctrl Pts',(72.0906420478076,14.9531076630768,0.));
#115025=CARTESIAN_POINT('Ctrl Pts',(72.112564494854,14.9684415851698,0.));
#115026=CARTESIAN_POINT('Ctrl Pts',(72.1345028134777,14.9838166869107,0.));
#115027=CARTESIAN_POINT('Ctrl Pts',(72.1564569011669,14.9992329554537,0.));
#115028=CARTESIAN_POINT('Ctrl Pts',(72.1784266553953,15.0146903779062,0.));
#115029=CARTESIAN_POINT('Ctrl Pts',(72.2004119736115,15.0301889413257,0.));
#115030=CARTESIAN_POINT('Ctrl Pts',(72.2224127535415,15.0457286327331,0.));
#115031=CARTESIAN_POINT('Ctrl Pts',(72.2444288934262,15.0613094391189,0.));
#115032=CARTESIAN_POINT('Ctrl Pts',(72.2664602922852,15.0769313474477,0.));
#115033=CARTESIAN_POINT('Ctrl Pts',(72.2885068501628,15.092594344659,0.));
#115034=CARTESIAN_POINT('Ctrl Pts',(72.3105684683944,15.1082984176649,0.));
#115035=CARTESIAN_POINT('Ctrl Pts',(72.3326450490177,15.124043553347,0.));
#115036=CARTESIAN_POINT('Ctrl Pts',(72.3547364941969,15.1398297385506,0.));
#115037=CARTESIAN_POINT('Ctrl Pts',(72.376842705589,15.1556569600745,0.));
#115038=CARTESIAN_POINT('Ctrl Pts',(72.3989635838492,15.1715252046606,0.));
#115039=CARTESIAN_POINT('Ctrl Pts',(72.421099027786,15.1874344589726,0.));
#115040=CARTESIAN_POINT('Ctrl Pts',(72.4432489350471,15.2033847096091,0.));
#115041=CARTESIAN_POINT('Ctrl Pts',(72.4654132036428,15.2193759431373,0.));
#115042=CARTESIAN_POINT('Ctrl Pts',(72.4875917332762,15.235408146116,0.));
#115043=CARTESIAN_POINT('Ctrl Pts',(72.5097844266075,15.2514813051172,0.));
#115044=CARTESIAN_POINT('Ctrl Pts',(72.5319911908917,15.2675954067479,0.));
#115045=CARTESIAN_POINT('Ctrl Pts',(72.5542119383642,15.2837504376536,0.));
#115046=CARTESIAN_POINT('Ctrl Pts',(72.5732713370618,15.297633502478,0.));
#115047=CARTESIAN_POINT('Ctrl Pts',(72.5878912620439,15.3082994603539,0.));
#115048=CARTESIAN_POINT('Ctrl Pts',(72.5980655789635,15.3157301930682,0.));
#115049=CARTESIAN_POINT('Ctrl Pts',(72.6037902604921,15.3199137230129,0.));
#115050=CARTESIAN_POINT('Ctrl Pts',(72.6050633494351,15.3208442077189,0.));
#115051=CARTESIAN_POINT('',(68.7831490561748,12.9953224629497,12.));
#115052=CARTESIAN_POINT('',(68.7831490561748,12.9953224629497,0.));
#115053=CARTESIAN_POINT('Ctrl Pts',(72.6050633494351,15.3208442077189,12.));
#115054=CARTESIAN_POINT('Ctrl Pts',(72.6037902604921,15.3199137230129,12.));
#115055=CARTESIAN_POINT('Ctrl Pts',(72.5980655789635,15.3157301930682,12.));
#115056=CARTESIAN_POINT('Ctrl Pts',(72.5878912620439,15.3082994603539,12.));
#115057=CARTESIAN_POINT('Ctrl Pts',(72.5732713370618,15.297633502478,12.));
#115058=CARTESIAN_POINT('Ctrl Pts',(72.5542119383642,15.2837504376536,12.));
#115059=CARTESIAN_POINT('Ctrl Pts',(72.5319911908917,15.2675954067479,12.));
#115060=CARTESIAN_POINT('Ctrl Pts',(72.5097844266075,15.2514813051172,12.));
#115061=CARTESIAN_POINT('Ctrl Pts',(72.4875917332762,15.235408146116,12.));
#115062=CARTESIAN_POINT('Ctrl Pts',(72.4654132036428,15.2193759431373,12.));
#115063=CARTESIAN_POINT('Ctrl Pts',(72.4432489350471,15.2033847096091,12.));
#115064=CARTESIAN_POINT('Ctrl Pts',(72.421099027786,15.1874344589726,12.));
#115065=CARTESIAN_POINT('Ctrl Pts',(72.3989635838492,15.1715252046606,12.));
#115066=CARTESIAN_POINT('Ctrl Pts',(72.376842705589,15.1556569600745,12.));
#115067=CARTESIAN_POINT('Ctrl Pts',(72.3547364941969,15.1398297385506,12.));
#115068=CARTESIAN_POINT('Ctrl Pts',(72.3326450490177,15.124043553347,12.));
#115069=CARTESIAN_POINT('Ctrl Pts',(72.3105684683944,15.1082984176649,12.));
#115070=CARTESIAN_POINT('Ctrl Pts',(72.2885068501628,15.092594344659,12.));
#115071=CARTESIAN_POINT('Ctrl Pts',(72.2664602922852,15.0769313474477,12.));
#115072=CARTESIAN_POINT('Ctrl Pts',(72.2444288934262,15.0613094391189,12.));
#115073=CARTESIAN_POINT('Ctrl Pts',(72.2224127535415,15.0457286327331,12.));
#115074=CARTESIAN_POINT('Ctrl Pts',(72.2004119736115,15.0301889413257,12.));
#115075=CARTESIAN_POINT('Ctrl Pts',(72.1784266553953,15.0146903779062,12.));
#115076=CARTESIAN_POINT('Ctrl Pts',(72.1564569011669,14.9992329554537,12.));
#115077=CARTESIAN_POINT('Ctrl Pts',(72.1345028134777,14.9838166869107,12.));
#115078=CARTESIAN_POINT('Ctrl Pts',(72.112564494854,14.9684415851698,12.));
#115079=CARTESIAN_POINT('Ctrl Pts',(72.0906420478076,14.9531076630768,12.));
#115080=CARTESIAN_POINT('Ctrl Pts',(72.0687355749807,14.9378149334388,12.));
#115081=CARTESIAN_POINT('Ctrl Pts',(72.0468451792505,14.9225634090268,12.));
#115082=CARTESIAN_POINT('Ctrl Pts',(72.0249709638422,14.9073531025764,12.));
#115083=CARTESIAN_POINT('Ctrl Pts',(72.0031130324529,14.8921840267832,12.));
#115084=CARTESIAN_POINT('Ctrl Pts',(71.9812714893102,14.8770561943014,12.));
#115085=CARTESIAN_POINT('Ctrl Pts',(71.9594464391078,14.8619696177507,12.));
#115086=CARTESIAN_POINT('Ctrl Pts',(71.9376379869678,14.8469243097163,12.));
#115087=CARTESIAN_POINT('Ctrl Pts',(71.9158462383914,14.8319202827482,12.));
#115088=CARTESIAN_POINT('Ctrl Pts',(71.8940712992109,14.8169575493557,12.));
#115089=CARTESIAN_POINT('Ctrl Pts',(71.8723132755446,14.8020361219998,12.));
#115090=CARTESIAN_POINT('Ctrl Pts',(71.8505722738272,14.7871560131017,12.));
#115091=CARTESIAN_POINT('Ctrl Pts',(71.8288484008333,14.7723172350451,12.));
#115092=CARTESIAN_POINT('Ctrl Pts',(71.8071417637017,14.7575198001776,12.));
#115093=CARTESIAN_POINT('Ctrl Pts',(71.7854524699569,14.7427637208073,12.));
#115094=CARTESIAN_POINT('Ctrl Pts',(71.7637806275328,14.7280490091957,12.));
#115095=CARTESIAN_POINT('Ctrl Pts',(71.7421263447719,14.7133756775626,12.));
#115096=CARTESIAN_POINT('Ctrl Pts',(71.7204897304194,14.6987437380901,12.));
#115097=CARTESIAN_POINT('Ctrl Pts',(71.6988708936172,14.6841532029232,12.));
#115098=CARTESIAN_POINT('Ctrl Pts',(71.6772699438963,14.6696040841678,12.));
#115099=CARTESIAN_POINT('Ctrl Pts',(71.6556869911662,14.6550963938829,12.));
#115100=CARTESIAN_POINT('Ctrl Pts',(71.6341221457169,14.6406301440814,12.));
#115101=CARTESIAN_POINT('Ctrl Pts',(71.612575518229,14.626205346737,12.));
#115102=CARTESIAN_POINT('Ctrl Pts',(71.5910472197813,14.6118220137849,12.));
#115103=CARTESIAN_POINT('Ctrl Pts',(71.5695373618562,14.597480157121,12.));
#115104=CARTESIAN_POINT('Ctrl Pts',(71.5480460563447,14.5831797885952,12.));
#115105=CARTESIAN_POINT('Ctrl Pts',(71.5265734155498,14.5689209200091,12.));
#115106=CARTESIAN_POINT('Ctrl Pts',(71.5051195521909,14.5547035631234,12.));
#115107=CARTESIAN_POINT('Ctrl Pts',(71.4836845794048,14.540527729659,12.));
#115108=CARTESIAN_POINT('Ctrl Pts',(71.4622686107475,14.5263934312969,12.));
#115109=CARTESIAN_POINT('Ctrl Pts',(71.4408717601923,14.5123006796728,12.));
#115110=CARTESIAN_POINT('Ctrl Pts',(71.4194941421292,14.4982494863718,12.));
#115111=CARTESIAN_POINT('Ctrl Pts',(71.3981358713723,14.4842398629355,12.));
#115112=CARTESIAN_POINT('Ctrl Pts',(71.376797063165,14.4702718208651,12.));
#115113=CARTESIAN_POINT('Ctrl Pts',(71.3554778331835,14.4563453716204,12.));
#115114=CARTESIAN_POINT('Ctrl Pts',(71.3341782975386,14.4424605266165,12.));
#115115=CARTESIAN_POINT('Ctrl Pts',(71.312898572777,14.4286172972167,12.));
#115116=CARTESIAN_POINT('Ctrl Pts',(71.2916387758861,14.4148156947384,12.));
#115117=CARTESIAN_POINT('Ctrl Pts',(71.2703990242988,14.401055730457,12.));
#115118=CARTESIAN_POINT('Ctrl Pts',(71.2491794358958,14.3873374156056,12.));
#115119=CARTESIAN_POINT('Ctrl Pts',(71.2279801290084,14.3736607613722,12.));
#115120=CARTESIAN_POINT('Ctrl Pts',(71.2068012224174,14.3600257788924,12.));
#115121=CARTESIAN_POINT('Ctrl Pts',(71.1856428353593,14.3464324792534,12.));
#115122=CARTESIAN_POINT('Ctrl Pts',(71.1645050875308,14.332880873499,12.));
#115123=CARTESIAN_POINT('Ctrl Pts',(71.1433880990929,14.3193709726294,12.));
#115124=CARTESIAN_POINT('Ctrl Pts',(71.1222919906727,14.3059027875994,12.));
#115125=CARTESIAN_POINT('Ctrl Pts',(71.1012168833643,14.2924763293105,12.));
#115126=CARTESIAN_POINT('Ctrl Pts',(71.0801628987332,14.2790916086133,12.));
#115127=CARTESIAN_POINT('Ctrl Pts',(71.0591301588231,14.2657486363139,12.));
#115128=CARTESIAN_POINT('Ctrl Pts',(71.0381187861588,14.2524474231733,12.));
#115129=CARTESIAN_POINT('Ctrl Pts',(71.0171289037488,14.2391879799062,12.));
#115130=CARTESIAN_POINT('Ctrl Pts',(70.9961606350861,14.2259703171737,12.));
#115131=CARTESIAN_POINT('Ctrl Pts',(70.9752141041518,14.2127944455839,12.));
#115132=CARTESIAN_POINT('Ctrl Pts',(70.9542894354216,14.1996603756982,12.));
#115133=CARTESIAN_POINT('Ctrl Pts',(70.9333867538704,14.1865681180321,12.));
#115134=CARTESIAN_POINT('Ctrl Pts',(70.9125061849745,14.1735176830533,12.));
#115135=CARTESIAN_POINT('Ctrl Pts',(70.8916478547132,14.1605090811754,12.));
#115136=CARTESIAN_POINT('Ctrl Pts',(70.8708118895715,14.1475423227568,12.));
#115137=CARTESIAN_POINT('Ctrl Pts',(70.8499984165489,14.1346174181079,12.));
#115138=CARTESIAN_POINT('Ctrl Pts',(70.8292075631621,14.1217343774913,12.));
#115139=CARTESIAN_POINT('Ctrl Pts',(70.8084394574493,14.1088932111214,12.));
#115140=CARTESIAN_POINT('Ctrl Pts',(70.7876942279697,14.0960939291569,12.));
#115141=CARTESIAN_POINT('Ctrl Pts',(70.7669720038077,14.0833365416996,12.));
#115142=CARTESIAN_POINT('Ctrl Pts',(70.7462729145807,14.0706210588016,12.));
#115143=CARTESIAN_POINT('Ctrl Pts',(70.7255970904436,14.0579474904657,12.));
#115144=CARTESIAN_POINT('Ctrl Pts',(70.7049446620928,14.0453158466451,12.));
#115145=CARTESIAN_POINT('Ctrl Pts',(70.6843157607668,14.0327261372362,12.));
#115146=CARTESIAN_POINT('Ctrl Pts',(70.6637105182484,14.020178372077,12.));
#115147=CARTESIAN_POINT('Ctrl Pts',(70.6431290668745,14.0076725609537,12.));
#115148=CARTESIAN_POINT('Ctrl Pts',(70.6225715395394,13.9952087136018,12.));
#115149=CARTESIAN_POINT('Ctrl Pts',(70.6020380697005,13.9827868397057,12.));
#115150=CARTESIAN_POINT('Ctrl Pts',(70.5815287913784,13.9704069488917,12.));
#115151=CARTESIAN_POINT('Ctrl Pts',(70.5610438391612,13.958069050726,12.));
#115152=CARTESIAN_POINT('Ctrl Pts',(70.5405833482112,13.9457731547215,12.));
#115153=CARTESIAN_POINT('Ctrl Pts',(70.520147454271,13.9335192703388,12.));
#115154=CARTESIAN_POINT('Ctrl Pts',(70.4997362936673,13.9213074069853,12.));
#115155=CARTESIAN_POINT('Ctrl Pts',(70.4793500033124,13.9091375740088,12.));
#115156=CARTESIAN_POINT('Ctrl Pts',(70.4589887207073,13.8970097806954,12.));
#115157=CARTESIAN_POINT('Ctrl Pts',(70.4386525839521,13.8849240362763,12.));
#115158=CARTESIAN_POINT('Ctrl Pts',(70.41834173175,13.8728803499287,12.));
#115159=CARTESIAN_POINT('Ctrl Pts',(70.3980563034133,13.8608787307752,12.));
#115160=CARTESIAN_POINT('Ctrl Pts',(70.3777964388632,13.8489191878767,12.));
#115161=CARTESIAN_POINT('Ctrl Pts',(70.3575622786335,13.8370017302309,12.));
#115162=CARTESIAN_POINT('Ctrl Pts',(70.3373539638809,13.8251263667791,12.));
#115163=CARTESIAN_POINT('Ctrl Pts',(70.3171716363897,13.8132931064064,12.));
#115164=CARTESIAN_POINT('Ctrl Pts',(70.2970154385774,13.8015019579414,12.));
#115165=CARTESIAN_POINT('Ctrl Pts',(70.2768855134947,13.7897529301491,12.));
#115166=CARTESIAN_POINT('Ctrl Pts',(70.2567820048303,13.7780460317294,12.));
#115167=CARTESIAN_POINT('Ctrl Pts',(70.2367050569216,13.7663812713243,12.));
#115168=CARTESIAN_POINT('Ctrl Pts',(70.2166548147604,13.7547586575181,12.));
#115169=CARTESIAN_POINT('Ctrl Pts',(70.1966314239995,13.7431781988365,12.));
#115170=CARTESIAN_POINT('Ctrl Pts',(70.1766350309518,13.7316399037393,12.));
#115171=CARTESIAN_POINT('Ctrl Pts',(70.156665782595,13.7201437806199,12.));
#115172=CARTESIAN_POINT('Ctrl Pts',(70.1367238265825,13.7086898378122,12.));
#115173=CARTESIAN_POINT('Ctrl Pts',(70.1168093112486,13.6972780835897,12.));
#115174=CARTESIAN_POINT('Ctrl Pts',(70.0969223856136,13.6859085261653,12.));
#115175=CARTESIAN_POINT('Ctrl Pts',(70.0770631993856,13.674581173683,12.));
#115176=CARTESIAN_POINT('Ctrl Pts',(70.0572319029676,13.6632960342196,12.));
#115177=CARTESIAN_POINT('Ctrl Pts',(70.0374286474677,13.6520531157907,12.));
#115178=CARTESIAN_POINT('Ctrl Pts',(70.0176535847049,13.6408524263496,12.));
#115179=CARTESIAN_POINT('Ctrl Pts',(69.9979068672153,13.6296939737865,12.));
#115180=CARTESIAN_POINT('Ctrl Pts',(69.9781886482528,13.6185777659198,12.));
#115181=CARTESIAN_POINT('Ctrl Pts',(69.9584990817974,13.6075038104999,12.));
#115182=CARTESIAN_POINT('Ctrl Pts',(69.9388383225648,13.5964721152135,12.));
#115183=CARTESIAN_POINT('Ctrl Pts',(69.9192065260108,13.5854826876835,12.));
#115184=CARTESIAN_POINT('Ctrl Pts',(69.8996038483361,13.5745355354657,12.));
#115185=CARTESIAN_POINT('Ctrl Pts',(69.8800304464882,13.5636306660422,12.));
#115186=CARTESIAN_POINT('Ctrl Pts',(69.8604864781706,13.5527680868255,12.));
#115187=CARTESIAN_POINT('Ctrl Pts',(69.840972101856,13.5419478051625,12.));
#115188=CARTESIAN_POINT('Ctrl Pts',(69.8214874767944,13.5311698283339,12.));
#115189=CARTESIAN_POINT('Ctrl Pts',(69.8020327630205,13.5204341635507,12.));
#115190=CARTESIAN_POINT('Ctrl Pts',(69.7826081213576,13.5097408179479,12.));
#115191=CARTESIAN_POINT('Ctrl Pts',(69.7632137134249,13.4990897985905,12.));
#115192=CARTESIAN_POINT('Ctrl Pts',(69.7438497016406,13.4884811124748,12.));
#115193=CARTESIAN_POINT('Ctrl Pts',(69.724516249225,13.4779147665285,12.));
#115194=CARTESIAN_POINT('Ctrl Pts',(69.7052135201998,13.4673907676044,12.));
#115195=CARTESIAN_POINT('Ctrl Pts',(69.6859416793885,13.456909122476,12.));
#115196=CARTESIAN_POINT('Ctrl Pts',(69.666700892444,13.4464698378453,12.));
#115197=CARTESIAN_POINT('Ctrl Pts',(69.6474913258675,13.4360729203442,12.));
#115198=CARTESIAN_POINT('Ctrl Pts',(69.6283131470273,13.4257183765341,12.));
#115199=CARTESIAN_POINT('Ctrl Pts',(69.6091665241765,13.4154062129002,12.));
#115200=CARTESIAN_POINT('Ctrl Pts',(69.5900516264553,13.40513643585,12.));
#115201=CARTESIAN_POINT('Ctrl Pts',(69.5709686238724,13.3949090517177,12.));
#115202=CARTESIAN_POINT('Ctrl Pts',(69.5519176872862,13.3847240667628,12.));
#115203=CARTESIAN_POINT('Ctrl Pts',(69.5328989883885,13.3745814871665,12.));
#115204=CARTESIAN_POINT('Ctrl Pts',(69.5139126996675,13.3644813190219,12.));
#115205=CARTESIAN_POINT('Ctrl Pts',(69.4949589944606,13.3544235683394,12.));
#115206=CARTESIAN_POINT('Ctrl Pts',(69.4760380470365,13.3444082410543,12.));
#115207=CARTESIAN_POINT('Ctrl Pts',(69.4571500326673,13.3344353430313,12.));
#115208=CARTESIAN_POINT('Ctrl Pts',(69.4382951276998,13.3245048800643,12.));
#115209=CARTESIAN_POINT('Ctrl Pts',(69.4194735096265,13.3146168578743,12.));
#115210=CARTESIAN_POINT('Ctrl Pts',(69.4006853569511,13.3047712821051,12.));
#115211=CARTESIAN_POINT('Ctrl Pts',(69.3819308490422,13.2949681583167,12.));
#115212=CARTESIAN_POINT('Ctrl Pts',(69.3632101660066,13.2852074919766,12.));
#115213=CARTESIAN_POINT('Ctrl Pts',(69.3445234885065,13.2754892884433,12.));
#115214=CARTESIAN_POINT('Ctrl Pts',(69.3258709977382,13.265813552961,12.));
#115215=CARTESIAN_POINT('Ctrl Pts',(69.3072528758518,13.2561802906896,12.));
#115216=CARTESIAN_POINT('Ctrl Pts',(69.2886693063182,13.2465895067262,12.));
#115217=CARTESIAN_POINT('Ctrl Pts',(69.270120474245,13.237041206122,12.));
#115218=CARTESIAN_POINT('Ctrl Pts',(69.2516065668844,13.2275353939051,12.));
#115219=CARTESIAN_POINT('Ctrl Pts',(69.2331277732861,13.2180720750594,12.));
#115220=CARTESIAN_POINT('Ctrl Pts',(69.2146842833537,13.2086512544735,12.));
#115221=CARTESIAN_POINT('Ctrl Pts',(69.1962762870527,13.1992729368929,12.));
#115222=CARTESIAN_POINT('Ctrl Pts',(69.1779039735996,13.1899371268683,12.));
#115223=CARTESIAN_POINT('Ctrl Pts',(69.1595675305245,13.1806438286934,12.));
#115224=CARTESIAN_POINT('Ctrl Pts',(69.1412671454564,13.1713930465133,12.));
#115225=CARTESIAN_POINT('Ctrl Pts',(69.1230030082573,13.1621847844528,12.));
#115226=CARTESIAN_POINT('Ctrl Pts',(69.1047753127643,13.1530190467183,12.));
#115227=CARTESIAN_POINT('Ctrl Pts',(69.0865842593102,13.1438958377404,12.));
#115228=CARTESIAN_POINT('Ctrl Pts',(69.0684300549477,13.1348151621834,12.));
#115229=CARTESIAN_POINT('Ctrl Pts',(69.0503129081817,13.1257770246386,12.));
#115230=CARTESIAN_POINT('Ctrl Pts',(69.0322330243348,13.1167814293497,12.));
#115231=CARTESIAN_POINT('Ctrl Pts',(69.0141906015113,13.1078283799722,12.));
#115232=CARTESIAN_POINT('Ctrl Pts',(68.9961858241519,13.0989178791834,12.));
#115233=CARTESIAN_POINT('Ctrl Pts',(68.9782188692581,13.090049929053,12.));
#115234=CARTESIAN_POINT('Ctrl Pts',(68.9602899187573,13.0812245317808,12.));
#115235=CARTESIAN_POINT('Ctrl Pts',(68.9423991694492,13.072441690283,12.));
#115236=CARTESIAN_POINT('Ctrl Pts',(68.9245468449945,13.0637014089029,12.));
#115237=CARTESIAN_POINT('Ctrl Pts',(68.9067332040985,13.0550036938813,12.));
#115238=CARTESIAN_POINT('Ctrl Pts',(68.8889585151585,13.0463485518207,12.));
#115239=CARTESIAN_POINT('Ctrl Pts',(68.8712230321906,13.0377359881875,12.));
#115240=CARTESIAN_POINT('Ctrl Pts',(68.8535269726793,13.0291660060107,12.));
#115241=CARTESIAN_POINT('Ctrl Pts',(68.8358704887468,13.0206386039691,12.));
#115242=CARTESIAN_POINT('Ctrl Pts',(68.8182536653656,13.0121537768946,12.));
#115243=CARTESIAN_POINT('Ctrl Pts',(68.804191966902,13.0053999700875,12.));
#115244=CARTESIAN_POINT('Ctrl Pts',(68.7936635625545,13.0003537683055,12.));
#115245=CARTESIAN_POINT('Ctrl Pts',(68.7866525680193,12.9969981460277,12.));
#115246=CARTESIAN_POINT('Ctrl Pts',(68.7831490561748,12.9953224629497,12.));
#115247=CARTESIAN_POINT('Ctrl Pts',(72.2774028393913,16.7988252568749,-5.55111512312578E-16));
#115248=CARTESIAN_POINT('Ctrl Pts',(72.2774028393913,16.7988252568749,4.));
#115249=CARTESIAN_POINT('Ctrl Pts',(72.2774028393913,16.7988252568749,8.));
#115250=CARTESIAN_POINT('Ctrl Pts',(72.2774028393913,16.7988252568749,12.));
#115251=CARTESIAN_POINT('Ctrl Pts',(72.3852065198824,16.7775526720894,-5.55111512312578E-16));
#115252=CARTESIAN_POINT('Ctrl Pts',(72.3852065198824,16.7775526720894,4.));
#115253=CARTESIAN_POINT('Ctrl Pts',(72.3852065198824,16.7775526720894,8.00000000000001));
#115254=CARTESIAN_POINT('Ctrl Pts',(72.3852065198824,16.7775526720894,12.));
#115255=CARTESIAN_POINT('Ctrl Pts',(72.560513354629,16.6758649025559,-5.55111512312578E-16));
#115256=CARTESIAN_POINT('Ctrl Pts',(72.560513354629,16.6758649025559,4.));
#115257=CARTESIAN_POINT('Ctrl Pts',(72.560513354629,16.6758649025559,7.99999999999999));
#115258=CARTESIAN_POINT('Ctrl Pts',(72.560513354629,16.6758649025559,12.));
#115259=CARTESIAN_POINT('Ctrl Pts',(72.6501505354463,16.4988611391808,-5.55111512312578E-16));
#115260=CARTESIAN_POINT('Ctrl Pts',(72.6501505354463,16.4988611391808,4.));
#115261=CARTESIAN_POINT('Ctrl Pts',(72.6501505354463,16.4988611391808,8.00000000000001));
#115262=CARTESIAN_POINT('Ctrl Pts',(72.6501505354463,16.4988611391808,12.));
#115263=CARTESIAN_POINT('Ctrl Pts',(72.6683126419586,16.4184755008061,-5.55111512312578E-16));
#115264=CARTESIAN_POINT('Ctrl Pts',(72.6683126419586,16.4184755008061,4.));
#115265=CARTESIAN_POINT('Ctrl Pts',(72.6683126419586,16.4184755008061,8.));
#115266=CARTESIAN_POINT('Ctrl Pts',(72.6683126419586,16.4184755008061,12.));
#115267=CARTESIAN_POINT('',(72.2774028393913,16.7988252568749,2.77555756156289E-16));
#115268=CARTESIAN_POINT('',(72.6683126419586,16.4184755008061,0.));
#115269=CARTESIAN_POINT('Ctrl Pts',(72.2774028393913,16.7988252568749,-1.38777878078145E-16));
#115270=CARTESIAN_POINT('Ctrl Pts',(72.3852065198824,16.7775526720894,-1.38777878078145E-16));
#115271=CARTESIAN_POINT('Ctrl Pts',(72.4853818540233,16.7194453752131,-1.38777878078144E-16));
#115272=CARTESIAN_POINT('Ctrl Pts',(72.5575834236159,16.6367451007559,-1.38777878078145E-16));
#115273=CARTESIAN_POINT('Ctrl Pts',(72.6117346008103,16.574719894913,-1.38777878078145E-16));
#115274=CARTESIAN_POINT('Ctrl Pts',(72.6501505354463,16.4988611391808,-1.38777878078145E-16));
#115275=CARTESIAN_POINT('Ctrl Pts',(72.6683126419586,16.4184755008061,-1.38777878078145E-16));
#115276=CARTESIAN_POINT('',(72.6683126419586,16.4184755008061,12.));
#115277=CARTESIAN_POINT('Ctrl Pts',(72.6683126419586,16.4184755008061,-5.55111512312578E-16));
#115278=CARTESIAN_POINT('Ctrl Pts',(72.6683126419586,16.4184755008061,4.));
#115279=CARTESIAN_POINT('Ctrl Pts',(72.6683126419586,16.4184755008061,8.));
#115280=CARTESIAN_POINT('Ctrl Pts',(72.6683126419586,16.4184755008061,12.));
#115281=CARTESIAN_POINT('',(72.2774028393913,16.7988252568749,12.));
#115282=CARTESIAN_POINT('Ctrl Pts',(72.6683126419586,16.4184755008061,12.));
#115283=CARTESIAN_POINT('Ctrl Pts',(72.6501505354463,16.4988611391808,12.));
#115284=CARTESIAN_POINT('Ctrl Pts',(72.6117346008103,16.574719894913,12.));
#115285=CARTESIAN_POINT('Ctrl Pts',(72.5575834236159,16.6367451007559,12.));
#115286=CARTESIAN_POINT('Ctrl Pts',(72.4853818540233,16.7194453752131,12.));
#115287=CARTESIAN_POINT('Ctrl Pts',(72.3852065198824,16.7775526720894,12.));
#115288=CARTESIAN_POINT('Ctrl Pts',(72.2774028393913,16.7988252568749,12.));
#115289=CARTESIAN_POINT('Ctrl Pts',(72.2774028393913,16.7988252568749,12.));
#115290=CARTESIAN_POINT('Ctrl Pts',(72.2774028393913,16.7988252568749,8.));
#115291=CARTESIAN_POINT('Ctrl Pts',(72.2774028393913,16.7988252568749,4.));
#115292=CARTESIAN_POINT('Ctrl Pts',(72.2774028393913,16.7988252568749,-5.55111512312578E-16));
#115293=CARTESIAN_POINT('Origin',(3.65936987487134E-10,8.12279454723526E-11,
0.));
#115294=CARTESIAN_POINT('Origin',(3.65936987487134E-10,8.12279454723526E-11,
12.));
#115295=CARTESIAN_POINT('Origin',(3.65936987487134E-10,8.12279454723526E-11,
0.));
#115296=CARTESIAN_POINT('Ctrl Pts',(73.9013264985861,9.42570643237831,0.));
#115297=CARTESIAN_POINT('Ctrl Pts',(73.9013264985861,9.42570643237831,4.));
#115298=CARTESIAN_POINT('Ctrl Pts',(73.9013264985861,9.42570643237828,8.));
#115299=CARTESIAN_POINT('Ctrl Pts',(73.9013264985861,9.42570643237828,12.));
#115300=CARTESIAN_POINT('Ctrl Pts',(73.9152287787081,9.31670696907632,0.));
#115301=CARTESIAN_POINT('Ctrl Pts',(73.9152287787081,9.31670696907632,4.));
#115302=CARTESIAN_POINT('Ctrl Pts',(73.9152287787081,9.31670696907632,8.));
#115303=CARTESIAN_POINT('Ctrl Pts',(73.9152287787081,9.31670696907632,12.));
#115304=CARTESIAN_POINT('Ctrl Pts',(73.8741839722668,9.11824194722592,0.));
#115305=CARTESIAN_POINT('Ctrl Pts',(73.8741839722668,9.11824194722592,4.));
#115306=CARTESIAN_POINT('Ctrl Pts',(73.8741839722668,9.11824194722597,7.99999999999999));
#115307=CARTESIAN_POINT('Ctrl Pts',(73.8741839722668,9.11824194722597,12.));
#115308=CARTESIAN_POINT('Ctrl Pts',(73.7345987226923,8.97724108745619,0.));
#115309=CARTESIAN_POINT('Ctrl Pts',(73.7345987226923,8.97724108745619,4.));
#115310=CARTESIAN_POINT('Ctrl Pts',(73.7345987226924,8.97724108745623,8.00000000000001));
#115311=CARTESIAN_POINT('Ctrl Pts',(73.7345987226924,8.97724108745623,12.));
#115312=CARTESIAN_POINT('Ctrl Pts',(73.6640787197678,8.93459554655875,0.));
#115313=CARTESIAN_POINT('Ctrl Pts',(73.6640787197678,8.93459554655875,4.));
#115314=CARTESIAN_POINT('Ctrl Pts',(73.664078719768,8.93459554655877,8.));
#115315=CARTESIAN_POINT('Ctrl Pts',(73.664078719768,8.93459554655877,12.));
#115316=CARTESIAN_POINT('',(73.9013264985861,9.42570643237831,0.));
#115317=CARTESIAN_POINT('',(73.6640787197679,8.93459554655866,0.));
#115318=CARTESIAN_POINT('Ctrl Pts',(73.9013264985861,9.42570643237831,2.77555756156289E-16));
#115319=CARTESIAN_POINT('Ctrl Pts',(73.9152287787081,9.31670696907632,2.77555756156289E-16));
#115320=CARTESIAN_POINT('Ctrl Pts',(73.8917746035988,9.20329838516181,2.77555756156289E-16));
#115321=CARTESIAN_POINT('Ctrl Pts',(73.8361439572623,9.10865360927363,2.77555756156289E-16));
#115322=CARTESIAN_POINT('Ctrl Pts',(73.7944209725099,9.0376700273575,2.77555756156289E-16));
#115323=CARTESIAN_POINT('Ctrl Pts',(73.7345987226923,8.97724108745619,2.77555756156289E-16));
#115324=CARTESIAN_POINT('Ctrl Pts',(73.6640787197678,8.93459554655875,2.77555756156289E-16));
#115325=CARTESIAN_POINT('',(73.664078719768,8.93459554655874,12.));
#115326=CARTESIAN_POINT('Ctrl Pts',(73.6640787197678,8.93459554655875,0.));
#115327=CARTESIAN_POINT('Ctrl Pts',(73.6640787197678,8.93459554655875,4.));
#115328=CARTESIAN_POINT('Ctrl Pts',(73.664078719768,8.93459554655877,8.));
#115329=CARTESIAN_POINT('Ctrl Pts',(73.664078719768,8.93459554655877,12.));
#115330=CARTESIAN_POINT('',(73.9013264985861,9.42570643237828,12.));
#115331=CARTESIAN_POINT('Ctrl Pts',(73.664078719768,8.93459554655877,12.));
#115332=CARTESIAN_POINT('Ctrl Pts',(73.7345987226924,8.97724108745623,12.));
#115333=CARTESIAN_POINT('Ctrl Pts',(73.79442097251,9.03767002735755,12.));
#115334=CARTESIAN_POINT('Ctrl Pts',(73.8361439572624,9.10865360927367,12.));
#115335=CARTESIAN_POINT('Ctrl Pts',(73.8917746035988,9.20329838516184,12.));
#115336=CARTESIAN_POINT('Ctrl Pts',(73.9152287787081,9.31670696907632,12.));
#115337=CARTESIAN_POINT('Ctrl Pts',(73.9013264985861,9.42570643237828,12.));
#115338=CARTESIAN_POINT('Ctrl Pts',(73.9013264985861,9.42570643237828,12.));
#115339=CARTESIAN_POINT('Ctrl Pts',(73.9013264985861,9.42570643237828,8.));
#115340=CARTESIAN_POINT('Ctrl Pts',(73.9013264985861,9.42570643237831,4.));
#115341=CARTESIAN_POINT('Ctrl Pts',(73.9013264985861,9.42570643237831,0.));
#115342=CARTESIAN_POINT('Ctrl Pts',(69.6540253893192,6.95102489306927,0.));
#115343=CARTESIAN_POINT('Ctrl Pts',(69.6540253893192,6.95102489306927,12.));
#115344=CARTESIAN_POINT('Ctrl Pts',(69.6576616146467,6.95238884849026,0.));
#115345=CARTESIAN_POINT('Ctrl Pts',(69.6576616146467,6.95238884849026,12.));
#115346=CARTESIAN_POINT('Ctrl Pts',(69.664938391983,6.95512065317601,0.));
#115347=CARTESIAN_POINT('Ctrl Pts',(69.664938391983,6.95512065317601,12.));
#115348=CARTESIAN_POINT('Ctrl Pts',(69.6758665380378,6.95923004173592,0.));
#115349=CARTESIAN_POINT('Ctrl Pts',(69.6758665380378,6.95923004173592,12.));
#115350=CARTESIAN_POINT('Ctrl Pts',(69.6904633605421,6.96473259049514,0.));
#115351=CARTESIAN_POINT('Ctrl Pts',(69.6904633605421,6.96473259049514,12.));
#115352=CARTESIAN_POINT('Ctrl Pts',(69.7087526479973,6.97164972291441,0.));
#115353=CARTESIAN_POINT('Ctrl Pts',(69.7087526479973,6.97164972291441,12.));
#115354=CARTESIAN_POINT('Ctrl Pts',(69.7270851557366,6.97860581164528,0.));
#115355=CARTESIAN_POINT('Ctrl Pts',(69.7270851557366,6.97860581164528,12.));
#115356=CARTESIAN_POINT('Ctrl Pts',(69.7454607995607,6.98560086924215,0.));
#115357=CARTESIAN_POINT('Ctrl Pts',(69.7454607995607,6.98560086924215,12.));
#115358=CARTESIAN_POINT('Ctrl Pts',(69.7638794280419,6.99263491027942,0.));
#115359=CARTESIAN_POINT('Ctrl Pts',(69.7638794280419,6.99263491027942,12.));
#115360=CARTESIAN_POINT('Ctrl Pts',(69.782340824259,6.99970795069477,0.));
#115361=CARTESIAN_POINT('Ctrl Pts',(69.782340824259,6.99970795069477,12.));
#115362=CARTESIAN_POINT('Ctrl Pts',(69.8008447346863,7.00682000718152,0.));
#115363=CARTESIAN_POINT('Ctrl Pts',(69.8008447346863,7.00682000718152,12.));
#115364=CARTESIAN_POINT('Ctrl Pts',(69.8193908913722,7.01397109655456,0.));
#115365=CARTESIAN_POINT('Ctrl Pts',(69.8193908913722,7.01397109655456,12.));
#115366=CARTESIAN_POINT('Ctrl Pts',(69.8379790360518,7.02116123514453,0.));
#115367=CARTESIAN_POINT('Ctrl Pts',(69.8379790360518,7.02116123514453,12.));
#115368=CARTESIAN_POINT('Ctrl Pts',(69.8566089455375,7.02839043811814,0.));
#115369=CARTESIAN_POINT('Ctrl Pts',(69.8566089455375,7.02839043811814,12.));
#115370=CARTESIAN_POINT('Ctrl Pts',(69.8752804235238,7.03565871972222,0.));
#115371=CARTESIAN_POINT('Ctrl Pts',(69.8752804235238,7.03565871972222,12.));
#115372=CARTESIAN_POINT('Ctrl Pts',(69.8939932885841,7.04296609362167,0.));
#115373=CARTESIAN_POINT('Ctrl Pts',(69.8939932885841,7.04296609362167,12.));
#115374=CARTESIAN_POINT('Ctrl Pts',(69.9127473642099,7.05031257318117,0.));
#115375=CARTESIAN_POINT('Ctrl Pts',(69.9127473642099,7.05031257318117,12.));
#115376=CARTESIAN_POINT('Ctrl Pts',(69.9315424664291,7.05769817180858,0.));
#115377=CARTESIAN_POINT('Ctrl Pts',(69.9315424664291,7.05769817180858,12.));
#115378=CARTESIAN_POINT('Ctrl Pts',(69.9503783975727,7.06512290312851,0.));
#115379=CARTESIAN_POINT('Ctrl Pts',(69.9503783975727,7.06512290312851,12.));
#115380=CARTESIAN_POINT('Ctrl Pts',(69.9692549527296,7.07258678080832,0.));
#115381=CARTESIAN_POINT('Ctrl Pts',(69.9692549527296,7.07258678080832,12.));
#115382=CARTESIAN_POINT('Ctrl Pts',(69.988171923788,7.08008981844653,0.));
#115383=CARTESIAN_POINT('Ctrl Pts',(69.988171923788,7.08008981844653,12.));
#115384=CARTESIAN_POINT('Ctrl Pts',(70.0071291040766,7.08763202944247,0.));
#115385=CARTESIAN_POINT('Ctrl Pts',(70.0071291040766,7.08763202944247,12.));
#115386=CARTESIAN_POINT('Ctrl Pts',(70.0261262936388,7.0952134268425,0.));
#115387=CARTESIAN_POINT('Ctrl Pts',(70.0261262936388,7.0952134268425,12.));
#115388=CARTESIAN_POINT('Ctrl Pts',(70.0451632990086,7.10283402335035,0.));
#115389=CARTESIAN_POINT('Ctrl Pts',(70.0451632990086,7.10283402335035,12.));
#115390=CARTESIAN_POINT('Ctrl Pts',(70.0642399306869,7.11049383140447,0.));
#115391=CARTESIAN_POINT('Ctrl Pts',(70.0642399306869,7.11049383140447,12.));
#115392=CARTESIAN_POINT('Ctrl Pts',(70.0833560013975,7.11819286322827,0.));
#115393=CARTESIAN_POINT('Ctrl Pts',(70.0833560013975,7.11819286322827,12.));
#115394=CARTESIAN_POINT('Ctrl Pts',(70.1025113239495,7.12593113088905,0.));
#115395=CARTESIAN_POINT('Ctrl Pts',(70.1025113239495,7.12593113088905,12.));
#115396=CARTESIAN_POINT('Ctrl Pts',(70.1217057094499,7.13370864634444,0.));
#115397=CARTESIAN_POINT('Ctrl Pts',(70.1217057094499,7.13370864634444,12.));
#115398=CARTESIAN_POINT('Ctrl Pts',(70.1409389682424,7.14152542142375,0.));
#115399=CARTESIAN_POINT('Ctrl Pts',(70.1409389682424,7.14152542142375,12.));
#115400=CARTESIAN_POINT('Ctrl Pts',(70.1602109107202,7.14938146780815,0.));
#115401=CARTESIAN_POINT('Ctrl Pts',(70.1602109107202,7.14938146780815,12.));
#115402=CARTESIAN_POINT('Ctrl Pts',(70.1795213481185,7.15727679700934,0.));
#115403=CARTESIAN_POINT('Ctrl Pts',(70.1795213481185,7.15727679700934,12.));
#115404=CARTESIAN_POINT('Ctrl Pts',(70.1988700934593,7.16521142033865,0.));
#115405=CARTESIAN_POINT('Ctrl Pts',(70.1988700934593,7.16521142033865,12.));
#115406=CARTESIAN_POINT('Ctrl Pts',(70.2182569618994,7.17318534889717,0.));
#115407=CARTESIAN_POINT('Ctrl Pts',(70.2182569618994,7.17318534889717,12.));
#115408=CARTESIAN_POINT('Ctrl Pts',(70.2376817702215,7.18119859359779,0.));
#115409=CARTESIAN_POINT('Ctrl Pts',(70.2376817702215,7.18119859359779,12.));
#115410=CARTESIAN_POINT('Ctrl Pts',(70.2571443365192,7.18925116517556,0.));
#115411=CARTESIAN_POINT('Ctrl Pts',(70.2571443365192,7.18925116517556,12.));
#115412=CARTESIAN_POINT('Ctrl Pts',(70.2766444798285,7.19734307419874,0.));
#115413=CARTESIAN_POINT('Ctrl Pts',(70.2766444798285,7.19734307419874,12.));
#115414=CARTESIAN_POINT('Ctrl Pts',(70.2961820197077,7.20547433107483,0.));
#115415=CARTESIAN_POINT('Ctrl Pts',(70.2961820197077,7.20547433107483,12.));
#115416=CARTESIAN_POINT('Ctrl Pts',(70.3157567762588,7.21364494605451,0.));
#115417=CARTESIAN_POINT('Ctrl Pts',(70.3157567762588,7.21364494605451,12.));
#115418=CARTESIAN_POINT('Ctrl Pts',(70.3353685703112,7.22185492923192,0.));
#115419=CARTESIAN_POINT('Ctrl Pts',(70.3353685703112,7.22185492923192,12.));
#115420=CARTESIAN_POINT('Ctrl Pts',(70.3550172235486,7.2301042905423,0.));
#115421=CARTESIAN_POINT('Ctrl Pts',(70.3550172235486,7.2301042905423,12.));
#115422=CARTESIAN_POINT('Ctrl Pts',(70.3747025586552,7.23839303975608,0.));
#115423=CARTESIAN_POINT('Ctrl Pts',(70.3747025586552,7.23839303975608,12.));
#115424=CARTESIAN_POINT('Ctrl Pts',(70.3944243994504,7.24672118647086,0.));
#115425=CARTESIAN_POINT('Ctrl Pts',(70.3944243994504,7.24672118647086,12.));
#115426=CARTESIAN_POINT('Ctrl Pts',(70.4141825708178,7.25508874012044,0.));
#115427=CARTESIAN_POINT('Ctrl Pts',(70.4141825708178,7.25508874012044,12.));
#115428=CARTESIAN_POINT('Ctrl Pts',(70.4339768986346,7.26349570998034,0.));
#115429=CARTESIAN_POINT('Ctrl Pts',(70.4339768986346,7.26349570998034,12.));
#115430=CARTESIAN_POINT('Ctrl Pts',(70.4538072096992,7.27194210517064,0.));
#115431=CARTESIAN_POINT('Ctrl Pts',(70.4538072096992,7.27194210517064,12.));
#115432=CARTESIAN_POINT('Ctrl Pts',(70.4736733316487,7.28042793465472,0.));
#115433=CARTESIAN_POINT('Ctrl Pts',(70.4736733316487,7.28042793465472,12.));
#115434=CARTESIAN_POINT('Ctrl Pts',(70.4935750929058,7.28895320723863,0.));
#115435=CARTESIAN_POINT('Ctrl Pts',(70.4935750929058,7.28895320723863,12.));
#115436=CARTESIAN_POINT('Ctrl Pts',(70.5135123227169,7.29751793157824,0.));
#115437=CARTESIAN_POINT('Ctrl Pts',(70.5135123227169,7.29751793157824,12.));
#115438=CARTESIAN_POINT('Ctrl Pts',(70.5334848511681,7.30612211618054,0.));
#115439=CARTESIAN_POINT('Ctrl Pts',(70.5334848511681,7.30612211618054,12.));
#115440=CARTESIAN_POINT('Ctrl Pts',(70.5534925092043,7.31476576940393,0.));
#115441=CARTESIAN_POINT('Ctrl Pts',(70.5534925092043,7.31476576940393,12.));
#115442=CARTESIAN_POINT('Ctrl Pts',(70.5735351286476,7.32344889945221,0.));
#115443=CARTESIAN_POINT('Ctrl Pts',(70.5735351286476,7.32344889945221,12.));
#115444=CARTESIAN_POINT('Ctrl Pts',(70.5936125421946,7.33217151437592,0.));
#115445=CARTESIAN_POINT('Ctrl Pts',(70.5936125421946,7.33217151437592,12.));
#115446=CARTESIAN_POINT('Ctrl Pts',(70.6137245833996,7.34093362208009,0.));
#115447=CARTESIAN_POINT('Ctrl Pts',(70.6137245833996,7.34093362208009,12.));
#115448=CARTESIAN_POINT('Ctrl Pts',(70.6338710866562,7.34973523032579,0.));
#115449=CARTESIAN_POINT('Ctrl Pts',(70.6338710866562,7.34973523032579,12.));
#115450=CARTESIAN_POINT('Ctrl Pts',(70.6540518871775,7.35857634673056,0.));
#115451=CARTESIAN_POINT('Ctrl Pts',(70.6540518871775,7.35857634673056,12.));
#115452=CARTESIAN_POINT('Ctrl Pts',(70.6742668209687,7.36745697876302,0.));
#115453=CARTESIAN_POINT('Ctrl Pts',(70.6742668209687,7.36745697876302,12.));
#115454=CARTESIAN_POINT('Ctrl Pts',(70.694515724827,7.37637713374769,0.));
#115455=CARTESIAN_POINT('Ctrl Pts',(70.694515724827,7.37637713374769,12.));
#115456=CARTESIAN_POINT('Ctrl Pts',(70.7147984363424,7.38533681887033,0.));
#115457=CARTESIAN_POINT('Ctrl Pts',(70.7147984363424,7.38533681887033,12.));
#115458=CARTESIAN_POINT('Ctrl Pts',(70.735114793895,7.39433604117892,0.));
#115459=CARTESIAN_POINT('Ctrl Pts',(70.735114793895,7.39433604117892,12.));
#115460=CARTESIAN_POINT('Ctrl Pts',(70.7554646366514,7.40337480758231,0.));
#115461=CARTESIAN_POINT('Ctrl Pts',(70.7554646366514,7.40337480758231,12.));
#115462=CARTESIAN_POINT('Ctrl Pts',(70.7758478045576,7.41245312484488,0.));
#115463=CARTESIAN_POINT('Ctrl Pts',(70.7758478045576,7.41245312484488,12.));
#115464=CARTESIAN_POINT('Ctrl Pts',(70.7962641383351,7.42157099959317,0.));
#115465=CARTESIAN_POINT('Ctrl Pts',(70.7962641383351,7.42157099959317,12.));
#115466=CARTESIAN_POINT('Ctrl Pts',(70.8167134794738,7.43072843832009,0.));
#115467=CARTESIAN_POINT('Ctrl Pts',(70.8167134794738,7.43072843832009,12.));
#115468=CARTESIAN_POINT('Ctrl Pts',(70.8371956702242,7.43992544738608,0.));
#115469=CARTESIAN_POINT('Ctrl Pts',(70.8371956702242,7.43992544738608,12.));
#115470=CARTESIAN_POINT('Ctrl Pts',(70.8577105535841,7.44916203301646,0.));
#115471=CARTESIAN_POINT('Ctrl Pts',(70.8577105535841,7.44916203301646,12.));
#115472=CARTESIAN_POINT('Ctrl Pts',(70.8782579732885,7.45843820129777,0.));
#115473=CARTESIAN_POINT('Ctrl Pts',(70.8782579732885,7.45843820129777,12.));
#115474=CARTESIAN_POINT('Ctrl Pts',(70.8988377738088,7.4677539581852,0.));
#115475=CARTESIAN_POINT('Ctrl Pts',(70.8988377738088,7.4677539581852,12.));
#115476=CARTESIAN_POINT('Ctrl Pts',(70.9194498003483,7.47710930950555,0.));
#115477=CARTESIAN_POINT('Ctrl Pts',(70.9194498003483,7.47710930950555,12.));
#115478=CARTESIAN_POINT('Ctrl Pts',(70.9400938988373,7.48650426095824,0.));
#115479=CARTESIAN_POINT('Ctrl Pts',(70.9400938988373,7.48650426095824,12.));
#115480=CARTESIAN_POINT('Ctrl Pts',(70.9607699159234,7.49593881811142,0.));
#115481=CARTESIAN_POINT('Ctrl Pts',(70.9607699159234,7.49593881811142,12.));
#115482=CARTESIAN_POINT('Ctrl Pts',(70.9814776989637,7.5054129863995,0.));
#115483=CARTESIAN_POINT('Ctrl Pts',(70.9814776989637,7.5054129863995,12.));
#115484=CARTESIAN_POINT('Ctrl Pts',(71.0022170960235,7.51492677113113,0.));
#115485=CARTESIAN_POINT('Ctrl Pts',(71.0022170960235,7.51492677113113,12.));
#115486=CARTESIAN_POINT('Ctrl Pts',(71.0229879558713,7.52448017749137,0.));
#115487=CARTESIAN_POINT('Ctrl Pts',(71.0229879558713,7.52448017749137,12.));
#115488=CARTESIAN_POINT('Ctrl Pts',(71.0437901279722,7.53407321054255,0.));
#115489=CARTESIAN_POINT('Ctrl Pts',(71.0437901279722,7.53407321054255,12.));
#115490=CARTESIAN_POINT('Ctrl Pts',(71.0646234624783,7.5437058752195,0.));
#115491=CARTESIAN_POINT('Ctrl Pts',(71.0646234624783,7.5437058752195,12.));
#115492=CARTESIAN_POINT('Ctrl Pts',(71.0854878102203,7.55337817632874,0.));
#115493=CARTESIAN_POINT('Ctrl Pts',(71.0854878102203,7.55337817632874,12.));
#115494=CARTESIAN_POINT('Ctrl Pts',(71.1063830227074,7.56309011855618,0.));
#115495=CARTESIAN_POINT('Ctrl Pts',(71.1063830227074,7.56309011855618,12.));
#115496=CARTESIAN_POINT('Ctrl Pts',(71.1273089521218,7.57284170646867,0.));
#115497=CARTESIAN_POINT('Ctrl Pts',(71.1273089521218,7.57284170646867,12.));
#115498=CARTESIAN_POINT('Ctrl Pts',(71.1482654513133,7.58263294451467,0.));
#115499=CARTESIAN_POINT('Ctrl Pts',(71.1482654513133,7.58263294451467,12.));
#115500=CARTESIAN_POINT('Ctrl Pts',(71.1692523737887,7.59246383701861,0.));
#115501=CARTESIAN_POINT('Ctrl Pts',(71.1692523737887,7.59246383701861,12.));
#115502=CARTESIAN_POINT('Ctrl Pts',(71.1902695737063,7.60233438818157,0.));
#115503=CARTESIAN_POINT('Ctrl Pts',(71.1902695737063,7.60233438818157,12.));
#115504=CARTESIAN_POINT('Ctrl Pts',(71.2113169058778,7.61224460208888,0.));
#115505=CARTESIAN_POINT('Ctrl Pts',(71.2113169058778,7.61224460208888,12.));
#115506=CARTESIAN_POINT('Ctrl Pts',(71.232394225762,7.62219448271126,0.));
#115507=CARTESIAN_POINT('Ctrl Pts',(71.232394225762,7.62219448271126,12.));
#115508=CARTESIAN_POINT('Ctrl Pts',(71.2535013894587,7.63218403390516,0.));
#115509=CARTESIAN_POINT('Ctrl Pts',(71.2535013894587,7.63218403390516,12.));
#115510=CARTESIAN_POINT('Ctrl Pts',(71.2746382536974,7.64221325940673,0.));
#115511=CARTESIAN_POINT('Ctrl Pts',(71.2746382536974,7.64221325940673,12.));
#115512=CARTESIAN_POINT('Ctrl Pts',(71.2958046758334,7.65228216283344,0.));
#115513=CARTESIAN_POINT('Ctrl Pts',(71.2958046758334,7.65228216283344,12.));
#115514=CARTESIAN_POINT('Ctrl Pts',(71.3170005138474,7.6623907476912,0.));
#115515=CARTESIAN_POINT('Ctrl Pts',(71.3170005138474,7.6623907476912,12.));
#115516=CARTESIAN_POINT('Ctrl Pts',(71.3382256263405,7.67253901737541,0.));
#115517=CARTESIAN_POINT('Ctrl Pts',(71.3382256263405,7.67253901737541,12.));
#115518=CARTESIAN_POINT('Ctrl Pts',(71.3594798725294,7.68272697517104,0.));
#115519=CARTESIAN_POINT('Ctrl Pts',(71.3594798725294,7.68272697517104,12.));
#115520=CARTESIAN_POINT('Ctrl Pts',(71.380763112236,7.69295462424648,0.));
#115521=CARTESIAN_POINT('Ctrl Pts',(71.380763112236,7.69295462424648,12.));
#115522=CARTESIAN_POINT('Ctrl Pts',(71.4020752058827,7.70322196765574,0.));
#115523=CARTESIAN_POINT('Ctrl Pts',(71.4020752058827,7.70322196765574,12.));
#115524=CARTESIAN_POINT('Ctrl Pts',(71.4234160144943,7.71352900834539,0.));
#115525=CARTESIAN_POINT('Ctrl Pts',(71.4234160144943,7.71352900834539,12.));
#115526=CARTESIAN_POINT('Ctrl Pts',(71.4447853996919,7.72387574915546,0.));
#115527=CARTESIAN_POINT('Ctrl Pts',(71.4447853996919,7.72387574915546,12.));
#115528=CARTESIAN_POINT('Ctrl Pts',(71.4661832236881,7.73426219281933,0.));
#115529=CARTESIAN_POINT('Ctrl Pts',(71.4661832236881,7.73426219281933,12.));
#115530=CARTESIAN_POINT('Ctrl Pts',(71.487609349277,7.74468834195735,0.));
#115531=CARTESIAN_POINT('Ctrl Pts',(71.487609349277,7.74468834195735,12.));
#115532=CARTESIAN_POINT('Ctrl Pts',(71.5090636398307,7.75515419907956,0.));
#115533=CARTESIAN_POINT('Ctrl Pts',(71.5090636398307,7.75515419907956,12.));
#115534=CARTESIAN_POINT('Ctrl Pts',(71.5305459592987,7.7656597665922,0.));
#115535=CARTESIAN_POINT('Ctrl Pts',(71.5305459592987,7.7656597665922,12.));
#115536=CARTESIAN_POINT('Ctrl Pts',(71.5520561722039,7.77620504679869,0.));
#115537=CARTESIAN_POINT('Ctrl Pts',(71.5520561722039,7.77620504679869,12.));
#115538=CARTESIAN_POINT('Ctrl Pts',(71.5735941436366,7.78679004189936,0.));
#115539=CARTESIAN_POINT('Ctrl Pts',(71.5735941436366,7.78679004189936,12.));
#115540=CARTESIAN_POINT('Ctrl Pts',(71.5951597392471,7.79741475398513,0.));
#115541=CARTESIAN_POINT('Ctrl Pts',(71.5951597392471,7.79741475398513,12.));
#115542=CARTESIAN_POINT('Ctrl Pts',(71.616752825242,7.80807918504018,0.));
#115543=CARTESIAN_POINT('Ctrl Pts',(71.616752825242,7.80807918504018,12.));
#115544=CARTESIAN_POINT('Ctrl Pts',(71.638373268384,7.81878333694857,0.));
#115545=CARTESIAN_POINT('Ctrl Pts',(71.638373268384,7.81878333694857,12.));
#115546=CARTESIAN_POINT('Ctrl Pts',(71.6600209359869,7.82952721149505,0.));
#115547=CARTESIAN_POINT('Ctrl Pts',(71.6600209359869,7.82952721149505,12.));
#115548=CARTESIAN_POINT('Ctrl Pts',(71.681695695912,7.8403108103649,0.));
#115549=CARTESIAN_POINT('Ctrl Pts',(71.681695695912,7.8403108103649,12.));
#115550=CARTESIAN_POINT('Ctrl Pts',(71.7033974165576,7.8511341351374,0.));
#115551=CARTESIAN_POINT('Ctrl Pts',(71.7033974165576,7.8511341351374,12.));
#115552=CARTESIAN_POINT('Ctrl Pts',(71.7251259668573,7.86199718728831,0.));
#115553=CARTESIAN_POINT('Ctrl Pts',(71.7251259668573,7.86199718728831,12.));
#115554=CARTESIAN_POINT('Ctrl Pts',(71.7468812162795,7.87289996819656,0.));
#115555=CARTESIAN_POINT('Ctrl Pts',(71.7468812162795,7.87289996819656,12.));
#115556=CARTESIAN_POINT('Ctrl Pts',(71.768663034824,7.88384247914523,0.));
#115557=CARTESIAN_POINT('Ctrl Pts',(71.768663034824,7.88384247914523,12.));
#115558=CARTESIAN_POINT('Ctrl Pts',(71.7904712930172,7.89482472132136,0.));
#115559=CARTESIAN_POINT('Ctrl Pts',(71.7904712930172,7.89482472132136,12.));
#115560=CARTESIAN_POINT('Ctrl Pts',(71.8123058619038,7.90584669580957,0.));
#115561=CARTESIAN_POINT('Ctrl Pts',(71.8123058619038,7.90584669580957,12.));
#115562=CARTESIAN_POINT('Ctrl Pts',(71.8341666130424,7.91690840359372,0.));
#115563=CARTESIAN_POINT('Ctrl Pts',(71.8341666130424,7.91690840359372,12.));
#115564=CARTESIAN_POINT('Ctrl Pts',(71.8560534185071,7.92800984556401,0.));
#115565=CARTESIAN_POINT('Ctrl Pts',(71.8560534185071,7.92800984556401,12.));
#115566=CARTESIAN_POINT('Ctrl Pts',(71.8779661508833,7.93915102251797,0.));
#115567=CARTESIAN_POINT('Ctrl Pts',(71.8779661508833,7.93915102251797,12.));
#115568=CARTESIAN_POINT('Ctrl Pts',(71.8999046832642,7.95033193516047,0.));
#115569=CARTESIAN_POINT('Ctrl Pts',(71.8999046832642,7.95033193516047,12.));
#115570=CARTESIAN_POINT('Ctrl Pts',(71.9218688892426,7.96155258409753,0.));
#115571=CARTESIAN_POINT('Ctrl Pts',(71.9218688892426,7.96155258409753,12.));
#115572=CARTESIAN_POINT('Ctrl Pts',(71.9438586429072,7.97281296983703,0.));
#115573=CARTESIAN_POINT('Ctrl Pts',(71.9438586429072,7.97281296983703,12.));
#115574=CARTESIAN_POINT('Ctrl Pts',(71.9658738188421,7.98411309279599,0.));
#115575=CARTESIAN_POINT('Ctrl Pts',(71.9658738188421,7.98411309279599,12.));
#115576=CARTESIAN_POINT('Ctrl Pts',(71.9879142921248,7.99545295330183,0.));
#115577=CARTESIAN_POINT('Ctrl Pts',(71.9879142921248,7.99545295330183,12.));
#115578=CARTESIAN_POINT('Ctrl Pts',(72.0099799383216,8.00683255159251,0.));
#115579=CARTESIAN_POINT('Ctrl Pts',(72.0099799383216,8.00683255159251,12.));
#115580=CARTESIAN_POINT('Ctrl Pts',(72.0320706334802,8.01825188781071,0.));
#115581=CARTESIAN_POINT('Ctrl Pts',(72.0320706334802,8.01825188781071,12.));
#115582=CARTESIAN_POINT('Ctrl Pts',(72.0541862541262,8.0297109620033,0.));
#115583=CARTESIAN_POINT('Ctrl Pts',(72.0541862541262,8.0297109620033,12.));
#115584=CARTESIAN_POINT('Ctrl Pts',(72.0763266772632,8.04120977412893,0.));
#115585=CARTESIAN_POINT('Ctrl Pts',(72.0763266772632,8.04120977412893,12.));
#115586=CARTESIAN_POINT('Ctrl Pts',(72.0984917803702,8.05274832405958,0.));
#115587=CARTESIAN_POINT('Ctrl Pts',(72.0984917803702,8.05274832405958,12.));
#115588=CARTESIAN_POINT('Ctrl Pts',(72.1206814413985,8.06432661158091,0.));
#115589=CARTESIAN_POINT('Ctrl Pts',(72.1206814413985,8.06432661158091,12.));
#115590=CARTESIAN_POINT('Ctrl Pts',(72.1428955387648,8.07594463638701,0.));
#115591=CARTESIAN_POINT('Ctrl Pts',(72.1428955387648,8.07594463638701,12.));
#115592=CARTESIAN_POINT('Ctrl Pts',(72.165133951346,8.08760239807816,0.));
#115593=CARTESIAN_POINT('Ctrl Pts',(72.165133951346,8.08760239807816,12.));
#115594=CARTESIAN_POINT('Ctrl Pts',(72.18739655848,8.09929989616875,0.));
#115595=CARTESIAN_POINT('Ctrl Pts',(72.18739655848,8.09929989616875,12.));
#115596=CARTESIAN_POINT('Ctrl Pts',(72.2096832399626,8.11103713008923,0.));
#115597=CARTESIAN_POINT('Ctrl Pts',(72.2096832399626,8.11103713008923,12.));
#115598=CARTESIAN_POINT('Ctrl Pts',(72.2319938760451,8.12281409918663,0.));
#115599=CARTESIAN_POINT('Ctrl Pts',(72.2319938760451,8.12281409918663,12.));
#115600=CARTESIAN_POINT('Ctrl Pts',(72.2543283474279,8.1346308027203,0.));
#115601=CARTESIAN_POINT('Ctrl Pts',(72.2543283474279,8.1346308027203,12.));
#115602=CARTESIAN_POINT('Ctrl Pts',(72.2766865352552,8.14648723985794,0.));
#115603=CARTESIAN_POINT('Ctrl Pts',(72.2766865352552,8.14648723985794,12.));
#115604=CARTESIAN_POINT('Ctrl Pts',(72.2990683211155,8.15838340968329,0.));
#115605=CARTESIAN_POINT('Ctrl Pts',(72.2990683211155,8.15838340968329,12.));
#115606=CARTESIAN_POINT('Ctrl Pts',(72.3214735870402,8.17031931119883,0.));
#115607=CARTESIAN_POINT('Ctrl Pts',(72.3214735870402,8.17031931119883,12.));
#115608=CARTESIAN_POINT('Ctrl Pts',(72.3439022155007,8.18229494332623,0.));
#115609=CARTESIAN_POINT('Ctrl Pts',(72.3439022155007,8.18229494332623,12.));
#115610=CARTESIAN_POINT('Ctrl Pts',(72.3663540894034,8.1943103049032,0.));
#115611=CARTESIAN_POINT('Ctrl Pts',(72.3663540894034,8.1943103049032,12.));
#115612=CARTESIAN_POINT('Ctrl Pts',(72.3888290920845,8.20636539467783,0.));
#115613=CARTESIAN_POINT('Ctrl Pts',(72.3888290920845,8.20636539467783,12.));
#115614=CARTESIAN_POINT('Ctrl Pts',(72.4113271073091,8.21846021131565,0.));
#115615=CARTESIAN_POINT('Ctrl Pts',(72.4113271073091,8.21846021131565,12.));
#115616=CARTESIAN_POINT('Ctrl Pts',(72.4338480192701,8.23059475340355,0.));
#115617=CARTESIAN_POINT('Ctrl Pts',(72.4338480192701,8.23059475340355,12.));
#115618=CARTESIAN_POINT('Ctrl Pts',(72.4563917125842,8.24276901945038,0.));
#115619=CARTESIAN_POINT('Ctrl Pts',(72.4563917125842,8.24276901945038,12.));
#115620=CARTESIAN_POINT('Ctrl Pts',(72.4789580722871,8.25498300788494,0.));
#115621=CARTESIAN_POINT('Ctrl Pts',(72.4789580722871,8.25498300788494,12.));
#115622=CARTESIAN_POINT('Ctrl Pts',(72.501546983825,8.26723671704925,0.));
#115623=CARTESIAN_POINT('Ctrl Pts',(72.501546983825,8.26723671704925,12.));
#115624=CARTESIAN_POINT('Ctrl Pts',(72.524158333056,8.27953014520386,0.));
#115625=CARTESIAN_POINT('Ctrl Pts',(72.524158333056,8.27953014520386,12.));
#115626=CARTESIAN_POINT('Ctrl Pts',(72.5467920062522,8.2918632905329,0.));
#115627=CARTESIAN_POINT('Ctrl Pts',(72.5467920062522,8.2918632905329,12.));
#115628=CARTESIAN_POINT('Ctrl Pts',(72.5694478900983,8.30423615114456,0.));
#115629=CARTESIAN_POINT('Ctrl Pts',(72.5694478900983,8.30423615114456,12.));
#115630=CARTESIAN_POINT('Ctrl Pts',(72.5921258716899,8.3166487250701,0.));
#115631=CARTESIAN_POINT('Ctrl Pts',(72.5921258716899,8.3166487250701,12.));
#115632=CARTESIAN_POINT('Ctrl Pts',(72.614825838529,8.32910101025654,0.));
#115633=CARTESIAN_POINT('Ctrl Pts',(72.614825838529,8.32910101025654,12.));
#115634=CARTESIAN_POINT('Ctrl Pts',(72.6375476785208,8.34159300456966,0.));
#115635=CARTESIAN_POINT('Ctrl Pts',(72.6375476785208,8.34159300456966,12.));
#115636=CARTESIAN_POINT('Ctrl Pts',(72.6602912799689,8.35412470580084,0.));
#115637=CARTESIAN_POINT('Ctrl Pts',(72.6602912799689,8.35412470580084,12.));
#115638=CARTESIAN_POINT('Ctrl Pts',(72.68305653157,8.36669611166835,0.));
#115639=CARTESIAN_POINT('Ctrl Pts',(72.68305653157,8.36669611166835,12.));
#115640=CARTESIAN_POINT('Ctrl Pts',(72.7058433224072,8.37930721981736,0.));
#115641=CARTESIAN_POINT('Ctrl Pts',(72.7058433224072,8.37930721981736,12.));
#115642=CARTESIAN_POINT('Ctrl Pts',(72.728651541938,8.39195802781408,0.));
#115643=CARTESIAN_POINT('Ctrl Pts',(72.728651541938,8.39195802781408,12.));
#115644=CARTESIAN_POINT('Ctrl Pts',(72.7514810799932,8.40464853314494,0.));
#115645=CARTESIAN_POINT('Ctrl Pts',(72.7514810799932,8.40464853314494,12.));
#115646=CARTESIAN_POINT('Ctrl Pts',(72.7743318267876,8.41737873322354,0.));
#115647=CARTESIAN_POINT('Ctrl Pts',(72.7743318267876,8.41737873322354,12.));
#115648=CARTESIAN_POINT('Ctrl Pts',(72.7972036729283,8.43014862539172,0.));
#115649=CARTESIAN_POINT('Ctrl Pts',(72.7972036729283,8.43014862539172,12.));
#115650=CARTESIAN_POINT('Ctrl Pts',(72.8200965094197,8.44295820691908,0.));
#115651=CARTESIAN_POINT('Ctrl Pts',(72.8200965094197,8.44295820691908,12.));
#115652=CARTESIAN_POINT('Ctrl Pts',(72.8430102276703,8.45580747499772,0.));
#115653=CARTESIAN_POINT('Ctrl Pts',(72.8430102276703,8.45580747499772,12.));
#115654=CARTESIAN_POINT('Ctrl Pts',(72.8659447194918,8.46869642673764,0.));
#115655=CARTESIAN_POINT('Ctrl Pts',(72.8659447194918,8.46869642673764,12.));
#115656=CARTESIAN_POINT('Ctrl Pts',(72.888899877077,8.48162505917629,0.));
#115657=CARTESIAN_POINT('Ctrl Pts',(72.888899877077,8.48162505917629,12.));
#115658=CARTESIAN_POINT('Ctrl Pts',(72.9118755929785,8.49459336928277,0.));
#115659=CARTESIAN_POINT('Ctrl Pts',(72.9118755929785,8.49459336928277,12.));
#115660=CARTESIAN_POINT('Ctrl Pts',(72.9348717600837,8.5076013539598,0.));
#115661=CARTESIAN_POINT('Ctrl Pts',(72.9348717600837,8.5076013539598,12.));
#115662=CARTESIAN_POINT('Ctrl Pts',(72.9578882715923,8.52064901004245,0.));
#115663=CARTESIAN_POINT('Ctrl Pts',(72.9578882715923,8.52064901004245,12.));
#115664=CARTESIAN_POINT('Ctrl Pts',(72.9809250209843,8.53373633429304,0.));
#115665=CARTESIAN_POINT('Ctrl Pts',(72.9809250209843,8.53373633429304,12.));
#115666=CARTESIAN_POINT('Ctrl Pts',(73.0039819020663,8.5468633234044,0.));
#115667=CARTESIAN_POINT('Ctrl Pts',(73.0039819020663,8.5468633234044,12.));
#115668=CARTESIAN_POINT('Ctrl Pts',(73.0270588090193,8.56002997400097,0.));
#115669=CARTESIAN_POINT('Ctrl Pts',(73.0270588090193,8.56002997400097,12.));
#115670=CARTESIAN_POINT('Ctrl Pts',(73.0501556364482,8.57323628263596,0.));
#115671=CARTESIAN_POINT('Ctrl Pts',(73.0501556364482,8.57323628263596,12.));
#115672=CARTESIAN_POINT('Ctrl Pts',(73.073272279419,8.58648224578724,0.));
#115673=CARTESIAN_POINT('Ctrl Pts',(73.073272279419,8.58648224578724,12.));
#115674=CARTESIAN_POINT('Ctrl Pts',(73.0964086335226,8.5997678598454,0.));
#115675=CARTESIAN_POINT('Ctrl Pts',(73.0964086335226,8.5997678598454,12.));
#115676=CARTESIAN_POINT('Ctrl Pts',(73.1195645948169,8.6130931211199,0.));
#115677=CARTESIAN_POINT('Ctrl Pts',(73.1195645948169,8.6130931211199,12.));
#115678=CARTESIAN_POINT('Ctrl Pts',(73.142740059703,8.62645802585476,0.));
#115679=CARTESIAN_POINT('Ctrl Pts',(73.142740059703,8.62645802585476,12.));
#115680=CARTESIAN_POINT('Ctrl Pts',(73.165934924813,8.63986257023736,0.));
#115681=CARTESIAN_POINT('Ctrl Pts',(73.165934924813,8.63986257023736,12.));
#115682=CARTESIAN_POINT('Ctrl Pts',(73.1891490869057,8.65330675040537,0.));
#115683=CARTESIAN_POINT('Ctrl Pts',(73.1891490869057,8.65330675040537,12.));
#115684=CARTESIAN_POINT('Ctrl Pts',(73.2123824427212,8.66679056245097,0.));
#115685=CARTESIAN_POINT('Ctrl Pts',(73.2123824427212,8.66679056245097,12.));
#115686=CARTESIAN_POINT('Ctrl Pts',(73.2356348889704,8.68031400241885,0.));
#115687=CARTESIAN_POINT('Ctrl Pts',(73.2356348889704,8.68031400241885,12.));
#115688=CARTESIAN_POINT('Ctrl Pts',(73.2589063226373,8.69387706629305,0.));
#115689=CARTESIAN_POINT('Ctrl Pts',(73.2589063226373,8.69387706629305,12.));
#115690=CARTESIAN_POINT('Ctrl Pts',(73.282196641216,8.70747974998246,0.));
#115691=CARTESIAN_POINT('Ctrl Pts',(73.282196641216,8.70747974998246,12.));
#115692=CARTESIAN_POINT('Ctrl Pts',(73.3055057429744,8.72112204930233,0.));
#115693=CARTESIAN_POINT('Ctrl Pts',(73.3055057429744,8.72112204930233,12.));
#115694=CARTESIAN_POINT('Ctrl Pts',(73.3288335271989,8.73480395995361,0.));
#115695=CARTESIAN_POINT('Ctrl Pts',(73.3288335271989,8.73480395995361,12.));
#115696=CARTESIAN_POINT('Ctrl Pts',(73.3521798944595,8.74852547749737,0.));
#115697=CARTESIAN_POINT('Ctrl Pts',(73.3521798944595,8.74852547749737,12.));
#115698=CARTESIAN_POINT('Ctrl Pts',(73.3755447460235,8.76228659740306,0.));
#115699=CARTESIAN_POINT('Ctrl Pts',(73.3755447460235,8.76228659740306,12.));
#115700=CARTESIAN_POINT('Ctrl Pts',(73.3989279832808,8.77608731509305,0.));
#115701=CARTESIAN_POINT('Ctrl Pts',(73.3989279832808,8.77608731509305,12.));
#115702=CARTESIAN_POINT('Ctrl Pts',(73.422329507112,8.78992762598739,0.));
#115703=CARTESIAN_POINT('Ctrl Pts',(73.422329507112,8.78992762598739,12.));
#115704=CARTESIAN_POINT('Ctrl Pts',(73.4457492173949,8.80380752553715,0.));
#115705=CARTESIAN_POINT('Ctrl Pts',(73.4457492173949,8.80380752553715,12.));
#115706=CARTESIAN_POINT('Ctrl Pts',(73.4691870121608,8.81772700927594,0.));
#115707=CARTESIAN_POINT('Ctrl Pts',(73.4691870121608,8.81772700927594,12.));
#115708=CARTESIAN_POINT('Ctrl Pts',(73.4926427882787,8.83168607277416,0.));
#115709=CARTESIAN_POINT('Ctrl Pts',(73.4926427882787,8.83168607277416,12.));
#115710=CARTESIAN_POINT('Ctrl Pts',(73.5161164429765,8.84568471153895,0.));
#115711=CARTESIAN_POINT('Ctrl Pts',(73.5161164429765,8.84568471153895,12.));
#115712=CARTESIAN_POINT('Ctrl Pts',(73.5396078751672,8.85972292092184,0.));
#115713=CARTESIAN_POINT('Ctrl Pts',(73.5396078751672,8.85972292092184,12.));
#115714=CARTESIAN_POINT('Ctrl Pts',(73.5631169867113,8.87380069602956,0.));
#115715=CARTESIAN_POINT('Ctrl Pts',(73.5631169867113,8.87380069602956,12.));
#115716=CARTESIAN_POINT('Ctrl Pts',(73.5866436840493,8.88791803160342,0.));
#115717=CARTESIAN_POINT('Ctrl Pts',(73.5866436840493,8.88791803160342,12.));
#115718=CARTESIAN_POINT('Ctrl Pts',(73.6101878785868,8.90207492198872,0.));
#115719=CARTESIAN_POINT('Ctrl Pts',(73.6101878785868,8.90207492198872,12.));
#115720=CARTESIAN_POINT('Ctrl Pts',(73.6337494830846,8.91627136139888,0.));
#115721=CARTESIAN_POINT('Ctrl Pts',(73.6337494830846,8.91627136139888,12.));
#115722=CARTESIAN_POINT('Ctrl Pts',(73.6573284088088,8.93050734411972,0.));
#115723=CARTESIAN_POINT('Ctrl Pts',(73.6573284088088,8.93050734411972,12.));
#115724=CARTESIAN_POINT('Ctrl Pts',(73.6809245622361,8.94478286474384,0.));
#115725=CARTESIAN_POINT('Ctrl Pts',(73.6809245622361,8.94478286474384,12.));
#115726=CARTESIAN_POINT('Ctrl Pts',(73.7045378422775,8.95909791836291,0.));
#115727=CARTESIAN_POINT('Ctrl Pts',(73.7045378422775,8.95909791836291,12.));
#115728=CARTESIAN_POINT('Ctrl Pts',(73.7281681364031,8.97345250083919,0.));
#115729=CARTESIAN_POINT('Ctrl Pts',(73.7281681364031,8.97345250083919,12.));
#115730=CARTESIAN_POINT('Ctrl Pts',(73.7518153262253,8.98784660837829,0.));
#115731=CARTESIAN_POINT('Ctrl Pts',(73.7518153262253,8.98784660837829,12.));
#115732=CARTESIAN_POINT('Ctrl Pts',(73.7754792943925,9.00228023701468,0.));
#115733=CARTESIAN_POINT('Ctrl Pts',(73.7754792943925,9.00228023701468,12.));
#115734=CARTESIAN_POINT('Ctrl Pts',(73.7991599312731,9.01675338208223,0.));
#115735=CARTESIAN_POINT('Ctrl Pts',(73.7991599312731,9.01675338208223,12.));
#115736=CARTESIAN_POINT('Ctrl Pts',(73.8228571411607,9.03126603777982,0.));
#115737=CARTESIAN_POINT('Ctrl Pts',(73.8228571411607,9.03126603777982,12.));
#115738=CARTESIAN_POINT('Ctrl Pts',(73.8465708500679,9.04581819646386,0.));
#115739=CARTESIAN_POINT('Ctrl Pts',(73.8465708500679,9.04581819646386,12.));
#115740=CARTESIAN_POINT('Ctrl Pts',(73.870301007746,9.06040984889251,0.));
#115741=CARTESIAN_POINT('Ctrl Pts',(73.870301007746,9.06040984889251,12.));
#115742=CARTESIAN_POINT('Ctrl Pts',(73.8940475821756,9.07504098570548,0.));
#115743=CARTESIAN_POINT('Ctrl Pts',(73.8940475821756,9.07504098570548,12.));
#115744=CARTESIAN_POINT('Ctrl Pts',(73.9130579611989,9.08677747601239,0.));
#115745=CARTESIAN_POINT('Ctrl Pts',(73.9130579611989,9.08677747601239,12.));
#115746=CARTESIAN_POINT('Ctrl Pts',(73.9273231219464,9.0955976052846,0.));
#115747=CARTESIAN_POINT('Ctrl Pts',(73.9273231219464,9.0955976052846,12.));
#115748=CARTESIAN_POINT('Ctrl Pts',(73.9368365074164,9.10148558516325,0.));
#115749=CARTESIAN_POINT('Ctrl Pts',(73.9368365074164,9.10148558516325,12.));
#115750=CARTESIAN_POINT('Ctrl Pts',(73.9415940197274,9.10443154852688,0.));
#115751=CARTESIAN_POINT('Ctrl Pts',(73.9415940197274,9.10443154852688,12.));
#115752=CARTESIAN_POINT('',(69.6540253893192,6.95102489306927,0.));
#115753=CARTESIAN_POINT('Ctrl Pts',(69.6540253893192,6.95102489306927,0.));
#115754=CARTESIAN_POINT('Ctrl Pts',(69.6576616146467,6.95238884849026,0.));
#115755=CARTESIAN_POINT('Ctrl Pts',(69.664938391983,6.95512065317601,0.));
#115756=CARTESIAN_POINT('Ctrl Pts',(69.6758665380378,6.95923004173592,0.));
#115757=CARTESIAN_POINT('Ctrl Pts',(69.6904633605421,6.96473259049514,0.));
#115758=CARTESIAN_POINT('Ctrl Pts',(69.7087526479973,6.97164972291441,0.));
#115759=CARTESIAN_POINT('Ctrl Pts',(69.7270851557366,6.97860581164528,0.));
#115760=CARTESIAN_POINT('Ctrl Pts',(69.7454607995607,6.98560086924215,0.));
#115761=CARTESIAN_POINT('Ctrl Pts',(69.7638794280419,6.99263491027942,0.));
#115762=CARTESIAN_POINT('Ctrl Pts',(69.782340824259,6.99970795069477,0.));
#115763=CARTESIAN_POINT('Ctrl Pts',(69.8008447346863,7.00682000718152,0.));
#115764=CARTESIAN_POINT('Ctrl Pts',(69.8193908913722,7.01397109655456,0.));
#115765=CARTESIAN_POINT('Ctrl Pts',(69.8379790360518,7.02116123514453,0.));
#115766=CARTESIAN_POINT('Ctrl Pts',(69.8566089455375,7.02839043811814,0.));
#115767=CARTESIAN_POINT('Ctrl Pts',(69.8752804235238,7.03565871972222,0.));
#115768=CARTESIAN_POINT('Ctrl Pts',(69.8939932885841,7.04296609362167,0.));
#115769=CARTESIAN_POINT('Ctrl Pts',(69.9127473642099,7.05031257318117,0.));
#115770=CARTESIAN_POINT('Ctrl Pts',(69.9315424664291,7.05769817180858,0.));
#115771=CARTESIAN_POINT('Ctrl Pts',(69.9503783975727,7.06512290312851,0.));
#115772=CARTESIAN_POINT('Ctrl Pts',(69.9692549527296,7.07258678080832,0.));
#115773=CARTESIAN_POINT('Ctrl Pts',(69.988171923788,7.08008981844653,0.));
#115774=CARTESIAN_POINT('Ctrl Pts',(70.0071291040766,7.08763202944247,0.));
#115775=CARTESIAN_POINT('Ctrl Pts',(70.0261262936388,7.0952134268425,0.));
#115776=CARTESIAN_POINT('Ctrl Pts',(70.0451632990086,7.10283402335035,0.));
#115777=CARTESIAN_POINT('Ctrl Pts',(70.0642399306869,7.11049383140447,0.));
#115778=CARTESIAN_POINT('Ctrl Pts',(70.0833560013975,7.11819286322827,0.));
#115779=CARTESIAN_POINT('Ctrl Pts',(70.1025113239495,7.12593113088905,0.));
#115780=CARTESIAN_POINT('Ctrl Pts',(70.1217057094499,7.13370864634444,0.));
#115781=CARTESIAN_POINT('Ctrl Pts',(70.1409389682424,7.14152542142375,0.));
#115782=CARTESIAN_POINT('Ctrl Pts',(70.1602109107202,7.14938146780815,0.));
#115783=CARTESIAN_POINT('Ctrl Pts',(70.1795213481185,7.15727679700934,0.));
#115784=CARTESIAN_POINT('Ctrl Pts',(70.1988700934593,7.16521142033865,0.));
#115785=CARTESIAN_POINT('Ctrl Pts',(70.2182569618994,7.17318534889717,0.));
#115786=CARTESIAN_POINT('Ctrl Pts',(70.2376817702215,7.18119859359779,0.));
#115787=CARTESIAN_POINT('Ctrl Pts',(70.2571443365192,7.18925116517556,0.));
#115788=CARTESIAN_POINT('Ctrl Pts',(70.2766444798285,7.19734307419874,0.));
#115789=CARTESIAN_POINT('Ctrl Pts',(70.2961820197077,7.20547433107483,0.));
#115790=CARTESIAN_POINT('Ctrl Pts',(70.3157567762588,7.21364494605451,0.));
#115791=CARTESIAN_POINT('Ctrl Pts',(70.3353685703112,7.22185492923192,0.));
#115792=CARTESIAN_POINT('Ctrl Pts',(70.3550172235486,7.2301042905423,0.));
#115793=CARTESIAN_POINT('Ctrl Pts',(70.3747025586552,7.23839303975608,0.));
#115794=CARTESIAN_POINT('Ctrl Pts',(70.3944243994504,7.24672118647086,0.));
#115795=CARTESIAN_POINT('Ctrl Pts',(70.4141825708178,7.25508874012044,0.));
#115796=CARTESIAN_POINT('Ctrl Pts',(70.4339768986346,7.26349570998034,0.));
#115797=CARTESIAN_POINT('Ctrl Pts',(70.4538072096992,7.27194210517064,0.));
#115798=CARTESIAN_POINT('Ctrl Pts',(70.4736733316487,7.28042793465472,0.));
#115799=CARTESIAN_POINT('Ctrl Pts',(70.4935750929058,7.28895320723863,0.));
#115800=CARTESIAN_POINT('Ctrl Pts',(70.5135123227169,7.29751793157824,0.));
#115801=CARTESIAN_POINT('Ctrl Pts',(70.5334848511681,7.30612211618054,0.));
#115802=CARTESIAN_POINT('Ctrl Pts',(70.5534925092043,7.31476576940393,0.));
#115803=CARTESIAN_POINT('Ctrl Pts',(70.5735351286476,7.32344889945221,0.));
#115804=CARTESIAN_POINT('Ctrl Pts',(70.5936125421946,7.33217151437592,0.));
#115805=CARTESIAN_POINT('Ctrl Pts',(70.6137245833996,7.34093362208009,0.));
#115806=CARTESIAN_POINT('Ctrl Pts',(70.6338710866562,7.34973523032579,0.));
#115807=CARTESIAN_POINT('Ctrl Pts',(70.6540518871775,7.35857634673056,0.));
#115808=CARTESIAN_POINT('Ctrl Pts',(70.6742668209687,7.36745697876302,0.));
#115809=CARTESIAN_POINT('Ctrl Pts',(70.694515724827,7.37637713374769,0.));
#115810=CARTESIAN_POINT('Ctrl Pts',(70.7147984363424,7.38533681887033,0.));
#115811=CARTESIAN_POINT('Ctrl Pts',(70.735114793895,7.39433604117892,0.));
#115812=CARTESIAN_POINT('Ctrl Pts',(70.7554646366514,7.40337480758231,0.));
#115813=CARTESIAN_POINT('Ctrl Pts',(70.7758478045576,7.41245312484488,0.));
#115814=CARTESIAN_POINT('Ctrl Pts',(70.7962641383351,7.42157099959317,0.));
#115815=CARTESIAN_POINT('Ctrl Pts',(70.8167134794738,7.43072843832009,0.));
#115816=CARTESIAN_POINT('Ctrl Pts',(70.8371956702242,7.43992544738608,0.));
#115817=CARTESIAN_POINT('Ctrl Pts',(70.8577105535841,7.44916203301646,0.));
#115818=CARTESIAN_POINT('Ctrl Pts',(70.8782579732885,7.45843820129777,0.));
#115819=CARTESIAN_POINT('Ctrl Pts',(70.8988377738088,7.4677539581852,0.));
#115820=CARTESIAN_POINT('Ctrl Pts',(70.9194498003483,7.47710930950555,0.));
#115821=CARTESIAN_POINT('Ctrl Pts',(70.9400938988373,7.48650426095824,0.));
#115822=CARTESIAN_POINT('Ctrl Pts',(70.9607699159234,7.49593881811142,0.));
#115823=CARTESIAN_POINT('Ctrl Pts',(70.9814776989637,7.5054129863995,0.));
#115824=CARTESIAN_POINT('Ctrl Pts',(71.0022170960235,7.51492677113113,0.));
#115825=CARTESIAN_POINT('Ctrl Pts',(71.0229879558713,7.52448017749137,0.));
#115826=CARTESIAN_POINT('Ctrl Pts',(71.0437901279722,7.53407321054255,0.));
#115827=CARTESIAN_POINT('Ctrl Pts',(71.0646234624783,7.5437058752195,0.));
#115828=CARTESIAN_POINT('Ctrl Pts',(71.0854878102203,7.55337817632874,0.));
#115829=CARTESIAN_POINT('Ctrl Pts',(71.1063830227074,7.56309011855618,0.));
#115830=CARTESIAN_POINT('Ctrl Pts',(71.1273089521218,7.57284170646867,0.));
#115831=CARTESIAN_POINT('Ctrl Pts',(71.1482654513133,7.58263294451467,0.));
#115832=CARTESIAN_POINT('Ctrl Pts',(71.1692523737887,7.59246383701861,0.));
#115833=CARTESIAN_POINT('Ctrl Pts',(71.1902695737063,7.60233438818157,0.));
#115834=CARTESIAN_POINT('Ctrl Pts',(71.2113169058778,7.61224460208888,0.));
#115835=CARTESIAN_POINT('Ctrl Pts',(71.232394225762,7.62219448271126,0.));
#115836=CARTESIAN_POINT('Ctrl Pts',(71.2535013894587,7.63218403390516,0.));
#115837=CARTESIAN_POINT('Ctrl Pts',(71.2746382536974,7.64221325940673,0.));
#115838=CARTESIAN_POINT('Ctrl Pts',(71.2958046758334,7.65228216283344,0.));
#115839=CARTESIAN_POINT('Ctrl Pts',(71.3170005138474,7.6623907476912,0.));
#115840=CARTESIAN_POINT('Ctrl Pts',(71.3382256263405,7.67253901737541,0.));
#115841=CARTESIAN_POINT('Ctrl Pts',(71.3594798725294,7.68272697517104,0.));
#115842=CARTESIAN_POINT('Ctrl Pts',(71.380763112236,7.69295462424648,0.));
#115843=CARTESIAN_POINT('Ctrl Pts',(71.4020752058827,7.70322196765574,0.));
#115844=CARTESIAN_POINT('Ctrl Pts',(71.4234160144943,7.71352900834539,0.));
#115845=CARTESIAN_POINT('Ctrl Pts',(71.4447853996919,7.72387574915546,0.));
#115846=CARTESIAN_POINT('Ctrl Pts',(71.4661832236881,7.73426219281933,0.));
#115847=CARTESIAN_POINT('Ctrl Pts',(71.487609349277,7.74468834195735,0.));
#115848=CARTESIAN_POINT('Ctrl Pts',(71.5090636398307,7.75515419907956,0.));
#115849=CARTESIAN_POINT('Ctrl Pts',(71.5305459592987,7.7656597665922,0.));
#115850=CARTESIAN_POINT('Ctrl Pts',(71.5520561722039,7.77620504679869,0.));
#115851=CARTESIAN_POINT('Ctrl Pts',(71.5735941436366,7.78679004189936,0.));
#115852=CARTESIAN_POINT('Ctrl Pts',(71.5951597392471,7.79741475398513,0.));
#115853=CARTESIAN_POINT('Ctrl Pts',(71.616752825242,7.80807918504018,0.));
#115854=CARTESIAN_POINT('Ctrl Pts',(71.638373268384,7.81878333694857,0.));
#115855=CARTESIAN_POINT('Ctrl Pts',(71.6600209359869,7.82952721149505,0.));
#115856=CARTESIAN_POINT('Ctrl Pts',(71.681695695912,7.8403108103649,0.));
#115857=CARTESIAN_POINT('Ctrl Pts',(71.7033974165576,7.8511341351374,0.));
#115858=CARTESIAN_POINT('Ctrl Pts',(71.7251259668573,7.86199718728831,0.));
#115859=CARTESIAN_POINT('Ctrl Pts',(71.7468812162795,7.87289996819656,0.));
#115860=CARTESIAN_POINT('Ctrl Pts',(71.768663034824,7.88384247914523,0.));
#115861=CARTESIAN_POINT('Ctrl Pts',(71.7904712930172,7.89482472132136,0.));
#115862=CARTESIAN_POINT('Ctrl Pts',(71.8123058619038,7.90584669580957,0.));
#115863=CARTESIAN_POINT('Ctrl Pts',(71.8341666130424,7.91690840359372,0.));
#115864=CARTESIAN_POINT('Ctrl Pts',(71.8560534185071,7.92800984556401,0.));
#115865=CARTESIAN_POINT('Ctrl Pts',(71.8779661508833,7.93915102251797,0.));
#115866=CARTESIAN_POINT('Ctrl Pts',(71.8999046832642,7.95033193516047,0.));
#115867=CARTESIAN_POINT('Ctrl Pts',(71.9218688892426,7.96155258409753,0.));
#115868=CARTESIAN_POINT('Ctrl Pts',(71.9438586429072,7.97281296983703,0.));
#115869=CARTESIAN_POINT('Ctrl Pts',(71.9658738188421,7.98411309279599,0.));
#115870=CARTESIAN_POINT('Ctrl Pts',(71.9879142921248,7.99545295330183,0.));
#115871=CARTESIAN_POINT('Ctrl Pts',(72.0099799383216,8.00683255159251,0.));
#115872=CARTESIAN_POINT('Ctrl Pts',(72.0320706334802,8.01825188781071,0.));
#115873=CARTESIAN_POINT('Ctrl Pts',(72.0541862541262,8.0297109620033,0.));
#115874=CARTESIAN_POINT('Ctrl Pts',(72.0763266772632,8.04120977412893,0.));
#115875=CARTESIAN_POINT('Ctrl Pts',(72.0984917803702,8.05274832405958,0.));
#115876=CARTESIAN_POINT('Ctrl Pts',(72.1206814413985,8.06432661158091,0.));
#115877=CARTESIAN_POINT('Ctrl Pts',(72.1428955387648,8.07594463638701,0.));
#115878=CARTESIAN_POINT('Ctrl Pts',(72.165133951346,8.08760239807816,0.));
#115879=CARTESIAN_POINT('Ctrl Pts',(72.18739655848,8.09929989616875,0.));
#115880=CARTESIAN_POINT('Ctrl Pts',(72.2096832399626,8.11103713008923,0.));
#115881=CARTESIAN_POINT('Ctrl Pts',(72.2319938760451,8.12281409918663,0.));
#115882=CARTESIAN_POINT('Ctrl Pts',(72.2543283474279,8.1346308027203,0.));
#115883=CARTESIAN_POINT('Ctrl Pts',(72.2766865352552,8.14648723985794,0.));
#115884=CARTESIAN_POINT('Ctrl Pts',(72.2990683211155,8.15838340968329,0.));
#115885=CARTESIAN_POINT('Ctrl Pts',(72.3214735870402,8.17031931119883,0.));
#115886=CARTESIAN_POINT('Ctrl Pts',(72.3439022155007,8.18229494332623,0.));
#115887=CARTESIAN_POINT('Ctrl Pts',(72.3663540894034,8.1943103049032,0.));
#115888=CARTESIAN_POINT('Ctrl Pts',(72.3888290920845,8.20636539467783,0.));
#115889=CARTESIAN_POINT('Ctrl Pts',(72.4113271073091,8.21846021131565,0.));
#115890=CARTESIAN_POINT('Ctrl Pts',(72.4338480192701,8.23059475340355,0.));
#115891=CARTESIAN_POINT('Ctrl Pts',(72.4563917125842,8.24276901945038,0.));
#115892=CARTESIAN_POINT('Ctrl Pts',(72.4789580722871,8.25498300788494,0.));
#115893=CARTESIAN_POINT('Ctrl Pts',(72.501546983825,8.26723671704925,0.));
#115894=CARTESIAN_POINT('Ctrl Pts',(72.524158333056,8.27953014520386,0.));
#115895=CARTESIAN_POINT('Ctrl Pts',(72.5467920062522,8.2918632905329,0.));
#115896=CARTESIAN_POINT('Ctrl Pts',(72.5694478900983,8.30423615114456,0.));
#115897=CARTESIAN_POINT('Ctrl Pts',(72.5921258716899,8.3166487250701,0.));
#115898=CARTESIAN_POINT('Ctrl Pts',(72.614825838529,8.32910101025654,0.));
#115899=CARTESIAN_POINT('Ctrl Pts',(72.6375476785208,8.34159300456966,0.));
#115900=CARTESIAN_POINT('Ctrl Pts',(72.6602912799689,8.35412470580084,0.));
#115901=CARTESIAN_POINT('Ctrl Pts',(72.68305653157,8.36669611166835,0.));
#115902=CARTESIAN_POINT('Ctrl Pts',(72.7058433224072,8.37930721981736,0.));
#115903=CARTESIAN_POINT('Ctrl Pts',(72.728651541938,8.39195802781408,0.));
#115904=CARTESIAN_POINT('Ctrl Pts',(72.7514810799932,8.40464853314494,0.));
#115905=CARTESIAN_POINT('Ctrl Pts',(72.7743318267876,8.41737873322354,0.));
#115906=CARTESIAN_POINT('Ctrl Pts',(72.7972036729283,8.43014862539172,0.));
#115907=CARTESIAN_POINT('Ctrl Pts',(72.8200965094197,8.44295820691908,0.));
#115908=CARTESIAN_POINT('Ctrl Pts',(72.8430102276703,8.45580747499772,0.));
#115909=CARTESIAN_POINT('Ctrl Pts',(72.8659447194918,8.46869642673764,0.));
#115910=CARTESIAN_POINT('Ctrl Pts',(72.888899877077,8.48162505917629,0.));
#115911=CARTESIAN_POINT('Ctrl Pts',(72.9118755929785,8.49459336928277,0.));
#115912=CARTESIAN_POINT('Ctrl Pts',(72.9348717600837,8.5076013539598,0.));
#115913=CARTESIAN_POINT('Ctrl Pts',(72.9578882715923,8.52064901004245,0.));
#115914=CARTESIAN_POINT('Ctrl Pts',(72.9809250209843,8.53373633429304,0.));
#115915=CARTESIAN_POINT('Ctrl Pts',(73.0039819020663,8.5468633234044,0.));
#115916=CARTESIAN_POINT('Ctrl Pts',(73.0270588090193,8.56002997400097,0.));
#115917=CARTESIAN_POINT('Ctrl Pts',(73.0501556364482,8.57323628263596,0.));
#115918=CARTESIAN_POINT('Ctrl Pts',(73.073272279419,8.58648224578724,0.));
#115919=CARTESIAN_POINT('Ctrl Pts',(73.0964086335226,8.5997678598454,0.));
#115920=CARTESIAN_POINT('Ctrl Pts',(73.1195645948169,8.6130931211199,0.));
#115921=CARTESIAN_POINT('Ctrl Pts',(73.142740059703,8.62645802585476,0.));
#115922=CARTESIAN_POINT('Ctrl Pts',(73.165934924813,8.63986257023736,0.));
#115923=CARTESIAN_POINT('Ctrl Pts',(73.1891490869057,8.65330675040537,0.));
#115924=CARTESIAN_POINT('Ctrl Pts',(73.2123824427212,8.66679056245097,0.));
#115925=CARTESIAN_POINT('Ctrl Pts',(73.2356348889704,8.68031400241885,0.));
#115926=CARTESIAN_POINT('Ctrl Pts',(73.2589063226373,8.69387706629305,0.));
#115927=CARTESIAN_POINT('Ctrl Pts',(73.282196641216,8.70747974998246,0.));
#115928=CARTESIAN_POINT('Ctrl Pts',(73.3055057429744,8.72112204930233,0.));
#115929=CARTESIAN_POINT('Ctrl Pts',(73.3288335271989,8.73480395995361,0.));
#115930=CARTESIAN_POINT('Ctrl Pts',(73.3521798944595,8.74852547749737,0.));
#115931=CARTESIAN_POINT('Ctrl Pts',(73.3755447460235,8.76228659740306,0.));
#115932=CARTESIAN_POINT('Ctrl Pts',(73.3989279832808,8.77608731509305,0.));
#115933=CARTESIAN_POINT('Ctrl Pts',(73.422329507112,8.78992762598739,0.));
#115934=CARTESIAN_POINT('Ctrl Pts',(73.4457492173949,8.80380752553715,0.));
#115935=CARTESIAN_POINT('Ctrl Pts',(73.4691870121608,8.81772700927594,0.));
#115936=CARTESIAN_POINT('Ctrl Pts',(73.4926427882787,8.83168607277416,0.));
#115937=CARTESIAN_POINT('Ctrl Pts',(73.5161164429765,8.84568471153895,0.));
#115938=CARTESIAN_POINT('Ctrl Pts',(73.5396078751672,8.85972292092184,0.));
#115939=CARTESIAN_POINT('Ctrl Pts',(73.5631169867113,8.87380069602956,0.));
#115940=CARTESIAN_POINT('Ctrl Pts',(73.5866436840493,8.88791803160342,0.));
#115941=CARTESIAN_POINT('Ctrl Pts',(73.6101878785868,8.90207492198872,0.));
#115942=CARTESIAN_POINT('Ctrl Pts',(73.6303847393446,8.91424402151035,0.));
#115943=CARTESIAN_POINT('Ctrl Pts',(73.6458786305791,8.92359518177574,0.));
#115944=CARTESIAN_POINT('Ctrl Pts',(73.6566618621802,8.93011088816058,0.));
#115945=CARTESIAN_POINT('Ctrl Pts',(73.6627293782269,8.93377955964027,0.));
#115946=CARTESIAN_POINT('Ctrl Pts',(73.6640787197679,8.93459554655865,0.));
#115947=CARTESIAN_POINT('',(69.6540253893192,6.95102489306927,12.));
#115948=CARTESIAN_POINT('',(69.6540253893192,6.95102489306927,0.));
#115949=CARTESIAN_POINT('Ctrl Pts',(73.664078719768,8.93459554655874,12.));
#115950=CARTESIAN_POINT('Ctrl Pts',(73.662729378227,8.93377955964033,12.));
#115951=CARTESIAN_POINT('Ctrl Pts',(73.6566618621802,8.93011088816063,12.));
#115952=CARTESIAN_POINT('Ctrl Pts',(73.6458786305792,8.92359518177578,12.));
#115953=CARTESIAN_POINT('Ctrl Pts',(73.6303847393446,8.91424402151036,12.));
#115954=CARTESIAN_POINT('Ctrl Pts',(73.6101878785868,8.90207492198872,12.));
#115955=CARTESIAN_POINT('Ctrl Pts',(73.5866436840493,8.88791803160342,12.));
#115956=CARTESIAN_POINT('Ctrl Pts',(73.5631169867113,8.87380069602956,12.));
#115957=CARTESIAN_POINT('Ctrl Pts',(73.5396078751672,8.85972292092184,12.));
#115958=CARTESIAN_POINT('Ctrl Pts',(73.5161164429765,8.84568471153895,12.));
#115959=CARTESIAN_POINT('Ctrl Pts',(73.4926427882787,8.83168607277416,12.));
#115960=CARTESIAN_POINT('Ctrl Pts',(73.4691870121608,8.81772700927594,12.));
#115961=CARTESIAN_POINT('Ctrl Pts',(73.4457492173949,8.80380752553715,12.));
#115962=CARTESIAN_POINT('Ctrl Pts',(73.422329507112,8.78992762598739,12.));
#115963=CARTESIAN_POINT('Ctrl Pts',(73.3989279832808,8.77608731509305,12.));
#115964=CARTESIAN_POINT('Ctrl Pts',(73.3755447460235,8.76228659740306,12.));
#115965=CARTESIAN_POINT('Ctrl Pts',(73.3521798944595,8.74852547749737,12.));
#115966=CARTESIAN_POINT('Ctrl Pts',(73.3288335271989,8.73480395995361,12.));
#115967=CARTESIAN_POINT('Ctrl Pts',(73.3055057429744,8.72112204930233,12.));
#115968=CARTESIAN_POINT('Ctrl Pts',(73.282196641216,8.70747974998246,12.));
#115969=CARTESIAN_POINT('Ctrl Pts',(73.2589063226373,8.69387706629305,12.));
#115970=CARTESIAN_POINT('Ctrl Pts',(73.2356348889704,8.68031400241885,12.));
#115971=CARTESIAN_POINT('Ctrl Pts',(73.2123824427212,8.66679056245097,12.));
#115972=CARTESIAN_POINT('Ctrl Pts',(73.1891490869057,8.65330675040537,12.));
#115973=CARTESIAN_POINT('Ctrl Pts',(73.165934924813,8.63986257023736,12.));
#115974=CARTESIAN_POINT('Ctrl Pts',(73.142740059703,8.62645802585476,12.));
#115975=CARTESIAN_POINT('Ctrl Pts',(73.1195645948169,8.6130931211199,12.));
#115976=CARTESIAN_POINT('Ctrl Pts',(73.0964086335226,8.5997678598454,12.));
#115977=CARTESIAN_POINT('Ctrl Pts',(73.073272279419,8.58648224578724,12.));
#115978=CARTESIAN_POINT('Ctrl Pts',(73.0501556364482,8.57323628263596,12.));
#115979=CARTESIAN_POINT('Ctrl Pts',(73.0270588090193,8.56002997400097,12.));
#115980=CARTESIAN_POINT('Ctrl Pts',(73.0039819020663,8.5468633234044,12.));
#115981=CARTESIAN_POINT('Ctrl Pts',(72.9809250209843,8.53373633429304,12.));
#115982=CARTESIAN_POINT('Ctrl Pts',(72.9578882715923,8.52064901004245,12.));
#115983=CARTESIAN_POINT('Ctrl Pts',(72.9348717600837,8.5076013539598,12.));
#115984=CARTESIAN_POINT('Ctrl Pts',(72.9118755929785,8.49459336928277,12.));
#115985=CARTESIAN_POINT('Ctrl Pts',(72.888899877077,8.48162505917629,12.));
#115986=CARTESIAN_POINT('Ctrl Pts',(72.8659447194918,8.46869642673764,12.));
#115987=CARTESIAN_POINT('Ctrl Pts',(72.8430102276703,8.45580747499772,12.));
#115988=CARTESIAN_POINT('Ctrl Pts',(72.8200965094197,8.44295820691908,12.));
#115989=CARTESIAN_POINT('Ctrl Pts',(72.7972036729283,8.43014862539172,12.));
#115990=CARTESIAN_POINT('Ctrl Pts',(72.7743318267876,8.41737873322354,12.));
#115991=CARTESIAN_POINT('Ctrl Pts',(72.7514810799932,8.40464853314494,12.));
#115992=CARTESIAN_POINT('Ctrl Pts',(72.728651541938,8.39195802781408,12.));
#115993=CARTESIAN_POINT('Ctrl Pts',(72.7058433224072,8.37930721981736,12.));
#115994=CARTESIAN_POINT('Ctrl Pts',(72.68305653157,8.36669611166835,12.));
#115995=CARTESIAN_POINT('Ctrl Pts',(72.6602912799689,8.35412470580084,12.));
#115996=CARTESIAN_POINT('Ctrl Pts',(72.6375476785208,8.34159300456966,12.));
#115997=CARTESIAN_POINT('Ctrl Pts',(72.614825838529,8.32910101025654,12.));
#115998=CARTESIAN_POINT('Ctrl Pts',(72.5921258716899,8.3166487250701,12.));
#115999=CARTESIAN_POINT('Ctrl Pts',(72.5694478900983,8.30423615114456,12.));
#116000=CARTESIAN_POINT('Ctrl Pts',(72.5467920062522,8.2918632905329,12.));
#116001=CARTESIAN_POINT('Ctrl Pts',(72.524158333056,8.27953014520386,12.));
#116002=CARTESIAN_POINT('Ctrl Pts',(72.501546983825,8.26723671704925,12.));
#116003=CARTESIAN_POINT('Ctrl Pts',(72.4789580722871,8.25498300788494,12.));
#116004=CARTESIAN_POINT('Ctrl Pts',(72.4563917125842,8.24276901945038,12.));
#116005=CARTESIAN_POINT('Ctrl Pts',(72.4338480192701,8.23059475340355,12.));
#116006=CARTESIAN_POINT('Ctrl Pts',(72.4113271073091,8.21846021131565,12.));
#116007=CARTESIAN_POINT('Ctrl Pts',(72.3888290920845,8.20636539467783,12.));
#116008=CARTESIAN_POINT('Ctrl Pts',(72.3663540894034,8.1943103049032,12.));
#116009=CARTESIAN_POINT('Ctrl Pts',(72.3439022155007,8.18229494332623,12.));
#116010=CARTESIAN_POINT('Ctrl Pts',(72.3214735870402,8.17031931119883,12.));
#116011=CARTESIAN_POINT('Ctrl Pts',(72.2990683211155,8.15838340968329,12.));
#116012=CARTESIAN_POINT('Ctrl Pts',(72.2766865352552,8.14648723985794,12.));
#116013=CARTESIAN_POINT('Ctrl Pts',(72.2543283474279,8.1346308027203,12.));
#116014=CARTESIAN_POINT('Ctrl Pts',(72.2319938760451,8.12281409918663,12.));
#116015=CARTESIAN_POINT('Ctrl Pts',(72.2096832399626,8.11103713008923,12.));
#116016=CARTESIAN_POINT('Ctrl Pts',(72.18739655848,8.09929989616875,12.));
#116017=CARTESIAN_POINT('Ctrl Pts',(72.165133951346,8.08760239807816,12.));
#116018=CARTESIAN_POINT('Ctrl Pts',(72.1428955387648,8.07594463638701,12.));
#116019=CARTESIAN_POINT('Ctrl Pts',(72.1206814413985,8.06432661158091,12.));
#116020=CARTESIAN_POINT('Ctrl Pts',(72.0984917803702,8.05274832405958,12.));
#116021=CARTESIAN_POINT('Ctrl Pts',(72.0763266772632,8.04120977412893,12.));
#116022=CARTESIAN_POINT('Ctrl Pts',(72.0541862541262,8.0297109620033,12.));
#116023=CARTESIAN_POINT('Ctrl Pts',(72.0320706334802,8.01825188781071,12.));
#116024=CARTESIAN_POINT('Ctrl Pts',(72.0099799383216,8.00683255159251,12.));
#116025=CARTESIAN_POINT('Ctrl Pts',(71.9879142921248,7.99545295330183,12.));
#116026=CARTESIAN_POINT('Ctrl Pts',(71.9658738188421,7.98411309279599,12.));
#116027=CARTESIAN_POINT('Ctrl Pts',(71.9438586429072,7.97281296983703,12.));
#116028=CARTESIAN_POINT('Ctrl Pts',(71.9218688892426,7.96155258409753,12.));
#116029=CARTESIAN_POINT('Ctrl Pts',(71.8999046832642,7.95033193516047,12.));
#116030=CARTESIAN_POINT('Ctrl Pts',(71.8779661508833,7.93915102251797,12.));
#116031=CARTESIAN_POINT('Ctrl Pts',(71.8560534185071,7.92800984556401,12.));
#116032=CARTESIAN_POINT('Ctrl Pts',(71.8341666130424,7.91690840359372,12.));
#116033=CARTESIAN_POINT('Ctrl Pts',(71.8123058619038,7.90584669580957,12.));
#116034=CARTESIAN_POINT('Ctrl Pts',(71.7904712930172,7.89482472132136,12.));
#116035=CARTESIAN_POINT('Ctrl Pts',(71.768663034824,7.88384247914523,12.));
#116036=CARTESIAN_POINT('Ctrl Pts',(71.7468812162795,7.87289996819656,12.));
#116037=CARTESIAN_POINT('Ctrl Pts',(71.7251259668573,7.86199718728831,12.));
#116038=CARTESIAN_POINT('Ctrl Pts',(71.7033974165576,7.8511341351374,12.));
#116039=CARTESIAN_POINT('Ctrl Pts',(71.681695695912,7.8403108103649,12.));
#116040=CARTESIAN_POINT('Ctrl Pts',(71.6600209359869,7.82952721149505,12.));
#116041=CARTESIAN_POINT('Ctrl Pts',(71.638373268384,7.81878333694857,12.));
#116042=CARTESIAN_POINT('Ctrl Pts',(71.616752825242,7.80807918504018,12.));
#116043=CARTESIAN_POINT('Ctrl Pts',(71.5951597392471,7.79741475398513,12.));
#116044=CARTESIAN_POINT('Ctrl Pts',(71.5735941436366,7.78679004189936,12.));
#116045=CARTESIAN_POINT('Ctrl Pts',(71.5520561722039,7.77620504679869,12.));
#116046=CARTESIAN_POINT('Ctrl Pts',(71.5305459592987,7.7656597665922,12.));
#116047=CARTESIAN_POINT('Ctrl Pts',(71.5090636398307,7.75515419907956,12.));
#116048=CARTESIAN_POINT('Ctrl Pts',(71.487609349277,7.74468834195735,12.));
#116049=CARTESIAN_POINT('Ctrl Pts',(71.4661832236881,7.73426219281933,12.));
#116050=CARTESIAN_POINT('Ctrl Pts',(71.4447853996919,7.72387574915546,12.));
#116051=CARTESIAN_POINT('Ctrl Pts',(71.4234160144943,7.71352900834539,12.));
#116052=CARTESIAN_POINT('Ctrl Pts',(71.4020752058827,7.70322196765574,12.));
#116053=CARTESIAN_POINT('Ctrl Pts',(71.380763112236,7.69295462424648,12.));
#116054=CARTESIAN_POINT('Ctrl Pts',(71.3594798725294,7.68272697517104,12.));
#116055=CARTESIAN_POINT('Ctrl Pts',(71.3382256263405,7.67253901737541,12.));
#116056=CARTESIAN_POINT('Ctrl Pts',(71.3170005138474,7.6623907476912,12.));
#116057=CARTESIAN_POINT('Ctrl Pts',(71.2958046758334,7.65228216283344,12.));
#116058=CARTESIAN_POINT('Ctrl Pts',(71.2746382536974,7.64221325940673,12.));
#116059=CARTESIAN_POINT('Ctrl Pts',(71.2535013894587,7.63218403390516,12.));
#116060=CARTESIAN_POINT('Ctrl Pts',(71.232394225762,7.62219448271126,12.));
#116061=CARTESIAN_POINT('Ctrl Pts',(71.2113169058778,7.61224460208888,12.));
#116062=CARTESIAN_POINT('Ctrl Pts',(71.1902695737063,7.60233438818157,12.));
#116063=CARTESIAN_POINT('Ctrl Pts',(71.1692523737887,7.59246383701861,12.));
#116064=CARTESIAN_POINT('Ctrl Pts',(71.1482654513133,7.58263294451467,12.));
#116065=CARTESIAN_POINT('Ctrl Pts',(71.1273089521218,7.57284170646867,12.));
#116066=CARTESIAN_POINT('Ctrl Pts',(71.1063830227074,7.56309011855618,12.));
#116067=CARTESIAN_POINT('Ctrl Pts',(71.0854878102203,7.55337817632874,12.));
#116068=CARTESIAN_POINT('Ctrl Pts',(71.0646234624783,7.5437058752195,12.));
#116069=CARTESIAN_POINT('Ctrl Pts',(71.0437901279722,7.53407321054255,12.));
#116070=CARTESIAN_POINT('Ctrl Pts',(71.0229879558713,7.52448017749137,12.));
#116071=CARTESIAN_POINT('Ctrl Pts',(71.0022170960235,7.51492677113113,12.));
#116072=CARTESIAN_POINT('Ctrl Pts',(70.9814776989637,7.5054129863995,12.));
#116073=CARTESIAN_POINT('Ctrl Pts',(70.9607699159234,7.49593881811142,12.));
#116074=CARTESIAN_POINT('Ctrl Pts',(70.9400938988373,7.48650426095824,12.));
#116075=CARTESIAN_POINT('Ctrl Pts',(70.9194498003483,7.47710930950555,12.));
#116076=CARTESIAN_POINT('Ctrl Pts',(70.8988377738088,7.4677539581852,12.));
#116077=CARTESIAN_POINT('Ctrl Pts',(70.8782579732885,7.45843820129777,12.));
#116078=CARTESIAN_POINT('Ctrl Pts',(70.8577105535841,7.44916203301646,12.));
#116079=CARTESIAN_POINT('Ctrl Pts',(70.8371956702242,7.43992544738608,12.));
#116080=CARTESIAN_POINT('Ctrl Pts',(70.8167134794738,7.43072843832009,12.));
#116081=CARTESIAN_POINT('Ctrl Pts',(70.7962641383351,7.42157099959317,12.));
#116082=CARTESIAN_POINT('Ctrl Pts',(70.7758478045576,7.41245312484488,12.));
#116083=CARTESIAN_POINT('Ctrl Pts',(70.7554646366514,7.40337480758231,12.));
#116084=CARTESIAN_POINT('Ctrl Pts',(70.735114793895,7.39433604117892,12.));
#116085=CARTESIAN_POINT('Ctrl Pts',(70.7147984363424,7.38533681887033,12.));
#116086=CARTESIAN_POINT('Ctrl Pts',(70.694515724827,7.37637713374769,12.));
#116087=CARTESIAN_POINT('Ctrl Pts',(70.6742668209687,7.36745697876302,12.));
#116088=CARTESIAN_POINT('Ctrl Pts',(70.6540518871775,7.35857634673056,12.));
#116089=CARTESIAN_POINT('Ctrl Pts',(70.6338710866562,7.34973523032579,12.));
#116090=CARTESIAN_POINT('Ctrl Pts',(70.6137245833996,7.34093362208009,12.));
#116091=CARTESIAN_POINT('Ctrl Pts',(70.5936125421946,7.33217151437592,12.));
#116092=CARTESIAN_POINT('Ctrl Pts',(70.5735351286476,7.32344889945221,12.));
#116093=CARTESIAN_POINT('Ctrl Pts',(70.5534925092043,7.31476576940393,12.));
#116094=CARTESIAN_POINT('Ctrl Pts',(70.5334848511681,7.30612211618054,12.));
#116095=CARTESIAN_POINT('Ctrl Pts',(70.5135123227169,7.29751793157824,12.));
#116096=CARTESIAN_POINT('Ctrl Pts',(70.4935750929058,7.28895320723863,12.));
#116097=CARTESIAN_POINT('Ctrl Pts',(70.4736733316487,7.28042793465472,12.));
#116098=CARTESIAN_POINT('Ctrl Pts',(70.4538072096992,7.27194210517064,12.));
#116099=CARTESIAN_POINT('Ctrl Pts',(70.4339768986346,7.26349570998034,12.));
#116100=CARTESIAN_POINT('Ctrl Pts',(70.4141825708178,7.25508874012044,12.));
#116101=CARTESIAN_POINT('Ctrl Pts',(70.3944243994504,7.24672118647086,12.));
#116102=CARTESIAN_POINT('Ctrl Pts',(70.3747025586552,7.23839303975608,12.));
#116103=CARTESIAN_POINT('Ctrl Pts',(70.3550172235486,7.2301042905423,12.));
#116104=CARTESIAN_POINT('Ctrl Pts',(70.3353685703112,7.22185492923192,12.));
#116105=CARTESIAN_POINT('Ctrl Pts',(70.3157567762588,7.21364494605451,12.));
#116106=CARTESIAN_POINT('Ctrl Pts',(70.2961820197077,7.20547433107483,12.));
#116107=CARTESIAN_POINT('Ctrl Pts',(70.2766444798285,7.19734307419874,12.));
#116108=CARTESIAN_POINT('Ctrl Pts',(70.2571443365192,7.18925116517556,12.));
#116109=CARTESIAN_POINT('Ctrl Pts',(70.2376817702215,7.18119859359779,12.));
#116110=CARTESIAN_POINT('Ctrl Pts',(70.2182569618994,7.17318534889717,12.));
#116111=CARTESIAN_POINT('Ctrl Pts',(70.1988700934593,7.16521142033865,12.));
#116112=CARTESIAN_POINT('Ctrl Pts',(70.1795213481185,7.15727679700934,12.));
#116113=CARTESIAN_POINT('Ctrl Pts',(70.1602109107202,7.14938146780815,12.));
#116114=CARTESIAN_POINT('Ctrl Pts',(70.1409389682424,7.14152542142375,12.));
#116115=CARTESIAN_POINT('Ctrl Pts',(70.1217057094499,7.13370864634444,12.));
#116116=CARTESIAN_POINT('Ctrl Pts',(70.1025113239495,7.12593113088905,12.));
#116117=CARTESIAN_POINT('Ctrl Pts',(70.0833560013975,7.11819286322827,12.));
#116118=CARTESIAN_POINT('Ctrl Pts',(70.0642399306869,7.11049383140447,12.));
#116119=CARTESIAN_POINT('Ctrl Pts',(70.0451632990086,7.10283402335035,12.));
#116120=CARTESIAN_POINT('Ctrl Pts',(70.0261262936388,7.0952134268425,12.));
#116121=CARTESIAN_POINT('Ctrl Pts',(70.0071291040766,7.08763202944247,12.));
#116122=CARTESIAN_POINT('Ctrl Pts',(69.988171923788,7.08008981844653,12.));
#116123=CARTESIAN_POINT('Ctrl Pts',(69.9692549527296,7.07258678080832,12.));
#116124=CARTESIAN_POINT('Ctrl Pts',(69.9503783975727,7.06512290312851,12.));
#116125=CARTESIAN_POINT('Ctrl Pts',(69.9315424664291,7.05769817180858,12.));
#116126=CARTESIAN_POINT('Ctrl Pts',(69.9127473642099,7.05031257318117,12.));
#116127=CARTESIAN_POINT('Ctrl Pts',(69.8939932885841,7.04296609362167,12.));
#116128=CARTESIAN_POINT('Ctrl Pts',(69.8752804235238,7.03565871972222,12.));
#116129=CARTESIAN_POINT('Ctrl Pts',(69.8566089455375,7.02839043811814,12.));
#116130=CARTESIAN_POINT('Ctrl Pts',(69.8379790360518,7.02116123514453,12.));
#116131=CARTESIAN_POINT('Ctrl Pts',(69.8193908913722,7.01397109655456,12.));
#116132=CARTESIAN_POINT('Ctrl Pts',(69.8008447346863,7.00682000718152,12.));
#116133=CARTESIAN_POINT('Ctrl Pts',(69.782340824259,6.99970795069477,12.));
#116134=CARTESIAN_POINT('Ctrl Pts',(69.7638794280419,6.99263491027942,12.));
#116135=CARTESIAN_POINT('Ctrl Pts',(69.7454607995607,6.98560086924215,12.));
#116136=CARTESIAN_POINT('Ctrl Pts',(69.7270851557366,6.97860581164528,12.));
#116137=CARTESIAN_POINT('Ctrl Pts',(69.7087526479973,6.97164972291441,12.));
#116138=CARTESIAN_POINT('Ctrl Pts',(69.6904633605421,6.96473259049514,12.));
#116139=CARTESIAN_POINT('Ctrl Pts',(69.6758665380378,6.95923004173592,12.));
#116140=CARTESIAN_POINT('Ctrl Pts',(69.664938391983,6.95512065317601,12.));
#116141=CARTESIAN_POINT('Ctrl Pts',(69.6576616146467,6.95238884849026,12.));
#116142=CARTESIAN_POINT('Ctrl Pts',(69.6540253893192,6.95102489306927,12.));
#116143=CARTESIAN_POINT('Ctrl Pts',(73.466479592994,10.4355099267296,-5.55111512312578E-16));
#116144=CARTESIAN_POINT('Ctrl Pts',(73.466479592994,10.4355099267296,4.));
#116145=CARTESIAN_POINT('Ctrl Pts',(73.466479592994,10.4355099267296,8.));
#116146=CARTESIAN_POINT('Ctrl Pts',(73.466479592994,10.4355099267296,12.));
#116147=CARTESIAN_POINT('Ctrl Pts',(73.5720190200069,10.4049225807075,-5.55111512312578E-16));
#116148=CARTESIAN_POINT('Ctrl Pts',(73.5720190200069,10.4049225807075,4.));
#116149=CARTESIAN_POINT('Ctrl Pts',(73.5720190200068,10.4049225807075,8.));
#116150=CARTESIAN_POINT('Ctrl Pts',(73.5720190200068,10.4049225807075,12.));
#116151=CARTESIAN_POINT('Ctrl Pts',(73.7377969500799,10.2883434191782,-5.55111512312578E-16));
#116152=CARTESIAN_POINT('Ctrl Pts',(73.7377969500799,10.2883434191782,4.));
#116153=CARTESIAN_POINT('Ctrl Pts',(73.7377969500798,10.2883434191783,7.99999999999999));
#116154=CARTESIAN_POINT('Ctrl Pts',(73.7377969500798,10.2883434191783,12.));
#116155=CARTESIAN_POINT('Ctrl Pts',(73.8116652760545,10.1042001607579,-5.55111512312578E-16));
#116156=CARTESIAN_POINT('Ctrl Pts',(73.8116652760545,10.1042001607579,4.));
#116157=CARTESIAN_POINT('Ctrl Pts',(73.8116652760545,10.1042001607579,8.00000000000001));
#116158=CARTESIAN_POINT('Ctrl Pts',(73.8116652760545,10.1042001607579,12.));
#116159=CARTESIAN_POINT('Ctrl Pts',(73.8227522002495,10.0225374821234,-5.55111512312578E-16));
#116160=CARTESIAN_POINT('Ctrl Pts',(73.8227522002495,10.0225374821234,4.));
#116161=CARTESIAN_POINT('Ctrl Pts',(73.8227522002494,10.0225374821234,8.));
#116162=CARTESIAN_POINT('Ctrl Pts',(73.8227522002494,10.0225374821234,12.));
#116163=CARTESIAN_POINT('',(73.466479592994,10.4355099267296,0.));
#116164=CARTESIAN_POINT('',(73.8227522002494,10.0225374821234,0.));
#116165=CARTESIAN_POINT('Ctrl Pts',(73.466479592994,10.4355099267296,2.77555756156289E-16));
#116166=CARTESIAN_POINT('Ctrl Pts',(73.5720190200069,10.4049225807075,2.77555756156289E-16));
#116167=CARTESIAN_POINT('Ctrl Pts',(73.6667492657629,10.3383059169765,2.7755575615629E-16));
#116168=CARTESIAN_POINT('Ctrl Pts',(73.7314682122214,10.2496275073218,2.77555756156289E-16));
#116169=CARTESIAN_POINT('Ctrl Pts',(73.7800074220654,10.1831187000809,2.77555756156289E-16));
#116170=CARTESIAN_POINT('Ctrl Pts',(73.8116652760545,10.1042001607579,2.77555756156288E-16));
#116171=CARTESIAN_POINT('Ctrl Pts',(73.8227522002495,10.0225374821234,2.77555756156289E-16));
#116172=CARTESIAN_POINT('',(73.8227522002494,10.0225374821234,12.));
#116173=CARTESIAN_POINT('Ctrl Pts',(73.8227522002495,10.0225374821234,-5.55111512312578E-16));
#116174=CARTESIAN_POINT('Ctrl Pts',(73.8227522002495,10.0225374821234,4.));
#116175=CARTESIAN_POINT('Ctrl Pts',(73.8227522002494,10.0225374821234,8.));
#116176=CARTESIAN_POINT('Ctrl Pts',(73.8227522002494,10.0225374821234,12.));
#116177=CARTESIAN_POINT('',(73.466479592994,10.4355099267296,12.));
#116178=CARTESIAN_POINT('Ctrl Pts',(73.8227522002494,10.0225374821234,12.));
#116179=CARTESIAN_POINT('Ctrl Pts',(73.8116652760545,10.1042001607579,12.));
#116180=CARTESIAN_POINT('Ctrl Pts',(73.7800074220654,10.1831187000809,12.));
#116181=CARTESIAN_POINT('Ctrl Pts',(73.7314682122214,10.2496275073219,12.));
#116182=CARTESIAN_POINT('Ctrl Pts',(73.6667492657628,10.3383059169765,12.));
#116183=CARTESIAN_POINT('Ctrl Pts',(73.5720190200068,10.4049225807075,12.));
#116184=CARTESIAN_POINT('Ctrl Pts',(73.466479592994,10.4355099267296,12.));
#116185=CARTESIAN_POINT('Ctrl Pts',(73.466479592994,10.4355099267296,12.));
#116186=CARTESIAN_POINT('Ctrl Pts',(73.466479592994,10.4355099267296,8.));
#116187=CARTESIAN_POINT('Ctrl Pts',(73.466479592994,10.4355099267296,4.));
#116188=CARTESIAN_POINT('Ctrl Pts',(73.466479592994,10.4355099267296,-5.55111512312578E-16));
#116189=CARTESIAN_POINT('Origin',(3.71623968689858E-10,4.90253386731614E-11,
0.));
#116190=CARTESIAN_POINT('Origin',(3.71623968689858E-10,4.90253386731614E-11,
12.));
#116191=CARTESIAN_POINT('Origin',(3.71623968689858E-10,4.90253386731614E-11,
0.));
#116192=CARTESIAN_POINT('Ctrl Pts',(74.4537274248118,-2.62535189104657,
0.));
#116193=CARTESIAN_POINT('Ctrl Pts',(74.4537274248118,-2.62535189104657,
12.));
#116194=CARTESIAN_POINT('Ctrl Pts',(74.4487312586601,-2.62283178248298,
0.));
#116195=CARTESIAN_POINT('Ctrl Pts',(74.4487312586601,-2.62283178248298,
12.));
#116196=CARTESIAN_POINT('Ctrl Pts',(74.4387409032582,-2.61779535432371,
0.));
#116197=CARTESIAN_POINT('Ctrl Pts',(74.4387409032582,-2.61779535432371,
12.));
#116198=CARTESIAN_POINT('Ctrl Pts',(74.4237613008609,-2.61025207898831,
0.));
#116199=CARTESIAN_POINT('Ctrl Pts',(74.4237613008609,-2.61025207898831,
12.));
#116200=CARTESIAN_POINT('Ctrl Pts',(74.4038003595514,-2.60021711327492,
0.));
#116201=CARTESIAN_POINT('Ctrl Pts',(74.4038003595514,-2.60021711327492,
12.));
#116202=CARTESIAN_POINT('Ctrl Pts',(74.3788689604,-2.58771130268619,0.));
#116203=CARTESIAN_POINT('Ctrl Pts',(74.3788689604,-2.58771130268619,12.));
#116204=CARTESIAN_POINT('Ctrl Pts',(74.3539573568054,-2.57524339541657,
0.));
#116205=CARTESIAN_POINT('Ctrl Pts',(74.3539573568054,-2.57524339541657,
12.));
#116206=CARTESIAN_POINT('Ctrl Pts',(74.3290655814922,-2.56281339800083,
0.));
#116207=CARTESIAN_POINT('Ctrl Pts',(74.3290655814922,-2.56281339800083,
12.));
#116208=CARTESIAN_POINT('Ctrl Pts',(74.3041936853329,-2.55042131526685,
0.));
#116209=CARTESIAN_POINT('Ctrl Pts',(74.3041936853329,-2.55042131526685,
12.));
#116210=CARTESIAN_POINT('Ctrl Pts',(74.2793417427044,-2.53806714838104,
0.));
#116211=CARTESIAN_POINT('Ctrl Pts',(74.2793417427044,-2.53806714838104,
12.));
#116212=CARTESIAN_POINT('Ctrl Pts',(74.2545098494549,-2.52575089478113,
0.));
#116213=CARTESIAN_POINT('Ctrl Pts',(74.2545098494549,-2.52575089478113,
12.));
#116214=CARTESIAN_POINT('Ctrl Pts',(74.2296981152027,-2.51347254956027,
0.));
#116215=CARTESIAN_POINT('Ctrl Pts',(74.2296981152027,-2.51347254956027,
12.));
#116216=CARTESIAN_POINT('Ctrl Pts',(74.2049066571942,-2.50123210644075,
0.));
#116217=CARTESIAN_POINT('Ctrl Pts',(74.2049066571942,-2.50123210644075,
12.));
#116218=CARTESIAN_POINT('Ctrl Pts',(74.180135593693,-2.48902955888402,0.));
#116219=CARTESIAN_POINT('Ctrl Pts',(74.180135593693,-2.48902955888402,12.));
#116220=CARTESIAN_POINT('Ctrl Pts',(74.1553850371577,-2.47686490120423,
0.));
#116221=CARTESIAN_POINT('Ctrl Pts',(74.1553850371577,-2.47686490120423,
12.));
#116222=CARTESIAN_POINT('Ctrl Pts',(74.1306550887196,-2.46473812948048,
0.));
#116223=CARTESIAN_POINT('Ctrl Pts',(74.1306550887196,-2.46473812948048,
12.));
#116224=CARTESIAN_POINT('Ctrl Pts',(74.1059458420175,-2.45264924094853,
0.));
#116225=CARTESIAN_POINT('Ctrl Pts',(74.1059458420175,-2.45264924094853,
12.));
#116226=CARTESIAN_POINT('Ctrl Pts',(74.0812573859474,-2.44059823356722,
0.));
#116227=CARTESIAN_POINT('Ctrl Pts',(74.0812573859474,-2.44059823356722,
12.));
#116228=CARTESIAN_POINT('Ctrl Pts',(74.0565898079227,-2.42858510549787,
0.));
#116229=CARTESIAN_POINT('Ctrl Pts',(74.0565898079227,-2.42858510549787,
12.));
#116230=CARTESIAN_POINT('Ctrl Pts',(74.0319431966956,-2.41660985465228,
0.));
#116231=CARTESIAN_POINT('Ctrl Pts',(74.0319431966956,-2.41660985465228,
12.));
#116232=CARTESIAN_POINT('Ctrl Pts',(74.0073176459287,-2.40467247811497,
0.));
#116233=CARTESIAN_POINT('Ctrl Pts',(74.0073176459287,-2.40467247811497,
12.));
#116234=CARTESIAN_POINT('Ctrl Pts',(73.9827132538149,-2.39277297220716,
0.));
#116235=CARTESIAN_POINT('Ctrl Pts',(73.9827132538149,-2.39277297220716,
12.));
#116236=CARTESIAN_POINT('Ctrl Pts',(73.9581301214609,-2.38091133274933,
0.));
#116237=CARTESIAN_POINT('Ctrl Pts',(73.9581301214609,-2.38091133274933,
12.));
#116238=CARTESIAN_POINT('Ctrl Pts',(73.9335683516388,-2.36908755525994,
0.));
#116239=CARTESIAN_POINT('Ctrl Pts',(73.9335683516388,-2.36908755525994,
12.));
#116240=CARTESIAN_POINT('Ctrl Pts',(73.9090280474723,-2.35730163516324,
0.));
#116241=CARTESIAN_POINT('Ctrl Pts',(73.9090280474723,-2.35730163516324,
12.));
#116242=CARTESIAN_POINT('Ctrl Pts',(73.8845093109302,-2.3455535680214,0.));
#116243=CARTESIAN_POINT('Ctrl Pts',(73.8845093109302,-2.3455535680214,12.));
#116244=CARTESIAN_POINT('Ctrl Pts',(73.8600122421502,-2.33384334963981,
0.));
#116245=CARTESIAN_POINT('Ctrl Pts',(73.8600122421502,-2.33384334963981,
12.));
#116246=CARTESIAN_POINT('Ctrl Pts',(73.8355369402733,-2.32217097594216,
0.));
#116247=CARTESIAN_POINT('Ctrl Pts',(73.8355369402733,-2.32217097594216,
12.));
#116248=CARTESIAN_POINT('Ctrl Pts',(73.8110835039341,-2.31053644289425,
0.));
#116249=CARTESIAN_POINT('Ctrl Pts',(73.8110835039341,-2.31053644289425,
12.));
#116250=CARTESIAN_POINT('Ctrl Pts',(73.7866520318849,-2.29893974640435,
0.));
#116251=CARTESIAN_POINT('Ctrl Pts',(73.7866520318849,-2.29893974640435,
12.));
#116252=CARTESIAN_POINT('Ctrl Pts',(73.7622426235648,-2.28738088222859,
0.));
#116253=CARTESIAN_POINT('Ctrl Pts',(73.7622426235648,-2.28738088222859,
12.));
#116254=CARTESIAN_POINT('Ctrl Pts',(73.7378553796792,-2.27585984587193,
0.));
#116255=CARTESIAN_POINT('Ctrl Pts',(73.7378553796792,-2.27585984587193,
12.));
#116256=CARTESIAN_POINT('Ctrl Pts',(73.7134904019378,-2.26437663263664,
0.));
#116257=CARTESIAN_POINT('Ctrl Pts',(73.7134904019378,-2.26437663263664,
12.));
#116258=CARTESIAN_POINT('Ctrl Pts',(73.6891477928124,-2.25293123766425,
0.));
#116259=CARTESIAN_POINT('Ctrl Pts',(73.6891477928124,-2.25293123766425,
12.));
#116260=CARTESIAN_POINT('Ctrl Pts',(73.6648276552766,-2.24152365597699,
0.));
#116261=CARTESIAN_POINT('Ctrl Pts',(73.6648276552766,-2.24152365597699,
12.));
#116262=CARTESIAN_POINT('Ctrl Pts',(73.6405300925714,-2.23015388251289,
0.));
#116263=CARTESIAN_POINT('Ctrl Pts',(73.6405300925714,-2.23015388251289,
12.));
#116264=CARTESIAN_POINT('Ctrl Pts',(73.6162552079044,-2.21882191216521,
0.));
#116265=CARTESIAN_POINT('Ctrl Pts',(73.6162552079044,-2.21882191216521,
12.));
#116266=CARTESIAN_POINT('Ctrl Pts',(73.5920031044604,-2.20752773978353,
0.));
#116267=CARTESIAN_POINT('Ctrl Pts',(73.5920031044604,-2.20752773978353,
12.));
#116268=CARTESIAN_POINT('Ctrl Pts',(73.5677738855461,-2.19627136015683,
0.));
#116269=CARTESIAN_POINT('Ctrl Pts',(73.5677738855461,-2.19627136015683,
12.));
#116270=CARTESIAN_POINT('Ctrl Pts',(73.5435676546934,-2.18505276799757,
0.));
#116271=CARTESIAN_POINT('Ctrl Pts',(73.5435676546934,-2.18505276799757,
12.));
#116272=CARTESIAN_POINT('Ctrl Pts',(73.5193845157705,-2.17387195792306,
0.));
#116273=CARTESIAN_POINT('Ctrl Pts',(73.5193845157705,-2.17387195792306,
12.));
#116274=CARTESIAN_POINT('Ctrl Pts',(73.4952245731044,-2.16272892442916,
0.));
#116275=CARTESIAN_POINT('Ctrl Pts',(73.4952245731044,-2.16272892442916,
12.));
#116276=CARTESIAN_POINT('Ctrl Pts',(73.4710879315367,-2.15162366187899,
0.));
#116277=CARTESIAN_POINT('Ctrl Pts',(73.4710879315367,-2.15162366187899,
12.));
#116278=CARTESIAN_POINT('Ctrl Pts',(73.4469746963622,-2.14055616452049,
0.));
#116279=CARTESIAN_POINT('Ctrl Pts',(73.4469746963622,-2.14055616452049,
12.));
#116280=CARTESIAN_POINT('Ctrl Pts',(73.4228849732914,-2.12952642649361,
0.));
#116281=CARTESIAN_POINT('Ctrl Pts',(73.4228849732914,-2.12952642649361,
12.));
#116282=CARTESIAN_POINT('Ctrl Pts',(73.3988188684022,-2.11853444183764,
0.));
#116283=CARTESIAN_POINT('Ctrl Pts',(73.3988188684022,-2.11853444183764,
12.));
#116284=CARTESIAN_POINT('Ctrl Pts',(73.3747764880903,-2.10758020449401,
0.));
#116285=CARTESIAN_POINT('Ctrl Pts',(73.3747764880903,-2.10758020449401,
12.));
#116286=CARTESIAN_POINT('Ctrl Pts',(73.3507579390254,-2.09666370830733,
0.));
#116287=CARTESIAN_POINT('Ctrl Pts',(73.3507579390254,-2.09666370830733,
12.));
#116288=CARTESIAN_POINT('Ctrl Pts',(73.3267633281822,-2.08578494702762,
0.));
#116289=CARTESIAN_POINT('Ctrl Pts',(73.3267633281822,-2.08578494702762,
12.));
#116290=CARTESIAN_POINT('Ctrl Pts',(73.3027927628636,-2.07494391430954,
0.));
#116291=CARTESIAN_POINT('Ctrl Pts',(73.3027927628636,-2.07494391430954,
12.));
#116292=CARTESIAN_POINT('Ctrl Pts',(73.2788463507248,-2.06414060370838,
0.));
#116293=CARTESIAN_POINT('Ctrl Pts',(73.2788463507248,-2.06414060370838,
12.));
#116294=CARTESIAN_POINT('Ctrl Pts',(73.2549241997946,-2.05337500867396,
0.));
#116295=CARTESIAN_POINT('Ctrl Pts',(73.2549241997946,-2.05337500867396,
12.));
#116296=CARTESIAN_POINT('Ctrl Pts',(73.2310264184965,-2.04264712253915,
0.));
#116297=CARTESIAN_POINT('Ctrl Pts',(73.2310264184965,-2.04264712253915,
12.));
#116298=CARTESIAN_POINT('Ctrl Pts',(73.2071531156492,-2.03195693852441,
0.));
#116299=CARTESIAN_POINT('Ctrl Pts',(73.2071531156492,-2.03195693852441,
12.));
#116300=CARTESIAN_POINT('Ctrl Pts',(73.1833044004612,-2.02130444974352,
0.));
#116301=CARTESIAN_POINT('Ctrl Pts',(73.1833044004612,-2.02130444974352,
12.));
#116302=CARTESIAN_POINT('Ctrl Pts',(73.159480382525,-2.01068964920465,0.));
#116303=CARTESIAN_POINT('Ctrl Pts',(73.159480382525,-2.01068964920465,12.));
#116304=CARTESIAN_POINT('Ctrl Pts',(73.1356811718094,-2.00011252980988,
0.));
#116305=CARTESIAN_POINT('Ctrl Pts',(73.1356811718094,-2.00011252980988,
12.));
#116306=CARTESIAN_POINT('Ctrl Pts',(73.1119068786482,-1.9895730843493,0.));
#116307=CARTESIAN_POINT('Ctrl Pts',(73.1119068786482,-1.9895730843493,12.));
#116308=CARTESIAN_POINT('Ctrl Pts',(73.0881576137415,-1.97907130550172,
0.));
#116309=CARTESIAN_POINT('Ctrl Pts',(73.0881576137415,-1.97907130550172,
12.));
#116310=CARTESIAN_POINT('Ctrl Pts',(73.0644334881679,-1.96860718583945,
0.));
#116311=CARTESIAN_POINT('Ctrl Pts',(73.0644334881679,-1.96860718583945,
12.));
#116312=CARTESIAN_POINT('Ctrl Pts',(73.0407346133912,-1.95818071782774,
0.));
#116313=CARTESIAN_POINT('Ctrl Pts',(73.0407346133912,-1.95818071782774,
12.));
#116314=CARTESIAN_POINT('Ctrl Pts',(73.0170611012659,-1.94779189382301,
0.));
#116315=CARTESIAN_POINT('Ctrl Pts',(73.0170611012659,-1.94779189382301,
12.));
#116316=CARTESIAN_POINT('Ctrl Pts',(72.9934130640414,-1.93744070606557,
0.));
#116317=CARTESIAN_POINT('Ctrl Pts',(72.9934130640414,-1.93744070606557,
12.));
#116318=CARTESIAN_POINT('Ctrl Pts',(72.9697906143638,-1.92712714667649,
0.));
#116319=CARTESIAN_POINT('Ctrl Pts',(72.9697906143638,-1.92712714667649,
12.));
#116320=CARTESIAN_POINT('Ctrl Pts',(72.9461938652816,-1.91685120766428,
0.));
#116321=CARTESIAN_POINT('Ctrl Pts',(72.9461938652816,-1.91685120766428,
12.));
#116322=CARTESIAN_POINT('Ctrl Pts',(72.9226229302483,-1.90661288092583,
0.));
#116323=CARTESIAN_POINT('Ctrl Pts',(72.9226229302483,-1.90661288092583,
12.));
#116324=CARTESIAN_POINT('Ctrl Pts',(72.8990779231226,-1.89641215824585,
0.));
#116325=CARTESIAN_POINT('Ctrl Pts',(72.8990779231226,-1.89641215824585,
12.));
#116326=CARTESIAN_POINT('Ctrl Pts',(72.8755589581674,-1.88624903129196,
0.));
#116327=CARTESIAN_POINT('Ctrl Pts',(72.8755589581674,-1.88624903129196,
12.));
#116328=CARTESIAN_POINT('Ctrl Pts',(72.8520661500465,-1.87612349160952,
0.));
#116329=CARTESIAN_POINT('Ctrl Pts',(72.8520661500465,-1.87612349160952,
12.));
#116330=CARTESIAN_POINT('Ctrl Pts',(72.8285996138346,-1.86603553062776,
0.));
#116331=CARTESIAN_POINT('Ctrl Pts',(72.8285996138346,-1.86603553062776,
12.));
#116332=CARTESIAN_POINT('Ctrl Pts',(72.8051594650214,-1.85598513966116,
0.));
#116333=CARTESIAN_POINT('Ctrl Pts',(72.8051594650214,-1.85598513966116,
12.));
#116334=CARTESIAN_POINT('Ctrl Pts',(72.7817458195155,-1.84597230990858,
0.));
#116335=CARTESIAN_POINT('Ctrl Pts',(72.7817458195155,-1.84597230990858,
12.));
#116336=CARTESIAN_POINT('Ctrl Pts',(72.7583587936454,-1.83599703244926,
0.));
#116337=CARTESIAN_POINT('Ctrl Pts',(72.7583587936454,-1.83599703244926,
12.));
#116338=CARTESIAN_POINT('Ctrl Pts',(72.73499850416,-1.82605929823566,0.));
#116339=CARTESIAN_POINT('Ctrl Pts',(72.73499850416,-1.82605929823566,12.));
#116340=CARTESIAN_POINT('Ctrl Pts',(72.7116650682347,-1.81615909809872,
0.));
#116341=CARTESIAN_POINT('Ctrl Pts',(72.7116650682347,-1.81615909809872,
12.));
#116342=CARTESIAN_POINT('Ctrl Pts',(72.6883586034768,-1.80629642275052,
0.));
#116343=CARTESIAN_POINT('Ctrl Pts',(72.6883586034768,-1.80629642275052,
12.));
#116344=CARTESIAN_POINT('Ctrl Pts',(72.6650792279271,-1.79647126278359,
0.));
#116345=CARTESIAN_POINT('Ctrl Pts',(72.6650792279271,-1.79647126278359,
12.));
#116346=CARTESIAN_POINT('Ctrl Pts',(72.6418270600623,-1.78668360866814,
0.));
#116347=CARTESIAN_POINT('Ctrl Pts',(72.6418270600623,-1.78668360866814,
12.));
#116348=CARTESIAN_POINT('Ctrl Pts',(72.618602218792,-1.77693345074431,0.));
#116349=CARTESIAN_POINT('Ctrl Pts',(72.618602218792,-1.77693345074431,12.));
#116350=CARTESIAN_POINT('Ctrl Pts',(72.5954048234655,-1.7672207792258,0.));
#116351=CARTESIAN_POINT('Ctrl Pts',(72.5954048234655,-1.7672207792258,12.));
#116352=CARTESIAN_POINT('Ctrl Pts',(72.5722349938789,-1.7575455842035,0.));
#116353=CARTESIAN_POINT('Ctrl Pts',(72.5722349938789,-1.7575455842035,12.));
#116354=CARTESIAN_POINT('Ctrl Pts',(72.5490928502773,-1.74790785564476,
0.));
#116355=CARTESIAN_POINT('Ctrl Pts',(72.5490928502773,-1.74790785564476,
12.));
#116356=CARTESIAN_POINT('Ctrl Pts',(72.5259785133586,-1.73830758339124,
0.));
#116357=CARTESIAN_POINT('Ctrl Pts',(72.5259785133586,-1.73830758339124,
12.));
#116358=CARTESIAN_POINT('Ctrl Pts',(72.5028921042704,-1.72874475715099,
0.));
#116359=CARTESIAN_POINT('Ctrl Pts',(72.5028921042704,-1.72874475715099,
12.));
#116360=CARTESIAN_POINT('Ctrl Pts',(72.4798337446162,-1.71921936650032,
0.));
#116361=CARTESIAN_POINT('Ctrl Pts',(72.4798337446162,-1.71921936650032,
12.));
#116362=CARTESIAN_POINT('Ctrl Pts',(72.4568035564618,-1.70973140088838,
0.));
#116363=CARTESIAN_POINT('Ctrl Pts',(72.4568035564618,-1.70973140088838,
12.));
#116364=CARTESIAN_POINT('Ctrl Pts',(72.4338016623388,-1.70028084963647,
0.));
#116365=CARTESIAN_POINT('Ctrl Pts',(72.4338016623388,-1.70028084963647,
12.));
#116366=CARTESIAN_POINT('Ctrl Pts',(72.4108281852473,-1.69086770193641,
0.));
#116367=CARTESIAN_POINT('Ctrl Pts',(72.4108281852473,-1.69086770193641,
12.));
#116368=CARTESIAN_POINT('Ctrl Pts',(72.3878832486549,-1.68149194684289,
0.));
#116369=CARTESIAN_POINT('Ctrl Pts',(72.3878832486549,-1.68149194684289,
12.));
#116370=CARTESIAN_POINT('Ctrl Pts',(72.3649669765013,-1.67215357327373,
0.));
#116371=CARTESIAN_POINT('Ctrl Pts',(72.3649669765013,-1.67215357327373,
12.));
#116372=CARTESIAN_POINT('Ctrl Pts',(72.3420794932052,-1.66285257001503,
0.));
#116373=CARTESIAN_POINT('Ctrl Pts',(72.3420794932052,-1.66285257001503,
12.));
#116374=CARTESIAN_POINT('Ctrl Pts',(72.3192209236691,-1.65358892572066,
0.));
#116375=CARTESIAN_POINT('Ctrl Pts',(72.3192209236691,-1.65358892572066,
12.));
#116376=CARTESIAN_POINT('Ctrl Pts',(72.2963913932811,-1.64436262891078,
0.));
#116377=CARTESIAN_POINT('Ctrl Pts',(72.2963913932811,-1.64436262891078,
12.));
#116378=CARTESIAN_POINT('Ctrl Pts',(72.2735910279149,-1.63517366796459,
0.));
#116379=CARTESIAN_POINT('Ctrl Pts',(72.2735910279149,-1.63517366796459,
12.));
#116380=CARTESIAN_POINT('Ctrl Pts',(72.2508199539325,-1.62602203111925,
0.));
#116381=CARTESIAN_POINT('Ctrl Pts',(72.2508199539325,-1.62602203111925,
12.));
#116382=CARTESIAN_POINT('Ctrl Pts',(72.2280782981941,-1.61690770647536,
0.));
#116383=CARTESIAN_POINT('Ctrl Pts',(72.2280782981941,-1.61690770647536,
12.));
#116384=CARTESIAN_POINT('Ctrl Pts',(72.2053661880611,-1.60783068199662,
0.));
#116385=CARTESIAN_POINT('Ctrl Pts',(72.2053661880611,-1.60783068199662,
12.));
#116386=CARTESIAN_POINT('Ctrl Pts',(72.1826837514,-1.5987909455085,0.));
#116387=CARTESIAN_POINT('Ctrl Pts',(72.1826837514,-1.5987909455085,12.));
#116388=CARTESIAN_POINT('Ctrl Pts',(72.1600311165813,-1.58978848469129,
0.));
#116389=CARTESIAN_POINT('Ctrl Pts',(72.1600311165813,-1.58978848469129,
12.));
#116390=CARTESIAN_POINT('Ctrl Pts',(72.1374084124829,-1.58082328707808,
0.));
#116391=CARTESIAN_POINT('Ctrl Pts',(72.1374084124829,-1.58082328707808,
12.));
#116392=CARTESIAN_POINT('Ctrl Pts',(72.1148157684987,-1.57189534006044,
0.));
#116393=CARTESIAN_POINT('Ctrl Pts',(72.1148157684987,-1.57189534006044,
12.));
#116394=CARTESIAN_POINT('Ctrl Pts',(72.092253314543,-1.56300463088811,0.));
#116395=CARTESIAN_POINT('Ctrl Pts',(72.092253314543,-1.56300463088811,12.));
#116396=CARTESIAN_POINT('Ctrl Pts',(72.0697211810548,-1.55415114666774,
0.));
#116397=CARTESIAN_POINT('Ctrl Pts',(72.0697211810548,-1.55415114666774,
12.));
#116398=CARTESIAN_POINT('Ctrl Pts',(72.0472194989968,-1.54533487435627,
0.));
#116399=CARTESIAN_POINT('Ctrl Pts',(72.0472194989968,-1.54533487435627,
12.));
#116400=CARTESIAN_POINT('Ctrl Pts',(72.0247483998582,-1.53655580075814,
0.));
#116401=CARTESIAN_POINT('Ctrl Pts',(72.0247483998582,-1.53655580075814,
12.));
#116402=CARTESIAN_POINT('Ctrl Pts',(72.0023080156647,-1.52781391253104,
0.));
#116403=CARTESIAN_POINT('Ctrl Pts',(72.0023080156647,-1.52781391253104,
12.));
#116404=CARTESIAN_POINT('Ctrl Pts',(71.9798984789828,-1.51910919618567,
0.));
#116405=CARTESIAN_POINT('Ctrl Pts',(71.9798984789828,-1.51910919618567,
12.));
#116406=CARTESIAN_POINT('Ctrl Pts',(71.9575199229241,-1.51044163808455,
0.));
#116407=CARTESIAN_POINT('Ctrl Pts',(71.9575199229241,-1.51044163808455,
12.));
#116408=CARTESIAN_POINT('Ctrl Pts',(71.935172481145,-1.50181122443536,0.));
#116409=CARTESIAN_POINT('Ctrl Pts',(71.935172481145,-1.50181122443536,12.));
#116410=CARTESIAN_POINT('Ctrl Pts',(71.9128562878491,-1.49321794128801,
0.));
#116411=CARTESIAN_POINT('Ctrl Pts',(71.9128562878491,-1.49321794128801,
12.));
#116412=CARTESIAN_POINT('Ctrl Pts',(71.8905714777972,-1.48466177454022,
0.));
#116413=CARTESIAN_POINT('Ctrl Pts',(71.8905714777972,-1.48466177454022,
12.));
#116414=CARTESIAN_POINT('Ctrl Pts',(71.8683181863123,-1.47614270993731,
0.));
#116415=CARTESIAN_POINT('Ctrl Pts',(71.8683181863123,-1.47614270993731,
12.));
#116416=CARTESIAN_POINT('Ctrl Pts',(71.8460965492836,-1.4676607330709,0.));
#116417=CARTESIAN_POINT('Ctrl Pts',(71.8460965492836,-1.4676607330709,12.));
#116418=CARTESIAN_POINT('Ctrl Pts',(71.8239067031664,-1.45921582937229,
0.));
#116419=CARTESIAN_POINT('Ctrl Pts',(71.8239067031664,-1.45921582937229,
12.));
#116420=CARTESIAN_POINT('Ctrl Pts',(71.8017487849865,-1.45080798410957,
0.));
#116421=CARTESIAN_POINT('Ctrl Pts',(71.8017487849865,-1.45080798410957,
12.));
#116422=CARTESIAN_POINT('Ctrl Pts',(71.7796229323496,-1.44243718239305,
0.));
#116423=CARTESIAN_POINT('Ctrl Pts',(71.7796229323496,-1.44243718239305,
12.));
#116424=CARTESIAN_POINT('Ctrl Pts',(71.7575292834456,-1.4341034091749,0.));
#116425=CARTESIAN_POINT('Ctrl Pts',(71.7575292834456,-1.4341034091749,12.));
#116426=CARTESIAN_POINT('Ctrl Pts',(71.7354679770537,-1.42580664924775,
0.));
#116427=CARTESIAN_POINT('Ctrl Pts',(71.7354679770537,-1.42580664924775,
12.));
#116428=CARTESIAN_POINT('Ctrl Pts',(71.7134391525417,-1.41754688723792,
0.));
#116429=CARTESIAN_POINT('Ctrl Pts',(71.7134391525417,-1.41754688723792,
12.));
#116430=CARTESIAN_POINT('Ctrl Pts',(71.6914429498702,-1.40932410760275,
0.));
#116431=CARTESIAN_POINT('Ctrl Pts',(71.6914429498702,-1.40932410760275,
12.));
#116432=CARTESIAN_POINT('Ctrl Pts',(71.6694795096034,-1.401138294636,0.));
#116433=CARTESIAN_POINT('Ctrl Pts',(71.6694795096034,-1.401138294636,12.));
#116434=CARTESIAN_POINT('Ctrl Pts',(71.6475489729149,-1.39298943246732,
0.));
#116435=CARTESIAN_POINT('Ctrl Pts',(71.6475489729149,-1.39298943246732,
12.));
#116436=CARTESIAN_POINT('Ctrl Pts',(71.6256514815918,-1.38487750506076,
0.));
#116437=CARTESIAN_POINT('Ctrl Pts',(71.6256514815918,-1.38487750506076,
12.));
#116438=CARTESIAN_POINT('Ctrl Pts',(71.6037871780347,-1.37680249620763,
0.));
#116439=CARTESIAN_POINT('Ctrl Pts',(71.6037871780347,-1.37680249620763,
12.));
#116440=CARTESIAN_POINT('Ctrl Pts',(71.5819562052613,-1.36876438952449,
0.));
#116441=CARTESIAN_POINT('Ctrl Pts',(71.5819562052613,-1.36876438952449,
12.));
#116442=CARTESIAN_POINT('Ctrl Pts',(71.5601587069175,-1.36076316845807,
0.));
#116443=CARTESIAN_POINT('Ctrl Pts',(71.5601587069175,-1.36076316845807,
12.));
#116444=CARTESIAN_POINT('Ctrl Pts',(71.538394827283,-1.35279881628454,0.));
#116445=CARTESIAN_POINT('Ctrl Pts',(71.538394827283,-1.35279881628454,12.));
#116446=CARTESIAN_POINT('Ctrl Pts',(71.5166647112766,-1.34487131610786,
0.));
#116447=CARTESIAN_POINT('Ctrl Pts',(71.5166647112766,-1.34487131610786,
12.));
#116448=CARTESIAN_POINT('Ctrl Pts',(71.4949685044559,-1.33698065085228,
0.));
#116449=CARTESIAN_POINT('Ctrl Pts',(71.4949685044559,-1.33698065085228,
12.));
#116450=CARTESIAN_POINT('Ctrl Pts',(71.4733063530227,-1.32912680326132,
0.));
#116451=CARTESIAN_POINT('Ctrl Pts',(71.4733063530227,-1.32912680326132,
12.));
#116452=CARTESIAN_POINT('Ctrl Pts',(71.4516784038346,-1.32130975590232,
0.));
#116453=CARTESIAN_POINT('Ctrl Pts',(71.4516784038346,-1.32130975590232,
12.));
#116454=CARTESIAN_POINT('Ctrl Pts',(71.4300848044095,-1.31352949116539,
0.));
#116455=CARTESIAN_POINT('Ctrl Pts',(71.4300848044095,-1.31352949116539,
12.));
#116456=CARTESIAN_POINT('Ctrl Pts',(71.4085257029308,-1.3057859912614,0.));
#116457=CARTESIAN_POINT('Ctrl Pts',(71.4085257029308,-1.3057859912614,12.));
#116458=CARTESIAN_POINT('Ctrl Pts',(71.3870012482474,-1.29807923821414,
0.));
#116459=CARTESIAN_POINT('Ctrl Pts',(71.3870012482474,-1.29807923821414,
12.));
#116460=CARTESIAN_POINT('Ctrl Pts',(71.3655115898801,-1.29040921386061,
0.));
#116461=CARTESIAN_POINT('Ctrl Pts',(71.3655115898801,-1.29040921386061,
12.));
#116462=CARTESIAN_POINT('Ctrl Pts',(71.344056878033,-1.28277589985475,0.));
#116463=CARTESIAN_POINT('Ctrl Pts',(71.344056878033,-1.28277589985475,12.));
#116464=CARTESIAN_POINT('Ctrl Pts',(71.3226372635993,-1.27517927766611,
0.));
#116465=CARTESIAN_POINT('Ctrl Pts',(71.3226372635993,-1.27517927766611,
12.));
#116466=CARTESIAN_POINT('Ctrl Pts',(71.301252898167,-1.26761932857724,0.));
#116467=CARTESIAN_POINT('Ctrl Pts',(71.301252898167,-1.26761932857724,12.));
#116468=CARTESIAN_POINT('Ctrl Pts',(71.2799039340191,-1.26009603367565,
0.));
#116469=CARTESIAN_POINT('Ctrl Pts',(71.2799039340191,-1.26009603367565,
12.));
#116470=CARTESIAN_POINT('Ctrl Pts',(71.2585905241422,-1.25260937385561,
0.));
#116471=CARTESIAN_POINT('Ctrl Pts',(71.2585905241422,-1.25260937385561,
12.));
#116472=CARTESIAN_POINT('Ctrl Pts',(71.2373128222359,-1.24515932982108,
0.));
#116473=CARTESIAN_POINT('Ctrl Pts',(71.2373128222359,-1.24515932982108,
12.));
#116474=CARTESIAN_POINT('Ctrl Pts',(71.2160709827189,-1.23774588208427,
0.));
#116475=CARTESIAN_POINT('Ctrl Pts',(71.2160709827189,-1.23774588208427,
12.));
#116476=CARTESIAN_POINT('Ctrl Pts',(71.1948651607319,-1.23036901096246,
0.));
#116477=CARTESIAN_POINT('Ctrl Pts',(71.1948651607319,-1.23036901096246,
12.));
#116478=CARTESIAN_POINT('Ctrl Pts',(71.1736955121361,-1.22302869657029,
0.));
#116479=CARTESIAN_POINT('Ctrl Pts',(71.1736955121361,-1.22302869657029,
12.));
#116480=CARTESIAN_POINT('Ctrl Pts',(71.1525621935266,-1.21572491882274,
0.));
#116481=CARTESIAN_POINT('Ctrl Pts',(71.1525621935266,-1.21572491882274,
12.));
#116482=CARTESIAN_POINT('Ctrl Pts',(71.1314653622442,-1.20845765743655,
0.));
#116483=CARTESIAN_POINT('Ctrl Pts',(71.1314653622442,-1.20845765743655,
12.));
#116484=CARTESIAN_POINT('Ctrl Pts',(71.1104051763839,-1.20122689192837,
0.));
#116485=CARTESIAN_POINT('Ctrl Pts',(71.1104051763839,-1.20122689192837,
12.));
#116486=CARTESIAN_POINT('Ctrl Pts',(71.089381794801,-1.19403260160998,0.));
#116487=CARTESIAN_POINT('Ctrl Pts',(71.089381794801,-1.19403260160998,12.));
#116488=CARTESIAN_POINT('Ctrl Pts',(71.0683953771147,-1.18687476558127,
0.));
#116489=CARTESIAN_POINT('Ctrl Pts',(71.0683953771147,-1.18687476558127,
12.));
#116490=CARTESIAN_POINT('Ctrl Pts',(71.0474460837157,-1.179753362735,0.));
#116491=CARTESIAN_POINT('Ctrl Pts',(71.0474460837157,-1.179753362735,12.));
#116492=CARTESIAN_POINT('Ctrl Pts',(71.0265340757697,-1.17266837175776,
0.));
#116493=CARTESIAN_POINT('Ctrl Pts',(71.0265340757697,-1.17266837175776,
12.));
#116494=CARTESIAN_POINT('Ctrl Pts',(71.0056595152204,-1.16561977112883,
0.));
#116495=CARTESIAN_POINT('Ctrl Pts',(71.0056595152204,-1.16561977112883,
12.));
#116496=CARTESIAN_POINT('Ctrl Pts',(70.9848225647876,-1.1586075391149,0.));
#116497=CARTESIAN_POINT('Ctrl Pts',(70.9848225647876,-1.1586075391149,12.));
#116498=CARTESIAN_POINT('Ctrl Pts',(70.9640233879671,-1.15163165376531,
0.));
#116499=CARTESIAN_POINT('Ctrl Pts',(70.9640233879671,-1.15163165376531,
12.));
#116500=CARTESIAN_POINT('Ctrl Pts',(70.943262149058,-1.14469209291494,0.));
#116501=CARTESIAN_POINT('Ctrl Pts',(70.943262149058,-1.14469209291494,12.));
#116502=CARTESIAN_POINT('Ctrl Pts',(70.9225390131835,-1.13778883418217,
0.));
#116503=CARTESIAN_POINT('Ctrl Pts',(70.9225390131835,-1.13778883418217,
12.));
#116504=CARTESIAN_POINT('Ctrl Pts',(70.9018541463083,-1.13092185496564,
0.));
#116505=CARTESIAN_POINT('Ctrl Pts',(70.9018541463083,-1.13092185496564,
12.));
#116506=CARTESIAN_POINT('Ctrl Pts',(70.8812077152564,-1.12409113243511,
0.));
#116507=CARTESIAN_POINT('Ctrl Pts',(70.8812077152564,-1.12409113243511,
12.));
#116508=CARTESIAN_POINT('Ctrl Pts',(70.860599887712,-1.11729664352991,0.));
#116509=CARTESIAN_POINT('Ctrl Pts',(70.860599887712,-1.11729664352991,12.));
#116510=CARTESIAN_POINT('Ctrl Pts',(70.8400308322013,-1.11053836496638,
0.));
#116511=CARTESIAN_POINT('Ctrl Pts',(70.8400308322013,-1.11053836496638,
12.));
#116512=CARTESIAN_POINT('Ctrl Pts',(70.8195007180739,-1.10381627323946,
0.));
#116513=CARTESIAN_POINT('Ctrl Pts',(70.8195007180739,-1.10381627323946,
12.));
#116514=CARTESIAN_POINT('Ctrl Pts',(70.7990097154855,-1.0971303446227,0.));
#116515=CARTESIAN_POINT('Ctrl Pts',(70.7990097154855,-1.0971303446227,12.));
#116516=CARTESIAN_POINT('Ctrl Pts',(70.7785579953611,-1.09048055516434,
0.));
#116517=CARTESIAN_POINT('Ctrl Pts',(70.7785579953611,-1.09048055516434,
12.));
#116518=CARTESIAN_POINT('Ctrl Pts',(70.7581457294475,-1.08386688068349,
0.));
#116519=CARTESIAN_POINT('Ctrl Pts',(70.7581457294475,-1.08386688068349,
12.));
#116520=CARTESIAN_POINT('Ctrl Pts',(70.737773090397,-1.07728929676412,0.));
#116521=CARTESIAN_POINT('Ctrl Pts',(70.737773090397,-1.07728929676412,12.));
#116522=CARTESIAN_POINT('Ctrl Pts',(70.7174402518378,-1.07074777874597,
0.));
#116523=CARTESIAN_POINT('Ctrl Pts',(70.7174402518378,-1.07074777874597,
12.));
#116524=CARTESIAN_POINT('Ctrl Pts',(70.6971473884443,-1.0642423017128,0.));
#116525=CARTESIAN_POINT('Ctrl Pts',(70.6971473884443,-1.0642423017128,12.));
#116526=CARTESIAN_POINT('Ctrl Pts',(70.6768946760063,-1.05777284047728,
0.));
#116527=CARTESIAN_POINT('Ctrl Pts',(70.6768946760063,-1.05777284047728,
12.));
#116528=CARTESIAN_POINT('Ctrl Pts',(70.6566822912965,-1.05133936960069,
0.));
#116529=CARTESIAN_POINT('Ctrl Pts',(70.6566822912965,-1.05133936960069,
12.));
#116530=CARTESIAN_POINT('Ctrl Pts',(70.6365104119238,-1.04494186341156,
0.));
#116531=CARTESIAN_POINT('Ctrl Pts',(70.6365104119238,-1.04494186341156,
12.));
#116532=CARTESIAN_POINT('Ctrl Pts',(70.6163792162079,-1.03858029601906,
0.));
#116533=CARTESIAN_POINT('Ctrl Pts',(70.6163792162079,-1.03858029601906,
12.));
#116534=CARTESIAN_POINT('Ctrl Pts',(70.5962888829958,-1.03225464132873,
0.));
#116535=CARTESIAN_POINT('Ctrl Pts',(70.5962888829958,-1.03225464132873,
12.));
#116536=CARTESIAN_POINT('Ctrl Pts',(70.5762395916412,-1.02596487304049,
0.));
#116537=CARTESIAN_POINT('Ctrl Pts',(70.5762395916412,-1.02596487304049,
12.));
#116538=CARTESIAN_POINT('Ctrl Pts',(70.5562315224219,-1.01971096460599,
0.));
#116539=CARTESIAN_POINT('Ctrl Pts',(70.5562315224219,-1.01971096460599,
12.));
#116540=CARTESIAN_POINT('Ctrl Pts',(70.5362648569072,-1.0134928891854,0.));
#116541=CARTESIAN_POINT('Ctrl Pts',(70.5362648569072,-1.0134928891854,12.));
#116542=CARTESIAN_POINT('Ctrl Pts',(70.5163397782699,-1.00731061960968,
0.));
#116543=CARTESIAN_POINT('Ctrl Pts',(70.5163397782699,-1.00731061960968,
12.));
#116544=CARTESIAN_POINT('Ctrl Pts',(70.4964564717917,-1.00116412831438,
0.));
#116545=CARTESIAN_POINT('Ctrl Pts',(70.4964564717917,-1.00116412831438,
12.));
#116546=CARTESIAN_POINT('Ctrl Pts',(70.476615124517,-0.995053387379685,
0.));
#116547=CARTESIAN_POINT('Ctrl Pts',(70.476615124517,-0.995053387379685,
12.));
#116548=CARTESIAN_POINT('Ctrl Pts',(70.4568159243131,-0.988978368643593,
0.));
#116549=CARTESIAN_POINT('Ctrl Pts',(70.4568159243131,-0.988978368643593,
12.));
#116550=CARTESIAN_POINT('Ctrl Pts',(70.4370590590839,-0.982939043792163,
0.));
#116551=CARTESIAN_POINT('Ctrl Pts',(70.4370590590839,-0.982939043792163,
12.));
#116552=CARTESIAN_POINT('Ctrl Pts',(70.41734471596,-0.976935384450131,0.));
#116553=CARTESIAN_POINT('Ctrl Pts',(70.41734471596,-0.976935384450131,12.));
#116554=CARTESIAN_POINT('Ctrl Pts',(70.3976730803664,-0.970967362281305,
0.));
#116555=CARTESIAN_POINT('Ctrl Pts',(70.3976730803664,-0.970967362281305,
12.));
#116556=CARTESIAN_POINT('Ctrl Pts',(70.3780443378003,-0.965034948786564,
0.));
#116557=CARTESIAN_POINT('Ctrl Pts',(70.3780443378003,-0.965034948786564,
12.));
#116558=CARTESIAN_POINT('Ctrl Pts',(70.3584586759561,-0.959138115058888,
0.));
#116559=CARTESIAN_POINT('Ctrl Pts',(70.3584586759561,-0.959138115058888,
12.));
#116560=CARTESIAN_POINT('Ctrl Pts',(70.338916286457,-0.953276831581237,
0.));
#116561=CARTESIAN_POINT('Ctrl Pts',(70.338916286457,-0.953276831581237,
12.));
#116562=CARTESIAN_POINT('Ctrl Pts',(70.3194173673635,-0.947451067929568,
0.));
#116563=CARTESIAN_POINT('Ctrl Pts',(70.3194173673635,-0.947451067929568,
12.));
#116564=CARTESIAN_POINT('Ctrl Pts',(70.2999621233938,-0.941660792742957,
0.));
#116565=CARTESIAN_POINT('Ctrl Pts',(70.2999621233938,-0.941660792742957,
12.));
#116566=CARTESIAN_POINT('Ctrl Pts',(70.2805507606832,-0.935905974336494,
0.));
#116567=CARTESIAN_POINT('Ctrl Pts',(70.2805507606832,-0.935905974336494,
12.));
#116568=CARTESIAN_POINT('Ctrl Pts',(70.2611834821711,-0.93018658123558,
0.));
#116569=CARTESIAN_POINT('Ctrl Pts',(70.2611834821711,-0.93018658123558,
12.));
#116570=CARTESIAN_POINT('Ctrl Pts',(70.241860483586,-0.924502582639455,
0.));
#116571=CARTESIAN_POINT('Ctrl Pts',(70.241860483586,-0.924502582639455,
12.));
#116572=CARTESIAN_POINT('Ctrl Pts',(70.2225819470306,-0.918853949157049,
0.));
#116573=CARTESIAN_POINT('Ctrl Pts',(70.2225819470306,-0.918853949157049,
12.));
#116574=CARTESIAN_POINT('Ctrl Pts',(70.2033480471749,-0.913240652090843,
0.));
#116575=CARTESIAN_POINT('Ctrl Pts',(70.2033480471749,-0.913240652090843,
12.));
#116576=CARTESIAN_POINT('Ctrl Pts',(70.184158963563,-0.907662662015655,
0.));
#116577=CARTESIAN_POINT('Ctrl Pts',(70.184158963563,-0.907662662015655,
12.));
#116578=CARTESIAN_POINT('Ctrl Pts',(70.1650148905109,-0.902119947629777,
0.));
#116579=CARTESIAN_POINT('Ctrl Pts',(70.1650148905109,-0.902119947629777,
12.));
#116580=CARTESIAN_POINT('Ctrl Pts',(70.1459160490366,-0.896612474372089,
0.));
#116581=CARTESIAN_POINT('Ctrl Pts',(70.1459160490366,-0.896612474372089,
12.));
#116582=CARTESIAN_POINT('Ctrl Pts',(70.1268626950031,-0.891140203464729,
0.));
#116583=CARTESIAN_POINT('Ctrl Pts',(70.1268626950031,-0.891140203464729,
12.));
#116584=CARTESIAN_POINT('Ctrl Pts',(70.1078550938801,-0.885703094803091,
0.));
#116585=CARTESIAN_POINT('Ctrl Pts',(70.1078550938801,-0.885703094803091,
12.));
#116586=CARTESIAN_POINT('Ctrl Pts',(70.0888934967772,-0.880301109661041,
0.));
#116587=CARTESIAN_POINT('Ctrl Pts',(70.0888934967772,-0.880301109661041,
12.));
#116588=CARTESIAN_POINT('Ctrl Pts',(70.0699781184013,-0.874934213255575,
0.));
#116589=CARTESIAN_POINT('Ctrl Pts',(70.0699781184013,-0.874934213255575,
12.));
#116590=CARTESIAN_POINT('Ctrl Pts',(70.0511091083285,-0.869602377870143,
0.));
#116591=CARTESIAN_POINT('Ctrl Pts',(70.0511091083285,-0.869602377870143,
12.));
#116592=CARTESIAN_POINT('Ctrl Pts',(70.0322865493339,-0.864305583660094,
0.));
#116593=CARTESIAN_POINT('Ctrl Pts',(70.0322865493339,-0.864305583660094,
12.));
#116594=CARTESIAN_POINT('Ctrl Pts',(70.0172656934192,-0.860096170667403,
0.));
#116595=CARTESIAN_POINT('Ctrl Pts',(70.0172656934192,-0.860096170667403,
12.));
#116596=CARTESIAN_POINT('Ctrl Pts',(70.0060209754332,-0.856954870258375,
0.));
#116597=CARTESIAN_POINT('Ctrl Pts',(70.0060209754332,-0.856954870258375,
12.));
#116598=CARTESIAN_POINT('Ctrl Pts',(69.9985337959499,-0.854867673848295,
0.));
#116599=CARTESIAN_POINT('Ctrl Pts',(69.9985337959499,-0.854867673848295,
12.));
#116600=CARTESIAN_POINT('Ctrl Pts',(69.9947925310006,-0.853825826608997,
0.));
#116601=CARTESIAN_POINT('Ctrl Pts',(69.9947925310006,-0.853825826608997,
12.));
#116602=CARTESIAN_POINT('',(69.9947925310006,-0.853825826608997,12.));
#116603=CARTESIAN_POINT('Ctrl Pts',(69.9947925310006,-0.853825826608997,
12.));
#116604=CARTESIAN_POINT('Ctrl Pts',(69.9985337959499,-0.854867673848295,
12.));
#116605=CARTESIAN_POINT('Ctrl Pts',(70.0060209754332,-0.856954870258375,
12.));
#116606=CARTESIAN_POINT('Ctrl Pts',(70.0172656934192,-0.860096170667403,
12.));
#116607=CARTESIAN_POINT('Ctrl Pts',(70.0322865493339,-0.864305583660094,
12.));
#116608=CARTESIAN_POINT('Ctrl Pts',(70.0511091083285,-0.869602377870143,
12.));
#116609=CARTESIAN_POINT('Ctrl Pts',(70.0699781184013,-0.874934213255575,
12.));
#116610=CARTESIAN_POINT('Ctrl Pts',(70.0888934967772,-0.880301109661041,
12.));
#116611=CARTESIAN_POINT('Ctrl Pts',(70.1078550938801,-0.885703094803091,
12.));
#116612=CARTESIAN_POINT('Ctrl Pts',(70.1268626950031,-0.891140203464729,
12.));
#116613=CARTESIAN_POINT('Ctrl Pts',(70.1459160490366,-0.896612474372089,
12.));
#116614=CARTESIAN_POINT('Ctrl Pts',(70.1650148905109,-0.902119947629777,
12.));
#116615=CARTESIAN_POINT('Ctrl Pts',(70.184158963563,-0.907662662015655,
12.));
#116616=CARTESIAN_POINT('Ctrl Pts',(70.2033480471749,-0.913240652090843,
12.));
#116617=CARTESIAN_POINT('Ctrl Pts',(70.2225819470306,-0.918853949157049,
12.));
#116618=CARTESIAN_POINT('Ctrl Pts',(70.241860483586,-0.924502582639455,
12.));
#116619=CARTESIAN_POINT('Ctrl Pts',(70.2611834821711,-0.93018658123558,
12.));
#116620=CARTESIAN_POINT('Ctrl Pts',(70.2805507606832,-0.935905974336494,
12.));
#116621=CARTESIAN_POINT('Ctrl Pts',(70.2999621233938,-0.941660792742957,
12.));
#116622=CARTESIAN_POINT('Ctrl Pts',(70.3194173673635,-0.947451067929568,
12.));
#116623=CARTESIAN_POINT('Ctrl Pts',(70.338916286457,-0.953276831581237,
12.));
#116624=CARTESIAN_POINT('Ctrl Pts',(70.3584586759561,-0.959138115058888,
12.));
#116625=CARTESIAN_POINT('Ctrl Pts',(70.3780443378003,-0.965034948786564,
12.));
#116626=CARTESIAN_POINT('Ctrl Pts',(70.3976730803664,-0.970967362281305,
12.));
#116627=CARTESIAN_POINT('Ctrl Pts',(70.41734471596,-0.976935384450131,12.));
#116628=CARTESIAN_POINT('Ctrl Pts',(70.4370590590839,-0.982939043792163,
12.));
#116629=CARTESIAN_POINT('Ctrl Pts',(70.4568159243131,-0.988978368643593,
12.));
#116630=CARTESIAN_POINT('Ctrl Pts',(70.476615124517,-0.995053387379685,
12.));
#116631=CARTESIAN_POINT('Ctrl Pts',(70.4964564717917,-1.00116412831438,
12.));
#116632=CARTESIAN_POINT('Ctrl Pts',(70.5163397782699,-1.00731061960968,
12.));
#116633=CARTESIAN_POINT('Ctrl Pts',(70.5362648569072,-1.0134928891854,12.));
#116634=CARTESIAN_POINT('Ctrl Pts',(70.5562315224219,-1.01971096460599,
12.));
#116635=CARTESIAN_POINT('Ctrl Pts',(70.5762395916412,-1.02596487304049,
12.));
#116636=CARTESIAN_POINT('Ctrl Pts',(70.5962888829958,-1.03225464132873,
12.));
#116637=CARTESIAN_POINT('Ctrl Pts',(70.6163792162079,-1.03858029601906,
12.));
#116638=CARTESIAN_POINT('Ctrl Pts',(70.6365104119238,-1.04494186341156,
12.));
#116639=CARTESIAN_POINT('Ctrl Pts',(70.6566822912965,-1.05133936960069,
12.));
#116640=CARTESIAN_POINT('Ctrl Pts',(70.6768946760063,-1.05777284047728,
12.));
#116641=CARTESIAN_POINT('Ctrl Pts',(70.6971473884443,-1.0642423017128,12.));
#116642=CARTESIAN_POINT('Ctrl Pts',(70.7174402518378,-1.07074777874597,
12.));
#116643=CARTESIAN_POINT('Ctrl Pts',(70.737773090397,-1.07728929676412,12.));
#116644=CARTESIAN_POINT('Ctrl Pts',(70.7581457294475,-1.08386688068349,
12.));
#116645=CARTESIAN_POINT('Ctrl Pts',(70.7785579953611,-1.09048055516434,
12.));
#116646=CARTESIAN_POINT('Ctrl Pts',(70.7990097154855,-1.0971303446227,12.));
#116647=CARTESIAN_POINT('Ctrl Pts',(70.8195007180739,-1.10381627323946,
12.));
#116648=CARTESIAN_POINT('Ctrl Pts',(70.8400308322013,-1.11053836496638,
12.));
#116649=CARTESIAN_POINT('Ctrl Pts',(70.860599887712,-1.11729664352991,12.));
#116650=CARTESIAN_POINT('Ctrl Pts',(70.8812077152564,-1.12409113243511,
12.));
#116651=CARTESIAN_POINT('Ctrl Pts',(70.9018541463083,-1.13092185496564,
12.));
#116652=CARTESIAN_POINT('Ctrl Pts',(70.9225390131835,-1.13778883418217,
12.));
#116653=CARTESIAN_POINT('Ctrl Pts',(70.943262149058,-1.14469209291494,12.));
#116654=CARTESIAN_POINT('Ctrl Pts',(70.9640233879671,-1.15163165376531,
12.));
#116655=CARTESIAN_POINT('Ctrl Pts',(70.9848225647876,-1.1586075391149,12.));
#116656=CARTESIAN_POINT('Ctrl Pts',(71.0056595152204,-1.16561977112883,
12.));
#116657=CARTESIAN_POINT('Ctrl Pts',(71.0265340757697,-1.17266837175776,
12.));
#116658=CARTESIAN_POINT('Ctrl Pts',(71.0474460837157,-1.179753362735,12.));
#116659=CARTESIAN_POINT('Ctrl Pts',(71.0683953771147,-1.18687476558127,
12.));
#116660=CARTESIAN_POINT('Ctrl Pts',(71.089381794801,-1.19403260160998,12.));
#116661=CARTESIAN_POINT('Ctrl Pts',(71.1104051763839,-1.20122689192837,
12.));
#116662=CARTESIAN_POINT('Ctrl Pts',(71.1314653622442,-1.20845765743655,
12.));
#116663=CARTESIAN_POINT('Ctrl Pts',(71.1525621935266,-1.21572491882274,
12.));
#116664=CARTESIAN_POINT('Ctrl Pts',(71.1736955121361,-1.22302869657029,
12.));
#116665=CARTESIAN_POINT('Ctrl Pts',(71.1948651607319,-1.23036901096246,
12.));
#116666=CARTESIAN_POINT('Ctrl Pts',(71.2160709827189,-1.23774588208427,
12.));
#116667=CARTESIAN_POINT('Ctrl Pts',(71.2373128222359,-1.24515932982108,
12.));
#116668=CARTESIAN_POINT('Ctrl Pts',(71.2585905241422,-1.25260937385561,
12.));
#116669=CARTESIAN_POINT('Ctrl Pts',(71.2799039340191,-1.26009603367565,
12.));
#116670=CARTESIAN_POINT('Ctrl Pts',(71.301252898167,-1.26761932857724,12.));
#116671=CARTESIAN_POINT('Ctrl Pts',(71.3226372635993,-1.27517927766611,
12.));
#116672=CARTESIAN_POINT('Ctrl Pts',(71.344056878033,-1.28277589985475,12.));
#116673=CARTESIAN_POINT('Ctrl Pts',(71.3655115898801,-1.29040921386061,
12.));
#116674=CARTESIAN_POINT('Ctrl Pts',(71.3870012482474,-1.29807923821414,
12.));
#116675=CARTESIAN_POINT('Ctrl Pts',(71.4085257029308,-1.3057859912614,12.));
#116676=CARTESIAN_POINT('Ctrl Pts',(71.4300848044095,-1.31352949116539,
12.));
#116677=CARTESIAN_POINT('Ctrl Pts',(71.4516784038346,-1.32130975590232,
12.));
#116678=CARTESIAN_POINT('Ctrl Pts',(71.4733063530227,-1.32912680326132,
12.));
#116679=CARTESIAN_POINT('Ctrl Pts',(71.4949685044559,-1.33698065085228,
12.));
#116680=CARTESIAN_POINT('Ctrl Pts',(71.5166647112766,-1.34487131610786,
12.));
#116681=CARTESIAN_POINT('Ctrl Pts',(71.538394827283,-1.35279881628454,12.));
#116682=CARTESIAN_POINT('Ctrl Pts',(71.5601587069175,-1.36076316845807,
12.));
#116683=CARTESIAN_POINT('Ctrl Pts',(71.5819562052613,-1.36876438952449,
12.));
#116684=CARTESIAN_POINT('Ctrl Pts',(71.6037871780347,-1.37680249620763,
12.));
#116685=CARTESIAN_POINT('Ctrl Pts',(71.6256514815918,-1.38487750506076,
12.));
#116686=CARTESIAN_POINT('Ctrl Pts',(71.6475489729149,-1.39298943246732,
12.));
#116687=CARTESIAN_POINT('Ctrl Pts',(71.6694795096034,-1.401138294636,12.));
#116688=CARTESIAN_POINT('Ctrl Pts',(71.6914429498702,-1.40932410760275,
12.));
#116689=CARTESIAN_POINT('Ctrl Pts',(71.7134391525417,-1.41754688723792,
12.));
#116690=CARTESIAN_POINT('Ctrl Pts',(71.7354679770537,-1.42580664924775,
12.));
#116691=CARTESIAN_POINT('Ctrl Pts',(71.7575292834456,-1.4341034091749,12.));
#116692=CARTESIAN_POINT('Ctrl Pts',(71.7796229323496,-1.44243718239305,
12.));
#116693=CARTESIAN_POINT('Ctrl Pts',(71.8017487849865,-1.45080798410957,
12.));
#116694=CARTESIAN_POINT('Ctrl Pts',(71.8239067031664,-1.45921582937229,
12.));
#116695=CARTESIAN_POINT('Ctrl Pts',(71.8460965492836,-1.4676607330709,12.));
#116696=CARTESIAN_POINT('Ctrl Pts',(71.8683181863123,-1.47614270993731,
12.));
#116697=CARTESIAN_POINT('Ctrl Pts',(71.8905714777972,-1.48466177454022,
12.));
#116698=CARTESIAN_POINT('Ctrl Pts',(71.9128562878491,-1.49321794128801,
12.));
#116699=CARTESIAN_POINT('Ctrl Pts',(71.935172481145,-1.50181122443536,12.));
#116700=CARTESIAN_POINT('Ctrl Pts',(71.9575199229241,-1.51044163808455,
12.));
#116701=CARTESIAN_POINT('Ctrl Pts',(71.9798984789828,-1.51910919618567,
12.));
#116702=CARTESIAN_POINT('Ctrl Pts',(72.0023080156647,-1.52781391253104,
12.));
#116703=CARTESIAN_POINT('Ctrl Pts',(72.0247483998582,-1.53655580075814,
12.));
#116704=CARTESIAN_POINT('Ctrl Pts',(72.0472194989968,-1.54533487435627,
12.));
#116705=CARTESIAN_POINT('Ctrl Pts',(72.0697211810548,-1.55415114666774,
12.));
#116706=CARTESIAN_POINT('Ctrl Pts',(72.092253314543,-1.56300463088811,12.));
#116707=CARTESIAN_POINT('Ctrl Pts',(72.1148157684987,-1.57189534006044,
12.));
#116708=CARTESIAN_POINT('Ctrl Pts',(72.1374084124829,-1.58082328707808,
12.));
#116709=CARTESIAN_POINT('Ctrl Pts',(72.1600311165813,-1.58978848469129,
12.));
#116710=CARTESIAN_POINT('Ctrl Pts',(72.1826837514,-1.5987909455085,12.));
#116711=CARTESIAN_POINT('Ctrl Pts',(72.2053661880611,-1.60783068199662,
12.));
#116712=CARTESIAN_POINT('Ctrl Pts',(72.2280782981941,-1.61690770647536,
12.));
#116713=CARTESIAN_POINT('Ctrl Pts',(72.2508199539325,-1.62602203111925,
12.));
#116714=CARTESIAN_POINT('Ctrl Pts',(72.2735910279149,-1.63517366796459,
12.));
#116715=CARTESIAN_POINT('Ctrl Pts',(72.2963913932811,-1.64436262891078,
12.));
#116716=CARTESIAN_POINT('Ctrl Pts',(72.3192209236691,-1.65358892572066,
12.));
#116717=CARTESIAN_POINT('Ctrl Pts',(72.3420794932052,-1.66285257001503,
12.));
#116718=CARTESIAN_POINT('Ctrl Pts',(72.3649669765013,-1.67215357327373,
12.));
#116719=CARTESIAN_POINT('Ctrl Pts',(72.3878832486549,-1.68149194684289,
12.));
#116720=CARTESIAN_POINT('Ctrl Pts',(72.4108281852473,-1.69086770193641,
12.));
#116721=CARTESIAN_POINT('Ctrl Pts',(72.4338016623388,-1.70028084963647,
12.));
#116722=CARTESIAN_POINT('Ctrl Pts',(72.4568035564618,-1.70973140088838,
12.));
#116723=CARTESIAN_POINT('Ctrl Pts',(72.4798337446162,-1.71921936650032,
12.));
#116724=CARTESIAN_POINT('Ctrl Pts',(72.5028921042704,-1.72874475715099,
12.));
#116725=CARTESIAN_POINT('Ctrl Pts',(72.5259785133586,-1.73830758339124,
12.));
#116726=CARTESIAN_POINT('Ctrl Pts',(72.5490928502773,-1.74790785564476,
12.));
#116727=CARTESIAN_POINT('Ctrl Pts',(72.5722349938789,-1.7575455842035,12.));
#116728=CARTESIAN_POINT('Ctrl Pts',(72.5954048234655,-1.7672207792258,12.));
#116729=CARTESIAN_POINT('Ctrl Pts',(72.618602218792,-1.77693345074431,12.));
#116730=CARTESIAN_POINT('Ctrl Pts',(72.6418270600623,-1.78668360866814,
12.));
#116731=CARTESIAN_POINT('Ctrl Pts',(72.6650792279271,-1.79647126278359,
12.));
#116732=CARTESIAN_POINT('Ctrl Pts',(72.6883586034768,-1.80629642275052,
12.));
#116733=CARTESIAN_POINT('Ctrl Pts',(72.7116650682347,-1.81615909809872,
12.));
#116734=CARTESIAN_POINT('Ctrl Pts',(72.73499850416,-1.82605929823566,12.));
#116735=CARTESIAN_POINT('Ctrl Pts',(72.7583587936454,-1.83599703244926,
12.));
#116736=CARTESIAN_POINT('Ctrl Pts',(72.7817458195155,-1.84597230990858,
12.));
#116737=CARTESIAN_POINT('Ctrl Pts',(72.8051594650214,-1.85598513966116,
12.));
#116738=CARTESIAN_POINT('Ctrl Pts',(72.8285996138346,-1.86603553062776,
12.));
#116739=CARTESIAN_POINT('Ctrl Pts',(72.8520661500465,-1.87612349160952,
12.));
#116740=CARTESIAN_POINT('Ctrl Pts',(72.8755589581674,-1.88624903129196,
12.));
#116741=CARTESIAN_POINT('Ctrl Pts',(72.8990779231226,-1.89641215824585,
12.));
#116742=CARTESIAN_POINT('Ctrl Pts',(72.9226229302483,-1.90661288092583,
12.));
#116743=CARTESIAN_POINT('Ctrl Pts',(72.9461938652816,-1.91685120766428,
12.));
#116744=CARTESIAN_POINT('Ctrl Pts',(72.9697906143638,-1.92712714667649,
12.));
#116745=CARTESIAN_POINT('Ctrl Pts',(72.9934130640414,-1.93744070606557,
12.));
#116746=CARTESIAN_POINT('Ctrl Pts',(73.0170611012659,-1.94779189382301,
12.));
#116747=CARTESIAN_POINT('Ctrl Pts',(73.0407346133912,-1.95818071782774,
12.));
#116748=CARTESIAN_POINT('Ctrl Pts',(73.0644334881679,-1.96860718583945,
12.));
#116749=CARTESIAN_POINT('Ctrl Pts',(73.0881576137415,-1.97907130550172,
12.));
#116750=CARTESIAN_POINT('Ctrl Pts',(73.1119068786482,-1.9895730843493,12.));
#116751=CARTESIAN_POINT('Ctrl Pts',(73.1356811718094,-2.00011252980988,
12.));
#116752=CARTESIAN_POINT('Ctrl Pts',(73.159480382525,-2.01068964920465,12.));
#116753=CARTESIAN_POINT('Ctrl Pts',(73.1833044004612,-2.02130444974352,
12.));
#116754=CARTESIAN_POINT('Ctrl Pts',(73.2071531156492,-2.03195693852441,
12.));
#116755=CARTESIAN_POINT('Ctrl Pts',(73.2310264184965,-2.04264712253915,
12.));
#116756=CARTESIAN_POINT('Ctrl Pts',(73.2549241997946,-2.05337500867396,
12.));
#116757=CARTESIAN_POINT('Ctrl Pts',(73.2788463507248,-2.06414060370838,
12.));
#116758=CARTESIAN_POINT('Ctrl Pts',(73.3027927628636,-2.07494391430954,
12.));
#116759=CARTESIAN_POINT('Ctrl Pts',(73.3267633281822,-2.08578494702762,
12.));
#116760=CARTESIAN_POINT('Ctrl Pts',(73.3507579390254,-2.09666370830733,
12.));
#116761=CARTESIAN_POINT('Ctrl Pts',(73.3747764880903,-2.10758020449401,
12.));
#116762=CARTESIAN_POINT('Ctrl Pts',(73.3988188684022,-2.11853444183764,
12.));
#116763=CARTESIAN_POINT('Ctrl Pts',(73.4228849732914,-2.12952642649361,
12.));
#116764=CARTESIAN_POINT('Ctrl Pts',(73.4469746963622,-2.14055616452049,
12.));
#116765=CARTESIAN_POINT('Ctrl Pts',(73.4710879315367,-2.15162366187899,
12.));
#116766=CARTESIAN_POINT('Ctrl Pts',(73.4952245731044,-2.16272892442916,
12.));
#116767=CARTESIAN_POINT('Ctrl Pts',(73.5193845157705,-2.17387195792306,
12.));
#116768=CARTESIAN_POINT('Ctrl Pts',(73.5435676546934,-2.18505276799757,
12.));
#116769=CARTESIAN_POINT('Ctrl Pts',(73.5677738855461,-2.19627136015683,
12.));
#116770=CARTESIAN_POINT('Ctrl Pts',(73.5920031044604,-2.20752773978353,
12.));
#116771=CARTESIAN_POINT('Ctrl Pts',(73.6162552079044,-2.21882191216521,
12.));
#116772=CARTESIAN_POINT('Ctrl Pts',(73.6405300925714,-2.23015388251289,
12.));
#116773=CARTESIAN_POINT('Ctrl Pts',(73.6648276552766,-2.24152365597699,
12.));
#116774=CARTESIAN_POINT('Ctrl Pts',(73.6891477928124,-2.25293123766425,
12.));
#116775=CARTESIAN_POINT('Ctrl Pts',(73.7134904019378,-2.26437663263664,
12.));
#116776=CARTESIAN_POINT('Ctrl Pts',(73.7378553796792,-2.27585984587193,
12.));
#116777=CARTESIAN_POINT('Ctrl Pts',(73.7622426235648,-2.28738088222859,
12.));
#116778=CARTESIAN_POINT('Ctrl Pts',(73.7866520318849,-2.29893974640435,
12.));
#116779=CARTESIAN_POINT('Ctrl Pts',(73.8110835039341,-2.31053644289425,
12.));
#116780=CARTESIAN_POINT('Ctrl Pts',(73.8355369402733,-2.32217097594216,
12.));
#116781=CARTESIAN_POINT('Ctrl Pts',(73.8600122421502,-2.33384334963981,
12.));
#116782=CARTESIAN_POINT('Ctrl Pts',(73.8845093109302,-2.3455535680214,12.));
#116783=CARTESIAN_POINT('Ctrl Pts',(73.9090280474723,-2.35730163516324,
12.));
#116784=CARTESIAN_POINT('Ctrl Pts',(73.9335683516388,-2.36908755525994,
12.));
#116785=CARTESIAN_POINT('Ctrl Pts',(73.9581301214609,-2.38091133274933,
12.));
#116786=CARTESIAN_POINT('Ctrl Pts',(73.9827132538149,-2.39277297220716,
12.));
#116787=CARTESIAN_POINT('Ctrl Pts',(74.0073176459287,-2.40467247811497,
12.));
#116788=CARTESIAN_POINT('Ctrl Pts',(74.0319431966956,-2.41660985465228,
12.));
#116789=CARTESIAN_POINT('Ctrl Pts',(74.0565898079227,-2.42858510549787,
12.));
#116790=CARTESIAN_POINT('Ctrl Pts',(74.0812573859474,-2.44059823356722,
12.));
#116791=CARTESIAN_POINT('Ctrl Pts',(74.1059458420175,-2.45264924094853,
12.));
#116792=CARTESIAN_POINT('Ctrl Pts',(74.1271264545378,-2.46301176097528,
12.));
#116793=CARTESIAN_POINT('Ctrl Pts',(74.1433763941622,-2.47097695565718,
12.));
#116794=CARTESIAN_POINT('Ctrl Pts',(74.1546864735453,-2.47652804725573,
12.));
#116795=CARTESIAN_POINT('Ctrl Pts',(74.1610506466543,-2.47965393946825,
12.));
#116796=CARTESIAN_POINT('Ctrl Pts',(74.1624659714955,-2.48034921844901,
12.));
#116797=CARTESIAN_POINT('',(69.9947925310006,-0.853825826608997,0.));
#116798=CARTESIAN_POINT('',(69.9947925310006,-0.853825826608997,0.));
#116799=CARTESIAN_POINT('Ctrl Pts',(74.1624659714955,-2.48034921844903,
0.));
#116800=CARTESIAN_POINT('Ctrl Pts',(74.1610506466543,-2.47965393946827,
0.));
#116801=CARTESIAN_POINT('Ctrl Pts',(74.1546864735453,-2.47652804725574,
0.));
#116802=CARTESIAN_POINT('Ctrl Pts',(74.1433763941622,-2.47097695565719,
0.));
#116803=CARTESIAN_POINT('Ctrl Pts',(74.1271264545378,-2.46301176097528,
0.));
#116804=CARTESIAN_POINT('Ctrl Pts',(74.1059458420175,-2.45264924094853,
0.));
#116805=CARTESIAN_POINT('Ctrl Pts',(74.0812573859474,-2.44059823356722,
0.));
#116806=CARTESIAN_POINT('Ctrl Pts',(74.0565898079227,-2.42858510549787,
0.));
#116807=CARTESIAN_POINT('Ctrl Pts',(74.0319431966956,-2.41660985465228,
0.));
#116808=CARTESIAN_POINT('Ctrl Pts',(74.0073176459287,-2.40467247811497,
0.));
#116809=CARTESIAN_POINT('Ctrl Pts',(73.9827132538149,-2.39277297220716,
0.));
#116810=CARTESIAN_POINT('Ctrl Pts',(73.9581301214609,-2.38091133274933,
0.));
#116811=CARTESIAN_POINT('Ctrl Pts',(73.9335683516388,-2.36908755525994,
0.));
#116812=CARTESIAN_POINT('Ctrl Pts',(73.9090280474723,-2.35730163516324,
0.));
#116813=CARTESIAN_POINT('Ctrl Pts',(73.8845093109302,-2.3455535680214,0.));
#116814=CARTESIAN_POINT('Ctrl Pts',(73.8600122421502,-2.33384334963981,
0.));
#116815=CARTESIAN_POINT('Ctrl Pts',(73.8355369402733,-2.32217097594216,
0.));
#116816=CARTESIAN_POINT('Ctrl Pts',(73.8110835039341,-2.31053644289425,
0.));
#116817=CARTESIAN_POINT('Ctrl Pts',(73.7866520318849,-2.29893974640435,
0.));
#116818=CARTESIAN_POINT('Ctrl Pts',(73.7622426235648,-2.28738088222859,
0.));
#116819=CARTESIAN_POINT('Ctrl Pts',(73.7378553796792,-2.27585984587193,
0.));
#116820=CARTESIAN_POINT('Ctrl Pts',(73.7134904019378,-2.26437663263664,
0.));
#116821=CARTESIAN_POINT('Ctrl Pts',(73.6891477928124,-2.25293123766425,
0.));
#116822=CARTESIAN_POINT('Ctrl Pts',(73.6648276552766,-2.24152365597699,
0.));
#116823=CARTESIAN_POINT('Ctrl Pts',(73.6405300925714,-2.23015388251289,
0.));
#116824=CARTESIAN_POINT('Ctrl Pts',(73.6162552079044,-2.21882191216521,
0.));
#116825=CARTESIAN_POINT('Ctrl Pts',(73.5920031044604,-2.20752773978353,
0.));
#116826=CARTESIAN_POINT('Ctrl Pts',(73.5677738855461,-2.19627136015683,
0.));
#116827=CARTESIAN_POINT('Ctrl Pts',(73.5435676546934,-2.18505276799757,
0.));
#116828=CARTESIAN_POINT('Ctrl Pts',(73.5193845157705,-2.17387195792306,
0.));
#116829=CARTESIAN_POINT('Ctrl Pts',(73.4952245731044,-2.16272892442916,
0.));
#116830=CARTESIAN_POINT('Ctrl Pts',(73.4710879315367,-2.15162366187899,
0.));
#116831=CARTESIAN_POINT('Ctrl Pts',(73.4469746963622,-2.14055616452049,
0.));
#116832=CARTESIAN_POINT('Ctrl Pts',(73.4228849732914,-2.12952642649361,
0.));
#116833=CARTESIAN_POINT('Ctrl Pts',(73.3988188684022,-2.11853444183764,
0.));
#116834=CARTESIAN_POINT('Ctrl Pts',(73.3747764880903,-2.10758020449401,
0.));
#116835=CARTESIAN_POINT('Ctrl Pts',(73.3507579390254,-2.09666370830733,
0.));
#116836=CARTESIAN_POINT('Ctrl Pts',(73.3267633281822,-2.08578494702762,
0.));
#116837=CARTESIAN_POINT('Ctrl Pts',(73.3027927628636,-2.07494391430954,
0.));
#116838=CARTESIAN_POINT('Ctrl Pts',(73.2788463507248,-2.06414060370838,
0.));
#116839=CARTESIAN_POINT('Ctrl Pts',(73.2549241997946,-2.05337500867396,
0.));
#116840=CARTESIAN_POINT('Ctrl Pts',(73.2310264184965,-2.04264712253915,
0.));
#116841=CARTESIAN_POINT('Ctrl Pts',(73.2071531156492,-2.03195693852441,
0.));
#116842=CARTESIAN_POINT('Ctrl Pts',(73.1833044004612,-2.02130444974352,
0.));
#116843=CARTESIAN_POINT('Ctrl Pts',(73.159480382525,-2.01068964920465,0.));
#116844=CARTESIAN_POINT('Ctrl Pts',(73.1356811718094,-2.00011252980988,
0.));
#116845=CARTESIAN_POINT('Ctrl Pts',(73.1119068786482,-1.9895730843493,0.));
#116846=CARTESIAN_POINT('Ctrl Pts',(73.0881576137415,-1.97907130550172,
0.));
#116847=CARTESIAN_POINT('Ctrl Pts',(73.0644334881679,-1.96860718583945,
0.));
#116848=CARTESIAN_POINT('Ctrl Pts',(73.0407346133912,-1.95818071782774,
0.));
#116849=CARTESIAN_POINT('Ctrl Pts',(73.0170611012659,-1.94779189382301,
0.));
#116850=CARTESIAN_POINT('Ctrl Pts',(72.9934130640414,-1.93744070606557,
0.));
#116851=CARTESIAN_POINT('Ctrl Pts',(72.9697906143638,-1.92712714667649,
0.));
#116852=CARTESIAN_POINT('Ctrl Pts',(72.9461938652816,-1.91685120766428,
0.));
#116853=CARTESIAN_POINT('Ctrl Pts',(72.9226229302483,-1.90661288092583,
0.));
#116854=CARTESIAN_POINT('Ctrl Pts',(72.8990779231226,-1.89641215824585,
0.));
#116855=CARTESIAN_POINT('Ctrl Pts',(72.8755589581674,-1.88624903129196,
0.));
#116856=CARTESIAN_POINT('Ctrl Pts',(72.8520661500465,-1.87612349160952,
0.));
#116857=CARTESIAN_POINT('Ctrl Pts',(72.8285996138346,-1.86603553062776,
0.));
#116858=CARTESIAN_POINT('Ctrl Pts',(72.8051594650214,-1.85598513966116,
0.));
#116859=CARTESIAN_POINT('Ctrl Pts',(72.7817458195155,-1.84597230990858,
0.));
#116860=CARTESIAN_POINT('Ctrl Pts',(72.7583587936454,-1.83599703244926,
0.));
#116861=CARTESIAN_POINT('Ctrl Pts',(72.73499850416,-1.82605929823566,0.));
#116862=CARTESIAN_POINT('Ctrl Pts',(72.7116650682347,-1.81615909809872,
0.));
#116863=CARTESIAN_POINT('Ctrl Pts',(72.6883586034768,-1.80629642275052,
0.));
#116864=CARTESIAN_POINT('Ctrl Pts',(72.6650792279271,-1.79647126278359,
0.));
#116865=CARTESIAN_POINT('Ctrl Pts',(72.6418270600623,-1.78668360866814,
0.));
#116866=CARTESIAN_POINT('Ctrl Pts',(72.618602218792,-1.77693345074431,0.));
#116867=CARTESIAN_POINT('Ctrl Pts',(72.5954048234655,-1.7672207792258,0.));
#116868=CARTESIAN_POINT('Ctrl Pts',(72.5722349938789,-1.7575455842035,0.));
#116869=CARTESIAN_POINT('Ctrl Pts',(72.5490928502773,-1.74790785564476,
0.));
#116870=CARTESIAN_POINT('Ctrl Pts',(72.5259785133586,-1.73830758339124,
0.));
#116871=CARTESIAN_POINT('Ctrl Pts',(72.5028921042704,-1.72874475715099,
0.));
#116872=CARTESIAN_POINT('Ctrl Pts',(72.4798337446162,-1.71921936650032,
0.));
#116873=CARTESIAN_POINT('Ctrl Pts',(72.4568035564618,-1.70973140088838,
0.));
#116874=CARTESIAN_POINT('Ctrl Pts',(72.4338016623388,-1.70028084963647,
0.));
#116875=CARTESIAN_POINT('Ctrl Pts',(72.4108281852473,-1.69086770193641,
0.));
#116876=CARTESIAN_POINT('Ctrl Pts',(72.3878832486549,-1.68149194684289,
0.));
#116877=CARTESIAN_POINT('Ctrl Pts',(72.3649669765013,-1.67215357327373,
0.));
#116878=CARTESIAN_POINT('Ctrl Pts',(72.3420794932052,-1.66285257001503,
0.));
#116879=CARTESIAN_POINT('Ctrl Pts',(72.3192209236691,-1.65358892572066,
0.));
#116880=CARTESIAN_POINT('Ctrl Pts',(72.2963913932811,-1.64436262891078,
0.));
#116881=CARTESIAN_POINT('Ctrl Pts',(72.2735910279149,-1.63517366796459,
0.));
#116882=CARTESIAN_POINT('Ctrl Pts',(72.2508199539325,-1.62602203111925,
0.));
#116883=CARTESIAN_POINT('Ctrl Pts',(72.2280782981941,-1.61690770647536,
0.));
#116884=CARTESIAN_POINT('Ctrl Pts',(72.2053661880611,-1.60783068199662,
0.));
#116885=CARTESIAN_POINT('Ctrl Pts',(72.1826837514,-1.5987909455085,0.));
#116886=CARTESIAN_POINT('Ctrl Pts',(72.1600311165813,-1.58978848469129,
0.));
#116887=CARTESIAN_POINT('Ctrl Pts',(72.1374084124829,-1.58082328707808,
0.));
#116888=CARTESIAN_POINT('Ctrl Pts',(72.1148157684987,-1.57189534006044,
0.));
#116889=CARTESIAN_POINT('Ctrl Pts',(72.092253314543,-1.56300463088811,0.));
#116890=CARTESIAN_POINT('Ctrl Pts',(72.0697211810548,-1.55415114666774,
0.));
#116891=CARTESIAN_POINT('Ctrl Pts',(72.0472194989968,-1.54533487435627,
0.));
#116892=CARTESIAN_POINT('Ctrl Pts',(72.0247483998582,-1.53655580075814,
0.));
#116893=CARTESIAN_POINT('Ctrl Pts',(72.0023080156647,-1.52781391253104,
0.));
#116894=CARTESIAN_POINT('Ctrl Pts',(71.9798984789828,-1.51910919618567,
0.));
#116895=CARTESIAN_POINT('Ctrl Pts',(71.9575199229241,-1.51044163808455,
0.));
#116896=CARTESIAN_POINT('Ctrl Pts',(71.935172481145,-1.50181122443536,0.));
#116897=CARTESIAN_POINT('Ctrl Pts',(71.9128562878491,-1.49321794128801,
0.));
#116898=CARTESIAN_POINT('Ctrl Pts',(71.8905714777972,-1.48466177454022,
0.));
#116899=CARTESIAN_POINT('Ctrl Pts',(71.8683181863123,-1.47614270993731,
0.));
#116900=CARTESIAN_POINT('Ctrl Pts',(71.8460965492836,-1.4676607330709,0.));
#116901=CARTESIAN_POINT('Ctrl Pts',(71.8239067031664,-1.45921582937229,
0.));
#116902=CARTESIAN_POINT('Ctrl Pts',(71.8017487849865,-1.45080798410957,
0.));
#116903=CARTESIAN_POINT('Ctrl Pts',(71.7796229323496,-1.44243718239305,
0.));
#116904=CARTESIAN_POINT('Ctrl Pts',(71.7575292834456,-1.4341034091749,0.));
#116905=CARTESIAN_POINT('Ctrl Pts',(71.7354679770537,-1.42580664924775,
0.));
#116906=CARTESIAN_POINT('Ctrl Pts',(71.7134391525417,-1.41754688723792,
0.));
#116907=CARTESIAN_POINT('Ctrl Pts',(71.6914429498702,-1.40932410760275,
0.));
#116908=CARTESIAN_POINT('Ctrl Pts',(71.6694795096034,-1.401138294636,0.));
#116909=CARTESIAN_POINT('Ctrl Pts',(71.6475489729149,-1.39298943246732,
0.));
#116910=CARTESIAN_POINT('Ctrl Pts',(71.6256514815918,-1.38487750506076,
0.));
#116911=CARTESIAN_POINT('Ctrl Pts',(71.6037871780347,-1.37680249620763,
0.));
#116912=CARTESIAN_POINT('Ctrl Pts',(71.5819562052613,-1.36876438952449,
0.));
#116913=CARTESIAN_POINT('Ctrl Pts',(71.5601587069175,-1.36076316845807,
0.));
#116914=CARTESIAN_POINT('Ctrl Pts',(71.538394827283,-1.35279881628454,0.));
#116915=CARTESIAN_POINT('Ctrl Pts',(71.5166647112766,-1.34487131610786,
0.));
#116916=CARTESIAN_POINT('Ctrl Pts',(71.4949685044559,-1.33698065085228,
0.));
#116917=CARTESIAN_POINT('Ctrl Pts',(71.4733063530227,-1.32912680326132,
0.));
#116918=CARTESIAN_POINT('Ctrl Pts',(71.4516784038346,-1.32130975590232,
0.));
#116919=CARTESIAN_POINT('Ctrl Pts',(71.4300848044095,-1.31352949116539,
0.));
#116920=CARTESIAN_POINT('Ctrl Pts',(71.4085257029308,-1.3057859912614,0.));
#116921=CARTESIAN_POINT('Ctrl Pts',(71.3870012482474,-1.29807923821414,
0.));
#116922=CARTESIAN_POINT('Ctrl Pts',(71.3655115898801,-1.29040921386061,
0.));
#116923=CARTESIAN_POINT('Ctrl Pts',(71.344056878033,-1.28277589985475,0.));
#116924=CARTESIAN_POINT('Ctrl Pts',(71.3226372635993,-1.27517927766611,
0.));
#116925=CARTESIAN_POINT('Ctrl Pts',(71.301252898167,-1.26761932857724,0.));
#116926=CARTESIAN_POINT('Ctrl Pts',(71.2799039340191,-1.26009603367565,
0.));
#116927=CARTESIAN_POINT('Ctrl Pts',(71.2585905241422,-1.25260937385561,
0.));
#116928=CARTESIAN_POINT('Ctrl Pts',(71.2373128222359,-1.24515932982108,
0.));
#116929=CARTESIAN_POINT('Ctrl Pts',(71.2160709827189,-1.23774588208427,
0.));
#116930=CARTESIAN_POINT('Ctrl Pts',(71.1948651607319,-1.23036901096246,
0.));
#116931=CARTESIAN_POINT('Ctrl Pts',(71.1736955121361,-1.22302869657029,
0.));
#116932=CARTESIAN_POINT('Ctrl Pts',(71.1525621935266,-1.21572491882274,
0.));
#116933=CARTESIAN_POINT('Ctrl Pts',(71.1314653622442,-1.20845765743655,
0.));
#116934=CARTESIAN_POINT('Ctrl Pts',(71.1104051763839,-1.20122689192837,
0.));
#116935=CARTESIAN_POINT('Ctrl Pts',(71.089381794801,-1.19403260160998,0.));
#116936=CARTESIAN_POINT('Ctrl Pts',(71.0683953771147,-1.18687476558127,
0.));
#116937=CARTESIAN_POINT('Ctrl Pts',(71.0474460837157,-1.179753362735,0.));
#116938=CARTESIAN_POINT('Ctrl Pts',(71.0265340757697,-1.17266837175776,
0.));
#116939=CARTESIAN_POINT('Ctrl Pts',(71.0056595152204,-1.16561977112883,
0.));
#116940=CARTESIAN_POINT('Ctrl Pts',(70.9848225647876,-1.1586075391149,0.));
#116941=CARTESIAN_POINT('Ctrl Pts',(70.9640233879671,-1.15163165376531,
0.));
#116942=CARTESIAN_POINT('Ctrl Pts',(70.943262149058,-1.14469209291494,0.));
#116943=CARTESIAN_POINT('Ctrl Pts',(70.9225390131835,-1.13778883418217,
0.));
#116944=CARTESIAN_POINT('Ctrl Pts',(70.9018541463083,-1.13092185496564,
0.));
#116945=CARTESIAN_POINT('Ctrl Pts',(70.8812077152564,-1.12409113243511,
0.));
#116946=CARTESIAN_POINT('Ctrl Pts',(70.860599887712,-1.11729664352991,0.));
#116947=CARTESIAN_POINT('Ctrl Pts',(70.8400308322013,-1.11053836496638,
0.));
#116948=CARTESIAN_POINT('Ctrl Pts',(70.8195007180739,-1.10381627323946,
0.));
#116949=CARTESIAN_POINT('Ctrl Pts',(70.7990097154855,-1.0971303446227,0.));
#116950=CARTESIAN_POINT('Ctrl Pts',(70.7785579953611,-1.09048055516434,
0.));
#116951=CARTESIAN_POINT('Ctrl Pts',(70.7581457294475,-1.08386688068349,
0.));
#116952=CARTESIAN_POINT('Ctrl Pts',(70.737773090397,-1.07728929676412,0.));
#116953=CARTESIAN_POINT('Ctrl Pts',(70.7174402518378,-1.07074777874597,
0.));
#116954=CARTESIAN_POINT('Ctrl Pts',(70.6971473884443,-1.0642423017128,0.));
#116955=CARTESIAN_POINT('Ctrl Pts',(70.6768946760063,-1.05777284047728,
0.));
#116956=CARTESIAN_POINT('Ctrl Pts',(70.6566822912965,-1.05133936960069,
0.));
#116957=CARTESIAN_POINT('Ctrl Pts',(70.6365104119238,-1.04494186341156,
0.));
#116958=CARTESIAN_POINT('Ctrl Pts',(70.6163792162079,-1.03858029601906,
0.));
#116959=CARTESIAN_POINT('Ctrl Pts',(70.5962888829958,-1.03225464132873,
0.));
#116960=CARTESIAN_POINT('Ctrl Pts',(70.5762395916412,-1.02596487304049,
0.));
#116961=CARTESIAN_POINT('Ctrl Pts',(70.5562315224219,-1.01971096460599,
0.));
#116962=CARTESIAN_POINT('Ctrl Pts',(70.5362648569072,-1.0134928891854,0.));
#116963=CARTESIAN_POINT('Ctrl Pts',(70.5163397782699,-1.00731061960968,
0.));
#116964=CARTESIAN_POINT('Ctrl Pts',(70.4964564717917,-1.00116412831438,
0.));
#116965=CARTESIAN_POINT('Ctrl Pts',(70.476615124517,-0.995053387379685,
0.));
#116966=CARTESIAN_POINT('Ctrl Pts',(70.4568159243131,-0.988978368643593,
0.));
#116967=CARTESIAN_POINT('Ctrl Pts',(70.4370590590839,-0.982939043792163,
0.));
#116968=CARTESIAN_POINT('Ctrl Pts',(70.41734471596,-0.976935384450131,0.));
#116969=CARTESIAN_POINT('Ctrl Pts',(70.3976730803664,-0.970967362281305,
0.));
#116970=CARTESIAN_POINT('Ctrl Pts',(70.3780443378003,-0.965034948786564,
0.));
#116971=CARTESIAN_POINT('Ctrl Pts',(70.3584586759561,-0.959138115058888,
0.));
#116972=CARTESIAN_POINT('Ctrl Pts',(70.338916286457,-0.953276831581237,
0.));
#116973=CARTESIAN_POINT('Ctrl Pts',(70.3194173673635,-0.947451067929568,
0.));
#116974=CARTESIAN_POINT('Ctrl Pts',(70.2999621233938,-0.941660792742957,
0.));
#116975=CARTESIAN_POINT('Ctrl Pts',(70.2805507606832,-0.935905974336494,
0.));
#116976=CARTESIAN_POINT('Ctrl Pts',(70.2611834821711,-0.93018658123558,
0.));
#116977=CARTESIAN_POINT('Ctrl Pts',(70.241860483586,-0.924502582639455,
0.));
#116978=CARTESIAN_POINT('Ctrl Pts',(70.2225819470306,-0.918853949157049,
0.));
#116979=CARTESIAN_POINT('Ctrl Pts',(70.2033480471749,-0.913240652090843,
0.));
#116980=CARTESIAN_POINT('Ctrl Pts',(70.184158963563,-0.907662662015655,
0.));
#116981=CARTESIAN_POINT('Ctrl Pts',(70.1650148905109,-0.902119947629777,
0.));
#116982=CARTESIAN_POINT('Ctrl Pts',(70.1459160490366,-0.896612474372089,
0.));
#116983=CARTESIAN_POINT('Ctrl Pts',(70.1268626950031,-0.891140203464729,
0.));
#116984=CARTESIAN_POINT('Ctrl Pts',(70.1078550938801,-0.885703094803091,
0.));
#116985=CARTESIAN_POINT('Ctrl Pts',(70.0888934967772,-0.880301109661041,
0.));
#116986=CARTESIAN_POINT('Ctrl Pts',(70.0699781184013,-0.874934213255575,
0.));
#116987=CARTESIAN_POINT('Ctrl Pts',(70.0511091083285,-0.869602377870143,
0.));
#116988=CARTESIAN_POINT('Ctrl Pts',(70.0322865493339,-0.864305583660094,
0.));
#116989=CARTESIAN_POINT('Ctrl Pts',(70.0172656934192,-0.860096170667403,
0.));
#116990=CARTESIAN_POINT('Ctrl Pts',(70.0060209754332,-0.856954870258375,
0.));
#116991=CARTESIAN_POINT('Ctrl Pts',(69.9985337959499,-0.854867673848295,
0.));
#116992=CARTESIAN_POINT('Ctrl Pts',(69.9947925310006,-0.853825826608997,
0.));
#116993=CARTESIAN_POINT('Ctrl Pts',(73.9415940197274,-9.10443154852689,
0.));
#116994=CARTESIAN_POINT('Ctrl Pts',(73.9415940197274,-9.10443154852689,
12.));
#116995=CARTESIAN_POINT('Ctrl Pts',(73.9368365074299,-9.10148558516537,
0.));
#116996=CARTESIAN_POINT('Ctrl Pts',(73.9368365074299,-9.10148558516537,
12.));
#116997=CARTESIAN_POINT('Ctrl Pts',(73.9273231219835,-9.09559760529042,
0.));
#116998=CARTESIAN_POINT('Ctrl Pts',(73.9273231219835,-9.09559760529042,
12.));
#116999=CARTESIAN_POINT('Ctrl Pts',(73.9130579612604,-9.08677747602206,
0.));
#117000=CARTESIAN_POINT('Ctrl Pts',(73.9130579612604,-9.08677747602206,
12.));
#117001=CARTESIAN_POINT('Ctrl Pts',(73.8940475822492,-9.07504098571707,
0.));
#117002=CARTESIAN_POINT('Ctrl Pts',(73.8940475822492,-9.07504098571707,
12.));
#117003=CARTESIAN_POINT('Ctrl Pts',(73.8703010078091,-9.06040984890246,
0.));
#117004=CARTESIAN_POINT('Ctrl Pts',(73.8703010078091,-9.06040984890246,
12.));
#117005=CARTESIAN_POINT('Ctrl Pts',(73.8465708501057,-9.04581819646985,
0.));
#117006=CARTESIAN_POINT('Ctrl Pts',(73.8465708501057,-9.04581819646985,
12.));
#117007=CARTESIAN_POINT('Ctrl Pts',(73.8228571411697,-9.03126603778126,
0.));
#117008=CARTESIAN_POINT('Ctrl Pts',(73.8228571411697,-9.03126603778126,
12.));
#117009=CARTESIAN_POINT('Ctrl Pts',(73.7991599312592,-9.01675338208004,
0.));
#117010=CARTESIAN_POINT('Ctrl Pts',(73.7991599312592,-9.01675338208004,
12.));
#117011=CARTESIAN_POINT('Ctrl Pts',(73.7754792943665,-9.00228023701055,
0.));
#117012=CARTESIAN_POINT('Ctrl Pts',(73.7754792943665,-9.00228023701055,
12.));
#117013=CARTESIAN_POINT('Ctrl Pts',(73.7518153261981,-8.98784660837398,
0.));
#117014=CARTESIAN_POINT('Ctrl Pts',(73.7518153261981,-8.98784660837398,
12.));
#117015=CARTESIAN_POINT('Ctrl Pts',(73.728168136383,-8.97345250083601,0.));
#117016=CARTESIAN_POINT('Ctrl Pts',(73.728168136383,-8.97345250083601,12.));
#117017=CARTESIAN_POINT('Ctrl Pts',(73.7045378422686,-8.95909791836153,
0.));
#117018=CARTESIAN_POINT('Ctrl Pts',(73.7045378422686,-8.95909791836153,
12.));
#117019=CARTESIAN_POINT('Ctrl Pts',(73.6809245622383,-8.94478286474419,
0.));
#117020=CARTESIAN_POINT('Ctrl Pts',(73.6809245622383,-8.94478286474419,
12.));
#117021=CARTESIAN_POINT('Ctrl Pts',(73.6573284088184,-8.93050734412124,
0.));
#117022=CARTESIAN_POINT('Ctrl Pts',(73.6573284088184,-8.93050734412124,
12.));
#117023=CARTESIAN_POINT('Ctrl Pts',(73.633749483097,-8.91627136140084,0.));
#117024=CARTESIAN_POINT('Ctrl Pts',(73.633749483097,-8.91627136140084,12.));
#117025=CARTESIAN_POINT('Ctrl Pts',(73.6101878785976,-8.90207492199043,
0.));
#117026=CARTESIAN_POINT('Ctrl Pts',(73.6101878785976,-8.90207492199043,
12.));
#117027=CARTESIAN_POINT('Ctrl Pts',(73.5866436840556,-8.88791803160442,
0.));
#117028=CARTESIAN_POINT('Ctrl Pts',(73.5866436840556,-8.88791803160442,
12.));
#117029=CARTESIAN_POINT('Ctrl Pts',(73.5631169867122,-8.8738006960297,0.));
#117030=CARTESIAN_POINT('Ctrl Pts',(73.5631169867122,-8.8738006960297,12.));
#117031=CARTESIAN_POINT('Ctrl Pts',(73.5396078751639,-8.8597229209213,0.));
#117032=CARTESIAN_POINT('Ctrl Pts',(73.5396078751639,-8.8597229209213,12.));
#117033=CARTESIAN_POINT('Ctrl Pts',(73.5161164429709,-8.84568471153805,
0.));
#117034=CARTESIAN_POINT('Ctrl Pts',(73.5161164429709,-8.84568471153805,
12.));
#117035=CARTESIAN_POINT('Ctrl Pts',(73.492642788273,-8.83168607277325,0.));
#117036=CARTESIAN_POINT('Ctrl Pts',(73.492642788273,-8.83168607277325,12.));
#117037=CARTESIAN_POINT('Ctrl Pts',(73.4691870121567,-8.8177270092753,0.));
#117038=CARTESIAN_POINT('Ctrl Pts',(73.4691870121567,-8.8177270092753,12.));
#117039=CARTESIAN_POINT('Ctrl Pts',(73.4457492173933,-8.80380752553692,
0.));
#117040=CARTESIAN_POINT('Ctrl Pts',(73.4457492173933,-8.80380752553692,
12.));
#117041=CARTESIAN_POINT('Ctrl Pts',(73.422329507113,-8.78992762598756,0.));
#117042=CARTESIAN_POINT('Ctrl Pts',(73.422329507113,-8.78992762598756,12.));
#117043=CARTESIAN_POINT('Ctrl Pts',(73.3989279832835,-8.77608731509348,
0.));
#117044=CARTESIAN_POINT('Ctrl Pts',(73.3989279832835,-8.77608731509348,
12.));
#117045=CARTESIAN_POINT('Ctrl Pts',(73.3755447460269,-8.76228659740357,
0.));
#117046=CARTESIAN_POINT('Ctrl Pts',(73.3755447460269,-8.76228659740357,
12.));
#117047=CARTESIAN_POINT('Ctrl Pts',(73.3521798944622,-8.74852547749778,
0.));
#117048=CARTESIAN_POINT('Ctrl Pts',(73.3521798944622,-8.74852547749778,
12.));
#117049=CARTESIAN_POINT('Ctrl Pts',(73.3288335272002,-8.7348039599538,0.));
#117050=CARTESIAN_POINT('Ctrl Pts',(73.3288335272002,-8.7348039599538,12.));
#117051=CARTESIAN_POINT('Ctrl Pts',(73.3055057429742,-8.72112204930232,
0.));
#117052=CARTESIAN_POINT('Ctrl Pts',(73.3055057429742,-8.72112204930232,
12.));
#117053=CARTESIAN_POINT('Ctrl Pts',(73.2821966412148,-8.70747974998229,
0.));
#117054=CARTESIAN_POINT('Ctrl Pts',(73.2821966412148,-8.70747974998229,
12.));
#117055=CARTESIAN_POINT('Ctrl Pts',(73.2589063226358,-8.69387706629285,
0.));
#117056=CARTESIAN_POINT('Ctrl Pts',(73.2589063226358,-8.69387706629285,
12.));
#117057=CARTESIAN_POINT('Ctrl Pts',(73.2356348889693,-8.68031400241872,
0.));
#117058=CARTESIAN_POINT('Ctrl Pts',(73.2356348889693,-8.68031400241872,
12.));
#117059=CARTESIAN_POINT('Ctrl Pts',(73.2123824427208,-8.66679056245092,
0.));
#117060=CARTESIAN_POINT('Ctrl Pts',(73.2123824427208,-8.66679056245092,
12.));
#117061=CARTESIAN_POINT('Ctrl Pts',(73.1891490869056,-8.65330675040537,
0.));
#117062=CARTESIAN_POINT('Ctrl Pts',(73.1891490869056,-8.65330675040537,
12.));
#117063=CARTESIAN_POINT('Ctrl Pts',(73.1659349248132,-8.63986257023739,
0.));
#117064=CARTESIAN_POINT('Ctrl Pts',(73.1659349248132,-8.63986257023739,
12.));
#117065=CARTESIAN_POINT('Ctrl Pts',(73.1427400597037,-8.62645802585484,
0.));
#117066=CARTESIAN_POINT('Ctrl Pts',(73.1427400597037,-8.62645802585484,
12.));
#117067=CARTESIAN_POINT('Ctrl Pts',(73.1195645948178,-8.61309312112002,
0.));
#117068=CARTESIAN_POINT('Ctrl Pts',(73.1195645948178,-8.61309312112002,
12.));
#117069=CARTESIAN_POINT('Ctrl Pts',(73.0964086335235,-8.59976785984551,
0.));
#117070=CARTESIAN_POINT('Ctrl Pts',(73.0964086335235,-8.59976785984551,
12.));
#117071=CARTESIAN_POINT('Ctrl Pts',(73.0732722794195,-8.58648224578731,
0.));
#117072=CARTESIAN_POINT('Ctrl Pts',(73.0732722794195,-8.58648224578731,
12.));
#117073=CARTESIAN_POINT('Ctrl Pts',(73.0501556364479,-8.57323628263593,
0.));
#117074=CARTESIAN_POINT('Ctrl Pts',(73.0501556364479,-8.57323628263593,
12.));
#117075=CARTESIAN_POINT('Ctrl Pts',(73.0270588090183,-8.56002997400084,
0.));
#117076=CARTESIAN_POINT('Ctrl Pts',(73.0270588090183,-8.56002997400084,
12.));
#117077=CARTESIAN_POINT('Ctrl Pts',(73.0039819020648,-8.54686332340418,
0.));
#117078=CARTESIAN_POINT('Ctrl Pts',(73.0039819020648,-8.54686332340418,
12.));
#117079=CARTESIAN_POINT('Ctrl Pts',(72.9809250209828,-8.53373633429281,
0.));
#117080=CARTESIAN_POINT('Ctrl Pts',(72.9809250209828,-8.53373633429281,
12.));
#117081=CARTESIAN_POINT('Ctrl Pts',(72.9578882715912,-8.52064901004227,
0.));
#117082=CARTESIAN_POINT('Ctrl Pts',(72.9578882715912,-8.52064901004227,
12.));
#117083=CARTESIAN_POINT('Ctrl Pts',(72.9348717600838,-8.50760135395983,
0.));
#117084=CARTESIAN_POINT('Ctrl Pts',(72.9348717600838,-8.50760135395983,
12.));
#117085=CARTESIAN_POINT('Ctrl Pts',(72.9118755929795,-8.49459336928296,
0.));
#117086=CARTESIAN_POINT('Ctrl Pts',(72.9118755929795,-8.49459336928296,
12.));
#117087=CARTESIAN_POINT('Ctrl Pts',(72.8888998770785,-8.48162505917658,
0.));
#117088=CARTESIAN_POINT('Ctrl Pts',(72.8888998770785,-8.48162505917658,
12.));
#117089=CARTESIAN_POINT('Ctrl Pts',(72.8659447194933,-8.46869642673794,
0.));
#117090=CARTESIAN_POINT('Ctrl Pts',(72.8659447194933,-8.46869642673794,
12.));
#117091=CARTESIAN_POINT('Ctrl Pts',(72.8430102276713,-8.45580747499793,
0.));
#117092=CARTESIAN_POINT('Ctrl Pts',(72.8430102276713,-8.45580747499793,
12.));
#117093=CARTESIAN_POINT('Ctrl Pts',(72.8200965094199,-8.44295820691911,
0.));
#117094=CARTESIAN_POINT('Ctrl Pts',(72.8200965094199,-8.44295820691911,
12.));
#117095=CARTESIAN_POINT('Ctrl Pts',(72.7972036729276,-8.43014862539158,
0.));
#117096=CARTESIAN_POINT('Ctrl Pts',(72.7972036729276,-8.43014862539158,
12.));
#117097=CARTESIAN_POINT('Ctrl Pts',(72.7743318267865,-8.4173787332233,0.));
#117098=CARTESIAN_POINT('Ctrl Pts',(72.7743318267865,-8.4173787332233,12.));
#117099=CARTESIAN_POINT('Ctrl Pts',(72.751481079992,-8.40464853314468,0.));
#117100=CARTESIAN_POINT('Ctrl Pts',(72.751481079992,-8.40464853314468,12.));
#117101=CARTESIAN_POINT('Ctrl Pts',(72.7286515419373,-8.3919580278139,0.));
#117102=CARTESIAN_POINT('Ctrl Pts',(72.7286515419373,-8.3919580278139,12.));
#117103=CARTESIAN_POINT('Ctrl Pts',(72.705843322407,-8.37930721981731,0.));
#117104=CARTESIAN_POINT('Ctrl Pts',(72.705843322407,-8.37930721981731,12.));
#117105=CARTESIAN_POINT('Ctrl Pts',(72.6830565315703,-8.36669611166842,
0.));
#117106=CARTESIAN_POINT('Ctrl Pts',(72.6830565315703,-8.36669611166842,
12.));
#117107=CARTESIAN_POINT('Ctrl Pts',(72.6602912799696,-8.35412470580101,
0.));
#117108=CARTESIAN_POINT('Ctrl Pts',(72.6602912799696,-8.35412470580101,
12.));
#117109=CARTESIAN_POINT('Ctrl Pts',(72.6375476785215,-8.34159300456986,
0.));
#117110=CARTESIAN_POINT('Ctrl Pts',(72.6375476785215,-8.34159300456986,
12.));
#117111=CARTESIAN_POINT('Ctrl Pts',(72.6148258385296,-8.3291010102567,0.));
#117112=CARTESIAN_POINT('Ctrl Pts',(72.6148258385296,-8.3291010102567,12.));
#117113=CARTESIAN_POINT('Ctrl Pts',(72.5921258716901,-8.31664872507016,
0.));
#117114=CARTESIAN_POINT('Ctrl Pts',(72.5921258716901,-8.31664872507016,
12.));
#117115=CARTESIAN_POINT('Ctrl Pts',(72.5694478900982,-8.30423615114453,
0.));
#117116=CARTESIAN_POINT('Ctrl Pts',(72.5694478900982,-8.30423615114453,
12.));
#117117=CARTESIAN_POINT('Ctrl Pts',(72.5467920062521,-8.29186329053279,
0.));
#117118=CARTESIAN_POINT('Ctrl Pts',(72.5467920062521,-8.29186329053279,
12.));
#117119=CARTESIAN_POINT('Ctrl Pts',(72.5241583330562,-8.27953014520376,
0.));
#117120=CARTESIAN_POINT('Ctrl Pts',(72.5241583330562,-8.27953014520376,
12.));
#117121=CARTESIAN_POINT('Ctrl Pts',(72.5015469838254,-8.2672367170492,0.));
#117122=CARTESIAN_POINT('Ctrl Pts',(72.5015469838254,-8.2672367170492,12.));
#117123=CARTESIAN_POINT('Ctrl Pts',(72.4789580722875,-8.25498300788493,
0.));
#117124=CARTESIAN_POINT('Ctrl Pts',(72.4789580722875,-8.25498300788493,
12.));
#117125=CARTESIAN_POINT('Ctrl Pts',(72.4563917125842,-8.2427690194504,0.));
#117126=CARTESIAN_POINT('Ctrl Pts',(72.4563917125842,-8.2427690194504,12.));
#117127=CARTESIAN_POINT('Ctrl Pts',(72.4338480192695,-8.23059475340357,
0.));
#117128=CARTESIAN_POINT('Ctrl Pts',(72.4338480192695,-8.23059475340357,
12.));
#117129=CARTESIAN_POINT('Ctrl Pts',(72.4113271073079,-8.21846021131561,
0.));
#117130=CARTESIAN_POINT('Ctrl Pts',(72.4113271073079,-8.21846021131561,
12.));
#117131=CARTESIAN_POINT('Ctrl Pts',(72.3888290920832,-8.20636539467776,
0.));
#117132=CARTESIAN_POINT('Ctrl Pts',(72.3888290920832,-8.20636539467776,
12.));
#117133=CARTESIAN_POINT('Ctrl Pts',(72.3663540894026,-8.19431030490314,
0.));
#117134=CARTESIAN_POINT('Ctrl Pts',(72.3663540894026,-8.19431030490314,
12.));
#117135=CARTESIAN_POINT('Ctrl Pts',(72.3439022155007,-8.18229494332624,
0.));
#117136=CARTESIAN_POINT('Ctrl Pts',(72.3439022155007,-8.18229494332624,
12.));
#117137=CARTESIAN_POINT('Ctrl Pts',(72.3214735870409,-8.1703193111989,0.));
#117138=CARTESIAN_POINT('Ctrl Pts',(72.3214735870409,-8.1703193111989,12.));
#117139=CARTESIAN_POINT('Ctrl Pts',(72.2990683211162,-8.15838340968336,
0.));
#117140=CARTESIAN_POINT('Ctrl Pts',(72.2990683211162,-8.15838340968336,
12.));
#117141=CARTESIAN_POINT('Ctrl Pts',(72.2766865352555,-8.14648723985797,
0.));
#117142=CARTESIAN_POINT('Ctrl Pts',(72.2766865352555,-8.14648723985797,
12.));
#117143=CARTESIAN_POINT('Ctrl Pts',(72.2543283474278,-8.13463080272029,
0.));
#117144=CARTESIAN_POINT('Ctrl Pts',(72.2543283474278,-8.13463080272029,
12.));
#117145=CARTESIAN_POINT('Ctrl Pts',(72.2319938760449,-8.12281409918661,
0.));
#117146=CARTESIAN_POINT('Ctrl Pts',(72.2319938760449,-8.12281409918661,
12.));
#117147=CARTESIAN_POINT('Ctrl Pts',(72.209683239963,-8.11103713008928,0.));
#117148=CARTESIAN_POINT('Ctrl Pts',(72.209683239963,-8.11103713008928,12.));
#117149=CARTESIAN_POINT('Ctrl Pts',(72.1873965584813,-8.0992998961689,0.));
#117150=CARTESIAN_POINT('Ctrl Pts',(72.1873965584813,-8.0992998961689,12.));
#117151=CARTESIAN_POINT('Ctrl Pts',(72.1651339513477,-8.08760239807836,
0.));
#117152=CARTESIAN_POINT('Ctrl Pts',(72.1651339513477,-8.08760239807836,
12.));
#117153=CARTESIAN_POINT('Ctrl Pts',(72.1428955387663,-8.07594463638719,
0.));
#117154=CARTESIAN_POINT('Ctrl Pts',(72.1428955387663,-8.07594463638719,
12.));
#117155=CARTESIAN_POINT('Ctrl Pts',(72.1206814413988,-8.06432661158096,
0.));
#117156=CARTESIAN_POINT('Ctrl Pts',(72.1206814413988,-8.06432661158096,
12.));
#117157=CARTESIAN_POINT('Ctrl Pts',(72.0984917803693,-8.05274832405948,
0.));
#117158=CARTESIAN_POINT('Ctrl Pts',(72.0984917803693,-8.05274832405948,
12.));
#117159=CARTESIAN_POINT('Ctrl Pts',(72.0763266772615,-8.04120977412872,
0.));
#117160=CARTESIAN_POINT('Ctrl Pts',(72.0763266772615,-8.04120977412872,
12.));
#117161=CARTESIAN_POINT('Ctrl Pts',(72.0541862541243,-8.02971096200307,
0.));
#117162=CARTESIAN_POINT('Ctrl Pts',(72.0541862541243,-8.02971096200307,
12.));
#117163=CARTESIAN_POINT('Ctrl Pts',(72.032070633479,-8.01825188781056,0.));
#117164=CARTESIAN_POINT('Ctrl Pts',(72.032070633479,-8.01825188781056,12.));
#117165=CARTESIAN_POINT('Ctrl Pts',(72.0099799383213,-8.00683255159247,
0.));
#117166=CARTESIAN_POINT('Ctrl Pts',(72.0099799383213,-8.00683255159247,
12.));
#117167=CARTESIAN_POINT('Ctrl Pts',(71.9879142921254,-7.99545295330191,
0.));
#117168=CARTESIAN_POINT('Ctrl Pts',(71.9879142921254,-7.99545295330191,
12.));
#117169=CARTESIAN_POINT('Ctrl Pts',(71.965873818843,-7.98411309279612,0.));
#117170=CARTESIAN_POINT('Ctrl Pts',(71.965873818843,-7.98411309279612,12.));
#117171=CARTESIAN_POINT('Ctrl Pts',(71.9438586429081,-7.97281296983718,
0.));
#117172=CARTESIAN_POINT('Ctrl Pts',(71.9438586429081,-7.97281296983718,
12.));
#117173=CARTESIAN_POINT('Ctrl Pts',(71.9218688892431,-7.96155258409763,
0.));
#117174=CARTESIAN_POINT('Ctrl Pts',(71.9218688892431,-7.96155258409763,
12.));
#117175=CARTESIAN_POINT('Ctrl Pts',(71.8999046832643,-7.9503319351605,0.));
#117176=CARTESIAN_POINT('Ctrl Pts',(71.8999046832643,-7.9503319351605,12.));
#117177=CARTESIAN_POINT('Ctrl Pts',(71.8779661508832,-7.93915102251794,
0.));
#117178=CARTESIAN_POINT('Ctrl Pts',(71.8779661508832,-7.93915102251794,
12.));
#117179=CARTESIAN_POINT('Ctrl Pts',(71.8560534185071,-7.92800984556396,
0.));
#117180=CARTESIAN_POINT('Ctrl Pts',(71.8560534185071,-7.92800984556396,
12.));
#117181=CARTESIAN_POINT('Ctrl Pts',(71.8341666130426,-7.91690840359367,
0.));
#117182=CARTESIAN_POINT('Ctrl Pts',(71.8341666130426,-7.91690840359367,
12.));
#117183=CARTESIAN_POINT('Ctrl Pts',(71.8123058619042,-7.90584669580955,
0.));
#117184=CARTESIAN_POINT('Ctrl Pts',(71.8123058619042,-7.90584669580955,
12.));
#117185=CARTESIAN_POINT('Ctrl Pts',(71.7904712930175,-7.89482472132137,
0.));
#117186=CARTESIAN_POINT('Ctrl Pts',(71.7904712930175,-7.89482472132137,
12.));
#117187=CARTESIAN_POINT('Ctrl Pts',(71.7686630348238,-7.88384247914524,
0.));
#117188=CARTESIAN_POINT('Ctrl Pts',(71.7686630348238,-7.88384247914524,
12.));
#117189=CARTESIAN_POINT('Ctrl Pts',(71.7468812162788,-7.87289996819653,
0.));
#117190=CARTESIAN_POINT('Ctrl Pts',(71.7468812162788,-7.87289996819653,
12.));
#117191=CARTESIAN_POINT('Ctrl Pts',(71.7251259668563,-7.86199718728826,
0.));
#117192=CARTESIAN_POINT('Ctrl Pts',(71.7251259668563,-7.86199718728826,
12.));
#117193=CARTESIAN_POINT('Ctrl Pts',(71.7033974165568,-7.85113413513736,
0.));
#117194=CARTESIAN_POINT('Ctrl Pts',(71.7033974165568,-7.85113413513736,
12.));
#117195=CARTESIAN_POINT('Ctrl Pts',(71.6816956959117,-7.84031081036489,
0.));
#117196=CARTESIAN_POINT('Ctrl Pts',(71.6816956959117,-7.84031081036489,
12.));
#117197=CARTESIAN_POINT('Ctrl Pts',(71.6600209359872,-7.82952721149507,
0.));
#117198=CARTESIAN_POINT('Ctrl Pts',(71.6600209359872,-7.82952721149507,
12.));
#117199=CARTESIAN_POINT('Ctrl Pts',(71.6383732683844,-7.8187833369486,0.));
#117200=CARTESIAN_POINT('Ctrl Pts',(71.6383732683844,-7.8187833369486,12.));
#117201=CARTESIAN_POINT('Ctrl Pts',(71.6167528252423,-7.80807918504021,
0.));
#117202=CARTESIAN_POINT('Ctrl Pts',(71.6167528252423,-7.80807918504021,
12.));
#117203=CARTESIAN_POINT('Ctrl Pts',(71.5951597392471,-7.79741475398513,
0.));
#117204=CARTESIAN_POINT('Ctrl Pts',(71.5951597392471,-7.79741475398513,
12.));
#117205=CARTESIAN_POINT('Ctrl Pts',(71.5735941436364,-7.78679004189935,
0.));
#117206=CARTESIAN_POINT('Ctrl Pts',(71.5735941436364,-7.78679004189935,
12.));
#117207=CARTESIAN_POINT('Ctrl Pts',(71.5520561722039,-7.77620504679869,
0.));
#117208=CARTESIAN_POINT('Ctrl Pts',(71.5520561722039,-7.77620504679869,
12.));
#117209=CARTESIAN_POINT('Ctrl Pts',(71.5305459592994,-7.76565976659226,
0.));
#117210=CARTESIAN_POINT('Ctrl Pts',(71.5305459592994,-7.76565976659226,
12.));
#117211=CARTESIAN_POINT('Ctrl Pts',(71.5090636398318,-7.75515419907966,
0.));
#117212=CARTESIAN_POINT('Ctrl Pts',(71.5090636398318,-7.75515419907966,
12.));
#117213=CARTESIAN_POINT('Ctrl Pts',(71.4876093492781,-7.74468834195746,
0.));
#117214=CARTESIAN_POINT('Ctrl Pts',(71.4876093492781,-7.74468834195746,
12.));
#117215=CARTESIAN_POINT('Ctrl Pts',(71.4661832236888,-7.7342621928194,0.));
#117216=CARTESIAN_POINT('Ctrl Pts',(71.4661832236888,-7.7342621928194,12.));
#117217=CARTESIAN_POINT('Ctrl Pts',(71.4447853996916,-7.72387574915544,
0.));
#117218=CARTESIAN_POINT('Ctrl Pts',(71.4447853996916,-7.72387574915544,
12.));
#117219=CARTESIAN_POINT('Ctrl Pts',(71.4234160144925,-7.7135290083452,0.));
#117220=CARTESIAN_POINT('Ctrl Pts',(71.4234160144925,-7.7135290083452,12.));
#117221=CARTESIAN_POINT('Ctrl Pts',(71.4020752058796,-7.70322196765538,
0.));
#117222=CARTESIAN_POINT('Ctrl Pts',(71.4020752058796,-7.70322196765538,
12.));
#117223=CARTESIAN_POINT('Ctrl Pts',(71.3807631122331,-7.69295462424612,
0.));
#117224=CARTESIAN_POINT('Ctrl Pts',(71.3807631122331,-7.69295462424612,
12.));
#117225=CARTESIAN_POINT('Ctrl Pts',(71.3594798725281,-7.68272697517086,
0.));
#117226=CARTESIAN_POINT('Ctrl Pts',(71.3594798725281,-7.68272697517086,
12.));
#117227=CARTESIAN_POINT('Ctrl Pts',(71.3382256263414,-7.67253901737552,
0.));
#117228=CARTESIAN_POINT('Ctrl Pts',(71.3382256263414,-7.67253901737552,
12.));
#117229=CARTESIAN_POINT('Ctrl Pts',(71.3170005138502,-7.66239074769163,
0.));
#117230=CARTESIAN_POINT('Ctrl Pts',(71.3170005138502,-7.66239074769163,
12.));
#117231=CARTESIAN_POINT('Ctrl Pts',(71.2958046758372,-7.65228216283404,
0.));
#117232=CARTESIAN_POINT('Ctrl Pts',(71.2958046758372,-7.65228216283404,
12.));
#117233=CARTESIAN_POINT('Ctrl Pts',(71.2746382537007,-7.64221325940724,
0.));
#117234=CARTESIAN_POINT('Ctrl Pts',(71.2746382537007,-7.64221325940724,
12.));
#117235=CARTESIAN_POINT('Ctrl Pts',(71.2535013894602,-7.63218403390537,
0.));
#117236=CARTESIAN_POINT('Ctrl Pts',(71.2535013894602,-7.63218403390537,
12.));
#117237=CARTESIAN_POINT('Ctrl Pts',(71.2323942257609,-7.62219448271109,
0.));
#117238=CARTESIAN_POINT('Ctrl Pts',(71.2323942257609,-7.62219448271109,
12.));
#117239=CARTESIAN_POINT('Ctrl Pts',(71.211316905874,-7.61224460208837,0.));
#117240=CARTESIAN_POINT('Ctrl Pts',(71.211316905874,-7.61224460208837,12.));
#117241=CARTESIAN_POINT('Ctrl Pts',(71.1902695737013,-7.60233438818096,
0.));
#117242=CARTESIAN_POINT('Ctrl Pts',(71.1902695737013,-7.60233438818096,
12.));
#117243=CARTESIAN_POINT('Ctrl Pts',(71.1692523737844,-7.59246383701814,
0.));
#117244=CARTESIAN_POINT('Ctrl Pts',(71.1692523737844,-7.59246383701814,
12.));
#117245=CARTESIAN_POINT('Ctrl Pts',(71.1482654513119,-7.58263294451452,
0.));
#117246=CARTESIAN_POINT('Ctrl Pts',(71.1482654513119,-7.58263294451452,
12.));
#117247=CARTESIAN_POINT('Ctrl Pts',(71.1273089521234,-7.57284170646886,
0.));
#117248=CARTESIAN_POINT('Ctrl Pts',(71.1273089521234,-7.57284170646886,
12.));
#117249=CARTESIAN_POINT('Ctrl Pts',(71.106383022711,-7.56309011855657,0.));
#117250=CARTESIAN_POINT('Ctrl Pts',(71.106383022711,-7.56309011855657,12.));
#117251=CARTESIAN_POINT('Ctrl Pts',(71.0854878102243,-7.55337817632916,
0.));
#117252=CARTESIAN_POINT('Ctrl Pts',(71.0854878102243,-7.55337817632916,
12.));
#117253=CARTESIAN_POINT('Ctrl Pts',(71.0646234624811,-7.54370587521979,
0.));
#117254=CARTESIAN_POINT('Ctrl Pts',(71.0646234624811,-7.54370587521979,
12.));
#117255=CARTESIAN_POINT('Ctrl Pts',(71.043790127973,-7.53407321054262,0.));
#117256=CARTESIAN_POINT('Ctrl Pts',(71.043790127973,-7.53407321054262,12.));
#117257=CARTESIAN_POINT('Ctrl Pts',(71.0229879558699,-7.52448017749125,
0.));
#117258=CARTESIAN_POINT('Ctrl Pts',(71.0229879558699,-7.52448017749125,
12.));
#117259=CARTESIAN_POINT('Ctrl Pts',(71.002217096021,-7.5149267711309,0.));
#117260=CARTESIAN_POINT('Ctrl Pts',(71.002217096021,-7.5149267711309,12.));
#117261=CARTESIAN_POINT('Ctrl Pts',(70.9814776989612,-7.50541298639928,
0.));
#117262=CARTESIAN_POINT('Ctrl Pts',(70.9814776989612,-7.50541298639928,
12.));
#117263=CARTESIAN_POINT('Ctrl Pts',(70.9607699159218,-7.4959388181113,0.));
#117264=CARTESIAN_POINT('Ctrl Pts',(70.9607699159218,-7.4959388181113,12.));
#117265=CARTESIAN_POINT('Ctrl Pts',(70.940093898837,-7.48650426095824,0.));
#117266=CARTESIAN_POINT('Ctrl Pts',(70.940093898837,-7.48650426095824,12.));
#117267=CARTESIAN_POINT('Ctrl Pts',(70.9194498003493,-7.47710930950562,
0.));
#117268=CARTESIAN_POINT('Ctrl Pts',(70.9194498003493,-7.47710930950562,
12.));
#117269=CARTESIAN_POINT('Ctrl Pts',(70.8988377738104,-7.46775395818527,
0.));
#117270=CARTESIAN_POINT('Ctrl Pts',(70.8988377738104,-7.46775395818527,
12.));
#117271=CARTESIAN_POINT('Ctrl Pts',(70.87825797329,-7.45843820129782,0.));
#117272=CARTESIAN_POINT('Ctrl Pts',(70.87825797329,-7.45843820129782,12.));
#117273=CARTESIAN_POINT('Ctrl Pts',(70.8577105535848,-7.44916203301647,
0.));
#117274=CARTESIAN_POINT('Ctrl Pts',(70.8577105535848,-7.44916203301647,
12.));
#117275=CARTESIAN_POINT('Ctrl Pts',(70.8371956702241,-7.43992544738606,
0.));
#117276=CARTESIAN_POINT('Ctrl Pts',(70.8371956702241,-7.43992544738606,
12.));
#117277=CARTESIAN_POINT('Ctrl Pts',(70.8167134794737,-7.43072843832014,
0.));
#117278=CARTESIAN_POINT('Ctrl Pts',(70.8167134794737,-7.43072843832014,
12.));
#117279=CARTESIAN_POINT('Ctrl Pts',(70.796264138335,-7.42157099959326,0.));
#117280=CARTESIAN_POINT('Ctrl Pts',(70.796264138335,-7.42157099959326,12.));
#117281=CARTESIAN_POINT('Ctrl Pts',(70.7758478045576,-7.41245312484498,
0.));
#117282=CARTESIAN_POINT('Ctrl Pts',(70.7758478045576,-7.41245312484498,
12.));
#117283=CARTESIAN_POINT('Ctrl Pts',(70.7554646366514,-7.40337480758237,
0.));
#117284=CARTESIAN_POINT('Ctrl Pts',(70.7554646366514,-7.40337480758237,
12.));
#117285=CARTESIAN_POINT('Ctrl Pts',(70.735114793895,-7.39433604117891,0.));
#117286=CARTESIAN_POINT('Ctrl Pts',(70.735114793895,-7.39433604117891,12.));
#117287=CARTESIAN_POINT('Ctrl Pts',(70.7147984363423,-7.38533681887028,
0.));
#117288=CARTESIAN_POINT('Ctrl Pts',(70.7147984363423,-7.38533681887028,
12.));
#117289=CARTESIAN_POINT('Ctrl Pts',(70.6945157248269,-7.37637713374761,
0.));
#117290=CARTESIAN_POINT('Ctrl Pts',(70.6945157248269,-7.37637713374761,
12.));
#117291=CARTESIAN_POINT('Ctrl Pts',(70.6742668209685,-7.36745697876295,
0.));
#117292=CARTESIAN_POINT('Ctrl Pts',(70.6742668209685,-7.36745697876295,
12.));
#117293=CARTESIAN_POINT('Ctrl Pts',(70.6540518871772,-7.35857634673052,
0.));
#117294=CARTESIAN_POINT('Ctrl Pts',(70.6540518871772,-7.35857634673052,
12.));
#117295=CARTESIAN_POINT('Ctrl Pts',(70.6338710866562,-7.3497352303258,0.));
#117296=CARTESIAN_POINT('Ctrl Pts',(70.6338710866562,-7.3497352303258,12.));
#117297=CARTESIAN_POINT('Ctrl Pts',(70.6137245834002,-7.34093362208018,
0.));
#117298=CARTESIAN_POINT('Ctrl Pts',(70.6137245834002,-7.34093362208018,
12.));
#117299=CARTESIAN_POINT('Ctrl Pts',(70.5936125421958,-7.33217151437608,
0.));
#117300=CARTESIAN_POINT('Ctrl Pts',(70.5936125421958,-7.33217151437608,
12.));
#117301=CARTESIAN_POINT('Ctrl Pts',(70.573535128649,-7.32344889945237,0.));
#117302=CARTESIAN_POINT('Ctrl Pts',(70.573535128649,-7.32344889945237,12.));
#117303=CARTESIAN_POINT('Ctrl Pts',(70.5534925092053,-7.31476576940403,
0.));
#117304=CARTESIAN_POINT('Ctrl Pts',(70.5534925092053,-7.31476576940403,
12.));
#117305=CARTESIAN_POINT('Ctrl Pts',(70.5334848511675,-7.30612211618047,
0.));
#117306=CARTESIAN_POINT('Ctrl Pts',(70.5334848511675,-7.30612211618047,
12.));
#117307=CARTESIAN_POINT('Ctrl Pts',(70.5135123227147,-7.29751793157801,
0.));
#117308=CARTESIAN_POINT('Ctrl Pts',(70.5135123227147,-7.29751793157801,
12.));
#117309=CARTESIAN_POINT('Ctrl Pts',(70.4935750929029,-7.28895320723835,
0.));
#117310=CARTESIAN_POINT('Ctrl Pts',(70.4935750929029,-7.28895320723835,
12.));
#117311=CARTESIAN_POINT('Ctrl Pts',(70.4736733316463,-7.28042793465449,
0.));
#117312=CARTESIAN_POINT('Ctrl Pts',(70.4736733316463,-7.28042793465449,
12.));
#117313=CARTESIAN_POINT('Ctrl Pts',(70.4538072096986,-7.27194210517057,
0.));
#117314=CARTESIAN_POINT('Ctrl Pts',(70.4538072096986,-7.27194210517057,
12.));
#117315=CARTESIAN_POINT('Ctrl Pts',(70.433976898636,-7.2634957099805,0.));
#117316=CARTESIAN_POINT('Ctrl Pts',(70.433976898636,-7.2634957099805,12.));
#117317=CARTESIAN_POINT('Ctrl Pts',(70.4141825708207,-7.25508874012076,
0.));
#117318=CARTESIAN_POINT('Ctrl Pts',(70.4141825708207,-7.25508874012076,
12.));
#117319=CARTESIAN_POINT('Ctrl Pts',(70.3944243994532,-7.24672118647116,
0.));
#117320=CARTESIAN_POINT('Ctrl Pts',(70.3944243994532,-7.24672118647116,
12.));
#117321=CARTESIAN_POINT('Ctrl Pts',(70.3747025586569,-7.23839303975626,
0.));
#117322=CARTESIAN_POINT('Ctrl Pts',(70.3747025586569,-7.23839303975626,
12.));
#117323=CARTESIAN_POINT('Ctrl Pts',(70.3550172235486,-7.23010429054231,
0.));
#117324=CARTESIAN_POINT('Ctrl Pts',(70.3550172235486,-7.23010429054231,
12.));
#117325=CARTESIAN_POINT('Ctrl Pts',(70.3353685703097,-7.22185492923178,
0.));
#117326=CARTESIAN_POINT('Ctrl Pts',(70.3353685703097,-7.22185492923178,
12.));
#117327=CARTESIAN_POINT('Ctrl Pts',(70.3157567762561,-7.21364494605425,
0.));
#117328=CARTESIAN_POINT('Ctrl Pts',(70.3157567762561,-7.21364494605425,
12.));
#117329=CARTESIAN_POINT('Ctrl Pts',(70.2961820197051,-7.20547433107457,
0.));
#117330=CARTESIAN_POINT('Ctrl Pts',(70.2961820197051,-7.20547433107457,
12.));
#117331=CARTESIAN_POINT('Ctrl Pts',(70.276644479827,-7.19734307419861,0.));
#117332=CARTESIAN_POINT('Ctrl Pts',(70.276644479827,-7.19734307419861,12.));
#117333=CARTESIAN_POINT('Ctrl Pts',(70.2571443365198,-7.18925116517562,
0.));
#117334=CARTESIAN_POINT('Ctrl Pts',(70.2571443365198,-7.18925116517562,
12.));
#117335=CARTESIAN_POINT('Ctrl Pts',(70.2376817702239,-7.181198593598,0.));
#117336=CARTESIAN_POINT('Ctrl Pts',(70.2376817702239,-7.181198593598,12.));
#117337=CARTESIAN_POINT('Ctrl Pts',(70.2182569619028,-7.17318534889747,
0.));
#117338=CARTESIAN_POINT('Ctrl Pts',(70.2182569619028,-7.17318534889747,
12.));
#117339=CARTESIAN_POINT('Ctrl Pts',(70.1988700934622,-7.16521142033892,
0.));
#117340=CARTESIAN_POINT('Ctrl Pts',(70.1988700934622,-7.16521142033892,
12.));
#117341=CARTESIAN_POINT('Ctrl Pts',(70.1795213481196,-7.15727679700946,
0.));
#117342=CARTESIAN_POINT('Ctrl Pts',(70.1795213481196,-7.15727679700946,
12.));
#117343=CARTESIAN_POINT('Ctrl Pts',(70.1602109107188,-7.14938146780801,
0.));
#117344=CARTESIAN_POINT('Ctrl Pts',(70.1602109107188,-7.14938146780801,
12.));
#117345=CARTESIAN_POINT('Ctrl Pts',(70.1409389682389,-7.14152542142339,
0.));
#117346=CARTESIAN_POINT('Ctrl Pts',(70.1409389682389,-7.14152542142339,
12.));
#117347=CARTESIAN_POINT('Ctrl Pts',(70.1217057094456,-7.13370864634398,
0.));
#117348=CARTESIAN_POINT('Ctrl Pts',(70.1217057094456,-7.13370864634398,
12.));
#117349=CARTESIAN_POINT('Ctrl Pts',(70.1025113239463,-7.12593113088871,
0.));
#117350=CARTESIAN_POINT('Ctrl Pts',(70.1025113239463,-7.12593113088871,
12.));
#117351=CARTESIAN_POINT('Ctrl Pts',(70.0833560013971,-7.11819286322824,
0.));
#117352=CARTESIAN_POINT('Ctrl Pts',(70.0833560013971,-7.11819286322824,
12.));
#117353=CARTESIAN_POINT('Ctrl Pts',(70.06423993069,-7.11049383140482,0.));
#117354=CARTESIAN_POINT('Ctrl Pts',(70.06423993069,-7.11049383140482,12.));
#117355=CARTESIAN_POINT('Ctrl Pts',(70.0451632990137,-7.10283402335091,
0.));
#117356=CARTESIAN_POINT('Ctrl Pts',(70.0451632990137,-7.10283402335091,
12.));
#117357=CARTESIAN_POINT('Ctrl Pts',(70.0261262936435,-7.09521342684301,
0.));
#117358=CARTESIAN_POINT('Ctrl Pts',(70.0261262936435,-7.09521342684301,
12.));
#117359=CARTESIAN_POINT('Ctrl Pts',(70.0071291040791,-7.08763202944274,
0.));
#117360=CARTESIAN_POINT('Ctrl Pts',(70.0071291040791,-7.08763202944274,
12.));
#117361=CARTESIAN_POINT('Ctrl Pts',(69.988171923787,-7.08008981844643,0.));
#117362=CARTESIAN_POINT('Ctrl Pts',(69.988171923787,-7.08008981844643,12.));
#117363=CARTESIAN_POINT('Ctrl Pts',(69.9692549527256,-7.07258678080793,
0.));
#117364=CARTESIAN_POINT('Ctrl Pts',(69.9692549527256,-7.07258678080793,
12.));
#117365=CARTESIAN_POINT('Ctrl Pts',(69.9503783975676,-7.06512290312803,
0.));
#117366=CARTESIAN_POINT('Ctrl Pts',(69.9503783975676,-7.06512290312803,
12.));
#117367=CARTESIAN_POINT('Ctrl Pts',(69.9315424664252,-7.05769817180824,
0.));
#117368=CARTESIAN_POINT('Ctrl Pts',(69.9315424664252,-7.05769817180824,
12.));
#117369=CARTESIAN_POINT('Ctrl Pts',(69.9127473642087,-7.05031257318108,
0.));
#117370=CARTESIAN_POINT('Ctrl Pts',(69.9127473642087,-7.05031257318108,
12.));
#117371=CARTESIAN_POINT('Ctrl Pts',(69.8939932885864,-7.04296609362187,
0.));
#117372=CARTESIAN_POINT('Ctrl Pts',(69.8939932885864,-7.04296609362187,
12.));
#117373=CARTESIAN_POINT('Ctrl Pts',(69.8752804235296,-7.03565871972265,
0.));
#117374=CARTESIAN_POINT('Ctrl Pts',(69.8752804235296,-7.03565871972265,
12.));
#117375=CARTESIAN_POINT('Ctrl Pts',(69.8566089455448,-7.02839043811863,
0.));
#117376=CARTESIAN_POINT('Ctrl Pts',(69.8566089455448,-7.02839043811863,
12.));
#117377=CARTESIAN_POINT('Ctrl Pts',(69.8379790360574,-7.02116123514487,
0.));
#117378=CARTESIAN_POINT('Ctrl Pts',(69.8379790360574,-7.02116123514487,
12.));
#117379=CARTESIAN_POINT('Ctrl Pts',(69.8193908913722,-7.01397109655455,
0.));
#117380=CARTESIAN_POINT('Ctrl Pts',(69.8193908913722,-7.01397109655455,
12.));
#117381=CARTESIAN_POINT('Ctrl Pts',(69.8008447346782,-7.00682000718105,
0.));
#117382=CARTESIAN_POINT('Ctrl Pts',(69.8008447346782,-7.00682000718105,
12.));
#117383=CARTESIAN_POINT('Ctrl Pts',(69.7823408242446,-6.99970795069399,
0.));
#117384=CARTESIAN_POINT('Ctrl Pts',(69.7823408242446,-6.99970795069399,
12.));
#117385=CARTESIAN_POINT('Ctrl Pts',(69.7638794280263,-6.9926349102786,0.));
#117386=CARTESIAN_POINT('Ctrl Pts',(69.7638794280263,-6.9926349102786,12.));
#117387=CARTESIAN_POINT('Ctrl Pts',(69.7454607995524,-6.98560086924173,
0.));
#117388=CARTESIAN_POINT('Ctrl Pts',(69.7454607995524,-6.98560086924173,
12.));
#117389=CARTESIAN_POINT('Ctrl Pts',(69.7270851557443,-6.97860581164569,
0.));
#117390=CARTESIAN_POINT('Ctrl Pts',(69.7270851557443,-6.97860581164569,
12.));
#117391=CARTESIAN_POINT('Ctrl Pts',(69.7087526480249,-6.97164972291582,
0.));
#117392=CARTESIAN_POINT('Ctrl Pts',(69.7087526480249,-6.97164972291582,
12.));
#117393=CARTESIAN_POINT('Ctrl Pts',(69.6904633605834,-6.96473259049729,
0.));
#117394=CARTESIAN_POINT('Ctrl Pts',(69.6904633605834,-6.96473259049729,
12.));
#117395=CARTESIAN_POINT('Ctrl Pts',(69.6758665380764,-6.95923004173795,
0.));
#117396=CARTESIAN_POINT('Ctrl Pts',(69.6758665380764,-6.95923004173795,
12.));
#117397=CARTESIAN_POINT('Ctrl Pts',(69.6649383920075,-6.95512065317731,
0.));
#117398=CARTESIAN_POINT('Ctrl Pts',(69.6649383920075,-6.95512065317731,
12.));
#117399=CARTESIAN_POINT('Ctrl Pts',(69.6576616146559,-6.95238884849075,
0.));
#117400=CARTESIAN_POINT('Ctrl Pts',(69.6576616146559,-6.95238884849075,
12.));
#117401=CARTESIAN_POINT('Ctrl Pts',(69.6540253893193,-6.95102489306927,
0.));
#117402=CARTESIAN_POINT('Ctrl Pts',(69.6540253893193,-6.95102489306927,
12.));
#117403=CARTESIAN_POINT('',(69.6540253893193,-6.95102489306927,12.));
#117404=CARTESIAN_POINT('Ctrl Pts',(69.6540253893193,-6.95102489306927,
12.));
#117405=CARTESIAN_POINT('Ctrl Pts',(69.6576616146559,-6.95238884849075,
12.));
#117406=CARTESIAN_POINT('Ctrl Pts',(69.6649383920075,-6.95512065317731,
12.));
#117407=CARTESIAN_POINT('Ctrl Pts',(69.6758665380764,-6.95923004173795,
12.));
#117408=CARTESIAN_POINT('Ctrl Pts',(69.6904633605834,-6.96473259049729,
12.));
#117409=CARTESIAN_POINT('Ctrl Pts',(69.7087526480249,-6.97164972291582,
12.));
#117410=CARTESIAN_POINT('Ctrl Pts',(69.7270851557443,-6.97860581164569,
12.));
#117411=CARTESIAN_POINT('Ctrl Pts',(69.7454607995524,-6.98560086924173,
12.));
#117412=CARTESIAN_POINT('Ctrl Pts',(69.7638794280263,-6.9926349102786,12.));
#117413=CARTESIAN_POINT('Ctrl Pts',(69.7823408242446,-6.99970795069399,
12.));
#117414=CARTESIAN_POINT('Ctrl Pts',(69.8008447346782,-7.00682000718105,
12.));
#117415=CARTESIAN_POINT('Ctrl Pts',(69.8193908913722,-7.01397109655455,
12.));
#117416=CARTESIAN_POINT('Ctrl Pts',(69.8379790360574,-7.02116123514487,
12.));
#117417=CARTESIAN_POINT('Ctrl Pts',(69.8566089455448,-7.02839043811863,
12.));
#117418=CARTESIAN_POINT('Ctrl Pts',(69.8752804235296,-7.03565871972265,
12.));
#117419=CARTESIAN_POINT('Ctrl Pts',(69.8939932885864,-7.04296609362187,
12.));
#117420=CARTESIAN_POINT('Ctrl Pts',(69.9127473642087,-7.05031257318108,
12.));
#117421=CARTESIAN_POINT('Ctrl Pts',(69.9315424664252,-7.05769817180824,
12.));
#117422=CARTESIAN_POINT('Ctrl Pts',(69.9503783975676,-7.06512290312803,
12.));
#117423=CARTESIAN_POINT('Ctrl Pts',(69.9692549527256,-7.07258678080793,
12.));
#117424=CARTESIAN_POINT('Ctrl Pts',(69.988171923787,-7.08008981844643,12.));
#117425=CARTESIAN_POINT('Ctrl Pts',(70.0071291040791,-7.08763202944274,
12.));
#117426=CARTESIAN_POINT('Ctrl Pts',(70.0261262936435,-7.09521342684301,
12.));
#117427=CARTESIAN_POINT('Ctrl Pts',(70.0451632990137,-7.10283402335091,
12.));
#117428=CARTESIAN_POINT('Ctrl Pts',(70.06423993069,-7.11049383140482,12.));
#117429=CARTESIAN_POINT('Ctrl Pts',(70.0833560013971,-7.11819286322824,
12.));
#117430=CARTESIAN_POINT('Ctrl Pts',(70.1025113239463,-7.12593113088871,
12.));
#117431=CARTESIAN_POINT('Ctrl Pts',(70.1217057094456,-7.13370864634398,
12.));
#117432=CARTESIAN_POINT('Ctrl Pts',(70.1409389682389,-7.14152542142339,
12.));
#117433=CARTESIAN_POINT('Ctrl Pts',(70.1602109107188,-7.14938146780801,
12.));
#117434=CARTESIAN_POINT('Ctrl Pts',(70.1795213481196,-7.15727679700946,
12.));
#117435=CARTESIAN_POINT('Ctrl Pts',(70.1988700934622,-7.16521142033892,
12.));
#117436=CARTESIAN_POINT('Ctrl Pts',(70.2182569619028,-7.17318534889747,
12.));
#117437=CARTESIAN_POINT('Ctrl Pts',(70.2376817702239,-7.181198593598,12.));
#117438=CARTESIAN_POINT('Ctrl Pts',(70.2571443365198,-7.18925116517562,
12.));
#117439=CARTESIAN_POINT('Ctrl Pts',(70.276644479827,-7.19734307419861,12.));
#117440=CARTESIAN_POINT('Ctrl Pts',(70.2961820197051,-7.20547433107457,
12.));
#117441=CARTESIAN_POINT('Ctrl Pts',(70.3157567762561,-7.21364494605425,
12.));
#117442=CARTESIAN_POINT('Ctrl Pts',(70.3353685703097,-7.22185492923178,
12.));
#117443=CARTESIAN_POINT('Ctrl Pts',(70.3550172235486,-7.23010429054231,
12.));
#117444=CARTESIAN_POINT('Ctrl Pts',(70.3747025586569,-7.23839303975626,
12.));
#117445=CARTESIAN_POINT('Ctrl Pts',(70.3944243994532,-7.24672118647116,
12.));
#117446=CARTESIAN_POINT('Ctrl Pts',(70.4141825708207,-7.25508874012076,
12.));
#117447=CARTESIAN_POINT('Ctrl Pts',(70.433976898636,-7.2634957099805,12.));
#117448=CARTESIAN_POINT('Ctrl Pts',(70.4538072096986,-7.27194210517057,
12.));
#117449=CARTESIAN_POINT('Ctrl Pts',(70.4736733316463,-7.28042793465449,
12.));
#117450=CARTESIAN_POINT('Ctrl Pts',(70.4935750929029,-7.28895320723835,
12.));
#117451=CARTESIAN_POINT('Ctrl Pts',(70.5135123227147,-7.29751793157801,
12.));
#117452=CARTESIAN_POINT('Ctrl Pts',(70.5334848511675,-7.30612211618047,
12.));
#117453=CARTESIAN_POINT('Ctrl Pts',(70.5534925092053,-7.31476576940403,
12.));
#117454=CARTESIAN_POINT('Ctrl Pts',(70.573535128649,-7.32344889945237,12.));
#117455=CARTESIAN_POINT('Ctrl Pts',(70.5936125421958,-7.33217151437608,
12.));
#117456=CARTESIAN_POINT('Ctrl Pts',(70.6137245834002,-7.34093362208018,
12.));
#117457=CARTESIAN_POINT('Ctrl Pts',(70.6338710866562,-7.3497352303258,12.));
#117458=CARTESIAN_POINT('Ctrl Pts',(70.6540518871772,-7.35857634673052,
12.));
#117459=CARTESIAN_POINT('Ctrl Pts',(70.6742668209685,-7.36745697876295,
12.));
#117460=CARTESIAN_POINT('Ctrl Pts',(70.6945157248269,-7.37637713374761,
12.));
#117461=CARTESIAN_POINT('Ctrl Pts',(70.7147984363423,-7.38533681887028,
12.));
#117462=CARTESIAN_POINT('Ctrl Pts',(70.735114793895,-7.39433604117891,12.));
#117463=CARTESIAN_POINT('Ctrl Pts',(70.7554646366514,-7.40337480758237,
12.));
#117464=CARTESIAN_POINT('Ctrl Pts',(70.7758478045576,-7.41245312484498,
12.));
#117465=CARTESIAN_POINT('Ctrl Pts',(70.796264138335,-7.42157099959326,12.));
#117466=CARTESIAN_POINT('Ctrl Pts',(70.8167134794737,-7.43072843832014,
12.));
#117467=CARTESIAN_POINT('Ctrl Pts',(70.8371956702241,-7.43992544738606,
12.));
#117468=CARTESIAN_POINT('Ctrl Pts',(70.8577105535848,-7.44916203301647,
12.));
#117469=CARTESIAN_POINT('Ctrl Pts',(70.87825797329,-7.45843820129782,12.));
#117470=CARTESIAN_POINT('Ctrl Pts',(70.8988377738104,-7.46775395818527,
12.));
#117471=CARTESIAN_POINT('Ctrl Pts',(70.9194498003493,-7.47710930950562,
12.));
#117472=CARTESIAN_POINT('Ctrl Pts',(70.940093898837,-7.48650426095824,12.));
#117473=CARTESIAN_POINT('Ctrl Pts',(70.9607699159218,-7.4959388181113,12.));
#117474=CARTESIAN_POINT('Ctrl Pts',(70.9814776989612,-7.50541298639928,
12.));
#117475=CARTESIAN_POINT('Ctrl Pts',(71.002217096021,-7.5149267711309,12.));
#117476=CARTESIAN_POINT('Ctrl Pts',(71.0229879558699,-7.52448017749125,
12.));
#117477=CARTESIAN_POINT('Ctrl Pts',(71.043790127973,-7.53407321054262,12.));
#117478=CARTESIAN_POINT('Ctrl Pts',(71.0646234624811,-7.54370587521979,
12.));
#117479=CARTESIAN_POINT('Ctrl Pts',(71.0854878102243,-7.55337817632916,
12.));
#117480=CARTESIAN_POINT('Ctrl Pts',(71.106383022711,-7.56309011855657,12.));
#117481=CARTESIAN_POINT('Ctrl Pts',(71.1273089521234,-7.57284170646886,
12.));
#117482=CARTESIAN_POINT('Ctrl Pts',(71.1482654513119,-7.58263294451452,
12.));
#117483=CARTESIAN_POINT('Ctrl Pts',(71.1692523737844,-7.59246383701814,
12.));
#117484=CARTESIAN_POINT('Ctrl Pts',(71.1902695737013,-7.60233438818096,
12.));
#117485=CARTESIAN_POINT('Ctrl Pts',(71.211316905874,-7.61224460208837,12.));
#117486=CARTESIAN_POINT('Ctrl Pts',(71.2323942257609,-7.62219448271109,
12.));
#117487=CARTESIAN_POINT('Ctrl Pts',(71.2535013894602,-7.63218403390537,
12.));
#117488=CARTESIAN_POINT('Ctrl Pts',(71.2746382537007,-7.64221325940724,
12.));
#117489=CARTESIAN_POINT('Ctrl Pts',(71.2958046758372,-7.65228216283404,
12.));
#117490=CARTESIAN_POINT('Ctrl Pts',(71.3170005138502,-7.66239074769163,
12.));
#117491=CARTESIAN_POINT('Ctrl Pts',(71.3382256263414,-7.67253901737552,
12.));
#117492=CARTESIAN_POINT('Ctrl Pts',(71.3594798725281,-7.68272697517086,
12.));
#117493=CARTESIAN_POINT('Ctrl Pts',(71.3807631122331,-7.69295462424612,
12.));
#117494=CARTESIAN_POINT('Ctrl Pts',(71.4020752058796,-7.70322196765538,
12.));
#117495=CARTESIAN_POINT('Ctrl Pts',(71.4234160144925,-7.7135290083452,12.));
#117496=CARTESIAN_POINT('Ctrl Pts',(71.4447853996916,-7.72387574915544,
12.));
#117497=CARTESIAN_POINT('Ctrl Pts',(71.4661832236888,-7.7342621928194,12.));
#117498=CARTESIAN_POINT('Ctrl Pts',(71.4876093492781,-7.74468834195746,
12.));
#117499=CARTESIAN_POINT('Ctrl Pts',(71.5090636398318,-7.75515419907966,
12.));
#117500=CARTESIAN_POINT('Ctrl Pts',(71.5305459592994,-7.76565976659226,
12.));
#117501=CARTESIAN_POINT('Ctrl Pts',(71.5520561722039,-7.77620504679869,
12.));
#117502=CARTESIAN_POINT('Ctrl Pts',(71.5735941436364,-7.78679004189935,
12.));
#117503=CARTESIAN_POINT('Ctrl Pts',(71.5951597392471,-7.79741475398513,
12.));
#117504=CARTESIAN_POINT('Ctrl Pts',(71.6167528252423,-7.80807918504021,
12.));
#117505=CARTESIAN_POINT('Ctrl Pts',(71.6383732683844,-7.8187833369486,12.));
#117506=CARTESIAN_POINT('Ctrl Pts',(71.6600209359872,-7.82952721149507,
12.));
#117507=CARTESIAN_POINT('Ctrl Pts',(71.6816956959117,-7.84031081036489,
12.));
#117508=CARTESIAN_POINT('Ctrl Pts',(71.7033974165568,-7.85113413513736,
12.));
#117509=CARTESIAN_POINT('Ctrl Pts',(71.7251259668563,-7.86199718728826,
12.));
#117510=CARTESIAN_POINT('Ctrl Pts',(71.7468812162788,-7.87289996819653,
12.));
#117511=CARTESIAN_POINT('Ctrl Pts',(71.7686630348238,-7.88384247914524,
12.));
#117512=CARTESIAN_POINT('Ctrl Pts',(71.7904712930175,-7.89482472132137,
12.));
#117513=CARTESIAN_POINT('Ctrl Pts',(71.8123058619042,-7.90584669580955,
12.));
#117514=CARTESIAN_POINT('Ctrl Pts',(71.8341666130426,-7.91690840359367,
12.));
#117515=CARTESIAN_POINT('Ctrl Pts',(71.8560534185071,-7.92800984556396,
12.));
#117516=CARTESIAN_POINT('Ctrl Pts',(71.8779661508832,-7.93915102251794,
12.));
#117517=CARTESIAN_POINT('Ctrl Pts',(71.8999046832643,-7.9503319351605,12.));
#117518=CARTESIAN_POINT('Ctrl Pts',(71.9218688892431,-7.96155258409763,
12.));
#117519=CARTESIAN_POINT('Ctrl Pts',(71.9438586429081,-7.97281296983718,
12.));
#117520=CARTESIAN_POINT('Ctrl Pts',(71.965873818843,-7.98411309279612,12.));
#117521=CARTESIAN_POINT('Ctrl Pts',(71.9879142921254,-7.99545295330191,
12.));
#117522=CARTESIAN_POINT('Ctrl Pts',(72.0099799383213,-8.00683255159247,
12.));
#117523=CARTESIAN_POINT('Ctrl Pts',(72.032070633479,-8.01825188781056,12.));
#117524=CARTESIAN_POINT('Ctrl Pts',(72.0541862541243,-8.02971096200307,
12.));
#117525=CARTESIAN_POINT('Ctrl Pts',(72.0763266772615,-8.04120977412872,
12.));
#117526=CARTESIAN_POINT('Ctrl Pts',(72.0984917803693,-8.05274832405948,
12.));
#117527=CARTESIAN_POINT('Ctrl Pts',(72.1206814413988,-8.06432661158096,
12.));
#117528=CARTESIAN_POINT('Ctrl Pts',(72.1428955387663,-8.07594463638719,
12.));
#117529=CARTESIAN_POINT('Ctrl Pts',(72.1651339513477,-8.08760239807836,
12.));
#117530=CARTESIAN_POINT('Ctrl Pts',(72.1873965584813,-8.0992998961689,12.));
#117531=CARTESIAN_POINT('Ctrl Pts',(72.209683239963,-8.11103713008928,12.));
#117532=CARTESIAN_POINT('Ctrl Pts',(72.2319938760449,-8.12281409918661,
12.));
#117533=CARTESIAN_POINT('Ctrl Pts',(72.2543283474278,-8.13463080272029,
12.));
#117534=CARTESIAN_POINT('Ctrl Pts',(72.2766865352555,-8.14648723985797,
12.));
#117535=CARTESIAN_POINT('Ctrl Pts',(72.2990683211162,-8.15838340968336,
12.));
#117536=CARTESIAN_POINT('Ctrl Pts',(72.3214735870409,-8.1703193111989,12.));
#117537=CARTESIAN_POINT('Ctrl Pts',(72.3439022155007,-8.18229494332624,
12.));
#117538=CARTESIAN_POINT('Ctrl Pts',(72.3663540894026,-8.19431030490314,
12.));
#117539=CARTESIAN_POINT('Ctrl Pts',(72.3888290920832,-8.20636539467776,
12.));
#117540=CARTESIAN_POINT('Ctrl Pts',(72.4113271073079,-8.21846021131561,
12.));
#117541=CARTESIAN_POINT('Ctrl Pts',(72.4338480192695,-8.23059475340357,
12.));
#117542=CARTESIAN_POINT('Ctrl Pts',(72.4563917125842,-8.2427690194504,12.));
#117543=CARTESIAN_POINT('Ctrl Pts',(72.4789580722875,-8.25498300788493,
12.));
#117544=CARTESIAN_POINT('Ctrl Pts',(72.5015469838254,-8.2672367170492,12.));
#117545=CARTESIAN_POINT('Ctrl Pts',(72.5241583330562,-8.27953014520376,
12.));
#117546=CARTESIAN_POINT('Ctrl Pts',(72.5467920062521,-8.29186329053279,
12.));
#117547=CARTESIAN_POINT('Ctrl Pts',(72.5694478900982,-8.30423615114453,
12.));
#117548=CARTESIAN_POINT('Ctrl Pts',(72.5921258716901,-8.31664872507016,
12.));
#117549=CARTESIAN_POINT('Ctrl Pts',(72.6148258385296,-8.3291010102567,12.));
#117550=CARTESIAN_POINT('Ctrl Pts',(72.6375476785215,-8.34159300456986,
12.));
#117551=CARTESIAN_POINT('Ctrl Pts',(72.6602912799696,-8.35412470580101,
12.));
#117552=CARTESIAN_POINT('Ctrl Pts',(72.6830565315703,-8.36669611166842,
12.));
#117553=CARTESIAN_POINT('Ctrl Pts',(72.705843322407,-8.37930721981731,12.));
#117554=CARTESIAN_POINT('Ctrl Pts',(72.7286515419373,-8.3919580278139,12.));
#117555=CARTESIAN_POINT('Ctrl Pts',(72.751481079992,-8.40464853314468,12.));
#117556=CARTESIAN_POINT('Ctrl Pts',(72.7743318267865,-8.4173787332233,12.));
#117557=CARTESIAN_POINT('Ctrl Pts',(72.7972036729276,-8.43014862539158,
12.));
#117558=CARTESIAN_POINT('Ctrl Pts',(72.8200965094199,-8.44295820691911,
12.));
#117559=CARTESIAN_POINT('Ctrl Pts',(72.8430102276713,-8.45580747499793,
12.));
#117560=CARTESIAN_POINT('Ctrl Pts',(72.8659447194933,-8.46869642673794,
12.));
#117561=CARTESIAN_POINT('Ctrl Pts',(72.8888998770785,-8.48162505917658,
12.));
#117562=CARTESIAN_POINT('Ctrl Pts',(72.9118755929795,-8.49459336928296,
12.));
#117563=CARTESIAN_POINT('Ctrl Pts',(72.9348717600838,-8.50760135395983,
12.));
#117564=CARTESIAN_POINT('Ctrl Pts',(72.9578882715912,-8.52064901004227,
12.));
#117565=CARTESIAN_POINT('Ctrl Pts',(72.9809250209828,-8.53373633429281,
12.));
#117566=CARTESIAN_POINT('Ctrl Pts',(73.0039819020648,-8.54686332340418,
12.));
#117567=CARTESIAN_POINT('Ctrl Pts',(73.0270588090183,-8.56002997400084,
12.));
#117568=CARTESIAN_POINT('Ctrl Pts',(73.0501556364479,-8.57323628263593,
12.));
#117569=CARTESIAN_POINT('Ctrl Pts',(73.0732722794195,-8.58648224578731,
12.));
#117570=CARTESIAN_POINT('Ctrl Pts',(73.0964086335235,-8.59976785984551,
12.));
#117571=CARTESIAN_POINT('Ctrl Pts',(73.1195645948178,-8.61309312112002,
12.));
#117572=CARTESIAN_POINT('Ctrl Pts',(73.1427400597037,-8.62645802585484,
12.));
#117573=CARTESIAN_POINT('Ctrl Pts',(73.1659349248132,-8.63986257023739,
12.));
#117574=CARTESIAN_POINT('Ctrl Pts',(73.1891490869056,-8.65330675040537,
12.));
#117575=CARTESIAN_POINT('Ctrl Pts',(73.2123824427208,-8.66679056245092,
12.));
#117576=CARTESIAN_POINT('Ctrl Pts',(73.2356348889693,-8.68031400241872,
12.));
#117577=CARTESIAN_POINT('Ctrl Pts',(73.2589063226358,-8.69387706629285,
12.));
#117578=CARTESIAN_POINT('Ctrl Pts',(73.2821966412148,-8.70747974998229,
12.));
#117579=CARTESIAN_POINT('Ctrl Pts',(73.3055057429742,-8.72112204930232,
12.));
#117580=CARTESIAN_POINT('Ctrl Pts',(73.3288335272002,-8.7348039599538,12.));
#117581=CARTESIAN_POINT('Ctrl Pts',(73.3521798944622,-8.74852547749778,
12.));
#117582=CARTESIAN_POINT('Ctrl Pts',(73.3755447460269,-8.76228659740357,
12.));
#117583=CARTESIAN_POINT('Ctrl Pts',(73.3989279832835,-8.77608731509348,
12.));
#117584=CARTESIAN_POINT('Ctrl Pts',(73.422329507113,-8.78992762598756,12.));
#117585=CARTESIAN_POINT('Ctrl Pts',(73.4457492173933,-8.80380752553692,
12.));
#117586=CARTESIAN_POINT('Ctrl Pts',(73.4691870121567,-8.8177270092753,12.));
#117587=CARTESIAN_POINT('Ctrl Pts',(73.492642788273,-8.83168607277325,12.));
#117588=CARTESIAN_POINT('Ctrl Pts',(73.5161164429709,-8.84568471153805,
12.));
#117589=CARTESIAN_POINT('Ctrl Pts',(73.5396078751639,-8.8597229209213,12.));
#117590=CARTESIAN_POINT('Ctrl Pts',(73.5631169867122,-8.8738006960297,12.));
#117591=CARTESIAN_POINT('Ctrl Pts',(73.5866436840556,-8.88791803160442,
12.));
#117592=CARTESIAN_POINT('Ctrl Pts',(73.6101878785976,-8.90207492199043,
12.));
#117593=CARTESIAN_POINT('Ctrl Pts',(73.630384739363,-8.91424402151603,12.));
#117594=CARTESIAN_POINT('Ctrl Pts',(73.6458786306025,-8.923595181785,12.));
#117595=CARTESIAN_POINT('Ctrl Pts',(73.6566618622077,-8.9301108881733,12.));
#117596=CARTESIAN_POINT('Ctrl Pts',(73.6627293782591,-8.93377955965654,
12.));
#117597=CARTESIAN_POINT('Ctrl Pts',(73.664078719806,-8.93459554657865,12.));
#117598=CARTESIAN_POINT('',(69.6540253893193,-6.95102489306927,0.));
#117599=CARTESIAN_POINT('',(69.6540253893193,-6.95102489306927,0.));
#117600=CARTESIAN_POINT('Ctrl Pts',(73.6640787198059,-8.93459554657863,
0.));
#117601=CARTESIAN_POINT('Ctrl Pts',(73.6627293782591,-8.93377955965652,
0.));
#117602=CARTESIAN_POINT('Ctrl Pts',(73.6566618622076,-8.93011088817329,
0.));
#117603=CARTESIAN_POINT('Ctrl Pts',(73.6458786306025,-8.92359518178499,
0.));
#117604=CARTESIAN_POINT('Ctrl Pts',(73.630384739363,-8.91424402151603,0.));
#117605=CARTESIAN_POINT('Ctrl Pts',(73.6101878785976,-8.90207492199043,
0.));
#117606=CARTESIAN_POINT('Ctrl Pts',(73.5866436840556,-8.88791803160442,
0.));
#117607=CARTESIAN_POINT('Ctrl Pts',(73.5631169867122,-8.8738006960297,0.));
#117608=CARTESIAN_POINT('Ctrl Pts',(73.5396078751639,-8.8597229209213,0.));
#117609=CARTESIAN_POINT('Ctrl Pts',(73.5161164429709,-8.84568471153805,
0.));
#117610=CARTESIAN_POINT('Ctrl Pts',(73.492642788273,-8.83168607277325,0.));
#117611=CARTESIAN_POINT('Ctrl Pts',(73.4691870121567,-8.8177270092753,0.));
#117612=CARTESIAN_POINT('Ctrl Pts',(73.4457492173933,-8.80380752553692,
0.));
#117613=CARTESIAN_POINT('Ctrl Pts',(73.422329507113,-8.78992762598756,0.));
#117614=CARTESIAN_POINT('Ctrl Pts',(73.3989279832835,-8.77608731509348,
0.));
#117615=CARTESIAN_POINT('Ctrl Pts',(73.3755447460269,-8.76228659740357,
0.));
#117616=CARTESIAN_POINT('Ctrl Pts',(73.3521798944622,-8.74852547749778,
0.));
#117617=CARTESIAN_POINT('Ctrl Pts',(73.3288335272002,-8.7348039599538,0.));
#117618=CARTESIAN_POINT('Ctrl Pts',(73.3055057429742,-8.72112204930232,
0.));
#117619=CARTESIAN_POINT('Ctrl Pts',(73.2821966412148,-8.70747974998229,
0.));
#117620=CARTESIAN_POINT('Ctrl Pts',(73.2589063226358,-8.69387706629285,
0.));
#117621=CARTESIAN_POINT('Ctrl Pts',(73.2356348889693,-8.68031400241872,
0.));
#117622=CARTESIAN_POINT('Ctrl Pts',(73.2123824427208,-8.66679056245092,
0.));
#117623=CARTESIAN_POINT('Ctrl Pts',(73.1891490869056,-8.65330675040537,
0.));
#117624=CARTESIAN_POINT('Ctrl Pts',(73.1659349248132,-8.63986257023739,
0.));
#117625=CARTESIAN_POINT('Ctrl Pts',(73.1427400597037,-8.62645802585484,
0.));
#117626=CARTESIAN_POINT('Ctrl Pts',(73.1195645948178,-8.61309312112002,
0.));
#117627=CARTESIAN_POINT('Ctrl Pts',(73.0964086335235,-8.59976785984551,
0.));
#117628=CARTESIAN_POINT('Ctrl Pts',(73.0732722794195,-8.58648224578731,
0.));
#117629=CARTESIAN_POINT('Ctrl Pts',(73.0501556364479,-8.57323628263593,
0.));
#117630=CARTESIAN_POINT('Ctrl Pts',(73.0270588090183,-8.56002997400084,
0.));
#117631=CARTESIAN_POINT('Ctrl Pts',(73.0039819020648,-8.54686332340418,
0.));
#117632=CARTESIAN_POINT('Ctrl Pts',(72.9809250209828,-8.53373633429281,
0.));
#117633=CARTESIAN_POINT('Ctrl Pts',(72.9578882715912,-8.52064901004227,
0.));
#117634=CARTESIAN_POINT('Ctrl Pts',(72.9348717600838,-8.50760135395983,
0.));
#117635=CARTESIAN_POINT('Ctrl Pts',(72.9118755929795,-8.49459336928296,
0.));
#117636=CARTESIAN_POINT('Ctrl Pts',(72.8888998770785,-8.48162505917658,
0.));
#117637=CARTESIAN_POINT('Ctrl Pts',(72.8659447194933,-8.46869642673794,
0.));
#117638=CARTESIAN_POINT('Ctrl Pts',(72.8430102276713,-8.45580747499793,
0.));
#117639=CARTESIAN_POINT('Ctrl Pts',(72.8200965094199,-8.44295820691911,
0.));
#117640=CARTESIAN_POINT('Ctrl Pts',(72.7972036729276,-8.43014862539158,
0.));
#117641=CARTESIAN_POINT('Ctrl Pts',(72.7743318267865,-8.4173787332233,0.));
#117642=CARTESIAN_POINT('Ctrl Pts',(72.751481079992,-8.40464853314468,0.));
#117643=CARTESIAN_POINT('Ctrl Pts',(72.7286515419373,-8.3919580278139,0.));
#117644=CARTESIAN_POINT('Ctrl Pts',(72.705843322407,-8.37930721981731,0.));
#117645=CARTESIAN_POINT('Ctrl Pts',(72.6830565315703,-8.36669611166842,
0.));
#117646=CARTESIAN_POINT('Ctrl Pts',(72.6602912799696,-8.35412470580101,
0.));
#117647=CARTESIAN_POINT('Ctrl Pts',(72.6375476785215,-8.34159300456986,
0.));
#117648=CARTESIAN_POINT('Ctrl Pts',(72.6148258385296,-8.3291010102567,0.));
#117649=CARTESIAN_POINT('Ctrl Pts',(72.5921258716901,-8.31664872507016,
0.));
#117650=CARTESIAN_POINT('Ctrl Pts',(72.5694478900982,-8.30423615114453,
0.));
#117651=CARTESIAN_POINT('Ctrl Pts',(72.5467920062521,-8.29186329053279,
0.));
#117652=CARTESIAN_POINT('Ctrl Pts',(72.5241583330562,-8.27953014520376,
0.));
#117653=CARTESIAN_POINT('Ctrl Pts',(72.5015469838254,-8.2672367170492,0.));
#117654=CARTESIAN_POINT('Ctrl Pts',(72.4789580722875,-8.25498300788493,
0.));
#117655=CARTESIAN_POINT('Ctrl Pts',(72.4563917125842,-8.2427690194504,0.));
#117656=CARTESIAN_POINT('Ctrl Pts',(72.4338480192695,-8.23059475340357,
0.));
#117657=CARTESIAN_POINT('Ctrl Pts',(72.4113271073079,-8.21846021131561,
0.));
#117658=CARTESIAN_POINT('Ctrl Pts',(72.3888290920832,-8.20636539467776,
0.));
#117659=CARTESIAN_POINT('Ctrl Pts',(72.3663540894026,-8.19431030490314,
0.));
#117660=CARTESIAN_POINT('Ctrl Pts',(72.3439022155007,-8.18229494332624,
0.));
#117661=CARTESIAN_POINT('Ctrl Pts',(72.3214735870409,-8.1703193111989,0.));
#117662=CARTESIAN_POINT('Ctrl Pts',(72.2990683211162,-8.15838340968336,
0.));
#117663=CARTESIAN_POINT('Ctrl Pts',(72.2766865352555,-8.14648723985797,
0.));
#117664=CARTESIAN_POINT('Ctrl Pts',(72.2543283474278,-8.13463080272029,
0.));
#117665=CARTESIAN_POINT('Ctrl Pts',(72.2319938760449,-8.12281409918661,
0.));
#117666=CARTESIAN_POINT('Ctrl Pts',(72.209683239963,-8.11103713008928,0.));
#117667=CARTESIAN_POINT('Ctrl Pts',(72.1873965584813,-8.0992998961689,0.));
#117668=CARTESIAN_POINT('Ctrl Pts',(72.1651339513477,-8.08760239807836,
0.));
#117669=CARTESIAN_POINT('Ctrl Pts',(72.1428955387663,-8.07594463638719,
0.));
#117670=CARTESIAN_POINT('Ctrl Pts',(72.1206814413988,-8.06432661158096,
0.));
#117671=CARTESIAN_POINT('Ctrl Pts',(72.0984917803693,-8.05274832405948,
0.));
#117672=CARTESIAN_POINT('Ctrl Pts',(72.0763266772615,-8.04120977412872,
0.));
#117673=CARTESIAN_POINT('Ctrl Pts',(72.0541862541243,-8.02971096200307,
0.));
#117674=CARTESIAN_POINT('Ctrl Pts',(72.032070633479,-8.01825188781056,0.));
#117675=CARTESIAN_POINT('Ctrl Pts',(72.0099799383213,-8.00683255159247,
0.));
#117676=CARTESIAN_POINT('Ctrl Pts',(71.9879142921254,-7.99545295330191,
0.));
#117677=CARTESIAN_POINT('Ctrl Pts',(71.965873818843,-7.98411309279612,0.));
#117678=CARTESIAN_POINT('Ctrl Pts',(71.9438586429081,-7.97281296983718,
0.));
#117679=CARTESIAN_POINT('Ctrl Pts',(71.9218688892431,-7.96155258409763,
0.));
#117680=CARTESIAN_POINT('Ctrl Pts',(71.8999046832643,-7.9503319351605,0.));
#117681=CARTESIAN_POINT('Ctrl Pts',(71.8779661508832,-7.93915102251794,
0.));
#117682=CARTESIAN_POINT('Ctrl Pts',(71.8560534185071,-7.92800984556396,
0.));
#117683=CARTESIAN_POINT('Ctrl Pts',(71.8341666130426,-7.91690840359367,
0.));
#117684=CARTESIAN_POINT('Ctrl Pts',(71.8123058619042,-7.90584669580955,
0.));
#117685=CARTESIAN_POINT('Ctrl Pts',(71.7904712930175,-7.89482472132137,
0.));
#117686=CARTESIAN_POINT('Ctrl Pts',(71.7686630348238,-7.88384247914524,
0.));
#117687=CARTESIAN_POINT('Ctrl Pts',(71.7468812162788,-7.87289996819653,
0.));
#117688=CARTESIAN_POINT('Ctrl Pts',(71.7251259668563,-7.86199718728826,
0.));
#117689=CARTESIAN_POINT('Ctrl Pts',(71.7033974165568,-7.85113413513736,
0.));
#117690=CARTESIAN_POINT('Ctrl Pts',(71.6816956959117,-7.84031081036489,
0.));
#117691=CARTESIAN_POINT('Ctrl Pts',(71.6600209359872,-7.82952721149507,
0.));
#117692=CARTESIAN_POINT('Ctrl Pts',(71.6383732683844,-7.8187833369486,0.));
#117693=CARTESIAN_POINT('Ctrl Pts',(71.6167528252423,-7.80807918504021,
0.));
#117694=CARTESIAN_POINT('Ctrl Pts',(71.5951597392471,-7.79741475398513,
0.));
#117695=CARTESIAN_POINT('Ctrl Pts',(71.5735941436364,-7.78679004189935,
0.));
#117696=CARTESIAN_POINT('Ctrl Pts',(71.5520561722039,-7.77620504679869,
0.));
#117697=CARTESIAN_POINT('Ctrl Pts',(71.5305459592994,-7.76565976659226,
0.));
#117698=CARTESIAN_POINT('Ctrl Pts',(71.5090636398318,-7.75515419907966,
0.));
#117699=CARTESIAN_POINT('Ctrl Pts',(71.4876093492781,-7.74468834195746,
0.));
#117700=CARTESIAN_POINT('Ctrl Pts',(71.4661832236888,-7.7342621928194,0.));
#117701=CARTESIAN_POINT('Ctrl Pts',(71.4447853996916,-7.72387574915544,
0.));
#117702=CARTESIAN_POINT('Ctrl Pts',(71.4234160144925,-7.7135290083452,0.));
#117703=CARTESIAN_POINT('Ctrl Pts',(71.4020752058796,-7.70322196765538,
0.));
#117704=CARTESIAN_POINT('Ctrl Pts',(71.3807631122331,-7.69295462424612,
0.));
#117705=CARTESIAN_POINT('Ctrl Pts',(71.3594798725281,-7.68272697517086,
0.));
#117706=CARTESIAN_POINT('Ctrl Pts',(71.3382256263414,-7.67253901737552,
0.));
#117707=CARTESIAN_POINT('Ctrl Pts',(71.3170005138502,-7.66239074769163,
0.));
#117708=CARTESIAN_POINT('Ctrl Pts',(71.2958046758372,-7.65228216283404,
0.));
#117709=CARTESIAN_POINT('Ctrl Pts',(71.2746382537007,-7.64221325940724,
0.));
#117710=CARTESIAN_POINT('Ctrl Pts',(71.2535013894602,-7.63218403390537,
0.));
#117711=CARTESIAN_POINT('Ctrl Pts',(71.2323942257609,-7.62219448271109,
0.));
#117712=CARTESIAN_POINT('Ctrl Pts',(71.211316905874,-7.61224460208837,0.));
#117713=CARTESIAN_POINT('Ctrl Pts',(71.1902695737013,-7.60233438818096,
0.));
#117714=CARTESIAN_POINT('Ctrl Pts',(71.1692523737844,-7.59246383701814,
0.));
#117715=CARTESIAN_POINT('Ctrl Pts',(71.1482654513119,-7.58263294451452,
0.));
#117716=CARTESIAN_POINT('Ctrl Pts',(71.1273089521234,-7.57284170646886,
0.));
#117717=CARTESIAN_POINT('Ctrl Pts',(71.106383022711,-7.56309011855657,0.));
#117718=CARTESIAN_POINT('Ctrl Pts',(71.0854878102243,-7.55337817632916,
0.));
#117719=CARTESIAN_POINT('Ctrl Pts',(71.0646234624811,-7.54370587521979,
0.));
#117720=CARTESIAN_POINT('Ctrl Pts',(71.043790127973,-7.53407321054262,0.));
#117721=CARTESIAN_POINT('Ctrl Pts',(71.0229879558699,-7.52448017749125,
0.));
#117722=CARTESIAN_POINT('Ctrl Pts',(71.002217096021,-7.5149267711309,0.));
#117723=CARTESIAN_POINT('Ctrl Pts',(70.9814776989612,-7.50541298639928,
0.));
#117724=CARTESIAN_POINT('Ctrl Pts',(70.9607699159218,-7.4959388181113,0.));
#117725=CARTESIAN_POINT('Ctrl Pts',(70.940093898837,-7.48650426095824,0.));
#117726=CARTESIAN_POINT('Ctrl Pts',(70.9194498003493,-7.47710930950562,
0.));
#117727=CARTESIAN_POINT('Ctrl Pts',(70.8988377738104,-7.46775395818527,
0.));
#117728=CARTESIAN_POINT('Ctrl Pts',(70.87825797329,-7.45843820129782,0.));
#117729=CARTESIAN_POINT('Ctrl Pts',(70.8577105535848,-7.44916203301647,
0.));
#117730=CARTESIAN_POINT('Ctrl Pts',(70.8371956702241,-7.43992544738606,
0.));
#117731=CARTESIAN_POINT('Ctrl Pts',(70.8167134794737,-7.43072843832014,
0.));
#117732=CARTESIAN_POINT('Ctrl Pts',(70.796264138335,-7.42157099959326,0.));
#117733=CARTESIAN_POINT('Ctrl Pts',(70.7758478045576,-7.41245312484498,
0.));
#117734=CARTESIAN_POINT('Ctrl Pts',(70.7554646366514,-7.40337480758237,
0.));
#117735=CARTESIAN_POINT('Ctrl Pts',(70.735114793895,-7.39433604117891,0.));
#117736=CARTESIAN_POINT('Ctrl Pts',(70.7147984363423,-7.38533681887028,
0.));
#117737=CARTESIAN_POINT('Ctrl Pts',(70.6945157248269,-7.37637713374761,
0.));
#117738=CARTESIAN_POINT('Ctrl Pts',(70.6742668209685,-7.36745697876295,
0.));
#117739=CARTESIAN_POINT('Ctrl Pts',(70.6540518871772,-7.35857634673052,
0.));
#117740=CARTESIAN_POINT('Ctrl Pts',(70.6338710866562,-7.3497352303258,0.));
#117741=CARTESIAN_POINT('Ctrl Pts',(70.6137245834002,-7.34093362208018,
0.));
#117742=CARTESIAN_POINT('Ctrl Pts',(70.5936125421958,-7.33217151437608,
0.));
#117743=CARTESIAN_POINT('Ctrl Pts',(70.573535128649,-7.32344889945237,0.));
#117744=CARTESIAN_POINT('Ctrl Pts',(70.5534925092053,-7.31476576940403,
0.));
#117745=CARTESIAN_POINT('Ctrl Pts',(70.5334848511675,-7.30612211618047,
0.));
#117746=CARTESIAN_POINT('Ctrl Pts',(70.5135123227147,-7.29751793157801,
0.));
#117747=CARTESIAN_POINT('Ctrl Pts',(70.4935750929029,-7.28895320723835,
0.));
#117748=CARTESIAN_POINT('Ctrl Pts',(70.4736733316463,-7.28042793465449,
0.));
#117749=CARTESIAN_POINT('Ctrl Pts',(70.4538072096986,-7.27194210517057,
0.));
#117750=CARTESIAN_POINT('Ctrl Pts',(70.433976898636,-7.2634957099805,0.));
#117751=CARTESIAN_POINT('Ctrl Pts',(70.4141825708207,-7.25508874012076,
0.));
#117752=CARTESIAN_POINT('Ctrl Pts',(70.3944243994532,-7.24672118647116,
0.));
#117753=CARTESIAN_POINT('Ctrl Pts',(70.3747025586569,-7.23839303975626,
0.));
#117754=CARTESIAN_POINT('Ctrl Pts',(70.3550172235486,-7.23010429054231,
0.));
#117755=CARTESIAN_POINT('Ctrl Pts',(70.3353685703097,-7.22185492923178,
0.));
#117756=CARTESIAN_POINT('Ctrl Pts',(70.3157567762561,-7.21364494605425,
0.));
#117757=CARTESIAN_POINT('Ctrl Pts',(70.2961820197051,-7.20547433107457,
0.));
#117758=CARTESIAN_POINT('Ctrl Pts',(70.276644479827,-7.19734307419861,0.));
#117759=CARTESIAN_POINT('Ctrl Pts',(70.2571443365198,-7.18925116517562,
0.));
#117760=CARTESIAN_POINT('Ctrl Pts',(70.2376817702239,-7.181198593598,0.));
#117761=CARTESIAN_POINT('Ctrl Pts',(70.2182569619028,-7.17318534889747,
0.));
#117762=CARTESIAN_POINT('Ctrl Pts',(70.1988700934622,-7.16521142033892,
0.));
#117763=CARTESIAN_POINT('Ctrl Pts',(70.1795213481196,-7.15727679700946,
0.));
#117764=CARTESIAN_POINT('Ctrl Pts',(70.1602109107188,-7.14938146780801,
0.));
#117765=CARTESIAN_POINT('Ctrl Pts',(70.1409389682389,-7.14152542142339,
0.));
#117766=CARTESIAN_POINT('Ctrl Pts',(70.1217057094456,-7.13370864634398,
0.));
#117767=CARTESIAN_POINT('Ctrl Pts',(70.1025113239463,-7.12593113088871,
0.));
#117768=CARTESIAN_POINT('Ctrl Pts',(70.0833560013971,-7.11819286322824,
0.));
#117769=CARTESIAN_POINT('Ctrl Pts',(70.06423993069,-7.11049383140482,0.));
#117770=CARTESIAN_POINT('Ctrl Pts',(70.0451632990137,-7.10283402335091,
0.));
#117771=CARTESIAN_POINT('Ctrl Pts',(70.0261262936435,-7.09521342684301,
0.));
#117772=CARTESIAN_POINT('Ctrl Pts',(70.0071291040791,-7.08763202944274,
0.));
#117773=CARTESIAN_POINT('Ctrl Pts',(69.988171923787,-7.08008981844643,0.));
#117774=CARTESIAN_POINT('Ctrl Pts',(69.9692549527256,-7.07258678080793,
0.));
#117775=CARTESIAN_POINT('Ctrl Pts',(69.9503783975676,-7.06512290312803,
0.));
#117776=CARTESIAN_POINT('Ctrl Pts',(69.9315424664252,-7.05769817180824,
0.));
#117777=CARTESIAN_POINT('Ctrl Pts',(69.9127473642087,-7.05031257318108,
0.));
#117778=CARTESIAN_POINT('Ctrl Pts',(69.8939932885864,-7.04296609362187,
0.));
#117779=CARTESIAN_POINT('Ctrl Pts',(69.8752804235296,-7.03565871972265,
0.));
#117780=CARTESIAN_POINT('Ctrl Pts',(69.8566089455448,-7.02839043811863,
0.));
#117781=CARTESIAN_POINT('Ctrl Pts',(69.8379790360574,-7.02116123514487,
0.));
#117782=CARTESIAN_POINT('Ctrl Pts',(69.8193908913722,-7.01397109655455,
0.));
#117783=CARTESIAN_POINT('Ctrl Pts',(69.8008447346782,-7.00682000718105,
0.));
#117784=CARTESIAN_POINT('Ctrl Pts',(69.7823408242446,-6.99970795069399,
0.));
#117785=CARTESIAN_POINT('Ctrl Pts',(69.7638794280263,-6.9926349102786,0.));
#117786=CARTESIAN_POINT('Ctrl Pts',(69.7454607995524,-6.98560086924173,
0.));
#117787=CARTESIAN_POINT('Ctrl Pts',(69.7270851557443,-6.97860581164569,
0.));
#117788=CARTESIAN_POINT('Ctrl Pts',(69.7087526480249,-6.97164972291582,
0.));
#117789=CARTESIAN_POINT('Ctrl Pts',(69.6904633605834,-6.96473259049729,
0.));
#117790=CARTESIAN_POINT('Ctrl Pts',(69.6758665380764,-6.95923004173795,
0.));
#117791=CARTESIAN_POINT('Ctrl Pts',(69.6649383920075,-6.95512065317731,
0.));
#117792=CARTESIAN_POINT('Ctrl Pts',(69.6576616146559,-6.95238884849075,
0.));
#117793=CARTESIAN_POINT('Ctrl Pts',(69.6540253893193,-6.95102489306927,
0.));
#117794=CARTESIAN_POINT('Ctrl Pts',(72.8667204369977,-15.5142209845168,
0.));
#117795=CARTESIAN_POINT('Ctrl Pts',(72.8667204369977,-15.5142209845168,
12.));
#117796=CARTESIAN_POINT('Ctrl Pts',(72.8622377860957,-15.5108715869174,
0.));
#117797=CARTESIAN_POINT('Ctrl Pts',(72.8622377860957,-15.5108715869174,
12.));
#117798=CARTESIAN_POINT('Ctrl Pts',(72.8532737732124,-15.5041768664089,
0.));
#117799=CARTESIAN_POINT('Ctrl Pts',(72.8532737732124,-15.5041768664089,
12.));
#117800=CARTESIAN_POINT('Ctrl Pts',(72.8398316206501,-15.494147009717,0.));
#117801=CARTESIAN_POINT('Ctrl Pts',(72.8398316206501,-15.494147009717,12.));
#117802=CARTESIAN_POINT('Ctrl Pts',(72.8219164844002,-15.4807983165984,
0.));
#117803=CARTESIAN_POINT('Ctrl Pts',(72.8219164844002,-15.4807983165984,
12.));
#117804=CARTESIAN_POINT('Ctrl Pts',(72.7995354604414,-15.4641532053435,
0.));
#117805=CARTESIAN_POINT('Ctrl Pts',(72.7995354604414,-15.4641532053435,
12.));
#117806=CARTESIAN_POINT('Ctrl Pts',(72.7771673494582,-15.4475488590336,
0.));
#117807=CARTESIAN_POINT('Ctrl Pts',(72.7771673494582,-15.4475488590336,
12.));
#117808=CARTESIAN_POINT('Ctrl Pts',(72.7548121825431,-15.4309852897866,
0.));
#117809=CARTESIAN_POINT('Ctrl Pts',(72.7548121825431,-15.4309852897866,
12.));
#117810=CARTESIAN_POINT('Ctrl Pts',(72.7324700089576,-15.4144625111911,
0.));
#117811=CARTESIAN_POINT('Ctrl Pts',(72.7324700089576,-15.4144625111911,
12.));
#117812=CARTESIAN_POINT('Ctrl Pts',(72.710140901746,-15.397980537311,0.));
#117813=CARTESIAN_POINT('Ctrl Pts',(72.710140901746,-15.397980537311,12.));
#117814=CARTESIAN_POINT('Ctrl Pts',(72.6878249557452,-15.3815393822669,
0.));
#117815=CARTESIAN_POINT('Ctrl Pts',(72.6878249557452,-15.3815393822669,
12.));
#117816=CARTESIAN_POINT('Ctrl Pts',(72.6655222797603,-15.3651390602616,
0.));
#117817=CARTESIAN_POINT('Ctrl Pts',(72.6655222797603,-15.3651390602616,
12.));
#117818=CARTESIAN_POINT('Ctrl Pts',(72.6432329903466,-15.3487795854723,
0.));
#117819=CARTESIAN_POINT('Ctrl Pts',(72.6432329903466,-15.3487795854723,
12.));
#117820=CARTESIAN_POINT('Ctrl Pts',(72.6209572051064,-15.3324609719961,
0.));
#117821=CARTESIAN_POINT('Ctrl Pts',(72.6209572051064,-15.3324609719961,
12.));
#117822=CARTESIAN_POINT('Ctrl Pts',(72.5986950357771,-15.3161832337617,
0.));
#117823=CARTESIAN_POINT('Ctrl Pts',(72.5986950357771,-15.3161832337617,
12.));
#117824=CARTESIAN_POINT('Ctrl Pts',(72.5764465826345,-15.2999463844691,
0.));
#117825=CARTESIAN_POINT('Ctrl Pts',(72.5764465826345,-15.2999463844691,
12.));
#117826=CARTESIAN_POINT('Ctrl Pts',(72.5542119383748,-15.2837504376562,
0.));
#117827=CARTESIAN_POINT('Ctrl Pts',(72.5542119383748,-15.2837504376562,
12.));
#117828=CARTESIAN_POINT('Ctrl Pts',(72.5319911908978,-15.2675954067495,
0.));
#117829=CARTESIAN_POINT('Ctrl Pts',(72.5319911908978,-15.2675954067495,
12.));
#117830=CARTESIAN_POINT('Ctrl Pts',(72.5097844266083,-15.2514813051174,
0.));
#117831=CARTESIAN_POINT('Ctrl Pts',(72.5097844266083,-15.2514813051174,
12.));
#117832=CARTESIAN_POINT('Ctrl Pts',(72.4875917332729,-15.2354081461151,
0.));
#117833=CARTESIAN_POINT('Ctrl Pts',(72.4875917332729,-15.2354081461151,
12.));
#117834=CARTESIAN_POINT('Ctrl Pts',(72.4654132036373,-15.2193759431359,
0.));
#117835=CARTESIAN_POINT('Ctrl Pts',(72.4654132036373,-15.2193759431359,
12.));
#117836=CARTESIAN_POINT('Ctrl Pts',(72.4432489350415,-15.2033847096077,
0.));
#117837=CARTESIAN_POINT('Ctrl Pts',(72.4432489350415,-15.2033847096077,
12.));
#117838=CARTESIAN_POINT('Ctrl Pts',(72.4210990277819,-15.1874344589716,
0.));
#117839=CARTESIAN_POINT('Ctrl Pts',(72.4210990277819,-15.1874344589716,
12.));
#117840=CARTESIAN_POINT('Ctrl Pts',(72.3989635838476,-15.1715252046602,
0.));
#117841=CARTESIAN_POINT('Ctrl Pts',(72.3989635838476,-15.1715252046602,
12.));
#117842=CARTESIAN_POINT('Ctrl Pts',(72.37684270559,-15.1556569600747,0.));
#117843=CARTESIAN_POINT('Ctrl Pts',(72.37684270559,-15.1556569600747,12.));
#117844=CARTESIAN_POINT('Ctrl Pts',(72.3547364941996,-15.1398297385513,
0.));
#117845=CARTESIAN_POINT('Ctrl Pts',(72.3547364941996,-15.1398297385513,
12.));
#117846=CARTESIAN_POINT('Ctrl Pts',(72.332645049021,-15.1240435533478,0.));
#117847=CARTESIAN_POINT('Ctrl Pts',(72.332645049021,-15.1240435533478,12.));
#117848=CARTESIAN_POINT('Ctrl Pts',(72.3105684683971,-15.1082984176655,
0.));
#117849=CARTESIAN_POINT('Ctrl Pts',(72.3105684683971,-15.1082984176655,
12.));
#117850=CARTESIAN_POINT('Ctrl Pts',(72.2885068501641,-15.0925943446593,
0.));
#117851=CARTESIAN_POINT('Ctrl Pts',(72.2885068501641,-15.0925943446593,
12.));
#117852=CARTESIAN_POINT('Ctrl Pts',(72.266460292285,-15.0769313474476,0.));
#117853=CARTESIAN_POINT('Ctrl Pts',(72.266460292285,-15.0769313474476,12.));
#117854=CARTESIAN_POINT('Ctrl Pts',(72.244428893425,-15.0613094391186,0.));
#117855=CARTESIAN_POINT('Ctrl Pts',(72.244428893425,-15.0613094391186,12.));
#117856=CARTESIAN_POINT('Ctrl Pts',(72.2224127535401,-15.0457286327328,
0.));
#117857=CARTESIAN_POINT('Ctrl Pts',(72.2224127535401,-15.0457286327328,
12.));
#117858=CARTESIAN_POINT('Ctrl Pts',(72.2004119736104,-15.0301889413255,
0.));
#117859=CARTESIAN_POINT('Ctrl Pts',(72.2004119736104,-15.0301889413255,
12.));
#117860=CARTESIAN_POINT('Ctrl Pts',(72.1784266553948,-15.0146903779061,
0.));
#117861=CARTESIAN_POINT('Ctrl Pts',(72.1784266553948,-15.0146903779061,
12.));
#117862=CARTESIAN_POINT('Ctrl Pts',(72.1564569011668,-14.9992329554537,
0.));
#117863=CARTESIAN_POINT('Ctrl Pts',(72.1564569011668,-14.9992329554537,
12.));
#117864=CARTESIAN_POINT('Ctrl Pts',(72.1345028134779,-14.9838166869107,
0.));
#117865=CARTESIAN_POINT('Ctrl Pts',(72.1345028134779,-14.9838166869107,
12.));
#117866=CARTESIAN_POINT('Ctrl Pts',(72.1125644948547,-14.9684415851699,
0.));
#117867=CARTESIAN_POINT('Ctrl Pts',(72.1125644948547,-14.9684415851699,
12.));
#117868=CARTESIAN_POINT('Ctrl Pts',(72.0906420478085,-14.953107663077,0.));
#117869=CARTESIAN_POINT('Ctrl Pts',(72.0906420478085,-14.953107663077,12.));
#117870=CARTESIAN_POINT('Ctrl Pts',(72.0687355749815,-14.937814933439,0.));
#117871=CARTESIAN_POINT('Ctrl Pts',(72.0687355749815,-14.937814933439,12.));
#117872=CARTESIAN_POINT('Ctrl Pts',(72.046845179251,-14.9225634090269,0.));
#117873=CARTESIAN_POINT('Ctrl Pts',(72.046845179251,-14.9225634090269,12.));
#117874=CARTESIAN_POINT('Ctrl Pts',(72.0249709638419,-14.9073531025763,
0.));
#117875=CARTESIAN_POINT('Ctrl Pts',(72.0249709638419,-14.9073531025763,
12.));
#117876=CARTESIAN_POINT('Ctrl Pts',(72.0031130324519,-14.8921840267829,
0.));
#117877=CARTESIAN_POINT('Ctrl Pts',(72.0031130324519,-14.8921840267829,
12.));
#117878=CARTESIAN_POINT('Ctrl Pts',(71.9812714893087,-14.8770561943011,
0.));
#117879=CARTESIAN_POINT('Ctrl Pts',(71.9812714893087,-14.8770561943011,
12.));
#117880=CARTESIAN_POINT('Ctrl Pts',(71.9594464391063,-14.8619696177503,
0.));
#117881=CARTESIAN_POINT('Ctrl Pts',(71.9594464391063,-14.8619696177503,
12.));
#117882=CARTESIAN_POINT('Ctrl Pts',(71.9376379869668,-14.846924309716,0.));
#117883=CARTESIAN_POINT('Ctrl Pts',(71.9376379869668,-14.846924309716,12.));
#117884=CARTESIAN_POINT('Ctrl Pts',(71.9158462383915,-14.8319202827482,
0.));
#117885=CARTESIAN_POINT('Ctrl Pts',(71.9158462383915,-14.8319202827482,
12.));
#117886=CARTESIAN_POINT('Ctrl Pts',(71.8940712992119,-14.8169575493559,
0.));
#117887=CARTESIAN_POINT('Ctrl Pts',(71.8940712992119,-14.8169575493559,
12.));
#117888=CARTESIAN_POINT('Ctrl Pts',(71.872313275546,-14.8020361220003,0.));
#117889=CARTESIAN_POINT('Ctrl Pts',(71.872313275546,-14.8020361220003,12.));
#117890=CARTESIAN_POINT('Ctrl Pts',(71.8505722738286,-14.7871560131021,
0.));
#117891=CARTESIAN_POINT('Ctrl Pts',(71.8505722738286,-14.7871560131021,
12.));
#117892=CARTESIAN_POINT('Ctrl Pts',(71.8288484008343,-14.7723172350454,
0.));
#117893=CARTESIAN_POINT('Ctrl Pts',(71.8288484008343,-14.7723172350454,
12.));
#117894=CARTESIAN_POINT('Ctrl Pts',(71.8071417637019,-14.7575198001776,
0.));
#117895=CARTESIAN_POINT('Ctrl Pts',(71.8071417637019,-14.7575198001776,
12.));
#117896=CARTESIAN_POINT('Ctrl Pts',(71.7854524699563,-14.7427637208071,
0.));
#117897=CARTESIAN_POINT('Ctrl Pts',(71.7854524699563,-14.7427637208071,
12.));
#117898=CARTESIAN_POINT('Ctrl Pts',(71.7637806275316,-14.7280490091954,
0.));
#117899=CARTESIAN_POINT('Ctrl Pts',(71.7637806275316,-14.7280490091954,
12.));
#117900=CARTESIAN_POINT('Ctrl Pts',(71.7421263447707,-14.7133756775622,
0.));
#117901=CARTESIAN_POINT('Ctrl Pts',(71.7421263447707,-14.7133756775622,
12.));
#117902=CARTESIAN_POINT('Ctrl Pts',(71.7204897304186,-14.6987437380898,
0.));
#117903=CARTESIAN_POINT('Ctrl Pts',(71.7204897304186,-14.6987437380898,
12.));
#117904=CARTESIAN_POINT('Ctrl Pts',(71.698870893617,-14.6841532029231,0.));
#117905=CARTESIAN_POINT('Ctrl Pts',(71.698870893617,-14.6841532029231,12.));
#117906=CARTESIAN_POINT('Ctrl Pts',(71.6772699438966,-14.6696040841679,
0.));
#117907=CARTESIAN_POINT('Ctrl Pts',(71.6772699438966,-14.6696040841679,
12.));
#117908=CARTESIAN_POINT('Ctrl Pts',(71.6556869911669,-14.6550963938832,
0.));
#117909=CARTESIAN_POINT('Ctrl Pts',(71.6556869911669,-14.6550963938832,
12.));
#117910=CARTESIAN_POINT('Ctrl Pts',(71.6341221457175,-14.6406301440817,
0.));
#117911=CARTESIAN_POINT('Ctrl Pts',(71.6341221457175,-14.6406301440817,
12.));
#117912=CARTESIAN_POINT('Ctrl Pts',(71.6125755182295,-14.6262053467372,
0.));
#117913=CARTESIAN_POINT('Ctrl Pts',(71.6125755182295,-14.6262053467372,
12.));
#117914=CARTESIAN_POINT('Ctrl Pts',(71.5910472197815,-14.611822013785,0.));
#117915=CARTESIAN_POINT('Ctrl Pts',(71.5910472197815,-14.611822013785,12.));
#117916=CARTESIAN_POINT('Ctrl Pts',(71.569537361856,-14.597480157121,0.));
#117917=CARTESIAN_POINT('Ctrl Pts',(71.569537361856,-14.597480157121,12.));
#117918=CARTESIAN_POINT('Ctrl Pts',(71.5480460563445,-14.5831797885951,
0.));
#117919=CARTESIAN_POINT('Ctrl Pts',(71.5480460563445,-14.5831797885951,
12.));
#117920=CARTESIAN_POINT('Ctrl Pts',(71.52657341555,-14.568920920009,0.));
#117921=CARTESIAN_POINT('Ctrl Pts',(71.52657341555,-14.568920920009,12.));
#117922=CARTESIAN_POINT('Ctrl Pts',(71.5051195521914,-14.5547035631234,
0.));
#117923=CARTESIAN_POINT('Ctrl Pts',(71.5051195521914,-14.5547035631234,
12.));
#117924=CARTESIAN_POINT('Ctrl Pts',(71.4836845794052,-14.540527729659,0.));
#117925=CARTESIAN_POINT('Ctrl Pts',(71.4836845794052,-14.540527729659,12.));
#117926=CARTESIAN_POINT('Ctrl Pts',(71.4622686107475,-14.5263934312969,
0.));
#117927=CARTESIAN_POINT('Ctrl Pts',(71.4622686107475,-14.5263934312969,
12.));
#117928=CARTESIAN_POINT('Ctrl Pts',(71.4408717601917,-14.5123006796728,
0.));
#117929=CARTESIAN_POINT('Ctrl Pts',(71.4408717601917,-14.5123006796728,
12.));
#117930=CARTESIAN_POINT('Ctrl Pts',(71.4194941421279,-14.4982494863716,
0.));
#117931=CARTESIAN_POINT('Ctrl Pts',(71.4194941421279,-14.4982494863716,
12.));
#117932=CARTESIAN_POINT('Ctrl Pts',(71.398135871371,-14.4842398629353,0.));
#117933=CARTESIAN_POINT('Ctrl Pts',(71.398135871371,-14.4842398629353,12.));
#117934=CARTESIAN_POINT('Ctrl Pts',(71.3767970631642,-14.470271820865,0.));
#117935=CARTESIAN_POINT('Ctrl Pts',(71.3767970631642,-14.470271820865,12.));
#117936=CARTESIAN_POINT('Ctrl Pts',(71.3554778331835,-14.4563453716204,
0.));
#117937=CARTESIAN_POINT('Ctrl Pts',(71.3554778331835,-14.4563453716204,
12.));
#117938=CARTESIAN_POINT('Ctrl Pts',(71.3341782975393,-14.4424605266166,
0.));
#117939=CARTESIAN_POINT('Ctrl Pts',(71.3341782975393,-14.4424605266166,
12.));
#117940=CARTESIAN_POINT('Ctrl Pts',(71.3128985727777,-14.4286172972168,
0.));
#117941=CARTESIAN_POINT('Ctrl Pts',(71.3128985727777,-14.4286172972168,
12.));
#117942=CARTESIAN_POINT('Ctrl Pts',(71.2916387758864,-14.4148156947384,
0.));
#117943=CARTESIAN_POINT('Ctrl Pts',(71.2916387758864,-14.4148156947384,
12.));
#117944=CARTESIAN_POINT('Ctrl Pts',(71.2703990242986,-14.401055730457,0.));
#117945=CARTESIAN_POINT('Ctrl Pts',(71.2703990242986,-14.401055730457,12.));
#117946=CARTESIAN_POINT('Ctrl Pts',(71.2491794358956,-14.3873374156056,
0.));
#117947=CARTESIAN_POINT('Ctrl Pts',(71.2491794358956,-14.3873374156056,
12.));
#117948=CARTESIAN_POINT('Ctrl Pts',(71.2279801290088,-14.3736607613723,
0.));
#117949=CARTESIAN_POINT('Ctrl Pts',(71.2279801290088,-14.3736607613723,
12.));
#117950=CARTESIAN_POINT('Ctrl Pts',(71.2068012224187,-14.3600257788927,
0.));
#117951=CARTESIAN_POINT('Ctrl Pts',(71.2068012224187,-14.3600257788927,
12.));
#117952=CARTESIAN_POINT('Ctrl Pts',(71.185642835361,-14.3464324792537,0.));
#117953=CARTESIAN_POINT('Ctrl Pts',(71.185642835361,-14.3464324792537,12.));
#117954=CARTESIAN_POINT('Ctrl Pts',(71.1645050875323,-14.3328808734993,
0.));
#117955=CARTESIAN_POINT('Ctrl Pts',(71.1645050875323,-14.3328808734993,
12.));
#117956=CARTESIAN_POINT('Ctrl Pts',(71.1433880990932,-14.3193709726295,
0.));
#117957=CARTESIAN_POINT('Ctrl Pts',(71.1433880990932,-14.3193709726295,
12.));
#117958=CARTESIAN_POINT('Ctrl Pts',(71.1222919906718,-14.3059027875993,
0.));
#117959=CARTESIAN_POINT('Ctrl Pts',(71.1222919906718,-14.3059027875993,
12.));
#117960=CARTESIAN_POINT('Ctrl Pts',(71.1012168833626,-14.2924763293101,
0.));
#117961=CARTESIAN_POINT('Ctrl Pts',(71.1012168833626,-14.2924763293101,
12.));
#117962=CARTESIAN_POINT('Ctrl Pts',(71.0801628987314,-14.2790916086129,
0.));
#117963=CARTESIAN_POINT('Ctrl Pts',(71.0801628987314,-14.2790916086129,
12.));
#117964=CARTESIAN_POINT('Ctrl Pts',(71.059130158822,-14.2657486363136,0.));
#117965=CARTESIAN_POINT('Ctrl Pts',(71.059130158822,-14.2657486363136,12.));
#117966=CARTESIAN_POINT('Ctrl Pts',(71.0381187861585,-14.2524474231732,
0.));
#117967=CARTESIAN_POINT('Ctrl Pts',(71.0381187861585,-14.2524474231732,
12.));
#117968=CARTESIAN_POINT('Ctrl Pts',(71.0171289037493,-14.2391879799063,
0.));
#117969=CARTESIAN_POINT('Ctrl Pts',(71.0171289037493,-14.2391879799063,
12.));
#117970=CARTESIAN_POINT('Ctrl Pts',(70.996160635087,-14.2259703171739,0.));
#117971=CARTESIAN_POINT('Ctrl Pts',(70.996160635087,-14.2259703171739,12.));
#117972=CARTESIAN_POINT('Ctrl Pts',(70.9752141041527,-14.2127944455841,
0.));
#117973=CARTESIAN_POINT('Ctrl Pts',(70.9752141041527,-14.2127944455841,
12.));
#117974=CARTESIAN_POINT('Ctrl Pts',(70.9542894354221,-14.1996603756984,
0.));
#117975=CARTESIAN_POINT('Ctrl Pts',(70.9542894354221,-14.1996603756984,
12.));
#117976=CARTESIAN_POINT('Ctrl Pts',(70.9333867538705,-14.1865681180321,
0.));
#117977=CARTESIAN_POINT('Ctrl Pts',(70.9333867538705,-14.1865681180321,
12.));
#117978=CARTESIAN_POINT('Ctrl Pts',(70.9125061849744,-14.1735176830533,
0.));
#117979=CARTESIAN_POINT('Ctrl Pts',(70.9125061849744,-14.1735176830533,
12.));
#117980=CARTESIAN_POINT('Ctrl Pts',(70.8916478547131,-14.1605090811754,
0.));
#117981=CARTESIAN_POINT('Ctrl Pts',(70.8916478547131,-14.1605090811754,
12.));
#117982=CARTESIAN_POINT('Ctrl Pts',(70.8708118895718,-14.1475423227567,
0.));
#117983=CARTESIAN_POINT('Ctrl Pts',(70.8708118895718,-14.1475423227567,
12.));
#117984=CARTESIAN_POINT('Ctrl Pts',(70.8499984165493,-14.1346174181079,
0.));
#117985=CARTESIAN_POINT('Ctrl Pts',(70.8499984165493,-14.1346174181079,
12.));
#117986=CARTESIAN_POINT('Ctrl Pts',(70.8292075631624,-14.1217343774914,
0.));
#117987=CARTESIAN_POINT('Ctrl Pts',(70.8292075631624,-14.1217343774914,
12.));
#117988=CARTESIAN_POINT('Ctrl Pts',(70.8084394574491,-14.1088932111214,
0.));
#117989=CARTESIAN_POINT('Ctrl Pts',(70.8084394574491,-14.1088932111214,
12.));
#117990=CARTESIAN_POINT('Ctrl Pts',(70.787694227969,-14.0960939291568,0.));
#117991=CARTESIAN_POINT('Ctrl Pts',(70.787694227969,-14.0960939291568,12.));
#117992=CARTESIAN_POINT('Ctrl Pts',(70.7669720038067,-14.0833365416995,
0.));
#117993=CARTESIAN_POINT('Ctrl Pts',(70.7669720038067,-14.0833365416995,
12.));
#117994=CARTESIAN_POINT('Ctrl Pts',(70.7462729145799,-14.0706210588015,
0.));
#117995=CARTESIAN_POINT('Ctrl Pts',(70.7462729145799,-14.0706210588015,
12.));
#117996=CARTESIAN_POINT('Ctrl Pts',(70.7255970904433,-14.0579474904657,
0.));
#117997=CARTESIAN_POINT('Ctrl Pts',(70.7255970904433,-14.0579474904657,
12.));
#117998=CARTESIAN_POINT('Ctrl Pts',(70.7049446620931,-14.0453158466451,
0.));
#117999=CARTESIAN_POINT('Ctrl Pts',(70.7049446620931,-14.0453158466451,
12.));
#118000=CARTESIAN_POINT('Ctrl Pts',(70.6843157607672,-14.0327261372363,
0.));
#118001=CARTESIAN_POINT('Ctrl Pts',(70.6843157607672,-14.0327261372363,
12.));
#118002=CARTESIAN_POINT('Ctrl Pts',(70.6637105182487,-14.020178372077,0.));
#118003=CARTESIAN_POINT('Ctrl Pts',(70.6637105182487,-14.020178372077,12.));
#118004=CARTESIAN_POINT('Ctrl Pts',(70.6431290668744,-14.0076725609537,
0.));
#118005=CARTESIAN_POINT('Ctrl Pts',(70.6431290668744,-14.0076725609537,
12.));
#118006=CARTESIAN_POINT('Ctrl Pts',(70.6225715395392,-13.9952087136018,
0.));
#118007=CARTESIAN_POINT('Ctrl Pts',(70.6225715395392,-13.9952087136018,
12.));
#118008=CARTESIAN_POINT('Ctrl Pts',(70.6020380697004,-13.9827868397057,
0.));
#118009=CARTESIAN_POINT('Ctrl Pts',(70.6020380697004,-13.9827868397057,
12.));
#118010=CARTESIAN_POINT('Ctrl Pts',(70.5815287913791,-13.9704069488918,
0.));
#118011=CARTESIAN_POINT('Ctrl Pts',(70.5815287913791,-13.9704069488918,
12.));
#118012=CARTESIAN_POINT('Ctrl Pts',(70.5610438391622,-13.9580690507262,
0.));
#118013=CARTESIAN_POINT('Ctrl Pts',(70.5610438391622,-13.9580690507262,
12.));
#118014=CARTESIAN_POINT('Ctrl Pts',(70.5405833482123,-13.9457731547217,
0.));
#118015=CARTESIAN_POINT('Ctrl Pts',(70.5405833482123,-13.9457731547217,
12.));
#118016=CARTESIAN_POINT('Ctrl Pts',(70.5201474542717,-13.9335192703389,
0.));
#118017=CARTESIAN_POINT('Ctrl Pts',(70.5201474542717,-13.9335192703389,
12.));
#118018=CARTESIAN_POINT('Ctrl Pts',(70.4997362936671,-13.9213074069852,
0.));
#118019=CARTESIAN_POINT('Ctrl Pts',(70.4997362936671,-13.9213074069852,
12.));
#118020=CARTESIAN_POINT('Ctrl Pts',(70.4793500033106,-13.9091375740084,
0.));
#118021=CARTESIAN_POINT('Ctrl Pts',(70.4793500033106,-13.9091375740084,
12.));
#118022=CARTESIAN_POINT('Ctrl Pts',(70.4589887207043,-13.8970097806947,
0.));
#118023=CARTESIAN_POINT('Ctrl Pts',(70.4589887207043,-13.8970097806947,
12.));
#118024=CARTESIAN_POINT('Ctrl Pts',(70.4386525839492,-13.8849240362757,
0.));
#118025=CARTESIAN_POINT('Ctrl Pts',(70.4386525839492,-13.8849240362757,
12.));
#118026=CARTESIAN_POINT('Ctrl Pts',(70.4183417317486,-13.8728803499284,
0.));
#118027=CARTESIAN_POINT('Ctrl Pts',(70.4183417317486,-13.8728803499284,
12.));
#118028=CARTESIAN_POINT('Ctrl Pts',(70.3980563034142,-13.8608787307753,
0.));
#118029=CARTESIAN_POINT('Ctrl Pts',(70.3980563034142,-13.8608787307753,
12.));
#118030=CARTESIAN_POINT('Ctrl Pts',(70.377796438866,-13.8489191878774,0.));
#118031=CARTESIAN_POINT('Ctrl Pts',(70.377796438866,-13.8489191878774,12.));
#118032=CARTESIAN_POINT('Ctrl Pts',(70.3575622786373,-13.8370017302319,
0.));
#118033=CARTESIAN_POINT('Ctrl Pts',(70.3575622786373,-13.8370017302319,
12.));
#118034=CARTESIAN_POINT('Ctrl Pts',(70.3373539638841,-13.8251263667799,
0.));
#118035=CARTESIAN_POINT('Ctrl Pts',(70.3373539638841,-13.8251263667799,
12.));
#118036=CARTESIAN_POINT('Ctrl Pts',(70.3171716363912,-13.8132931064067,
0.));
#118037=CARTESIAN_POINT('Ctrl Pts',(70.3171716363912,-13.8132931064067,
12.));
#118038=CARTESIAN_POINT('Ctrl Pts',(70.2970154385763,-13.8015019579411,
0.));
#118039=CARTESIAN_POINT('Ctrl Pts',(70.2970154385763,-13.8015019579411,
12.));
#118040=CARTESIAN_POINT('Ctrl Pts',(70.2768855134909,-13.7897529301483,
0.));
#118041=CARTESIAN_POINT('Ctrl Pts',(70.2768855134909,-13.7897529301483,
12.));
#118042=CARTESIAN_POINT('Ctrl Pts',(70.2567820048253,-13.7780460317284,
0.));
#118043=CARTESIAN_POINT('Ctrl Pts',(70.2567820048253,-13.7780460317284,
12.));
#118044=CARTESIAN_POINT('Ctrl Pts',(70.2367050569174,-13.7663812713235,
0.));
#118045=CARTESIAN_POINT('Ctrl Pts',(70.2367050569174,-13.7663812713235,
12.));
#118046=CARTESIAN_POINT('Ctrl Pts',(70.216654814759,-13.7547586575178,0.));
#118047=CARTESIAN_POINT('Ctrl Pts',(70.216654814759,-13.7547586575178,12.));
#118048=CARTESIAN_POINT('Ctrl Pts',(70.1966314240012,-13.7431781988368,
0.));
#118049=CARTESIAN_POINT('Ctrl Pts',(70.1966314240012,-13.7431781988368,
12.));
#118050=CARTESIAN_POINT('Ctrl Pts',(70.1766350309554,-13.73163990374,0.));
#118051=CARTESIAN_POINT('Ctrl Pts',(70.1766350309554,-13.73163990374,12.));
#118052=CARTESIAN_POINT('Ctrl Pts',(70.1566657825989,-13.7201437806207,
0.));
#118053=CARTESIAN_POINT('Ctrl Pts',(70.1566657825989,-13.7201437806207,
12.));
#118054=CARTESIAN_POINT('Ctrl Pts',(70.1367238265853,-13.7086898378127,
0.));
#118055=CARTESIAN_POINT('Ctrl Pts',(70.1367238265853,-13.7086898378127,
12.));
#118056=CARTESIAN_POINT('Ctrl Pts',(70.1168093112493,-13.6972780835898,
0.));
#118057=CARTESIAN_POINT('Ctrl Pts',(70.1168093112493,-13.6972780835898,
12.));
#118058=CARTESIAN_POINT('Ctrl Pts',(70.0969223856123,-13.685908526165,0.));
#118059=CARTESIAN_POINT('Ctrl Pts',(70.0969223856123,-13.685908526165,12.));
#118060=CARTESIAN_POINT('Ctrl Pts',(70.0770631993831,-13.6745811736825,
0.));
#118061=CARTESIAN_POINT('Ctrl Pts',(70.0770631993831,-13.6745811736825,
12.));
#118062=CARTESIAN_POINT('Ctrl Pts',(70.057231902965,-13.6632960342192,0.));
#118063=CARTESIAN_POINT('Ctrl Pts',(70.057231902965,-13.6632960342192,12.));
#118064=CARTESIAN_POINT('Ctrl Pts',(70.037428647466,-13.6520531157904,0.));
#118065=CARTESIAN_POINT('Ctrl Pts',(70.037428647466,-13.6520531157904,12.));
#118066=CARTESIAN_POINT('Ctrl Pts',(70.0176535847047,-13.6408524263496,
0.));
#118067=CARTESIAN_POINT('Ctrl Pts',(70.0176535847047,-13.6408524263496,
12.));
#118068=CARTESIAN_POINT('Ctrl Pts',(69.9979068672163,-13.6296939737866,
0.));
#118069=CARTESIAN_POINT('Ctrl Pts',(69.9979068672163,-13.6296939737866,
12.));
#118070=CARTESIAN_POINT('Ctrl Pts',(69.9781886482543,-13.61857776592,0.));
#118071=CARTESIAN_POINT('Ctrl Pts',(69.9781886482543,-13.61857776592,12.));
#118072=CARTESIAN_POINT('Ctrl Pts',(69.9584990817989,-13.6075038105,0.));
#118073=CARTESIAN_POINT('Ctrl Pts',(69.9584990817989,-13.6075038105,12.));
#118074=CARTESIAN_POINT('Ctrl Pts',(69.9388383225655,-13.5964721152136,
0.));
#118075=CARTESIAN_POINT('Ctrl Pts',(69.9388383225655,-13.5964721152136,
12.));
#118076=CARTESIAN_POINT('Ctrl Pts',(69.9192065260107,-13.5854826876834,
0.));
#118077=CARTESIAN_POINT('Ctrl Pts',(69.9192065260107,-13.5854826876834,
12.));
#118078=CARTESIAN_POINT('Ctrl Pts',(69.899603848336,-13.5745355354657,0.));
#118079=CARTESIAN_POINT('Ctrl Pts',(69.899603848336,-13.5745355354657,12.));
#118080=CARTESIAN_POINT('Ctrl Pts',(69.880030446488,-13.5636306660422,0.));
#118081=CARTESIAN_POINT('Ctrl Pts',(69.880030446488,-13.5636306660422,12.));
#118082=CARTESIAN_POINT('Ctrl Pts',(69.8604864781705,-13.5527680868256,
0.));
#118083=CARTESIAN_POINT('Ctrl Pts',(69.8604864781705,-13.5527680868256,
12.));
#118084=CARTESIAN_POINT('Ctrl Pts',(69.840972101856,-13.5419478051626,0.));
#118085=CARTESIAN_POINT('Ctrl Pts',(69.840972101856,-13.5419478051626,12.));
#118086=CARTESIAN_POINT('Ctrl Pts',(69.8214874767944,-13.5311698283339,
0.));
#118087=CARTESIAN_POINT('Ctrl Pts',(69.8214874767944,-13.5311698283339,
12.));
#118088=CARTESIAN_POINT('Ctrl Pts',(69.8020327630204,-13.5204341635507,
0.));
#118089=CARTESIAN_POINT('Ctrl Pts',(69.8020327630204,-13.5204341635507,
12.));
#118090=CARTESIAN_POINT('Ctrl Pts',(69.7826081213575,-13.5097408179478,
0.));
#118091=CARTESIAN_POINT('Ctrl Pts',(69.7826081213575,-13.5097408179478,
12.));
#118092=CARTESIAN_POINT('Ctrl Pts',(69.7632137134247,-13.4990897985904,
0.));
#118093=CARTESIAN_POINT('Ctrl Pts',(69.7632137134247,-13.4990897985904,
12.));
#118094=CARTESIAN_POINT('Ctrl Pts',(69.7438497016404,-13.4884811124748,
0.));
#118095=CARTESIAN_POINT('Ctrl Pts',(69.7438497016404,-13.4884811124748,
12.));
#118096=CARTESIAN_POINT('Ctrl Pts',(69.7245162492251,-13.4779147665285,
0.));
#118097=CARTESIAN_POINT('Ctrl Pts',(69.7245162492251,-13.4779147665285,
12.));
#118098=CARTESIAN_POINT('Ctrl Pts',(69.7052135202003,-13.4673907676045,
0.));
#118099=CARTESIAN_POINT('Ctrl Pts',(69.7052135202003,-13.4673907676045,
12.));
#118100=CARTESIAN_POINT('Ctrl Pts',(69.6859416793898,-13.4569091224762,
0.));
#118101=CARTESIAN_POINT('Ctrl Pts',(69.6859416793898,-13.4569091224762,
12.));
#118102=CARTESIAN_POINT('Ctrl Pts',(69.6667008924454,-13.4464698378456,
0.));
#118103=CARTESIAN_POINT('Ctrl Pts',(69.6667008924454,-13.4464698378456,
12.));
#118104=CARTESIAN_POINT('Ctrl Pts',(69.6474913258684,-13.4360729203444,
0.));
#118105=CARTESIAN_POINT('Ctrl Pts',(69.6474913258684,-13.4360729203444,
12.));
#118106=CARTESIAN_POINT('Ctrl Pts',(69.6283131470267,-13.425718376534,0.));
#118107=CARTESIAN_POINT('Ctrl Pts',(69.6283131470267,-13.425718376534,12.));
#118108=CARTESIAN_POINT('Ctrl Pts',(69.6091665241743,-13.4154062128998,
0.));
#118109=CARTESIAN_POINT('Ctrl Pts',(69.6091665241743,-13.4154062128998,
12.));
#118110=CARTESIAN_POINT('Ctrl Pts',(69.5900516264524,-13.4051364358494,
0.));
#118111=CARTESIAN_POINT('Ctrl Pts',(69.5900516264524,-13.4051364358494,
12.));
#118112=CARTESIAN_POINT('Ctrl Pts',(69.5709686238701,-13.3949090517173,
0.));
#118113=CARTESIAN_POINT('Ctrl Pts',(69.5709686238701,-13.3949090517173,
12.));
#118114=CARTESIAN_POINT('Ctrl Pts',(69.5519176872857,-13.3847240667626,
0.));
#118115=CARTESIAN_POINT('Ctrl Pts',(69.5519176872857,-13.3847240667626,
12.));
#118116=CARTESIAN_POINT('Ctrl Pts',(69.5328989883899,-13.3745814871667,
0.));
#118117=CARTESIAN_POINT('Ctrl Pts',(69.5328989883899,-13.3745814871667,
12.));
#118118=CARTESIAN_POINT('Ctrl Pts',(69.5139126996703,-13.3644813190225,
0.));
#118119=CARTESIAN_POINT('Ctrl Pts',(69.5139126996703,-13.3644813190225,
12.));
#118120=CARTESIAN_POINT('Ctrl Pts',(69.4949589944633,-13.3544235683399,
0.));
#118121=CARTESIAN_POINT('Ctrl Pts',(69.4949589944633,-13.3544235683399,
12.));
#118122=CARTESIAN_POINT('Ctrl Pts',(69.4760380470382,-13.3444082410546,
0.));
#118123=CARTESIAN_POINT('Ctrl Pts',(69.4760380470382,-13.3444082410546,
12.));
#118124=CARTESIAN_POINT('Ctrl Pts',(69.4571500326673,-13.3344353430313,
0.));
#118125=CARTESIAN_POINT('Ctrl Pts',(69.4571500326673,-13.3344353430313,
12.));
#118126=CARTESIAN_POINT('Ctrl Pts',(69.4382951276983,-13.3245048800641,
0.));
#118127=CARTESIAN_POINT('Ctrl Pts',(69.4382951276983,-13.3245048800641,
12.));
#118128=CARTESIAN_POINT('Ctrl Pts',(69.4194735096238,-13.3146168578738,
0.));
#118129=CARTESIAN_POINT('Ctrl Pts',(69.4194735096238,-13.3146168578738,
12.));
#118130=CARTESIAN_POINT('Ctrl Pts',(69.4006853569485,-13.3047712821046,
0.));
#118131=CARTESIAN_POINT('Ctrl Pts',(69.4006853569485,-13.3047712821046,
12.));
#118132=CARTESIAN_POINT('Ctrl Pts',(69.3819308490408,-13.2949681583164,
0.));
#118133=CARTESIAN_POINT('Ctrl Pts',(69.3819308490408,-13.2949681583164,
12.));
#118134=CARTESIAN_POINT('Ctrl Pts',(69.3632101660072,-13.2852074919767,
0.));
#118135=CARTESIAN_POINT('Ctrl Pts',(69.3632101660072,-13.2852074919767,
12.));
#118136=CARTESIAN_POINT('Ctrl Pts',(69.3445234885088,-13.2754892884437,
0.));
#118137=CARTESIAN_POINT('Ctrl Pts',(69.3445234885088,-13.2754892884437,
12.));
#118138=CARTESIAN_POINT('Ctrl Pts',(69.3258709977416,-13.2658135529616,
0.));
#118139=CARTESIAN_POINT('Ctrl Pts',(69.3258709977416,-13.2658135529616,
12.));
#118140=CARTESIAN_POINT('Ctrl Pts',(69.3072528758546,-13.2561802906901,
0.));
#118141=CARTESIAN_POINT('Ctrl Pts',(69.3072528758546,-13.2561802906901,
12.));
#118142=CARTESIAN_POINT('Ctrl Pts',(69.2886693063193,-13.2465895067264,
0.));
#118143=CARTESIAN_POINT('Ctrl Pts',(69.2886693063193,-13.2465895067264,
12.));
#118144=CARTESIAN_POINT('Ctrl Pts',(69.2701204742436,-13.2370412061218,
0.));
#118145=CARTESIAN_POINT('Ctrl Pts',(69.2701204742436,-13.2370412061218,
12.));
#118146=CARTESIAN_POINT('Ctrl Pts',(69.2516065668809,-13.2275353939044,
0.));
#118147=CARTESIAN_POINT('Ctrl Pts',(69.2516065668809,-13.2275353939044,
12.));
#118148=CARTESIAN_POINT('Ctrl Pts',(69.2331277732819,-13.2180720750585,
0.));
#118149=CARTESIAN_POINT('Ctrl Pts',(69.2331277732819,-13.2180720750585,
12.));
#118150=CARTESIAN_POINT('Ctrl Pts',(69.2146842833506,-13.2086512544729,
0.));
#118151=CARTESIAN_POINT('Ctrl Pts',(69.2146842833506,-13.2086512544729,
12.));
#118152=CARTESIAN_POINT('Ctrl Pts',(69.1962762870524,-13.1992729368928,
0.));
#118153=CARTESIAN_POINT('Ctrl Pts',(69.1962762870524,-13.1992729368928,
12.));
#118154=CARTESIAN_POINT('Ctrl Pts',(69.1779039736026,-13.1899371268689,
0.));
#118155=CARTESIAN_POINT('Ctrl Pts',(69.1779039736026,-13.1899371268689,
12.));
#118156=CARTESIAN_POINT('Ctrl Pts',(69.1595675305294,-13.1806438286944,
0.));
#118157=CARTESIAN_POINT('Ctrl Pts',(69.1595675305294,-13.1806438286944,
12.));
#118158=CARTESIAN_POINT('Ctrl Pts',(69.141267145461,-13.1713930465142,0.));
#118159=CARTESIAN_POINT('Ctrl Pts',(69.141267145461,-13.1713930465142,12.));
#118160=CARTESIAN_POINT('Ctrl Pts',(69.1230030082597,-13.1621847844533,
0.));
#118161=CARTESIAN_POINT('Ctrl Pts',(69.1230030082597,-13.1621847844533,
12.));
#118162=CARTESIAN_POINT('Ctrl Pts',(69.1047753127633,-13.1530190467181,
0.));
#118163=CARTESIAN_POINT('Ctrl Pts',(69.1047753127633,-13.1530190467181,
12.));
#118164=CARTESIAN_POINT('Ctrl Pts',(69.0865842593063,-13.1438958377397,
0.));
#118165=CARTESIAN_POINT('Ctrl Pts',(69.0865842593063,-13.1438958377397,
12.));
#118166=CARTESIAN_POINT('Ctrl Pts',(69.0684300549426,-13.1348151621824,
0.));
#118167=CARTESIAN_POINT('Ctrl Pts',(69.0684300549426,-13.1348151621824,
12.));
#118168=CARTESIAN_POINT('Ctrl Pts',(69.0503129081778,-13.1257770246379,
0.));
#118169=CARTESIAN_POINT('Ctrl Pts',(69.0503129081778,-13.1257770246379,
12.));
#118170=CARTESIAN_POINT('Ctrl Pts',(69.0322330243336,-13.1167814293495,
0.));
#118171=CARTESIAN_POINT('Ctrl Pts',(69.0322330243336,-13.1167814293495,
12.));
#118172=CARTESIAN_POINT('Ctrl Pts',(69.0141906015137,-13.1078283799726,
0.));
#118173=CARTESIAN_POINT('Ctrl Pts',(69.0141906015137,-13.1078283799726,
12.));
#118174=CARTESIAN_POINT('Ctrl Pts',(68.9961858241577,-13.0989178791843,
0.));
#118175=CARTESIAN_POINT('Ctrl Pts',(68.9961858241577,-13.0989178791843,
12.));
#118176=CARTESIAN_POINT('Ctrl Pts',(68.9782188692654,-13.0900499290541,
0.));
#118177=CARTESIAN_POINT('Ctrl Pts',(68.9782188692654,-13.0900499290541,
12.));
#118178=CARTESIAN_POINT('Ctrl Pts',(68.9602899187628,-13.0812245317816,
0.));
#118179=CARTESIAN_POINT('Ctrl Pts',(68.9602899187628,-13.0812245317816,
12.));
#118180=CARTESIAN_POINT('Ctrl Pts',(68.9423991694493,-13.072441690283,0.));
#118181=CARTESIAN_POINT('Ctrl Pts',(68.9423991694493,-13.072441690283,12.));
#118182=CARTESIAN_POINT('Ctrl Pts',(68.9245468449865,-13.0637014089018,
0.));
#118183=CARTESIAN_POINT('Ctrl Pts',(68.9245468449865,-13.0637014089018,
12.));
#118184=CARTESIAN_POINT('Ctrl Pts',(68.9067332040842,-13.0550036938793,
0.));
#118185=CARTESIAN_POINT('Ctrl Pts',(68.9067332040842,-13.0550036938793,
12.));
#118186=CARTESIAN_POINT('Ctrl Pts',(68.8889585151431,-13.0463485518185,
0.));
#118187=CARTESIAN_POINT('Ctrl Pts',(68.8889585151431,-13.0463485518185,
12.));
#118188=CARTESIAN_POINT('Ctrl Pts',(68.8712230321823,-13.0377359881864,
0.));
#118189=CARTESIAN_POINT('Ctrl Pts',(68.8712230321823,-13.0377359881864,
12.));
#118190=CARTESIAN_POINT('Ctrl Pts',(68.8535269726871,-13.0291660060118,
0.));
#118191=CARTESIAN_POINT('Ctrl Pts',(68.8535269726871,-13.0291660060118,
12.));
#118192=CARTESIAN_POINT('Ctrl Pts',(68.835870488774,-13.0206386039729,0.));
#118193=CARTESIAN_POINT('Ctrl Pts',(68.835870488774,-13.0206386039729,12.));
#118194=CARTESIAN_POINT('Ctrl Pts',(68.8182536654067,-13.0121537769003,
0.));
#118195=CARTESIAN_POINT('Ctrl Pts',(68.8182536654067,-13.0121537769003,
12.));
#118196=CARTESIAN_POINT('Ctrl Pts',(68.8041919669403,-13.0053999700929,
0.));
#118197=CARTESIAN_POINT('Ctrl Pts',(68.8041919669403,-13.0053999700929,
12.));
#118198=CARTESIAN_POINT('Ctrl Pts',(68.7936635625788,-13.0003537683089,
0.));
#118199=CARTESIAN_POINT('Ctrl Pts',(68.7936635625788,-13.0003537683089,
12.));
#118200=CARTESIAN_POINT('Ctrl Pts',(68.7866525680284,-12.996998146029,0.));
#118201=CARTESIAN_POINT('Ctrl Pts',(68.7866525680284,-12.996998146029,12.));
#118202=CARTESIAN_POINT('Ctrl Pts',(68.7831490561748,-12.9953224629497,
0.));
#118203=CARTESIAN_POINT('Ctrl Pts',(68.7831490561748,-12.9953224629497,
12.));
#118204=CARTESIAN_POINT('',(68.7831490561748,-12.9953224629497,12.));
#118205=CARTESIAN_POINT('Ctrl Pts',(68.7831490561748,-12.9953224629497,
12.));
#118206=CARTESIAN_POINT('Ctrl Pts',(68.7866525680284,-12.996998146029,12.));
#118207=CARTESIAN_POINT('Ctrl Pts',(68.7936635625788,-13.0003537683089,
12.));
#118208=CARTESIAN_POINT('Ctrl Pts',(68.8041919669403,-13.0053999700929,
12.));
#118209=CARTESIAN_POINT('Ctrl Pts',(68.8182536654067,-13.0121537769003,
12.));
#118210=CARTESIAN_POINT('Ctrl Pts',(68.835870488774,-13.0206386039729,12.));
#118211=CARTESIAN_POINT('Ctrl Pts',(68.8535269726871,-13.0291660060118,
12.));
#118212=CARTESIAN_POINT('Ctrl Pts',(68.8712230321823,-13.0377359881864,
12.));
#118213=CARTESIAN_POINT('Ctrl Pts',(68.8889585151431,-13.0463485518185,
12.));
#118214=CARTESIAN_POINT('Ctrl Pts',(68.9067332040842,-13.0550036938793,
12.));
#118215=CARTESIAN_POINT('Ctrl Pts',(68.9245468449865,-13.0637014089018,
12.));
#118216=CARTESIAN_POINT('Ctrl Pts',(68.9423991694493,-13.072441690283,12.));
#118217=CARTESIAN_POINT('Ctrl Pts',(68.9602899187628,-13.0812245317816,
12.));
#118218=CARTESIAN_POINT('Ctrl Pts',(68.9782188692654,-13.0900499290541,
12.));
#118219=CARTESIAN_POINT('Ctrl Pts',(68.9961858241577,-13.0989178791843,
12.));
#118220=CARTESIAN_POINT('Ctrl Pts',(69.0141906015137,-13.1078283799726,
12.));
#118221=CARTESIAN_POINT('Ctrl Pts',(69.0322330243336,-13.1167814293495,
12.));
#118222=CARTESIAN_POINT('Ctrl Pts',(69.0503129081778,-13.1257770246379,
12.));
#118223=CARTESIAN_POINT('Ctrl Pts',(69.0684300549426,-13.1348151621824,
12.));
#118224=CARTESIAN_POINT('Ctrl Pts',(69.0865842593063,-13.1438958377397,
12.));
#118225=CARTESIAN_POINT('Ctrl Pts',(69.1047753127633,-13.1530190467181,
12.));
#118226=CARTESIAN_POINT('Ctrl Pts',(69.1230030082597,-13.1621847844533,
12.));
#118227=CARTESIAN_POINT('Ctrl Pts',(69.141267145461,-13.1713930465142,12.));
#118228=CARTESIAN_POINT('Ctrl Pts',(69.1595675305294,-13.1806438286944,
12.));
#118229=CARTESIAN_POINT('Ctrl Pts',(69.1779039736026,-13.1899371268689,
12.));
#118230=CARTESIAN_POINT('Ctrl Pts',(69.1962762870524,-13.1992729368928,
12.));
#118231=CARTESIAN_POINT('Ctrl Pts',(69.2146842833506,-13.2086512544729,
12.));
#118232=CARTESIAN_POINT('Ctrl Pts',(69.2331277732819,-13.2180720750585,
12.));
#118233=CARTESIAN_POINT('Ctrl Pts',(69.2516065668809,-13.2275353939044,
12.));
#118234=CARTESIAN_POINT('Ctrl Pts',(69.2701204742436,-13.2370412061218,
12.));
#118235=CARTESIAN_POINT('Ctrl Pts',(69.2886693063193,-13.2465895067264,
12.));
#118236=CARTESIAN_POINT('Ctrl Pts',(69.3072528758546,-13.2561802906901,
12.));
#118237=CARTESIAN_POINT('Ctrl Pts',(69.3258709977416,-13.2658135529616,
12.));
#118238=CARTESIAN_POINT('Ctrl Pts',(69.3445234885088,-13.2754892884437,
12.));
#118239=CARTESIAN_POINT('Ctrl Pts',(69.3632101660072,-13.2852074919767,
12.));
#118240=CARTESIAN_POINT('Ctrl Pts',(69.3819308490408,-13.2949681583164,
12.));
#118241=CARTESIAN_POINT('Ctrl Pts',(69.4006853569485,-13.3047712821046,
12.));
#118242=CARTESIAN_POINT('Ctrl Pts',(69.4194735096238,-13.3146168578738,
12.));
#118243=CARTESIAN_POINT('Ctrl Pts',(69.4382951276983,-13.3245048800641,
12.));
#118244=CARTESIAN_POINT('Ctrl Pts',(69.4571500326673,-13.3344353430313,
12.));
#118245=CARTESIAN_POINT('Ctrl Pts',(69.4760380470382,-13.3444082410546,
12.));
#118246=CARTESIAN_POINT('Ctrl Pts',(69.4949589944633,-13.3544235683399,
12.));
#118247=CARTESIAN_POINT('Ctrl Pts',(69.5139126996703,-13.3644813190225,
12.));
#118248=CARTESIAN_POINT('Ctrl Pts',(69.5328989883899,-13.3745814871667,
12.));
#118249=CARTESIAN_POINT('Ctrl Pts',(69.5519176872857,-13.3847240667626,
12.));
#118250=CARTESIAN_POINT('Ctrl Pts',(69.5709686238701,-13.3949090517173,
12.));
#118251=CARTESIAN_POINT('Ctrl Pts',(69.5900516264524,-13.4051364358494,
12.));
#118252=CARTESIAN_POINT('Ctrl Pts',(69.6091665241743,-13.4154062128998,
12.));
#118253=CARTESIAN_POINT('Ctrl Pts',(69.6283131470267,-13.425718376534,12.));
#118254=CARTESIAN_POINT('Ctrl Pts',(69.6474913258684,-13.4360729203444,
12.));
#118255=CARTESIAN_POINT('Ctrl Pts',(69.6667008924454,-13.4464698378456,
12.));
#118256=CARTESIAN_POINT('Ctrl Pts',(69.6859416793898,-13.4569091224762,
12.));
#118257=CARTESIAN_POINT('Ctrl Pts',(69.7052135202003,-13.4673907676045,
12.));
#118258=CARTESIAN_POINT('Ctrl Pts',(69.7245162492251,-13.4779147665285,
12.));
#118259=CARTESIAN_POINT('Ctrl Pts',(69.7438497016404,-13.4884811124748,
12.));
#118260=CARTESIAN_POINT('Ctrl Pts',(69.7632137134247,-13.4990897985904,
12.));
#118261=CARTESIAN_POINT('Ctrl Pts',(69.7826081213575,-13.5097408179478,
12.));
#118262=CARTESIAN_POINT('Ctrl Pts',(69.8020327630204,-13.5204341635507,
12.));
#118263=CARTESIAN_POINT('Ctrl Pts',(69.8214874767944,-13.5311698283339,
12.));
#118264=CARTESIAN_POINT('Ctrl Pts',(69.840972101856,-13.5419478051626,12.));
#118265=CARTESIAN_POINT('Ctrl Pts',(69.8604864781705,-13.5527680868256,
12.));
#118266=CARTESIAN_POINT('Ctrl Pts',(69.880030446488,-13.5636306660422,12.));
#118267=CARTESIAN_POINT('Ctrl Pts',(69.899603848336,-13.5745355354657,12.));
#118268=CARTESIAN_POINT('Ctrl Pts',(69.9192065260107,-13.5854826876834,
12.));
#118269=CARTESIAN_POINT('Ctrl Pts',(69.9388383225655,-13.5964721152136,
12.));
#118270=CARTESIAN_POINT('Ctrl Pts',(69.9584990817989,-13.6075038105,12.));
#118271=CARTESIAN_POINT('Ctrl Pts',(69.9781886482543,-13.61857776592,12.));
#118272=CARTESIAN_POINT('Ctrl Pts',(69.9979068672163,-13.6296939737866,
12.));
#118273=CARTESIAN_POINT('Ctrl Pts',(70.0176535847047,-13.6408524263496,
12.));
#118274=CARTESIAN_POINT('Ctrl Pts',(70.037428647466,-13.6520531157904,12.));
#118275=CARTESIAN_POINT('Ctrl Pts',(70.057231902965,-13.6632960342192,12.));
#118276=CARTESIAN_POINT('Ctrl Pts',(70.0770631993831,-13.6745811736825,
12.));
#118277=CARTESIAN_POINT('Ctrl Pts',(70.0969223856123,-13.685908526165,12.));
#118278=CARTESIAN_POINT('Ctrl Pts',(70.1168093112493,-13.6972780835898,
12.));
#118279=CARTESIAN_POINT('Ctrl Pts',(70.1367238265853,-13.7086898378127,
12.));
#118280=CARTESIAN_POINT('Ctrl Pts',(70.1566657825989,-13.7201437806207,
12.));
#118281=CARTESIAN_POINT('Ctrl Pts',(70.1766350309554,-13.73163990374,12.));
#118282=CARTESIAN_POINT('Ctrl Pts',(70.1966314240012,-13.7431781988368,
12.));
#118283=CARTESIAN_POINT('Ctrl Pts',(70.216654814759,-13.7547586575178,12.));
#118284=CARTESIAN_POINT('Ctrl Pts',(70.2367050569174,-13.7663812713235,
12.));
#118285=CARTESIAN_POINT('Ctrl Pts',(70.2567820048253,-13.7780460317284,
12.));
#118286=CARTESIAN_POINT('Ctrl Pts',(70.2768855134909,-13.7897529301483,
12.));
#118287=CARTESIAN_POINT('Ctrl Pts',(70.2970154385763,-13.8015019579411,
12.));
#118288=CARTESIAN_POINT('Ctrl Pts',(70.3171716363912,-13.8132931064067,
12.));
#118289=CARTESIAN_POINT('Ctrl Pts',(70.3373539638841,-13.8251263667799,
12.));
#118290=CARTESIAN_POINT('Ctrl Pts',(70.3575622786373,-13.8370017302319,
12.));
#118291=CARTESIAN_POINT('Ctrl Pts',(70.377796438866,-13.8489191878774,12.));
#118292=CARTESIAN_POINT('Ctrl Pts',(70.3980563034142,-13.8608787307753,
12.));
#118293=CARTESIAN_POINT('Ctrl Pts',(70.4183417317486,-13.8728803499284,
12.));
#118294=CARTESIAN_POINT('Ctrl Pts',(70.4386525839492,-13.8849240362757,
12.));
#118295=CARTESIAN_POINT('Ctrl Pts',(70.4589887207043,-13.8970097806947,
12.));
#118296=CARTESIAN_POINT('Ctrl Pts',(70.4793500033106,-13.9091375740084,
12.));
#118297=CARTESIAN_POINT('Ctrl Pts',(70.4997362936671,-13.9213074069852,
12.));
#118298=CARTESIAN_POINT('Ctrl Pts',(70.5201474542717,-13.9335192703389,
12.));
#118299=CARTESIAN_POINT('Ctrl Pts',(70.5405833482123,-13.9457731547217,
12.));
#118300=CARTESIAN_POINT('Ctrl Pts',(70.5610438391622,-13.9580690507262,
12.));
#118301=CARTESIAN_POINT('Ctrl Pts',(70.5815287913791,-13.9704069488918,
12.));
#118302=CARTESIAN_POINT('Ctrl Pts',(70.6020380697004,-13.9827868397057,
12.));
#118303=CARTESIAN_POINT('Ctrl Pts',(70.6225715395392,-13.9952087136018,
12.));
#118304=CARTESIAN_POINT('Ctrl Pts',(70.6431290668744,-14.0076725609537,
12.));
#118305=CARTESIAN_POINT('Ctrl Pts',(70.6637105182487,-14.020178372077,12.));
#118306=CARTESIAN_POINT('Ctrl Pts',(70.6843157607672,-14.0327261372363,
12.));
#118307=CARTESIAN_POINT('Ctrl Pts',(70.7049446620931,-14.0453158466451,
12.));
#118308=CARTESIAN_POINT('Ctrl Pts',(70.7255970904433,-14.0579474904657,
12.));
#118309=CARTESIAN_POINT('Ctrl Pts',(70.7462729145799,-14.0706210588015,
12.));
#118310=CARTESIAN_POINT('Ctrl Pts',(70.7669720038067,-14.0833365416995,
12.));
#118311=CARTESIAN_POINT('Ctrl Pts',(70.787694227969,-14.0960939291568,12.));
#118312=CARTESIAN_POINT('Ctrl Pts',(70.8084394574491,-14.1088932111214,
12.));
#118313=CARTESIAN_POINT('Ctrl Pts',(70.8292075631624,-14.1217343774914,
12.));
#118314=CARTESIAN_POINT('Ctrl Pts',(70.8499984165493,-14.1346174181079,
12.));
#118315=CARTESIAN_POINT('Ctrl Pts',(70.8708118895718,-14.1475423227567,
12.));
#118316=CARTESIAN_POINT('Ctrl Pts',(70.8916478547131,-14.1605090811754,
12.));
#118317=CARTESIAN_POINT('Ctrl Pts',(70.9125061849744,-14.1735176830533,
12.));
#118318=CARTESIAN_POINT('Ctrl Pts',(70.9333867538705,-14.1865681180321,
12.));
#118319=CARTESIAN_POINT('Ctrl Pts',(70.9542894354221,-14.1996603756984,
12.));
#118320=CARTESIAN_POINT('Ctrl Pts',(70.9752141041527,-14.2127944455841,
12.));
#118321=CARTESIAN_POINT('Ctrl Pts',(70.996160635087,-14.2259703171739,12.));
#118322=CARTESIAN_POINT('Ctrl Pts',(71.0171289037493,-14.2391879799063,
12.));
#118323=CARTESIAN_POINT('Ctrl Pts',(71.0381187861585,-14.2524474231732,
12.));
#118324=CARTESIAN_POINT('Ctrl Pts',(71.059130158822,-14.2657486363136,12.));
#118325=CARTESIAN_POINT('Ctrl Pts',(71.0801628987314,-14.2790916086129,
12.));
#118326=CARTESIAN_POINT('Ctrl Pts',(71.1012168833626,-14.2924763293101,
12.));
#118327=CARTESIAN_POINT('Ctrl Pts',(71.1222919906718,-14.3059027875993,
12.));
#118328=CARTESIAN_POINT('Ctrl Pts',(71.1433880990932,-14.3193709726295,
12.));
#118329=CARTESIAN_POINT('Ctrl Pts',(71.1645050875323,-14.3328808734993,
12.));
#118330=CARTESIAN_POINT('Ctrl Pts',(71.185642835361,-14.3464324792537,12.));
#118331=CARTESIAN_POINT('Ctrl Pts',(71.2068012224187,-14.3600257788927,
12.));
#118332=CARTESIAN_POINT('Ctrl Pts',(71.2279801290088,-14.3736607613723,
12.));
#118333=CARTESIAN_POINT('Ctrl Pts',(71.2491794358956,-14.3873374156056,
12.));
#118334=CARTESIAN_POINT('Ctrl Pts',(71.2703990242986,-14.401055730457,12.));
#118335=CARTESIAN_POINT('Ctrl Pts',(71.2916387758864,-14.4148156947384,
12.));
#118336=CARTESIAN_POINT('Ctrl Pts',(71.3128985727777,-14.4286172972168,
12.));
#118337=CARTESIAN_POINT('Ctrl Pts',(71.3341782975393,-14.4424605266166,
12.));
#118338=CARTESIAN_POINT('Ctrl Pts',(71.3554778331835,-14.4563453716204,
12.));
#118339=CARTESIAN_POINT('Ctrl Pts',(71.3767970631642,-14.470271820865,12.));
#118340=CARTESIAN_POINT('Ctrl Pts',(71.398135871371,-14.4842398629353,12.));
#118341=CARTESIAN_POINT('Ctrl Pts',(71.4194941421279,-14.4982494863716,
12.));
#118342=CARTESIAN_POINT('Ctrl Pts',(71.4408717601917,-14.5123006796728,
12.));
#118343=CARTESIAN_POINT('Ctrl Pts',(71.4622686107475,-14.5263934312969,
12.));
#118344=CARTESIAN_POINT('Ctrl Pts',(71.4836845794052,-14.540527729659,12.));
#118345=CARTESIAN_POINT('Ctrl Pts',(71.5051195521914,-14.5547035631234,
12.));
#118346=CARTESIAN_POINT('Ctrl Pts',(71.52657341555,-14.568920920009,12.));
#118347=CARTESIAN_POINT('Ctrl Pts',(71.5480460563445,-14.5831797885951,
12.));
#118348=CARTESIAN_POINT('Ctrl Pts',(71.569537361856,-14.597480157121,12.));
#118349=CARTESIAN_POINT('Ctrl Pts',(71.5910472197815,-14.611822013785,12.));
#118350=CARTESIAN_POINT('Ctrl Pts',(71.6125755182295,-14.6262053467372,
12.));
#118351=CARTESIAN_POINT('Ctrl Pts',(71.6341221457175,-14.6406301440817,
12.));
#118352=CARTESIAN_POINT('Ctrl Pts',(71.6556869911669,-14.6550963938832,
12.));
#118353=CARTESIAN_POINT('Ctrl Pts',(71.6772699438966,-14.6696040841679,
12.));
#118354=CARTESIAN_POINT('Ctrl Pts',(71.698870893617,-14.6841532029231,12.));
#118355=CARTESIAN_POINT('Ctrl Pts',(71.7204897304186,-14.6987437380898,
12.));
#118356=CARTESIAN_POINT('Ctrl Pts',(71.7421263447707,-14.7133756775622,
12.));
#118357=CARTESIAN_POINT('Ctrl Pts',(71.7637806275316,-14.7280490091954,
12.));
#118358=CARTESIAN_POINT('Ctrl Pts',(71.7854524699563,-14.7427637208071,
12.));
#118359=CARTESIAN_POINT('Ctrl Pts',(71.8071417637019,-14.7575198001776,
12.));
#118360=CARTESIAN_POINT('Ctrl Pts',(71.8288484008343,-14.7723172350454,
12.));
#118361=CARTESIAN_POINT('Ctrl Pts',(71.8505722738286,-14.7871560131021,
12.));
#118362=CARTESIAN_POINT('Ctrl Pts',(71.872313275546,-14.8020361220003,12.));
#118363=CARTESIAN_POINT('Ctrl Pts',(71.8940712992119,-14.8169575493559,
12.));
#118364=CARTESIAN_POINT('Ctrl Pts',(71.9158462383915,-14.8319202827482,
12.));
#118365=CARTESIAN_POINT('Ctrl Pts',(71.9376379869668,-14.846924309716,12.));
#118366=CARTESIAN_POINT('Ctrl Pts',(71.9594464391063,-14.8619696177503,
12.));
#118367=CARTESIAN_POINT('Ctrl Pts',(71.9812714893087,-14.8770561943011,
12.));
#118368=CARTESIAN_POINT('Ctrl Pts',(72.0031130324519,-14.8921840267829,
12.));
#118369=CARTESIAN_POINT('Ctrl Pts',(72.0249709638419,-14.9073531025763,
12.));
#118370=CARTESIAN_POINT('Ctrl Pts',(72.046845179251,-14.9225634090269,12.));
#118371=CARTESIAN_POINT('Ctrl Pts',(72.0687355749815,-14.937814933439,12.));
#118372=CARTESIAN_POINT('Ctrl Pts',(72.0906420478085,-14.953107663077,12.));
#118373=CARTESIAN_POINT('Ctrl Pts',(72.1125644948547,-14.9684415851699,
12.));
#118374=CARTESIAN_POINT('Ctrl Pts',(72.1345028134779,-14.9838166869107,
12.));
#118375=CARTESIAN_POINT('Ctrl Pts',(72.1564569011668,-14.9992329554537,
12.));
#118376=CARTESIAN_POINT('Ctrl Pts',(72.1784266553948,-15.0146903779061,
12.));
#118377=CARTESIAN_POINT('Ctrl Pts',(72.2004119736104,-15.0301889413255,
12.));
#118378=CARTESIAN_POINT('Ctrl Pts',(72.2224127535401,-15.0457286327328,
12.));
#118379=CARTESIAN_POINT('Ctrl Pts',(72.244428893425,-15.0613094391186,12.));
#118380=CARTESIAN_POINT('Ctrl Pts',(72.266460292285,-15.0769313474476,12.));
#118381=CARTESIAN_POINT('Ctrl Pts',(72.2885068501641,-15.0925943446593,
12.));
#118382=CARTESIAN_POINT('Ctrl Pts',(72.3105684683971,-15.1082984176655,
12.));
#118383=CARTESIAN_POINT('Ctrl Pts',(72.332645049021,-15.1240435533478,12.));
#118384=CARTESIAN_POINT('Ctrl Pts',(72.3547364941996,-15.1398297385513,
12.));
#118385=CARTESIAN_POINT('Ctrl Pts',(72.37684270559,-15.1556569600747,12.));
#118386=CARTESIAN_POINT('Ctrl Pts',(72.3989635838476,-15.1715252046602,
12.));
#118387=CARTESIAN_POINT('Ctrl Pts',(72.4210990277819,-15.1874344589716,
12.));
#118388=CARTESIAN_POINT('Ctrl Pts',(72.4432489350415,-15.2033847096077,
12.));
#118389=CARTESIAN_POINT('Ctrl Pts',(72.4654132036373,-15.2193759431359,
12.));
#118390=CARTESIAN_POINT('Ctrl Pts',(72.4875917332729,-15.2354081461151,
12.));
#118391=CARTESIAN_POINT('Ctrl Pts',(72.5097844266083,-15.2514813051174,
12.));
#118392=CARTESIAN_POINT('Ctrl Pts',(72.5319911908978,-15.2675954067495,
12.));
#118393=CARTESIAN_POINT('Ctrl Pts',(72.5542119383748,-15.2837504376562,
12.));
#118394=CARTESIAN_POINT('Ctrl Pts',(72.5732713370797,-15.2976335024853,
12.));
#118395=CARTESIAN_POINT('Ctrl Pts',(72.5878912620665,-15.3082994603653,
12.));
#118396=CARTESIAN_POINT('Ctrl Pts',(72.59806557899,-15.3157301930834,12.));
#118397=CARTESIAN_POINT('Ctrl Pts',(72.6037902605231,-15.3199137230322,
12.));
#118398=CARTESIAN_POINT('Ctrl Pts',(72.6050633494717,-15.3208442077424,
12.));
#118399=CARTESIAN_POINT('',(68.7831490561748,-12.9953224629497,0.));
#118400=CARTESIAN_POINT('',(68.7831490561748,-12.9953224629497,0.));
#118401=CARTESIAN_POINT('Ctrl Pts',(72.6050633494716,-15.3208442077424,
0.));
#118402=CARTESIAN_POINT('Ctrl Pts',(72.603790260523,-15.3199137230321,0.));
#118403=CARTESIAN_POINT('Ctrl Pts',(72.59806557899,-15.3157301930834,0.));
#118404=CARTESIAN_POINT('Ctrl Pts',(72.5878912620664,-15.3082994603653,
0.));
#118405=CARTESIAN_POINT('Ctrl Pts',(72.5732713370797,-15.2976335024853,
0.));
#118406=CARTESIAN_POINT('Ctrl Pts',(72.5542119383748,-15.2837504376562,
0.));
#118407=CARTESIAN_POINT('Ctrl Pts',(72.5319911908978,-15.2675954067495,
0.));
#118408=CARTESIAN_POINT('Ctrl Pts',(72.5097844266083,-15.2514813051174,
0.));
#118409=CARTESIAN_POINT('Ctrl Pts',(72.4875917332729,-15.2354081461151,
0.));
#118410=CARTESIAN_POINT('Ctrl Pts',(72.4654132036373,-15.2193759431359,
0.));
#118411=CARTESIAN_POINT('Ctrl Pts',(72.4432489350415,-15.2033847096077,
0.));
#118412=CARTESIAN_POINT('Ctrl Pts',(72.4210990277819,-15.1874344589716,
0.));
#118413=CARTESIAN_POINT('Ctrl Pts',(72.3989635838476,-15.1715252046602,
0.));
#118414=CARTESIAN_POINT('Ctrl Pts',(72.37684270559,-15.1556569600747,0.));
#118415=CARTESIAN_POINT('Ctrl Pts',(72.3547364941996,-15.1398297385513,
0.));
#118416=CARTESIAN_POINT('Ctrl Pts',(72.332645049021,-15.1240435533478,0.));
#118417=CARTESIAN_POINT('Ctrl Pts',(72.3105684683971,-15.1082984176655,
0.));
#118418=CARTESIAN_POINT('Ctrl Pts',(72.2885068501641,-15.0925943446593,
0.));
#118419=CARTESIAN_POINT('Ctrl Pts',(72.266460292285,-15.0769313474476,0.));
#118420=CARTESIAN_POINT('Ctrl Pts',(72.244428893425,-15.0613094391186,0.));
#118421=CARTESIAN_POINT('Ctrl Pts',(72.2224127535401,-15.0457286327328,
0.));
#118422=CARTESIAN_POINT('Ctrl Pts',(72.2004119736104,-15.0301889413255,
0.));
#118423=CARTESIAN_POINT('Ctrl Pts',(72.1784266553948,-15.0146903779061,
0.));
#118424=CARTESIAN_POINT('Ctrl Pts',(72.1564569011668,-14.9992329554537,
0.));
#118425=CARTESIAN_POINT('Ctrl Pts',(72.1345028134779,-14.9838166869107,
0.));
#118426=CARTESIAN_POINT('Ctrl Pts',(72.1125644948547,-14.9684415851699,
0.));
#118427=CARTESIAN_POINT('Ctrl Pts',(72.0906420478085,-14.953107663077,0.));
#118428=CARTESIAN_POINT('Ctrl Pts',(72.0687355749815,-14.937814933439,0.));
#118429=CARTESIAN_POINT('Ctrl Pts',(72.046845179251,-14.9225634090269,0.));
#118430=CARTESIAN_POINT('Ctrl Pts',(72.0249709638419,-14.9073531025763,
0.));
#118431=CARTESIAN_POINT('Ctrl Pts',(72.0031130324519,-14.8921840267829,
0.));
#118432=CARTESIAN_POINT('Ctrl Pts',(71.9812714893087,-14.8770561943011,
0.));
#118433=CARTESIAN_POINT('Ctrl Pts',(71.9594464391063,-14.8619696177503,
0.));
#118434=CARTESIAN_POINT('Ctrl Pts',(71.9376379869668,-14.846924309716,0.));
#118435=CARTESIAN_POINT('Ctrl Pts',(71.9158462383915,-14.8319202827482,
0.));
#118436=CARTESIAN_POINT('Ctrl Pts',(71.8940712992119,-14.8169575493559,
0.));
#118437=CARTESIAN_POINT('Ctrl Pts',(71.872313275546,-14.8020361220003,0.));
#118438=CARTESIAN_POINT('Ctrl Pts',(71.8505722738286,-14.7871560131021,
0.));
#118439=CARTESIAN_POINT('Ctrl Pts',(71.8288484008343,-14.7723172350454,
0.));
#118440=CARTESIAN_POINT('Ctrl Pts',(71.8071417637019,-14.7575198001776,
0.));
#118441=CARTESIAN_POINT('Ctrl Pts',(71.7854524699563,-14.7427637208071,
0.));
#118442=CARTESIAN_POINT('Ctrl Pts',(71.7637806275316,-14.7280490091954,
0.));
#118443=CARTESIAN_POINT('Ctrl Pts',(71.7421263447707,-14.7133756775622,
0.));
#118444=CARTESIAN_POINT('Ctrl Pts',(71.7204897304186,-14.6987437380898,
0.));
#118445=CARTESIAN_POINT('Ctrl Pts',(71.698870893617,-14.6841532029231,0.));
#118446=CARTESIAN_POINT('Ctrl Pts',(71.6772699438966,-14.6696040841679,
0.));
#118447=CARTESIAN_POINT('Ctrl Pts',(71.6556869911669,-14.6550963938832,
0.));
#118448=CARTESIAN_POINT('Ctrl Pts',(71.6341221457175,-14.6406301440817,
0.));
#118449=CARTESIAN_POINT('Ctrl Pts',(71.6125755182295,-14.6262053467372,
0.));
#118450=CARTESIAN_POINT('Ctrl Pts',(71.5910472197815,-14.611822013785,0.));
#118451=CARTESIAN_POINT('Ctrl Pts',(71.569537361856,-14.597480157121,0.));
#118452=CARTESIAN_POINT('Ctrl Pts',(71.5480460563445,-14.5831797885951,
0.));
#118453=CARTESIAN_POINT('Ctrl Pts',(71.52657341555,-14.568920920009,0.));
#118454=CARTESIAN_POINT('Ctrl Pts',(71.5051195521914,-14.5547035631234,
0.));
#118455=CARTESIAN_POINT('Ctrl Pts',(71.4836845794052,-14.540527729659,0.));
#118456=CARTESIAN_POINT('Ctrl Pts',(71.4622686107475,-14.5263934312969,
0.));
#118457=CARTESIAN_POINT('Ctrl Pts',(71.4408717601917,-14.5123006796728,
0.));
#118458=CARTESIAN_POINT('Ctrl Pts',(71.4194941421279,-14.4982494863716,
0.));
#118459=CARTESIAN_POINT('Ctrl Pts',(71.398135871371,-14.4842398629353,0.));
#118460=CARTESIAN_POINT('Ctrl Pts',(71.3767970631642,-14.470271820865,0.));
#118461=CARTESIAN_POINT('Ctrl Pts',(71.3554778331835,-14.4563453716204,
0.));
#118462=CARTESIAN_POINT('Ctrl Pts',(71.3341782975393,-14.4424605266166,
0.));
#118463=CARTESIAN_POINT('Ctrl Pts',(71.3128985727777,-14.4286172972168,
0.));
#118464=CARTESIAN_POINT('Ctrl Pts',(71.2916387758864,-14.4148156947384,
0.));
#118465=CARTESIAN_POINT('Ctrl Pts',(71.2703990242986,-14.401055730457,0.));
#118466=CARTESIAN_POINT('Ctrl Pts',(71.2491794358956,-14.3873374156056,
0.));
#118467=CARTESIAN_POINT('Ctrl Pts',(71.2279801290088,-14.3736607613723,
0.));
#118468=CARTESIAN_POINT('Ctrl Pts',(71.2068012224187,-14.3600257788927,
0.));
#118469=CARTESIAN_POINT('Ctrl Pts',(71.185642835361,-14.3464324792537,0.));
#118470=CARTESIAN_POINT('Ctrl Pts',(71.1645050875323,-14.3328808734993,
0.));
#118471=CARTESIAN_POINT('Ctrl Pts',(71.1433880990932,-14.3193709726295,
0.));
#118472=CARTESIAN_POINT('Ctrl Pts',(71.1222919906718,-14.3059027875993,
0.));
#118473=CARTESIAN_POINT('Ctrl Pts',(71.1012168833626,-14.2924763293101,
0.));
#118474=CARTESIAN_POINT('Ctrl Pts',(71.0801628987314,-14.2790916086129,
0.));
#118475=CARTESIAN_POINT('Ctrl Pts',(71.059130158822,-14.2657486363136,0.));
#118476=CARTESIAN_POINT('Ctrl Pts',(71.0381187861585,-14.2524474231732,
0.));
#118477=CARTESIAN_POINT('Ctrl Pts',(71.0171289037493,-14.2391879799063,
0.));
#118478=CARTESIAN_POINT('Ctrl Pts',(70.996160635087,-14.2259703171739,0.));
#118479=CARTESIAN_POINT('Ctrl Pts',(70.9752141041527,-14.2127944455841,
0.));
#118480=CARTESIAN_POINT('Ctrl Pts',(70.9542894354221,-14.1996603756984,
0.));
#118481=CARTESIAN_POINT('Ctrl Pts',(70.9333867538705,-14.1865681180321,
0.));
#118482=CARTESIAN_POINT('Ctrl Pts',(70.9125061849744,-14.1735176830533,
0.));
#118483=CARTESIAN_POINT('Ctrl Pts',(70.8916478547131,-14.1605090811754,
0.));
#118484=CARTESIAN_POINT('Ctrl Pts',(70.8708118895718,-14.1475423227567,
0.));
#118485=CARTESIAN_POINT('Ctrl Pts',(70.8499984165493,-14.1346174181079,
0.));
#118486=CARTESIAN_POINT('Ctrl Pts',(70.8292075631624,-14.1217343774914,
0.));
#118487=CARTESIAN_POINT('Ctrl Pts',(70.8084394574491,-14.1088932111214,
0.));
#118488=CARTESIAN_POINT('Ctrl Pts',(70.787694227969,-14.0960939291568,0.));
#118489=CARTESIAN_POINT('Ctrl Pts',(70.7669720038067,-14.0833365416995,
0.));
#118490=CARTESIAN_POINT('Ctrl Pts',(70.7462729145799,-14.0706210588015,
0.));
#118491=CARTESIAN_POINT('Ctrl Pts',(70.7255970904433,-14.0579474904657,
0.));
#118492=CARTESIAN_POINT('Ctrl Pts',(70.7049446620931,-14.0453158466451,
0.));
#118493=CARTESIAN_POINT('Ctrl Pts',(70.6843157607672,-14.0327261372363,
0.));
#118494=CARTESIAN_POINT('Ctrl Pts',(70.6637105182487,-14.020178372077,0.));
#118495=CARTESIAN_POINT('Ctrl Pts',(70.6431290668744,-14.0076725609537,
0.));
#118496=CARTESIAN_POINT('Ctrl Pts',(70.6225715395392,-13.9952087136018,
0.));
#118497=CARTESIAN_POINT('Ctrl Pts',(70.6020380697004,-13.9827868397057,
0.));
#118498=CARTESIAN_POINT('Ctrl Pts',(70.5815287913791,-13.9704069488918,
0.));
#118499=CARTESIAN_POINT('Ctrl Pts',(70.5610438391622,-13.9580690507262,
0.));
#118500=CARTESIAN_POINT('Ctrl Pts',(70.5405833482123,-13.9457731547217,
0.));
#118501=CARTESIAN_POINT('Ctrl Pts',(70.5201474542717,-13.9335192703389,
0.));
#118502=CARTESIAN_POINT('Ctrl Pts',(70.4997362936671,-13.9213074069852,
0.));
#118503=CARTESIAN_POINT('Ctrl Pts',(70.4793500033106,-13.9091375740084,
0.));
#118504=CARTESIAN_POINT('Ctrl Pts',(70.4589887207043,-13.8970097806947,
0.));
#118505=CARTESIAN_POINT('Ctrl Pts',(70.4386525839492,-13.8849240362757,
0.));
#118506=CARTESIAN_POINT('Ctrl Pts',(70.4183417317486,-13.8728803499284,
0.));
#118507=CARTESIAN_POINT('Ctrl Pts',(70.3980563034142,-13.8608787307753,
0.));
#118508=CARTESIAN_POINT('Ctrl Pts',(70.377796438866,-13.8489191878774,0.));
#118509=CARTESIAN_POINT('Ctrl Pts',(70.3575622786373,-13.8370017302319,
0.));
#118510=CARTESIAN_POINT('Ctrl Pts',(70.3373539638841,-13.8251263667799,
0.));
#118511=CARTESIAN_POINT('Ctrl Pts',(70.3171716363912,-13.8132931064067,
0.));
#118512=CARTESIAN_POINT('Ctrl Pts',(70.2970154385763,-13.8015019579411,
0.));
#118513=CARTESIAN_POINT('Ctrl Pts',(70.2768855134909,-13.7897529301483,
0.));
#118514=CARTESIAN_POINT('Ctrl Pts',(70.2567820048253,-13.7780460317284,
0.));
#118515=CARTESIAN_POINT('Ctrl Pts',(70.2367050569174,-13.7663812713235,
0.));
#118516=CARTESIAN_POINT('Ctrl Pts',(70.216654814759,-13.7547586575178,0.));
#118517=CARTESIAN_POINT('Ctrl Pts',(70.1966314240012,-13.7431781988368,
0.));
#118518=CARTESIAN_POINT('Ctrl Pts',(70.1766350309554,-13.73163990374,0.));
#118519=CARTESIAN_POINT('Ctrl Pts',(70.1566657825989,-13.7201437806207,
0.));
#118520=CARTESIAN_POINT('Ctrl Pts',(70.1367238265853,-13.7086898378127,
0.));
#118521=CARTESIAN_POINT('Ctrl Pts',(70.1168093112493,-13.6972780835898,
0.));
#118522=CARTESIAN_POINT('Ctrl Pts',(70.0969223856123,-13.685908526165,0.));
#118523=CARTESIAN_POINT('Ctrl Pts',(70.0770631993831,-13.6745811736825,
0.));
#118524=CARTESIAN_POINT('Ctrl Pts',(70.057231902965,-13.6632960342192,0.));
#118525=CARTESIAN_POINT('Ctrl Pts',(70.037428647466,-13.6520531157904,0.));
#118526=CARTESIAN_POINT('Ctrl Pts',(70.0176535847047,-13.6408524263496,
0.));
#118527=CARTESIAN_POINT('Ctrl Pts',(69.9979068672163,-13.6296939737866,
0.));
#118528=CARTESIAN_POINT('Ctrl Pts',(69.9781886482543,-13.61857776592,0.));
#118529=CARTESIAN_POINT('Ctrl Pts',(69.9584990817989,-13.6075038105,0.));
#118530=CARTESIAN_POINT('Ctrl Pts',(69.9388383225655,-13.5964721152136,
0.));
#118531=CARTESIAN_POINT('Ctrl Pts',(69.9192065260107,-13.5854826876834,
0.));
#118532=CARTESIAN_POINT('Ctrl Pts',(69.899603848336,-13.5745355354657,0.));
#118533=CARTESIAN_POINT('Ctrl Pts',(69.880030446488,-13.5636306660422,0.));
#118534=CARTESIAN_POINT('Ctrl Pts',(69.8604864781705,-13.5527680868256,
0.));
#118535=CARTESIAN_POINT('Ctrl Pts',(69.840972101856,-13.5419478051626,0.));
#118536=CARTESIAN_POINT('Ctrl Pts',(69.8214874767944,-13.5311698283339,
0.));
#118537=CARTESIAN_POINT('Ctrl Pts',(69.8020327630204,-13.5204341635507,
0.));
#118538=CARTESIAN_POINT('Ctrl Pts',(69.7826081213575,-13.5097408179478,
0.));
#118539=CARTESIAN_POINT('Ctrl Pts',(69.7632137134247,-13.4990897985904,
0.));
#118540=CARTESIAN_POINT('Ctrl Pts',(69.7438497016404,-13.4884811124748,
0.));
#118541=CARTESIAN_POINT('Ctrl Pts',(69.7245162492251,-13.4779147665285,
0.));
#118542=CARTESIAN_POINT('Ctrl Pts',(69.7052135202003,-13.4673907676045,
0.));
#118543=CARTESIAN_POINT('Ctrl Pts',(69.6859416793898,-13.4569091224762,
0.));
#118544=CARTESIAN_POINT('Ctrl Pts',(69.6667008924454,-13.4464698378456,
0.));
#118545=CARTESIAN_POINT('Ctrl Pts',(69.6474913258684,-13.4360729203444,
0.));
#118546=CARTESIAN_POINT('Ctrl Pts',(69.6283131470267,-13.425718376534,0.));
#118547=CARTESIAN_POINT('Ctrl Pts',(69.6091665241743,-13.4154062128998,
0.));
#118548=CARTESIAN_POINT('Ctrl Pts',(69.5900516264524,-13.4051364358494,
0.));
#118549=CARTESIAN_POINT('Ctrl Pts',(69.5709686238701,-13.3949090517173,
0.));
#118550=CARTESIAN_POINT('Ctrl Pts',(69.5519176872857,-13.3847240667626,
0.));
#118551=CARTESIAN_POINT('Ctrl Pts',(69.5328989883899,-13.3745814871667,
0.));
#118552=CARTESIAN_POINT('Ctrl Pts',(69.5139126996703,-13.3644813190225,
0.));
#118553=CARTESIAN_POINT('Ctrl Pts',(69.4949589944633,-13.3544235683399,
0.));
#118554=CARTESIAN_POINT('Ctrl Pts',(69.4760380470382,-13.3444082410546,
0.));
#118555=CARTESIAN_POINT('Ctrl Pts',(69.4571500326673,-13.3344353430313,
0.));
#118556=CARTESIAN_POINT('Ctrl Pts',(69.4382951276983,-13.3245048800641,
0.));
#118557=CARTESIAN_POINT('Ctrl Pts',(69.4194735096238,-13.3146168578738,
0.));
#118558=CARTESIAN_POINT('Ctrl Pts',(69.4006853569485,-13.3047712821046,
0.));
#118559=CARTESIAN_POINT('Ctrl Pts',(69.3819308490408,-13.2949681583164,
0.));
#118560=CARTESIAN_POINT('Ctrl Pts',(69.3632101660072,-13.2852074919767,
0.));
#118561=CARTESIAN_POINT('Ctrl Pts',(69.3445234885088,-13.2754892884437,
0.));
#118562=CARTESIAN_POINT('Ctrl Pts',(69.3258709977416,-13.2658135529616,
0.));
#118563=CARTESIAN_POINT('Ctrl Pts',(69.3072528758546,-13.2561802906901,
0.));
#118564=CARTESIAN_POINT('Ctrl Pts',(69.2886693063193,-13.2465895067264,
0.));
#118565=CARTESIAN_POINT('Ctrl Pts',(69.2701204742436,-13.2370412061218,
0.));
#118566=CARTESIAN_POINT('Ctrl Pts',(69.2516065668809,-13.2275353939044,
0.));
#118567=CARTESIAN_POINT('Ctrl Pts',(69.2331277732819,-13.2180720750585,
0.));
#118568=CARTESIAN_POINT('Ctrl Pts',(69.2146842833506,-13.2086512544729,
0.));
#118569=CARTESIAN_POINT('Ctrl Pts',(69.1962762870524,-13.1992729368928,
0.));
#118570=CARTESIAN_POINT('Ctrl Pts',(69.1779039736026,-13.1899371268689,
0.));
#118571=CARTESIAN_POINT('Ctrl Pts',(69.1595675305294,-13.1806438286944,
0.));
#118572=CARTESIAN_POINT('Ctrl Pts',(69.141267145461,-13.1713930465142,0.));
#118573=CARTESIAN_POINT('Ctrl Pts',(69.1230030082597,-13.1621847844533,
0.));
#118574=CARTESIAN_POINT('Ctrl Pts',(69.1047753127633,-13.1530190467181,
0.));
#118575=CARTESIAN_POINT('Ctrl Pts',(69.0865842593063,-13.1438958377397,
0.));
#118576=CARTESIAN_POINT('Ctrl Pts',(69.0684300549426,-13.1348151621824,
0.));
#118577=CARTESIAN_POINT('Ctrl Pts',(69.0503129081778,-13.1257770246379,
0.));
#118578=CARTESIAN_POINT('Ctrl Pts',(69.0322330243336,-13.1167814293495,
0.));
#118579=CARTESIAN_POINT('Ctrl Pts',(69.0141906015137,-13.1078283799726,
0.));
#118580=CARTESIAN_POINT('Ctrl Pts',(68.9961858241577,-13.0989178791843,
0.));
#118581=CARTESIAN_POINT('Ctrl Pts',(68.9782188692654,-13.0900499290541,
0.));
#118582=CARTESIAN_POINT('Ctrl Pts',(68.9602899187628,-13.0812245317816,
0.));
#118583=CARTESIAN_POINT('Ctrl Pts',(68.9423991694493,-13.072441690283,0.));
#118584=CARTESIAN_POINT('Ctrl Pts',(68.9245468449865,-13.0637014089018,
0.));
#118585=CARTESIAN_POINT('Ctrl Pts',(68.9067332040842,-13.0550036938793,
0.));
#118586=CARTESIAN_POINT('Ctrl Pts',(68.8889585151431,-13.0463485518185,
0.));
#118587=CARTESIAN_POINT('Ctrl Pts',(68.8712230321823,-13.0377359881864,
0.));
#118588=CARTESIAN_POINT('Ctrl Pts',(68.8535269726871,-13.0291660060118,
0.));
#118589=CARTESIAN_POINT('Ctrl Pts',(68.835870488774,-13.0206386039729,0.));
#118590=CARTESIAN_POINT('Ctrl Pts',(68.8182536654067,-13.0121537769003,
0.));
#118591=CARTESIAN_POINT('Ctrl Pts',(68.8041919669403,-13.0053999700929,
0.));
#118592=CARTESIAN_POINT('Ctrl Pts',(68.7936635625788,-13.0003537683089,
0.));
#118593=CARTESIAN_POINT('Ctrl Pts',(68.7866525680284,-12.996998146029,0.));
#118594=CARTESIAN_POINT('Ctrl Pts',(68.7831490561748,-12.9953224629497,
0.));
#118595=CARTESIAN_POINT('Ctrl Pts',(71.2372871136136,-21.8059378310719,
0.));
#118596=CARTESIAN_POINT('Ctrl Pts',(71.2372871136136,-21.8059378310719,
12.));
#118597=CARTESIAN_POINT('Ctrl Pts',(71.2331134397872,-21.8022104901727,
0.));
#118598=CARTESIAN_POINT('Ctrl Pts',(71.2331134397872,-21.8022104901727,
12.));
#118599=CARTESIAN_POINT('Ctrl Pts',(71.2247670210176,-21.7947599798961,
0.));
#118600=CARTESIAN_POINT('Ctrl Pts',(71.2247670210176,-21.7947599798961,
12.));
#118601=CARTESIAN_POINT('Ctrl Pts',(71.2122501795138,-21.7835967290463,
0.));
#118602=CARTESIAN_POINT('Ctrl Pts',(71.2122501795138,-21.7835967290463,
12.));
#118603=CARTESIAN_POINT('Ctrl Pts',(71.1955666310295,-21.7687374247288,
0.));
#118604=CARTESIAN_POINT('Ctrl Pts',(71.1955666310295,-21.7687374247288,
12.));
#118605=CARTESIAN_POINT('Ctrl Pts',(71.1747214906585,-21.750205018381,0.));
#118606=CARTESIAN_POINT('Ctrl Pts',(71.1747214906585,-21.750205018381,12.));
#118607=CARTESIAN_POINT('Ctrl Pts',(71.1538856612261,-21.7317143472952,
0.));
#118608=CARTESIAN_POINT('Ctrl Pts',(71.1538856612261,-21.7317143472952,
12.));
#118609=CARTESIAN_POINT('Ctrl Pts',(71.1330591726506,-21.7132654262531,
0.));
#118610=CARTESIAN_POINT('Ctrl Pts',(71.1330591726506,-21.7132654262531,
12.));
#118611=CARTESIAN_POINT('Ctrl Pts',(71.1122420728216,-21.694858273085,0.));
#118612=CARTESIAN_POINT('Ctrl Pts',(71.1122420728216,-21.694858273085,12.));
#118613=CARTESIAN_POINT('Ctrl Pts',(71.0914344332798,-21.6764929081677,
0.));
#118614=CARTESIAN_POINT('Ctrl Pts',(71.0914344332798,-21.6764929081677,
12.));
#118615=CARTESIAN_POINT('Ctrl Pts',(71.0706363472704,-21.6581693538335,
0.));
#118616=CARTESIAN_POINT('Ctrl Pts',(71.0706363472704,-21.6581693538335,
12.));
#118617=CARTESIAN_POINT('Ctrl Pts',(71.0498479219467,-21.6398876337141,
0.));
#118618=CARTESIAN_POINT('Ctrl Pts',(71.0498479219467,-21.6398876337141,
12.));
#118619=CARTESIAN_POINT('Ctrl Pts',(71.0290692721847,-21.6216477720913,
0.));
#118620=CARTESIAN_POINT('Ctrl Pts',(71.0290692721847,-21.6216477720913,
12.));
#118621=CARTESIAN_POINT('Ctrl Pts',(71.0083005139107,-21.6034497932581,
0.));
#118622=CARTESIAN_POINT('Ctrl Pts',(71.0083005139107,-21.6034497932581,
12.));
#118623=CARTESIAN_POINT('Ctrl Pts',(70.987541757223,-21.585293720829,0.));
#118624=CARTESIAN_POINT('Ctrl Pts',(70.987541757223,-21.585293720829,12.));
#118625=CARTESIAN_POINT('Ctrl Pts',(70.9667931008215,-21.5671795771914,
0.));
#118626=CARTESIAN_POINT('Ctrl Pts',(70.9667931008215,-21.5671795771914,
12.));
#118627=CARTESIAN_POINT('Ctrl Pts',(70.94605463587,-21.5491073839106,0.));
#118628=CARTESIAN_POINT('Ctrl Pts',(70.94605463587,-21.5491073839106,12.));
#118629=CARTESIAN_POINT('Ctrl Pts',(70.9253264487636,-21.5310771620231,
0.));
#118630=CARTESIAN_POINT('Ctrl Pts',(70.9253264487636,-21.5310771620231,
12.));
#118631=CARTESIAN_POINT('Ctrl Pts',(70.9046086244131,-21.513088932377,0.));
#118632=CARTESIAN_POINT('Ctrl Pts',(70.9046086244131,-21.513088932377,12.));
#118633=CARTESIAN_POINT('Ctrl Pts',(70.8839012490871,-21.4951427159262,
0.));
#118634=CARTESIAN_POINT('Ctrl Pts',(70.8839012490871,-21.4951427159262,
12.));
#118635=CARTESIAN_POINT('Ctrl Pts',(70.8632044140112,-21.477238534096,0.));
#118636=CARTESIAN_POINT('Ctrl Pts',(70.8632044140112,-21.477238534096,12.));
#118637=CARTESIAN_POINT('Ctrl Pts',(70.8425182149846,-21.4593764087474,
0.));
#118638=CARTESIAN_POINT('Ctrl Pts',(70.8425182149846,-21.4593764087474,
12.));
#118639=CARTESIAN_POINT('Ctrl Pts',(70.8218427507506,-21.4415563620114,
0.));
#118640=CARTESIAN_POINT('Ctrl Pts',(70.8218427507506,-21.4415563620114,
12.));
#118641=CARTESIAN_POINT('Ctrl Pts',(70.8011781217394,-21.4237784161588,
0.));
#118642=CARTESIAN_POINT('Ctrl Pts',(70.8011781217394,-21.4237784161588,
12.));
#118643=CARTESIAN_POINT('Ctrl Pts',(70.780524428745,-21.4060425934599,0.));
#118644=CARTESIAN_POINT('Ctrl Pts',(70.780524428745,-21.4060425934599,12.));
#118645=CARTESIAN_POINT('Ctrl Pts',(70.7598817714105,-21.3883489160196,
0.));
#118646=CARTESIAN_POINT('Ctrl Pts',(70.7598817714105,-21.3883489160196,
12.));
#118647=CARTESIAN_POINT('Ctrl Pts',(70.7392502475469,-21.3706974057039,
0.));
#118648=CARTESIAN_POINT('Ctrl Pts',(70.7392502475469,-21.3706974057039,
12.));
#118649=CARTESIAN_POINT('Ctrl Pts',(70.7186299539724,-21.3530880842349,
0.));
#118650=CARTESIAN_POINT('Ctrl Pts',(70.7186299539724,-21.3530880842349,
12.));
#118651=CARTESIAN_POINT('Ctrl Pts',(70.6980209870044,-21.3355209732443,
0.));
#118652=CARTESIAN_POINT('Ctrl Pts',(70.6980209870044,-21.3355209732443,
12.));
#118653=CARTESIAN_POINT('Ctrl Pts',(70.6774234430897,-21.3179960943389,
0.));
#118654=CARTESIAN_POINT('Ctrl Pts',(70.6774234430897,-21.3179960943389,
12.));
#118655=CARTESIAN_POINT('Ctrl Pts',(70.6568374193774,-21.300513469156,0.));
#118656=CARTESIAN_POINT('Ctrl Pts',(70.6568374193774,-21.300513469156,12.));
#118657=CARTESIAN_POINT('Ctrl Pts',(70.6362630143047,-21.2830731194183,
0.));
#118658=CARTESIAN_POINT('Ctrl Pts',(70.6362630143047,-21.2830731194183,
12.));
#118659=CARTESIAN_POINT('Ctrl Pts',(70.6157003273316,-21.2656750669126,
0.));
#118660=CARTESIAN_POINT('Ctrl Pts',(70.6157003273316,-21.2656750669126,
12.));
#118661=CARTESIAN_POINT('Ctrl Pts',(70.5951494586957,-21.2483193334676,
0.));
#118662=CARTESIAN_POINT('Ctrl Pts',(70.5951494586957,-21.2483193334676,
12.));
#118663=CARTESIAN_POINT('Ctrl Pts',(70.5746105091502,-21.2310059409266,
0.));
#118664=CARTESIAN_POINT('Ctrl Pts',(70.5746105091502,-21.2310059409266,
12.));
#118665=CARTESIAN_POINT('Ctrl Pts',(70.5540835797283,-21.2137349111208,
0.));
#118666=CARTESIAN_POINT('Ctrl Pts',(70.5540835797283,-21.2137349111208,
12.));
#118667=CARTESIAN_POINT('Ctrl Pts',(70.5335687714428,-21.1965062658298,
0.));
#118668=CARTESIAN_POINT('Ctrl Pts',(70.5335687714428,-21.1965062658298,
12.));
#118669=CARTESIAN_POINT('Ctrl Pts',(70.5130661852955,-21.1793200267847,
0.));
#118670=CARTESIAN_POINT('Ctrl Pts',(70.5130661852955,-21.1793200267847,
12.));
#118671=CARTESIAN_POINT('Ctrl Pts',(70.4925759224216,-21.1621762156897,
0.));
#118672=CARTESIAN_POINT('Ctrl Pts',(70.4925759224216,-21.1621762156897,
12.));
#118673=CARTESIAN_POINT('Ctrl Pts',(70.4720980841939,-21.1450748542337,
0.));
#118674=CARTESIAN_POINT('Ctrl Pts',(70.4720980841939,-21.1450748542337,
12.));
#118675=CARTESIAN_POINT('Ctrl Pts',(70.4516327723346,-21.1280159641003,
0.));
#118676=CARTESIAN_POINT('Ctrl Pts',(70.4516327723346,-21.1280159641003,
12.));
#118677=CARTESIAN_POINT('Ctrl Pts',(70.4311800890401,-21.1109995669747,
0.));
#118678=CARTESIAN_POINT('Ctrl Pts',(70.4311800890401,-21.1109995669747,
12.));
#118679=CARTESIAN_POINT('Ctrl Pts',(70.4107401370389,-21.0940256845473,
0.));
#118680=CARTESIAN_POINT('Ctrl Pts',(70.4107401370389,-21.0940256845473,
12.));
#118681=CARTESIAN_POINT('Ctrl Pts',(70.3903130195264,-21.0770943385141,
0.));
#118682=CARTESIAN_POINT('Ctrl Pts',(70.3903130195264,-21.0770943385141,
12.));
#118683=CARTESIAN_POINT('Ctrl Pts',(70.3698988401281,-21.0602055505748,
0.));
#118684=CARTESIAN_POINT('Ctrl Pts',(70.3698988401281,-21.0602055505748,
12.));
#118685=CARTESIAN_POINT('Ctrl Pts',(70.3494977028498,-21.0433593424267,
0.));
#118686=CARTESIAN_POINT('Ctrl Pts',(70.3494977028498,-21.0433593424267,
12.));
#118687=CARTESIAN_POINT('Ctrl Pts',(70.3291097120302,-21.0265557357548,
0.));
#118688=CARTESIAN_POINT('Ctrl Pts',(70.3291097120302,-21.0265557357548,
12.));
#118689=CARTESIAN_POINT('Ctrl Pts',(70.3087349722973,-21.0097947522218,
0.));
#118690=CARTESIAN_POINT('Ctrl Pts',(70.3087349722973,-21.0097947522218,
12.));
#118691=CARTESIAN_POINT('Ctrl Pts',(70.2883735885984,-20.9930764134776,
0.));
#118692=CARTESIAN_POINT('Ctrl Pts',(70.2883735885984,-20.9930764134776,
12.));
#118693=CARTESIAN_POINT('Ctrl Pts',(70.2680256662224,-20.9764007411653,
0.));
#118694=CARTESIAN_POINT('Ctrl Pts',(70.2680256662224,-20.9764007411653,
12.));
#118695=CARTESIAN_POINT('Ctrl Pts',(70.2476913108244,-20.9597677569228,
0.));
#118696=CARTESIAN_POINT('Ctrl Pts',(70.2476913108244,-20.9597677569228,
12.));
#118697=CARTESIAN_POINT('Ctrl Pts',(70.2273706284472,-20.9431774823831,
0.));
#118698=CARTESIAN_POINT('Ctrl Pts',(70.2273706284472,-20.9431774823831,
12.));
#118699=CARTESIAN_POINT('Ctrl Pts',(70.2070637255458,-20.9266299391684,
0.));
#118700=CARTESIAN_POINT('Ctrl Pts',(70.2070637255458,-20.9266299391684,
12.));
#118701=CARTESIAN_POINT('Ctrl Pts',(70.1867707089854,-20.9101251488944,
0.));
#118702=CARTESIAN_POINT('Ctrl Pts',(70.1867707089854,-20.9101251488944,
12.));
#118703=CARTESIAN_POINT('Ctrl Pts',(70.1664916860358,-20.8936631331748,
0.));
#118704=CARTESIAN_POINT('Ctrl Pts',(70.1664916860358,-20.8936631331748,
12.));
#118705=CARTESIAN_POINT('Ctrl Pts',(70.1462267643646,-20.8772439136206,
0.));
#118706=CARTESIAN_POINT('Ctrl Pts',(70.1462267643646,-20.8772439136206,
12.));
#118707=CARTESIAN_POINT('Ctrl Pts',(70.1259760520309,-20.8608675118379,
0.));
#118708=CARTESIAN_POINT('Ctrl Pts',(70.1259760520309,-20.8608675118379,
12.));
#118709=CARTESIAN_POINT('Ctrl Pts',(70.1057396574747,-20.8445339494188,
0.));
#118710=CARTESIAN_POINT('Ctrl Pts',(70.1057396574747,-20.8445339494188,
12.));
#118711=CARTESIAN_POINT('Ctrl Pts',(70.0855176895191,-20.8282432479429,
0.));
#118712=CARTESIAN_POINT('Ctrl Pts',(70.0855176895191,-20.8282432479429,
12.));
#118713=CARTESIAN_POINT('Ctrl Pts',(70.0653102573803,-20.8119954289849,
0.));
#118714=CARTESIAN_POINT('Ctrl Pts',(70.0653102573803,-20.8119954289849,
12.));
#118715=CARTESIAN_POINT('Ctrl Pts',(70.0451174706741,-20.7957905141157,
0.));
#118716=CARTESIAN_POINT('Ctrl Pts',(70.0451174706741,-20.7957905141157,
12.));
#118717=CARTESIAN_POINT('Ctrl Pts',(70.024939439422,-20.7796285249022,0.));
#118718=CARTESIAN_POINT('Ctrl Pts',(70.024939439422,-20.7796285249022,12.));
#118719=CARTESIAN_POINT('Ctrl Pts',(70.0047762740568,-20.7635094829016,
0.));
#118720=CARTESIAN_POINT('Ctrl Pts',(70.0047762740568,-20.7635094829016,
12.));
#118721=CARTESIAN_POINT('Ctrl Pts',(69.9846280854257,-20.7474334096581,
0.));
#118722=CARTESIAN_POINT('Ctrl Pts',(69.9846280854257,-20.7474334096581,
12.));
#118723=CARTESIAN_POINT('Ctrl Pts',(69.9644949847934,-20.7314003267119,
0.));
#118724=CARTESIAN_POINT('Ctrl Pts',(69.9644949847934,-20.7314003267119,
12.));
#118725=CARTESIAN_POINT('Ctrl Pts',(69.9443770838448,-20.7154102555997,
0.));
#118726=CARTESIAN_POINT('Ctrl Pts',(69.9443770838448,-20.7154102555997,
12.));
#118727=CARTESIAN_POINT('Ctrl Pts',(69.9242744946854,-20.6994632178552,
0.));
#118728=CARTESIAN_POINT('Ctrl Pts',(69.9242744946854,-20.6994632178552,
12.));
#118729=CARTESIAN_POINT('Ctrl Pts',(69.904187329841,-20.683559235003,0.));
#118730=CARTESIAN_POINT('Ctrl Pts',(69.904187329841,-20.683559235003,12.));
#118731=CARTESIAN_POINT('Ctrl Pts',(69.8841157022567,-20.667698328554,0.));
#118732=CARTESIAN_POINT('Ctrl Pts',(69.8841157022567,-20.667698328554,12.));
#118733=CARTESIAN_POINT('Ctrl Pts',(69.8640597253045,-20.6518805200129,
0.));
#118734=CARTESIAN_POINT('Ctrl Pts',(69.8640597253045,-20.6518805200129,
12.));
#118735=CARTESIAN_POINT('Ctrl Pts',(69.8440195127866,-20.6361058308811,
0.));
#118736=CARTESIAN_POINT('Ctrl Pts',(69.8440195127866,-20.6361058308811,
12.));
#118737=CARTESIAN_POINT('Ctrl Pts',(69.8239951789402,-20.6203742826566,
0.));
#118738=CARTESIAN_POINT('Ctrl Pts',(69.8239951789402,-20.6203742826566,
12.));
#118739=CARTESIAN_POINT('Ctrl Pts',(69.8039868384389,-20.6046858968308,
0.));
#118740=CARTESIAN_POINT('Ctrl Pts',(69.8039868384389,-20.6046858968308,
12.));
#118741=CARTESIAN_POINT('Ctrl Pts',(69.7839946063949,-20.5890406948811,
0.));
#118742=CARTESIAN_POINT('Ctrl Pts',(69.7839946063949,-20.5890406948811,
12.));
#118743=CARTESIAN_POINT('Ctrl Pts',(69.7640185983644,-20.5734386982783,
0.));
#118744=CARTESIAN_POINT('Ctrl Pts',(69.7640185983644,-20.5734386982783,
12.));
#118745=CARTESIAN_POINT('Ctrl Pts',(69.744058930351,-20.5578799284898,0.));
#118746=CARTESIAN_POINT('Ctrl Pts',(69.744058930351,-20.5578799284898,12.));
#118747=CARTESIAN_POINT('Ctrl Pts',(69.7241157188083,-20.54236440698,0.));
#118748=CARTESIAN_POINT('Ctrl Pts',(69.7241157188083,-20.54236440698,12.));
#118749=CARTESIAN_POINT('Ctrl Pts',(69.7041890806424,-20.5268921552077,
0.));
#118750=CARTESIAN_POINT('Ctrl Pts',(69.7041890806424,-20.5268921552077,
12.));
#118751=CARTESIAN_POINT('Ctrl Pts',(69.6842791332115,-20.5114631946185,
0.));
#118752=CARTESIAN_POINT('Ctrl Pts',(69.6842791332115,-20.5114631946185,
12.));
#118753=CARTESIAN_POINT('Ctrl Pts',(69.6643859943308,-20.4960775466492,
0.));
#118754=CARTESIAN_POINT('Ctrl Pts',(69.6643859943308,-20.4960775466492,
12.));
#118755=CARTESIAN_POINT('Ctrl Pts',(69.6445097822792,-20.480735232734,0.));
#118756=CARTESIAN_POINT('Ctrl Pts',(69.6445097822792,-20.480735232734,12.));
#118757=CARTESIAN_POINT('Ctrl Pts',(69.6246506158013,-20.4654362743038,
0.));
#118758=CARTESIAN_POINT('Ctrl Pts',(69.6246506158013,-20.4654362743038,
12.));
#118759=CARTESIAN_POINT('Ctrl Pts',(69.6048086141113,-20.4501806927852,
0.));
#118760=CARTESIAN_POINT('Ctrl Pts',(69.6048086141113,-20.4501806927852,
12.));
#118761=CARTESIAN_POINT('Ctrl Pts',(69.5849838968928,-20.4349685095924,
0.));
#118762=CARTESIAN_POINT('Ctrl Pts',(69.5849838968928,-20.4349685095924,
12.));
#118763=CARTESIAN_POINT('Ctrl Pts',(69.5651765843033,-20.4197997461301,
0.));
#118764=CARTESIAN_POINT('Ctrl Pts',(69.5651765843033,-20.4197997461301,
12.));
#118765=CARTESIAN_POINT('Ctrl Pts',(69.5453867969804,-20.4046744237999,
0.));
#118766=CARTESIAN_POINT('Ctrl Pts',(69.5453867969804,-20.4046744237999,
12.));
#118767=CARTESIAN_POINT('Ctrl Pts',(69.5256146560441,-20.3895925640005,
0.));
#118768=CARTESIAN_POINT('Ctrl Pts',(69.5256146560441,-20.3895925640005,
12.));
#118769=CARTESIAN_POINT('Ctrl Pts',(69.5058602831008,-20.3745541881269,
0.));
#118770=CARTESIAN_POINT('Ctrl Pts',(69.5058602831008,-20.3745541881269,
12.));
#118771=CARTESIAN_POINT('Ctrl Pts',(69.4861238002441,-20.3595593175623,
0.));
#118772=CARTESIAN_POINT('Ctrl Pts',(69.4861238002441,-20.3595593175623,
12.));
#118773=CARTESIAN_POINT('Ctrl Pts',(69.4664053300587,-20.3446079736802,
0.));
#118774=CARTESIAN_POINT('Ctrl Pts',(69.4664053300587,-20.3446079736802,
12.));
#118775=CARTESIAN_POINT('Ctrl Pts',(69.4467049956262,-20.3297001778507,
0.));
#118776=CARTESIAN_POINT('Ctrl Pts',(69.4467049956262,-20.3297001778507,
12.));
#118777=CARTESIAN_POINT('Ctrl Pts',(69.4270229205296,-20.3148359514415,
0.));
#118778=CARTESIAN_POINT('Ctrl Pts',(69.4270229205296,-20.3148359514415,
12.));
#118779=CARTESIAN_POINT('Ctrl Pts',(69.407359228856,-20.3000153158167,0.));
#118780=CARTESIAN_POINT('Ctrl Pts',(69.407359228856,-20.3000153158167,12.));
#118781=CARTESIAN_POINT('Ctrl Pts',(69.3877140451975,-20.2852382923299,
0.));
#118782=CARTESIAN_POINT('Ctrl Pts',(69.3877140451975,-20.2852382923299,
12.));
#118783=CARTESIAN_POINT('Ctrl Pts',(69.368087494655,-20.2705049023241,0.));
#118784=CARTESIAN_POINT('Ctrl Pts',(69.368087494655,-20.2705049023241,12.));
#118785=CARTESIAN_POINT('Ctrl Pts',(69.3484797028458,-20.2558151671391,
0.));
#118786=CARTESIAN_POINT('Ctrl Pts',(69.3484797028458,-20.2558151671391,
12.));
#118787=CARTESIAN_POINT('Ctrl Pts',(69.3288907959067,-20.2411691081123,
0.));
#118788=CARTESIAN_POINT('Ctrl Pts',(69.3288907959067,-20.2411691081123,
12.));
#118789=CARTESIAN_POINT('Ctrl Pts',(69.3093209004984,-20.2265667465784,
0.));
#118790=CARTESIAN_POINT('Ctrl Pts',(69.3093209004984,-20.2265667465784,
12.));
#118791=CARTESIAN_POINT('Ctrl Pts',(69.2897701438059,-20.2120081038621,
0.));
#118792=CARTESIAN_POINT('Ctrl Pts',(69.2897701438059,-20.2120081038621,
12.));
#118793=CARTESIAN_POINT('Ctrl Pts',(69.2702386535422,-20.1974932012773,
0.));
#118794=CARTESIAN_POINT('Ctrl Pts',(69.2702386535422,-20.1974932012773,
12.));
#118795=CARTESIAN_POINT('Ctrl Pts',(69.2507265579554,-20.1830220601349,
0.));
#118796=CARTESIAN_POINT('Ctrl Pts',(69.2507265579554,-20.1830220601349,
12.));
#118797=CARTESIAN_POINT('Ctrl Pts',(69.2312339858335,-20.1685947017433,
0.));
#118798=CARTESIAN_POINT('Ctrl Pts',(69.2312339858335,-20.1685947017433,
12.));
#118799=CARTESIAN_POINT('Ctrl Pts',(69.2117610665076,-20.1542111474087,
0.));
#118800=CARTESIAN_POINT('Ctrl Pts',(69.2117610665076,-20.1542111474087,
12.));
#118801=CARTESIAN_POINT('Ctrl Pts',(69.1923079298538,-20.139871418428,0.));
#118802=CARTESIAN_POINT('Ctrl Pts',(69.1923079298538,-20.139871418428,12.));
#118803=CARTESIAN_POINT('Ctrl Pts',(69.1728747062963,-20.1255755360872,
0.));
#118804=CARTESIAN_POINT('Ctrl Pts',(69.1728747062963,-20.1255755360872,
12.));
#118805=CARTESIAN_POINT('Ctrl Pts',(69.1534615268152,-20.1113235216694,
0.));
#118806=CARTESIAN_POINT('Ctrl Pts',(69.1534615268152,-20.1113235216694,
12.));
#118807=CARTESIAN_POINT('Ctrl Pts',(69.1340685229514,-20.0971153964557,
0.));
#118808=CARTESIAN_POINT('Ctrl Pts',(69.1340685229514,-20.0971153964557,
12.));
#118809=CARTESIAN_POINT('Ctrl Pts',(69.1146958268104,-20.0829511817251,
0.));
#118810=CARTESIAN_POINT('Ctrl Pts',(69.1146958268104,-20.0829511817251,
12.));
#118811=CARTESIAN_POINT('Ctrl Pts',(69.095343571064,-20.068830898748,0.));
#118812=CARTESIAN_POINT('Ctrl Pts',(69.095343571064,-20.068830898748,12.));
#118813=CARTESIAN_POINT('Ctrl Pts',(69.0760118889535,-20.0547545687842,
0.));
#118814=CARTESIAN_POINT('Ctrl Pts',(69.0760118889535,-20.0547545687842,
12.));
#118815=CARTESIAN_POINT('Ctrl Pts',(69.0567009142978,-20.0407222130906,
0.));
#118816=CARTESIAN_POINT('Ctrl Pts',(69.0567009142978,-20.0407222130906,
12.));
#118817=CARTESIAN_POINT('Ctrl Pts',(69.0374107814984,-20.0267338529223,
0.));
#118818=CARTESIAN_POINT('Ctrl Pts',(69.0374107814984,-20.0267338529223,
12.));
#118819=CARTESIAN_POINT('Ctrl Pts',(69.0181416255431,-20.0127895095327,
0.));
#118820=CARTESIAN_POINT('Ctrl Pts',(69.0181416255431,-20.0127895095327,
12.));
#118821=CARTESIAN_POINT('Ctrl Pts',(68.9988935820084,-19.9988892041666,
0.));
#118822=CARTESIAN_POINT('Ctrl Pts',(68.9988935820084,-19.9988892041666,
12.));
#118823=CARTESIAN_POINT('Ctrl Pts',(68.9796667870638,-19.9850329580591,
0.));
#118824=CARTESIAN_POINT('Ctrl Pts',(68.9796667870638,-19.9850329580591,
12.));
#118825=CARTESIAN_POINT('Ctrl Pts',(68.9604613774802,-19.9712207924429,
0.));
#118826=CARTESIAN_POINT('Ctrl Pts',(68.9604613774802,-19.9712207924429,
12.));
#118827=CARTESIAN_POINT('Ctrl Pts',(68.9412774906333,-19.9574527285488,
0.));
#118828=CARTESIAN_POINT('Ctrl Pts',(68.9412774906333,-19.9574527285488,
12.));
#118829=CARTESIAN_POINT('Ctrl Pts',(68.9221152645095,-19.9437287876066,
0.));
#118830=CARTESIAN_POINT('Ctrl Pts',(68.9221152645095,-19.9437287876066,
12.));
#118831=CARTESIAN_POINT('Ctrl Pts',(68.9029748377067,-19.9300489908374,
0.));
#118832=CARTESIAN_POINT('Ctrl Pts',(68.9029748377067,-19.9300489908374,
12.));
#118833=CARTESIAN_POINT('Ctrl Pts',(68.8838563494393,-19.9164133594526,
0.));
#118834=CARTESIAN_POINT('Ctrl Pts',(68.8838563494393,-19.9164133594526,
12.));
#118835=CARTESIAN_POINT('Ctrl Pts',(68.8647599395469,-19.9028219146618,
0.));
#118836=CARTESIAN_POINT('Ctrl Pts',(68.8647599395469,-19.9028219146618,
12.));
#118837=CARTESIAN_POINT('Ctrl Pts',(68.8456857485002,-19.8892746776739,
0.));
#118838=CARTESIAN_POINT('Ctrl Pts',(68.8456857485002,-19.8892746776739,
12.));
#118839=CARTESIAN_POINT('Ctrl Pts',(68.8266339174056,-19.8757716696966,
0.));
#118840=CARTESIAN_POINT('Ctrl Pts',(68.8266339174056,-19.8757716696966,
12.));
#118841=CARTESIAN_POINT('Ctrl Pts',(68.8076045880065,-19.8623129119293,
0.));
#118842=CARTESIAN_POINT('Ctrl Pts',(68.8076045880065,-19.8623129119293,
12.));
#118843=CARTESIAN_POINT('Ctrl Pts',(68.7885979026878,-19.8488984255627,
0.));
#118844=CARTESIAN_POINT('Ctrl Pts',(68.7885979026878,-19.8488984255627,
12.));
#118845=CARTESIAN_POINT('Ctrl Pts',(68.7696140044851,-19.8355282317858,
0.));
#118846=CARTESIAN_POINT('Ctrl Pts',(68.7696140044851,-19.8355282317858,
12.));
#118847=CARTESIAN_POINT('Ctrl Pts',(68.7506530370904,-19.8222023517871,
0.));
#118848=CARTESIAN_POINT('Ctrl Pts',(68.7506530370904,-19.8222023517871,
12.));
#118849=CARTESIAN_POINT('Ctrl Pts',(68.7317151448573,-19.8089208067538,
0.));
#118850=CARTESIAN_POINT('Ctrl Pts',(68.7317151448573,-19.8089208067538,
12.));
#118851=CARTESIAN_POINT('Ctrl Pts',(68.7128004728033,-19.7956836178651,
0.));
#118852=CARTESIAN_POINT('Ctrl Pts',(68.7128004728033,-19.7956836178651,
12.));
#118853=CARTESIAN_POINT('Ctrl Pts',(68.6939091666149,-19.7824908062925,
0.));
#118854=CARTESIAN_POINT('Ctrl Pts',(68.6939091666149,-19.7824908062925,
12.));
#118855=CARTESIAN_POINT('Ctrl Pts',(68.6750413726574,-19.7693423932067,
0.));
#118856=CARTESIAN_POINT('Ctrl Pts',(68.6750413726574,-19.7693423932067,
12.));
#118857=CARTESIAN_POINT('Ctrl Pts',(68.65619723798,-19.7562383997784,0.));
#118858=CARTESIAN_POINT('Ctrl Pts',(68.65619723798,-19.7562383997784,12.));
#118859=CARTESIAN_POINT('Ctrl Pts',(68.6373769103211,-19.7431788471773,
0.));
#118860=CARTESIAN_POINT('Ctrl Pts',(68.6373769103211,-19.7431788471773,
12.));
#118861=CARTESIAN_POINT('Ctrl Pts',(68.6185805381102,-19.7301637565646,
0.));
#118862=CARTESIAN_POINT('Ctrl Pts',(68.6185805381102,-19.7301637565646,
12.));
#118863=CARTESIAN_POINT('Ctrl Pts',(68.5998082704741,-19.717193149095,0.));
#118864=CARTESIAN_POINT('Ctrl Pts',(68.5998082704741,-19.717193149095,12.));
#118865=CARTESIAN_POINT('Ctrl Pts',(68.5810602572474,-19.7042670459234,
0.));
#118866=CARTESIAN_POINT('Ctrl Pts',(68.5810602572474,-19.7042670459234,
12.));
#118867=CARTESIAN_POINT('Ctrl Pts',(68.5623366489776,-19.6913854682046,
0.));
#118868=CARTESIAN_POINT('Ctrl Pts',(68.5623366489776,-19.6913854682046,
12.));
#118869=CARTESIAN_POINT('Ctrl Pts',(68.543637596932,-19.6785484370929,0.));
#118870=CARTESIAN_POINT('Ctrl Pts',(68.543637596932,-19.6785484370929,12.));
#118871=CARTESIAN_POINT('Ctrl Pts',(68.5249632530994,-19.665755973734,0.));
#118872=CARTESIAN_POINT('Ctrl Pts',(68.5249632530994,-19.665755973734,12.));
#118873=CARTESIAN_POINT('Ctrl Pts',(68.5063137701986,-19.653008099269,0.));
#118874=CARTESIAN_POINT('Ctrl Pts',(68.5063137701986,-19.653008099269,12.));
#118875=CARTESIAN_POINT('Ctrl Pts',(68.4876893016863,-19.6403048348397,
0.));
#118876=CARTESIAN_POINT('Ctrl Pts',(68.4876893016863,-19.6403048348397,
12.));
#118877=CARTESIAN_POINT('Ctrl Pts',(68.4690900017631,-19.6276462015888,
0.));
#118878=CARTESIAN_POINT('Ctrl Pts',(68.4690900017631,-19.6276462015888,
12.));
#118879=CARTESIAN_POINT('Ctrl Pts',(68.4505160253777,-19.6150322206578,
0.));
#118880=CARTESIAN_POINT('Ctrl Pts',(68.4505160253777,-19.6150322206578,
12.));
#118881=CARTESIAN_POINT('Ctrl Pts',(68.4319675282273,-19.6024629131786,
0.));
#118882=CARTESIAN_POINT('Ctrl Pts',(68.4319675282273,-19.6024629131786,
12.));
#118883=CARTESIAN_POINT('Ctrl Pts',(68.4134446667695,-19.5899383002804,
0.));
#118884=CARTESIAN_POINT('Ctrl Pts',(68.4134446667695,-19.5899383002804,
12.));
#118885=CARTESIAN_POINT('Ctrl Pts',(68.3949475982334,-19.5774584030939,
0.));
#118886=CARTESIAN_POINT('Ctrl Pts',(68.3949475982334,-19.5774584030939,
12.));
#118887=CARTESIAN_POINT('Ctrl Pts',(68.3764764806287,-19.5650232427516,
0.));
#118888=CARTESIAN_POINT('Ctrl Pts',(68.3764764806287,-19.5650232427516,
12.));
#118889=CARTESIAN_POINT('Ctrl Pts',(68.3580314727522,-19.5526328403852,
0.));
#118890=CARTESIAN_POINT('Ctrl Pts',(68.3580314727522,-19.5526328403852,
12.));
#118891=CARTESIAN_POINT('Ctrl Pts',(68.3396127341937,-19.540287217119,0.));
#118892=CARTESIAN_POINT('Ctrl Pts',(68.3396127341937,-19.540287217119,12.));
#118893=CARTESIAN_POINT('Ctrl Pts',(68.3212204253415,-19.5279863940773,
0.));
#118894=CARTESIAN_POINT('Ctrl Pts',(68.3212204253415,-19.5279863940773,
12.));
#118895=CARTESIAN_POINT('Ctrl Pts',(68.3028547073862,-19.5157303923856,
0.));
#118896=CARTESIAN_POINT('Ctrl Pts',(68.3028547073862,-19.5157303923856,
12.));
#118897=CARTESIAN_POINT('Ctrl Pts',(68.2845157423233,-19.5035192331706,
0.));
#118898=CARTESIAN_POINT('Ctrl Pts',(68.2845157423233,-19.5035192331706,
12.));
#118899=CARTESIAN_POINT('Ctrl Pts',(68.2662036929531,-19.4913529375546,
0.));
#118900=CARTESIAN_POINT('Ctrl Pts',(68.2662036929531,-19.4913529375546,
12.));
#118901=CARTESIAN_POINT('Ctrl Pts',(68.2479187228815,-19.4792315266505,
0.));
#118902=CARTESIAN_POINT('Ctrl Pts',(68.2479187228815,-19.4792315266505,
12.));
#118903=CARTESIAN_POINT('Ctrl Pts',(68.2296609965461,-19.4671550215725,
0.));
#118904=CARTESIAN_POINT('Ctrl Pts',(68.2296609965461,-19.4671550215725,
12.));
#118905=CARTESIAN_POINT('Ctrl Pts',(68.2114306792366,-19.4551234434384,
0.));
#118906=CARTESIAN_POINT('Ctrl Pts',(68.2114306792366,-19.4551234434384,
12.));
#118907=CARTESIAN_POINT('Ctrl Pts',(68.193227937112,-19.4431368133718,0.));
#118908=CARTESIAN_POINT('Ctrl Pts',(68.193227937112,-19.4431368133718,12.));
#118909=CARTESIAN_POINT('Ctrl Pts',(68.1750529372211,-19.4311951524977,
0.));
#118910=CARTESIAN_POINT('Ctrl Pts',(68.1750529372211,-19.4311951524977,
12.));
#118911=CARTESIAN_POINT('Ctrl Pts',(68.1569058475026,-19.4192984819411,
0.));
#118912=CARTESIAN_POINT('Ctrl Pts',(68.1569058475026,-19.4192984819411,
12.));
#118913=CARTESIAN_POINT('Ctrl Pts',(68.1387868367668,-19.4074468228294,
0.));
#118914=CARTESIAN_POINT('Ctrl Pts',(68.1387868367668,-19.4074468228294,
12.));
#118915=CARTESIAN_POINT('Ctrl Pts',(68.1206960746763,-19.3956401962894,
0.));
#118916=CARTESIAN_POINT('Ctrl Pts',(68.1206960746763,-19.3956401962894,
12.));
#118917=CARTESIAN_POINT('Ctrl Pts',(68.1026337317298,-19.3838786234426,
0.));
#118918=CARTESIAN_POINT('Ctrl Pts',(68.1026337317298,-19.3838786234426,
12.));
#118919=CARTESIAN_POINT('Ctrl Pts',(68.0845999792274,-19.3721621253921,
0.));
#118920=CARTESIAN_POINT('Ctrl Pts',(68.0845999792274,-19.3721621253921,
12.));
#118921=CARTESIAN_POINT('Ctrl Pts',(68.0665949893221,-19.3604907232322,
0.));
#118922=CARTESIAN_POINT('Ctrl Pts',(68.0665949893221,-19.3604907232322,
12.));
#118923=CARTESIAN_POINT('Ctrl Pts',(68.0486189351027,-19.3488644380646,
0.));
#118924=CARTESIAN_POINT('Ctrl Pts',(68.0486189351027,-19.3488644380646,
12.));
#118925=CARTESIAN_POINT('Ctrl Pts',(68.0306719906636,-19.3372832910077,
0.));
#118926=CARTESIAN_POINT('Ctrl Pts',(68.0306719906636,-19.3372832910077,
12.));
#118927=CARTESIAN_POINT('Ctrl Pts',(68.0127543311761,-19.3257473032031,
0.));
#118928=CARTESIAN_POINT('Ctrl Pts',(68.0127543311761,-19.3257473032031,
12.));
#118929=CARTESIAN_POINT('Ctrl Pts',(67.9948661329591,-19.3142564958196,
0.));
#118930=CARTESIAN_POINT('Ctrl Pts',(67.9948661329591,-19.3142564958196,
12.));
#118931=CARTESIAN_POINT('Ctrl Pts',(67.977007573346,-19.3028108900374,0.));
#118932=CARTESIAN_POINT('Ctrl Pts',(67.977007573346,-19.3028108900374,12.));
#118933=CARTESIAN_POINT('Ctrl Pts',(67.959178830538,-19.2914105070283,0.));
#118934=CARTESIAN_POINT('Ctrl Pts',(67.959178830538,-19.2914105070283,12.));
#118935=CARTESIAN_POINT('Ctrl Pts',(67.9413800834798,-19.2800553679362,
0.));
#118936=CARTESIAN_POINT('Ctrl Pts',(67.9413800834798,-19.2800553679362,
12.));
#118937=CARTESIAN_POINT('Ctrl Pts',(67.9236115116781,-19.2687454938449,
0.));
#118938=CARTESIAN_POINT('Ctrl Pts',(67.9236115116781,-19.2687454938449,
12.));
#118939=CARTESIAN_POINT('Ctrl Pts',(67.9058732951822,-19.2574809057705,
0.));
#118940=CARTESIAN_POINT('Ctrl Pts',(67.9058732951822,-19.2574809057705,
12.));
#118941=CARTESIAN_POINT('Ctrl Pts',(67.8881656149983,-19.2462616247287,
0.));
#118942=CARTESIAN_POINT('Ctrl Pts',(67.8881656149983,-19.2462616247287,
12.));
#118943=CARTESIAN_POINT('Ctrl Pts',(67.8704886534555,-19.2350876717878,
0.));
#118944=CARTESIAN_POINT('Ctrl Pts',(67.8704886534555,-19.2350876717878,
12.));
#118945=CARTESIAN_POINT('Ctrl Pts',(67.852842594517,-19.223959068113,0.));
#118946=CARTESIAN_POINT('Ctrl Pts',(67.852842594517,-19.223959068113,12.));
#118947=CARTESIAN_POINT('Ctrl Pts',(67.8352276242856,-19.2128758350336,
0.));
#118948=CARTESIAN_POINT('Ctrl Pts',(67.8352276242856,-19.2128758350336,
12.));
#118949=CARTESIAN_POINT('Ctrl Pts',(67.817643930658,-19.2018379939918,0.));
#118950=CARTESIAN_POINT('Ctrl Pts',(67.817643930658,-19.2018379939918,12.));
#118951=CARTESIAN_POINT('Ctrl Pts',(67.8000917023896,-19.1908455664089,
0.));
#118952=CARTESIAN_POINT('Ctrl Pts',(67.8000917023896,-19.1908455664089,
12.));
#118953=CARTESIAN_POINT('Ctrl Pts',(67.7825711283092,-19.1798985735687,
0.));
#118954=CARTESIAN_POINT('Ctrl Pts',(67.7825711283092,-19.1798985735687,
12.));
#118955=CARTESIAN_POINT('Ctrl Pts',(67.7650823965156,-19.1689970364959,
0.));
#118956=CARTESIAN_POINT('Ctrl Pts',(67.7650823965156,-19.1689970364959,
12.));
#118957=CARTESIAN_POINT('Ctrl Pts',(67.7476256934492,-19.1581409758112,
0.));
#118958=CARTESIAN_POINT('Ctrl Pts',(67.7476256934492,-19.1581409758112,
12.));
#118959=CARTESIAN_POINT('Ctrl Pts',(67.7302012056629,-19.1473304119969,
0.));
#118960=CARTESIAN_POINT('Ctrl Pts',(67.7302012056629,-19.1473304119969,
12.));
#118961=CARTESIAN_POINT('Ctrl Pts',(67.7128091219372,-19.1365653657098,
0.));
#118962=CARTESIAN_POINT('Ctrl Pts',(67.7128091219372,-19.1365653657098,
12.));
#118963=CARTESIAN_POINT('Ctrl Pts',(67.6954496350053,-19.1258458580343,
0.));
#118964=CARTESIAN_POINT('Ctrl Pts',(67.6954496350053,-19.1258458580343,
12.));
#118965=CARTESIAN_POINT('Ctrl Pts',(67.6781229440535,-19.115171910845,0.));
#118966=CARTESIAN_POINT('Ctrl Pts',(67.6781229440535,-19.115171910845,12.));
#118967=CARTESIAN_POINT('Ctrl Pts',(67.6608292549412,-19.1045435468345,
0.));
#118968=CARTESIAN_POINT('Ctrl Pts',(67.6608292549412,-19.1045435468345,
12.));
#118969=CARTESIAN_POINT('Ctrl Pts',(67.6435687749802,-19.0939607887492,
0.));
#118970=CARTESIAN_POINT('Ctrl Pts',(67.6435687749802,-19.0939607887492,
12.));
#118971=CARTESIAN_POINT('Ctrl Pts',(67.6263417083413,-19.0834236587115,
0.));
#118972=CARTESIAN_POINT('Ctrl Pts',(67.6263417083413,-19.0834236587115,
12.));
#118973=CARTESIAN_POINT('Ctrl Pts',(67.6091482520557,-19.0729321776287,
0.));
#118974=CARTESIAN_POINT('Ctrl Pts',(67.6091482520557,-19.0729321776287,
12.));
#118975=CARTESIAN_POINT('Ctrl Pts',(67.5919885896278,-19.0624863642425,
0.));
#118976=CARTESIAN_POINT('Ctrl Pts',(67.5919885896278,-19.0624863642425,
12.));
#118977=CARTESIAN_POINT('Ctrl Pts',(67.5748628972035,-19.0520862360414,
0.));
#118978=CARTESIAN_POINT('Ctrl Pts',(67.5748628972035,-19.0520862360414,
12.));
#118979=CARTESIAN_POINT('Ctrl Pts',(67.5577713558248,-19.0417318110721,
0.));
#118980=CARTESIAN_POINT('Ctrl Pts',(67.5577713558248,-19.0417318110721,
12.));
#118981=CARTESIAN_POINT('Ctrl Pts',(67.540714161288,-19.0314231093924,0.));
#118982=CARTESIAN_POINT('Ctrl Pts',(67.540714161288,-19.0314231093924,12.));
#118983=CARTESIAN_POINT('Ctrl Pts',(67.5236915360253,-19.0211601548222,
0.));
#118984=CARTESIAN_POINT('Ctrl Pts',(67.5236915360253,-19.0211601548222,
12.));
#118985=CARTESIAN_POINT('Ctrl Pts',(67.5067037372177,-19.0109429761274,
0.));
#118986=CARTESIAN_POINT('Ctrl Pts',(67.5067037372177,-19.0109429761274,
12.));
#118987=CARTESIAN_POINT('Ctrl Pts',(67.4897510316692,-19.0007716032785,
0.));
#118988=CARTESIAN_POINT('Ctrl Pts',(67.4897510316692,-19.0007716032785,
12.));
#118989=CARTESIAN_POINT('Ctrl Pts',(67.4728336719558,-18.9906460638607,
0.));
#118990=CARTESIAN_POINT('Ctrl Pts',(67.4728336719558,-18.9906460638607,
12.));
#118991=CARTESIAN_POINT('Ctrl Pts',(67.4559518744713,-18.9805663798466,
0.));
#118992=CARTESIAN_POINT('Ctrl Pts',(67.4559518744713,-18.9805663798466,
12.));
#118993=CARTESIAN_POINT('Ctrl Pts',(67.4391057908687,-18.9705325631773,
0.));
#118994=CARTESIAN_POINT('Ctrl Pts',(67.4391057908687,-18.9705325631773,
12.));
#118995=CARTESIAN_POINT('Ctrl Pts',(67.4222955062384,-18.9605446161079,
0.));
#118996=CARTESIAN_POINT('Ctrl Pts',(67.4222955062384,-18.9605446161079,
12.));
#118997=CARTESIAN_POINT('Ctrl Pts',(67.4088759498287,-18.9525909518003,
0.));
#118998=CARTESIAN_POINT('Ctrl Pts',(67.4088759498287,-18.9525909518003,
12.));
#118999=CARTESIAN_POINT('Ctrl Pts',(67.398827414689,-18.9466463414355,0.));
#119000=CARTESIAN_POINT('Ctrl Pts',(67.398827414689,-18.9466463414355,12.));
#119001=CARTESIAN_POINT('Ctrl Pts',(67.3921355608417,-18.942692439874,0.));
#119002=CARTESIAN_POINT('Ctrl Pts',(67.3921355608417,-18.942692439874,12.));
#119003=CARTESIAN_POINT('Ctrl Pts',(67.3887914263118,-18.9407177820969,
0.));
#119004=CARTESIAN_POINT('Ctrl Pts',(67.3887914263118,-18.9407177820969,
12.));
#119005=CARTESIAN_POINT('',(67.3887914263118,-18.9407177820969,12.));
#119006=CARTESIAN_POINT('Ctrl Pts',(67.3887914263118,-18.9407177820969,
12.));
#119007=CARTESIAN_POINT('Ctrl Pts',(67.3921355608417,-18.942692439874,12.));
#119008=CARTESIAN_POINT('Ctrl Pts',(67.398827414689,-18.9466463414355,12.));
#119009=CARTESIAN_POINT('Ctrl Pts',(67.4088759498287,-18.9525909518003,
12.));
#119010=CARTESIAN_POINT('Ctrl Pts',(67.4222955062384,-18.9605446161079,
12.));
#119011=CARTESIAN_POINT('Ctrl Pts',(67.4391057908687,-18.9705325631773,
12.));
#119012=CARTESIAN_POINT('Ctrl Pts',(67.4559518744713,-18.9805663798466,
12.));
#119013=CARTESIAN_POINT('Ctrl Pts',(67.4728336719558,-18.9906460638607,
12.));
#119014=CARTESIAN_POINT('Ctrl Pts',(67.4897510316692,-19.0007716032785,
12.));
#119015=CARTESIAN_POINT('Ctrl Pts',(67.5067037372177,-19.0109429761274,
12.));
#119016=CARTESIAN_POINT('Ctrl Pts',(67.5236915360253,-19.0211601548222,
12.));
#119017=CARTESIAN_POINT('Ctrl Pts',(67.540714161288,-19.0314231093924,12.));
#119018=CARTESIAN_POINT('Ctrl Pts',(67.5577713558248,-19.0417318110721,
12.));
#119019=CARTESIAN_POINT('Ctrl Pts',(67.5748628972035,-19.0520862360414,
12.));
#119020=CARTESIAN_POINT('Ctrl Pts',(67.5919885896278,-19.0624863642425,
12.));
#119021=CARTESIAN_POINT('Ctrl Pts',(67.6091482520557,-19.0729321776287,
12.));
#119022=CARTESIAN_POINT('Ctrl Pts',(67.6263417083413,-19.0834236587115,
12.));
#119023=CARTESIAN_POINT('Ctrl Pts',(67.6435687749802,-19.0939607887492,
12.));
#119024=CARTESIAN_POINT('Ctrl Pts',(67.6608292549412,-19.1045435468345,
12.));
#119025=CARTESIAN_POINT('Ctrl Pts',(67.6781229440535,-19.115171910845,12.));
#119026=CARTESIAN_POINT('Ctrl Pts',(67.6954496350053,-19.1258458580343,
12.));
#119027=CARTESIAN_POINT('Ctrl Pts',(67.7128091219372,-19.1365653657098,
12.));
#119028=CARTESIAN_POINT('Ctrl Pts',(67.7302012056629,-19.1473304119969,
12.));
#119029=CARTESIAN_POINT('Ctrl Pts',(67.7476256934492,-19.1581409758112,
12.));
#119030=CARTESIAN_POINT('Ctrl Pts',(67.7650823965156,-19.1689970364959,
12.));
#119031=CARTESIAN_POINT('Ctrl Pts',(67.7825711283092,-19.1798985735687,
12.));
#119032=CARTESIAN_POINT('Ctrl Pts',(67.8000917023896,-19.1908455664089,
12.));
#119033=CARTESIAN_POINT('Ctrl Pts',(67.817643930658,-19.2018379939918,12.));
#119034=CARTESIAN_POINT('Ctrl Pts',(67.8352276242856,-19.2128758350336,
12.));
#119035=CARTESIAN_POINT('Ctrl Pts',(67.852842594517,-19.223959068113,12.));
#119036=CARTESIAN_POINT('Ctrl Pts',(67.8704886534555,-19.2350876717878,
12.));
#119037=CARTESIAN_POINT('Ctrl Pts',(67.8881656149983,-19.2462616247287,
12.));
#119038=CARTESIAN_POINT('Ctrl Pts',(67.9058732951822,-19.2574809057705,
12.));
#119039=CARTESIAN_POINT('Ctrl Pts',(67.9236115116781,-19.2687454938449,
12.));
#119040=CARTESIAN_POINT('Ctrl Pts',(67.9413800834798,-19.2800553679362,
12.));
#119041=CARTESIAN_POINT('Ctrl Pts',(67.959178830538,-19.2914105070283,12.));
#119042=CARTESIAN_POINT('Ctrl Pts',(67.977007573346,-19.3028108900374,12.));
#119043=CARTESIAN_POINT('Ctrl Pts',(67.9948661329591,-19.3142564958196,
12.));
#119044=CARTESIAN_POINT('Ctrl Pts',(68.0127543311761,-19.3257473032031,
12.));
#119045=CARTESIAN_POINT('Ctrl Pts',(68.0306719906636,-19.3372832910077,
12.));
#119046=CARTESIAN_POINT('Ctrl Pts',(68.0486189351027,-19.3488644380646,
12.));
#119047=CARTESIAN_POINT('Ctrl Pts',(68.0665949893221,-19.3604907232322,
12.));
#119048=CARTESIAN_POINT('Ctrl Pts',(68.0845999792274,-19.3721621253921,
12.));
#119049=CARTESIAN_POINT('Ctrl Pts',(68.1026337317298,-19.3838786234426,
12.));
#119050=CARTESIAN_POINT('Ctrl Pts',(68.1206960746763,-19.3956401962894,
12.));
#119051=CARTESIAN_POINT('Ctrl Pts',(68.1387868367668,-19.4074468228294,
12.));
#119052=CARTESIAN_POINT('Ctrl Pts',(68.1569058475026,-19.4192984819411,
12.));
#119053=CARTESIAN_POINT('Ctrl Pts',(68.1750529372211,-19.4311951524977,
12.));
#119054=CARTESIAN_POINT('Ctrl Pts',(68.193227937112,-19.4431368133718,12.));
#119055=CARTESIAN_POINT('Ctrl Pts',(68.2114306792366,-19.4551234434384,
12.));
#119056=CARTESIAN_POINT('Ctrl Pts',(68.2296609965461,-19.4671550215725,
12.));
#119057=CARTESIAN_POINT('Ctrl Pts',(68.2479187228815,-19.4792315266505,
12.));
#119058=CARTESIAN_POINT('Ctrl Pts',(68.2662036929531,-19.4913529375546,
12.));
#119059=CARTESIAN_POINT('Ctrl Pts',(68.2845157423233,-19.5035192331706,
12.));
#119060=CARTESIAN_POINT('Ctrl Pts',(68.3028547073862,-19.5157303923856,
12.));
#119061=CARTESIAN_POINT('Ctrl Pts',(68.3212204253415,-19.5279863940773,
12.));
#119062=CARTESIAN_POINT('Ctrl Pts',(68.3396127341937,-19.540287217119,12.));
#119063=CARTESIAN_POINT('Ctrl Pts',(68.3580314727522,-19.5526328403852,
12.));
#119064=CARTESIAN_POINT('Ctrl Pts',(68.3764764806287,-19.5650232427516,
12.));
#119065=CARTESIAN_POINT('Ctrl Pts',(68.3949475982334,-19.5774584030939,
12.));
#119066=CARTESIAN_POINT('Ctrl Pts',(68.4134446667695,-19.5899383002804,
12.));
#119067=CARTESIAN_POINT('Ctrl Pts',(68.4319675282273,-19.6024629131786,
12.));
#119068=CARTESIAN_POINT('Ctrl Pts',(68.4505160253777,-19.6150322206578,
12.));
#119069=CARTESIAN_POINT('Ctrl Pts',(68.4690900017631,-19.6276462015888,
12.));
#119070=CARTESIAN_POINT('Ctrl Pts',(68.4876893016863,-19.6403048348397,
12.));
#119071=CARTESIAN_POINT('Ctrl Pts',(68.5063137701986,-19.653008099269,12.));
#119072=CARTESIAN_POINT('Ctrl Pts',(68.5249632530994,-19.665755973734,12.));
#119073=CARTESIAN_POINT('Ctrl Pts',(68.543637596932,-19.6785484370929,12.));
#119074=CARTESIAN_POINT('Ctrl Pts',(68.5623366489776,-19.6913854682046,
12.));
#119075=CARTESIAN_POINT('Ctrl Pts',(68.5810602572474,-19.7042670459234,
12.));
#119076=CARTESIAN_POINT('Ctrl Pts',(68.5998082704741,-19.717193149095,12.));
#119077=CARTESIAN_POINT('Ctrl Pts',(68.6185805381102,-19.7301637565646,
12.));
#119078=CARTESIAN_POINT('Ctrl Pts',(68.6373769103211,-19.7431788471773,
12.));
#119079=CARTESIAN_POINT('Ctrl Pts',(68.65619723798,-19.7562383997784,12.));
#119080=CARTESIAN_POINT('Ctrl Pts',(68.6750413726574,-19.7693423932067,
12.));
#119081=CARTESIAN_POINT('Ctrl Pts',(68.6939091666149,-19.7824908062925,
12.));
#119082=CARTESIAN_POINT('Ctrl Pts',(68.7128004728033,-19.7956836178651,
12.));
#119083=CARTESIAN_POINT('Ctrl Pts',(68.7317151448573,-19.8089208067538,
12.));
#119084=CARTESIAN_POINT('Ctrl Pts',(68.7506530370904,-19.8222023517871,
12.));
#119085=CARTESIAN_POINT('Ctrl Pts',(68.7696140044851,-19.8355282317858,
12.));
#119086=CARTESIAN_POINT('Ctrl Pts',(68.7885979026878,-19.8488984255627,
12.));
#119087=CARTESIAN_POINT('Ctrl Pts',(68.8076045880065,-19.8623129119293,
12.));
#119088=CARTESIAN_POINT('Ctrl Pts',(68.8266339174056,-19.8757716696966,
12.));
#119089=CARTESIAN_POINT('Ctrl Pts',(68.8456857485002,-19.8892746776739,
12.));
#119090=CARTESIAN_POINT('Ctrl Pts',(68.8647599395469,-19.9028219146618,
12.));
#119091=CARTESIAN_POINT('Ctrl Pts',(68.8838563494393,-19.9164133594526,
12.));
#119092=CARTESIAN_POINT('Ctrl Pts',(68.9029748377067,-19.9300489908374,
12.));
#119093=CARTESIAN_POINT('Ctrl Pts',(68.9221152645095,-19.9437287876066,
12.));
#119094=CARTESIAN_POINT('Ctrl Pts',(68.9412774906333,-19.9574527285488,
12.));
#119095=CARTESIAN_POINT('Ctrl Pts',(68.9604613774802,-19.9712207924429,
12.));
#119096=CARTESIAN_POINT('Ctrl Pts',(68.9796667870638,-19.9850329580591,
12.));
#119097=CARTESIAN_POINT('Ctrl Pts',(68.9988935820084,-19.9988892041666,
12.));
#119098=CARTESIAN_POINT('Ctrl Pts',(69.0181416255431,-20.0127895095327,
12.));
#119099=CARTESIAN_POINT('Ctrl Pts',(69.0374107814984,-20.0267338529223,
12.));
#119100=CARTESIAN_POINT('Ctrl Pts',(69.0567009142978,-20.0407222130906,
12.));
#119101=CARTESIAN_POINT('Ctrl Pts',(69.0760118889535,-20.0547545687842,
12.));
#119102=CARTESIAN_POINT('Ctrl Pts',(69.095343571064,-20.068830898748,12.));
#119103=CARTESIAN_POINT('Ctrl Pts',(69.1146958268104,-20.0829511817251,
12.));
#119104=CARTESIAN_POINT('Ctrl Pts',(69.1340685229514,-20.0971153964557,
12.));
#119105=CARTESIAN_POINT('Ctrl Pts',(69.1534615268152,-20.1113235216694,
12.));
#119106=CARTESIAN_POINT('Ctrl Pts',(69.1728747062963,-20.1255755360872,
12.));
#119107=CARTESIAN_POINT('Ctrl Pts',(69.1923079298538,-20.139871418428,12.));
#119108=CARTESIAN_POINT('Ctrl Pts',(69.2117610665076,-20.1542111474087,
12.));
#119109=CARTESIAN_POINT('Ctrl Pts',(69.2312339858335,-20.1685947017433,
12.));
#119110=CARTESIAN_POINT('Ctrl Pts',(69.2507265579554,-20.1830220601349,
12.));
#119111=CARTESIAN_POINT('Ctrl Pts',(69.2702386535422,-20.1974932012773,
12.));
#119112=CARTESIAN_POINT('Ctrl Pts',(69.2897701438059,-20.2120081038621,
12.));
#119113=CARTESIAN_POINT('Ctrl Pts',(69.3093209004984,-20.2265667465784,
12.));
#119114=CARTESIAN_POINT('Ctrl Pts',(69.3288907959067,-20.2411691081123,
12.));
#119115=CARTESIAN_POINT('Ctrl Pts',(69.3484797028458,-20.2558151671391,
12.));
#119116=CARTESIAN_POINT('Ctrl Pts',(69.368087494655,-20.2705049023241,12.));
#119117=CARTESIAN_POINT('Ctrl Pts',(69.3877140451975,-20.2852382923299,
12.));
#119118=CARTESIAN_POINT('Ctrl Pts',(69.407359228856,-20.3000153158167,12.));
#119119=CARTESIAN_POINT('Ctrl Pts',(69.4270229205296,-20.3148359514415,
12.));
#119120=CARTESIAN_POINT('Ctrl Pts',(69.4467049956262,-20.3297001778507,
12.));
#119121=CARTESIAN_POINT('Ctrl Pts',(69.4664053300587,-20.3446079736802,
12.));
#119122=CARTESIAN_POINT('Ctrl Pts',(69.4861238002441,-20.3595593175623,
12.));
#119123=CARTESIAN_POINT('Ctrl Pts',(69.5058602831008,-20.3745541881269,
12.));
#119124=CARTESIAN_POINT('Ctrl Pts',(69.5256146560441,-20.3895925640005,
12.));
#119125=CARTESIAN_POINT('Ctrl Pts',(69.5453867969804,-20.4046744237999,
12.));
#119126=CARTESIAN_POINT('Ctrl Pts',(69.5651765843033,-20.4197997461301,
12.));
#119127=CARTESIAN_POINT('Ctrl Pts',(69.5849838968928,-20.4349685095924,
12.));
#119128=CARTESIAN_POINT('Ctrl Pts',(69.6048086141113,-20.4501806927852,
12.));
#119129=CARTESIAN_POINT('Ctrl Pts',(69.6246506158013,-20.4654362743038,
12.));
#119130=CARTESIAN_POINT('Ctrl Pts',(69.6445097822792,-20.480735232734,12.));
#119131=CARTESIAN_POINT('Ctrl Pts',(69.6643859943308,-20.4960775466492,
12.));
#119132=CARTESIAN_POINT('Ctrl Pts',(69.6842791332115,-20.5114631946185,
12.));
#119133=CARTESIAN_POINT('Ctrl Pts',(69.7041890806424,-20.5268921552077,
12.));
#119134=CARTESIAN_POINT('Ctrl Pts',(69.7241157188083,-20.54236440698,12.));
#119135=CARTESIAN_POINT('Ctrl Pts',(69.744058930351,-20.5578799284898,12.));
#119136=CARTESIAN_POINT('Ctrl Pts',(69.7640185983644,-20.5734386982783,
12.));
#119137=CARTESIAN_POINT('Ctrl Pts',(69.7839946063949,-20.5890406948811,
12.));
#119138=CARTESIAN_POINT('Ctrl Pts',(69.8039868384389,-20.6046858968308,
12.));
#119139=CARTESIAN_POINT('Ctrl Pts',(69.8239951789402,-20.6203742826566,
12.));
#119140=CARTESIAN_POINT('Ctrl Pts',(69.8440195127866,-20.6361058308811,
12.));
#119141=CARTESIAN_POINT('Ctrl Pts',(69.8640597253045,-20.6518805200129,
12.));
#119142=CARTESIAN_POINT('Ctrl Pts',(69.8841157022567,-20.667698328554,12.));
#119143=CARTESIAN_POINT('Ctrl Pts',(69.904187329841,-20.683559235003,12.));
#119144=CARTESIAN_POINT('Ctrl Pts',(69.9242744946854,-20.6994632178552,
12.));
#119145=CARTESIAN_POINT('Ctrl Pts',(69.9443770838448,-20.7154102555997,
12.));
#119146=CARTESIAN_POINT('Ctrl Pts',(69.9644949847934,-20.7314003267119,
12.));
#119147=CARTESIAN_POINT('Ctrl Pts',(69.9846280854257,-20.7474334096581,
12.));
#119148=CARTESIAN_POINT('Ctrl Pts',(70.0047762740568,-20.7635094829016,
12.));
#119149=CARTESIAN_POINT('Ctrl Pts',(70.024939439422,-20.7796285249022,12.));
#119150=CARTESIAN_POINT('Ctrl Pts',(70.0451174706741,-20.7957905141157,
12.));
#119151=CARTESIAN_POINT('Ctrl Pts',(70.0653102573803,-20.8119954289849,
12.));
#119152=CARTESIAN_POINT('Ctrl Pts',(70.0855176895191,-20.8282432479429,
12.));
#119153=CARTESIAN_POINT('Ctrl Pts',(70.1057396574747,-20.8445339494188,
12.));
#119154=CARTESIAN_POINT('Ctrl Pts',(70.1259760520309,-20.8608675118379,
12.));
#119155=CARTESIAN_POINT('Ctrl Pts',(70.1462267643646,-20.8772439136206,
12.));
#119156=CARTESIAN_POINT('Ctrl Pts',(70.1664916860358,-20.8936631331748,
12.));
#119157=CARTESIAN_POINT('Ctrl Pts',(70.1867707089854,-20.9101251488944,
12.));
#119158=CARTESIAN_POINT('Ctrl Pts',(70.2070637255458,-20.9266299391684,
12.));
#119159=CARTESIAN_POINT('Ctrl Pts',(70.2273706284472,-20.9431774823831,
12.));
#119160=CARTESIAN_POINT('Ctrl Pts',(70.2476913108244,-20.9597677569228,
12.));
#119161=CARTESIAN_POINT('Ctrl Pts',(70.2680256662224,-20.9764007411653,
12.));
#119162=CARTESIAN_POINT('Ctrl Pts',(70.2883735885984,-20.9930764134776,
12.));
#119163=CARTESIAN_POINT('Ctrl Pts',(70.3087349722973,-21.0097947522218,
12.));
#119164=CARTESIAN_POINT('Ctrl Pts',(70.3291097120302,-21.0265557357548,
12.));
#119165=CARTESIAN_POINT('Ctrl Pts',(70.3494977028498,-21.0433593424267,
12.));
#119166=CARTESIAN_POINT('Ctrl Pts',(70.3698988401281,-21.0602055505748,
12.));
#119167=CARTESIAN_POINT('Ctrl Pts',(70.3903130195264,-21.0770943385141,
12.));
#119168=CARTESIAN_POINT('Ctrl Pts',(70.4107401370389,-21.0940256845473,
12.));
#119169=CARTESIAN_POINT('Ctrl Pts',(70.4311800890401,-21.1109995669747,
12.));
#119170=CARTESIAN_POINT('Ctrl Pts',(70.4516327723346,-21.1280159641003,
12.));
#119171=CARTESIAN_POINT('Ctrl Pts',(70.4720980841939,-21.1450748542337,
12.));
#119172=CARTESIAN_POINT('Ctrl Pts',(70.4925759224216,-21.1621762156897,
12.));
#119173=CARTESIAN_POINT('Ctrl Pts',(70.5130661852955,-21.1793200267847,
12.));
#119174=CARTESIAN_POINT('Ctrl Pts',(70.5335687714428,-21.1965062658298,
12.));
#119175=CARTESIAN_POINT('Ctrl Pts',(70.5540835797283,-21.2137349111208,
12.));
#119176=CARTESIAN_POINT('Ctrl Pts',(70.5746105091502,-21.2310059409266,
12.));
#119177=CARTESIAN_POINT('Ctrl Pts',(70.5951494586957,-21.2483193334676,
12.));
#119178=CARTESIAN_POINT('Ctrl Pts',(70.6157003273316,-21.2656750669126,
12.));
#119179=CARTESIAN_POINT('Ctrl Pts',(70.6362630143047,-21.2830731194183,
12.));
#119180=CARTESIAN_POINT('Ctrl Pts',(70.6568374193774,-21.300513469156,12.));
#119181=CARTESIAN_POINT('Ctrl Pts',(70.6774234430897,-21.3179960943389,
12.));
#119182=CARTESIAN_POINT('Ctrl Pts',(70.6980209870044,-21.3355209732443,
12.));
#119183=CARTESIAN_POINT('Ctrl Pts',(70.7186299539724,-21.3530880842349,
12.));
#119184=CARTESIAN_POINT('Ctrl Pts',(70.7392502475469,-21.3706974057039,
12.));
#119185=CARTESIAN_POINT('Ctrl Pts',(70.7598817714105,-21.3883489160196,
12.));
#119186=CARTESIAN_POINT('Ctrl Pts',(70.780524428745,-21.4060425934599,12.));
#119187=CARTESIAN_POINT('Ctrl Pts',(70.8011781217394,-21.4237784161588,
12.));
#119188=CARTESIAN_POINT('Ctrl Pts',(70.8218427507506,-21.4415563620114,
12.));
#119189=CARTESIAN_POINT('Ctrl Pts',(70.8425182149846,-21.4593764087474,
12.));
#119190=CARTESIAN_POINT('Ctrl Pts',(70.8632044140112,-21.477238534096,12.));
#119191=CARTESIAN_POINT('Ctrl Pts',(70.8839012490871,-21.4951427159262,
12.));
#119192=CARTESIAN_POINT('Ctrl Pts',(70.9046086244131,-21.513088932377,12.));
#119193=CARTESIAN_POINT('Ctrl Pts',(70.9253264487636,-21.5310771620231,
12.));
#119194=CARTESIAN_POINT('Ctrl Pts',(70.94605463587,-21.5491073839106,12.));
#119195=CARTESIAN_POINT('Ctrl Pts',(70.9638315189817,-21.564598755537,12.));
#119196=CARTESIAN_POINT('Ctrl Pts',(70.9774662112589,-21.5764983366482,
12.));
#119197=CARTESIAN_POINT('Ctrl Pts',(70.9869541808056,-21.5847875433333,
12.));
#119198=CARTESIAN_POINT('Ctrl Pts',(70.9922924595369,-21.5894540925585,
12.));
#119199=CARTESIAN_POINT('Ctrl Pts',(70.9934796069117,-21.5904919935063,
12.));
#119200=CARTESIAN_POINT('',(67.3887914263118,-18.9407177820969,0.));
#119201=CARTESIAN_POINT('',(67.3887914263118,-18.9407177820969,0.));
#119202=CARTESIAN_POINT('Ctrl Pts',(70.9934796069117,-21.5904919935063,
0.));
#119203=CARTESIAN_POINT('Ctrl Pts',(70.9922924595369,-21.5894540925585,
0.));
#119204=CARTESIAN_POINT('Ctrl Pts',(70.9869541808056,-21.5847875433333,
0.));
#119205=CARTESIAN_POINT('Ctrl Pts',(70.9774662112589,-21.5764983366482,
0.));
#119206=CARTESIAN_POINT('Ctrl Pts',(70.9638315189817,-21.564598755537,0.));
#119207=CARTESIAN_POINT('Ctrl Pts',(70.94605463587,-21.5491073839106,0.));
#119208=CARTESIAN_POINT('Ctrl Pts',(70.9253264487636,-21.5310771620231,
0.));
#119209=CARTESIAN_POINT('Ctrl Pts',(70.9046086244131,-21.513088932377,0.));
#119210=CARTESIAN_POINT('Ctrl Pts',(70.8839012490871,-21.4951427159262,
0.));
#119211=CARTESIAN_POINT('Ctrl Pts',(70.8632044140112,-21.477238534096,0.));
#119212=CARTESIAN_POINT('Ctrl Pts',(70.8425182149846,-21.4593764087474,
0.));
#119213=CARTESIAN_POINT('Ctrl Pts',(70.8218427507506,-21.4415563620114,
0.));
#119214=CARTESIAN_POINT('Ctrl Pts',(70.8011781217394,-21.4237784161588,
0.));
#119215=CARTESIAN_POINT('Ctrl Pts',(70.780524428745,-21.4060425934599,0.));
#119216=CARTESIAN_POINT('Ctrl Pts',(70.7598817714105,-21.3883489160196,
0.));
#119217=CARTESIAN_POINT('Ctrl Pts',(70.7392502475469,-21.3706974057039,
0.));
#119218=CARTESIAN_POINT('Ctrl Pts',(70.7186299539724,-21.3530880842349,
0.));
#119219=CARTESIAN_POINT('Ctrl Pts',(70.6980209870044,-21.3355209732443,
0.));
#119220=CARTESIAN_POINT('Ctrl Pts',(70.6774234430897,-21.3179960943389,
0.));
#119221=CARTESIAN_POINT('Ctrl Pts',(70.6568374193774,-21.300513469156,0.));
#119222=CARTESIAN_POINT('Ctrl Pts',(70.6362630143047,-21.2830731194183,
0.));
#119223=CARTESIAN_POINT('Ctrl Pts',(70.6157003273316,-21.2656750669126,
0.));
#119224=CARTESIAN_POINT('Ctrl Pts',(70.5951494586957,-21.2483193334676,
0.));
#119225=CARTESIAN_POINT('Ctrl Pts',(70.5746105091502,-21.2310059409266,
0.));
#119226=CARTESIAN_POINT('Ctrl Pts',(70.5540835797283,-21.2137349111208,
0.));
#119227=CARTESIAN_POINT('Ctrl Pts',(70.5335687714428,-21.1965062658298,
0.));
#119228=CARTESIAN_POINT('Ctrl Pts',(70.5130661852955,-21.1793200267847,
0.));
#119229=CARTESIAN_POINT('Ctrl Pts',(70.4925759224216,-21.1621762156897,
0.));
#119230=CARTESIAN_POINT('Ctrl Pts',(70.4720980841939,-21.1450748542337,
0.));
#119231=CARTESIAN_POINT('Ctrl Pts',(70.4516327723346,-21.1280159641003,
0.));
#119232=CARTESIAN_POINT('Ctrl Pts',(70.4311800890401,-21.1109995669747,
0.));
#119233=CARTESIAN_POINT('Ctrl Pts',(70.4107401370389,-21.0940256845473,
0.));
#119234=CARTESIAN_POINT('Ctrl Pts',(70.3903130195264,-21.0770943385141,
0.));
#119235=CARTESIAN_POINT('Ctrl Pts',(70.3698988401281,-21.0602055505748,
0.));
#119236=CARTESIAN_POINT('Ctrl Pts',(70.3494977028498,-21.0433593424267,
0.));
#119237=CARTESIAN_POINT('Ctrl Pts',(70.3291097120302,-21.0265557357548,
0.));
#119238=CARTESIAN_POINT('Ctrl Pts',(70.3087349722973,-21.0097947522218,
0.));
#119239=CARTESIAN_POINT('Ctrl Pts',(70.2883735885984,-20.9930764134776,
0.));
#119240=CARTESIAN_POINT('Ctrl Pts',(70.2680256662224,-20.9764007411653,
0.));
#119241=CARTESIAN_POINT('Ctrl Pts',(70.2476913108244,-20.9597677569228,
0.));
#119242=CARTESIAN_POINT('Ctrl Pts',(70.2273706284472,-20.9431774823831,
0.));
#119243=CARTESIAN_POINT('Ctrl Pts',(70.2070637255458,-20.9266299391684,
0.));
#119244=CARTESIAN_POINT('Ctrl Pts',(70.1867707089854,-20.9101251488944,
0.));
#119245=CARTESIAN_POINT('Ctrl Pts',(70.1664916860358,-20.8936631331748,
0.));
#119246=CARTESIAN_POINT('Ctrl Pts',(70.1462267643646,-20.8772439136206,
0.));
#119247=CARTESIAN_POINT('Ctrl Pts',(70.1259760520309,-20.8608675118379,
0.));
#119248=CARTESIAN_POINT('Ctrl Pts',(70.1057396574747,-20.8445339494188,
0.));
#119249=CARTESIAN_POINT('Ctrl Pts',(70.0855176895191,-20.8282432479429,
0.));
#119250=CARTESIAN_POINT('Ctrl Pts',(70.0653102573803,-20.8119954289849,
0.));
#119251=CARTESIAN_POINT('Ctrl Pts',(70.0451174706741,-20.7957905141157,
0.));
#119252=CARTESIAN_POINT('Ctrl Pts',(70.024939439422,-20.7796285249022,0.));
#119253=CARTESIAN_POINT('Ctrl Pts',(70.0047762740568,-20.7635094829016,
0.));
#119254=CARTESIAN_POINT('Ctrl Pts',(69.9846280854257,-20.7474334096581,
0.));
#119255=CARTESIAN_POINT('Ctrl Pts',(69.9644949847934,-20.7314003267119,
0.));
#119256=CARTESIAN_POINT('Ctrl Pts',(69.9443770838448,-20.7154102555997,
0.));
#119257=CARTESIAN_POINT('Ctrl Pts',(69.9242744946854,-20.6994632178552,
0.));
#119258=CARTESIAN_POINT('Ctrl Pts',(69.904187329841,-20.683559235003,0.));
#119259=CARTESIAN_POINT('Ctrl Pts',(69.8841157022567,-20.667698328554,0.));
#119260=CARTESIAN_POINT('Ctrl Pts',(69.8640597253045,-20.6518805200129,
0.));
#119261=CARTESIAN_POINT('Ctrl Pts',(69.8440195127866,-20.6361058308811,
0.));
#119262=CARTESIAN_POINT('Ctrl Pts',(69.8239951789402,-20.6203742826566,
0.));
#119263=CARTESIAN_POINT('Ctrl Pts',(69.8039868384389,-20.6046858968308,
0.));
#119264=CARTESIAN_POINT('Ctrl Pts',(69.7839946063949,-20.5890406948811,
0.));
#119265=CARTESIAN_POINT('Ctrl Pts',(69.7640185983644,-20.5734386982783,
0.));
#119266=CARTESIAN_POINT('Ctrl Pts',(69.744058930351,-20.5578799284898,0.));
#119267=CARTESIAN_POINT('Ctrl Pts',(69.7241157188083,-20.54236440698,0.));
#119268=CARTESIAN_POINT('Ctrl Pts',(69.7041890806424,-20.5268921552077,
0.));
#119269=CARTESIAN_POINT('Ctrl Pts',(69.6842791332115,-20.5114631946185,
0.));
#119270=CARTESIAN_POINT('Ctrl Pts',(69.6643859943308,-20.4960775466492,
0.));
#119271=CARTESIAN_POINT('Ctrl Pts',(69.6445097822792,-20.480735232734,0.));
#119272=CARTESIAN_POINT('Ctrl Pts',(69.6246506158013,-20.4654362743038,
0.));
#119273=CARTESIAN_POINT('Ctrl Pts',(69.6048086141113,-20.4501806927852,
0.));
#119274=CARTESIAN_POINT('Ctrl Pts',(69.5849838968928,-20.4349685095924,
0.));
#119275=CARTESIAN_POINT('Ctrl Pts',(69.5651765843033,-20.4197997461301,
0.));
#119276=CARTESIAN_POINT('Ctrl Pts',(69.5453867969804,-20.4046744237999,
0.));
#119277=CARTESIAN_POINT('Ctrl Pts',(69.5256146560441,-20.3895925640005,
0.));
#119278=CARTESIAN_POINT('Ctrl Pts',(69.5058602831008,-20.3745541881269,
0.));
#119279=CARTESIAN_POINT('Ctrl Pts',(69.4861238002441,-20.3595593175623,
0.));
#119280=CARTESIAN_POINT('Ctrl Pts',(69.4664053300587,-20.3446079736802,
0.));
#119281=CARTESIAN_POINT('Ctrl Pts',(69.4467049956262,-20.3297001778507,
0.));
#119282=CARTESIAN_POINT('Ctrl Pts',(69.4270229205296,-20.3148359514415,
0.));
#119283=CARTESIAN_POINT('Ctrl Pts',(69.407359228856,-20.3000153158167,0.));
#119284=CARTESIAN_POINT('Ctrl Pts',(69.3877140451975,-20.2852382923299,
0.));
#119285=CARTESIAN_POINT('Ctrl Pts',(69.368087494655,-20.2705049023241,0.));
#119286=CARTESIAN_POINT('Ctrl Pts',(69.3484797028458,-20.2558151671391,
0.));
#119287=CARTESIAN_POINT('Ctrl Pts',(69.3288907959067,-20.2411691081123,
0.));
#119288=CARTESIAN_POINT('Ctrl Pts',(69.3093209004984,-20.2265667465784,
0.));
#119289=CARTESIAN_POINT('Ctrl Pts',(69.2897701438059,-20.2120081038621,
0.));
#119290=CARTESIAN_POINT('Ctrl Pts',(69.2702386535422,-20.1974932012773,
0.));
#119291=CARTESIAN_POINT('Ctrl Pts',(69.2507265579554,-20.1830220601349,
0.));
#119292=CARTESIAN_POINT('Ctrl Pts',(69.2312339858335,-20.1685947017433,
0.));
#119293=CARTESIAN_POINT('Ctrl Pts',(69.2117610665076,-20.1542111474087,
0.));
#119294=CARTESIAN_POINT('Ctrl Pts',(69.1923079298538,-20.139871418428,0.));
#119295=CARTESIAN_POINT('Ctrl Pts',(69.1728747062963,-20.1255755360872,
0.));
#119296=CARTESIAN_POINT('Ctrl Pts',(69.1534615268152,-20.1113235216694,
0.));
#119297=CARTESIAN_POINT('Ctrl Pts',(69.1340685229514,-20.0971153964557,
0.));
#119298=CARTESIAN_POINT('Ctrl Pts',(69.1146958268104,-20.0829511817251,
0.));
#119299=CARTESIAN_POINT('Ctrl Pts',(69.095343571064,-20.068830898748,0.));
#119300=CARTESIAN_POINT('Ctrl Pts',(69.0760118889535,-20.0547545687842,
0.));
#119301=CARTESIAN_POINT('Ctrl Pts',(69.0567009142978,-20.0407222130906,
0.));
#119302=CARTESIAN_POINT('Ctrl Pts',(69.0374107814984,-20.0267338529223,
0.));
#119303=CARTESIAN_POINT('Ctrl Pts',(69.0181416255431,-20.0127895095327,
0.));
#119304=CARTESIAN_POINT('Ctrl Pts',(68.9988935820084,-19.9988892041666,
0.));
#119305=CARTESIAN_POINT('Ctrl Pts',(68.9796667870638,-19.9850329580591,
0.));
#119306=CARTESIAN_POINT('Ctrl Pts',(68.9604613774802,-19.9712207924429,
0.));
#119307=CARTESIAN_POINT('Ctrl Pts',(68.9412774906333,-19.9574527285488,
0.));
#119308=CARTESIAN_POINT('Ctrl Pts',(68.9221152645095,-19.9437287876066,
0.));
#119309=CARTESIAN_POINT('Ctrl Pts',(68.9029748377067,-19.9300489908374,
0.));
#119310=CARTESIAN_POINT('Ctrl Pts',(68.8838563494393,-19.9164133594526,
0.));
#119311=CARTESIAN_POINT('Ctrl Pts',(68.8647599395469,-19.9028219146618,
0.));
#119312=CARTESIAN_POINT('Ctrl Pts',(68.8456857485002,-19.8892746776739,
0.));
#119313=CARTESIAN_POINT('Ctrl Pts',(68.8266339174056,-19.8757716696966,
0.));
#119314=CARTESIAN_POINT('Ctrl Pts',(68.8076045880065,-19.8623129119293,
0.));
#119315=CARTESIAN_POINT('Ctrl Pts',(68.7885979026878,-19.8488984255627,
0.));
#119316=CARTESIAN_POINT('Ctrl Pts',(68.7696140044851,-19.8355282317858,
0.));
#119317=CARTESIAN_POINT('Ctrl Pts',(68.7506530370904,-19.8222023517871,
0.));
#119318=CARTESIAN_POINT('Ctrl Pts',(68.7317151448573,-19.8089208067538,
0.));
#119319=CARTESIAN_POINT('Ctrl Pts',(68.7128004728033,-19.7956836178651,
0.));
#119320=CARTESIAN_POINT('Ctrl Pts',(68.6939091666149,-19.7824908062925,
0.));
#119321=CARTESIAN_POINT('Ctrl Pts',(68.6750413726574,-19.7693423932067,
0.));
#119322=CARTESIAN_POINT('Ctrl Pts',(68.65619723798,-19.7562383997784,0.));
#119323=CARTESIAN_POINT('Ctrl Pts',(68.6373769103211,-19.7431788471773,
0.));
#119324=CARTESIAN_POINT('Ctrl Pts',(68.6185805381102,-19.7301637565646,
0.));
#119325=CARTESIAN_POINT('Ctrl Pts',(68.5998082704741,-19.717193149095,0.));
#119326=CARTESIAN_POINT('Ctrl Pts',(68.5810602572474,-19.7042670459234,
0.));
#119327=CARTESIAN_POINT('Ctrl Pts',(68.5623366489776,-19.6913854682046,
0.));
#119328=CARTESIAN_POINT('Ctrl Pts',(68.543637596932,-19.6785484370929,0.));
#119329=CARTESIAN_POINT('Ctrl Pts',(68.5249632530994,-19.665755973734,0.));
#119330=CARTESIAN_POINT('Ctrl Pts',(68.5063137701986,-19.653008099269,0.));
#119331=CARTESIAN_POINT('Ctrl Pts',(68.4876893016863,-19.6403048348397,
0.));
#119332=CARTESIAN_POINT('Ctrl Pts',(68.4690900017631,-19.6276462015888,
0.));
#119333=CARTESIAN_POINT('Ctrl Pts',(68.4505160253777,-19.6150322206578,
0.));
#119334=CARTESIAN_POINT('Ctrl Pts',(68.4319675282273,-19.6024629131786,
0.));
#119335=CARTESIAN_POINT('Ctrl Pts',(68.4134446667695,-19.5899383002804,
0.));
#119336=CARTESIAN_POINT('Ctrl Pts',(68.3949475982334,-19.5774584030939,
0.));
#119337=CARTESIAN_POINT('Ctrl Pts',(68.3764764806287,-19.5650232427516,
0.));
#119338=CARTESIAN_POINT('Ctrl Pts',(68.3580314727522,-19.5526328403852,
0.));
#119339=CARTESIAN_POINT('Ctrl Pts',(68.3396127341937,-19.540287217119,0.));
#119340=CARTESIAN_POINT('Ctrl Pts',(68.3212204253415,-19.5279863940773,
0.));
#119341=CARTESIAN_POINT('Ctrl Pts',(68.3028547073862,-19.5157303923856,
0.));
#119342=CARTESIAN_POINT('Ctrl Pts',(68.2845157423233,-19.5035192331706,
0.));
#119343=CARTESIAN_POINT('Ctrl Pts',(68.2662036929531,-19.4913529375546,
0.));
#119344=CARTESIAN_POINT('Ctrl Pts',(68.2479187228815,-19.4792315266505,
0.));
#119345=CARTESIAN_POINT('Ctrl Pts',(68.2296609965461,-19.4671550215725,
0.));
#119346=CARTESIAN_POINT('Ctrl Pts',(68.2114306792366,-19.4551234434384,
0.));
#119347=CARTESIAN_POINT('Ctrl Pts',(68.193227937112,-19.4431368133718,0.));
#119348=CARTESIAN_POINT('Ctrl Pts',(68.1750529372211,-19.4311951524977,
0.));
#119349=CARTESIAN_POINT('Ctrl Pts',(68.1569058475026,-19.4192984819411,
0.));
#119350=CARTESIAN_POINT('Ctrl Pts',(68.1387868367668,-19.4074468228294,
0.));
#119351=CARTESIAN_POINT('Ctrl Pts',(68.1206960746763,-19.3956401962894,
0.));
#119352=CARTESIAN_POINT('Ctrl Pts',(68.1026337317298,-19.3838786234426,
0.));
#119353=CARTESIAN_POINT('Ctrl Pts',(68.0845999792274,-19.3721621253921,
0.));
#119354=CARTESIAN_POINT('Ctrl Pts',(68.0665949893221,-19.3604907232322,
0.));
#119355=CARTESIAN_POINT('Ctrl Pts',(68.0486189351027,-19.3488644380646,
0.));
#119356=CARTESIAN_POINT('Ctrl Pts',(68.0306719906636,-19.3372832910077,
0.));
#119357=CARTESIAN_POINT('Ctrl Pts',(68.0127543311761,-19.3257473032031,
0.));
#119358=CARTESIAN_POINT('Ctrl Pts',(67.9948661329591,-19.3142564958196,
0.));
#119359=CARTESIAN_POINT('Ctrl Pts',(67.977007573346,-19.3028108900374,0.));
#119360=CARTESIAN_POINT('Ctrl Pts',(67.959178830538,-19.2914105070283,0.));
#119361=CARTESIAN_POINT('Ctrl Pts',(67.9413800834798,-19.2800553679362,
0.));
#119362=CARTESIAN_POINT('Ctrl Pts',(67.9236115116781,-19.2687454938449,
0.));
#119363=CARTESIAN_POINT('Ctrl Pts',(67.9058732951822,-19.2574809057705,
0.));
#119364=CARTESIAN_POINT('Ctrl Pts',(67.8881656149983,-19.2462616247287,
0.));
#119365=CARTESIAN_POINT('Ctrl Pts',(67.8704886534555,-19.2350876717878,
0.));
#119366=CARTESIAN_POINT('Ctrl Pts',(67.852842594517,-19.223959068113,0.));
#119367=CARTESIAN_POINT('Ctrl Pts',(67.8352276242856,-19.2128758350336,
0.));
#119368=CARTESIAN_POINT('Ctrl Pts',(67.817643930658,-19.2018379939918,0.));
#119369=CARTESIAN_POINT('Ctrl Pts',(67.8000917023896,-19.1908455664089,
0.));
#119370=CARTESIAN_POINT('Ctrl Pts',(67.7825711283092,-19.1798985735687,
0.));
#119371=CARTESIAN_POINT('Ctrl Pts',(67.7650823965156,-19.1689970364959,
0.));
#119372=CARTESIAN_POINT('Ctrl Pts',(67.7476256934492,-19.1581409758112,
0.));
#119373=CARTESIAN_POINT('Ctrl Pts',(67.7302012056629,-19.1473304119969,
0.));
#119374=CARTESIAN_POINT('Ctrl Pts',(67.7128091219372,-19.1365653657098,
0.));
#119375=CARTESIAN_POINT('Ctrl Pts',(67.6954496350053,-19.1258458580343,
0.));
#119376=CARTESIAN_POINT('Ctrl Pts',(67.6781229440535,-19.115171910845,0.));
#119377=CARTESIAN_POINT('Ctrl Pts',(67.6608292549412,-19.1045435468345,
0.));
#119378=CARTESIAN_POINT('Ctrl Pts',(67.6435687749802,-19.0939607887492,
0.));
#119379=CARTESIAN_POINT('Ctrl Pts',(67.6263417083413,-19.0834236587115,
0.));
#119380=CARTESIAN_POINT('Ctrl Pts',(67.6091482520557,-19.0729321776287,
0.));
#119381=CARTESIAN_POINT('Ctrl Pts',(67.5919885896278,-19.0624863642425,
0.));
#119382=CARTESIAN_POINT('Ctrl Pts',(67.5748628972035,-19.0520862360414,
0.));
#119383=CARTESIAN_POINT('Ctrl Pts',(67.5577713558248,-19.0417318110721,
0.));
#119384=CARTESIAN_POINT('Ctrl Pts',(67.540714161288,-19.0314231093924,0.));
#119385=CARTESIAN_POINT('Ctrl Pts',(67.5236915360253,-19.0211601548222,
0.));
#119386=CARTESIAN_POINT('Ctrl Pts',(67.5067037372177,-19.0109429761274,
0.));
#119387=CARTESIAN_POINT('Ctrl Pts',(67.4897510316692,-19.0007716032785,
0.));
#119388=CARTESIAN_POINT('Ctrl Pts',(67.4728336719558,-18.9906460638607,
0.));
#119389=CARTESIAN_POINT('Ctrl Pts',(67.4559518744713,-18.9805663798466,
0.));
#119390=CARTESIAN_POINT('Ctrl Pts',(67.4391057908687,-18.9705325631773,
0.));
#119391=CARTESIAN_POINT('Ctrl Pts',(67.4222955062384,-18.9605446161079,
0.));
#119392=CARTESIAN_POINT('Ctrl Pts',(67.4088759498287,-18.9525909518003,
0.));
#119393=CARTESIAN_POINT('Ctrl Pts',(67.398827414689,-18.9466463414355,0.));
#119394=CARTESIAN_POINT('Ctrl Pts',(67.3921355608417,-18.942692439874,0.));
#119395=CARTESIAN_POINT('Ctrl Pts',(67.3887914263118,-18.9407177820969,
0.));
#119396=CARTESIAN_POINT('Ctrl Pts',(69.065695021045,-27.9316983239472,0.));
#119397=CARTESIAN_POINT('Ctrl Pts',(69.065695021045,-27.9316983239472,12.));
#119398=CARTESIAN_POINT('Ctrl Pts',(69.0618620884721,-27.9276214070632,
0.));
#119399=CARTESIAN_POINT('Ctrl Pts',(69.0618620884721,-27.9276214070632,
12.));
#119400=CARTESIAN_POINT('Ctrl Pts',(69.0541967851028,-27.9194718099003,
0.));
#119401=CARTESIAN_POINT('Ctrl Pts',(69.0541967851028,-27.9194718099003,
12.));
#119402=CARTESIAN_POINT('Ctrl Pts',(69.0427005153791,-27.9072601239722,
0.));
#119403=CARTESIAN_POINT('Ctrl Pts',(69.0427005153791,-27.9072601239722,
12.));
#119404=CARTESIAN_POINT('Ctrl Pts',(69.0273755265382,-27.8910032967339,
0.));
#119405=CARTESIAN_POINT('Ctrl Pts',(69.0273755265382,-27.8910032967339,
12.));
#119406=CARTESIAN_POINT('Ctrl Pts',(69.0082249138598,-27.8707246380957,
0.));
#119407=CARTESIAN_POINT('Ctrl Pts',(69.0082249138598,-27.8707246380957,
12.));
#119408=CARTESIAN_POINT('Ctrl Pts',(68.9890799392213,-27.8504883674059,
0.));
#119409=CARTESIAN_POINT('Ctrl Pts',(68.9890799392213,-27.8504883674059,
12.));
#119410=CARTESIAN_POINT('Ctrl Pts',(68.9699406311389,-27.8302945019977,
0.));
#119411=CARTESIAN_POINT('Ctrl Pts',(68.9699406311389,-27.8302945019977,
12.));
#119412=CARTESIAN_POINT('Ctrl Pts',(68.9508070357658,-27.8101430638072,
0.));
#119413=CARTESIAN_POINT('Ctrl Pts',(68.9508070357658,-27.8101430638072,
12.));
#119414=CARTESIAN_POINT('Ctrl Pts',(68.9316792225946,-27.7900340793689,
0.));
#119415=CARTESIAN_POINT('Ctrl Pts',(68.9316792225946,-27.7900340793689,
12.));
#119416=CARTESIAN_POINT('Ctrl Pts',(68.9125572825693,-27.7699675790571,
0.));
#119417=CARTESIAN_POINT('Ctrl Pts',(68.9125572825693,-27.7699675790571,
12.));
#119418=CARTESIAN_POINT('Ctrl Pts',(68.8934413203759,-27.7499435957525,
0.));
#119419=CARTESIAN_POINT('Ctrl Pts',(68.8934413203759,-27.7499435957525,
12.));
#119420=CARTESIAN_POINT('Ctrl Pts',(68.8743314483369,-27.7299621636566,
0.));
#119421=CARTESIAN_POINT('Ctrl Pts',(68.8743314483369,-27.7299621636566,
12.));
#119422=CARTESIAN_POINT('Ctrl Pts',(68.85522777982,-27.7100233170738,0.));
#119423=CARTESIAN_POINT('Ctrl Pts',(68.85522777982,-27.7100233170738,12.));
#119424=CARTESIAN_POINT('Ctrl Pts',(68.8361304224467,-27.6901270891241,
0.));
#119425=CARTESIAN_POINT('Ctrl Pts',(68.8361304224467,-27.6901270891241,
12.));
#119426=CARTESIAN_POINT('Ctrl Pts',(68.81703947259,-27.6702735107121,0.));
#119427=CARTESIAN_POINT('Ctrl Pts',(68.81703947259,-27.6702735107121,12.));
#119428=CARTESIAN_POINT('Ctrl Pts',(68.7979550191872,-27.6504626112666,
0.));
#119429=CARTESIAN_POINT('Ctrl Pts',(68.7979550191872,-27.6504626112666,
12.));
#119430=CARTESIAN_POINT('Ctrl Pts',(68.7788771464713,-27.6306944192738,
0.));
#119431=CARTESIAN_POINT('Ctrl Pts',(68.7788771464713,-27.6306944192738,
12.));
#119432=CARTESIAN_POINT('Ctrl Pts',(68.7598059372129,-27.6109689629029,
0.));
#119433=CARTESIAN_POINT('Ctrl Pts',(68.7598059372129,-27.6109689629029,
12.));
#119434=CARTESIAN_POINT('Ctrl Pts',(68.7407414755259,-27.5912862705469,
0.));
#119435=CARTESIAN_POINT('Ctrl Pts',(68.7407414755259,-27.5912862705469,
12.));
#119436=CARTESIAN_POINT('Ctrl Pts',(68.7216838504218,-27.5716463715005,
0.));
#119437=CARTESIAN_POINT('Ctrl Pts',(68.7216838504218,-27.5716463715005,
12.));
#119438=CARTESIAN_POINT('Ctrl Pts',(68.7026331554296,-27.5520492958907,
0.));
#119439=CARTESIAN_POINT('Ctrl Pts',(68.7026331554296,-27.5520492958907,
12.));
#119440=CARTESIAN_POINT('Ctrl Pts',(68.6835894869882,-27.5324950743706,
0.));
#119441=CARTESIAN_POINT('Ctrl Pts',(68.6835894869882,-27.5324950743706,
12.));
#119442=CARTESIAN_POINT('Ctrl Pts',(68.6645529432045,-27.5129837378792,
0.));
#119443=CARTESIAN_POINT('Ctrl Pts',(68.6645529432045,-27.5129837378792,
12.));
#119444=CARTESIAN_POINT('Ctrl Pts',(68.645523622548,-27.4935153173868,0.));
#119445=CARTESIAN_POINT('Ctrl Pts',(68.645523622548,-27.4935153173868,12.));
#119446=CARTESIAN_POINT('Ctrl Pts',(68.6265016223561,-27.4740898435989,
0.));
#119447=CARTESIAN_POINT('Ctrl Pts',(68.6265016223561,-27.4740898435989,
12.));
#119448=CARTESIAN_POINT('Ctrl Pts',(68.6074870381619,-27.4547073468227,
0.));
#119449=CARTESIAN_POINT('Ctrl Pts',(68.6074870381619,-27.4547073468227,
12.));
#119450=CARTESIAN_POINT('Ctrl Pts',(68.5884799645218,-27.4353678571361,
0.));
#119451=CARTESIAN_POINT('Ctrl Pts',(68.5884799645218,-27.4353678571361,
12.));
#119452=CARTESIAN_POINT('Ctrl Pts',(68.5694804955014,-27.4160714044831,
0.));
#119453=CARTESIAN_POINT('Ctrl Pts',(68.5694804955014,-27.4160714044831,
12.));
#119454=CARTESIAN_POINT('Ctrl Pts',(68.5504887252975,-27.3968180187941,
0.));
#119455=CARTESIAN_POINT('Ctrl Pts',(68.5504887252975,-27.3968180187941,
12.));
#119456=CARTESIAN_POINT('Ctrl Pts',(68.5315047488035,-27.3776077300914,
0.));
#119457=CARTESIAN_POINT('Ctrl Pts',(68.5315047488035,-27.3776077300914,
12.));
#119458=CARTESIAN_POINT('Ctrl Pts',(68.5125286621888,-27.3584405685942,
0.));
#119459=CARTESIAN_POINT('Ctrl Pts',(68.5125286621888,-27.3584405685942,
12.));
#119460=CARTESIAN_POINT('Ctrl Pts',(68.4935605626361,-27.3393165646748,
0.));
#119461=CARTESIAN_POINT('Ctrl Pts',(68.4935605626361,-27.3393165646748,
12.));
#119462=CARTESIAN_POINT('Ctrl Pts',(68.4746005480992,-27.3202357488153,
0.));
#119463=CARTESIAN_POINT('Ctrl Pts',(68.4746005480992,-27.3202357488153,
12.));
#119464=CARTESIAN_POINT('Ctrl Pts',(68.455648717044,-27.3011981515571,0.));
#119465=CARTESIAN_POINT('Ctrl Pts',(68.455648717044,-27.3011981515571,12.));
#119466=CARTESIAN_POINT('Ctrl Pts',(68.4367051682166,-27.2822038034539,
0.));
#119467=CARTESIAN_POINT('Ctrl Pts',(68.4367051682166,-27.2822038034539,
12.));
#119468=CARTESIAN_POINT('Ctrl Pts',(68.4177700003471,-27.2632527350062,
0.));
#119469=CARTESIAN_POINT('Ctrl Pts',(68.4177700003471,-27.2632527350062,
12.));
#119470=CARTESIAN_POINT('Ctrl Pts',(68.3988433121589,-27.2443449766654,
0.));
#119471=CARTESIAN_POINT('Ctrl Pts',(68.3988433121589,-27.2443449766654,
12.));
#119472=CARTESIAN_POINT('Ctrl Pts',(68.379925202511,-27.2254805588677,0.));
#119473=CARTESIAN_POINT('Ctrl Pts',(68.379925202511,-27.2254805588677,12.));
#119474=CARTESIAN_POINT('Ctrl Pts',(68.3610157704999,-27.2066595120544,
0.));
#119475=CARTESIAN_POINT('Ctrl Pts',(68.3610157704999,-27.2066595120544,
12.));
#119476=CARTESIAN_POINT('Ctrl Pts',(68.3421151155708,-27.1878818666925,
0.));
#119477=CARTESIAN_POINT('Ctrl Pts',(68.3421151155708,-27.1878818666925,
12.));
#119478=CARTESIAN_POINT('Ctrl Pts',(68.3232233376415,-27.1691476532917,
0.));
#119479=CARTESIAN_POINT('Ctrl Pts',(68.3232233376415,-27.1691476532917,
12.));
#119480=CARTESIAN_POINT('Ctrl Pts',(68.3043405371589,-27.1504569024131,
0.));
#119481=CARTESIAN_POINT('Ctrl Pts',(68.3043405371589,-27.1504569024131,
12.));
#119482=CARTESIAN_POINT('Ctrl Pts',(68.285466815035,-27.1318096446643,0.));
#119483=CARTESIAN_POINT('Ctrl Pts',(68.285466815035,-27.1318096446643,12.));
#119484=CARTESIAN_POINT('Ctrl Pts',(68.2666022726094,-27.1132059106939,
0.));
#119485=CARTESIAN_POINT('Ctrl Pts',(68.2666022726094,-27.1132059106939,
12.));
#119486=CARTESIAN_POINT('Ctrl Pts',(68.2477470116014,-27.0946457311814,
0.));
#119487=CARTESIAN_POINT('Ctrl Pts',(68.2477470116014,-27.0946457311814,
12.));
#119488=CARTESIAN_POINT('Ctrl Pts',(68.2289011340624,-27.0761291368231,
0.));
#119489=CARTESIAN_POINT('Ctrl Pts',(68.2289011340624,-27.0761291368231,
12.));
#119490=CARTESIAN_POINT('Ctrl Pts',(68.2100647423345,-27.0576561583179,
0.));
#119491=CARTESIAN_POINT('Ctrl Pts',(68.2100647423345,-27.0576561583179,
12.));
#119492=CARTESIAN_POINT('Ctrl Pts',(68.1912379390786,-27.0392268263805,
0.));
#119493=CARTESIAN_POINT('Ctrl Pts',(68.1912379390786,-27.0392268263805,
12.));
#119494=CARTESIAN_POINT('Ctrl Pts',(68.1724208272967,-27.0208411717477,
0.));
#119495=CARTESIAN_POINT('Ctrl Pts',(68.1724208272967,-27.0208411717477,
12.));
#119496=CARTESIAN_POINT('Ctrl Pts',(68.1536135103558,-27.0024992251839,
0.));
#119497=CARTESIAN_POINT('Ctrl Pts',(68.1536135103558,-27.0024992251839,
12.));
#119498=CARTESIAN_POINT('Ctrl Pts',(68.13481609201,-26.9842010174819,0.));
#119499=CARTESIAN_POINT('Ctrl Pts',(68.13481609201,-26.9842010174819,12.));
#119500=CARTESIAN_POINT('Ctrl Pts',(68.1160286764244,-26.9659465794596,
0.));
#119501=CARTESIAN_POINT('Ctrl Pts',(68.1160286764244,-26.9659465794596,
12.));
#119502=CARTESIAN_POINT('Ctrl Pts',(68.0972513681739,-26.9477359419647,
0.));
#119503=CARTESIAN_POINT('Ctrl Pts',(68.0972513681739,-26.9477359419647,
12.));
#119504=CARTESIAN_POINT('Ctrl Pts',(68.0784842722362,-26.9295691358775,
0.));
#119505=CARTESIAN_POINT('Ctrl Pts',(68.0784842722362,-26.9295691358775,
12.));
#119506=CARTESIAN_POINT('Ctrl Pts',(68.0597274939857,-26.9114461921109,
0.));
#119507=CARTESIAN_POINT('Ctrl Pts',(68.0597274939857,-26.9114461921109,
12.));
#119508=CARTESIAN_POINT('Ctrl Pts',(68.0409811391871,-26.8933671416065,
0.));
#119509=CARTESIAN_POINT('Ctrl Pts',(68.0409811391871,-26.8933671416065,
12.));
#119510=CARTESIAN_POINT('Ctrl Pts',(68.0222453139862,-26.8753320153255,
0.));
#119511=CARTESIAN_POINT('Ctrl Pts',(68.0222453139862,-26.8753320153255,
12.));
#119512=CARTESIAN_POINT('Ctrl Pts',(68.0035201249108,-26.85734084425,0.));
#119513=CARTESIAN_POINT('Ctrl Pts',(68.0035201249108,-26.85734084425,12.));
#119514=CARTESIAN_POINT('Ctrl Pts',(67.9848056788814,-26.8393936593914,
0.));
#119515=CARTESIAN_POINT('Ctrl Pts',(67.9848056788814,-26.8393936593914,
12.));
#119516=CARTESIAN_POINT('Ctrl Pts',(67.9661020832165,-26.8214904917922,
0.));
#119517=CARTESIAN_POINT('Ctrl Pts',(67.9661020832165,-26.8214904917922,
12.));
#119518=CARTESIAN_POINT('Ctrl Pts',(67.9474094456395,-26.8036313725262,
0.));
#119519=CARTESIAN_POINT('Ctrl Pts',(67.9474094456395,-26.8036313725262,
12.));
#119520=CARTESIAN_POINT('Ctrl Pts',(67.9287278742839,-26.7858163326933,
0.));
#119521=CARTESIAN_POINT('Ctrl Pts',(67.9287278742839,-26.7858163326933,
12.));
#119522=CARTESIAN_POINT('Ctrl Pts',(67.9100574776974,-26.7680454034169,
0.));
#119523=CARTESIAN_POINT('Ctrl Pts',(67.9100574776974,-26.7680454034169,
12.));
#119524=CARTESIAN_POINT('Ctrl Pts',(67.8913983648441,-26.7503186158524,
0.));
#119525=CARTESIAN_POINT('Ctrl Pts',(67.8913983648441,-26.7503186158524,
12.));
#119526=CARTESIAN_POINT('Ctrl Pts',(67.8727506451067,-26.7326360011886,
0.));
#119527=CARTESIAN_POINT('Ctrl Pts',(67.8727506451067,-26.7326360011886,
12.));
#119528=CARTESIAN_POINT('Ctrl Pts',(67.8541144282875,-26.7149975906478,
0.));
#119529=CARTESIAN_POINT('Ctrl Pts',(67.8541144282875,-26.7149975906478,
12.));
#119530=CARTESIAN_POINT('Ctrl Pts',(67.8354898246079,-26.6974034154803,
0.));
#119531=CARTESIAN_POINT('Ctrl Pts',(67.8354898246079,-26.6974034154803,
12.));
#119532=CARTESIAN_POINT('Ctrl Pts',(67.8168769447086,-26.6798535069586,
0.));
#119533=CARTESIAN_POINT('Ctrl Pts',(67.8168769447086,-26.6798535069586,
12.));
#119534=CARTESIAN_POINT('Ctrl Pts',(67.7982758996557,-26.6623478963867,
0.));
#119535=CARTESIAN_POINT('Ctrl Pts',(67.7982758996557,-26.6623478963867,
12.));
#119536=CARTESIAN_POINT('Ctrl Pts',(67.7796868009447,-26.6448866151027,
0.));
#119537=CARTESIAN_POINT('Ctrl Pts',(67.7796868009447,-26.6448866151027,
12.));
#119538=CARTESIAN_POINT('Ctrl Pts',(67.7611097605042,-26.6274696944793,
0.));
#119539=CARTESIAN_POINT('Ctrl Pts',(67.7611097605042,-26.6274696944793,
12.));
#119540=CARTESIAN_POINT('Ctrl Pts',(67.7425448906983,-26.6100971659205,
0.));
#119541=CARTESIAN_POINT('Ctrl Pts',(67.7425448906983,-26.6100971659205,
12.));
#119542=CARTESIAN_POINT('Ctrl Pts',(67.7239923043295,-26.5927690608547,
0.));
#119543=CARTESIAN_POINT('Ctrl Pts',(67.7239923043295,-26.5927690608547,
12.));
#119544=CARTESIAN_POINT('Ctrl Pts',(67.7054521146427,-26.5754854107422,
0.));
#119545=CARTESIAN_POINT('Ctrl Pts',(67.7054521146427,-26.5754854107422,
12.));
#119546=CARTESIAN_POINT('Ctrl Pts',(67.6869244353292,-26.5582462470794,
0.));
#119547=CARTESIAN_POINT('Ctrl Pts',(67.6869244353292,-26.5582462470794,
12.));
#119548=CARTESIAN_POINT('Ctrl Pts',(67.6684093805288,-26.5410516013984,
0.));
#119549=CARTESIAN_POINT('Ctrl Pts',(67.6684093805288,-26.5410516013984,
12.));
#119550=CARTESIAN_POINT('Ctrl Pts',(67.6499070648323,-26.5239015052656,
0.));
#119551=CARTESIAN_POINT('Ctrl Pts',(67.6499070648323,-26.5239015052656,
12.));
#119552=CARTESIAN_POINT('Ctrl Pts',(67.6314176032823,-26.5067959902731,
0.));
#119553=CARTESIAN_POINT('Ctrl Pts',(67.6314176032823,-26.5067959902731,
12.));
#119554=CARTESIAN_POINT('Ctrl Pts',(67.6129411113774,-26.4897350880447,
0.));
#119555=CARTESIAN_POINT('Ctrl Pts',(67.6129411113774,-26.4897350880447,
12.));
#119556=CARTESIAN_POINT('Ctrl Pts',(67.5944777050782,-26.4727188302415,
0.));
#119557=CARTESIAN_POINT('Ctrl Pts',(67.5944777050782,-26.4727188302415,
12.));
#119558=CARTESIAN_POINT('Ctrl Pts',(67.5760275008096,-26.4557472485622,
0.));
#119559=CARTESIAN_POINT('Ctrl Pts',(67.5760275008096,-26.4557472485622,
12.));
#119560=CARTESIAN_POINT('Ctrl Pts',(67.5575906154648,-26.4388203747422,
0.));
#119561=CARTESIAN_POINT('Ctrl Pts',(67.5575906154648,-26.4388203747422,
12.));
#119562=CARTESIAN_POINT('Ctrl Pts',(67.5391671664055,-26.4219382405452,
0.));
#119563=CARTESIAN_POINT('Ctrl Pts',(67.5391671664055,-26.4219382405452,
12.));
#119564=CARTESIAN_POINT('Ctrl Pts',(67.5207572714666,-26.4051008777669,
0.));
#119565=CARTESIAN_POINT('Ctrl Pts',(67.5207572714666,-26.4051008777669,
12.));
#119566=CARTESIAN_POINT('Ctrl Pts',(67.5023610489611,-26.3883083182417,
0.));
#119567=CARTESIAN_POINT('Ctrl Pts',(67.5023610489611,-26.3883083182417,
12.));
#119568=CARTESIAN_POINT('Ctrl Pts',(67.4839786176833,-26.3715605938432,
0.));
#119569=CARTESIAN_POINT('Ctrl Pts',(67.4839786176833,-26.3715605938432,
12.));
#119570=CARTESIAN_POINT('Ctrl Pts',(67.4656100969121,-26.3548577364835,
0.));
#119571=CARTESIAN_POINT('Ctrl Pts',(67.4656100969121,-26.3548577364835,
12.));
#119572=CARTESIAN_POINT('Ctrl Pts',(67.4472556064127,-26.3381997781059,
0.));
#119573=CARTESIAN_POINT('Ctrl Pts',(67.4472556064127,-26.3381997781059,
12.));
#119574=CARTESIAN_POINT('Ctrl Pts',(67.4289152664406,-26.3215867506864,
0.));
#119575=CARTESIAN_POINT('Ctrl Pts',(67.4289152664406,-26.3215867506864,
12.));
#119576=CARTESIAN_POINT('Ctrl Pts',(67.4105891977465,-26.305018686241,0.));
#119577=CARTESIAN_POINT('Ctrl Pts',(67.4105891977465,-26.305018686241,12.));
#119578=CARTESIAN_POINT('Ctrl Pts',(67.392277521581,-26.2884956168271,0.));
#119579=CARTESIAN_POINT('Ctrl Pts',(67.392277521581,-26.2884956168271,12.));
#119580=CARTESIAN_POINT('Ctrl Pts',(67.3739803596967,-26.2720175745423,
0.));
#119581=CARTESIAN_POINT('Ctrl Pts',(67.3739803596967,-26.2720175745423,
12.));
#119582=CARTESIAN_POINT('Ctrl Pts',(67.3556978343506,-26.255584591518,0.));
#119583=CARTESIAN_POINT('Ctrl Pts',(67.3556978343506,-26.255584591518,12.));
#119584=CARTESIAN_POINT('Ctrl Pts',(67.3374300683076,-26.2391966999192,
0.));
#119585=CARTESIAN_POINT('Ctrl Pts',(67.3374300683076,-26.2391966999192,
12.));
#119586=CARTESIAN_POINT('Ctrl Pts',(67.3191771848468,-26.2228539319528,
0.));
#119587=CARTESIAN_POINT('Ctrl Pts',(67.3191771848468,-26.2228539319528,
12.));
#119588=CARTESIAN_POINT('Ctrl Pts',(67.3009393077654,-26.2065563198685,
0.));
#119589=CARTESIAN_POINT('Ctrl Pts',(67.3009393077654,-26.2065563198685,
12.));
#119590=CARTESIAN_POINT('Ctrl Pts',(67.2827165613828,-26.1903038959589,
0.));
#119591=CARTESIAN_POINT('Ctrl Pts',(67.2827165613828,-26.1903038959589,
12.));
#119592=CARTESIAN_POINT('Ctrl Pts',(67.2645090705414,-26.1740966925527,
0.));
#119593=CARTESIAN_POINT('Ctrl Pts',(67.2645090705414,-26.1740966925527,
12.));
#119594=CARTESIAN_POINT('Ctrl Pts',(67.2463169606105,-26.1579347420135,
0.));
#119595=CARTESIAN_POINT('Ctrl Pts',(67.2463169606105,-26.1579347420135,
12.));
#119596=CARTESIAN_POINT('Ctrl Pts',(67.228140357493,-26.1418180767487,0.));
#119597=CARTESIAN_POINT('Ctrl Pts',(67.228140357493,-26.1418180767487,12.));
#119598=CARTESIAN_POINT('Ctrl Pts',(67.2099793876295,-26.1257467292102,
0.));
#119599=CARTESIAN_POINT('Ctrl Pts',(67.2099793876295,-26.1257467292102,
12.));
#119600=CARTESIAN_POINT('Ctrl Pts',(67.191834178002,-26.109720731895,0.));
#119601=CARTESIAN_POINT('Ctrl Pts',(67.191834178002,-26.109720731895,12.));
#119602=CARTESIAN_POINT('Ctrl Pts',(67.1737048561364,-26.0937401173385,
0.));
#119603=CARTESIAN_POINT('Ctrl Pts',(67.1737048561364,-26.0937401173385,
12.));
#119604=CARTESIAN_POINT('Ctrl Pts',(67.1555915501052,-26.077804918113,0.));
#119605=CARTESIAN_POINT('Ctrl Pts',(67.1555915501052,-26.077804918113,12.));
#119606=CARTESIAN_POINT('Ctrl Pts',(67.1374943885353,-26.0619151668361,
0.));
#119607=CARTESIAN_POINT('Ctrl Pts',(67.1374943885353,-26.0619151668361,
12.));
#119608=CARTESIAN_POINT('Ctrl Pts',(67.1194135006122,-26.0460708961725,
0.));
#119609=CARTESIAN_POINT('Ctrl Pts',(67.1194135006122,-26.0460708961725,
12.));
#119610=CARTESIAN_POINT('Ctrl Pts',(67.101349016084,-26.030272138834,0.));
#119611=CARTESIAN_POINT('Ctrl Pts',(67.101349016084,-26.030272138834,12.));
#119612=CARTESIAN_POINT('Ctrl Pts',(67.083301065264,-26.0145189275733,0.));
#119613=CARTESIAN_POINT('Ctrl Pts',(67.083301065264,-26.0145189275733,12.));
#119614=CARTESIAN_POINT('Ctrl Pts',(67.0652697790335,-25.9988112951819,
0.));
#119615=CARTESIAN_POINT('Ctrl Pts',(67.0652697790335,-25.9988112951819,
12.));
#119616=CARTESIAN_POINT('Ctrl Pts',(67.0472552888495,-25.9831492744988,
0.));
#119617=CARTESIAN_POINT('Ctrl Pts',(67.0472552888495,-25.9831492744988,
12.));
#119618=CARTESIAN_POINT('Ctrl Pts',(67.0292577267495,-25.9675328984123,
0.));
#119619=CARTESIAN_POINT('Ctrl Pts',(67.0292577267495,-25.9675328984123,
12.));
#119620=CARTESIAN_POINT('Ctrl Pts',(67.0112772253553,-25.9519621998598,
0.));
#119621=CARTESIAN_POINT('Ctrl Pts',(67.0112772253553,-25.9519621998598,
12.));
#119622=CARTESIAN_POINT('Ctrl Pts',(66.993313917876,-25.9364372118216,0.));
#119623=CARTESIAN_POINT('Ctrl Pts',(66.993313917876,-25.9364372118216,12.));
#119624=CARTESIAN_POINT('Ctrl Pts',(66.9753679381122,-25.9209579673198,
0.));
#119625=CARTESIAN_POINT('Ctrl Pts',(66.9753679381122,-25.9209579673198,
12.));
#119626=CARTESIAN_POINT('Ctrl Pts',(66.9574394204635,-25.9055244994267,
0.));
#119627=CARTESIAN_POINT('Ctrl Pts',(66.9574394204635,-25.9055244994267,
12.));
#119628=CARTESIAN_POINT('Ctrl Pts',(66.9395284999327,-25.8901368412655,
0.));
#119629=CARTESIAN_POINT('Ctrl Pts',(66.9395284999327,-25.8901368412655,
12.));
#119630=CARTESIAN_POINT('Ctrl Pts',(66.9216353121308,-25.8747950260115,
0.));
#119631=CARTESIAN_POINT('Ctrl Pts',(66.9216353121308,-25.8747950260115,
12.));
#119632=CARTESIAN_POINT('Ctrl Pts',(66.9037599932787,-25.8594990868845,
0.));
#119633=CARTESIAN_POINT('Ctrl Pts',(66.9037599932787,-25.8594990868845,
12.));
#119634=CARTESIAN_POINT('Ctrl Pts',(66.8859026802123,-25.8442490571486,
0.));
#119635=CARTESIAN_POINT('Ctrl Pts',(66.8859026802123,-25.8442490571486,
12.));
#119636=CARTESIAN_POINT('Ctrl Pts',(66.8680635103907,-25.8290449701207,
0.));
#119637=CARTESIAN_POINT('Ctrl Pts',(66.8680635103907,-25.8290449701207,
12.));
#119638=CARTESIAN_POINT('Ctrl Pts',(66.8502426219015,-25.8138868591715,
0.));
#119639=CARTESIAN_POINT('Ctrl Pts',(66.8502426219015,-25.8138868591715,
12.));
#119640=CARTESIAN_POINT('Ctrl Pts',(66.8324401534657,-25.7987747577265,
0.));
#119641=CARTESIAN_POINT('Ctrl Pts',(66.8324401534657,-25.7987747577265,
12.));
#119642=CARTESIAN_POINT('Ctrl Pts',(66.8146562444397,-25.7837086992581,
0.));
#119643=CARTESIAN_POINT('Ctrl Pts',(66.8146562444397,-25.7837086992581,
12.));
#119644=CARTESIAN_POINT('Ctrl Pts',(66.7968910348199,-25.7686887172859,
0.));
#119645=CARTESIAN_POINT('Ctrl Pts',(66.7968910348199,-25.7686887172859,
12.));
#119646=CARTESIAN_POINT('Ctrl Pts',(66.7791446652505,-25.7537148453848,
0.));
#119647=CARTESIAN_POINT('Ctrl Pts',(66.7791446652505,-25.7537148453848,
12.));
#119648=CARTESIAN_POINT('Ctrl Pts',(66.7614172770302,-25.7387871171861,
0.));
#119649=CARTESIAN_POINT('Ctrl Pts',(66.7614172770302,-25.7387871171861,
12.));
#119650=CARTESIAN_POINT('Ctrl Pts',(66.7437090121168,-25.7239055663778,
0.));
#119651=CARTESIAN_POINT('Ctrl Pts',(66.7437090121168,-25.7239055663778,
12.));
#119652=CARTESIAN_POINT('Ctrl Pts',(66.72602001313,-25.7090702266976,0.));
#119653=CARTESIAN_POINT('Ctrl Pts',(66.72602001313,-25.7090702266976,12.));
#119654=CARTESIAN_POINT('Ctrl Pts',(66.7083504233566,-25.6942811319337,
0.));
#119655=CARTESIAN_POINT('Ctrl Pts',(66.7083504233566,-25.6942811319337,
12.));
#119656=CARTESIAN_POINT('Ctrl Pts',(66.6907003867599,-25.679538315933,0.));
#119657=CARTESIAN_POINT('Ctrl Pts',(66.6907003867599,-25.679538315933,12.));
#119658=CARTESIAN_POINT('Ctrl Pts',(66.6730700479843,-25.6648418126016,
0.));
#119659=CARTESIAN_POINT('Ctrl Pts',(66.6730700479843,-25.6648418126016,
12.));
#119660=CARTESIAN_POINT('Ctrl Pts',(66.6554595523611,-25.6501916559051,
0.));
#119661=CARTESIAN_POINT('Ctrl Pts',(66.6554595523611,-25.6501916559051,
12.));
#119662=CARTESIAN_POINT('Ctrl Pts',(66.6378690459105,-25.6355878798605,
0.));
#119663=CARTESIAN_POINT('Ctrl Pts',(66.6378690459105,-25.6355878798605,
12.));
#119664=CARTESIAN_POINT('Ctrl Pts',(66.6202986753482,-25.6210305185395,
0.));
#119665=CARTESIAN_POINT('Ctrl Pts',(66.6202986753482,-25.6210305185395,
12.));
#119666=CARTESIAN_POINT('Ctrl Pts',(66.6027485880947,-25.6065196060751,
0.));
#119667=CARTESIAN_POINT('Ctrl Pts',(66.6027485880947,-25.6065196060751,
12.));
#119668=CARTESIAN_POINT('Ctrl Pts',(66.585218932281,-25.5920551766629,0.));
#119669=CARTESIAN_POINT('Ctrl Pts',(66.585218932281,-25.5920551766629,12.));
#119670=CARTESIAN_POINT('Ctrl Pts',(66.567709856755,-25.5776372645605,0.));
#119671=CARTESIAN_POINT('Ctrl Pts',(66.567709856755,-25.5776372645605,12.));
#119672=CARTESIAN_POINT('Ctrl Pts',(66.5502215110843,-25.5632659040797,
0.));
#119673=CARTESIAN_POINT('Ctrl Pts',(66.5502215110843,-25.5632659040797,
12.));
#119674=CARTESIAN_POINT('Ctrl Pts',(66.5327540455638,-25.5489411295917,
0.));
#119675=CARTESIAN_POINT('Ctrl Pts',(66.5327540455638,-25.5489411295917,
12.));
#119676=CARTESIAN_POINT('Ctrl Pts',(66.5153076112237,-25.5346629755323,
0.));
#119677=CARTESIAN_POINT('Ctrl Pts',(66.5153076112237,-25.5346629755323,
12.));
#119678=CARTESIAN_POINT('Ctrl Pts',(66.4978823598352,-25.5204314764033,
0.));
#119679=CARTESIAN_POINT('Ctrl Pts',(66.4978823598352,-25.5204314764033,
12.));
#119680=CARTESIAN_POINT('Ctrl Pts',(66.4804784439146,-25.5062466667703,
0.));
#119681=CARTESIAN_POINT('Ctrl Pts',(66.4804784439146,-25.5062466667703,
12.));
#119682=CARTESIAN_POINT('Ctrl Pts',(66.463096016725,-25.4921085812548,0.));
#119683=CARTESIAN_POINT('Ctrl Pts',(66.463096016725,-25.4921085812548,12.));
#119684=CARTESIAN_POINT('Ctrl Pts',(66.445735232287,-25.4780172545418,0.));
#119685=CARTESIAN_POINT('Ctrl Pts',(66.445735232287,-25.4780172545418,12.));
#119686=CARTESIAN_POINT('Ctrl Pts',(66.4283962453899,-25.463972721385,0.));
#119687=CARTESIAN_POINT('Ctrl Pts',(66.4283962453899,-25.463972721385,12.));
#119688=CARTESIAN_POINT('Ctrl Pts',(66.4110792116,-25.4499750166079,0.));
#119689=CARTESIAN_POINT('Ctrl Pts',(66.4110792116,-25.4499750166079,12.));
#119690=CARTESIAN_POINT('Ctrl Pts',(66.3937842872684,-25.4360241751017,
0.));
#119691=CARTESIAN_POINT('Ctrl Pts',(66.3937842872684,-25.4360241751017,
12.));
#119692=CARTESIAN_POINT('Ctrl Pts',(66.3765116295363,-25.4221202318198,
0.));
#119693=CARTESIAN_POINT('Ctrl Pts',(66.3765116295363,-25.4221202318198,
12.));
#119694=CARTESIAN_POINT('Ctrl Pts',(66.3592613963407,-25.4082632217846,
0.));
#119695=CARTESIAN_POINT('Ctrl Pts',(66.3592613963407,-25.4082632217846,
12.));
#119696=CARTESIAN_POINT('Ctrl Pts',(66.3420337464176,-25.3944531800901,
0.));
#119697=CARTESIAN_POINT('Ctrl Pts',(66.3420337464176,-25.3944531800901,
12.));
#119698=CARTESIAN_POINT('Ctrl Pts',(66.3248288393046,-25.3806901419013,
0.));
#119699=CARTESIAN_POINT('Ctrl Pts',(66.3248288393046,-25.3806901419013,
12.));
#119700=CARTESIAN_POINT('Ctrl Pts',(66.3076468353417,-25.3669741424491,
0.));
#119701=CARTESIAN_POINT('Ctrl Pts',(66.3076468353417,-25.3669741424491,
12.));
#119702=CARTESIAN_POINT('Ctrl Pts',(66.2904878956721,-25.3533052170254,
0.));
#119703=CARTESIAN_POINT('Ctrl Pts',(66.2904878956721,-25.3533052170254,
12.));
#119704=CARTESIAN_POINT('Ctrl Pts',(66.2733521822675,-25.3396834009955,
0.));
#119705=CARTESIAN_POINT('Ctrl Pts',(66.2733521822675,-25.3396834009955,
12.));
#119706=CARTESIAN_POINT('Ctrl Pts',(66.2562398579479,-25.326108729803,0.));
#119707=CARTESIAN_POINT('Ctrl Pts',(66.2562398579479,-25.326108729803,12.));
#119708=CARTESIAN_POINT('Ctrl Pts',(66.2391510863992,-25.3125812389728,
0.));
#119709=CARTESIAN_POINT('Ctrl Pts',(66.2391510863992,-25.3125812389728,
12.));
#119710=CARTESIAN_POINT('Ctrl Pts',(66.2220860321931,-25.2991009641087,
0.));
#119711=CARTESIAN_POINT('Ctrl Pts',(66.2220860321931,-25.2991009641087,
12.));
#119712=CARTESIAN_POINT('Ctrl Pts',(66.2050448607883,-25.2856679408921,
0.));
#119713=CARTESIAN_POINT('Ctrl Pts',(66.2050448607883,-25.2856679408921,
12.));
#119714=CARTESIAN_POINT('Ctrl Pts',(66.1880277385114,-25.2722822050829,
0.));
#119715=CARTESIAN_POINT('Ctrl Pts',(66.1880277385114,-25.2722822050829,
12.));
#119716=CARTESIAN_POINT('Ctrl Pts',(66.1710348325378,-25.2589437925145,
0.));
#119717=CARTESIAN_POINT('Ctrl Pts',(66.1710348325378,-25.2589437925145,
12.));
#119718=CARTESIAN_POINT('Ctrl Pts',(66.1540663108767,-25.245652739088,0.));
#119719=CARTESIAN_POINT('Ctrl Pts',(66.1540663108767,-25.245652739088,12.));
#119720=CARTESIAN_POINT('Ctrl Pts',(66.1371223423371,-25.2324090807561,
0.));
#119721=CARTESIAN_POINT('Ctrl Pts',(66.1371223423371,-25.2324090807561,
12.));
#119722=CARTESIAN_POINT('Ctrl Pts',(66.1202030965784,-25.2192128535367,
0.));
#119723=CARTESIAN_POINT('Ctrl Pts',(66.1202030965784,-25.2192128535367,
12.));
#119724=CARTESIAN_POINT('Ctrl Pts',(66.1033087441916,-25.2060640935372,
0.));
#119725=CARTESIAN_POINT('Ctrl Pts',(66.1033087441916,-25.2060640935372,
12.));
#119726=CARTESIAN_POINT('Ctrl Pts',(66.086439456768,-25.1929628369685,0.));
#119727=CARTESIAN_POINT('Ctrl Pts',(66.086439456768,-25.1929628369685,12.));
#119728=CARTESIAN_POINT('Ctrl Pts',(66.0695954069698,-25.1799091201594,
0.));
#119729=CARTESIAN_POINT('Ctrl Pts',(66.0695954069698,-25.1799091201594,
12.));
#119730=CARTESIAN_POINT('Ctrl Pts',(66.0527767686,-25.1669029795652,0.));
#119731=CARTESIAN_POINT('Ctrl Pts',(66.0527767686,-25.1669029795652,12.));
#119732=CARTESIAN_POINT('Ctrl Pts',(66.0359837164709,-25.153944451741,0.));
#119733=CARTESIAN_POINT('Ctrl Pts',(66.0359837164709,-25.153944451741,12.));
#119734=CARTESIAN_POINT('Ctrl Pts',(66.0192164262607,-25.1410335733094,
0.));
#119735=CARTESIAN_POINT('Ctrl Pts',(66.0192164262607,-25.1410335733094,
12.));
#119736=CARTESIAN_POINT('Ctrl Pts',(66.0024750743902,-25.12817038093,0.));
#119737=CARTESIAN_POINT('Ctrl Pts',(66.0024750743902,-25.12817038093,12.));
#119738=CARTESIAN_POINT('Ctrl Pts',(65.9857598378455,-25.1153549112512,
0.));
#119739=CARTESIAN_POINT('Ctrl Pts',(65.9857598378455,-25.1153549112512,
12.));
#119740=CARTESIAN_POINT('Ctrl Pts',(65.9690708941591,-25.1025872009016,
0.));
#119741=CARTESIAN_POINT('Ctrl Pts',(65.9690708941591,-25.1025872009016,
12.));
#119742=CARTESIAN_POINT('Ctrl Pts',(65.9524084218167,-25.0898672865926,
0.));
#119743=CARTESIAN_POINT('Ctrl Pts',(65.9524084218167,-25.0898672865926,
12.));
#119744=CARTESIAN_POINT('Ctrl Pts',(65.9357726006174,-25.0771952052033,
0.));
#119745=CARTESIAN_POINT('Ctrl Pts',(65.9357726006174,-25.0771952052033,
12.));
#119746=CARTESIAN_POINT('Ctrl Pts',(65.9191636119796,-25.0645709938519,
0.));
#119747=CARTESIAN_POINT('Ctrl Pts',(65.9191636119796,-25.0645709938519,
12.));
#119748=CARTESIAN_POINT('Ctrl Pts',(65.9025816394391,-25.0519946900066,
0.));
#119749=CARTESIAN_POINT('Ctrl Pts',(65.9025816394391,-25.0519946900066,
12.));
#119750=CARTESIAN_POINT('Ctrl Pts',(65.8860268683088,-25.039466331404,0.));
#119751=CARTESIAN_POINT('Ctrl Pts',(65.8860268683088,-25.039466331404,12.));
#119752=CARTESIAN_POINT('Ctrl Pts',(65.8694994847587,-25.0269859558351,
0.));
#119753=CARTESIAN_POINT('Ctrl Pts',(65.8694994847587,-25.0269859558351,
12.));
#119754=CARTESIAN_POINT('Ctrl Pts',(65.8529996750441,-25.0145536009604,
0.));
#119755=CARTESIAN_POINT('Ctrl Pts',(65.8529996750441,-25.0145536009604,
12.));
#119756=CARTESIAN_POINT('Ctrl Pts',(65.8365276247157,-25.0021693041181,
0.));
#119757=CARTESIAN_POINT('Ctrl Pts',(65.8365276247157,-25.0021693041181,
12.));
#119758=CARTESIAN_POINT('Ctrl Pts',(65.8200835177071,-24.9898331021002,
0.));
#119759=CARTESIAN_POINT('Ctrl Pts',(65.8200835177071,-24.9898331021002,
12.));
#119760=CARTESIAN_POINT('Ctrl Pts',(65.8036675380761,-24.97754503157,0.));
#119761=CARTESIAN_POINT('Ctrl Pts',(65.8036675380761,-24.97754503157,12.));
#119762=CARTESIAN_POINT('Ctrl Pts',(65.7872798720847,-24.965305129559,0.));
#119763=CARTESIAN_POINT('Ctrl Pts',(65.7872798720847,-24.965305129559,12.));
#119764=CARTESIAN_POINT('Ctrl Pts',(65.7709207098949,-24.9531134338693,
0.));
#119765=CARTESIAN_POINT('Ctrl Pts',(65.7709207098949,-24.9531134338693,
12.));
#119766=CARTESIAN_POINT('Ctrl Pts',(65.7545902480286,-24.9409699836524,
0.));
#119767=CARTESIAN_POINT('Ctrl Pts',(65.7545902480286,-24.9409699836524,
12.));
#119768=CARTESIAN_POINT('Ctrl Pts',(65.7382886895839,-24.9288748194562,
0.));
#119769=CARTESIAN_POINT('Ctrl Pts',(65.7382886895839,-24.9288748194562,
12.));
#119770=CARTESIAN_POINT('Ctrl Pts',(65.7220162391016,-24.9168279820093,
0.));
#119771=CARTESIAN_POINT('Ctrl Pts',(65.7220162391016,-24.9168279820093,
12.));
#119772=CARTESIAN_POINT('Ctrl Pts',(65.7057730980471,-24.9048295111444,
0.));
#119773=CARTESIAN_POINT('Ctrl Pts',(65.7057730980471,-24.9048295111444,
12.));
#119774=CARTESIAN_POINT('Ctrl Pts',(65.6895594608798,-24.8928794448616,
0.));
#119775=CARTESIAN_POINT('Ctrl Pts',(65.6895594608798,-24.8928794448616,
12.));
#119776=CARTESIAN_POINT('Ctrl Pts',(65.6733755087723,-24.8809778178248,
0.));
#119777=CARTESIAN_POINT('Ctrl Pts',(65.6733755087723,-24.8809778178248,
12.));
#119778=CARTESIAN_POINT('Ctrl Pts',(65.6572214156761,-24.8691246628081,
0.));
#119779=CARTESIAN_POINT('Ctrl Pts',(65.6572214156761,-24.8691246628081,
12.));
#119780=CARTESIAN_POINT('Ctrl Pts',(65.6410973603713,-24.8573200135684,
0.));
#119781=CARTESIAN_POINT('Ctrl Pts',(65.6410973603713,-24.8573200135684,
12.));
#119782=CARTESIAN_POINT('Ctrl Pts',(65.6250035361612,-24.8455639071517,
0.));
#119783=CARTESIAN_POINT('Ctrl Pts',(65.6250035361612,-24.8455639071517,
12.));
#119784=CARTESIAN_POINT('Ctrl Pts',(65.6089401625551,-24.8338563866739,
0.));
#119785=CARTESIAN_POINT('Ctrl Pts',(65.6089401625551,-24.8338563866739,
12.));
#119786=CARTESIAN_POINT('Ctrl Pts',(65.5929074932487,-24.8221975032059,
0.));
#119787=CARTESIAN_POINT('Ctrl Pts',(65.5929074932487,-24.8221975032059,
12.));
#119788=CARTESIAN_POINT('Ctrl Pts',(65.5769057914184,-24.8105873098578,
0.));
#119789=CARTESIAN_POINT('Ctrl Pts',(65.5769057914184,-24.8105873098578,
12.));
#119790=CARTESIAN_POINT('Ctrl Pts',(65.5609353062749,-24.7990258561234,
0.));
#119791=CARTESIAN_POINT('Ctrl Pts',(65.5609353062749,-24.7990258561234,
12.));
#119792=CARTESIAN_POINT('Ctrl Pts',(65.5449962514735,-24.7875131827515,
0.));
#119793=CARTESIAN_POINT('Ctrl Pts',(65.5449962514735,-24.7875131827515,
12.));
#119794=CARTESIAN_POINT('Ctrl Pts',(65.5290887770493,-24.7760493148551,
0.));
#119795=CARTESIAN_POINT('Ctrl Pts',(65.5290887770493,-24.7760493148551,
12.));
#119796=CARTESIAN_POINT('Ctrl Pts',(65.5132129675727,-24.764634262097,0.));
#119797=CARTESIAN_POINT('Ctrl Pts',(65.5132129675727,-24.764634262097,12.));
#119798=CARTESIAN_POINT('Ctrl Pts',(65.5005376841469,-24.7555412724771,
0.));
#119799=CARTESIAN_POINT('Ctrl Pts',(65.5005376841469,-24.7555412724771,
12.));
#119800=CARTESIAN_POINT('Ctrl Pts',(65.4910454936487,-24.7487434956058,
0.));
#119801=CARTESIAN_POINT('Ctrl Pts',(65.4910454936487,-24.7487434956058,
12.));
#119802=CARTESIAN_POINT('Ctrl Pts',(65.484723709553,-24.7442214063411,0.));
#119803=CARTESIAN_POINT('Ctrl Pts',(65.484723709553,-24.7442214063411,12.));
#119804=CARTESIAN_POINT('Ctrl Pts',(65.4815644032299,-24.7419628022042,
0.));
#119805=CARTESIAN_POINT('Ctrl Pts',(65.4815644032299,-24.7419628022042,
12.));
#119806=CARTESIAN_POINT('',(65.4815644032299,-24.7419628022042,12.));
#119807=CARTESIAN_POINT('Ctrl Pts',(65.4815644032299,-24.7419628022042,
12.));
#119808=CARTESIAN_POINT('Ctrl Pts',(65.484723709553,-24.7442214063411,12.));
#119809=CARTESIAN_POINT('Ctrl Pts',(65.4910454936487,-24.7487434956058,
12.));
#119810=CARTESIAN_POINT('Ctrl Pts',(65.5005376841469,-24.7555412724771,
12.));
#119811=CARTESIAN_POINT('Ctrl Pts',(65.5132129675727,-24.764634262097,12.));
#119812=CARTESIAN_POINT('Ctrl Pts',(65.5290887770493,-24.7760493148551,
12.));
#119813=CARTESIAN_POINT('Ctrl Pts',(65.5449962514735,-24.7875131827515,
12.));
#119814=CARTESIAN_POINT('Ctrl Pts',(65.5609353062749,-24.7990258561234,
12.));
#119815=CARTESIAN_POINT('Ctrl Pts',(65.5769057914184,-24.8105873098578,
12.));
#119816=CARTESIAN_POINT('Ctrl Pts',(65.5929074932487,-24.8221975032059,
12.));
#119817=CARTESIAN_POINT('Ctrl Pts',(65.6089401625551,-24.8338563866739,
12.));
#119818=CARTESIAN_POINT('Ctrl Pts',(65.6250035361612,-24.8455639071517,
12.));
#119819=CARTESIAN_POINT('Ctrl Pts',(65.6410973603713,-24.8573200135684,
12.));
#119820=CARTESIAN_POINT('Ctrl Pts',(65.6572214156761,-24.8691246628081,
12.));
#119821=CARTESIAN_POINT('Ctrl Pts',(65.6733755087723,-24.8809778178248,
12.));
#119822=CARTESIAN_POINT('Ctrl Pts',(65.6895594608798,-24.8928794448616,
12.));
#119823=CARTESIAN_POINT('Ctrl Pts',(65.7057730980471,-24.9048295111444,
12.));
#119824=CARTESIAN_POINT('Ctrl Pts',(65.7220162391016,-24.9168279820093,
12.));
#119825=CARTESIAN_POINT('Ctrl Pts',(65.7382886895839,-24.9288748194562,
12.));
#119826=CARTESIAN_POINT('Ctrl Pts',(65.7545902480286,-24.9409699836524,
12.));
#119827=CARTESIAN_POINT('Ctrl Pts',(65.7709207098949,-24.9531134338693,
12.));
#119828=CARTESIAN_POINT('Ctrl Pts',(65.7872798720847,-24.965305129559,12.));
#119829=CARTESIAN_POINT('Ctrl Pts',(65.8036675380761,-24.97754503157,12.));
#119830=CARTESIAN_POINT('Ctrl Pts',(65.8200835177071,-24.9898331021002,
12.));
#119831=CARTESIAN_POINT('Ctrl Pts',(65.8365276247157,-25.0021693041181,
12.));
#119832=CARTESIAN_POINT('Ctrl Pts',(65.8529996750441,-25.0145536009604,
12.));
#119833=CARTESIAN_POINT('Ctrl Pts',(65.8694994847587,-25.0269859558351,
12.));
#119834=CARTESIAN_POINT('Ctrl Pts',(65.8860268683088,-25.039466331404,12.));
#119835=CARTESIAN_POINT('Ctrl Pts',(65.9025816394391,-25.0519946900066,
12.));
#119836=CARTESIAN_POINT('Ctrl Pts',(65.9191636119796,-25.0645709938519,
12.));
#119837=CARTESIAN_POINT('Ctrl Pts',(65.9357726006174,-25.0771952052033,
12.));
#119838=CARTESIAN_POINT('Ctrl Pts',(65.9524084218167,-25.0898672865926,
12.));
#119839=CARTESIAN_POINT('Ctrl Pts',(65.9690708941591,-25.1025872009016,
12.));
#119840=CARTESIAN_POINT('Ctrl Pts',(65.9857598378455,-25.1153549112512,
12.));
#119841=CARTESIAN_POINT('Ctrl Pts',(66.0024750743902,-25.12817038093,12.));
#119842=CARTESIAN_POINT('Ctrl Pts',(66.0192164262607,-25.1410335733094,
12.));
#119843=CARTESIAN_POINT('Ctrl Pts',(66.0359837164709,-25.153944451741,12.));
#119844=CARTESIAN_POINT('Ctrl Pts',(66.0527767686,-25.1669029795652,12.));
#119845=CARTESIAN_POINT('Ctrl Pts',(66.0695954069698,-25.1799091201594,
12.));
#119846=CARTESIAN_POINT('Ctrl Pts',(66.086439456768,-25.1929628369685,12.));
#119847=CARTESIAN_POINT('Ctrl Pts',(66.1033087441916,-25.2060640935372,
12.));
#119848=CARTESIAN_POINT('Ctrl Pts',(66.1202030965784,-25.2192128535367,
12.));
#119849=CARTESIAN_POINT('Ctrl Pts',(66.1371223423371,-25.2324090807561,
12.));
#119850=CARTESIAN_POINT('Ctrl Pts',(66.1540663108767,-25.245652739088,12.));
#119851=CARTESIAN_POINT('Ctrl Pts',(66.1710348325378,-25.2589437925145,
12.));
#119852=CARTESIAN_POINT('Ctrl Pts',(66.1880277385114,-25.2722822050829,
12.));
#119853=CARTESIAN_POINT('Ctrl Pts',(66.2050448607883,-25.2856679408921,
12.));
#119854=CARTESIAN_POINT('Ctrl Pts',(66.2220860321931,-25.2991009641087,
12.));
#119855=CARTESIAN_POINT('Ctrl Pts',(66.2391510863992,-25.3125812389728,
12.));
#119856=CARTESIAN_POINT('Ctrl Pts',(66.2562398579479,-25.326108729803,12.));
#119857=CARTESIAN_POINT('Ctrl Pts',(66.2733521822675,-25.3396834009955,
12.));
#119858=CARTESIAN_POINT('Ctrl Pts',(66.2904878956721,-25.3533052170254,
12.));
#119859=CARTESIAN_POINT('Ctrl Pts',(66.3076468353417,-25.3669741424491,
12.));
#119860=CARTESIAN_POINT('Ctrl Pts',(66.3248288393046,-25.3806901419013,
12.));
#119861=CARTESIAN_POINT('Ctrl Pts',(66.3420337464176,-25.3944531800901,
12.));
#119862=CARTESIAN_POINT('Ctrl Pts',(66.3592613963407,-25.4082632217846,
12.));
#119863=CARTESIAN_POINT('Ctrl Pts',(66.3765116295363,-25.4221202318198,
12.));
#119864=CARTESIAN_POINT('Ctrl Pts',(66.3937842872684,-25.4360241751017,
12.));
#119865=CARTESIAN_POINT('Ctrl Pts',(66.4110792116,-25.4499750166079,12.));
#119866=CARTESIAN_POINT('Ctrl Pts',(66.4283962453899,-25.463972721385,12.));
#119867=CARTESIAN_POINT('Ctrl Pts',(66.445735232287,-25.4780172545418,12.));
#119868=CARTESIAN_POINT('Ctrl Pts',(66.463096016725,-25.4921085812548,12.));
#119869=CARTESIAN_POINT('Ctrl Pts',(66.4804784439146,-25.5062466667703,
12.));
#119870=CARTESIAN_POINT('Ctrl Pts',(66.4978823598352,-25.5204314764033,
12.));
#119871=CARTESIAN_POINT('Ctrl Pts',(66.5153076112237,-25.5346629755323,
12.));
#119872=CARTESIAN_POINT('Ctrl Pts',(66.5327540455638,-25.5489411295917,
12.));
#119873=CARTESIAN_POINT('Ctrl Pts',(66.5502215110843,-25.5632659040797,
12.));
#119874=CARTESIAN_POINT('Ctrl Pts',(66.567709856755,-25.5776372645605,12.));
#119875=CARTESIAN_POINT('Ctrl Pts',(66.585218932281,-25.5920551766629,12.));
#119876=CARTESIAN_POINT('Ctrl Pts',(66.6027485880947,-25.6065196060751,
12.));
#119877=CARTESIAN_POINT('Ctrl Pts',(66.6202986753482,-25.6210305185395,
12.));
#119878=CARTESIAN_POINT('Ctrl Pts',(66.6378690459105,-25.6355878798605,
12.));
#119879=CARTESIAN_POINT('Ctrl Pts',(66.6554595523611,-25.6501916559051,
12.));
#119880=CARTESIAN_POINT('Ctrl Pts',(66.6730700479843,-25.6648418126016,
12.));
#119881=CARTESIAN_POINT('Ctrl Pts',(66.6907003867599,-25.679538315933,12.));
#119882=CARTESIAN_POINT('Ctrl Pts',(66.7083504233566,-25.6942811319337,
12.));
#119883=CARTESIAN_POINT('Ctrl Pts',(66.72602001313,-25.7090702266976,12.));
#119884=CARTESIAN_POINT('Ctrl Pts',(66.7437090121168,-25.7239055663778,
12.));
#119885=CARTESIAN_POINT('Ctrl Pts',(66.7614172770302,-25.7387871171861,
12.));
#119886=CARTESIAN_POINT('Ctrl Pts',(66.7791446652505,-25.7537148453848,
12.));
#119887=CARTESIAN_POINT('Ctrl Pts',(66.7968910348199,-25.7686887172859,
12.));
#119888=CARTESIAN_POINT('Ctrl Pts',(66.8146562444397,-25.7837086992581,
12.));
#119889=CARTESIAN_POINT('Ctrl Pts',(66.8324401534657,-25.7987747577265,
12.));
#119890=CARTESIAN_POINT('Ctrl Pts',(66.8502426219015,-25.8138868591715,
12.));
#119891=CARTESIAN_POINT('Ctrl Pts',(66.8680635103907,-25.8290449701207,
12.));
#119892=CARTESIAN_POINT('Ctrl Pts',(66.8859026802123,-25.8442490571486,
12.));
#119893=CARTESIAN_POINT('Ctrl Pts',(66.9037599932787,-25.8594990868845,
12.));
#119894=CARTESIAN_POINT('Ctrl Pts',(66.9216353121308,-25.8747950260115,
12.));
#119895=CARTESIAN_POINT('Ctrl Pts',(66.9395284999327,-25.8901368412655,
12.));
#119896=CARTESIAN_POINT('Ctrl Pts',(66.9574394204635,-25.9055244994267,
12.));
#119897=CARTESIAN_POINT('Ctrl Pts',(66.9753679381122,-25.9209579673198,
12.));
#119898=CARTESIAN_POINT('Ctrl Pts',(66.993313917876,-25.9364372118216,12.));
#119899=CARTESIAN_POINT('Ctrl Pts',(67.0112772253553,-25.9519621998598,
12.));
#119900=CARTESIAN_POINT('Ctrl Pts',(67.0292577267495,-25.9675328984123,
12.));
#119901=CARTESIAN_POINT('Ctrl Pts',(67.0472552888495,-25.9831492744988,
12.));
#119902=CARTESIAN_POINT('Ctrl Pts',(67.0652697790335,-25.9988112951819,
12.));
#119903=CARTESIAN_POINT('Ctrl Pts',(67.083301065264,-26.0145189275733,12.));
#119904=CARTESIAN_POINT('Ctrl Pts',(67.101349016084,-26.030272138834,12.));
#119905=CARTESIAN_POINT('Ctrl Pts',(67.1194135006122,-26.0460708961725,
12.));
#119906=CARTESIAN_POINT('Ctrl Pts',(67.1374943885353,-26.0619151668361,
12.));
#119907=CARTESIAN_POINT('Ctrl Pts',(67.1555915501052,-26.077804918113,12.));
#119908=CARTESIAN_POINT('Ctrl Pts',(67.1737048561364,-26.0937401173385,
12.));
#119909=CARTESIAN_POINT('Ctrl Pts',(67.191834178002,-26.109720731895,12.));
#119910=CARTESIAN_POINT('Ctrl Pts',(67.2099793876295,-26.1257467292102,
12.));
#119911=CARTESIAN_POINT('Ctrl Pts',(67.228140357493,-26.1418180767487,12.));
#119912=CARTESIAN_POINT('Ctrl Pts',(67.2463169606105,-26.1579347420135,
12.));
#119913=CARTESIAN_POINT('Ctrl Pts',(67.2645090705414,-26.1740966925527,
12.));
#119914=CARTESIAN_POINT('Ctrl Pts',(67.2827165613828,-26.1903038959589,
12.));
#119915=CARTESIAN_POINT('Ctrl Pts',(67.3009393077654,-26.2065563198685,
12.));
#119916=CARTESIAN_POINT('Ctrl Pts',(67.3191771848468,-26.2228539319528,
12.));
#119917=CARTESIAN_POINT('Ctrl Pts',(67.3374300683076,-26.2391966999192,
12.));
#119918=CARTESIAN_POINT('Ctrl Pts',(67.3556978343506,-26.255584591518,12.));
#119919=CARTESIAN_POINT('Ctrl Pts',(67.3739803596967,-26.2720175745423,
12.));
#119920=CARTESIAN_POINT('Ctrl Pts',(67.392277521581,-26.2884956168271,12.));
#119921=CARTESIAN_POINT('Ctrl Pts',(67.4105891977465,-26.305018686241,12.));
#119922=CARTESIAN_POINT('Ctrl Pts',(67.4289152664406,-26.3215867506864,
12.));
#119923=CARTESIAN_POINT('Ctrl Pts',(67.4472556064127,-26.3381997781059,
12.));
#119924=CARTESIAN_POINT('Ctrl Pts',(67.4656100969121,-26.3548577364835,
12.));
#119925=CARTESIAN_POINT('Ctrl Pts',(67.4839786176833,-26.3715605938432,
12.));
#119926=CARTESIAN_POINT('Ctrl Pts',(67.5023610489611,-26.3883083182417,
12.));
#119927=CARTESIAN_POINT('Ctrl Pts',(67.5207572714666,-26.4051008777669,
12.));
#119928=CARTESIAN_POINT('Ctrl Pts',(67.5391671664055,-26.4219382405452,
12.));
#119929=CARTESIAN_POINT('Ctrl Pts',(67.5575906154648,-26.4388203747422,
12.));
#119930=CARTESIAN_POINT('Ctrl Pts',(67.5760275008096,-26.4557472485622,
12.));
#119931=CARTESIAN_POINT('Ctrl Pts',(67.5944777050782,-26.4727188302415,
12.));
#119932=CARTESIAN_POINT('Ctrl Pts',(67.6129411113774,-26.4897350880447,
12.));
#119933=CARTESIAN_POINT('Ctrl Pts',(67.6314176032823,-26.5067959902731,
12.));
#119934=CARTESIAN_POINT('Ctrl Pts',(67.6499070648323,-26.5239015052656,
12.));
#119935=CARTESIAN_POINT('Ctrl Pts',(67.6684093805288,-26.5410516013984,
12.));
#119936=CARTESIAN_POINT('Ctrl Pts',(67.6869244353292,-26.5582462470794,
12.));
#119937=CARTESIAN_POINT('Ctrl Pts',(67.7054521146427,-26.5754854107422,
12.));
#119938=CARTESIAN_POINT('Ctrl Pts',(67.7239923043295,-26.5927690608547,
12.));
#119939=CARTESIAN_POINT('Ctrl Pts',(67.7425448906983,-26.6100971659205,
12.));
#119940=CARTESIAN_POINT('Ctrl Pts',(67.7611097605042,-26.6274696944793,
12.));
#119941=CARTESIAN_POINT('Ctrl Pts',(67.7796868009447,-26.6448866151027,
12.));
#119942=CARTESIAN_POINT('Ctrl Pts',(67.7982758996557,-26.6623478963867,
12.));
#119943=CARTESIAN_POINT('Ctrl Pts',(67.8168769447086,-26.6798535069586,
12.));
#119944=CARTESIAN_POINT('Ctrl Pts',(67.8354898246079,-26.6974034154803,
12.));
#119945=CARTESIAN_POINT('Ctrl Pts',(67.8541144282875,-26.7149975906478,
12.));
#119946=CARTESIAN_POINT('Ctrl Pts',(67.8727506451067,-26.7326360011886,
12.));
#119947=CARTESIAN_POINT('Ctrl Pts',(67.8913983648441,-26.7503186158524,
12.));
#119948=CARTESIAN_POINT('Ctrl Pts',(67.9100574776974,-26.7680454034169,
12.));
#119949=CARTESIAN_POINT('Ctrl Pts',(67.9287278742839,-26.7858163326933,
12.));
#119950=CARTESIAN_POINT('Ctrl Pts',(67.9474094456395,-26.8036313725262,
12.));
#119951=CARTESIAN_POINT('Ctrl Pts',(67.9661020832165,-26.8214904917922,
12.));
#119952=CARTESIAN_POINT('Ctrl Pts',(67.9848056788814,-26.8393936593914,
12.));
#119953=CARTESIAN_POINT('Ctrl Pts',(68.0035201249108,-26.85734084425,12.));
#119954=CARTESIAN_POINT('Ctrl Pts',(68.0222453139862,-26.8753320153255,
12.));
#119955=CARTESIAN_POINT('Ctrl Pts',(68.0409811391871,-26.8933671416065,
12.));
#119956=CARTESIAN_POINT('Ctrl Pts',(68.0597274939857,-26.9114461921109,
12.));
#119957=CARTESIAN_POINT('Ctrl Pts',(68.0784842722362,-26.9295691358775,
12.));
#119958=CARTESIAN_POINT('Ctrl Pts',(68.0972513681739,-26.9477359419647,
12.));
#119959=CARTESIAN_POINT('Ctrl Pts',(68.1160286764244,-26.9659465794596,
12.));
#119960=CARTESIAN_POINT('Ctrl Pts',(68.13481609201,-26.9842010174819,12.));
#119961=CARTESIAN_POINT('Ctrl Pts',(68.1536135103558,-27.0024992251839,
12.));
#119962=CARTESIAN_POINT('Ctrl Pts',(68.1724208272967,-27.0208411717477,
12.));
#119963=CARTESIAN_POINT('Ctrl Pts',(68.1912379390786,-27.0392268263805,
12.));
#119964=CARTESIAN_POINT('Ctrl Pts',(68.2100647423345,-27.0576561583179,
12.));
#119965=CARTESIAN_POINT('Ctrl Pts',(68.2289011340624,-27.0761291368231,
12.));
#119966=CARTESIAN_POINT('Ctrl Pts',(68.2477470116014,-27.0946457311814,
12.));
#119967=CARTESIAN_POINT('Ctrl Pts',(68.2666022726094,-27.1132059106939,
12.));
#119968=CARTESIAN_POINT('Ctrl Pts',(68.285466815035,-27.1318096446643,12.));
#119969=CARTESIAN_POINT('Ctrl Pts',(68.3043405371589,-27.1504569024131,
12.));
#119970=CARTESIAN_POINT('Ctrl Pts',(68.3232233376415,-27.1691476532917,
12.));
#119971=CARTESIAN_POINT('Ctrl Pts',(68.3421151155708,-27.1878818666925,
12.));
#119972=CARTESIAN_POINT('Ctrl Pts',(68.3610157704999,-27.2066595120544,
12.));
#119973=CARTESIAN_POINT('Ctrl Pts',(68.379925202511,-27.2254805588677,12.));
#119974=CARTESIAN_POINT('Ctrl Pts',(68.3988433121589,-27.2443449766654,
12.));
#119975=CARTESIAN_POINT('Ctrl Pts',(68.4177700003471,-27.2632527350062,
12.));
#119976=CARTESIAN_POINT('Ctrl Pts',(68.4367051682166,-27.2822038034539,
12.));
#119977=CARTESIAN_POINT('Ctrl Pts',(68.455648717044,-27.3011981515571,12.));
#119978=CARTESIAN_POINT('Ctrl Pts',(68.4746005480992,-27.3202357488153,
12.));
#119979=CARTESIAN_POINT('Ctrl Pts',(68.4935605626361,-27.3393165646748,
12.));
#119980=CARTESIAN_POINT('Ctrl Pts',(68.5125286621888,-27.3584405685942,
12.));
#119981=CARTESIAN_POINT('Ctrl Pts',(68.5315047488035,-27.3776077300914,
12.));
#119982=CARTESIAN_POINT('Ctrl Pts',(68.5504887252975,-27.3968180187941,
12.));
#119983=CARTESIAN_POINT('Ctrl Pts',(68.5694804955014,-27.4160714044831,
12.));
#119984=CARTESIAN_POINT('Ctrl Pts',(68.5884799645218,-27.4353678571361,
12.));
#119985=CARTESIAN_POINT('Ctrl Pts',(68.6074870381619,-27.4547073468227,
12.));
#119986=CARTESIAN_POINT('Ctrl Pts',(68.6265016223561,-27.4740898435989,
12.));
#119987=CARTESIAN_POINT('Ctrl Pts',(68.645523622548,-27.4935153173868,12.));
#119988=CARTESIAN_POINT('Ctrl Pts',(68.6645529432045,-27.5129837378792,
12.));
#119989=CARTESIAN_POINT('Ctrl Pts',(68.6835894869882,-27.5324950743706,
12.));
#119990=CARTESIAN_POINT('Ctrl Pts',(68.7026331554296,-27.5520492958907,
12.));
#119991=CARTESIAN_POINT('Ctrl Pts',(68.7216838504218,-27.5716463715005,
12.));
#119992=CARTESIAN_POINT('Ctrl Pts',(68.7407414755259,-27.5912862705469,
12.));
#119993=CARTESIAN_POINT('Ctrl Pts',(68.7598059372129,-27.6109689629029,
12.));
#119994=CARTESIAN_POINT('Ctrl Pts',(68.7788771464713,-27.6306944192738,
12.));
#119995=CARTESIAN_POINT('Ctrl Pts',(68.7979550191872,-27.6504626112666,
12.));
#119996=CARTESIAN_POINT('Ctrl Pts',(68.8143140938914,-27.6674443909983,
12.));
#119997=CARTESIAN_POINT('Ctrl Pts',(68.8268597852178,-27.6804870323433,
12.));
#119998=CARTESIAN_POINT('Ctrl Pts',(68.8355891982104,-27.6895716271273,
12.));
#119999=CARTESIAN_POINT('Ctrl Pts',(68.8405004466157,-27.6946856803716,
12.));
#120000=CARTESIAN_POINT('Ctrl Pts',(68.8415926175082,-27.6958230985041,
12.));
#120001=CARTESIAN_POINT('',(65.4815644032299,-24.7419628022042,0.));
#120002=CARTESIAN_POINT('',(65.4815644032299,-24.7419628022042,0.));
#120003=CARTESIAN_POINT('Ctrl Pts',(68.8415926175082,-27.6958230985041,
0.));
#120004=CARTESIAN_POINT('Ctrl Pts',(68.8405004466157,-27.6946856803716,
0.));
#120005=CARTESIAN_POINT('Ctrl Pts',(68.8355891982104,-27.6895716271273,
0.));
#120006=CARTESIAN_POINT('Ctrl Pts',(68.8268597852178,-27.6804870323433,
0.));
#120007=CARTESIAN_POINT('Ctrl Pts',(68.8143140938914,-27.6674443909983,
0.));
#120008=CARTESIAN_POINT('Ctrl Pts',(68.7979550191872,-27.6504626112666,
0.));
#120009=CARTESIAN_POINT('Ctrl Pts',(68.7788771464713,-27.6306944192738,
0.));
#120010=CARTESIAN_POINT('Ctrl Pts',(68.7598059372129,-27.6109689629029,
0.));
#120011=CARTESIAN_POINT('Ctrl Pts',(68.7407414755259,-27.5912862705469,
0.));
#120012=CARTESIAN_POINT('Ctrl Pts',(68.7216838504218,-27.5716463715005,
0.));
#120013=CARTESIAN_POINT('Ctrl Pts',(68.7026331554296,-27.5520492958907,
0.));
#120014=CARTESIAN_POINT('Ctrl Pts',(68.6835894869882,-27.5324950743706,
0.));
#120015=CARTESIAN_POINT('Ctrl Pts',(68.6645529432045,-27.5129837378792,
0.));
#120016=CARTESIAN_POINT('Ctrl Pts',(68.645523622548,-27.4935153173868,0.));
#120017=CARTESIAN_POINT('Ctrl Pts',(68.6265016223561,-27.4740898435989,
0.));
#120018=CARTESIAN_POINT('Ctrl Pts',(68.6074870381619,-27.4547073468227,
0.));
#120019=CARTESIAN_POINT('Ctrl Pts',(68.5884799645218,-27.4353678571361,
0.));
#120020=CARTESIAN_POINT('Ctrl Pts',(68.5694804955014,-27.4160714044831,
0.));
#120021=CARTESIAN_POINT('Ctrl Pts',(68.5504887252975,-27.3968180187941,
0.));
#120022=CARTESIAN_POINT('Ctrl Pts',(68.5315047488035,-27.3776077300914,
0.));
#120023=CARTESIAN_POINT('Ctrl Pts',(68.5125286621888,-27.3584405685942,
0.));
#120024=CARTESIAN_POINT('Ctrl Pts',(68.4935605626361,-27.3393165646748,
0.));
#120025=CARTESIAN_POINT('Ctrl Pts',(68.4746005480992,-27.3202357488153,
0.));
#120026=CARTESIAN_POINT('Ctrl Pts',(68.455648717044,-27.3011981515571,0.));
#120027=CARTESIAN_POINT('Ctrl Pts',(68.4367051682166,-27.2822038034539,
0.));
#120028=CARTESIAN_POINT('Ctrl Pts',(68.4177700003471,-27.2632527350062,
0.));
#120029=CARTESIAN_POINT('Ctrl Pts',(68.3988433121589,-27.2443449766654,
0.));
#120030=CARTESIAN_POINT('Ctrl Pts',(68.379925202511,-27.2254805588677,0.));
#120031=CARTESIAN_POINT('Ctrl Pts',(68.3610157704999,-27.2066595120544,
0.));
#120032=CARTESIAN_POINT('Ctrl Pts',(68.3421151155708,-27.1878818666925,
0.));
#120033=CARTESIAN_POINT('Ctrl Pts',(68.3232233376415,-27.1691476532917,
0.));
#120034=CARTESIAN_POINT('Ctrl Pts',(68.3043405371589,-27.1504569024131,
0.));
#120035=CARTESIAN_POINT('Ctrl Pts',(68.285466815035,-27.1318096446643,0.));
#120036=CARTESIAN_POINT('Ctrl Pts',(68.2666022726094,-27.1132059106939,
0.));
#120037=CARTESIAN_POINT('Ctrl Pts',(68.2477470116014,-27.0946457311814,
0.));
#120038=CARTESIAN_POINT('Ctrl Pts',(68.2289011340624,-27.0761291368231,
0.));
#120039=CARTESIAN_POINT('Ctrl Pts',(68.2100647423345,-27.0576561583179,
0.));
#120040=CARTESIAN_POINT('Ctrl Pts',(68.1912379390786,-27.0392268263805,
0.));
#120041=CARTESIAN_POINT('Ctrl Pts',(68.1724208272967,-27.0208411717477,
0.));
#120042=CARTESIAN_POINT('Ctrl Pts',(68.1536135103558,-27.0024992251839,
0.));
#120043=CARTESIAN_POINT('Ctrl Pts',(68.13481609201,-26.9842010174819,0.));
#120044=CARTESIAN_POINT('Ctrl Pts',(68.1160286764244,-26.9659465794596,
0.));
#120045=CARTESIAN_POINT('Ctrl Pts',(68.0972513681739,-26.9477359419647,
0.));
#120046=CARTESIAN_POINT('Ctrl Pts',(68.0784842722362,-26.9295691358775,
0.));
#120047=CARTESIAN_POINT('Ctrl Pts',(68.0597274939857,-26.9114461921109,
0.));
#120048=CARTESIAN_POINT('Ctrl Pts',(68.0409811391871,-26.8933671416065,
0.));
#120049=CARTESIAN_POINT('Ctrl Pts',(68.0222453139862,-26.8753320153255,
0.));
#120050=CARTESIAN_POINT('Ctrl Pts',(68.0035201249108,-26.85734084425,0.));
#120051=CARTESIAN_POINT('Ctrl Pts',(67.9848056788814,-26.8393936593914,
0.));
#120052=CARTESIAN_POINT('Ctrl Pts',(67.9661020832165,-26.8214904917922,
0.));
#120053=CARTESIAN_POINT('Ctrl Pts',(67.9474094456395,-26.8036313725262,
0.));
#120054=CARTESIAN_POINT('Ctrl Pts',(67.9287278742839,-26.7858163326933,
0.));
#120055=CARTESIAN_POINT('Ctrl Pts',(67.9100574776974,-26.7680454034169,
0.));
#120056=CARTESIAN_POINT('Ctrl Pts',(67.8913983648441,-26.7503186158524,
0.));
#120057=CARTESIAN_POINT('Ctrl Pts',(67.8727506451067,-26.7326360011886,
0.));
#120058=CARTESIAN_POINT('Ctrl Pts',(67.8541144282875,-26.7149975906478,
0.));
#120059=CARTESIAN_POINT('Ctrl Pts',(67.8354898246079,-26.6974034154803,
0.));
#120060=CARTESIAN_POINT('Ctrl Pts',(67.8168769447086,-26.6798535069586,
0.));
#120061=CARTESIAN_POINT('Ctrl Pts',(67.7982758996557,-26.6623478963867,
0.));
#120062=CARTESIAN_POINT('Ctrl Pts',(67.7796868009447,-26.6448866151027,
0.));
#120063=CARTESIAN_POINT('Ctrl Pts',(67.7611097605042,-26.6274696944793,
0.));
#120064=CARTESIAN_POINT('Ctrl Pts',(67.7425448906983,-26.6100971659205,
0.));
#120065=CARTESIAN_POINT('Ctrl Pts',(67.7239923043295,-26.5927690608547,
0.));
#120066=CARTESIAN_POINT('Ctrl Pts',(67.7054521146427,-26.5754854107422,
0.));
#120067=CARTESIAN_POINT('Ctrl Pts',(67.6869244353292,-26.5582462470794,
0.));
#120068=CARTESIAN_POINT('Ctrl Pts',(67.6684093805288,-26.5410516013984,
0.));
#120069=CARTESIAN_POINT('Ctrl Pts',(67.6499070648323,-26.5239015052656,
0.));
#120070=CARTESIAN_POINT('Ctrl Pts',(67.6314176032823,-26.5067959902731,
0.));
#120071=CARTESIAN_POINT('Ctrl Pts',(67.6129411113774,-26.4897350880447,
0.));
#120072=CARTESIAN_POINT('Ctrl Pts',(67.5944777050782,-26.4727188302415,
0.));
#120073=CARTESIAN_POINT('Ctrl Pts',(67.5760275008096,-26.4557472485622,
0.));
#120074=CARTESIAN_POINT('Ctrl Pts',(67.5575906154648,-26.4388203747422,
0.));
#120075=CARTESIAN_POINT('Ctrl Pts',(67.5391671664055,-26.4219382405452,
0.));
#120076=CARTESIAN_POINT('Ctrl Pts',(67.5207572714666,-26.4051008777669,
0.));
#120077=CARTESIAN_POINT('Ctrl Pts',(67.5023610489611,-26.3883083182417,
0.));
#120078=CARTESIAN_POINT('Ctrl Pts',(67.4839786176833,-26.3715605938432,
0.));
#120079=CARTESIAN_POINT('Ctrl Pts',(67.4656100969121,-26.3548577364835,
0.));
#120080=CARTESIAN_POINT('Ctrl Pts',(67.4472556064127,-26.3381997781059,
0.));
#120081=CARTESIAN_POINT('Ctrl Pts',(67.4289152664406,-26.3215867506864,
0.));
#120082=CARTESIAN_POINT('Ctrl Pts',(67.4105891977465,-26.305018686241,0.));
#120083=CARTESIAN_POINT('Ctrl Pts',(67.392277521581,-26.2884956168271,0.));
#120084=CARTESIAN_POINT('Ctrl Pts',(67.3739803596967,-26.2720175745423,
0.));
#120085=CARTESIAN_POINT('Ctrl Pts',(67.3556978343506,-26.255584591518,0.));
#120086=CARTESIAN_POINT('Ctrl Pts',(67.3374300683076,-26.2391966999192,
0.));
#120087=CARTESIAN_POINT('Ctrl Pts',(67.3191771848468,-26.2228539319528,
0.));
#120088=CARTESIAN_POINT('Ctrl Pts',(67.3009393077654,-26.2065563198685,
0.));
#120089=CARTESIAN_POINT('Ctrl Pts',(67.2827165613828,-26.1903038959589,
0.));
#120090=CARTESIAN_POINT('Ctrl Pts',(67.2645090705414,-26.1740966925527,
0.));
#120091=CARTESIAN_POINT('Ctrl Pts',(67.2463169606105,-26.1579347420135,
0.));
#120092=CARTESIAN_POINT('Ctrl Pts',(67.228140357493,-26.1418180767487,0.));
#120093=CARTESIAN_POINT('Ctrl Pts',(67.2099793876295,-26.1257467292102,
0.));
#120094=CARTESIAN_POINT('Ctrl Pts',(67.191834178002,-26.109720731895,0.));
#120095=CARTESIAN_POINT('Ctrl Pts',(67.1737048561364,-26.0937401173385,
0.));
#120096=CARTESIAN_POINT('Ctrl Pts',(67.1555915501052,-26.077804918113,0.));
#120097=CARTESIAN_POINT('Ctrl Pts',(67.1374943885353,-26.0619151668361,
0.));
#120098=CARTESIAN_POINT('Ctrl Pts',(67.1194135006122,-26.0460708961725,
0.));
#120099=CARTESIAN_POINT('Ctrl Pts',(67.101349016084,-26.030272138834,0.));
#120100=CARTESIAN_POINT('Ctrl Pts',(67.083301065264,-26.0145189275733,0.));
#120101=CARTESIAN_POINT('Ctrl Pts',(67.0652697790335,-25.9988112951819,
0.));
#120102=CARTESIAN_POINT('Ctrl Pts',(67.0472552888495,-25.9831492744988,
0.));
#120103=CARTESIAN_POINT('Ctrl Pts',(67.0292577267495,-25.9675328984123,
0.));
#120104=CARTESIAN_POINT('Ctrl Pts',(67.0112772253553,-25.9519621998598,
0.));
#120105=CARTESIAN_POINT('Ctrl Pts',(66.993313917876,-25.9364372118216,0.));
#120106=CARTESIAN_POINT('Ctrl Pts',(66.9753679381122,-25.9209579673198,
0.));
#120107=CARTESIAN_POINT('Ctrl Pts',(66.9574394204635,-25.9055244994267,
0.));
#120108=CARTESIAN_POINT('Ctrl Pts',(66.9395284999327,-25.8901368412655,
0.));
#120109=CARTESIAN_POINT('Ctrl Pts',(66.9216353121308,-25.8747950260115,
0.));
#120110=CARTESIAN_POINT('Ctrl Pts',(66.9037599932787,-25.8594990868845,
0.));
#120111=CARTESIAN_POINT('Ctrl Pts',(66.8859026802123,-25.8442490571486,
0.));
#120112=CARTESIAN_POINT('Ctrl Pts',(66.8680635103907,-25.8290449701207,
0.));
#120113=CARTESIAN_POINT('Ctrl Pts',(66.8502426219015,-25.8138868591715,
0.));
#120114=CARTESIAN_POINT('Ctrl Pts',(66.8324401534657,-25.7987747577265,
0.));
#120115=CARTESIAN_POINT('Ctrl Pts',(66.8146562444397,-25.7837086992581,
0.));
#120116=CARTESIAN_POINT('Ctrl Pts',(66.7968910348199,-25.7686887172859,
0.));
#120117=CARTESIAN_POINT('Ctrl Pts',(66.7791446652505,-25.7537148453848,
0.));
#120118=CARTESIAN_POINT('Ctrl Pts',(66.7614172770302,-25.7387871171861,
0.));
#120119=CARTESIAN_POINT('Ctrl Pts',(66.7437090121168,-25.7239055663778,
0.));
#120120=CARTESIAN_POINT('Ctrl Pts',(66.72602001313,-25.7090702266976,0.));
#120121=CARTESIAN_POINT('Ctrl Pts',(66.7083504233566,-25.6942811319337,
0.));
#120122=CARTESIAN_POINT('Ctrl Pts',(66.6907003867599,-25.679538315933,0.));
#120123=CARTESIAN_POINT('Ctrl Pts',(66.6730700479843,-25.6648418126016,
0.));
#120124=CARTESIAN_POINT('Ctrl Pts',(66.6554595523611,-25.6501916559051,
0.));
#120125=CARTESIAN_POINT('Ctrl Pts',(66.6378690459105,-25.6355878798605,
0.));
#120126=CARTESIAN_POINT('Ctrl Pts',(66.6202986753482,-25.6210305185395,
0.));
#120127=CARTESIAN_POINT('Ctrl Pts',(66.6027485880947,-25.6065196060751,
0.));
#120128=CARTESIAN_POINT('Ctrl Pts',(66.585218932281,-25.5920551766629,0.));
#120129=CARTESIAN_POINT('Ctrl Pts',(66.567709856755,-25.5776372645605,0.));
#120130=CARTESIAN_POINT('Ctrl Pts',(66.5502215110843,-25.5632659040797,
0.));
#120131=CARTESIAN_POINT('Ctrl Pts',(66.5327540455638,-25.5489411295917,
0.));
#120132=CARTESIAN_POINT('Ctrl Pts',(66.5153076112237,-25.5346629755323,
0.));
#120133=CARTESIAN_POINT('Ctrl Pts',(66.4978823598352,-25.5204314764033,
0.));
#120134=CARTESIAN_POINT('Ctrl Pts',(66.4804784439146,-25.5062466667703,
0.));
#120135=CARTESIAN_POINT('Ctrl Pts',(66.463096016725,-25.4921085812548,0.));
#120136=CARTESIAN_POINT('Ctrl Pts',(66.445735232287,-25.4780172545418,0.));
#120137=CARTESIAN_POINT('Ctrl Pts',(66.4283962453899,-25.463972721385,0.));
#120138=CARTESIAN_POINT('Ctrl Pts',(66.4110792116,-25.4499750166079,0.));
#120139=CARTESIAN_POINT('Ctrl Pts',(66.3937842872684,-25.4360241751017,
0.));
#120140=CARTESIAN_POINT('Ctrl Pts',(66.3765116295363,-25.4221202318198,
0.));
#120141=CARTESIAN_POINT('Ctrl Pts',(66.3592613963407,-25.4082632217846,
0.));
#120142=CARTESIAN_POINT('Ctrl Pts',(66.3420337464176,-25.3944531800901,
0.));
#120143=CARTESIAN_POINT('Ctrl Pts',(66.3248288393046,-25.3806901419013,
0.));
#120144=CARTESIAN_POINT('Ctrl Pts',(66.3076468353417,-25.3669741424491,
0.));
#120145=CARTESIAN_POINT('Ctrl Pts',(66.2904878956721,-25.3533052170254,
0.));
#120146=CARTESIAN_POINT('Ctrl Pts',(66.2733521822675,-25.3396834009955,
0.));
#120147=CARTESIAN_POINT('Ctrl Pts',(66.2562398579479,-25.326108729803,0.));
#120148=CARTESIAN_POINT('Ctrl Pts',(66.2391510863992,-25.3125812389728,
0.));
#120149=CARTESIAN_POINT('Ctrl Pts',(66.2220860321931,-25.2991009641087,
0.));
#120150=CARTESIAN_POINT('Ctrl Pts',(66.2050448607883,-25.2856679408921,
0.));
#120151=CARTESIAN_POINT('Ctrl Pts',(66.1880277385114,-25.2722822050829,
0.));
#120152=CARTESIAN_POINT('Ctrl Pts',(66.1710348325378,-25.2589437925145,
0.));
#120153=CARTESIAN_POINT('Ctrl Pts',(66.1540663108767,-25.245652739088,0.));
#120154=CARTESIAN_POINT('Ctrl Pts',(66.1371223423371,-25.2324090807561,
0.));
#120155=CARTESIAN_POINT('Ctrl Pts',(66.1202030965784,-25.2192128535367,
0.));
#120156=CARTESIAN_POINT('Ctrl Pts',(66.1033087441916,-25.2060640935372,
0.));
#120157=CARTESIAN_POINT('Ctrl Pts',(66.086439456768,-25.1929628369685,0.));
#120158=CARTESIAN_POINT('Ctrl Pts',(66.0695954069698,-25.1799091201594,
0.));
#120159=CARTESIAN_POINT('Ctrl Pts',(66.0527767686,-25.1669029795652,0.));
#120160=CARTESIAN_POINT('Ctrl Pts',(66.0359837164709,-25.153944451741,0.));
#120161=CARTESIAN_POINT('Ctrl Pts',(66.0192164262607,-25.1410335733094,
0.));
#120162=CARTESIAN_POINT('Ctrl Pts',(66.0024750743902,-25.12817038093,0.));
#120163=CARTESIAN_POINT('Ctrl Pts',(65.9857598378455,-25.1153549112512,
0.));
#120164=CARTESIAN_POINT('Ctrl Pts',(65.9690708941591,-25.1025872009016,
0.));
#120165=CARTESIAN_POINT('Ctrl Pts',(65.9524084218167,-25.0898672865926,
0.));
#120166=CARTESIAN_POINT('Ctrl Pts',(65.9357726006174,-25.0771952052033,
0.));
#120167=CARTESIAN_POINT('Ctrl Pts',(65.9191636119796,-25.0645709938519,
0.));
#120168=CARTESIAN_POINT('Ctrl Pts',(65.9025816394391,-25.0519946900066,
0.));
#120169=CARTESIAN_POINT('Ctrl Pts',(65.8860268683088,-25.039466331404,0.));
#120170=CARTESIAN_POINT('Ctrl Pts',(65.8694994847587,-25.0269859558351,
0.));
#120171=CARTESIAN_POINT('Ctrl Pts',(65.8529996750441,-25.0145536009604,
0.));
#120172=CARTESIAN_POINT('Ctrl Pts',(65.8365276247157,-25.0021693041181,
0.));
#120173=CARTESIAN_POINT('Ctrl Pts',(65.8200835177071,-24.9898331021002,
0.));
#120174=CARTESIAN_POINT('Ctrl Pts',(65.8036675380761,-24.97754503157,0.));
#120175=CARTESIAN_POINT('Ctrl Pts',(65.7872798720847,-24.965305129559,0.));
#120176=CARTESIAN_POINT('Ctrl Pts',(65.7709207098949,-24.9531134338693,
0.));
#120177=CARTESIAN_POINT('Ctrl Pts',(65.7545902480286,-24.9409699836524,
0.));
#120178=CARTESIAN_POINT('Ctrl Pts',(65.7382886895839,-24.9288748194562,
0.));
#120179=CARTESIAN_POINT('Ctrl Pts',(65.7220162391016,-24.9168279820093,
0.));
#120180=CARTESIAN_POINT('Ctrl Pts',(65.7057730980471,-24.9048295111444,
0.));
#120181=CARTESIAN_POINT('Ctrl Pts',(65.6895594608798,-24.8928794448616,
0.));
#120182=CARTESIAN_POINT('Ctrl Pts',(65.6733755087723,-24.8809778178248,
0.));
#120183=CARTESIAN_POINT('Ctrl Pts',(65.6572214156761,-24.8691246628081,
0.));
#120184=CARTESIAN_POINT('Ctrl Pts',(65.6410973603713,-24.8573200135684,
0.));
#120185=CARTESIAN_POINT('Ctrl Pts',(65.6250035361612,-24.8455639071517,
0.));
#120186=CARTESIAN_POINT('Ctrl Pts',(65.6089401625551,-24.8338563866739,
0.));
#120187=CARTESIAN_POINT('Ctrl Pts',(65.5929074932487,-24.8221975032059,
0.));
#120188=CARTESIAN_POINT('Ctrl Pts',(65.5769057914184,-24.8105873098578,
0.));
#120189=CARTESIAN_POINT('Ctrl Pts',(65.5609353062749,-24.7990258561234,
0.));
#120190=CARTESIAN_POINT('Ctrl Pts',(65.5449962514735,-24.7875131827515,
0.));
#120191=CARTESIAN_POINT('Ctrl Pts',(65.5290887770493,-24.7760493148551,
0.));
#120192=CARTESIAN_POINT('Ctrl Pts',(65.5132129675727,-24.764634262097,0.));
#120193=CARTESIAN_POINT('Ctrl Pts',(65.5005376841469,-24.7555412724771,
0.));
#120194=CARTESIAN_POINT('Ctrl Pts',(65.4910454936487,-24.7487434956058,
0.));
#120195=CARTESIAN_POINT('Ctrl Pts',(65.484723709553,-24.7442214063411,0.));
#120196=CARTESIAN_POINT('Ctrl Pts',(65.4815644032299,-24.7419628022042,
0.));
#120197=CARTESIAN_POINT('Ctrl Pts',(66.3684712863594,-33.8448817269567,
0.));
#120198=CARTESIAN_POINT('Ctrl Pts',(66.3684712863594,-33.8448817269567,
12.));
#120199=CARTESIAN_POINT('Ctrl Pts',(66.3650082659712,-33.840486261887,0.));
#120200=CARTESIAN_POINT('Ctrl Pts',(66.3650082659712,-33.840486261887,12.));
#120201=CARTESIAN_POINT('Ctrl Pts',(66.3580824155893,-33.8316996011932,
0.));
#120202=CARTESIAN_POINT('Ctrl Pts',(66.3580824155893,-33.8316996011932,
12.));
#120203=CARTESIAN_POINT('Ctrl Pts',(66.3476942112,-33.8185324184903,0.));
#120204=CARTESIAN_POINT('Ctrl Pts',(66.3476942112,-33.8185324184903,12.));
#120205=CARTESIAN_POINT('Ctrl Pts',(66.3338444144211,-33.8010017926027,
0.));
#120206=CARTESIAN_POINT('Ctrl Pts',(66.3338444144211,-33.8010017926027,
12.));
#120207=CARTESIAN_POINT('Ctrl Pts',(66.3165340771611,-33.7791312145108,
0.));
#120208=CARTESIAN_POINT('Ctrl Pts',(66.3165340771611,-33.7791312145108,
12.));
#120209=CARTESIAN_POINT('Ctrl Pts',(66.2992256621336,-33.7573033544559,
0.));
#120210=CARTESIAN_POINT('Ctrl Pts',(66.2992256621336,-33.7573033544559,
12.));
#120211=CARTESIAN_POINT('Ctrl Pts',(66.2819191962353,-33.7355182321907,
0.));
#120212=CARTESIAN_POINT('Ctrl Pts',(66.2819191962353,-33.7355182321907,
12.));
#120213=CARTESIAN_POINT('Ctrl Pts',(66.2646147235321,-33.7137758735903,
0.));
#120214=CARTESIAN_POINT('Ctrl Pts',(66.2646147235321,-33.7137758735903,
12.));
#120215=CARTESIAN_POINT('Ctrl Pts',(66.2473123109395,-33.6920763111448,
0.));
#120216=CARTESIAN_POINT('Ctrl Pts',(66.2473123109395,-33.6920763111448,
12.));
#120217=CARTESIAN_POINT('Ctrl Pts',(66.2300120464082,-33.6704195830392,
0.));
#120218=CARTESIAN_POINT('Ctrl Pts',(66.2300120464082,-33.6704195830392,
12.));
#120219=CARTESIAN_POINT('Ctrl Pts',(66.2127140313598,-33.6488057311532,
0.));
#120220=CARTESIAN_POINT('Ctrl Pts',(66.2127140313598,-33.6488057311532,
12.));
#120221=CARTESIAN_POINT('Ctrl Pts',(66.1954183747088,-33.6272347993476,
0.));
#120222=CARTESIAN_POINT('Ctrl Pts',(66.1954183747088,-33.6272347993476,
12.));
#120223=CARTESIAN_POINT('Ctrl Pts',(66.1781251864017,-33.6057068316769,
0.));
#120224=CARTESIAN_POINT('Ctrl Pts',(66.1781251864017,-33.6057068316769,
12.));
#120225=CARTESIAN_POINT('Ctrl Pts',(66.1608345707636,-33.5842218705151,
0.));
#120226=CARTESIAN_POINT('Ctrl Pts',(66.1608345707636,-33.5842218705151,
12.));
#120227=CARTESIAN_POINT('Ctrl Pts',(66.1435466211076,-33.5627799550483,
0.));
#120228=CARTESIAN_POINT('Ctrl Pts',(66.1435466211076,-33.5627799550483,
12.));
#120229=CARTESIAN_POINT('Ctrl Pts',(66.1262614234674,-33.5413811223451,
0.));
#120230=CARTESIAN_POINT('Ctrl Pts',(66.1262614234674,-33.5413811223451,
12.));
#120231=CARTESIAN_POINT('Ctrl Pts',(66.1089790592729,-33.5200254081243,
0.));
#120232=CARTESIAN_POINT('Ctrl Pts',(66.1089790592729,-33.5200254081243,
12.));
#120233=CARTESIAN_POINT('Ctrl Pts',(66.0916996085244,-33.4987128476622,
0.));
#120234=CARTESIAN_POINT('Ctrl Pts',(66.0916996085244,-33.4987128476622,
12.));
#120235=CARTESIAN_POINT('Ctrl Pts',(66.0744231525415,-33.4774434765746,
0.));
#120236=CARTESIAN_POINT('Ctrl Pts',(66.0744231525415,-33.4774434765746,
12.));
#120237=CARTESIAN_POINT('Ctrl Pts',(66.0571497774434,-33.4562173318025,
0.));
#120238=CARTESIAN_POINT('Ctrl Pts',(66.0571497774434,-33.4562173318025,
12.));
#120239=CARTESIAN_POINT('Ctrl Pts',(66.0398795737777,-33.4350344515101,
0.));
#120240=CARTESIAN_POINT('Ctrl Pts',(66.0398795737777,-33.4350344515101,
12.));
#120241=CARTESIAN_POINT('Ctrl Pts',(66.0226126349446,-33.4138948746388,
0.));
#120242=CARTESIAN_POINT('Ctrl Pts',(66.0226126349446,-33.4138948746388,
12.));
#120243=CARTESIAN_POINT('Ctrl Pts',(66.0053490559812,-33.3927986405605,
0.));
#120244=CARTESIAN_POINT('Ctrl Pts',(66.0053490559812,-33.3927986405605,
12.));
#120245=CARTESIAN_POINT('Ctrl Pts',(65.9880889322831,-33.37174578871,0.));
#120246=CARTESIAN_POINT('Ctrl Pts',(65.9880889322831,-33.37174578871,12.));
#120247=CARTESIAN_POINT('Ctrl Pts',(65.970832358141,-33.3507363581593,0.));
#120248=CARTESIAN_POINT('Ctrl Pts',(65.970832358141,-33.3507363581593,12.));
#120249=CARTESIAN_POINT('Ctrl Pts',(65.9535794260831,-33.3297703874266,
0.));
#120250=CARTESIAN_POINT('Ctrl Pts',(65.9535794260831,-33.3297703874266,
12.));
#120251=CARTESIAN_POINT('Ctrl Pts',(65.9363302276846,-33.3088479147164,
0.));
#120252=CARTESIAN_POINT('Ctrl Pts',(65.9363302276846,-33.3088479147164,
12.));
#120253=CARTESIAN_POINT('Ctrl Pts',(65.9190848540433,-33.2879689780573,
0.));
#120254=CARTESIAN_POINT('Ctrl Pts',(65.9190848540433,-33.2879689780573,
12.));
#120255=CARTESIAN_POINT('Ctrl Pts',(65.9018433963889,-33.2671336154754,
0.));
#120256=CARTESIAN_POINT('Ctrl Pts',(65.9018433963889,-33.2671336154754,
12.));
#120257=CARTESIAN_POINT('Ctrl Pts',(65.8846059466371,-33.2463418651493,
0.));
#120258=CARTESIAN_POINT('Ctrl Pts',(65.8846059466371,-33.2463418651493,
12.));
#120259=CARTESIAN_POINT('Ctrl Pts',(65.8673725979577,-33.2255937655649,
0.));
#120260=CARTESIAN_POINT('Ctrl Pts',(65.8673725979577,-33.2255937655649,
12.));
#120261=CARTESIAN_POINT('Ctrl Pts',(65.8501434445164,-33.2048893554491,
0.));
#120262=CARTESIAN_POINT('Ctrl Pts',(65.8501434445164,-33.2048893554491,
12.));
#120263=CARTESIAN_POINT('Ctrl Pts',(65.8329185812375,-33.1842286737051,
0.));
#120264=CARTESIAN_POINT('Ctrl Pts',(65.8329185812375,-33.1842286737051,
12.));
#120265=CARTESIAN_POINT('Ctrl Pts',(65.8156981035503,-33.16361175934,0.));
#120266=CARTESIAN_POINT('Ctrl Pts',(65.8156981035503,-33.16361175934,12.));
#120267=CARTESIAN_POINT('Ctrl Pts',(65.7984821071623,-33.1430386513976,
0.));
#120268=CARTESIAN_POINT('Ctrl Pts',(65.7984821071623,-33.1430386513976,
12.));
#120269=CARTESIAN_POINT('Ctrl Pts',(65.7812706877696,-33.1225093888672,
0.));
#120270=CARTESIAN_POINT('Ctrl Pts',(65.7812706877696,-33.1225093888672,
12.));
#120271=CARTESIAN_POINT('Ctrl Pts',(65.7640639410661,-33.1020240106885,
0.));
#120272=CARTESIAN_POINT('Ctrl Pts',(65.7640639410661,-33.1020240106885,
12.));
#120273=CARTESIAN_POINT('Ctrl Pts',(65.7468619628815,-33.081582555798,0.));
#120274=CARTESIAN_POINT('Ctrl Pts',(65.7468619628815,-33.081582555798,12.));
#120275=CARTESIAN_POINT('Ctrl Pts',(65.7296648492824,-33.0611850631582,
0.));
#120276=CARTESIAN_POINT('Ctrl Pts',(65.7296648492824,-33.0611850631582,
12.));
#120277=CARTESIAN_POINT('Ctrl Pts',(65.7124726966802,-33.0408315717873,
0.));
#120278=CARTESIAN_POINT('Ctrl Pts',(65.7124726966802,-33.0408315717873,
12.));
#120279=CARTESIAN_POINT('Ctrl Pts',(65.6952856019533,-33.0205221207873,
0.));
#120280=CARTESIAN_POINT('Ctrl Pts',(65.6952856019533,-33.0205221207873,
12.));
#120281=CARTESIAN_POINT('Ctrl Pts',(65.6781036625027,-33.0002567493574,
0.));
#120282=CARTESIAN_POINT('Ctrl Pts',(65.6781036625027,-33.0002567493574,
12.));
#120283=CARTESIAN_POINT('Ctrl Pts',(65.6609269761888,-32.980035496784,0.));
#120284=CARTESIAN_POINT('Ctrl Pts',(65.6609269761888,-32.980035496784,12.));
#120285=CARTESIAN_POINT('Ctrl Pts',(65.6437556412946,-32.9598584024313,
0.));
#120286=CARTESIAN_POINT('Ctrl Pts',(65.6437556412946,-32.9598584024313,
12.));
#120287=CARTESIAN_POINT('Ctrl Pts',(65.6265897564783,-32.9397255057274,
0.));
#120288=CARTESIAN_POINT('Ctrl Pts',(65.6265897564783,-32.9397255057274,
12.));
#120289=CARTESIAN_POINT('Ctrl Pts',(65.6094294207276,-32.9196368461463,
0.));
#120290=CARTESIAN_POINT('Ctrl Pts',(65.6094294207276,-32.9196368461463,
12.));
#120291=CARTESIAN_POINT('Ctrl Pts',(65.5922747333194,-32.8995924631898,
0.));
#120292=CARTESIAN_POINT('Ctrl Pts',(65.5922747333194,-32.8995924631898,
12.));
#120293=CARTESIAN_POINT('Ctrl Pts',(65.5751257938472,-32.879592396403,0.));
#120294=CARTESIAN_POINT('Ctrl Pts',(65.5751257938472,-32.879592396403,12.));
#120295=CARTESIAN_POINT('Ctrl Pts',(65.5579827022421,-32.8596366853832,
0.));
#120296=CARTESIAN_POINT('Ctrl Pts',(65.5579827022421,-32.8596366853832,
12.));
#120297=CARTESIAN_POINT('Ctrl Pts',(65.5408455587964,-32.8397253697866,
0.));
#120298=CARTESIAN_POINT('Ctrl Pts',(65.5408455587964,-32.8397253697866,
12.));
#120299=CARTESIAN_POINT('Ctrl Pts',(65.5237144641857,-32.8198584893316,
0.));
#120300=CARTESIAN_POINT('Ctrl Pts',(65.5237144641857,-32.8198584893316,
12.));
#120301=CARTESIAN_POINT('Ctrl Pts',(65.5065895194928,-32.8000360837975,
0.));
#120302=CARTESIAN_POINT('Ctrl Pts',(65.5065895194928,-32.8000360837975,
12.));
#120303=CARTESIAN_POINT('Ctrl Pts',(65.489470826206,-32.7802581930287,0.));
#120304=CARTESIAN_POINT('Ctrl Pts',(65.489470826206,-32.7802581930287,12.));
#120305=CARTESIAN_POINT('Ctrl Pts',(65.4723584862122,-32.7605248569378,
0.));
#120306=CARTESIAN_POINT('Ctrl Pts',(65.4723584862122,-32.7605248569378,
12.));
#120307=CARTESIAN_POINT('Ctrl Pts',(65.4552526017905,-32.7408361155037,
0.));
#120308=CARTESIAN_POINT('Ctrl Pts',(65.4552526017905,-32.7408361155037,
12.));
#120309=CARTESIAN_POINT('Ctrl Pts',(65.4381532756065,-32.7211920087684,
0.));
#120310=CARTESIAN_POINT('Ctrl Pts',(65.4381532756065,-32.7211920087684,
12.));
#120311=CARTESIAN_POINT('Ctrl Pts',(65.4210606107035,-32.7015925768265,
0.));
#120312=CARTESIAN_POINT('Ctrl Pts',(65.4210606107035,-32.7015925768265,
12.));
#120313=CARTESIAN_POINT('Ctrl Pts',(65.4039747105038,-32.6820378598267,
0.));
#120314=CARTESIAN_POINT('Ctrl Pts',(65.4039747105038,-32.6820378598267,
12.));
#120315=CARTESIAN_POINT('Ctrl Pts',(65.3868956788182,-32.6625278979811,
0.));
#120316=CARTESIAN_POINT('Ctrl Pts',(65.3868956788182,-32.6625278979811,
12.));
#120317=CARTESIAN_POINT('Ctrl Pts',(65.3698236198512,-32.6430627315674,
0.));
#120318=CARTESIAN_POINT('Ctrl Pts',(65.3698236198512,-32.6430627315674,
12.));
#120319=CARTESIAN_POINT('Ctrl Pts',(65.3527586382081,-32.6236424009301,
0.));
#120320=CARTESIAN_POINT('Ctrl Pts',(65.3527586382081,-32.6236424009301,
12.));
#120321=CARTESIAN_POINT('Ctrl Pts',(65.3357008389003,-32.6042669464751,
0.));
#120322=CARTESIAN_POINT('Ctrl Pts',(65.3357008389003,-32.6042669464751,
12.));
#120323=CARTESIAN_POINT('Ctrl Pts',(65.31865032735,-32.5849364086679,0.));
#120324=CARTESIAN_POINT('Ctrl Pts',(65.31865032735,-32.5849364086679,12.));
#120325=CARTESIAN_POINT('Ctrl Pts',(65.3016072093912,-32.5656508280422,
0.));
#120326=CARTESIAN_POINT('Ctrl Pts',(65.3016072093912,-32.5656508280422,
12.));
#120327=CARTESIAN_POINT('Ctrl Pts',(65.2845715912721,-32.5464102452015,
0.));
#120328=CARTESIAN_POINT('Ctrl Pts',(65.2845715912721,-32.5464102452015,
12.));
#120329=CARTESIAN_POINT('Ctrl Pts',(65.2675435796558,-32.5272147008191,
0.));
#120330=CARTESIAN_POINT('Ctrl Pts',(65.2675435796558,-32.5272147008191,
12.));
#120331=CARTESIAN_POINT('Ctrl Pts',(65.2505232816209,-32.5080642356328,
0.));
#120332=CARTESIAN_POINT('Ctrl Pts',(65.2505232816209,-32.5080642356328,
12.));
#120333=CARTESIAN_POINT('Ctrl Pts',(65.2335108046614,-32.4889588904392,
0.));
#120334=CARTESIAN_POINT('Ctrl Pts',(65.2335108046614,-32.4889588904392,
12.));
#120335=CARTESIAN_POINT('Ctrl Pts',(65.2165062566924,-32.4698987061032,
0.));
#120336=CARTESIAN_POINT('Ctrl Pts',(65.2165062566924,-32.4698987061032,
12.));
#120337=CARTESIAN_POINT('Ctrl Pts',(65.1995097460538,-32.450883723561,0.));
#120338=CARTESIAN_POINT('Ctrl Pts',(65.1995097460538,-32.450883723561,12.));
#120339=CARTESIAN_POINT('Ctrl Pts',(65.182521381514,-32.4319139838213,0.));
#120340=CARTESIAN_POINT('Ctrl Pts',(65.182521381514,-32.4319139838213,12.));
#120341=CARTESIAN_POINT('Ctrl Pts',(65.1655412722725,-32.4129895279615,
0.));
#120342=CARTESIAN_POINT('Ctrl Pts',(65.1655412722725,-32.4129895279615,
12.));
#120343=CARTESIAN_POINT('Ctrl Pts',(65.1485695279635,-32.3941103971221,
0.));
#120344=CARTESIAN_POINT('Ctrl Pts',(65.1485695279635,-32.3941103971221,
12.));
#120345=CARTESIAN_POINT('Ctrl Pts',(65.1316062586588,-32.3752766325136,
0.));
#120346=CARTESIAN_POINT('Ctrl Pts',(65.1316062586588,-32.3752766325136,
12.));
#120347=CARTESIAN_POINT('Ctrl Pts',(65.1146515748722,-32.3564882754212,
0.));
#120348=CARTESIAN_POINT('Ctrl Pts',(65.1146515748722,-32.3564882754212,
12.));
#120349=CARTESIAN_POINT('Ctrl Pts',(65.0977055875607,-32.3377453672051,
0.));
#120350=CARTESIAN_POINT('Ctrl Pts',(65.0977055875607,-32.3377453672051,
12.));
#120351=CARTESIAN_POINT('Ctrl Pts',(65.0807684081281,-32.3190479492987,
0.));
#120352=CARTESIAN_POINT('Ctrl Pts',(65.0807684081281,-32.3190479492987,
12.));
#120353=CARTESIAN_POINT('Ctrl Pts',(65.0638401484257,-32.3003960632007,
0.));
#120354=CARTESIAN_POINT('Ctrl Pts',(65.0638401484257,-32.3003960632007,
12.));
#120355=CARTESIAN_POINT('Ctrl Pts',(65.0469209207563,-32.2817897504807,
0.));
#120356=CARTESIAN_POINT('Ctrl Pts',(65.0469209207563,-32.2817897504807,
12.));
#120357=CARTESIAN_POINT('Ctrl Pts',(65.03001083788,-32.2632290527862,0.));
#120358=CARTESIAN_POINT('Ctrl Pts',(65.03001083788,-32.2632290527862,12.));
#120359=CARTESIAN_POINT('Ctrl Pts',(65.0131100130157,-32.2447140118422,
0.));
#120360=CARTESIAN_POINT('Ctrl Pts',(65.0131100130157,-32.2447140118422,
12.));
#120361=CARTESIAN_POINT('Ctrl Pts',(64.9962185598461,-32.2262446694513,
0.));
#120362=CARTESIAN_POINT('Ctrl Pts',(64.9962185598461,-32.2262446694513,
12.));
#120363=CARTESIAN_POINT('Ctrl Pts',(64.9793365925178,-32.207821067485,0.));
#120364=CARTESIAN_POINT('Ctrl Pts',(64.9793365925178,-32.207821067485,12.));
#120365=CARTESIAN_POINT('Ctrl Pts',(64.9624642256461,-32.1894432478881,
0.));
#120366=CARTESIAN_POINT('Ctrl Pts',(64.9624642256461,-32.1894432478881,
12.));
#120367=CARTESIAN_POINT('Ctrl Pts',(64.9456015743192,-32.1711112526855,
0.));
#120368=CARTESIAN_POINT('Ctrl Pts',(64.9456015743192,-32.1711112526855,
12.));
#120369=CARTESIAN_POINT('Ctrl Pts',(64.9287487541015,-32.1528251239831,
0.));
#120370=CARTESIAN_POINT('Ctrl Pts',(64.9287487541015,-32.1528251239831,
12.));
#120371=CARTESIAN_POINT('Ctrl Pts',(64.9119058810366,-32.1345849039674,
0.));
#120372=CARTESIAN_POINT('Ctrl Pts',(64.9119058810366,-32.1345849039674,
12.));
#120373=CARTESIAN_POINT('Ctrl Pts',(64.8950730716501,-32.1163906348984,
0.));
#120374=CARTESIAN_POINT('Ctrl Pts',(64.8950730716501,-32.1163906348984,
12.));
#120375=CARTESIAN_POINT('Ctrl Pts',(64.8782504429527,-32.0982423591113,
0.));
#120376=CARTESIAN_POINT('Ctrl Pts',(64.8782504429527,-32.0982423591113,
12.));
#120377=CARTESIAN_POINT('Ctrl Pts',(64.8614381124454,-32.0801401190244,
0.));
#120378=CARTESIAN_POINT('Ctrl Pts',(64.8614381124454,-32.0801401190244,
12.));
#120379=CARTESIAN_POINT('Ctrl Pts',(64.8446361981234,-32.0620839571409,
0.));
#120380=CARTESIAN_POINT('Ctrl Pts',(64.8446361981234,-32.0620839571409,
12.));
#120381=CARTESIAN_POINT('Ctrl Pts',(64.8278448184785,-32.0440739160477,
0.));
#120382=CARTESIAN_POINT('Ctrl Pts',(64.8278448184785,-32.0440739160477,
12.));
#120383=CARTESIAN_POINT('Ctrl Pts',(64.811064092502,-32.0261100384092,0.));
#120384=CARTESIAN_POINT('Ctrl Pts',(64.811064092502,-32.0261100384092,12.));
#120385=CARTESIAN_POINT('Ctrl Pts',(64.7942941396883,-32.0081923669678,
0.));
#120386=CARTESIAN_POINT('Ctrl Pts',(64.7942941396883,-32.0081923669678,
12.));
#120387=CARTESIAN_POINT('Ctrl Pts',(64.7775350800404,-31.9903209445522,
0.));
#120388=CARTESIAN_POINT('Ctrl Pts',(64.7775350800404,-31.9903209445522,
12.));
#120389=CARTESIAN_POINT('Ctrl Pts',(64.7607870340738,-31.9724958140791,
0.));
#120390=CARTESIAN_POINT('Ctrl Pts',(64.7607870340738,-31.9724958140791,
12.));
#120391=CARTESIAN_POINT('Ctrl Pts',(64.74405012282,-31.9547170185533,0.));
#120392=CARTESIAN_POINT('Ctrl Pts',(64.74405012282,-31.9547170185533,12.));
#120393=CARTESIAN_POINT('Ctrl Pts',(64.727324467829,-31.9369846010613,0.));
#120394=CARTESIAN_POINT('Ctrl Pts',(64.727324467829,-31.9369846010613,12.));
#120395=CARTESIAN_POINT('Ctrl Pts',(64.7106101911722,-31.9192986047702,
0.));
#120396=CARTESIAN_POINT('Ctrl Pts',(64.7106101911722,-31.9192986047702,
12.));
#120397=CARTESIAN_POINT('Ctrl Pts',(64.693907415449,-31.9016590729371,0.));
#120398=CARTESIAN_POINT('Ctrl Pts',(64.693907415449,-31.9016590729371,12.));
#120399=CARTESIAN_POINT('Ctrl Pts',(64.6772162637904,-31.8840660489106,
0.));
#120400=CARTESIAN_POINT('Ctrl Pts',(64.6772162637904,-31.8840660489106,
12.));
#120401=CARTESIAN_POINT('Ctrl Pts',(64.6605368598631,-31.8665195761312,
0.));
#120402=CARTESIAN_POINT('Ctrl Pts',(64.6605368598631,-31.8665195761312,
12.));
#120403=CARTESIAN_POINT('Ctrl Pts',(64.6438693278718,-31.849019698125,0.));
#120404=CARTESIAN_POINT('Ctrl Pts',(64.6438693278718,-31.849019698125,12.));
#120405=CARTESIAN_POINT('Ctrl Pts',(64.6272137925629,-31.8315664585027,
0.));
#120406=CARTESIAN_POINT('Ctrl Pts',(64.6272137925629,-31.8315664585027,
12.));
#120407=CARTESIAN_POINT('Ctrl Pts',(64.6105703792311,-31.8141599009685,
0.));
#120408=CARTESIAN_POINT('Ctrl Pts',(64.6105703792311,-31.8141599009685,
12.));
#120409=CARTESIAN_POINT('Ctrl Pts',(64.5939392137233,-31.7968000693218,
0.));
#120410=CARTESIAN_POINT('Ctrl Pts',(64.5939392137233,-31.7968000693218,
12.));
#120411=CARTESIAN_POINT('Ctrl Pts',(64.5773204224429,-31.7794870074584,
0.));
#120412=CARTESIAN_POINT('Ctrl Pts',(64.5773204224429,-31.7794870074584,
12.));
#120413=CARTESIAN_POINT('Ctrl Pts',(64.5607141323527,-31.7622207593637,
0.));
#120414=CARTESIAN_POINT('Ctrl Pts',(64.5607141323527,-31.7622207593637,
12.));
#120415=CARTESIAN_POINT('Ctrl Pts',(64.5441204709779,-31.7450013691117,
0.));
#120416=CARTESIAN_POINT('Ctrl Pts',(64.5441204709779,-31.7450013691117,
12.));
#120417=CARTESIAN_POINT('Ctrl Pts',(64.5275395664134,-31.7278288808736,
0.));
#120418=CARTESIAN_POINT('Ctrl Pts',(64.5275395664134,-31.7278288808736,
12.));
#120419=CARTESIAN_POINT('Ctrl Pts',(64.5109715473276,-31.7107033389204,
0.));
#120420=CARTESIAN_POINT('Ctrl Pts',(64.5109715473276,-31.7107033389204,
12.));
#120421=CARTESIAN_POINT('Ctrl Pts',(64.4944165429672,-31.6936247876228,
0.));
#120422=CARTESIAN_POINT('Ctrl Pts',(64.4944165429672,-31.6936247876228,
12.));
#120423=CARTESIAN_POINT('Ctrl Pts',(64.4778746831597,-31.6765932714456,
0.));
#120424=CARTESIAN_POINT('Ctrl Pts',(64.4778746831597,-31.6765932714456,
12.));
#120425=CARTESIAN_POINT('Ctrl Pts',(64.4613460983186,-31.6596088349468,
0.));
#120426=CARTESIAN_POINT('Ctrl Pts',(64.4613460983186,-31.6596088349468,
12.));
#120427=CARTESIAN_POINT('Ctrl Pts',(64.4448309194498,-31.6426715227865,
0.));
#120428=CARTESIAN_POINT('Ctrl Pts',(64.4448309194498,-31.6426715227865,
12.));
#120429=CARTESIAN_POINT('Ctrl Pts',(64.4283292781553,-31.6257813797282,
0.));
#120430=CARTESIAN_POINT('Ctrl Pts',(64.4283292781553,-31.6257813797282,
12.));
#120431=CARTESIAN_POINT('Ctrl Pts',(64.4118413066386,-31.6089384506399,
0.));
#120432=CARTESIAN_POINT('Ctrl Pts',(64.4118413066386,-31.6089384506399,
12.));
#120433=CARTESIAN_POINT('Ctrl Pts',(64.3953671377071,-31.5921427804879,
0.));
#120434=CARTESIAN_POINT('Ctrl Pts',(64.3953671377071,-31.5921427804879,
12.));
#120435=CARTESIAN_POINT('Ctrl Pts',(64.3789069047768,-31.5753944143355,
0.));
#120436=CARTESIAN_POINT('Ctrl Pts',(64.3789069047768,-31.5753944143355,
12.));
#120437=CARTESIAN_POINT('Ctrl Pts',(64.3624607418798,-31.5586933973532,
0.));
#120438=CARTESIAN_POINT('Ctrl Pts',(64.3624607418798,-31.5586933973532,
12.));
#120439=CARTESIAN_POINT('Ctrl Pts',(64.34602878367,-31.5420397748198,0.));
#120440=CARTESIAN_POINT('Ctrl Pts',(64.34602878367,-31.5420397748198,12.));
#120441=CARTESIAN_POINT('Ctrl Pts',(64.3296111654273,-31.525433592124,0.));
#120442=CARTESIAN_POINT('Ctrl Pts',(64.3296111654273,-31.525433592124,12.));
#120443=CARTESIAN_POINT('Ctrl Pts',(64.3132080230603,-31.5088748947565,
0.));
#120444=CARTESIAN_POINT('Ctrl Pts',(64.3132080230603,-31.5088748947565,
12.));
#120445=CARTESIAN_POINT('Ctrl Pts',(64.2968194931113,-31.4923637283109,
0.));
#120446=CARTESIAN_POINT('Ctrl Pts',(64.2968194931113,-31.4923637283109,
12.));
#120447=CARTESIAN_POINT('Ctrl Pts',(64.2804457127633,-31.4759001384923,
0.));
#120448=CARTESIAN_POINT('Ctrl Pts',(64.2804457127633,-31.4759001384923,
12.));
#120449=CARTESIAN_POINT('Ctrl Pts',(64.264086819846,-31.4594841711189,0.));
#120450=CARTESIAN_POINT('Ctrl Pts',(64.264086819846,-31.4594841711189,12.));
#120451=CARTESIAN_POINT('Ctrl Pts',(64.2477429528408,-31.443115872123,0.));
#120452=CARTESIAN_POINT('Ctrl Pts',(64.2477429528408,-31.443115872123,12.));
#120453=CARTESIAN_POINT('Ctrl Pts',(64.2314142508843,-31.426795287544,0.));
#120454=CARTESIAN_POINT('Ctrl Pts',(64.2314142508843,-31.426795287544,12.));
#120455=CARTESIAN_POINT('Ctrl Pts',(64.2151008537733,-31.4105224635298,
0.));
#120456=CARTESIAN_POINT('Ctrl Pts',(64.2151008537733,-31.4105224635298,
12.));
#120457=CARTESIAN_POINT('Ctrl Pts',(64.1988029019733,-31.3942974463458,
0.));
#120458=CARTESIAN_POINT('Ctrl Pts',(64.1988029019733,-31.3942974463458,
12.));
#120459=CARTESIAN_POINT('Ctrl Pts',(64.1825205366231,-31.3781202823758,
0.));
#120460=CARTESIAN_POINT('Ctrl Pts',(64.1825205366231,-31.3781202823758,
12.));
#120461=CARTESIAN_POINT('Ctrl Pts',(64.1662538995407,-31.3619910181223,
0.));
#120462=CARTESIAN_POINT('Ctrl Pts',(64.1662538995407,-31.3619910181223,
12.));
#120463=CARTESIAN_POINT('Ctrl Pts',(64.150003133226,-31.3459097001996,0.));
#120464=CARTESIAN_POINT('Ctrl Pts',(64.150003133226,-31.3459097001996,12.));
#120465=CARTESIAN_POINT('Ctrl Pts',(64.1337683808667,-31.3298763753366,
0.));
#120466=CARTESIAN_POINT('Ctrl Pts',(64.1337683808667,-31.3298763753366,
12.));
#120467=CARTESIAN_POINT('Ctrl Pts',(64.1175497863475,-31.3138910903852,
0.));
#120468=CARTESIAN_POINT('Ctrl Pts',(64.1175497863475,-31.3138910903852,
12.));
#120469=CARTESIAN_POINT('Ctrl Pts',(64.1013474942554,-31.2979538923214,
0.));
#120470=CARTESIAN_POINT('Ctrl Pts',(64.1013474942554,-31.2979538923214,
12.));
#120471=CARTESIAN_POINT('Ctrl Pts',(64.0851616498861,-31.2820648282451,
0.));
#120472=CARTESIAN_POINT('Ctrl Pts',(64.0851616498861,-31.2820648282451,
12.));
#120473=CARTESIAN_POINT('Ctrl Pts',(64.0689923992474,-31.2662239453734,
0.));
#120474=CARTESIAN_POINT('Ctrl Pts',(64.0689923992474,-31.2662239453734,
12.));
#120475=CARTESIAN_POINT('Ctrl Pts',(64.0528398890671,-31.2504312910457,
0.));
#120476=CARTESIAN_POINT('Ctrl Pts',(64.0528398890671,-31.2504312910457,
12.));
#120477=CARTESIAN_POINT('Ctrl Pts',(64.036704266799,-31.23468691273,0.));
#120478=CARTESIAN_POINT('Ctrl Pts',(64.036704266799,-31.23468691273,12.));
#120479=CARTESIAN_POINT('Ctrl Pts',(64.0205856806298,-31.2189908580245,
0.));
#120480=CARTESIAN_POINT('Ctrl Pts',(64.0205856806298,-31.2189908580245,
12.));
#120481=CARTESIAN_POINT('Ctrl Pts',(64.004484279483,-31.2033431746559,0.));
#120482=CARTESIAN_POINT('Ctrl Pts',(64.004484279483,-31.2033431746559,12.));
#120483=CARTESIAN_POINT('Ctrl Pts',(63.9884002130209,-31.1877439104717,
0.));
#120484=CARTESIAN_POINT('Ctrl Pts',(63.9884002130209,-31.1877439104717,
12.));
#120485=CARTESIAN_POINT('Ctrl Pts',(63.972333631655,-31.1721931134488,0.));
#120486=CARTESIAN_POINT('Ctrl Pts',(63.972333631655,-31.1721931134488,12.));
#120487=CARTESIAN_POINT('Ctrl Pts',(63.9562846865566,-31.1566908316993,
0.));
#120488=CARTESIAN_POINT('Ctrl Pts',(63.9562846865566,-31.1566908316993,
12.));
#120489=CARTESIAN_POINT('Ctrl Pts',(63.940253529665,-31.1412371134727,0.));
#120490=CARTESIAN_POINT('Ctrl Pts',(63.940253529665,-31.1412371134727,12.));
#120491=CARTESIAN_POINT('Ctrl Pts',(63.9242403136954,-31.1258320071545,
0.));
#120492=CARTESIAN_POINT('Ctrl Pts',(63.9242403136954,-31.1258320071545,
12.));
#120493=CARTESIAN_POINT('Ctrl Pts',(63.9082451921447,-31.1104755612606,
0.));
#120494=CARTESIAN_POINT('Ctrl Pts',(63.9082451921447,-31.1104755612606,
12.));
#120495=CARTESIAN_POINT('Ctrl Pts',(63.8922683192962,-31.0951678244454,
0.));
#120496=CARTESIAN_POINT('Ctrl Pts',(63.8922683192962,-31.0951678244454,
12.));
#120497=CARTESIAN_POINT('Ctrl Pts',(63.8763098502235,-31.079908845504,0.));
#120498=CARTESIAN_POINT('Ctrl Pts',(63.8763098502235,-31.079908845504,12.));
#120499=CARTESIAN_POINT('Ctrl Pts',(63.8603699407922,-31.0646986733724,
0.));
#120500=CARTESIAN_POINT('Ctrl Pts',(63.8603699407922,-31.0646986733724,
12.));
#120501=CARTESIAN_POINT('Ctrl Pts',(63.8444487476615,-31.0495373571218,
0.));
#120502=CARTESIAN_POINT('Ctrl Pts',(63.8444487476615,-31.0495373571218,
12.));
#120503=CARTESIAN_POINT('Ctrl Pts',(63.8285464282857,-31.0344249459544,
0.));
#120504=CARTESIAN_POINT('Ctrl Pts',(63.8285464282857,-31.0344249459544,
12.));
#120505=CARTESIAN_POINT('Ctrl Pts',(63.8126631409376,-31.0193614892177,
0.));
#120506=CARTESIAN_POINT('Ctrl Pts',(63.8126631409376,-31.0193614892177,
12.));
#120507=CARTESIAN_POINT('Ctrl Pts',(63.7967990447287,-31.0043470364112,
0.));
#120508=CARTESIAN_POINT('Ctrl Pts',(63.7967990447287,-31.0043470364112,
12.));
#120509=CARTESIAN_POINT('Ctrl Pts',(63.7809542996258,-30.9893816371907,
0.));
#120510=CARTESIAN_POINT('Ctrl Pts',(63.7809542996258,-30.9893816371907,
12.));
#120511=CARTESIAN_POINT('Ctrl Pts',(63.7651290664713,-30.9744653413679,
0.));
#120512=CARTESIAN_POINT('Ctrl Pts',(63.7651290664713,-30.9744653413679,
12.));
#120513=CARTESIAN_POINT('Ctrl Pts',(63.7493235069844,-30.9595981989091,
0.));
#120514=CARTESIAN_POINT('Ctrl Pts',(63.7493235069844,-30.9595981989091,
12.));
#120515=CARTESIAN_POINT('Ctrl Pts',(63.733537783742,-30.9447802599345,0.));
#120516=CARTESIAN_POINT('Ctrl Pts',(63.733537783742,-30.9447802599345,12.));
#120517=CARTESIAN_POINT('Ctrl Pts',(63.7177720601604,-30.9300115747113,
0.));
#120518=CARTESIAN_POINT('Ctrl Pts',(63.7177720601604,-30.9300115747113,
12.));
#120519=CARTESIAN_POINT('Ctrl Pts',(63.7020265004805,-30.9152921936471,
0.));
#120520=CARTESIAN_POINT('Ctrl Pts',(63.7020265004805,-30.9152921936471,
12.));
#120521=CARTESIAN_POINT('Ctrl Pts',(63.6863012697353,-30.9006221672703,
0.));
#120522=CARTESIAN_POINT('Ctrl Pts',(63.6863012697353,-30.9006221672703,
12.));
#120523=CARTESIAN_POINT('Ctrl Pts',(63.6705965337996,-30.8860015462488,
0.));
#120524=CARTESIAN_POINT('Ctrl Pts',(63.6705965337996,-30.8860015462488,
12.));
#120525=CARTESIAN_POINT('Ctrl Pts',(63.6549124594681,-30.8714303814202,
0.));
#120526=CARTESIAN_POINT('Ctrl Pts',(63.6549124594681,-30.8714303814202,
12.));
#120527=CARTESIAN_POINT('Ctrl Pts',(63.6392492145233,-30.8569087238132,
0.));
#120528=CARTESIAN_POINT('Ctrl Pts',(63.6392492145233,-30.8569087238132,
12.));
#120529=CARTESIAN_POINT('Ctrl Pts',(63.6236069678041,-30.8424366246665,
0.));
#120530=CARTESIAN_POINT('Ctrl Pts',(63.6236069678041,-30.8424366246665,
12.));
#120531=CARTESIAN_POINT('Ctrl Pts',(63.6079858892746,-30.8280141354448,
0.));
#120532=CARTESIAN_POINT('Ctrl Pts',(63.6079858892746,-30.8280141354448,
12.));
#120533=CARTESIAN_POINT('Ctrl Pts',(63.5923861498963,-30.8136413077999,
0.));
#120534=CARTESIAN_POINT('Ctrl Pts',(63.5923861498963,-30.8136413077999,
12.));
#120535=CARTESIAN_POINT('Ctrl Pts',(63.5768079214868,-30.7993181935265,
0.));
#120536=CARTESIAN_POINT('Ctrl Pts',(63.5768079214868,-30.7993181935265,
12.));
#120537=CARTESIAN_POINT('Ctrl Pts',(63.5612513766005,-30.7850448445207,
0.));
#120538=CARTESIAN_POINT('Ctrl Pts',(63.5612513766005,-30.7850448445207,
12.));
#120539=CARTESIAN_POINT('Ctrl Pts',(63.5457166883558,-30.7708213127169,
0.));
#120540=CARTESIAN_POINT('Ctrl Pts',(63.5457166883558,-30.7708213127169,
12.));
#120541=CARTESIAN_POINT('Ctrl Pts',(63.5302040304173,-30.7566476500772,
0.));
#120542=CARTESIAN_POINT('Ctrl Pts',(63.5302040304173,-30.7566476500772,
12.));
#120543=CARTESIAN_POINT('Ctrl Pts',(63.514713577392,-30.7425239087294,0.));
#120544=CARTESIAN_POINT('Ctrl Pts',(63.514713577392,-30.7425239087294,12.));
#120545=CARTESIAN_POINT('Ctrl Pts',(63.4992455051805,-30.7284501410827,
0.));
#120546=CARTESIAN_POINT('Ctrl Pts',(63.4992455051805,-30.7284501410827,
12.));
#120547=CARTESIAN_POINT('Ctrl Pts',(63.4837999912758,-30.7144263999259,
0.));
#120548=CARTESIAN_POINT('Ctrl Pts',(63.4837999912758,-30.7144263999259,
12.));
#120549=CARTESIAN_POINT('Ctrl Pts',(63.4683772152497,-30.7004527385806,
0.));
#120550=CARTESIAN_POINT('Ctrl Pts',(63.4683772152497,-30.7004527385806,
12.));
#120551=CARTESIAN_POINT('Ctrl Pts',(63.452977358421,-30.6865292107911,0.));
#120552=CARTESIAN_POINT('Ctrl Pts',(63.452977358421,-30.6865292107911,12.));
#120553=CARTESIAN_POINT('Ctrl Pts',(63.4376006029575,-30.6726558704302,
0.));
#120554=CARTESIAN_POINT('Ctrl Pts',(63.4376006029575,-30.6726558704302,
12.));
#120555=CARTESIAN_POINT('Ctrl Pts',(63.4222471311236,-30.6588327712482,
0.));
#120556=CARTESIAN_POINT('Ctrl Pts',(63.4222471311236,-30.6588327712482,
12.));
#120557=CARTESIAN_POINT('Ctrl Pts',(63.4069171245093,-30.6450599666135,
0.));
#120558=CARTESIAN_POINT('Ctrl Pts',(63.4069171245093,-30.6450599666135,
12.));
#120559=CARTESIAN_POINT('Ctrl Pts',(63.3916107631421,-30.6313375092085,
0.));
#120560=CARTESIAN_POINT('Ctrl Pts',(63.3916107631421,-30.6313375092085,
12.));
#120561=CARTESIAN_POINT('Ctrl Pts',(63.3763282271838,-30.6176654515988,
0.));
#120562=CARTESIAN_POINT('Ctrl Pts',(63.3763282271838,-30.6176654515988,
12.));
#120563=CARTESIAN_POINT('Ctrl Pts',(63.3610696989599,-30.604043846909,0.));
#120564=CARTESIAN_POINT('Ctrl Pts',(63.3610696989599,-30.604043846909,12.));
#120565=CARTESIAN_POINT('Ctrl Pts',(63.3458353646144,-30.5904727493707,
0.));
#120566=CARTESIAN_POINT('Ctrl Pts',(63.3458353646144,-30.5904727493707,
12.));
#120567=CARTESIAN_POINT('Ctrl Pts',(63.330625416509,-30.5769522151147,0.));
#120568=CARTESIAN_POINT('Ctrl Pts',(63.330625416509,-30.5769522151147,12.));
#120569=CARTESIAN_POINT('Ctrl Pts',(63.315440053435,-30.5634823022358,0.));
#120570=CARTESIAN_POINT('Ctrl Pts',(63.315440053435,-30.5634823022358,12.));
#120571=CARTESIAN_POINT('Ctrl Pts',(63.3002794756049,-30.5500630691343,
0.));
#120572=CARTESIAN_POINT('Ctrl Pts',(63.3002794756049,-30.5500630691343,
12.));
#120573=CARTESIAN_POINT('Ctrl Pts',(63.2851438802462,-30.5366945730503,
0.));
#120574=CARTESIAN_POINT('Ctrl Pts',(63.2851438802462,-30.5366945730503,
12.));
#120575=CARTESIAN_POINT('Ctrl Pts',(63.2700334577661,-30.5233768687875,
0.));
#120576=CARTESIAN_POINT('Ctrl Pts',(63.2700334577661,-30.5233768687875,
12.));
#120577=CARTESIAN_POINT('Ctrl Pts',(63.2549483856268,-30.5101100066683,
0.));
#120578=CARTESIAN_POINT('Ctrl Pts',(63.2549483856268,-30.5101100066683,
12.));
#120579=CARTESIAN_POINT('Ctrl Pts',(63.2398888342612,-30.4968940345028,
0.));
#120580=CARTESIAN_POINT('Ctrl Pts',(63.2398888342612,-30.4968940345028,
12.));
#120581=CARTESIAN_POINT('Ctrl Pts',(63.2248549788272,-30.4837290015011,
0.));
#120582=CARTESIAN_POINT('Ctrl Pts',(63.2248549788272,-30.4837290015011,
12.));
#120583=CARTESIAN_POINT('Ctrl Pts',(63.2098470086636,-30.470614961416,0.));
#120584=CARTESIAN_POINT('Ctrl Pts',(63.2098470086636,-30.470614961416,12.));
#120585=CARTESIAN_POINT('Ctrl Pts',(63.1948651386868,-30.4575519763305,
0.));
#120586=CARTESIAN_POINT('Ctrl Pts',(63.1948651386868,-30.4575519763305,
12.));
#120587=CARTESIAN_POINT('Ctrl Pts',(63.1799096171757,-30.4445401192324,
0.));
#120588=CARTESIAN_POINT('Ctrl Pts',(63.1799096171757,-30.4445401192324,
12.));
#120589=CARTESIAN_POINT('Ctrl Pts',(63.1649807016766,-30.431579465967,0.));
#120590=CARTESIAN_POINT('Ctrl Pts',(63.1649807016766,-30.431579465967,12.));
#120591=CARTESIAN_POINT('Ctrl Pts',(63.1500786361382,-30.4186700875598,
0.));
#120592=CARTESIAN_POINT('Ctrl Pts',(63.1500786361382,-30.4186700875598,
12.));
#120593=CARTESIAN_POINT('Ctrl Pts',(63.1352036298512,-30.4058120432259,
0.));
#120594=CARTESIAN_POINT('Ctrl Pts',(63.1352036298512,-30.4058120432259,
12.));
#120595=CARTESIAN_POINT('Ctrl Pts',(63.1203558300911,-30.3930053710592,
0.));
#120596=CARTESIAN_POINT('Ctrl Pts',(63.1203558300911,-30.3930053710592,
12.));
#120597=CARTESIAN_POINT('Ctrl Pts',(63.1055353202641,-30.3802500880565,
0.));
#120598=CARTESIAN_POINT('Ctrl Pts',(63.1055353202641,-30.3802500880565,
12.));
#120599=CARTESIAN_POINT('Ctrl Pts',(63.0937007763826,-30.3700869762658,
0.));
#120600=CARTESIAN_POINT('Ctrl Pts',(63.0937007763826,-30.3700869762658,
12.));
#120601=CARTESIAN_POINT('Ctrl Pts',(63.0848371718274,-30.3624877680747,
0.));
#120602=CARTESIAN_POINT('Ctrl Pts',(63.0848371718274,-30.3624877680747,
12.));
#120603=CARTESIAN_POINT('Ctrl Pts',(63.0789335700774,-30.3574319069366,
0.));
#120604=CARTESIAN_POINT('Ctrl Pts',(63.0789335700774,-30.3574319069366,
12.));
#120605=CARTESIAN_POINT('Ctrl Pts',(63.0759831361898,-30.3549065457811,
0.));
#120606=CARTESIAN_POINT('Ctrl Pts',(63.0759831361898,-30.3549065457811,
12.));
#120607=CARTESIAN_POINT('',(63.0759831361898,-30.3549065457811,12.));
#120608=CARTESIAN_POINT('Ctrl Pts',(63.0759831361898,-30.3549065457811,
12.));
#120609=CARTESIAN_POINT('Ctrl Pts',(63.0789335700774,-30.3574319069366,
12.));
#120610=CARTESIAN_POINT('Ctrl Pts',(63.0848371718274,-30.3624877680747,
12.));
#120611=CARTESIAN_POINT('Ctrl Pts',(63.0937007763826,-30.3700869762658,
12.));
#120612=CARTESIAN_POINT('Ctrl Pts',(63.1055353202641,-30.3802500880565,
12.));
#120613=CARTESIAN_POINT('Ctrl Pts',(63.1203558300911,-30.3930053710592,
12.));
#120614=CARTESIAN_POINT('Ctrl Pts',(63.1352036298512,-30.4058120432259,
12.));
#120615=CARTESIAN_POINT('Ctrl Pts',(63.1500786361382,-30.4186700875598,
12.));
#120616=CARTESIAN_POINT('Ctrl Pts',(63.1649807016766,-30.431579465967,12.));
#120617=CARTESIAN_POINT('Ctrl Pts',(63.1799096171757,-30.4445401192324,
12.));
#120618=CARTESIAN_POINT('Ctrl Pts',(63.1948651386868,-30.4575519763305,
12.));
#120619=CARTESIAN_POINT('Ctrl Pts',(63.2098470086636,-30.470614961416,12.));
#120620=CARTESIAN_POINT('Ctrl Pts',(63.2248549788272,-30.4837290015011,
12.));
#120621=CARTESIAN_POINT('Ctrl Pts',(63.2398888342612,-30.4968940345028,
12.));
#120622=CARTESIAN_POINT('Ctrl Pts',(63.2549483856268,-30.5101100066683,
12.));
#120623=CARTESIAN_POINT('Ctrl Pts',(63.2700334577661,-30.5233768687875,
12.));
#120624=CARTESIAN_POINT('Ctrl Pts',(63.2851438802462,-30.5366945730503,
12.));
#120625=CARTESIAN_POINT('Ctrl Pts',(63.3002794756049,-30.5500630691343,
12.));
#120626=CARTESIAN_POINT('Ctrl Pts',(63.315440053435,-30.5634823022358,12.));
#120627=CARTESIAN_POINT('Ctrl Pts',(63.330625416509,-30.5769522151147,12.));
#120628=CARTESIAN_POINT('Ctrl Pts',(63.3458353646144,-30.5904727493707,
12.));
#120629=CARTESIAN_POINT('Ctrl Pts',(63.3610696989599,-30.604043846909,12.));
#120630=CARTESIAN_POINT('Ctrl Pts',(63.3763282271838,-30.6176654515988,
12.));
#120631=CARTESIAN_POINT('Ctrl Pts',(63.3916107631421,-30.6313375092085,
12.));
#120632=CARTESIAN_POINT('Ctrl Pts',(63.4069171245093,-30.6450599666135,
12.));
#120633=CARTESIAN_POINT('Ctrl Pts',(63.4222471311236,-30.6588327712482,
12.));
#120634=CARTESIAN_POINT('Ctrl Pts',(63.4376006029575,-30.6726558704302,
12.));
#120635=CARTESIAN_POINT('Ctrl Pts',(63.452977358421,-30.6865292107911,12.));
#120636=CARTESIAN_POINT('Ctrl Pts',(63.4683772152497,-30.7004527385806,
12.));
#120637=CARTESIAN_POINT('Ctrl Pts',(63.4837999912758,-30.7144263999259,
12.));
#120638=CARTESIAN_POINT('Ctrl Pts',(63.4992455051805,-30.7284501410827,
12.));
#120639=CARTESIAN_POINT('Ctrl Pts',(63.514713577392,-30.7425239087294,12.));
#120640=CARTESIAN_POINT('Ctrl Pts',(63.5302040304173,-30.7566476500772,
12.));
#120641=CARTESIAN_POINT('Ctrl Pts',(63.5457166883558,-30.7708213127169,
12.));
#120642=CARTESIAN_POINT('Ctrl Pts',(63.5612513766005,-30.7850448445207,
12.));
#120643=CARTESIAN_POINT('Ctrl Pts',(63.5768079214868,-30.7993181935265,
12.));
#120644=CARTESIAN_POINT('Ctrl Pts',(63.5923861498963,-30.8136413077999,
12.));
#120645=CARTESIAN_POINT('Ctrl Pts',(63.6079858892746,-30.8280141354448,
12.));
#120646=CARTESIAN_POINT('Ctrl Pts',(63.6236069678041,-30.8424366246665,
12.));
#120647=CARTESIAN_POINT('Ctrl Pts',(63.6392492145233,-30.8569087238132,
12.));
#120648=CARTESIAN_POINT('Ctrl Pts',(63.6549124594681,-30.8714303814202,
12.));
#120649=CARTESIAN_POINT('Ctrl Pts',(63.6705965337996,-30.8860015462488,
12.));
#120650=CARTESIAN_POINT('Ctrl Pts',(63.6863012697353,-30.9006221672703,
12.));
#120651=CARTESIAN_POINT('Ctrl Pts',(63.7020265004805,-30.9152921936471,
12.));
#120652=CARTESIAN_POINT('Ctrl Pts',(63.7177720601604,-30.9300115747113,
12.));
#120653=CARTESIAN_POINT('Ctrl Pts',(63.733537783742,-30.9447802599345,12.));
#120654=CARTESIAN_POINT('Ctrl Pts',(63.7493235069844,-30.9595981989091,
12.));
#120655=CARTESIAN_POINT('Ctrl Pts',(63.7651290664713,-30.9744653413679,
12.));
#120656=CARTESIAN_POINT('Ctrl Pts',(63.7809542996258,-30.9893816371907,
12.));
#120657=CARTESIAN_POINT('Ctrl Pts',(63.7967990447287,-31.0043470364112,
12.));
#120658=CARTESIAN_POINT('Ctrl Pts',(63.8126631409376,-31.0193614892177,
12.));
#120659=CARTESIAN_POINT('Ctrl Pts',(63.8285464282857,-31.0344249459544,
12.));
#120660=CARTESIAN_POINT('Ctrl Pts',(63.8444487476615,-31.0495373571218,
12.));
#120661=CARTESIAN_POINT('Ctrl Pts',(63.8603699407922,-31.0646986733724,
12.));
#120662=CARTESIAN_POINT('Ctrl Pts',(63.8763098502235,-31.079908845504,12.));
#120663=CARTESIAN_POINT('Ctrl Pts',(63.8922683192962,-31.0951678244454,
12.));
#120664=CARTESIAN_POINT('Ctrl Pts',(63.9082451921447,-31.1104755612606,
12.));
#120665=CARTESIAN_POINT('Ctrl Pts',(63.9242403136954,-31.1258320071545,
12.));
#120666=CARTESIAN_POINT('Ctrl Pts',(63.940253529665,-31.1412371134727,12.));
#120667=CARTESIAN_POINT('Ctrl Pts',(63.9562846865566,-31.1566908316993,
12.));
#120668=CARTESIAN_POINT('Ctrl Pts',(63.972333631655,-31.1721931134488,12.));
#120669=CARTESIAN_POINT('Ctrl Pts',(63.9884002130209,-31.1877439104717,
12.));
#120670=CARTESIAN_POINT('Ctrl Pts',(64.004484279483,-31.2033431746559,12.));
#120671=CARTESIAN_POINT('Ctrl Pts',(64.0205856806298,-31.2189908580245,
12.));
#120672=CARTESIAN_POINT('Ctrl Pts',(64.036704266799,-31.23468691273,12.));
#120673=CARTESIAN_POINT('Ctrl Pts',(64.0528398890671,-31.2504312910457,
12.));
#120674=CARTESIAN_POINT('Ctrl Pts',(64.0689923992474,-31.2662239453734,
12.));
#120675=CARTESIAN_POINT('Ctrl Pts',(64.0851616498861,-31.2820648282451,
12.));
#120676=CARTESIAN_POINT('Ctrl Pts',(64.1013474942554,-31.2979538923214,
12.));
#120677=CARTESIAN_POINT('Ctrl Pts',(64.1175497863475,-31.3138910903852,
12.));
#120678=CARTESIAN_POINT('Ctrl Pts',(64.1337683808667,-31.3298763753366,
12.));
#120679=CARTESIAN_POINT('Ctrl Pts',(64.150003133226,-31.3459097001996,12.));
#120680=CARTESIAN_POINT('Ctrl Pts',(64.1662538995407,-31.3619910181223,
12.));
#120681=CARTESIAN_POINT('Ctrl Pts',(64.1825205366231,-31.3781202823758,
12.));
#120682=CARTESIAN_POINT('Ctrl Pts',(64.1988029019733,-31.3942974463458,
12.));
#120683=CARTESIAN_POINT('Ctrl Pts',(64.2151008537733,-31.4105224635298,
12.));
#120684=CARTESIAN_POINT('Ctrl Pts',(64.2314142508843,-31.426795287544,12.));
#120685=CARTESIAN_POINT('Ctrl Pts',(64.2477429528408,-31.443115872123,12.));
#120686=CARTESIAN_POINT('Ctrl Pts',(64.264086819846,-31.4594841711189,12.));
#120687=CARTESIAN_POINT('Ctrl Pts',(64.2804457127633,-31.4759001384923,
12.));
#120688=CARTESIAN_POINT('Ctrl Pts',(64.2968194931113,-31.4923637283109,
12.));
#120689=CARTESIAN_POINT('Ctrl Pts',(64.3132080230603,-31.5088748947565,
12.));
#120690=CARTESIAN_POINT('Ctrl Pts',(64.3296111654273,-31.525433592124,12.));
#120691=CARTESIAN_POINT('Ctrl Pts',(64.34602878367,-31.5420397748198,12.));
#120692=CARTESIAN_POINT('Ctrl Pts',(64.3624607418798,-31.5586933973532,
12.));
#120693=CARTESIAN_POINT('Ctrl Pts',(64.3789069047768,-31.5753944143355,
12.));
#120694=CARTESIAN_POINT('Ctrl Pts',(64.3953671377071,-31.5921427804879,
12.));
#120695=CARTESIAN_POINT('Ctrl Pts',(64.4118413066386,-31.6089384506399,
12.));
#120696=CARTESIAN_POINT('Ctrl Pts',(64.4283292781553,-31.6257813797282,
12.));
#120697=CARTESIAN_POINT('Ctrl Pts',(64.4448309194498,-31.6426715227865,
12.));
#120698=CARTESIAN_POINT('Ctrl Pts',(64.4613460983186,-31.6596088349468,
12.));
#120699=CARTESIAN_POINT('Ctrl Pts',(64.4778746831597,-31.6765932714456,
12.));
#120700=CARTESIAN_POINT('Ctrl Pts',(64.4944165429672,-31.6936247876228,
12.));
#120701=CARTESIAN_POINT('Ctrl Pts',(64.5109715473276,-31.7107033389204,
12.));
#120702=CARTESIAN_POINT('Ctrl Pts',(64.5275395664134,-31.7278288808736,
12.));
#120703=CARTESIAN_POINT('Ctrl Pts',(64.5441204709779,-31.7450013691117,
12.));
#120704=CARTESIAN_POINT('Ctrl Pts',(64.5607141323527,-31.7622207593637,
12.));
#120705=CARTESIAN_POINT('Ctrl Pts',(64.5773204224429,-31.7794870074584,
12.));
#120706=CARTESIAN_POINT('Ctrl Pts',(64.5939392137233,-31.7968000693218,
12.));
#120707=CARTESIAN_POINT('Ctrl Pts',(64.6105703792311,-31.8141599009685,
12.));
#120708=CARTESIAN_POINT('Ctrl Pts',(64.6272137925629,-31.8315664585027,
12.));
#120709=CARTESIAN_POINT('Ctrl Pts',(64.6438693278718,-31.849019698125,12.));
#120710=CARTESIAN_POINT('Ctrl Pts',(64.6605368598631,-31.8665195761312,
12.));
#120711=CARTESIAN_POINT('Ctrl Pts',(64.6772162637904,-31.8840660489106,
12.));
#120712=CARTESIAN_POINT('Ctrl Pts',(64.693907415449,-31.9016590729371,12.));
#120713=CARTESIAN_POINT('Ctrl Pts',(64.7106101911722,-31.9192986047702,
12.));
#120714=CARTESIAN_POINT('Ctrl Pts',(64.727324467829,-31.9369846010613,12.));
#120715=CARTESIAN_POINT('Ctrl Pts',(64.74405012282,-31.9547170185533,12.));
#120716=CARTESIAN_POINT('Ctrl Pts',(64.7607870340738,-31.9724958140791,
12.));
#120717=CARTESIAN_POINT('Ctrl Pts',(64.7775350800404,-31.9903209445522,
12.));
#120718=CARTESIAN_POINT('Ctrl Pts',(64.7942941396883,-32.0081923669678,
12.));
#120719=CARTESIAN_POINT('Ctrl Pts',(64.811064092502,-32.0261100384092,12.));
#120720=CARTESIAN_POINT('Ctrl Pts',(64.8278448184785,-32.0440739160477,
12.));
#120721=CARTESIAN_POINT('Ctrl Pts',(64.8446361981234,-32.0620839571409,
12.));
#120722=CARTESIAN_POINT('Ctrl Pts',(64.8614381124454,-32.0801401190244,
12.));
#120723=CARTESIAN_POINT('Ctrl Pts',(64.8782504429527,-32.0982423591113,
12.));
#120724=CARTESIAN_POINT('Ctrl Pts',(64.8950730716501,-32.1163906348984,
12.));
#120725=CARTESIAN_POINT('Ctrl Pts',(64.9119058810366,-32.1345849039674,
12.));
#120726=CARTESIAN_POINT('Ctrl Pts',(64.9287487541015,-32.1528251239831,
12.));
#120727=CARTESIAN_POINT('Ctrl Pts',(64.9456015743192,-32.1711112526855,
12.));
#120728=CARTESIAN_POINT('Ctrl Pts',(64.9624642256461,-32.1894432478881,
12.));
#120729=CARTESIAN_POINT('Ctrl Pts',(64.9793365925178,-32.207821067485,12.));
#120730=CARTESIAN_POINT('Ctrl Pts',(64.9962185598461,-32.2262446694513,
12.));
#120731=CARTESIAN_POINT('Ctrl Pts',(65.0131100130157,-32.2447140118422,
12.));
#120732=CARTESIAN_POINT('Ctrl Pts',(65.03001083788,-32.2632290527862,12.));
#120733=CARTESIAN_POINT('Ctrl Pts',(65.0469209207563,-32.2817897504807,
12.));
#120734=CARTESIAN_POINT('Ctrl Pts',(65.0638401484257,-32.3003960632007,
12.));
#120735=CARTESIAN_POINT('Ctrl Pts',(65.0807684081281,-32.3190479492987,
12.));
#120736=CARTESIAN_POINT('Ctrl Pts',(65.0977055875607,-32.3377453672051,
12.));
#120737=CARTESIAN_POINT('Ctrl Pts',(65.1146515748722,-32.3564882754212,
12.));
#120738=CARTESIAN_POINT('Ctrl Pts',(65.1316062586588,-32.3752766325136,
12.));
#120739=CARTESIAN_POINT('Ctrl Pts',(65.1485695279635,-32.3941103971221,
12.));
#120740=CARTESIAN_POINT('Ctrl Pts',(65.1655412722725,-32.4129895279615,
12.));
#120741=CARTESIAN_POINT('Ctrl Pts',(65.182521381514,-32.4319139838213,12.));
#120742=CARTESIAN_POINT('Ctrl Pts',(65.1995097460538,-32.450883723561,12.));
#120743=CARTESIAN_POINT('Ctrl Pts',(65.2165062566924,-32.4698987061032,
12.));
#120744=CARTESIAN_POINT('Ctrl Pts',(65.2335108046614,-32.4889588904392,
12.));
#120745=CARTESIAN_POINT('Ctrl Pts',(65.2505232816209,-32.5080642356328,
12.));
#120746=CARTESIAN_POINT('Ctrl Pts',(65.2675435796558,-32.5272147008191,
12.));
#120747=CARTESIAN_POINT('Ctrl Pts',(65.2845715912721,-32.5464102452015,
12.));
#120748=CARTESIAN_POINT('Ctrl Pts',(65.3016072093912,-32.5656508280422,
12.));
#120749=CARTESIAN_POINT('Ctrl Pts',(65.31865032735,-32.5849364086679,12.));
#120750=CARTESIAN_POINT('Ctrl Pts',(65.3357008389003,-32.6042669464751,
12.));
#120751=CARTESIAN_POINT('Ctrl Pts',(65.3527586382081,-32.6236424009301,
12.));
#120752=CARTESIAN_POINT('Ctrl Pts',(65.3698236198512,-32.6430627315674,
12.));
#120753=CARTESIAN_POINT('Ctrl Pts',(65.3868956788182,-32.6625278979811,
12.));
#120754=CARTESIAN_POINT('Ctrl Pts',(65.4039747105038,-32.6820378598267,
12.));
#120755=CARTESIAN_POINT('Ctrl Pts',(65.4210606107035,-32.7015925768265,
12.));
#120756=CARTESIAN_POINT('Ctrl Pts',(65.4381532756065,-32.7211920087684,
12.));
#120757=CARTESIAN_POINT('Ctrl Pts',(65.4552526017905,-32.7408361155037,
12.));
#120758=CARTESIAN_POINT('Ctrl Pts',(65.4723584862122,-32.7605248569378,
12.));
#120759=CARTESIAN_POINT('Ctrl Pts',(65.489470826206,-32.7802581930287,12.));
#120760=CARTESIAN_POINT('Ctrl Pts',(65.5065895194928,-32.8000360837975,
12.));
#120761=CARTESIAN_POINT('Ctrl Pts',(65.5237144641857,-32.8198584893316,
12.));
#120762=CARTESIAN_POINT('Ctrl Pts',(65.5408455587964,-32.8397253697866,
12.));
#120763=CARTESIAN_POINT('Ctrl Pts',(65.5579827022421,-32.8596366853832,
12.));
#120764=CARTESIAN_POINT('Ctrl Pts',(65.5751257938472,-32.879592396403,12.));
#120765=CARTESIAN_POINT('Ctrl Pts',(65.5922747333194,-32.8995924631898,
12.));
#120766=CARTESIAN_POINT('Ctrl Pts',(65.6094294207276,-32.9196368461463,
12.));
#120767=CARTESIAN_POINT('Ctrl Pts',(65.6265897564783,-32.9397255057274,
12.));
#120768=CARTESIAN_POINT('Ctrl Pts',(65.6437556412946,-32.9598584024313,
12.));
#120769=CARTESIAN_POINT('Ctrl Pts',(65.6609269761888,-32.980035496784,12.));
#120770=CARTESIAN_POINT('Ctrl Pts',(65.6781036625027,-33.0002567493574,
12.));
#120771=CARTESIAN_POINT('Ctrl Pts',(65.6952856019533,-33.0205221207873,
12.));
#120772=CARTESIAN_POINT('Ctrl Pts',(65.7124726966802,-33.0408315717873,
12.));
#120773=CARTESIAN_POINT('Ctrl Pts',(65.7296648492824,-33.0611850631582,
12.));
#120774=CARTESIAN_POINT('Ctrl Pts',(65.7468619628815,-33.081582555798,12.));
#120775=CARTESIAN_POINT('Ctrl Pts',(65.7640639410661,-33.1020240106885,
12.));
#120776=CARTESIAN_POINT('Ctrl Pts',(65.7812706877696,-33.1225093888672,
12.));
#120777=CARTESIAN_POINT('Ctrl Pts',(65.7984821071623,-33.1430386513976,
12.));
#120778=CARTESIAN_POINT('Ctrl Pts',(65.8156981035503,-33.16361175934,12.));
#120779=CARTESIAN_POINT('Ctrl Pts',(65.8329185812375,-33.1842286737051,
12.));
#120780=CARTESIAN_POINT('Ctrl Pts',(65.8501434445164,-33.2048893554491,
12.));
#120781=CARTESIAN_POINT('Ctrl Pts',(65.8673725979577,-33.2255937655649,
12.));
#120782=CARTESIAN_POINT('Ctrl Pts',(65.8846059466371,-33.2463418651493,
12.));
#120783=CARTESIAN_POINT('Ctrl Pts',(65.9018433963889,-33.2671336154754,
12.));
#120784=CARTESIAN_POINT('Ctrl Pts',(65.9190848540433,-33.2879689780573,
12.));
#120785=CARTESIAN_POINT('Ctrl Pts',(65.9363302276846,-33.3088479147164,
12.));
#120786=CARTESIAN_POINT('Ctrl Pts',(65.9535794260831,-33.3297703874266,
12.));
#120787=CARTESIAN_POINT('Ctrl Pts',(65.970832358141,-33.3507363581593,12.));
#120788=CARTESIAN_POINT('Ctrl Pts',(65.9880889322831,-33.37174578871,12.));
#120789=CARTESIAN_POINT('Ctrl Pts',(66.0053490559812,-33.3927986405605,
12.));
#120790=CARTESIAN_POINT('Ctrl Pts',(66.0226126349446,-33.4138948746388,
12.));
#120791=CARTESIAN_POINT('Ctrl Pts',(66.0398795737777,-33.4350344515101,
12.));
#120792=CARTESIAN_POINT('Ctrl Pts',(66.0571497774434,-33.4562173318025,
12.));
#120793=CARTESIAN_POINT('Ctrl Pts',(66.0744231525415,-33.4774434765746,
12.));
#120794=CARTESIAN_POINT('Ctrl Pts',(66.0916996085244,-33.4987128476622,
12.));
#120795=CARTESIAN_POINT('Ctrl Pts',(66.1089790592729,-33.5200254081243,
12.));
#120796=CARTESIAN_POINT('Ctrl Pts',(66.1262614234674,-33.5413811223451,
12.));
#120797=CARTESIAN_POINT('Ctrl Pts',(66.1410781873278,-33.5597240685846,
12.));
#120798=CARTESIAN_POINT('Ctrl Pts',(66.1524393974174,-33.5738105077875,
12.));
#120799=CARTESIAN_POINT('Ctrl Pts',(66.1603438177522,-33.5836213514189,
12.));
#120800=CARTESIAN_POINT('Ctrl Pts',(66.1647906582657,-33.5891439876494,
12.));
#120801=CARTESIAN_POINT('Ctrl Pts',(66.1657795405962,-33.590372266528,12.));
#120802=CARTESIAN_POINT('',(63.0759831361898,-30.3549065457811,0.));
#120803=CARTESIAN_POINT('',(63.0759831361898,-30.3549065457811,0.));
#120804=CARTESIAN_POINT('Ctrl Pts',(66.1657795405962,-33.590372266528,0.));
#120805=CARTESIAN_POINT('Ctrl Pts',(66.1647906582657,-33.5891439876494,
0.));
#120806=CARTESIAN_POINT('Ctrl Pts',(66.1603438177522,-33.5836213514189,
0.));
#120807=CARTESIAN_POINT('Ctrl Pts',(66.1524393974174,-33.5738105077875,
0.));
#120808=CARTESIAN_POINT('Ctrl Pts',(66.1410781873278,-33.5597240685846,
0.));
#120809=CARTESIAN_POINT('Ctrl Pts',(66.1262614234674,-33.5413811223451,
0.));
#120810=CARTESIAN_POINT('Ctrl Pts',(66.1089790592729,-33.5200254081243,
0.));
#120811=CARTESIAN_POINT('Ctrl Pts',(66.0916996085244,-33.4987128476622,
0.));
#120812=CARTESIAN_POINT('Ctrl Pts',(66.0744231525415,-33.4774434765746,
0.));
#120813=CARTESIAN_POINT('Ctrl Pts',(66.0571497774434,-33.4562173318025,
0.));
#120814=CARTESIAN_POINT('Ctrl Pts',(66.0398795737777,-33.4350344515101,
0.));
#120815=CARTESIAN_POINT('Ctrl Pts',(66.0226126349446,-33.4138948746388,
0.));
#120816=CARTESIAN_POINT('Ctrl Pts',(66.0053490559812,-33.3927986405605,
0.));
#120817=CARTESIAN_POINT('Ctrl Pts',(65.9880889322831,-33.37174578871,0.));
#120818=CARTESIAN_POINT('Ctrl Pts',(65.970832358141,-33.3507363581593,0.));
#120819=CARTESIAN_POINT('Ctrl Pts',(65.9535794260831,-33.3297703874266,
0.));
#120820=CARTESIAN_POINT('Ctrl Pts',(65.9363302276846,-33.3088479147164,
0.));
#120821=CARTESIAN_POINT('Ctrl Pts',(65.9190848540433,-33.2879689780573,
0.));
#120822=CARTESIAN_POINT('Ctrl Pts',(65.9018433963889,-33.2671336154754,
0.));
#120823=CARTESIAN_POINT('Ctrl Pts',(65.8846059466371,-33.2463418651493,
0.));
#120824=CARTESIAN_POINT('Ctrl Pts',(65.8673725979577,-33.2255937655649,
0.));
#120825=CARTESIAN_POINT('Ctrl Pts',(65.8501434445164,-33.2048893554491,
0.));
#120826=CARTESIAN_POINT('Ctrl Pts',(65.8329185812375,-33.1842286737051,
0.));
#120827=CARTESIAN_POINT('Ctrl Pts',(65.8156981035503,-33.16361175934,0.));
#120828=CARTESIAN_POINT('Ctrl Pts',(65.7984821071623,-33.1430386513976,
0.));
#120829=CARTESIAN_POINT('Ctrl Pts',(65.7812706877696,-33.1225093888672,
0.));
#120830=CARTESIAN_POINT('Ctrl Pts',(65.7640639410661,-33.1020240106885,
0.));
#120831=CARTESIAN_POINT('Ctrl Pts',(65.7468619628815,-33.081582555798,0.));
#120832=CARTESIAN_POINT('Ctrl Pts',(65.7296648492824,-33.0611850631582,
0.));
#120833=CARTESIAN_POINT('Ctrl Pts',(65.7124726966802,-33.0408315717873,
0.));
#120834=CARTESIAN_POINT('Ctrl Pts',(65.6952856019533,-33.0205221207873,
0.));
#120835=CARTESIAN_POINT('Ctrl Pts',(65.6781036625027,-33.0002567493574,
0.));
#120836=CARTESIAN_POINT('Ctrl Pts',(65.6609269761888,-32.980035496784,0.));
#120837=CARTESIAN_POINT('Ctrl Pts',(65.6437556412946,-32.9598584024313,
0.));
#120838=CARTESIAN_POINT('Ctrl Pts',(65.6265897564783,-32.9397255057274,
0.));
#120839=CARTESIAN_POINT('Ctrl Pts',(65.6094294207276,-32.9196368461463,
0.));
#120840=CARTESIAN_POINT('Ctrl Pts',(65.5922747333194,-32.8995924631898,
0.));
#120841=CARTESIAN_POINT('Ctrl Pts',(65.5751257938472,-32.879592396403,0.));
#120842=CARTESIAN_POINT('Ctrl Pts',(65.5579827022421,-32.8596366853832,
0.));
#120843=CARTESIAN_POINT('Ctrl Pts',(65.5408455587964,-32.8397253697866,
0.));
#120844=CARTESIAN_POINT('Ctrl Pts',(65.5237144641857,-32.8198584893316,
0.));
#120845=CARTESIAN_POINT('Ctrl Pts',(65.5065895194928,-32.8000360837975,
0.));
#120846=CARTESIAN_POINT('Ctrl Pts',(65.489470826206,-32.7802581930287,0.));
#120847=CARTESIAN_POINT('Ctrl Pts',(65.4723584862122,-32.7605248569378,
0.));
#120848=CARTESIAN_POINT('Ctrl Pts',(65.4552526017905,-32.7408361155037,
0.));
#120849=CARTESIAN_POINT('Ctrl Pts',(65.4381532756065,-32.7211920087684,
0.));
#120850=CARTESIAN_POINT('Ctrl Pts',(65.4210606107035,-32.7015925768265,
0.));
#120851=CARTESIAN_POINT('Ctrl Pts',(65.4039747105038,-32.6820378598267,
0.));
#120852=CARTESIAN_POINT('Ctrl Pts',(65.3868956788182,-32.6625278979811,
0.));
#120853=CARTESIAN_POINT('Ctrl Pts',(65.3698236198512,-32.6430627315674,
0.));
#120854=CARTESIAN_POINT('Ctrl Pts',(65.3527586382081,-32.6236424009301,
0.));
#120855=CARTESIAN_POINT('Ctrl Pts',(65.3357008389003,-32.6042669464751,
0.));
#120856=CARTESIAN_POINT('Ctrl Pts',(65.31865032735,-32.5849364086679,0.));
#120857=CARTESIAN_POINT('Ctrl Pts',(65.3016072093912,-32.5656508280422,
0.));
#120858=CARTESIAN_POINT('Ctrl Pts',(65.2845715912721,-32.5464102452015,
0.));
#120859=CARTESIAN_POINT('Ctrl Pts',(65.2675435796558,-32.5272147008191,
0.));
#120860=CARTESIAN_POINT('Ctrl Pts',(65.2505232816209,-32.5080642356328,
0.));
#120861=CARTESIAN_POINT('Ctrl Pts',(65.2335108046614,-32.4889588904392,
0.));
#120862=CARTESIAN_POINT('Ctrl Pts',(65.2165062566924,-32.4698987061032,
0.));
#120863=CARTESIAN_POINT('Ctrl Pts',(65.1995097460538,-32.450883723561,0.));
#120864=CARTESIAN_POINT('Ctrl Pts',(65.182521381514,-32.4319139838213,0.));
#120865=CARTESIAN_POINT('Ctrl Pts',(65.1655412722725,-32.4129895279615,
0.));
#120866=CARTESIAN_POINT('Ctrl Pts',(65.1485695279635,-32.3941103971221,
0.));
#120867=CARTESIAN_POINT('Ctrl Pts',(65.1316062586588,-32.3752766325136,
0.));
#120868=CARTESIAN_POINT('Ctrl Pts',(65.1146515748722,-32.3564882754212,
0.));
#120869=CARTESIAN_POINT('Ctrl Pts',(65.0977055875607,-32.3377453672051,
0.));
#120870=CARTESIAN_POINT('Ctrl Pts',(65.0807684081281,-32.3190479492987,
0.));
#120871=CARTESIAN_POINT('Ctrl Pts',(65.0638401484257,-32.3003960632007,
0.));
#120872=CARTESIAN_POINT('Ctrl Pts',(65.0469209207563,-32.2817897504807,
0.));
#120873=CARTESIAN_POINT('Ctrl Pts',(65.03001083788,-32.2632290527862,0.));
#120874=CARTESIAN_POINT('Ctrl Pts',(65.0131100130157,-32.2447140118422,
0.));
#120875=CARTESIAN_POINT('Ctrl Pts',(64.9962185598461,-32.2262446694513,
0.));
#120876=CARTESIAN_POINT('Ctrl Pts',(64.9793365925178,-32.207821067485,0.));
#120877=CARTESIAN_POINT('Ctrl Pts',(64.9624642256461,-32.1894432478881,
0.));
#120878=CARTESIAN_POINT('Ctrl Pts',(64.9456015743192,-32.1711112526855,
0.));
#120879=CARTESIAN_POINT('Ctrl Pts',(64.9287487541015,-32.1528251239831,
0.));
#120880=CARTESIAN_POINT('Ctrl Pts',(64.9119058810366,-32.1345849039674,
0.));
#120881=CARTESIAN_POINT('Ctrl Pts',(64.8950730716501,-32.1163906348984,
0.));
#120882=CARTESIAN_POINT('Ctrl Pts',(64.8782504429527,-32.0982423591113,
0.));
#120883=CARTESIAN_POINT('Ctrl Pts',(64.8614381124454,-32.0801401190244,
0.));
#120884=CARTESIAN_POINT('Ctrl Pts',(64.8446361981234,-32.0620839571409,
0.));
#120885=CARTESIAN_POINT('Ctrl Pts',(64.8278448184785,-32.0440739160477,
0.));
#120886=CARTESIAN_POINT('Ctrl Pts',(64.811064092502,-32.0261100384092,0.));
#120887=CARTESIAN_POINT('Ctrl Pts',(64.7942941396883,-32.0081923669678,
0.));
#120888=CARTESIAN_POINT('Ctrl Pts',(64.7775350800404,-31.9903209445522,
0.));
#120889=CARTESIAN_POINT('Ctrl Pts',(64.7607870340738,-31.9724958140791,
0.));
#120890=CARTESIAN_POINT('Ctrl Pts',(64.74405012282,-31.9547170185533,0.));
#120891=CARTESIAN_POINT('Ctrl Pts',(64.727324467829,-31.9369846010613,0.));
#120892=CARTESIAN_POINT('Ctrl Pts',(64.7106101911722,-31.9192986047702,
0.));
#120893=CARTESIAN_POINT('Ctrl Pts',(64.693907415449,-31.9016590729371,0.));
#120894=CARTESIAN_POINT('Ctrl Pts',(64.6772162637904,-31.8840660489106,
0.));
#120895=CARTESIAN_POINT('Ctrl Pts',(64.6605368598631,-31.8665195761312,
0.));
#120896=CARTESIAN_POINT('Ctrl Pts',(64.6438693278718,-31.849019698125,0.));
#120897=CARTESIAN_POINT('Ctrl Pts',(64.6272137925629,-31.8315664585027,
0.));
#120898=CARTESIAN_POINT('Ctrl Pts',(64.6105703792311,-31.8141599009685,
0.));
#120899=CARTESIAN_POINT('Ctrl Pts',(64.5939392137233,-31.7968000693218,
0.));
#120900=CARTESIAN_POINT('Ctrl Pts',(64.5773204224429,-31.7794870074584,
0.));
#120901=CARTESIAN_POINT('Ctrl Pts',(64.5607141323527,-31.7622207593637,
0.));
#120902=CARTESIAN_POINT('Ctrl Pts',(64.5441204709779,-31.7450013691117,
0.));
#120903=CARTESIAN_POINT('Ctrl Pts',(64.5275395664134,-31.7278288808736,
0.));
#120904=CARTESIAN_POINT('Ctrl Pts',(64.5109715473276,-31.7107033389204,
0.));
#120905=CARTESIAN_POINT('Ctrl Pts',(64.4944165429672,-31.6936247876228,
0.));
#120906=CARTESIAN_POINT('Ctrl Pts',(64.4778746831597,-31.6765932714456,
0.));
#120907=CARTESIAN_POINT('Ctrl Pts',(64.4613460983186,-31.6596088349468,
0.));
#120908=CARTESIAN_POINT('Ctrl Pts',(64.4448309194498,-31.6426715227865,
0.));
#120909=CARTESIAN_POINT('Ctrl Pts',(64.4283292781553,-31.6257813797282,
0.));
#120910=CARTESIAN_POINT('Ctrl Pts',(64.4118413066386,-31.6089384506399,
0.));
#120911=CARTESIAN_POINT('Ctrl Pts',(64.3953671377071,-31.5921427804879,
0.));
#120912=CARTESIAN_POINT('Ctrl Pts',(64.3789069047768,-31.5753944143355,
0.));
#120913=CARTESIAN_POINT('Ctrl Pts',(64.3624607418798,-31.5586933973532,
0.));
#120914=CARTESIAN_POINT('Ctrl Pts',(64.34602878367,-31.5420397748198,0.));
#120915=CARTESIAN_POINT('Ctrl Pts',(64.3296111654273,-31.525433592124,0.));
#120916=CARTESIAN_POINT('Ctrl Pts',(64.3132080230603,-31.5088748947565,
0.));
#120917=CARTESIAN_POINT('Ctrl Pts',(64.2968194931113,-31.4923637283109,
0.));
#120918=CARTESIAN_POINT('Ctrl Pts',(64.2804457127633,-31.4759001384923,
0.));
#120919=CARTESIAN_POINT('Ctrl Pts',(64.264086819846,-31.4594841711189,0.));
#120920=CARTESIAN_POINT('Ctrl Pts',(64.2477429528408,-31.443115872123,0.));
#120921=CARTESIAN_POINT('Ctrl Pts',(64.2314142508843,-31.426795287544,0.));
#120922=CARTESIAN_POINT('Ctrl Pts',(64.2151008537733,-31.4105224635298,
0.));
#120923=CARTESIAN_POINT('Ctrl Pts',(64.1988029019733,-31.3942974463458,
0.));
#120924=CARTESIAN_POINT('Ctrl Pts',(64.1825205366231,-31.3781202823758,
0.));
#120925=CARTESIAN_POINT('Ctrl Pts',(64.1662538995407,-31.3619910181223,
0.));
#120926=CARTESIAN_POINT('Ctrl Pts',(64.150003133226,-31.3459097001996,0.));
#120927=CARTESIAN_POINT('Ctrl Pts',(64.1337683808667,-31.3298763753366,
0.));
#120928=CARTESIAN_POINT('Ctrl Pts',(64.1175497863475,-31.3138910903852,
0.));
#120929=CARTESIAN_POINT('Ctrl Pts',(64.1013474942554,-31.2979538923214,
0.));
#120930=CARTESIAN_POINT('Ctrl Pts',(64.0851616498861,-31.2820648282451,
0.));
#120931=CARTESIAN_POINT('Ctrl Pts',(64.0689923992474,-31.2662239453734,
0.));
#120932=CARTESIAN_POINT('Ctrl Pts',(64.0528398890671,-31.2504312910457,
0.));
#120933=CARTESIAN_POINT('Ctrl Pts',(64.036704266799,-31.23468691273,0.));
#120934=CARTESIAN_POINT('Ctrl Pts',(64.0205856806298,-31.2189908580245,
0.));
#120935=CARTESIAN_POINT('Ctrl Pts',(64.004484279483,-31.2033431746559,0.));
#120936=CARTESIAN_POINT('Ctrl Pts',(63.9884002130209,-31.1877439104717,
0.));
#120937=CARTESIAN_POINT('Ctrl Pts',(63.972333631655,-31.1721931134488,0.));
#120938=CARTESIAN_POINT('Ctrl Pts',(63.9562846865566,-31.1566908316993,
0.));
#120939=CARTESIAN_POINT('Ctrl Pts',(63.940253529665,-31.1412371134727,0.));
#120940=CARTESIAN_POINT('Ctrl Pts',(63.9242403136954,-31.1258320071545,
0.));
#120941=CARTESIAN_POINT('Ctrl Pts',(63.9082451921447,-31.1104755612606,
0.));
#120942=CARTESIAN_POINT('Ctrl Pts',(63.8922683192962,-31.0951678244454,
0.));
#120943=CARTESIAN_POINT('Ctrl Pts',(63.8763098502235,-31.079908845504,0.));
#120944=CARTESIAN_POINT('Ctrl Pts',(63.8603699407922,-31.0646986733724,
0.));
#120945=CARTESIAN_POINT('Ctrl Pts',(63.8444487476615,-31.0495373571218,
0.));
#120946=CARTESIAN_POINT('Ctrl Pts',(63.8285464282857,-31.0344249459544,
0.));
#120947=CARTESIAN_POINT('Ctrl Pts',(63.8126631409376,-31.0193614892177,
0.));
#120948=CARTESIAN_POINT('Ctrl Pts',(63.7967990447287,-31.0043470364112,
0.));
#120949=CARTESIAN_POINT('Ctrl Pts',(63.7809542996258,-30.9893816371907,
0.));
#120950=CARTESIAN_POINT('Ctrl Pts',(63.7651290664713,-30.9744653413679,
0.));
#120951=CARTESIAN_POINT('Ctrl Pts',(63.7493235069844,-30.9595981989091,
0.));
#120952=CARTESIAN_POINT('Ctrl Pts',(63.733537783742,-30.9447802599345,0.));
#120953=CARTESIAN_POINT('Ctrl Pts',(63.7177720601604,-30.9300115747113,
0.));
#120954=CARTESIAN_POINT('Ctrl Pts',(63.7020265004805,-30.9152921936471,
0.));
#120955=CARTESIAN_POINT('Ctrl Pts',(63.6863012697353,-30.9006221672703,
0.));
#120956=CARTESIAN_POINT('Ctrl Pts',(63.6705965337996,-30.8860015462488,
0.));
#120957=CARTESIAN_POINT('Ctrl Pts',(63.6549124594681,-30.8714303814202,
0.));
#120958=CARTESIAN_POINT('Ctrl Pts',(63.6392492145233,-30.8569087238132,
0.));
#120959=CARTESIAN_POINT('Ctrl Pts',(63.6236069678041,-30.8424366246665,
0.));
#120960=CARTESIAN_POINT('Ctrl Pts',(63.6079858892746,-30.8280141354448,
0.));
#120961=CARTESIAN_POINT('Ctrl Pts',(63.5923861498963,-30.8136413077999,
0.));
#120962=CARTESIAN_POINT('Ctrl Pts',(63.5768079214868,-30.7993181935265,
0.));
#120963=CARTESIAN_POINT('Ctrl Pts',(63.5612513766005,-30.7850448445207,
0.));
#120964=CARTESIAN_POINT('Ctrl Pts',(63.5457166883558,-30.7708213127169,
0.));
#120965=CARTESIAN_POINT('Ctrl Pts',(63.5302040304173,-30.7566476500772,
0.));
#120966=CARTESIAN_POINT('Ctrl Pts',(63.514713577392,-30.7425239087294,0.));
#120967=CARTESIAN_POINT('Ctrl Pts',(63.4992455051805,-30.7284501410827,
0.));
#120968=CARTESIAN_POINT('Ctrl Pts',(63.4837999912758,-30.7144263999259,
0.));
#120969=CARTESIAN_POINT('Ctrl Pts',(63.4683772152497,-30.7004527385806,
0.));
#120970=CARTESIAN_POINT('Ctrl Pts',(63.452977358421,-30.6865292107911,0.));
#120971=CARTESIAN_POINT('Ctrl Pts',(63.4376006029575,-30.6726558704302,
0.));
#120972=CARTESIAN_POINT('Ctrl Pts',(63.4222471311236,-30.6588327712482,
0.));
#120973=CARTESIAN_POINT('Ctrl Pts',(63.4069171245093,-30.6450599666135,
0.));
#120974=CARTESIAN_POINT('Ctrl Pts',(63.3916107631421,-30.6313375092085,
0.));
#120975=CARTESIAN_POINT('Ctrl Pts',(63.3763282271838,-30.6176654515988,
0.));
#120976=CARTESIAN_POINT('Ctrl Pts',(63.3610696989599,-30.604043846909,0.));
#120977=CARTESIAN_POINT('Ctrl Pts',(63.3458353646144,-30.5904727493707,
0.));
#120978=CARTESIAN_POINT('Ctrl Pts',(63.330625416509,-30.5769522151147,0.));
#120979=CARTESIAN_POINT('Ctrl Pts',(63.315440053435,-30.5634823022358,0.));
#120980=CARTESIAN_POINT('Ctrl Pts',(63.3002794756049,-30.5500630691343,
0.));
#120981=CARTESIAN_POINT('Ctrl Pts',(63.2851438802462,-30.5366945730503,
0.));
#120982=CARTESIAN_POINT('Ctrl Pts',(63.2700334577661,-30.5233768687875,
0.));
#120983=CARTESIAN_POINT('Ctrl Pts',(63.2549483856268,-30.5101100066683,
0.));
#120984=CARTESIAN_POINT('Ctrl Pts',(63.2398888342612,-30.4968940345028,
0.));
#120985=CARTESIAN_POINT('Ctrl Pts',(63.2248549788272,-30.4837290015011,
0.));
#120986=CARTESIAN_POINT('Ctrl Pts',(63.2098470086636,-30.470614961416,0.));
#120987=CARTESIAN_POINT('Ctrl Pts',(63.1948651386868,-30.4575519763305,
0.));
#120988=CARTESIAN_POINT('Ctrl Pts',(63.1799096171757,-30.4445401192324,
0.));
#120989=CARTESIAN_POINT('Ctrl Pts',(63.1649807016766,-30.431579465967,0.));
#120990=CARTESIAN_POINT('Ctrl Pts',(63.1500786361382,-30.4186700875598,
0.));
#120991=CARTESIAN_POINT('Ctrl Pts',(63.1352036298512,-30.4058120432259,
0.));
#120992=CARTESIAN_POINT('Ctrl Pts',(63.1203558300911,-30.3930053710592,
0.));
#120993=CARTESIAN_POINT('Ctrl Pts',(63.1055353202641,-30.3802500880565,
0.));
#120994=CARTESIAN_POINT('Ctrl Pts',(63.0937007763826,-30.3700869762658,
0.));
#120995=CARTESIAN_POINT('Ctrl Pts',(63.0848371718274,-30.3624877680747,
0.));
#120996=CARTESIAN_POINT('Ctrl Pts',(63.0789335700774,-30.3574319069366,
0.));
#120997=CARTESIAN_POINT('Ctrl Pts',(63.0759831361898,-30.3549065457811,
0.));
#120998=CARTESIAN_POINT('Ctrl Pts',(63.1661434108059,-39.5004851439258,
0.));
#120999=CARTESIAN_POINT('Ctrl Pts',(63.1661434108059,-39.5004851439258,
12.));
#121000=CARTESIAN_POINT('Ctrl Pts',(63.1630766582787,-39.4958045828135,
0.));
#121001=CARTESIAN_POINT('Ctrl Pts',(63.1630766582787,-39.4958045828135,
12.));
#121002=CARTESIAN_POINT('Ctrl Pts',(63.1569429707875,-39.4864477303823,
0.));
#121003=CARTESIAN_POINT('Ctrl Pts',(63.1569429707875,-39.4864477303823,
12.));
#121004=CARTESIAN_POINT('Ctrl Pts',(63.1477418922405,-39.4724252611155,
0.));
#121005=CARTESIAN_POINT('Ctrl Pts',(63.1477418922405,-39.4724252611155,
12.));
#121006=CARTESIAN_POINT('Ctrl Pts',(63.1354726928398,-39.4537542552269,
0.));
#121007=CARTESIAN_POINT('Ctrl Pts',(63.1354726928398,-39.4537542552269,
12.));
#121008=CARTESIAN_POINT('Ctrl Pts',(63.1201343731172,-39.4304582059864,
0.));
#121009=CARTESIAN_POINT('Ctrl Pts',(63.1201343731172,-39.4304582059864,
12.));
#121010=CARTESIAN_POINT('Ctrl Pts',(63.10479424519,-39.4072048797616,0.));
#121011=CARTESIAN_POINT('Ctrl Pts',(63.10479424519,-39.4072048797616,12.));
#121012=CARTESIAN_POINT('Ctrl Pts',(63.0894523341314,-39.383994298574,0.));
#121013=CARTESIAN_POINT('Ctrl Pts',(63.0894523341314,-39.383994298574,12.));
#121014=CARTESIAN_POINT('Ctrl Pts',(63.0741086815841,-39.3608264920409,
0.));
#121015=CARTESIAN_POINT('Ctrl Pts',(63.0741086815841,-39.3608264920409,
12.));
#121016=CARTESIAN_POINT('Ctrl Pts',(63.0587633513774,-39.3377014983609,
0.));
#121017=CARTESIAN_POINT('Ctrl Pts',(63.0587633513774,-39.3377014983609,
12.));
#121018=CARTESIAN_POINT('Ctrl Pts',(63.0434164277992,-39.3146193632392,
0.));
#121019=CARTESIAN_POINT('Ctrl Pts',(63.0434164277992,-39.3146193632392,
12.));
#121020=CARTESIAN_POINT('Ctrl Pts',(63.0280680082352,-39.2915801372354,
0.));
#121021=CARTESIAN_POINT('Ctrl Pts',(63.0280680082352,-39.2915801372354,
12.));
#121022=CARTESIAN_POINT('Ctrl Pts',(63.0127181973628,-39.2685838735361,
0.));
#121023=CARTESIAN_POINT('Ctrl Pts',(63.0127181973628,-39.2685838735361,
12.));
#121024=CARTESIAN_POINT('Ctrl Pts',(62.9973671008703,-39.2456306256104,
0.));
#121025=CARTESIAN_POINT('Ctrl Pts',(62.9973671008703,-39.2456306256104,
12.));
#121026=CARTESIAN_POINT('Ctrl Pts',(62.9820148189929,-39.2227204447638,
0.));
#121027=CARTESIAN_POINT('Ctrl Pts',(62.9820148189929,-39.2227204447638,
12.));
#121028=CARTESIAN_POINT('Ctrl Pts',(62.9666614412731,-39.1998533781661,
0.));
#121029=CARTESIAN_POINT('Ctrl Pts',(62.9666614412731,-39.1998533781661,
12.));
#121030=CARTESIAN_POINT('Ctrl Pts',(62.9513070501867,-39.1770294702428,
0.));
#121031=CARTESIAN_POINT('Ctrl Pts',(62.9513070501867,-39.1770294702428,
12.));
#121032=CARTESIAN_POINT('Ctrl Pts',(62.9359517237404,-39.1542487636744,
0.));
#121033=CARTESIAN_POINT('Ctrl Pts',(62.9359517237404,-39.1542487636744,
12.));
#121034=CARTESIAN_POINT('Ctrl Pts',(62.9205955385558,-39.131511300575,0.));
#121035=CARTESIAN_POINT('Ctrl Pts',(62.9205955385558,-39.131511300575,12.));
#121036=CARTESIAN_POINT('Ctrl Pts',(62.9052385725387,-39.1088171235125,
0.));
#121037=CARTESIAN_POINT('Ctrl Pts',(62.9052385725387,-39.1088171235125,
12.));
#121038=CARTESIAN_POINT('Ctrl Pts',(62.8898809082611,-39.0861662767932,
0.));
#121039=CARTESIAN_POINT('Ctrl Pts',(62.8898809082611,-39.0861662767932,
12.));
#121040=CARTESIAN_POINT('Ctrl Pts',(62.8745226325998,-39.0635588063277,
0.));
#121041=CARTESIAN_POINT('Ctrl Pts',(62.8745226325998,-39.0635588063277,
12.));
#121042=CARTESIAN_POINT('Ctrl Pts',(62.8591638352055,-39.0409947590497,
0.));
#121043=CARTESIAN_POINT('Ctrl Pts',(62.8591638352055,-39.0409947590497,
12.));
#121044=CARTESIAN_POINT('Ctrl Pts',(62.8438046073224,-39.0184741824641,
0.));
#121045=CARTESIAN_POINT('Ctrl Pts',(62.8438046073224,-39.0184741824641,
12.));
#121046=CARTESIAN_POINT('Ctrl Pts',(62.8284450405459,-38.9959971241701,
0.));
#121047=CARTESIAN_POINT('Ctrl Pts',(62.8284450405459,-38.9959971241701,
12.));
#121048=CARTESIAN_POINT('Ctrl Pts',(62.8130852254027,-38.9735636313089,
0.));
#121049=CARTESIAN_POINT('Ctrl Pts',(62.8130852254027,-38.9735636313089,
12.));
#121050=CARTESIAN_POINT('Ctrl Pts',(62.7977252507117,-38.9511737503165,
0.));
#121051=CARTESIAN_POINT('Ctrl Pts',(62.7977252507117,-38.9511737503165,
12.));
#121052=CARTESIAN_POINT('Ctrl Pts',(62.78236520437,-38.9288275272335,0.));
#121053=CARTESIAN_POINT('Ctrl Pts',(62.78236520437,-38.9288275272335,12.));
#121054=CARTESIAN_POINT('Ctrl Pts',(62.7670051738143,-38.9065250078832,
0.));
#121055=CARTESIAN_POINT('Ctrl Pts',(62.7670051738143,-38.9065250078832,
12.));
#121056=CARTESIAN_POINT('Ctrl Pts',(62.7516452466128,-38.8842662380984,
0.));
#121057=CARTESIAN_POINT('Ctrl Pts',(62.7516452466128,-38.8842662380984,
12.));
#121058=CARTESIAN_POINT('Ctrl Pts',(62.7362855110042,-38.8620512639233,
0.));
#121059=CARTESIAN_POINT('Ctrl Pts',(62.7362855110042,-38.8620512639233,
12.));
#121060=CARTESIAN_POINT('Ctrl Pts',(62.7209260564493,-38.8398801318177,
0.));
#121061=CARTESIAN_POINT('Ctrl Pts',(62.7209260564493,-38.8398801318177,
12.));
#121062=CARTESIAN_POINT('Ctrl Pts',(62.7055669733802,-38.8177528885681,
0.));
#121063=CARTESIAN_POINT('Ctrl Pts',(62.7055669733802,-38.8177528885681,
12.));
#121064=CARTESIAN_POINT('Ctrl Pts',(62.6902083529694,-38.795669581203,0.));
#121065=CARTESIAN_POINT('Ctrl Pts',(62.6902083529694,-38.795669581203,12.));
#121066=CARTESIAN_POINT('Ctrl Pts',(62.6748502868835,-38.7736302568982,
0.));
#121067=CARTESIAN_POINT('Ctrl Pts',(62.6748502868835,-38.7736302568982,
12.));
#121068=CARTESIAN_POINT('Ctrl Pts',(62.6594928670628,-38.7516349628904,
0.));
#121069=CARTESIAN_POINT('Ctrl Pts',(62.6594928670628,-38.7516349628904,
12.));
#121070=CARTESIAN_POINT('Ctrl Pts',(62.6441361854411,-38.7296837463609,
0.));
#121071=CARTESIAN_POINT('Ctrl Pts',(62.6441361854411,-38.7296837463609,
12.));
#121072=CARTESIAN_POINT('Ctrl Pts',(62.6287803339542,-38.7077766544416,
0.));
#121073=CARTESIAN_POINT('Ctrl Pts',(62.6287803339542,-38.7077766544416,
12.));
#121074=CARTESIAN_POINT('Ctrl Pts',(62.6134254046739,-38.6859137342731,
0.));
#121075=CARTESIAN_POINT('Ctrl Pts',(62.6134254046739,-38.6859137342731,
12.));
#121076=CARTESIAN_POINT('Ctrl Pts',(62.5980714899052,-38.6640950330421,
0.));
#121077=CARTESIAN_POINT('Ctrl Pts',(62.5980714899052,-38.6640950330421,
12.));
#121078=CARTESIAN_POINT('Ctrl Pts',(62.582718682292,-38.6423205980213,0.));
#121079=CARTESIAN_POINT('Ctrl Pts',(62.582718682292,-38.6423205980213,12.));
#121080=CARTESIAN_POINT('Ctrl Pts',(62.5673670749361,-38.6205904766073,
0.));
#121081=CARTESIAN_POINT('Ctrl Pts',(62.5673670749361,-38.6205904766073,
12.));
#121082=CARTESIAN_POINT('Ctrl Pts',(62.5520167614516,-38.5989047163393,
0.));
#121083=CARTESIAN_POINT('Ctrl Pts',(62.5520167614516,-38.5989047163393,
12.));
#121084=CARTESIAN_POINT('Ctrl Pts',(62.5366678359023,-38.5772633648833,
0.));
#121085=CARTESIAN_POINT('Ctrl Pts',(62.5366678359023,-38.5772633648833,
12.));
#121086=CARTESIAN_POINT('Ctrl Pts',(62.5213203927663,-38.5556664700195,
0.));
#121087=CARTESIAN_POINT('Ctrl Pts',(62.5213203927663,-38.5556664700195,
12.));
#121088=CARTESIAN_POINT('Ctrl Pts',(62.5059745268901,-38.5341140796248,
0.));
#121089=CARTESIAN_POINT('Ctrl Pts',(62.5059745268901,-38.5341140796248,
12.));
#121090=CARTESIAN_POINT('Ctrl Pts',(62.4906303334443,-38.5126062416502,
0.));
#121091=CARTESIAN_POINT('Ctrl Pts',(62.4906303334443,-38.5126062416502,
12.));
#121092=CARTESIAN_POINT('Ctrl Pts',(62.4752879078854,-38.4911430040997,
0.));
#121093=CARTESIAN_POINT('Ctrl Pts',(62.4752879078854,-38.4911430040997,
12.));
#121094=CARTESIAN_POINT('Ctrl Pts',(62.4599473459811,-38.4697244150482,
0.));
#121095=CARTESIAN_POINT('Ctrl Pts',(62.4599473459811,-38.4697244150482,
12.));
#121096=CARTESIAN_POINT('Ctrl Pts',(62.4446087438312,-38.4483505226518,
0.));
#121097=CARTESIAN_POINT('Ctrl Pts',(62.4446087438312,-38.4483505226518,
12.));
#121098=CARTESIAN_POINT('Ctrl Pts',(62.4292721978901,-38.4270213751568,
0.));
#121099=CARTESIAN_POINT('Ctrl Pts',(62.4292721978901,-38.4270213751568,
12.));
#121100=CARTESIAN_POINT('Ctrl Pts',(62.4139378049885,-38.405737020905,0.));
#121101=CARTESIAN_POINT('Ctrl Pts',(62.4139378049885,-38.405737020905,12.));
#121102=CARTESIAN_POINT('Ctrl Pts',(62.3986056623577,-38.3844975083344,
0.));
#121103=CARTESIAN_POINT('Ctrl Pts',(62.3986056623577,-38.3844975083344,
12.));
#121104=CARTESIAN_POINT('Ctrl Pts',(62.3832758676271,-38.3633028859828,
0.));
#121105=CARTESIAN_POINT('Ctrl Pts',(62.3832758676271,-38.3633028859828,
12.));
#121106=CARTESIAN_POINT('Ctrl Pts',(62.3679485188171,-38.342153202491,0.));
#121107=CARTESIAN_POINT('Ctrl Pts',(62.3679485188171,-38.342153202491,12.));
#121108=CARTESIAN_POINT('Ctrl Pts',(62.3526237143336,-38.3210485066001,
0.));
#121109=CARTESIAN_POINT('Ctrl Pts',(62.3526237143336,-38.3210485066001,
12.));
#121110=CARTESIAN_POINT('Ctrl Pts',(62.3373015529613,-38.2999888471476,
0.));
#121111=CARTESIAN_POINT('Ctrl Pts',(62.3373015529613,-38.2999888471476,
12.));
#121112=CARTESIAN_POINT('Ctrl Pts',(62.3219821338569,-38.2789742730564,
0.));
#121113=CARTESIAN_POINT('Ctrl Pts',(62.3219821338569,-38.2789742730564,
12.));
#121114=CARTESIAN_POINT('Ctrl Pts',(62.3066655565503,-38.2580048333361,
0.));
#121115=CARTESIAN_POINT('Ctrl Pts',(62.3066655565503,-38.2580048333361,
12.));
#121116=CARTESIAN_POINT('Ctrl Pts',(62.2913519209521,-38.2370805770935,
0.));
#121117=CARTESIAN_POINT('Ctrl Pts',(62.2913519209521,-38.2370805770935,
12.));
#121118=CARTESIAN_POINT('Ctrl Pts',(62.2760413273602,-38.2162015535353,
0.));
#121119=CARTESIAN_POINT('Ctrl Pts',(62.2760413273602,-38.2162015535353,
12.));
#121120=CARTESIAN_POINT('Ctrl Pts',(62.2607338764654,-38.1953678119691,
0.));
#121121=CARTESIAN_POINT('Ctrl Pts',(62.2607338764654,-38.1953678119691,
12.));
#121122=CARTESIAN_POINT('Ctrl Pts',(62.245429669358,-38.1745794017996,0.));
#121123=CARTESIAN_POINT('Ctrl Pts',(62.245429669358,-38.1745794017996,12.));
#121124=CARTESIAN_POINT('Ctrl Pts',(62.2301288075321,-38.1538363725264,
0.));
#121125=CARTESIAN_POINT('Ctrl Pts',(62.2301288075321,-38.1538363725264,
12.));
#121126=CARTESIAN_POINT('Ctrl Pts',(62.2148313928863,-38.133138773753,0.));
#121127=CARTESIAN_POINT('Ctrl Pts',(62.2148313928863,-38.133138773753,12.));
#121128=CARTESIAN_POINT('Ctrl Pts',(62.1995375277257,-38.1124866551886,
0.));
#121129=CARTESIAN_POINT('Ctrl Pts',(62.1995375277257,-38.1124866551886,
12.));
#121130=CARTESIAN_POINT('Ctrl Pts',(62.1842473147626,-38.0918800666479,
0.));
#121131=CARTESIAN_POINT('Ctrl Pts',(62.1842473147626,-38.0918800666479,
12.));
#121132=CARTESIAN_POINT('Ctrl Pts',(62.1689608571176,-38.0713190580463,
0.));
#121133=CARTESIAN_POINT('Ctrl Pts',(62.1689608571176,-38.0713190580463,
12.));
#121134=CARTESIAN_POINT('Ctrl Pts',(62.1536782583199,-38.0508036793939,
0.));
#121135=CARTESIAN_POINT('Ctrl Pts',(62.1536782583199,-38.0508036793939,
12.));
#121136=CARTESIAN_POINT('Ctrl Pts',(62.1383996223124,-38.0303339808053,
0.));
#121137=CARTESIAN_POINT('Ctrl Pts',(62.1383996223124,-38.0303339808053,
12.));
#121138=CARTESIAN_POINT('Ctrl Pts',(62.123125053455,-38.0099100125037,0.));
#121139=CARTESIAN_POINT('Ctrl Pts',(62.123125053455,-38.0099100125037,12.));
#121140=CARTESIAN_POINT('Ctrl Pts',(62.107854656528,-37.9895318248212,0.));
#121141=CARTESIAN_POINT('Ctrl Pts',(62.107854656528,-37.9895318248212,12.));
#121142=CARTESIAN_POINT('Ctrl Pts',(62.0925885367352,-37.9691994681966,
0.));
#121143=CARTESIAN_POINT('Ctrl Pts',(62.0925885367352,-37.9691994681966,
12.));
#121144=CARTESIAN_POINT('Ctrl Pts',(62.0773267997078,-37.9489129931689,
0.));
#121145=CARTESIAN_POINT('Ctrl Pts',(62.0773267997078,-37.9489129931689,
12.));
#121146=CARTESIAN_POINT('Ctrl Pts',(62.0620695515074,-37.9286724503851,
0.));
#121147=CARTESIAN_POINT('Ctrl Pts',(62.0620695515074,-37.9286724503851,
12.));
#121148=CARTESIAN_POINT('Ctrl Pts',(62.0468168986288,-37.9084778906053,
0.));
#121149=CARTESIAN_POINT('Ctrl Pts',(62.0468168986288,-37.9084778906053,
12.));
#121150=CARTESIAN_POINT('Ctrl Pts',(62.031568948002,-37.8883293647029,0.));
#121151=CARTESIAN_POINT('Ctrl Pts',(62.031568948002,-37.8883293647029,12.));
#121152=CARTESIAN_POINT('Ctrl Pts',(62.0163258069957,-37.868226923663,0.));
#121153=CARTESIAN_POINT('Ctrl Pts',(62.0163258069957,-37.868226923663,12.));
#121154=CARTESIAN_POINT('Ctrl Pts',(62.0010875834187,-37.8481706185749,
0.));
#121155=CARTESIAN_POINT('Ctrl Pts',(62.0010875834187,-37.8481706185749,
12.));
#121156=CARTESIAN_POINT('Ctrl Pts',(61.9858543855236,-37.8281605006381,
0.));
#121157=CARTESIAN_POINT('Ctrl Pts',(61.9858543855236,-37.8281605006381,
12.));
#121158=CARTESIAN_POINT('Ctrl Pts',(61.9706263220114,-37.8081966211689,
0.));
#121159=CARTESIAN_POINT('Ctrl Pts',(61.9706263220114,-37.8081966211689,
12.));
#121160=CARTESIAN_POINT('Ctrl Pts',(61.9554035020338,-37.7882790316014,
0.));
#121161=CARTESIAN_POINT('Ctrl Pts',(61.9554035020338,-37.7882790316014,
12.));
#121162=CARTESIAN_POINT('Ctrl Pts',(61.9401860351972,-37.7684077834873,
0.));
#121163=CARTESIAN_POINT('Ctrl Pts',(61.9401860351972,-37.7684077834873,
12.));
#121164=CARTESIAN_POINT('Ctrl Pts',(61.9249740315649,-37.7485829284872,
0.));
#121165=CARTESIAN_POINT('Ctrl Pts',(61.9249740315649,-37.7485829284872,
12.));
#121166=CARTESIAN_POINT('Ctrl Pts',(61.9097676016601,-37.7288045183756,
0.));
#121167=CARTESIAN_POINT('Ctrl Pts',(61.9097676016601,-37.7288045183756,
12.));
#121168=CARTESIAN_POINT('Ctrl Pts',(61.8945668564704,-37.7090726050482,
0.));
#121169=CARTESIAN_POINT('Ctrl Pts',(61.8945668564704,-37.7090726050482,
12.));
#121170=CARTESIAN_POINT('Ctrl Pts',(61.8793719074507,-37.6893872405228,
0.));
#121171=CARTESIAN_POINT('Ctrl Pts',(61.8793719074507,-37.6893872405228,
12.));
#121172=CARTESIAN_POINT('Ctrl Pts',(61.8641828665261,-37.6697484769392,
0.));
#121173=CARTESIAN_POINT('Ctrl Pts',(61.8641828665261,-37.6697484769392,
12.));
#121174=CARTESIAN_POINT('Ctrl Pts',(61.8489998460957,-37.6501563665524,
0.));
#121175=CARTESIAN_POINT('Ctrl Pts',(61.8489998460957,-37.6501563665524,
12.));
#121176=CARTESIAN_POINT('Ctrl Pts',(61.8338229590352,-37.6306109617347,
0.));
#121177=CARTESIAN_POINT('Ctrl Pts',(61.8338229590352,-37.6306109617347,
12.));
#121178=CARTESIAN_POINT('Ctrl Pts',(61.8186523187015,-37.6111123149839,
0.));
#121179=CARTESIAN_POINT('Ctrl Pts',(61.8186523187015,-37.6111123149839,
12.));
#121180=CARTESIAN_POINT('Ctrl Pts',(61.8034880389362,-37.5916604789253,
0.));
#121181=CARTESIAN_POINT('Ctrl Pts',(61.8034880389362,-37.5916604789253,
12.));
#121182=CARTESIAN_POINT('Ctrl Pts',(61.7883302340687,-37.5722555063111,
0.));
#121183=CARTESIAN_POINT('Ctrl Pts',(61.7883302340687,-37.5722555063111,
12.));
#121184=CARTESIAN_POINT('Ctrl Pts',(61.773179018919,-37.5528974500142,0.));
#121185=CARTESIAN_POINT('Ctrl Pts',(61.773179018919,-37.5528974500142,12.));
#121186=CARTESIAN_POINT('Ctrl Pts',(61.7580345088016,-37.5335863630287,
0.));
#121187=CARTESIAN_POINT('Ctrl Pts',(61.7580345088016,-37.5335863630287,
12.));
#121188=CARTESIAN_POINT('Ctrl Pts',(61.7428968195299,-37.5143222984796,
0.));
#121189=CARTESIAN_POINT('Ctrl Pts',(61.7428968195299,-37.5143222984796,
12.));
#121190=CARTESIAN_POINT('Ctrl Pts',(61.7277660674205,-37.4951053096237,
0.));
#121191=CARTESIAN_POINT('Ctrl Pts',(61.7277660674205,-37.4951053096237,
12.));
#121192=CARTESIAN_POINT('Ctrl Pts',(61.7126423692963,-37.4759354498509,
0.));
#121193=CARTESIAN_POINT('Ctrl Pts',(61.7126423692963,-37.4759354498509,
12.));
#121194=CARTESIAN_POINT('Ctrl Pts',(61.6975258424894,-37.4568127726773,
0.));
#121195=CARTESIAN_POINT('Ctrl Pts',(61.6975258424894,-37.4568127726773,
12.));
#121196=CARTESIAN_POINT('Ctrl Pts',(61.6824166048444,-37.4377373317451,
0.));
#121197=CARTESIAN_POINT('Ctrl Pts',(61.6824166048444,-37.4377373317451,
12.));
#121198=CARTESIAN_POINT('Ctrl Pts',(61.6673147747242,-37.4187091808321,
0.));
#121199=CARTESIAN_POINT('Ctrl Pts',(61.6673147747242,-37.4187091808321,
12.));
#121200=CARTESIAN_POINT('Ctrl Pts',(61.6522204710131,-37.3997283738533,
0.));
#121201=CARTESIAN_POINT('Ctrl Pts',(61.6522204710131,-37.3997283738533,
12.));
#121202=CARTESIAN_POINT('Ctrl Pts',(61.637133813121,-37.3807949648624,0.));
#121203=CARTESIAN_POINT('Ctrl Pts',(61.637133813121,-37.3807949648624,12.));
#121204=CARTESIAN_POINT('Ctrl Pts',(61.6220549209866,-37.361909008045,0.));
#121205=CARTESIAN_POINT('Ctrl Pts',(61.6220549209866,-37.361909008045,12.));
#121206=CARTESIAN_POINT('Ctrl Pts',(61.6069839150807,-37.343070557718,0.));
#121207=CARTESIAN_POINT('Ctrl Pts',(61.6069839150807,-37.343070557718,12.));
#121208=CARTESIAN_POINT('Ctrl Pts',(61.591920916412,-37.3242796683395,0.));
#121209=CARTESIAN_POINT('Ctrl Pts',(61.591920916412,-37.3242796683395,12.));
#121210=CARTESIAN_POINT('Ctrl Pts',(61.5768660465311,-37.3055363945108,
0.));
#121211=CARTESIAN_POINT('Ctrl Pts',(61.5768660465311,-37.3055363945108,
12.));
#121212=CARTESIAN_POINT('Ctrl Pts',(61.5618194275348,-37.2868407909771,
0.));
#121213=CARTESIAN_POINT('Ctrl Pts',(61.5618194275348,-37.2868407909771,
12.));
#121214=CARTESIAN_POINT('Ctrl Pts',(61.5467811820691,-37.2681929126221,
0.));
#121215=CARTESIAN_POINT('Ctrl Pts',(61.5467811820691,-37.2681929126221,
12.));
#121216=CARTESIAN_POINT('Ctrl Pts',(61.5317514333328,-37.2495928144667,
0.));
#121217=CARTESIAN_POINT('Ctrl Pts',(61.5317514333328,-37.2495928144667,
12.));
#121218=CARTESIAN_POINT('Ctrl Pts',(61.5167303050832,-37.2310405516781,
0.));
#121219=CARTESIAN_POINT('Ctrl Pts',(61.5167303050832,-37.2310405516781,
12.));
#121220=CARTESIAN_POINT('Ctrl Pts',(61.501717921641,-37.2125361795731,0.));
#121221=CARTESIAN_POINT('Ctrl Pts',(61.501717921641,-37.2125361795731,12.));
#121222=CARTESIAN_POINT('Ctrl Pts',(61.4867144078936,-37.1940797536181,
0.));
#121223=CARTESIAN_POINT('Ctrl Pts',(61.4867144078936,-37.1940797536181,
12.));
#121224=CARTESIAN_POINT('Ctrl Pts',(61.4717198892994,-37.175671329424,0.));
#121225=CARTESIAN_POINT('Ctrl Pts',(61.4717198892994,-37.175671329424,12.));
#121226=CARTESIAN_POINT('Ctrl Pts',(61.4567344918919,-37.1573109627454,
0.));
#121227=CARTESIAN_POINT('Ctrl Pts',(61.4567344918919,-37.1573109627454,
12.));
#121228=CARTESIAN_POINT('Ctrl Pts',(61.4417583422863,-37.1389987094905,
0.));
#121229=CARTESIAN_POINT('Ctrl Pts',(61.4417583422863,-37.1389987094905,
12.));
#121230=CARTESIAN_POINT('Ctrl Pts',(61.4267915676822,-37.1207346257222,
0.));
#121231=CARTESIAN_POINT('Ctrl Pts',(61.4267915676822,-37.1207346257222,
12.));
#121232=CARTESIAN_POINT('Ctrl Pts',(61.4118342958697,-37.1025187676602,
0.));
#121233=CARTESIAN_POINT('Ctrl Pts',(61.4118342958697,-37.1025187676602,
12.));
#121234=CARTESIAN_POINT('Ctrl Pts',(61.3968866552317,-37.0843511916745,
0.));
#121235=CARTESIAN_POINT('Ctrl Pts',(61.3968866552317,-37.0843511916745,
12.));
#121236=CARTESIAN_POINT('Ctrl Pts',(61.381948774749,-37.0662319542849,0.));
#121237=CARTESIAN_POINT('Ctrl Pts',(61.381948774749,-37.0662319542849,12.));
#121238=CARTESIAN_POINT('Ctrl Pts',(61.3670207840068,-37.0481611121717,
0.));
#121239=CARTESIAN_POINT('Ctrl Pts',(61.3670207840068,-37.0481611121717,
12.));
#121240=CARTESIAN_POINT('Ctrl Pts',(61.3521028132003,-37.0301387221774,
0.));
#121241=CARTESIAN_POINT('Ctrl Pts',(61.3521028132003,-37.0301387221774,
12.));
#121242=CARTESIAN_POINT('Ctrl Pts',(61.3371949931387,-37.0121648413082,
0.));
#121243=CARTESIAN_POINT('Ctrl Pts',(61.3371949931387,-37.0121648413082,
12.));
#121244=CARTESIAN_POINT('Ctrl Pts',(61.3222974552486,-36.994239526727,0.));
#121245=CARTESIAN_POINT('Ctrl Pts',(61.3222974552486,-36.994239526727,12.));
#121246=CARTESIAN_POINT('Ctrl Pts',(61.3074103315791,-36.9763628357544,
0.));
#121247=CARTESIAN_POINT('Ctrl Pts',(61.3074103315791,-36.9763628357544,
12.));
#121248=CARTESIAN_POINT('Ctrl Pts',(61.2925337548077,-36.9585348258776,
0.));
#121249=CARTESIAN_POINT('Ctrl Pts',(61.2925337548077,-36.9585348258776,
12.));
#121250=CARTESIAN_POINT('Ctrl Pts',(61.2776678582461,-36.9407555547535,
0.));
#121251=CARTESIAN_POINT('Ctrl Pts',(61.2776678582461,-36.9407555547535,
12.));
#121252=CARTESIAN_POINT('Ctrl Pts',(61.2628127758457,-36.9230250802088,
0.));
#121253=CARTESIAN_POINT('Ctrl Pts',(61.2628127758457,-36.9230250802088,
12.));
#121254=CARTESIAN_POINT('Ctrl Pts',(61.247968642201,-36.9053434602343,0.));
#121255=CARTESIAN_POINT('Ctrl Pts',(61.247968642201,-36.9053434602343,12.));
#121256=CARTESIAN_POINT('Ctrl Pts',(61.2331355925547,-36.8877107529865,
0.));
#121257=CARTESIAN_POINT('Ctrl Pts',(61.2331355925547,-36.8877107529865,
12.));
#121258=CARTESIAN_POINT('Ctrl Pts',(61.2183137628056,-36.8701270167969,
0.));
#121259=CARTESIAN_POINT('Ctrl Pts',(61.2183137628056,-36.8701270167969,
12.));
#121260=CARTESIAN_POINT('Ctrl Pts',(61.2035032895127,-36.852592310174,0.));
#121261=CARTESIAN_POINT('Ctrl Pts',(61.2035032895127,-36.852592310174,12.));
#121262=CARTESIAN_POINT('Ctrl Pts',(61.1887043099014,-36.8351066918036,
0.));
#121263=CARTESIAN_POINT('Ctrl Pts',(61.1887043099014,-36.8351066918036,
12.));
#121264=CARTESIAN_POINT('Ctrl Pts',(61.1739169618666,-36.8176702205423,
0.));
#121265=CARTESIAN_POINT('Ctrl Pts',(61.1739169618666,-36.8176702205423,
12.));
#121266=CARTESIAN_POINT('Ctrl Pts',(61.1591413839787,-36.8002829554209,
0.));
#121267=CARTESIAN_POINT('Ctrl Pts',(61.1591413839787,-36.8002829554209,
12.));
#121268=CARTESIAN_POINT('Ctrl Pts',(61.1443777154911,-36.7829449556532,
0.));
#121269=CARTESIAN_POINT('Ctrl Pts',(61.1443777154911,-36.7829449556532,
12.));
#121270=CARTESIAN_POINT('Ctrl Pts',(61.1296260963466,-36.765656280638,0.));
#121271=CARTESIAN_POINT('Ctrl Pts',(61.1296260963466,-36.765656280638,12.));
#121272=CARTESIAN_POINT('Ctrl Pts',(61.1148866671829,-36.7484169899596,
0.));
#121273=CARTESIAN_POINT('Ctrl Pts',(61.1148866671829,-36.7484169899596,
12.));
#121274=CARTESIAN_POINT('Ctrl Pts',(61.100159569337,-36.7312271433807,0.));
#121275=CARTESIAN_POINT('Ctrl Pts',(61.100159569337,-36.7312271433807,12.));
#121276=CARTESIAN_POINT('Ctrl Pts',(61.0854449448524,-36.7140868008486,
0.));
#121277=CARTESIAN_POINT('Ctrl Pts',(61.0854449448524,-36.7140868008486,
12.));
#121278=CARTESIAN_POINT('Ctrl Pts',(61.0707429364847,-36.6969960225022,
0.));
#121279=CARTESIAN_POINT('Ctrl Pts',(61.0707429364847,-36.6969960225022,
12.));
#121280=CARTESIAN_POINT('Ctrl Pts',(61.0560536877083,-36.679954868674,0.));
#121281=CARTESIAN_POINT('Ctrl Pts',(61.0560536877083,-36.679954868674,12.));
#121282=CARTESIAN_POINT('Ctrl Pts',(61.0413773427203,-36.6629633998886,
0.));
#121283=CARTESIAN_POINT('Ctrl Pts',(61.0413773427203,-36.6629633998886,
12.));
#121284=CARTESIAN_POINT('Ctrl Pts',(61.0267140464432,-36.6460216768553,
0.));
#121285=CARTESIAN_POINT('Ctrl Pts',(61.0267140464432,-36.6460216768553,
12.));
#121286=CARTESIAN_POINT('Ctrl Pts',(61.0120639445349,-36.6291297604776,
0.));
#121287=CARTESIAN_POINT('Ctrl Pts',(61.0120639445349,-36.6291297604776,
12.));
#121288=CARTESIAN_POINT('Ctrl Pts',(60.9974271833981,-36.61228771186,0.));
#121289=CARTESIAN_POINT('Ctrl Pts',(60.9974271833981,-36.61228771186,12.));
#121290=CARTESIAN_POINT('Ctrl Pts',(60.9828039101887,-36.5954955923109,
0.));
#121291=CARTESIAN_POINT('Ctrl Pts',(60.9828039101887,-36.5954955923109,
12.));
#121292=CARTESIAN_POINT('Ctrl Pts',(60.9681942728236,-36.5787534633416,
0.));
#121293=CARTESIAN_POINT('Ctrl Pts',(60.9681942728236,-36.5787534633416,
12.));
#121294=CARTESIAN_POINT('Ctrl Pts',(60.9535984199873,-36.5620613866615,
0.));
#121295=CARTESIAN_POINT('Ctrl Pts',(60.9535984199873,-36.5620613866615,
12.));
#121296=CARTESIAN_POINT('Ctrl Pts',(60.9390165011355,-36.5454194241865,
0.));
#121297=CARTESIAN_POINT('Ctrl Pts',(60.9390165011355,-36.5454194241865,
12.));
#121298=CARTESIAN_POINT('Ctrl Pts',(60.9244486664987,-36.5288276380416,
0.));
#121299=CARTESIAN_POINT('Ctrl Pts',(60.9244486664987,-36.5288276380416,
12.));
#121300=CARTESIAN_POINT('Ctrl Pts',(60.9098950670847,-36.5122860905612,
0.));
#121301=CARTESIAN_POINT('Ctrl Pts',(60.9098950670847,-36.5122860905612,
12.));
#121302=CARTESIAN_POINT('Ctrl Pts',(60.8953558546795,-36.4957948442835,
0.));
#121303=CARTESIAN_POINT('Ctrl Pts',(60.8953558546795,-36.4957948442835,
12.));
#121304=CARTESIAN_POINT('Ctrl Pts',(60.8808311818499,-36.4793539619466,
0.));
#121305=CARTESIAN_POINT('Ctrl Pts',(60.8808311818499,-36.4793539619466,
12.));
#121306=CARTESIAN_POINT('Ctrl Pts',(60.8663212019657,-36.4629635065045,
0.));
#121307=CARTESIAN_POINT('Ctrl Pts',(60.8663212019657,-36.4629635065045,
12.));
#121308=CARTESIAN_POINT('Ctrl Pts',(60.8518260692188,-36.4466235411358,
0.));
#121309=CARTESIAN_POINT('Ctrl Pts',(60.8518260692188,-36.4466235411358,
12.));
#121310=CARTESIAN_POINT('Ctrl Pts',(60.8373459386392,-36.4303341292494,
0.));
#121311=CARTESIAN_POINT('Ctrl Pts',(60.8373459386392,-36.4303341292494,
12.));
#121312=CARTESIAN_POINT('Ctrl Pts',(60.822880966116,-36.4140953344859,0.));
#121313=CARTESIAN_POINT('Ctrl Pts',(60.822880966116,-36.4140953344859,12.));
#121314=CARTESIAN_POINT('Ctrl Pts',(60.8084313083984,-36.397907220716,0.));
#121315=CARTESIAN_POINT('Ctrl Pts',(60.8084313083984,-36.397907220716,12.));
#121316=CARTESIAN_POINT('Ctrl Pts',(60.793997123076,-36.3817698520388,0.));
#121317=CARTESIAN_POINT('Ctrl Pts',(60.793997123076,-36.3817698520388,12.));
#121318=CARTESIAN_POINT('Ctrl Pts',(60.7795785685625,-36.365683292773,0.));
#121319=CARTESIAN_POINT('Ctrl Pts',(60.7795785685625,-36.365683292773,12.));
#121320=CARTESIAN_POINT('Ctrl Pts',(60.7651758040803,-36.3496476074488,
0.));
#121321=CARTESIAN_POINT('Ctrl Pts',(60.7651758040803,-36.3496476074488,
12.));
#121322=CARTESIAN_POINT('Ctrl Pts',(60.7507889896308,-36.3336628607859,
0.));
#121323=CARTESIAN_POINT('Ctrl Pts',(60.7507889896308,-36.3336628607859,
12.));
#121324=CARTESIAN_POINT('Ctrl Pts',(60.7364182860412,-36.3177291177163,
0.));
#121325=CARTESIAN_POINT('Ctrl Pts',(60.7364182860412,-36.3177291177163,
12.));
#121326=CARTESIAN_POINT('Ctrl Pts',(60.722063855041,-36.3018464434214,0.));
#121327=CARTESIAN_POINT('Ctrl Pts',(60.722063855041,-36.3018464434214,12.));
#121328=CARTESIAN_POINT('Ctrl Pts',(60.7077258593268,-36.2860149033587,
0.));
#121329=CARTESIAN_POINT('Ctrl Pts',(60.7077258593268,-36.2860149033587,
12.));
#121330=CARTESIAN_POINT('Ctrl Pts',(60.6934044626291,-36.2702345632875,
0.));
#121331=CARTESIAN_POINT('Ctrl Pts',(60.6934044626291,-36.2702345632875,
12.));
#121332=CARTESIAN_POINT('Ctrl Pts',(60.67909982978,-36.2545054892897,0.));
#121333=CARTESIAN_POINT('Ctrl Pts',(60.67909982978,-36.2545054892897,12.));
#121334=CARTESIAN_POINT('Ctrl Pts',(60.6648121265885,-36.2388277477212,
0.));
#121335=CARTESIAN_POINT('Ctrl Pts',(60.6648121265885,-36.2388277477212,
12.));
#121336=CARTESIAN_POINT('Ctrl Pts',(60.6505415197042,-36.2232014051541,
0.));
#121337=CARTESIAN_POINT('Ctrl Pts',(60.6505415197042,-36.2232014051541,
12.));
#121338=CARTESIAN_POINT('Ctrl Pts',(60.6362881765019,-36.2076265283264,
0.));
#121339=CARTESIAN_POINT('Ctrl Pts',(60.6362881765019,-36.2076265283264,
12.));
#121340=CARTESIAN_POINT('Ctrl Pts',(60.6220522649149,-36.192103184063,0.));
#121341=CARTESIAN_POINT('Ctrl Pts',(60.6220522649149,-36.192103184063,12.));
#121342=CARTESIAN_POINT('Ctrl Pts',(60.6078339534181,-36.1766314392641,
0.));
#121343=CARTESIAN_POINT('Ctrl Pts',(60.6078339534181,-36.1766314392641,
12.));
#121344=CARTESIAN_POINT('Ctrl Pts',(60.5936334114108,-36.1612113610773,
0.));
#121345=CARTESIAN_POINT('Ctrl Pts',(60.5936334114108,-36.1612113610773,
12.));
#121346=CARTESIAN_POINT('Ctrl Pts',(60.5794508095564,-36.1458430170431,
0.));
#121347=CARTESIAN_POINT('Ctrl Pts',(60.5794508095564,-36.1458430170431,
12.));
#121348=CARTESIAN_POINT('Ctrl Pts',(60.565286320072,-36.1305264752188,0.));
#121349=CARTESIAN_POINT('Ctrl Pts',(60.565286320072,-36.1305264752188,12.));
#121350=CARTESIAN_POINT('Ctrl Pts',(60.5511401171984,-36.1152618043739,
0.));
#121351=CARTESIAN_POINT('Ctrl Pts',(60.5511401171984,-36.1152618043739,
12.));
#121352=CARTESIAN_POINT('Ctrl Pts',(60.5370123768804,-36.1000490738511,
0.));
#121353=CARTESIAN_POINT('Ctrl Pts',(60.5370123768804,-36.1000490738511,
12.));
#121354=CARTESIAN_POINT('Ctrl Pts',(60.5229032758973,-36.0848883531952,
0.));
#121355=CARTESIAN_POINT('Ctrl Pts',(60.5229032758973,-36.0848883531952,
12.));
#121356=CARTESIAN_POINT('Ctrl Pts',(60.5088129911354,-36.0697797118376,
0.));
#121357=CARTESIAN_POINT('Ctrl Pts',(60.5088129911354,-36.0697797118376,
12.));
#121358=CARTESIAN_POINT('Ctrl Pts',(60.4947416988422,-36.0547232187698,
0.));
#121359=CARTESIAN_POINT('Ctrl Pts',(60.4947416988422,-36.0547232187698,
12.));
#121360=CARTESIAN_POINT('Ctrl Pts',(60.4806895737686,-36.0397189421644,
0.));
#121361=CARTESIAN_POINT('Ctrl Pts',(60.4806895737686,-36.0397189421644,
12.));
#121362=CARTESIAN_POINT('Ctrl Pts',(60.4666567908093,-36.0247669500892,
0.));
#121363=CARTESIAN_POINT('Ctrl Pts',(60.4666567908093,-36.0247669500892,
12.));
#121364=CARTESIAN_POINT('Ctrl Pts',(60.4526435269662,-36.009867311357,0.));
#121365=CARTESIAN_POINT('Ctrl Pts',(60.4526435269662,-36.009867311357,12.));
#121366=CARTESIAN_POINT('Ctrl Pts',(60.4386499629481,-35.995020096217,0.));
#121367=CARTESIAN_POINT('Ctrl Pts',(60.4386499629481,-35.995020096217,12.));
#121368=CARTESIAN_POINT('Ctrl Pts',(60.4246762854926,-35.9802253773515,
0.));
#121369=CARTESIAN_POINT('Ctrl Pts',(60.4246762854926,-35.9802253773515,
12.));
#121370=CARTESIAN_POINT('Ctrl Pts',(60.4107226875714,-35.9654832299601,
0.));
#121371=CARTESIAN_POINT('Ctrl Pts',(60.4107226875714,-35.9654832299601,
12.));
#121372=CARTESIAN_POINT('Ctrl Pts',(60.3967893635452,-35.9507937296707,
0.));
#121373=CARTESIAN_POINT('Ctrl Pts',(60.3967893635452,-35.9507937296707,
12.));
#121374=CARTESIAN_POINT('Ctrl Pts',(60.3828765049019,-35.936156950695,0.));
#121375=CARTESIAN_POINT('Ctrl Pts',(60.3828765049019,-35.936156950695,12.));
#121376=CARTESIAN_POINT('Ctrl Pts',(60.3689842965481,-35.9215729642231,
0.));
#121377=CARTESIAN_POINT('Ctrl Pts',(60.3689842965481,-35.9215729642231,
12.));
#121378=CARTESIAN_POINT('Ctrl Pts',(60.3551129108845,-35.907041835853,0.));
#121379=CARTESIAN_POINT('Ctrl Pts',(60.3551129108845,-35.907041835853,12.));
#121380=CARTESIAN_POINT('Ctrl Pts',(60.3412625135287,-35.8925636280668,
0.));
#121381=CARTESIAN_POINT('Ctrl Pts',(60.3412625135287,-35.8925636280668,
12.));
#121382=CARTESIAN_POINT('Ctrl Pts',(60.327433274683,-35.8781384051537,0.));
#121383=CARTESIAN_POINT('Ctrl Pts',(60.327433274683,-35.8781384051537,12.));
#121384=CARTESIAN_POINT('Ctrl Pts',(60.3136253782809,-35.8637662371635,
0.));
#121385=CARTESIAN_POINT('Ctrl Pts',(60.3136253782809,-35.8637662371635,
12.));
#121386=CARTESIAN_POINT('Ctrl Pts',(60.2998390330102,-35.8494472046746,
0.));
#121387=CARTESIAN_POINT('Ctrl Pts',(60.2998390330102,-35.8494472046746,
12.));
#121388=CARTESIAN_POINT('Ctrl Pts',(60.2860744798436,-35.8351814020357,
0.));
#121389=CARTESIAN_POINT('Ctrl Pts',(60.2860744798436,-35.8351814020357,
12.));
#121390=CARTESIAN_POINT('Ctrl Pts',(60.2723319687369,-35.8209689272501,
0.));
#121391=CARTESIAN_POINT('Ctrl Pts',(60.2723319687369,-35.8209689272501,
12.));
#121392=CARTESIAN_POINT('Ctrl Pts',(60.2586117365205,-35.8068098723347,
0.));
#121393=CARTESIAN_POINT('Ctrl Pts',(60.2586117365205,-35.8068098723347,
12.));
#121394=CARTESIAN_POINT('Ctrl Pts',(60.2449139865274,-35.7927043145201,
0.));
#121395=CARTESIAN_POINT('Ctrl Pts',(60.2449139865274,-35.7927043145201,
12.));
#121396=CARTESIAN_POINT('Ctrl Pts',(60.2312388621529,-35.7786523045912,
0.));
#121397=CARTESIAN_POINT('Ctrl Pts',(60.2312388621529,-35.7786523045912,
12.));
#121398=CARTESIAN_POINT('Ctrl Pts',(60.2175864450043,-35.7646538667493,
0.));
#121399=CARTESIAN_POINT('Ctrl Pts',(60.2175864450043,-35.7646538667493,
12.));
#121400=CARTESIAN_POINT('Ctrl Pts',(60.206682708692,-35.7534979802053,0.));
#121401=CARTESIAN_POINT('Ctrl Pts',(60.206682708692,-35.7534979802053,12.));
#121402=CARTESIAN_POINT('Ctrl Pts',(60.1985151474623,-35.7451551752572,
0.));
#121403=CARTESIAN_POINT('Ctrl Pts',(60.1985151474623,-35.7451551752572,
12.));
#121404=CARTESIAN_POINT('Ctrl Pts',(60.193074658032,-35.7396040204017,0.));
#121405=CARTESIAN_POINT('Ctrl Pts',(60.193074658032,-35.7396040204017,12.));
#121406=CARTESIAN_POINT('Ctrl Pts',(60.1903555511633,-35.736831121751,0.));
#121407=CARTESIAN_POINT('Ctrl Pts',(60.1903555511633,-35.736831121751,12.));
#121408=CARTESIAN_POINT('',(60.1903555511633,-35.736831121751,12.));
#121409=CARTESIAN_POINT('Ctrl Pts',(60.1903555511633,-35.736831121751,12.));
#121410=CARTESIAN_POINT('Ctrl Pts',(60.193074658032,-35.7396040204017,12.));
#121411=CARTESIAN_POINT('Ctrl Pts',(60.1985151474623,-35.7451551752572,
12.));
#121412=CARTESIAN_POINT('Ctrl Pts',(60.206682708692,-35.7534979802053,12.));
#121413=CARTESIAN_POINT('Ctrl Pts',(60.2175864450043,-35.7646538667493,
12.));
#121414=CARTESIAN_POINT('Ctrl Pts',(60.2312388621529,-35.7786523045912,
12.));
#121415=CARTESIAN_POINT('Ctrl Pts',(60.2449139865274,-35.7927043145201,
12.));
#121416=CARTESIAN_POINT('Ctrl Pts',(60.2586117365205,-35.8068098723347,
12.));
#121417=CARTESIAN_POINT('Ctrl Pts',(60.2723319687369,-35.8209689272501,
12.));
#121418=CARTESIAN_POINT('Ctrl Pts',(60.2860744798436,-35.8351814020357,
12.));
#121419=CARTESIAN_POINT('Ctrl Pts',(60.2998390330102,-35.8494472046746,
12.));
#121420=CARTESIAN_POINT('Ctrl Pts',(60.3136253782809,-35.8637662371635,
12.));
#121421=CARTESIAN_POINT('Ctrl Pts',(60.327433274683,-35.8781384051537,12.));
#121422=CARTESIAN_POINT('Ctrl Pts',(60.3412625135287,-35.8925636280668,
12.));
#121423=CARTESIAN_POINT('Ctrl Pts',(60.3551129108845,-35.907041835853,12.));
#121424=CARTESIAN_POINT('Ctrl Pts',(60.3689842965481,-35.9215729642231,
12.));
#121425=CARTESIAN_POINT('Ctrl Pts',(60.3828765049019,-35.936156950695,12.));
#121426=CARTESIAN_POINT('Ctrl Pts',(60.3967893635452,-35.9507937296707,
12.));
#121427=CARTESIAN_POINT('Ctrl Pts',(60.4107226875714,-35.9654832299601,
12.));
#121428=CARTESIAN_POINT('Ctrl Pts',(60.4246762854926,-35.9802253773515,
12.));
#121429=CARTESIAN_POINT('Ctrl Pts',(60.4386499629481,-35.995020096217,12.));
#121430=CARTESIAN_POINT('Ctrl Pts',(60.4526435269662,-36.009867311357,12.));
#121431=CARTESIAN_POINT('Ctrl Pts',(60.4666567908093,-36.0247669500892,
12.));
#121432=CARTESIAN_POINT('Ctrl Pts',(60.4806895737686,-36.0397189421644,
12.));
#121433=CARTESIAN_POINT('Ctrl Pts',(60.4947416988422,-36.0547232187698,
12.));
#121434=CARTESIAN_POINT('Ctrl Pts',(60.5088129911354,-36.0697797118376,
12.));
#121435=CARTESIAN_POINT('Ctrl Pts',(60.5229032758973,-36.0848883531952,
12.));
#121436=CARTESIAN_POINT('Ctrl Pts',(60.5370123768804,-36.1000490738511,
12.));
#121437=CARTESIAN_POINT('Ctrl Pts',(60.5511401171984,-36.1152618043739,
12.));
#121438=CARTESIAN_POINT('Ctrl Pts',(60.565286320072,-36.1305264752188,12.));
#121439=CARTESIAN_POINT('Ctrl Pts',(60.5794508095564,-36.1458430170431,
12.));
#121440=CARTESIAN_POINT('Ctrl Pts',(60.5936334114108,-36.1612113610773,
12.));
#121441=CARTESIAN_POINT('Ctrl Pts',(60.6078339534181,-36.1766314392641,
12.));
#121442=CARTESIAN_POINT('Ctrl Pts',(60.6220522649149,-36.192103184063,12.));
#121443=CARTESIAN_POINT('Ctrl Pts',(60.6362881765019,-36.2076265283264,
12.));
#121444=CARTESIAN_POINT('Ctrl Pts',(60.6505415197042,-36.2232014051541,
12.));
#121445=CARTESIAN_POINT('Ctrl Pts',(60.6648121265885,-36.2388277477212,
12.));
#121446=CARTESIAN_POINT('Ctrl Pts',(60.67909982978,-36.2545054892897,12.));
#121447=CARTESIAN_POINT('Ctrl Pts',(60.6934044626291,-36.2702345632875,
12.));
#121448=CARTESIAN_POINT('Ctrl Pts',(60.7077258593268,-36.2860149033587,
12.));
#121449=CARTESIAN_POINT('Ctrl Pts',(60.722063855041,-36.3018464434214,12.));
#121450=CARTESIAN_POINT('Ctrl Pts',(60.7364182860412,-36.3177291177163,
12.));
#121451=CARTESIAN_POINT('Ctrl Pts',(60.7507889896308,-36.3336628607859,
12.));
#121452=CARTESIAN_POINT('Ctrl Pts',(60.7651758040803,-36.3496476074488,
12.));
#121453=CARTESIAN_POINT('Ctrl Pts',(60.7795785685625,-36.365683292773,12.));
#121454=CARTESIAN_POINT('Ctrl Pts',(60.793997123076,-36.3817698520388,12.));
#121455=CARTESIAN_POINT('Ctrl Pts',(60.8084313083984,-36.397907220716,12.));
#121456=CARTESIAN_POINT('Ctrl Pts',(60.822880966116,-36.4140953344859,12.));
#121457=CARTESIAN_POINT('Ctrl Pts',(60.8373459386392,-36.4303341292494,
12.));
#121458=CARTESIAN_POINT('Ctrl Pts',(60.8518260692188,-36.4466235411358,
12.));
#121459=CARTESIAN_POINT('Ctrl Pts',(60.8663212019657,-36.4629635065045,
12.));
#121460=CARTESIAN_POINT('Ctrl Pts',(60.8808311818499,-36.4793539619466,
12.));
#121461=CARTESIAN_POINT('Ctrl Pts',(60.8953558546795,-36.4957948442835,
12.));
#121462=CARTESIAN_POINT('Ctrl Pts',(60.9098950670847,-36.5122860905612,
12.));
#121463=CARTESIAN_POINT('Ctrl Pts',(60.9244486664987,-36.5288276380416,
12.));
#121464=CARTESIAN_POINT('Ctrl Pts',(60.9390165011355,-36.5454194241865,
12.));
#121465=CARTESIAN_POINT('Ctrl Pts',(60.9535984199873,-36.5620613866615,
12.));
#121466=CARTESIAN_POINT('Ctrl Pts',(60.9681942728236,-36.5787534633416,
12.));
#121467=CARTESIAN_POINT('Ctrl Pts',(60.9828039101887,-36.5954955923109,
12.));
#121468=CARTESIAN_POINT('Ctrl Pts',(60.9974271833981,-36.61228771186,12.));
#121469=CARTESIAN_POINT('Ctrl Pts',(61.0120639445349,-36.6291297604776,
12.));
#121470=CARTESIAN_POINT('Ctrl Pts',(61.0267140464432,-36.6460216768553,
12.));
#121471=CARTESIAN_POINT('Ctrl Pts',(61.0413773427203,-36.6629633998886,
12.));
#121472=CARTESIAN_POINT('Ctrl Pts',(61.0560536877083,-36.679954868674,12.));
#121473=CARTESIAN_POINT('Ctrl Pts',(61.0707429364847,-36.6969960225022,
12.));
#121474=CARTESIAN_POINT('Ctrl Pts',(61.0854449448524,-36.7140868008486,
12.));
#121475=CARTESIAN_POINT('Ctrl Pts',(61.100159569337,-36.7312271433807,12.));
#121476=CARTESIAN_POINT('Ctrl Pts',(61.1148866671829,-36.7484169899596,
12.));
#121477=CARTESIAN_POINT('Ctrl Pts',(61.1296260963466,-36.765656280638,12.));
#121478=CARTESIAN_POINT('Ctrl Pts',(61.1443777154911,-36.7829449556532,
12.));
#121479=CARTESIAN_POINT('Ctrl Pts',(61.1591413839787,-36.8002829554209,
12.));
#121480=CARTESIAN_POINT('Ctrl Pts',(61.1739169618666,-36.8176702205423,
12.));
#121481=CARTESIAN_POINT('Ctrl Pts',(61.1887043099014,-36.8351066918036,
12.));
#121482=CARTESIAN_POINT('Ctrl Pts',(61.2035032895127,-36.852592310174,12.));
#121483=CARTESIAN_POINT('Ctrl Pts',(61.2183137628056,-36.8701270167969,
12.));
#121484=CARTESIAN_POINT('Ctrl Pts',(61.2331355925547,-36.8877107529865,
12.));
#121485=CARTESIAN_POINT('Ctrl Pts',(61.247968642201,-36.9053434602343,12.));
#121486=CARTESIAN_POINT('Ctrl Pts',(61.2628127758457,-36.9230250802088,
12.));
#121487=CARTESIAN_POINT('Ctrl Pts',(61.2776678582461,-36.9407555547535,
12.));
#121488=CARTESIAN_POINT('Ctrl Pts',(61.2925337548077,-36.9585348258776,
12.));
#121489=CARTESIAN_POINT('Ctrl Pts',(61.3074103315791,-36.9763628357544,
12.));
#121490=CARTESIAN_POINT('Ctrl Pts',(61.3222974552486,-36.994239526727,12.));
#121491=CARTESIAN_POINT('Ctrl Pts',(61.3371949931387,-37.0121648413082,
12.));
#121492=CARTESIAN_POINT('Ctrl Pts',(61.3521028132003,-37.0301387221774,
12.));
#121493=CARTESIAN_POINT('Ctrl Pts',(61.3670207840068,-37.0481611121717,
12.));
#121494=CARTESIAN_POINT('Ctrl Pts',(61.381948774749,-37.0662319542849,12.));
#121495=CARTESIAN_POINT('Ctrl Pts',(61.3968866552317,-37.0843511916745,
12.));
#121496=CARTESIAN_POINT('Ctrl Pts',(61.4118342958697,-37.1025187676602,
12.));
#121497=CARTESIAN_POINT('Ctrl Pts',(61.4267915676822,-37.1207346257222,
12.));
#121498=CARTESIAN_POINT('Ctrl Pts',(61.4417583422863,-37.1389987094905,
12.));
#121499=CARTESIAN_POINT('Ctrl Pts',(61.4567344918919,-37.1573109627454,
12.));
#121500=CARTESIAN_POINT('Ctrl Pts',(61.4717198892994,-37.175671329424,12.));
#121501=CARTESIAN_POINT('Ctrl Pts',(61.4867144078936,-37.1940797536181,
12.));
#121502=CARTESIAN_POINT('Ctrl Pts',(61.501717921641,-37.2125361795731,12.));
#121503=CARTESIAN_POINT('Ctrl Pts',(61.5167303050832,-37.2310405516781,
12.));
#121504=CARTESIAN_POINT('Ctrl Pts',(61.5317514333328,-37.2495928144667,
12.));
#121505=CARTESIAN_POINT('Ctrl Pts',(61.5467811820691,-37.2681929126221,
12.));
#121506=CARTESIAN_POINT('Ctrl Pts',(61.5618194275348,-37.2868407909771,
12.));
#121507=CARTESIAN_POINT('Ctrl Pts',(61.5768660465311,-37.3055363945108,
12.));
#121508=CARTESIAN_POINT('Ctrl Pts',(61.591920916412,-37.3242796683395,12.));
#121509=CARTESIAN_POINT('Ctrl Pts',(61.6069839150807,-37.343070557718,12.));
#121510=CARTESIAN_POINT('Ctrl Pts',(61.6220549209866,-37.361909008045,12.));
#121511=CARTESIAN_POINT('Ctrl Pts',(61.637133813121,-37.3807949648624,12.));
#121512=CARTESIAN_POINT('Ctrl Pts',(61.6522204710131,-37.3997283738533,
12.));
#121513=CARTESIAN_POINT('Ctrl Pts',(61.6673147747242,-37.4187091808321,
12.));
#121514=CARTESIAN_POINT('Ctrl Pts',(61.6824166048444,-37.4377373317451,
12.));
#121515=CARTESIAN_POINT('Ctrl Pts',(61.6975258424894,-37.4568127726773,
12.));
#121516=CARTESIAN_POINT('Ctrl Pts',(61.7126423692963,-37.4759354498509,
12.));
#121517=CARTESIAN_POINT('Ctrl Pts',(61.7277660674205,-37.4951053096237,
12.));
#121518=CARTESIAN_POINT('Ctrl Pts',(61.7428968195299,-37.5143222984796,
12.));
#121519=CARTESIAN_POINT('Ctrl Pts',(61.7580345088016,-37.5335863630287,
12.));
#121520=CARTESIAN_POINT('Ctrl Pts',(61.773179018919,-37.5528974500142,12.));
#121521=CARTESIAN_POINT('Ctrl Pts',(61.7883302340687,-37.5722555063111,
12.));
#121522=CARTESIAN_POINT('Ctrl Pts',(61.8034880389362,-37.5916604789253,
12.));
#121523=CARTESIAN_POINT('Ctrl Pts',(61.8186523187015,-37.6111123149839,
12.));
#121524=CARTESIAN_POINT('Ctrl Pts',(61.8338229590352,-37.6306109617347,
12.));
#121525=CARTESIAN_POINT('Ctrl Pts',(61.8489998460957,-37.6501563665524,
12.));
#121526=CARTESIAN_POINT('Ctrl Pts',(61.8641828665261,-37.6697484769392,
12.));
#121527=CARTESIAN_POINT('Ctrl Pts',(61.8793719074507,-37.6893872405228,
12.));
#121528=CARTESIAN_POINT('Ctrl Pts',(61.8945668564704,-37.7090726050482,
12.));
#121529=CARTESIAN_POINT('Ctrl Pts',(61.9097676016601,-37.7288045183756,
12.));
#121530=CARTESIAN_POINT('Ctrl Pts',(61.9249740315649,-37.7485829284872,
12.));
#121531=CARTESIAN_POINT('Ctrl Pts',(61.9401860351972,-37.7684077834873,
12.));
#121532=CARTESIAN_POINT('Ctrl Pts',(61.9554035020338,-37.7882790316014,
12.));
#121533=CARTESIAN_POINT('Ctrl Pts',(61.9706263220114,-37.8081966211689,
12.));
#121534=CARTESIAN_POINT('Ctrl Pts',(61.9858543855236,-37.8281605006381,
12.));
#121535=CARTESIAN_POINT('Ctrl Pts',(62.0010875834187,-37.8481706185749,
12.));
#121536=CARTESIAN_POINT('Ctrl Pts',(62.0163258069957,-37.868226923663,12.));
#121537=CARTESIAN_POINT('Ctrl Pts',(62.031568948002,-37.8883293647029,12.));
#121538=CARTESIAN_POINT('Ctrl Pts',(62.0468168986288,-37.9084778906053,
12.));
#121539=CARTESIAN_POINT('Ctrl Pts',(62.0620695515074,-37.9286724503851,
12.));
#121540=CARTESIAN_POINT('Ctrl Pts',(62.0773267997078,-37.9489129931689,
12.));
#121541=CARTESIAN_POINT('Ctrl Pts',(62.0925885367352,-37.9691994681966,
12.));
#121542=CARTESIAN_POINT('Ctrl Pts',(62.107854656528,-37.9895318248212,12.));
#121543=CARTESIAN_POINT('Ctrl Pts',(62.123125053455,-38.0099100125037,12.));
#121544=CARTESIAN_POINT('Ctrl Pts',(62.1383996223124,-38.0303339808053,
12.));
#121545=CARTESIAN_POINT('Ctrl Pts',(62.1536782583199,-38.0508036793939,
12.));
#121546=CARTESIAN_POINT('Ctrl Pts',(62.1689608571176,-38.0713190580463,
12.));
#121547=CARTESIAN_POINT('Ctrl Pts',(62.1842473147626,-38.0918800666479,
12.));
#121548=CARTESIAN_POINT('Ctrl Pts',(62.1995375277257,-38.1124866551886,
12.));
#121549=CARTESIAN_POINT('Ctrl Pts',(62.2148313928863,-38.133138773753,12.));
#121550=CARTESIAN_POINT('Ctrl Pts',(62.2301288075321,-38.1538363725264,
12.));
#121551=CARTESIAN_POINT('Ctrl Pts',(62.245429669358,-38.1745794017996,12.));
#121552=CARTESIAN_POINT('Ctrl Pts',(62.2607338764654,-38.1953678119691,
12.));
#121553=CARTESIAN_POINT('Ctrl Pts',(62.2760413273602,-38.2162015535353,
12.));
#121554=CARTESIAN_POINT('Ctrl Pts',(62.2913519209521,-38.2370805770935,
12.));
#121555=CARTESIAN_POINT('Ctrl Pts',(62.3066655565503,-38.2580048333361,
12.));
#121556=CARTESIAN_POINT('Ctrl Pts',(62.3219821338569,-38.2789742730564,
12.));
#121557=CARTESIAN_POINT('Ctrl Pts',(62.3373015529613,-38.2999888471476,
12.));
#121558=CARTESIAN_POINT('Ctrl Pts',(62.3526237143336,-38.3210485066001,
12.));
#121559=CARTESIAN_POINT('Ctrl Pts',(62.3679485188171,-38.342153202491,12.));
#121560=CARTESIAN_POINT('Ctrl Pts',(62.3832758676271,-38.3633028859828,
12.));
#121561=CARTESIAN_POINT('Ctrl Pts',(62.3986056623577,-38.3844975083344,
12.));
#121562=CARTESIAN_POINT('Ctrl Pts',(62.4139378049885,-38.405737020905,12.));
#121563=CARTESIAN_POINT('Ctrl Pts',(62.4292721978901,-38.4270213751568,
12.));
#121564=CARTESIAN_POINT('Ctrl Pts',(62.4446087438312,-38.4483505226518,
12.));
#121565=CARTESIAN_POINT('Ctrl Pts',(62.4599473459811,-38.4697244150482,
12.));
#121566=CARTESIAN_POINT('Ctrl Pts',(62.4752879078854,-38.4911430040997,
12.));
#121567=CARTESIAN_POINT('Ctrl Pts',(62.4906303334443,-38.5126062416502,
12.));
#121568=CARTESIAN_POINT('Ctrl Pts',(62.5059745268901,-38.5341140796248,
12.));
#121569=CARTESIAN_POINT('Ctrl Pts',(62.5213203927663,-38.5556664700195,
12.));
#121570=CARTESIAN_POINT('Ctrl Pts',(62.5366678359023,-38.5772633648833,
12.));
#121571=CARTESIAN_POINT('Ctrl Pts',(62.5520167614516,-38.5989047163393,
12.));
#121572=CARTESIAN_POINT('Ctrl Pts',(62.5673670749361,-38.6205904766073,
12.));
#121573=CARTESIAN_POINT('Ctrl Pts',(62.582718682292,-38.6423205980213,12.));
#121574=CARTESIAN_POINT('Ctrl Pts',(62.5980714899052,-38.6640950330421,
12.));
#121575=CARTESIAN_POINT('Ctrl Pts',(62.6134254046739,-38.6859137342731,
12.));
#121576=CARTESIAN_POINT('Ctrl Pts',(62.6287803339542,-38.7077766544416,
12.));
#121577=CARTESIAN_POINT('Ctrl Pts',(62.6441361854411,-38.7296837463609,
12.));
#121578=CARTESIAN_POINT('Ctrl Pts',(62.6594928670628,-38.7516349628904,
12.));
#121579=CARTESIAN_POINT('Ctrl Pts',(62.6748502868835,-38.7736302568982,
12.));
#121580=CARTESIAN_POINT('Ctrl Pts',(62.6902083529694,-38.795669581203,12.));
#121581=CARTESIAN_POINT('Ctrl Pts',(62.7055669733802,-38.8177528885681,
12.));
#121582=CARTESIAN_POINT('Ctrl Pts',(62.7209260564493,-38.8398801318177,
12.));
#121583=CARTESIAN_POINT('Ctrl Pts',(62.7362855110042,-38.8620512639233,
12.));
#121584=CARTESIAN_POINT('Ctrl Pts',(62.7516452466128,-38.8842662380984,
12.));
#121585=CARTESIAN_POINT('Ctrl Pts',(62.7670051738143,-38.9065250078832,
12.));
#121586=CARTESIAN_POINT('Ctrl Pts',(62.78236520437,-38.9288275272335,12.));
#121587=CARTESIAN_POINT('Ctrl Pts',(62.7977252507117,-38.9511737503165,
12.));
#121588=CARTESIAN_POINT('Ctrl Pts',(62.8130852254027,-38.9735636313089,
12.));
#121589=CARTESIAN_POINT('Ctrl Pts',(62.8284450405459,-38.9959971241701,
12.));
#121590=CARTESIAN_POINT('Ctrl Pts',(62.8438046073224,-39.0184741824641,
12.));
#121591=CARTESIAN_POINT('Ctrl Pts',(62.8591638352055,-39.0409947590497,
12.));
#121592=CARTESIAN_POINT('Ctrl Pts',(62.8745226325998,-39.0635588063277,
12.));
#121593=CARTESIAN_POINT('Ctrl Pts',(62.8898809082611,-39.0861662767932,
12.));
#121594=CARTESIAN_POINT('Ctrl Pts',(62.9052385725387,-39.1088171235125,
12.));
#121595=CARTESIAN_POINT('Ctrl Pts',(62.9205955385558,-39.131511300575,12.));
#121596=CARTESIAN_POINT('Ctrl Pts',(62.9359517237404,-39.1542487636744,
12.));
#121597=CARTESIAN_POINT('Ctrl Pts',(62.9513070501867,-39.1770294702428,
12.));
#121598=CARTESIAN_POINT('Ctrl Pts',(62.9644687386836,-39.1965939820933,
12.));
#121599=CARTESIAN_POINT('Ctrl Pts',(62.9745590018672,-39.2116170128461,
12.));
#121600=CARTESIAN_POINT('Ctrl Pts',(62.9815782721325,-39.2220794388807,
12.));
#121601=CARTESIAN_POINT('Ctrl Pts',(62.9855268616127,-39.2279686275006,
12.));
#121602=CARTESIAN_POINT('Ctrl Pts',(62.9864049293894,-39.2292784191812,
12.));
#121603=CARTESIAN_POINT('',(60.1903555511633,-35.736831121751,0.));
#121604=CARTESIAN_POINT('',(60.1903555511633,-35.736831121751,0.));
#121605=CARTESIAN_POINT('Ctrl Pts',(62.9864049293894,-39.2292784191813,
0.));
#121606=CARTESIAN_POINT('Ctrl Pts',(62.9855268616127,-39.2279686275007,
0.));
#121607=CARTESIAN_POINT('Ctrl Pts',(62.9815782721326,-39.2220794388807,
0.));
#121608=CARTESIAN_POINT('Ctrl Pts',(62.9745590018672,-39.2116170128461,
0.));
#121609=CARTESIAN_POINT('Ctrl Pts',(62.9644687386836,-39.1965939820933,
0.));
#121610=CARTESIAN_POINT('Ctrl Pts',(62.9513070501867,-39.1770294702428,
0.));
#121611=CARTESIAN_POINT('Ctrl Pts',(62.9359517237404,-39.1542487636744,
0.));
#121612=CARTESIAN_POINT('Ctrl Pts',(62.9205955385558,-39.131511300575,0.));
#121613=CARTESIAN_POINT('Ctrl Pts',(62.9052385725387,-39.1088171235125,
0.));
#121614=CARTESIAN_POINT('Ctrl Pts',(62.8898809082611,-39.0861662767932,
0.));
#121615=CARTESIAN_POINT('Ctrl Pts',(62.8745226325998,-39.0635588063277,
0.));
#121616=CARTESIAN_POINT('Ctrl Pts',(62.8591638352055,-39.0409947590497,
0.));
#121617=CARTESIAN_POINT('Ctrl Pts',(62.8438046073224,-39.0184741824641,
0.));
#121618=CARTESIAN_POINT('Ctrl Pts',(62.8284450405459,-38.9959971241701,
0.));
#121619=CARTESIAN_POINT('Ctrl Pts',(62.8130852254027,-38.9735636313089,
0.));
#121620=CARTESIAN_POINT('Ctrl Pts',(62.7977252507117,-38.9511737503165,
0.));
#121621=CARTESIAN_POINT('Ctrl Pts',(62.78236520437,-38.9288275272335,0.));
#121622=CARTESIAN_POINT('Ctrl Pts',(62.7670051738143,-38.9065250078832,
0.));
#121623=CARTESIAN_POINT('Ctrl Pts',(62.7516452466128,-38.8842662380984,
0.));
#121624=CARTESIAN_POINT('Ctrl Pts',(62.7362855110042,-38.8620512639233,
0.));
#121625=CARTESIAN_POINT('Ctrl Pts',(62.7209260564493,-38.8398801318177,
0.));
#121626=CARTESIAN_POINT('Ctrl Pts',(62.7055669733802,-38.8177528885681,
0.));
#121627=CARTESIAN_POINT('Ctrl Pts',(62.6902083529694,-38.795669581203,0.));
#121628=CARTESIAN_POINT('Ctrl Pts',(62.6748502868835,-38.7736302568982,
0.));
#121629=CARTESIAN_POINT('Ctrl Pts',(62.6594928670628,-38.7516349628904,
0.));
#121630=CARTESIAN_POINT('Ctrl Pts',(62.6441361854411,-38.7296837463609,
0.));
#121631=CARTESIAN_POINT('Ctrl Pts',(62.6287803339542,-38.7077766544416,
0.));
#121632=CARTESIAN_POINT('Ctrl Pts',(62.6134254046739,-38.6859137342731,
0.));
#121633=CARTESIAN_POINT('Ctrl Pts',(62.5980714899052,-38.6640950330421,
0.));
#121634=CARTESIAN_POINT('Ctrl Pts',(62.582718682292,-38.6423205980213,0.));
#121635=CARTESIAN_POINT('Ctrl Pts',(62.5673670749361,-38.6205904766073,
0.));
#121636=CARTESIAN_POINT('Ctrl Pts',(62.5520167614516,-38.5989047163393,
0.));
#121637=CARTESIAN_POINT('Ctrl Pts',(62.5366678359023,-38.5772633648833,
0.));
#121638=CARTESIAN_POINT('Ctrl Pts',(62.5213203927663,-38.5556664700195,
0.));
#121639=CARTESIAN_POINT('Ctrl Pts',(62.5059745268901,-38.5341140796248,
0.));
#121640=CARTESIAN_POINT('Ctrl Pts',(62.4906303334443,-38.5126062416502,
0.));
#121641=CARTESIAN_POINT('Ctrl Pts',(62.4752879078854,-38.4911430040997,
0.));
#121642=CARTESIAN_POINT('Ctrl Pts',(62.4599473459811,-38.4697244150482,
0.));
#121643=CARTESIAN_POINT('Ctrl Pts',(62.4446087438312,-38.4483505226518,
0.));
#121644=CARTESIAN_POINT('Ctrl Pts',(62.4292721978901,-38.4270213751568,
0.));
#121645=CARTESIAN_POINT('Ctrl Pts',(62.4139378049885,-38.405737020905,0.));
#121646=CARTESIAN_POINT('Ctrl Pts',(62.3986056623577,-38.3844975083344,
0.));
#121647=CARTESIAN_POINT('Ctrl Pts',(62.3832758676271,-38.3633028859828,
0.));
#121648=CARTESIAN_POINT('Ctrl Pts',(62.3679485188171,-38.342153202491,0.));
#121649=CARTESIAN_POINT('Ctrl Pts',(62.3526237143336,-38.3210485066001,
0.));
#121650=CARTESIAN_POINT('Ctrl Pts',(62.3373015529613,-38.2999888471476,
0.));
#121651=CARTESIAN_POINT('Ctrl Pts',(62.3219821338569,-38.2789742730564,
0.));
#121652=CARTESIAN_POINT('Ctrl Pts',(62.3066655565503,-38.2580048333361,
0.));
#121653=CARTESIAN_POINT('Ctrl Pts',(62.2913519209521,-38.2370805770935,
0.));
#121654=CARTESIAN_POINT('Ctrl Pts',(62.2760413273602,-38.2162015535353,
0.));
#121655=CARTESIAN_POINT('Ctrl Pts',(62.2607338764654,-38.1953678119691,
0.));
#121656=CARTESIAN_POINT('Ctrl Pts',(62.245429669358,-38.1745794017996,0.));
#121657=CARTESIAN_POINT('Ctrl Pts',(62.2301288075321,-38.1538363725264,
0.));
#121658=CARTESIAN_POINT('Ctrl Pts',(62.2148313928863,-38.133138773753,0.));
#121659=CARTESIAN_POINT('Ctrl Pts',(62.1995375277257,-38.1124866551886,
0.));
#121660=CARTESIAN_POINT('Ctrl Pts',(62.1842473147626,-38.0918800666479,
0.));
#121661=CARTESIAN_POINT('Ctrl Pts',(62.1689608571176,-38.0713190580463,
0.));
#121662=CARTESIAN_POINT('Ctrl Pts',(62.1536782583199,-38.0508036793939,
0.));
#121663=CARTESIAN_POINT('Ctrl Pts',(62.1383996223124,-38.0303339808053,
0.));
#121664=CARTESIAN_POINT('Ctrl Pts',(62.123125053455,-38.0099100125037,0.));
#121665=CARTESIAN_POINT('Ctrl Pts',(62.107854656528,-37.9895318248212,0.));
#121666=CARTESIAN_POINT('Ctrl Pts',(62.0925885367352,-37.9691994681966,
0.));
#121667=CARTESIAN_POINT('Ctrl Pts',(62.0773267997078,-37.9489129931689,
0.));
#121668=CARTESIAN_POINT('Ctrl Pts',(62.0620695515074,-37.9286724503851,
0.));
#121669=CARTESIAN_POINT('Ctrl Pts',(62.0468168986288,-37.9084778906053,
0.));
#121670=CARTESIAN_POINT('Ctrl Pts',(62.031568948002,-37.8883293647029,0.));
#121671=CARTESIAN_POINT('Ctrl Pts',(62.0163258069957,-37.868226923663,0.));
#121672=CARTESIAN_POINT('Ctrl Pts',(62.0010875834187,-37.8481706185749,
0.));
#121673=CARTESIAN_POINT('Ctrl Pts',(61.9858543855236,-37.8281605006381,
0.));
#121674=CARTESIAN_POINT('Ctrl Pts',(61.9706263220114,-37.8081966211689,
0.));
#121675=CARTESIAN_POINT('Ctrl Pts',(61.9554035020338,-37.7882790316014,
0.));
#121676=CARTESIAN_POINT('Ctrl Pts',(61.9401860351972,-37.7684077834873,
0.));
#121677=CARTESIAN_POINT('Ctrl Pts',(61.9249740315649,-37.7485829284872,
0.));
#121678=CARTESIAN_POINT('Ctrl Pts',(61.9097676016601,-37.7288045183756,
0.));
#121679=CARTESIAN_POINT('Ctrl Pts',(61.8945668564704,-37.7090726050482,
0.));
#121680=CARTESIAN_POINT('Ctrl Pts',(61.8793719074507,-37.6893872405228,
0.));
#121681=CARTESIAN_POINT('Ctrl Pts',(61.8641828665261,-37.6697484769392,
0.));
#121682=CARTESIAN_POINT('Ctrl Pts',(61.8489998460957,-37.6501563665524,
0.));
#121683=CARTESIAN_POINT('Ctrl Pts',(61.8338229590352,-37.6306109617347,
0.));
#121684=CARTESIAN_POINT('Ctrl Pts',(61.8186523187015,-37.6111123149839,
0.));
#121685=CARTESIAN_POINT('Ctrl Pts',(61.8034880389362,-37.5916604789253,
0.));
#121686=CARTESIAN_POINT('Ctrl Pts',(61.7883302340687,-37.5722555063111,
0.));
#121687=CARTESIAN_POINT('Ctrl Pts',(61.773179018919,-37.5528974500142,0.));
#121688=CARTESIAN_POINT('Ctrl Pts',(61.7580345088016,-37.5335863630287,
0.));
#121689=CARTESIAN_POINT('Ctrl Pts',(61.7428968195299,-37.5143222984796,
0.));
#121690=CARTESIAN_POINT('Ctrl Pts',(61.7277660674205,-37.4951053096237,
0.));
#121691=CARTESIAN_POINT('Ctrl Pts',(61.7126423692963,-37.4759354498509,
0.));
#121692=CARTESIAN_POINT('Ctrl Pts',(61.6975258424894,-37.4568127726773,
0.));
#121693=CARTESIAN_POINT('Ctrl Pts',(61.6824166048444,-37.4377373317451,
0.));
#121694=CARTESIAN_POINT('Ctrl Pts',(61.6673147747242,-37.4187091808321,
0.));
#121695=CARTESIAN_POINT('Ctrl Pts',(61.6522204710131,-37.3997283738533,
0.));
#121696=CARTESIAN_POINT('Ctrl Pts',(61.637133813121,-37.3807949648624,0.));
#121697=CARTESIAN_POINT('Ctrl Pts',(61.6220549209866,-37.361909008045,0.));
#121698=CARTESIAN_POINT('Ctrl Pts',(61.6069839150807,-37.343070557718,0.));
#121699=CARTESIAN_POINT('Ctrl Pts',(61.591920916412,-37.3242796683395,0.));
#121700=CARTESIAN_POINT('Ctrl Pts',(61.5768660465311,-37.3055363945108,
0.));
#121701=CARTESIAN_POINT('Ctrl Pts',(61.5618194275348,-37.2868407909771,
0.));
#121702=CARTESIAN_POINT('Ctrl Pts',(61.5467811820691,-37.2681929126221,
0.));
#121703=CARTESIAN_POINT('Ctrl Pts',(61.5317514333328,-37.2495928144667,
0.));
#121704=CARTESIAN_POINT('Ctrl Pts',(61.5167303050832,-37.2310405516781,
0.));
#121705=CARTESIAN_POINT('Ctrl Pts',(61.501717921641,-37.2125361795731,0.));
#121706=CARTESIAN_POINT('Ctrl Pts',(61.4867144078936,-37.1940797536181,
0.));
#121707=CARTESIAN_POINT('Ctrl Pts',(61.4717198892994,-37.175671329424,0.));
#121708=CARTESIAN_POINT('Ctrl Pts',(61.4567344918919,-37.1573109627454,
0.));
#121709=CARTESIAN_POINT('Ctrl Pts',(61.4417583422863,-37.1389987094905,
0.));
#121710=CARTESIAN_POINT('Ctrl Pts',(61.4267915676822,-37.1207346257222,
0.));
#121711=CARTESIAN_POINT('Ctrl Pts',(61.4118342958697,-37.1025187676602,
0.));
#121712=CARTESIAN_POINT('Ctrl Pts',(61.3968866552317,-37.0843511916745,
0.));
#121713=CARTESIAN_POINT('Ctrl Pts',(61.381948774749,-37.0662319542849,0.));
#121714=CARTESIAN_POINT('Ctrl Pts',(61.3670207840068,-37.0481611121717,
0.));
#121715=CARTESIAN_POINT('Ctrl Pts',(61.3521028132003,-37.0301387221774,
0.));
#121716=CARTESIAN_POINT('Ctrl Pts',(61.3371949931387,-37.0121648413082,
0.));
#121717=CARTESIAN_POINT('Ctrl Pts',(61.3222974552486,-36.994239526727,0.));
#121718=CARTESIAN_POINT('Ctrl Pts',(61.3074103315791,-36.9763628357544,
0.));
#121719=CARTESIAN_POINT('Ctrl Pts',(61.2925337548077,-36.9585348258776,
0.));
#121720=CARTESIAN_POINT('Ctrl Pts',(61.2776678582461,-36.9407555547535,
0.));
#121721=CARTESIAN_POINT('Ctrl Pts',(61.2628127758457,-36.9230250802088,
0.));
#121722=CARTESIAN_POINT('Ctrl Pts',(61.247968642201,-36.9053434602343,0.));
#121723=CARTESIAN_POINT('Ctrl Pts',(61.2331355925547,-36.8877107529865,
0.));
#121724=CARTESIAN_POINT('Ctrl Pts',(61.2183137628056,-36.8701270167969,
0.));
#121725=CARTESIAN_POINT('Ctrl Pts',(61.2035032895127,-36.852592310174,0.));
#121726=CARTESIAN_POINT('Ctrl Pts',(61.1887043099014,-36.8351066918036,
0.));
#121727=CARTESIAN_POINT('Ctrl Pts',(61.1739169618666,-36.8176702205423,
0.));
#121728=CARTESIAN_POINT('Ctrl Pts',(61.1591413839787,-36.8002829554209,
0.));
#121729=CARTESIAN_POINT('Ctrl Pts',(61.1443777154911,-36.7829449556532,
0.));
#121730=CARTESIAN_POINT('Ctrl Pts',(61.1296260963466,-36.765656280638,0.));
#121731=CARTESIAN_POINT('Ctrl Pts',(61.1148866671829,-36.7484169899596,
0.));
#121732=CARTESIAN_POINT('Ctrl Pts',(61.100159569337,-36.7312271433807,0.));
#121733=CARTESIAN_POINT('Ctrl Pts',(61.0854449448524,-36.7140868008486,
0.));
#121734=CARTESIAN_POINT('Ctrl Pts',(61.0707429364847,-36.6969960225022,
0.));
#121735=CARTESIAN_POINT('Ctrl Pts',(61.0560536877083,-36.679954868674,0.));
#121736=CARTESIAN_POINT('Ctrl Pts',(61.0413773427203,-36.6629633998886,
0.));
#121737=CARTESIAN_POINT('Ctrl Pts',(61.0267140464432,-36.6460216768553,
0.));
#121738=CARTESIAN_POINT('Ctrl Pts',(61.0120639445349,-36.6291297604776,
0.));
#121739=CARTESIAN_POINT('Ctrl Pts',(60.9974271833981,-36.61228771186,0.));
#121740=CARTESIAN_POINT('Ctrl Pts',(60.9828039101887,-36.5954955923109,
0.));
#121741=CARTESIAN_POINT('Ctrl Pts',(60.9681942728236,-36.5787534633416,
0.));
#121742=CARTESIAN_POINT('Ctrl Pts',(60.9535984199873,-36.5620613866615,
0.));
#121743=CARTESIAN_POINT('Ctrl Pts',(60.9390165011355,-36.5454194241865,
0.));
#121744=CARTESIAN_POINT('Ctrl Pts',(60.9244486664987,-36.5288276380416,
0.));
#121745=CARTESIAN_POINT('Ctrl Pts',(60.9098950670847,-36.5122860905612,
0.));
#121746=CARTESIAN_POINT('Ctrl Pts',(60.8953558546795,-36.4957948442835,
0.));
#121747=CARTESIAN_POINT('Ctrl Pts',(60.8808311818499,-36.4793539619466,
0.));
#121748=CARTESIAN_POINT('Ctrl Pts',(60.8663212019657,-36.4629635065045,
0.));
#121749=CARTESIAN_POINT('Ctrl Pts',(60.8518260692188,-36.4466235411358,
0.));
#121750=CARTESIAN_POINT('Ctrl Pts',(60.8373459386392,-36.4303341292494,
0.));
#121751=CARTESIAN_POINT('Ctrl Pts',(60.822880966116,-36.4140953344859,0.));
#121752=CARTESIAN_POINT('Ctrl Pts',(60.8084313083984,-36.397907220716,0.));
#121753=CARTESIAN_POINT('Ctrl Pts',(60.793997123076,-36.3817698520388,0.));
#121754=CARTESIAN_POINT('Ctrl Pts',(60.7795785685625,-36.365683292773,0.));
#121755=CARTESIAN_POINT('Ctrl Pts',(60.7651758040803,-36.3496476074488,
0.));
#121756=CARTESIAN_POINT('Ctrl Pts',(60.7507889896308,-36.3336628607859,
0.));
#121757=CARTESIAN_POINT('Ctrl Pts',(60.7364182860412,-36.3177291177163,
0.));
#121758=CARTESIAN_POINT('Ctrl Pts',(60.722063855041,-36.3018464434214,0.));
#121759=CARTESIAN_POINT('Ctrl Pts',(60.7077258593268,-36.2860149033587,
0.));
#121760=CARTESIAN_POINT('Ctrl Pts',(60.6934044626291,-36.2702345632875,
0.));
#121761=CARTESIAN_POINT('Ctrl Pts',(60.67909982978,-36.2545054892897,0.));
#121762=CARTESIAN_POINT('Ctrl Pts',(60.6648121265885,-36.2388277477212,
0.));
#121763=CARTESIAN_POINT('Ctrl Pts',(60.6505415197042,-36.2232014051541,
0.));
#121764=CARTESIAN_POINT('Ctrl Pts',(60.6362881765019,-36.2076265283264,
0.));
#121765=CARTESIAN_POINT('Ctrl Pts',(60.6220522649149,-36.192103184063,0.));
#121766=CARTESIAN_POINT('Ctrl Pts',(60.6078339534181,-36.1766314392641,
0.));
#121767=CARTESIAN_POINT('Ctrl Pts',(60.5936334114108,-36.1612113610773,
0.));
#121768=CARTESIAN_POINT('Ctrl Pts',(60.5794508095564,-36.1458430170431,
0.));
#121769=CARTESIAN_POINT('Ctrl Pts',(60.565286320072,-36.1305264752188,0.));
#121770=CARTESIAN_POINT('Ctrl Pts',(60.5511401171984,-36.1152618043739,
0.));
#121771=CARTESIAN_POINT('Ctrl Pts',(60.5370123768804,-36.1000490738511,
0.));
#121772=CARTESIAN_POINT('Ctrl Pts',(60.5229032758973,-36.0848883531952,
0.));
#121773=CARTESIAN_POINT('Ctrl Pts',(60.5088129911354,-36.0697797118376,
0.));
#121774=CARTESIAN_POINT('Ctrl Pts',(60.4947416988422,-36.0547232187698,
0.));
#121775=CARTESIAN_POINT('Ctrl Pts',(60.4806895737686,-36.0397189421644,
0.));
#121776=CARTESIAN_POINT('Ctrl Pts',(60.4666567908093,-36.0247669500892,
0.));
#121777=CARTESIAN_POINT('Ctrl Pts',(60.4526435269662,-36.009867311357,0.));
#121778=CARTESIAN_POINT('Ctrl Pts',(60.4386499629481,-35.995020096217,0.));
#121779=CARTESIAN_POINT('Ctrl Pts',(60.4246762854926,-35.9802253773515,
0.));
#121780=CARTESIAN_POINT('Ctrl Pts',(60.4107226875714,-35.9654832299601,
0.));
#121781=CARTESIAN_POINT('Ctrl Pts',(60.3967893635452,-35.9507937296707,
0.));
#121782=CARTESIAN_POINT('Ctrl Pts',(60.3828765049019,-35.936156950695,0.));
#121783=CARTESIAN_POINT('Ctrl Pts',(60.3689842965481,-35.9215729642231,
0.));
#121784=CARTESIAN_POINT('Ctrl Pts',(60.3551129108845,-35.907041835853,0.));
#121785=CARTESIAN_POINT('Ctrl Pts',(60.3412625135287,-35.8925636280668,
0.));
#121786=CARTESIAN_POINT('Ctrl Pts',(60.327433274683,-35.8781384051537,0.));
#121787=CARTESIAN_POINT('Ctrl Pts',(60.3136253782809,-35.8637662371635,
0.));
#121788=CARTESIAN_POINT('Ctrl Pts',(60.2998390330102,-35.8494472046746,
0.));
#121789=CARTESIAN_POINT('Ctrl Pts',(60.2860744798436,-35.8351814020357,
0.));
#121790=CARTESIAN_POINT('Ctrl Pts',(60.2723319687369,-35.8209689272501,
0.));
#121791=CARTESIAN_POINT('Ctrl Pts',(60.2586117365205,-35.8068098723347,
0.));
#121792=CARTESIAN_POINT('Ctrl Pts',(60.2449139865274,-35.7927043145201,
0.));
#121793=CARTESIAN_POINT('Ctrl Pts',(60.2312388621529,-35.7786523045912,
0.));
#121794=CARTESIAN_POINT('Ctrl Pts',(60.2175864450043,-35.7646538667493,
0.));
#121795=CARTESIAN_POINT('Ctrl Pts',(60.206682708692,-35.7534979802053,0.));
#121796=CARTESIAN_POINT('Ctrl Pts',(60.1985151474623,-35.7451551752572,
0.));
#121797=CARTESIAN_POINT('Ctrl Pts',(60.193074658032,-35.7396040204017,0.));
#121798=CARTESIAN_POINT('Ctrl Pts',(60.1903555511633,-35.736831121751,0.));
#121799=CARTESIAN_POINT('Ctrl Pts',(59.483083043136,-44.8554660179045,0.));
#121800=CARTESIAN_POINT('Ctrl Pts',(59.483083043136,-44.8554660179045,12.));
#121801=CARTESIAN_POINT('Ctrl Pts',(59.4804358983083,-44.8505359826461,
0.));
#121802=CARTESIAN_POINT('Ctrl Pts',(59.4804358983083,-44.8505359826461,
12.));
#121803=CARTESIAN_POINT('Ctrl Pts',(59.4751410547732,-44.8406801497742,
0.));
#121804=CARTESIAN_POINT('Ctrl Pts',(59.4751410547732,-44.8406801497742,
12.));
#121805=CARTESIAN_POINT('Ctrl Pts',(59.4671971278321,-44.8259091134016,
0.));
#121806=CARTESIAN_POINT('Ctrl Pts',(59.4671971278321,-44.8259091134016,
12.));
#121807=CARTESIAN_POINT('Ctrl Pts',(59.4566019018253,-44.8062398251406,
0.));
#121808=CARTESIAN_POINT('Ctrl Pts',(59.4566019018253,-44.8062398251406,
12.));
#121809=CARTESIAN_POINT('Ctrl Pts',(59.4433523335147,-44.7816956017528,
0.));
#121810=CARTESIAN_POINT('Ctrl Pts',(59.4433523335147,-44.7816956017528,
12.));
#121811=CARTESIAN_POINT('Ctrl Pts',(59.430097240324,-44.7571937812113,0.));
#121812=CARTESIAN_POINT('Ctrl Pts',(59.430097240324,-44.7571937812113,12.));
#121813=CARTESIAN_POINT('Ctrl Pts',(59.4168366453118,-44.7327343876391,
0.));
#121814=CARTESIAN_POINT('Ctrl Pts',(59.4168366453118,-44.7327343876391,
12.));
#121815=CARTESIAN_POINT('Ctrl Pts',(59.4035705873811,-44.7083174541702,
0.));
#121816=CARTESIAN_POINT('Ctrl Pts',(59.4035705873811,-44.7083174541702,
12.));
#121817=CARTESIAN_POINT('Ctrl Pts',(59.3902991267889,-44.683943024421,0.));
#121818=CARTESIAN_POINT('Ctrl Pts',(59.3902991267889,-44.683943024421,12.));
#121819=CARTESIAN_POINT('Ctrl Pts',(59.377022343519,-44.6596111512687,0.));
#121820=CARTESIAN_POINT('Ctrl Pts',(59.377022343519,-44.6596111512687,12.));
#121821=CARTESIAN_POINT('Ctrl Pts',(59.36374033018,-44.6353218935685,0.));
#121822=CARTESIAN_POINT('Ctrl Pts',(59.36374033018,-44.6353218935685,12.));
#121823=CARTESIAN_POINT('Ctrl Pts',(59.3504531864154,-44.6110753134277,
0.));
#121824=CARTESIAN_POINT('Ctrl Pts',(59.3504531864154,-44.6110753134277,
12.));
#121825=CARTESIAN_POINT('Ctrl Pts',(59.3371610128511,-44.5868714733234,
0.));
#121826=CARTESIAN_POINT('Ctrl Pts',(59.3371610128511,-44.5868714733234,
12.));
#121827=CARTESIAN_POINT('Ctrl Pts',(59.3238639048694,-44.5627104331017,
0.));
#121828=CARTESIAN_POINT('Ctrl Pts',(59.3238639048694,-44.5627104331017,
12.));
#121829=CARTESIAN_POINT('Ctrl Pts',(59.3105619475609,-44.5385922475573,
0.));
#121830=CARTESIAN_POINT('Ctrl Pts',(59.3105619475609,-44.5385922475573,
12.));
#121831=CARTESIAN_POINT('Ctrl Pts',(59.2972552192156,-44.5145169681349,
0.));
#121832=CARTESIAN_POINT('Ctrl Pts',(59.2972552192156,-44.5145169681349,
12.));
#121833=CARTESIAN_POINT('Ctrl Pts',(59.2839437938237,-44.490484644151,0.));
#121834=CARTESIAN_POINT('Ctrl Pts',(59.2839437938237,-44.490484644151,12.));
#121835=CARTESIAN_POINT('Ctrl Pts',(59.2706277440445,-44.4664953242379,
0.));
#121836=CARTESIAN_POINT('Ctrl Pts',(59.2706277440445,-44.4664953242379,
12.));
#121837=CARTESIAN_POINT('Ctrl Pts',(59.2573071437774,-44.4425490575911,
0.));
#121838=CARTESIAN_POINT('Ctrl Pts',(59.2573071437774,-44.4425490575911,
12.));
#121839=CARTESIAN_POINT('Ctrl Pts',(59.2439820714187,-44.4186458955451,
0.));
#121840=CARTESIAN_POINT('Ctrl Pts',(59.2439820714187,-44.4186458955451,
12.));
#121841=CARTESIAN_POINT('Ctrl Pts',(59.2306526095131,-44.3947858914074,
0.));
#121842=CARTESIAN_POINT('Ctrl Pts',(59.2306526095131,-44.3947858914074,
12.));
#121843=CARTESIAN_POINT('Ctrl Pts',(59.2173188432798,-44.370969099747,0.));
#121844=CARTESIAN_POINT('Ctrl Pts',(59.2173188432798,-44.370969099747,12.));
#121845=CARTESIAN_POINT('Ctrl Pts',(59.2039808594752,-44.3471955758403,
0.));
#121846=CARTESIAN_POINT('Ctrl Pts',(59.2039808594752,-44.3471955758403,
12.));
#121847=CARTESIAN_POINT('Ctrl Pts',(59.1906387451979,-44.3234653750884,
0.));
#121848=CARTESIAN_POINT('Ctrl Pts',(59.1906387451979,-44.3234653750884,
12.));
#121849=CARTESIAN_POINT('Ctrl Pts',(59.1772925865213,-44.2997785523431,
0.));
#121850=CARTESIAN_POINT('Ctrl Pts',(59.1772925865213,-44.2997785523431,
12.));
#121851=CARTESIAN_POINT('Ctrl Pts',(59.1639424678793,-44.2761351616048,
0.));
#121852=CARTESIAN_POINT('Ctrl Pts',(59.1639424678793,-44.2761351616048,
12.));
#121853=CARTESIAN_POINT('Ctrl Pts',(59.1505884728215,-44.2525352563996,
0.));
#121854=CARTESIAN_POINT('Ctrl Pts',(59.1505884728215,-44.2525352563996,
12.));
#121855=CARTESIAN_POINT('Ctrl Pts',(59.1372306844585,-44.228978889997,0.));
#121856=CARTESIAN_POINT('Ctrl Pts',(59.1372306844585,-44.228978889997,12.));
#121857=CARTESIAN_POINT('Ctrl Pts',(59.1238691860306,-44.2054661156875,
0.));
#121858=CARTESIAN_POINT('Ctrl Pts',(59.1238691860306,-44.2054661156875,
12.));
#121859=CARTESIAN_POINT('Ctrl Pts',(59.1105040614275,-44.1819969870307,
0.));
#121860=CARTESIAN_POINT('Ctrl Pts',(59.1105040614275,-44.1819969870307,
12.));
#121861=CARTESIAN_POINT('Ctrl Pts',(59.0971353957206,-44.1585715581065,
0.));
#121862=CARTESIAN_POINT('Ctrl Pts',(59.0971353957206,-44.1585715581065,
12.));
#121863=CARTESIAN_POINT('Ctrl Pts',(59.08376327492,-44.1351898834051,0.));
#121864=CARTESIAN_POINT('Ctrl Pts',(59.08376327492,-44.1351898834051,12.));
#121865=CARTESIAN_POINT('Ctrl Pts',(59.0703877857525,-44.1118520177221,
0.));
#121866=CARTESIAN_POINT('Ctrl Pts',(59.0703877857525,-44.1118520177221,
12.));
#121867=CARTESIAN_POINT('Ctrl Pts',(59.0570090154242,-44.0885580160433,
0.));
#121868=CARTESIAN_POINT('Ctrl Pts',(59.0570090154242,-44.0885580160433,
12.));
#121869=CARTESIAN_POINT('Ctrl Pts',(59.0436270514086,-44.0653079334385,
0.));
#121870=CARTESIAN_POINT('Ctrl Pts',(59.0436270514086,-44.0653079334385,
12.));
#121871=CARTESIAN_POINT('Ctrl Pts',(59.0302419811777,-44.0421018249223,
0.));
#121872=CARTESIAN_POINT('Ctrl Pts',(59.0302419811777,-44.0421018249223,
12.));
#121873=CARTESIAN_POINT('Ctrl Pts',(59.0168538922095,-44.0189397454599,
0.));
#121874=CARTESIAN_POINT('Ctrl Pts',(59.0168538922095,-44.0189397454599,
12.));
#121875=CARTESIAN_POINT('Ctrl Pts',(59.0034628721167,-43.9958217500369,
0.));
#121876=CARTESIAN_POINT('Ctrl Pts',(59.0034628721167,-43.9958217500369,
12.));
#121877=CARTESIAN_POINT('Ctrl Pts',(58.9900690087408,-43.9727478937056,
0.));
#121878=CARTESIAN_POINT('Ctrl Pts',(58.9900690087408,-43.9727478937056,
12.));
#121879=CARTESIAN_POINT('Ctrl Pts',(58.9766723902529,-43.9497182316331,
0.));
#121880=CARTESIAN_POINT('Ctrl Pts',(58.9766723902529,-43.9497182316331,
12.));
#121881=CARTESIAN_POINT('Ctrl Pts',(58.9632731052696,-43.9267328191501,
0.));
#121882=CARTESIAN_POINT('Ctrl Pts',(58.9632731052696,-43.9267328191501,
12.));
#121883=CARTESIAN_POINT('Ctrl Pts',(58.9498712429054,-43.9037917117739,
0.));
#121884=CARTESIAN_POINT('Ctrl Pts',(58.9498712429054,-43.9037917117739,
12.));
#121885=CARTESIAN_POINT('Ctrl Pts',(58.936466892712,-43.8808949651873,0.));
#121886=CARTESIAN_POINT('Ctrl Pts',(58.936466892712,-43.8808949651873,12.));
#121887=CARTESIAN_POINT('Ctrl Pts',(58.9230601446436,-43.858042635223,0.));
#121888=CARTESIAN_POINT('Ctrl Pts',(58.9230601446436,-43.858042635223,12.));
#121889=CARTESIAN_POINT('Ctrl Pts',(58.9096510890129,-43.835234777842,0.));
#121890=CARTESIAN_POINT('Ctrl Pts',(58.9096510890129,-43.835234777842,12.));
#121891=CARTESIAN_POINT('Ctrl Pts',(58.8962398164493,-43.8124714491077,
0.));
#121892=CARTESIAN_POINT('Ctrl Pts',(58.8962398164493,-43.8124714491077,
12.));
#121893=CARTESIAN_POINT('Ctrl Pts',(58.8828264178621,-43.7897527051609,
0.));
#121894=CARTESIAN_POINT('Ctrl Pts',(58.8828264178621,-43.7897527051609,
12.));
#121895=CARTESIAN_POINT('Ctrl Pts',(58.8694109844647,-43.7670786022402,
0.));
#121896=CARTESIAN_POINT('Ctrl Pts',(58.8694109844647,-43.7670786022402,
12.));
#121897=CARTESIAN_POINT('Ctrl Pts',(58.855993607794,-43.7444491966942,0.));
#121898=CARTESIAN_POINT('Ctrl Pts',(58.855993607794,-43.7444491966942,12.));
#121899=CARTESIAN_POINT('Ctrl Pts',(58.8425743797326,-43.7218645449922,
0.));
#121900=CARTESIAN_POINT('Ctrl Pts',(58.8425743797326,-43.7218645449922,
12.));
#121901=CARTESIAN_POINT('Ctrl Pts',(58.8291533925293,-43.6993247037314,
0.));
#121902=CARTESIAN_POINT('Ctrl Pts',(58.8291533925293,-43.6993247037314,
12.));
#121903=CARTESIAN_POINT('Ctrl Pts',(58.8157307388238,-43.6768297296395,
0.));
#121904=CARTESIAN_POINT('Ctrl Pts',(58.8157307388238,-43.6768297296395,
12.));
#121905=CARTESIAN_POINT('Ctrl Pts',(58.8023065116436,-43.6543796795789,
0.));
#121906=CARTESIAN_POINT('Ctrl Pts',(58.8023065116436,-43.6543796795789,
12.));
#121907=CARTESIAN_POINT('Ctrl Pts',(58.788880804397,-43.6319746105482,0.));
#121908=CARTESIAN_POINT('Ctrl Pts',(58.788880804397,-43.6319746105482,12.));
#121909=CARTESIAN_POINT('Ctrl Pts',(58.775453710867,-43.6096145796797,0.));
#121910=CARTESIAN_POINT('Ctrl Pts',(58.775453710867,-43.6096145796797,12.));
#121911=CARTESIAN_POINT('Ctrl Pts',(58.7620253252062,-43.5872996442345,
0.));
#121912=CARTESIAN_POINT('Ctrl Pts',(58.7620253252062,-43.5872996442345,
12.));
#121913=CARTESIAN_POINT('Ctrl Pts',(58.74859574193,-43.5650298615917,0.));
#121914=CARTESIAN_POINT('Ctrl Pts',(58.74859574193,-43.5650298615917,12.));
#121915=CARTESIAN_POINT('Ctrl Pts',(58.735165055918,-43.5428052892488,0.));
#121916=CARTESIAN_POINT('Ctrl Pts',(58.735165055918,-43.5428052892488,12.));
#121917=CARTESIAN_POINT('Ctrl Pts',(58.7217333624209,-43.5206259848338,
0.));
#121918=CARTESIAN_POINT('Ctrl Pts',(58.7217333624209,-43.5206259848338,
12.));
#121919=CARTESIAN_POINT('Ctrl Pts',(58.7083007570661,-43.4984920061073,
0.));
#121920=CARTESIAN_POINT('Ctrl Pts',(58.7083007570661,-43.4984920061073,
12.));
#121921=CARTESIAN_POINT('Ctrl Pts',(58.6948673358638,-43.4764034109654,
0.));
#121922=CARTESIAN_POINT('Ctrl Pts',(58.6948673358638,-43.4764034109654,
12.));
#121923=CARTESIAN_POINT('Ctrl Pts',(58.6814331952138,-43.4543602574351,
0.));
#121924=CARTESIAN_POINT('Ctrl Pts',(58.6814331952138,-43.4543602574351,
12.));
#121925=CARTESIAN_POINT('Ctrl Pts',(58.6679984319097,-43.4323626036737,
0.));
#121926=CARTESIAN_POINT('Ctrl Pts',(58.6679984319097,-43.4323626036737,
12.));
#121927=CARTESIAN_POINT('Ctrl Pts',(58.6545631431393,-43.4104105079768,
0.));
#121928=CARTESIAN_POINT('Ctrl Pts',(58.6545631431393,-43.4104105079768,
12.));
#121929=CARTESIAN_POINT('Ctrl Pts',(58.6411274264857,-43.388504028781,0.));
#121930=CARTESIAN_POINT('Ctrl Pts',(58.6411274264857,-43.388504028781,12.));
#121931=CARTESIAN_POINT('Ctrl Pts',(58.627691379929,-43.3666432246635,0.));
#121932=CARTESIAN_POINT('Ctrl Pts',(58.627691379929,-43.3666432246635,12.));
#121933=CARTESIAN_POINT('Ctrl Pts',(58.6142551018467,-43.3448281543372,
0.));
#121934=CARTESIAN_POINT('Ctrl Pts',(58.6142551018467,-43.3448281543372,
12.));
#121935=CARTESIAN_POINT('Ctrl Pts',(58.6008186910156,-43.3230588766449,
0.));
#121936=CARTESIAN_POINT('Ctrl Pts',(58.6008186910156,-43.3230588766449,
12.));
#121937=CARTESIAN_POINT('Ctrl Pts',(58.5873822466152,-43.3013354505701,
0.));
#121938=CARTESIAN_POINT('Ctrl Pts',(58.5873822466152,-43.3013354505701,
12.));
#121939=CARTESIAN_POINT('Ctrl Pts',(58.573945868231,-43.2796579352401,0.));
#121940=CARTESIAN_POINT('Ctrl Pts',(58.573945868231,-43.2796579352401,12.));
#121941=CARTESIAN_POINT('Ctrl Pts',(58.5605096558578,-43.2580263899278,
0.));
#121942=CARTESIAN_POINT('Ctrl Pts',(58.5605096558578,-43.2580263899278,
12.));
#121943=CARTESIAN_POINT('Ctrl Pts',(58.5470737099032,-43.2364408740493,
0.));
#121944=CARTESIAN_POINT('Ctrl Pts',(58.5470737099032,-43.2364408740493,
12.));
#121945=CARTESIAN_POINT('Ctrl Pts',(58.5336381311917,-43.2149014471574,
0.));
#121946=CARTESIAN_POINT('Ctrl Pts',(58.5336381311917,-43.2149014471574,
12.));
#121947=CARTESIAN_POINT('Ctrl Pts',(58.5202030209669,-43.1934081689505,
0.));
#121948=CARTESIAN_POINT('Ctrl Pts',(58.5202030209669,-43.1934081689505,
12.));
#121949=CARTESIAN_POINT('Ctrl Pts',(58.5067684808944,-43.1719610992771,
0.));
#121950=CARTESIAN_POINT('Ctrl Pts',(58.5067684808944,-43.1719610992771,
12.));
#121951=CARTESIAN_POINT('Ctrl Pts',(58.4933346130636,-43.1505602981365,
0.));
#121952=CARTESIAN_POINT('Ctrl Pts',(58.4933346130636,-43.1505602981365,
12.));
#121953=CARTESIAN_POINT('Ctrl Pts',(58.4799015199907,-43.1292058256777,
0.));
#121954=CARTESIAN_POINT('Ctrl Pts',(58.4799015199907,-43.1292058256777,
12.));
#121955=CARTESIAN_POINT('Ctrl Pts',(58.4664693046217,-43.1078977421916,
0.));
#121956=CARTESIAN_POINT('Ctrl Pts',(58.4664693046217,-43.1078977421916,
12.));
#121957=CARTESIAN_POINT('Ctrl Pts',(58.4530380703348,-43.0866361081177,
0.));
#121958=CARTESIAN_POINT('Ctrl Pts',(58.4530380703348,-43.0866361081177,
12.));
#121959=CARTESIAN_POINT('Ctrl Pts',(58.439607920945,-43.0654209840511,0.));
#121960=CARTESIAN_POINT('Ctrl Pts',(58.439607920945,-43.0654209840511,12.));
#121961=CARTESIAN_POINT('Ctrl Pts',(58.4261789607058,-43.0442524307434,
0.));
#121962=CARTESIAN_POINT('Ctrl Pts',(58.4261789607058,-43.0442524307434,
12.));
#121963=CARTESIAN_POINT('Ctrl Pts',(58.4127512943136,-43.0231305091027,
0.));
#121964=CARTESIAN_POINT('Ctrl Pts',(58.4127512943136,-43.0231305091027,
12.));
#121965=CARTESIAN_POINT('Ctrl Pts',(58.3993250269101,-43.0020552801859,
0.));
#121966=CARTESIAN_POINT('Ctrl Pts',(58.3993250269101,-43.0020552801859,
12.));
#121967=CARTESIAN_POINT('Ctrl Pts',(58.3859002640856,-42.9810268052032,
0.));
#121968=CARTESIAN_POINT('Ctrl Pts',(58.3859002640856,-42.9810268052032,
12.));
#121969=CARTESIAN_POINT('Ctrl Pts',(58.3724771118826,-42.960045145526,0.));
#121970=CARTESIAN_POINT('Ctrl Pts',(58.3724771118826,-42.960045145526,12.));
#121971=CARTESIAN_POINT('Ctrl Pts',(58.3590556767978,-42.9391103626879,
0.));
#121972=CARTESIAN_POINT('Ctrl Pts',(58.3590556767978,-42.9391103626879,
12.));
#121973=CARTESIAN_POINT('Ctrl Pts',(58.3456360657865,-42.9182225183855,
0.));
#121974=CARTESIAN_POINT('Ctrl Pts',(58.3456360657865,-42.9182225183855,
12.));
#121975=CARTESIAN_POINT('Ctrl Pts',(58.3322183862654,-42.8973816744709,
0.));
#121976=CARTESIAN_POINT('Ctrl Pts',(58.3322183862654,-42.8973816744709,
12.));
#121977=CARTESIAN_POINT('Ctrl Pts',(58.3188027461164,-42.8765878929551,
0.));
#121978=CARTESIAN_POINT('Ctrl Pts',(58.3188027461164,-42.8765878929551,
12.));
#121979=CARTESIAN_POINT('Ctrl Pts',(58.3053892536894,-42.8558412360158,
0.));
#121980=CARTESIAN_POINT('Ctrl Pts',(58.3053892536894,-42.8558412360158,
12.));
#121981=CARTESIAN_POINT('Ctrl Pts',(58.2919780178064,-42.8351417659999,
0.));
#121982=CARTESIAN_POINT('Ctrl Pts',(58.2919780178064,-42.8351417659999,
12.));
#121983=CARTESIAN_POINT('Ctrl Pts',(58.2785691477638,-42.8144895454233,
0.));
#121984=CARTESIAN_POINT('Ctrl Pts',(58.2785691477638,-42.8144895454233,
12.));
#121985=CARTESIAN_POINT('Ctrl Pts',(58.2651627533368,-42.7938846369651,
0.));
#121986=CARTESIAN_POINT('Ctrl Pts',(58.2651627533368,-42.7938846369651,
12.));
#121987=CARTESIAN_POINT('Ctrl Pts',(58.251758944782,-42.773327103468,0.));
#121988=CARTESIAN_POINT('Ctrl Pts',(58.251758944782,-42.773327103468,12.));
#121989=CARTESIAN_POINT('Ctrl Pts',(58.2383578328424,-42.7528170079485,
0.));
#121990=CARTESIAN_POINT('Ctrl Pts',(58.2383578328424,-42.7528170079485,
12.));
#121991=CARTESIAN_POINT('Ctrl Pts',(58.22495952875,-42.7323544135985,0.));
#121992=CARTESIAN_POINT('Ctrl Pts',(58.22495952875,-42.7323544135985,12.));
#121993=CARTESIAN_POINT('Ctrl Pts',(58.21156414423,-42.7119393837866,0.));
#121994=CARTESIAN_POINT('Ctrl Pts',(58.21156414423,-42.7119393837866,12.));
#121995=CARTESIAN_POINT('Ctrl Pts',(58.1981717915037,-42.6915719820513,
0.));
#121996=CARTESIAN_POINT('Ctrl Pts',(58.1981717915037,-42.6915719820513,
12.));
#121997=CARTESIAN_POINT('Ctrl Pts',(58.1847825832923,-42.6712522721016,
0.));
#121998=CARTESIAN_POINT('Ctrl Pts',(58.1847825832923,-42.6712522721016,
12.));
#121999=CARTESIAN_POINT('Ctrl Pts',(58.171396632821,-42.6509803178265,0.));
#122000=CARTESIAN_POINT('Ctrl Pts',(58.171396632821,-42.6509803178265,12.));
#122001=CARTESIAN_POINT('Ctrl Pts',(58.1580140538228,-42.6307561832976,
0.));
#122002=CARTESIAN_POINT('Ctrl Pts',(58.1580140538228,-42.6307561832976,
12.));
#122003=CARTESIAN_POINT('Ctrl Pts',(58.1446349605421,-42.6105799327699,
0.));
#122004=CARTESIAN_POINT('Ctrl Pts',(58.1446349605421,-42.6105799327699,
12.));
#122005=CARTESIAN_POINT('Ctrl Pts',(58.1312594677386,-42.5904516306762,
0.));
#122006=CARTESIAN_POINT('Ctrl Pts',(58.1312594677386,-42.5904516306762,
12.));
#122007=CARTESIAN_POINT('Ctrl Pts',(58.1178876906907,-42.5703713416265,
0.));
#122008=CARTESIAN_POINT('Ctrl Pts',(58.1178876906907,-42.5703713416265,
12.));
#122009=CARTESIAN_POINT('Ctrl Pts',(58.1045197452002,-42.5503391304183,
0.));
#122010=CARTESIAN_POINT('Ctrl Pts',(58.1045197452002,-42.5503391304183,
12.));
#122011=CARTESIAN_POINT('Ctrl Pts',(58.0911557475965,-42.5303550620387,
0.));
#122012=CARTESIAN_POINT('Ctrl Pts',(58.0911557475965,-42.5303550620387,
12.));
#122013=CARTESIAN_POINT('Ctrl Pts',(58.0777958147403,-42.5104192016664,
0.));
#122014=CARTESIAN_POINT('Ctrl Pts',(58.0777958147403,-42.5104192016664,
12.));
#122015=CARTESIAN_POINT('Ctrl Pts',(58.0644400640275,-42.4905316146654,
0.));
#122016=CARTESIAN_POINT('Ctrl Pts',(58.0644400640275,-42.4905316146654,
12.));
#122017=CARTESIAN_POINT('Ctrl Pts',(58.0510886133926,-42.4706923665845,
0.));
#122018=CARTESIAN_POINT('Ctrl Pts',(58.0510886133926,-42.4706923665845,
12.));
#122019=CARTESIAN_POINT('Ctrl Pts',(58.037741581314,-42.4509015231674,0.));
#122020=CARTESIAN_POINT('Ctrl Pts',(58.037741581314,-42.4509015231674,12.));
#122021=CARTESIAN_POINT('Ctrl Pts',(58.0243990868181,-42.4311591503555,
0.));
#122022=CARTESIAN_POINT('Ctrl Pts',(58.0243990868181,-42.4311591503555,
12.));
#122023=CARTESIAN_POINT('Ctrl Pts',(58.0110612494828,-42.411465314289,0.));
#122024=CARTESIAN_POINT('Ctrl Pts',(58.0110612494828,-42.411465314289,12.));
#122025=CARTESIAN_POINT('Ctrl Pts',(57.9977281894422,-42.3918200813014,
0.));
#122026=CARTESIAN_POINT('Ctrl Pts',(57.9977281894422,-42.3918200813014,
12.));
#122027=CARTESIAN_POINT('Ctrl Pts',(57.9844000273911,-42.3722235179198,
0.));
#122028=CARTESIAN_POINT('Ctrl Pts',(57.9844000273911,-42.3722235179198,
12.));
#122029=CARTESIAN_POINT('Ctrl Pts',(57.9710768845899,-42.3526756908747,
0.));
#122030=CARTESIAN_POINT('Ctrl Pts',(57.9710768845899,-42.3526756908747,
12.));
#122031=CARTESIAN_POINT('Ctrl Pts',(57.9577588828682,-42.333176667102,0.));
#122032=CARTESIAN_POINT('Ctrl Pts',(57.9577588828682,-42.333176667102,12.));
#122033=CARTESIAN_POINT('Ctrl Pts',(57.9444461446299,-42.3137265137452,
0.));
#122034=CARTESIAN_POINT('Ctrl Pts',(57.9444461446299,-42.3137265137452,
12.));
#122035=CARTESIAN_POINT('Ctrl Pts',(57.9311387928563,-42.2943252981489,
0.));
#122036=CARTESIAN_POINT('Ctrl Pts',(57.9311387928563,-42.2943252981489,
12.));
#122037=CARTESIAN_POINT('Ctrl Pts',(57.9178369511114,-42.2749730878595,
0.));
#122038=CARTESIAN_POINT('Ctrl Pts',(57.9178369511114,-42.2749730878595,
12.));
#122039=CARTESIAN_POINT('Ctrl Pts',(57.9045407435474,-42.2556699506353,
0.));
#122040=CARTESIAN_POINT('Ctrl Pts',(57.9045407435474,-42.2556699506353,
12.));
#122041=CARTESIAN_POINT('Ctrl Pts',(57.8912502949096,-42.2364159544501,
0.));
#122042=CARTESIAN_POINT('Ctrl Pts',(57.8912502949096,-42.2364159544501,
12.));
#122043=CARTESIAN_POINT('Ctrl Pts',(57.8779657305413,-42.2172111674938,
0.));
#122044=CARTESIAN_POINT('Ctrl Pts',(57.8779657305413,-42.2172111674938,
12.));
#122045=CARTESIAN_POINT('Ctrl Pts',(57.864687176387,-42.1980556581665,0.));
#122046=CARTESIAN_POINT('Ctrl Pts',(57.864687176387,-42.1980556581665,12.));
#122047=CARTESIAN_POINT('Ctrl Pts',(57.8514147589972,-42.1789494950794,
0.));
#122048=CARTESIAN_POINT('Ctrl Pts',(57.8514147589972,-42.1789494950794,
12.));
#122049=CARTESIAN_POINT('Ctrl Pts',(57.8381486055342,-42.1598927470646,
0.));
#122050=CARTESIAN_POINT('Ctrl Pts',(57.8381486055342,-42.1598927470646,
12.));
#122051=CARTESIAN_POINT('Ctrl Pts',(57.8248888437775,-42.1408854831783,
0.));
#122052=CARTESIAN_POINT('Ctrl Pts',(57.8248888437775,-42.1408854831783,
12.));
#122053=CARTESIAN_POINT('Ctrl Pts',(57.8116356021288,-42.1219277727021,
0.));
#122054=CARTESIAN_POINT('Ctrl Pts',(57.8116356021288,-42.1219277727021,
12.));
#122055=CARTESIAN_POINT('Ctrl Pts',(57.798389009616,-42.1030196851366,0.));
#122056=CARTESIAN_POINT('Ctrl Pts',(57.798389009616,-42.1030196851366,12.));
#122057=CARTESIAN_POINT('Ctrl Pts',(57.7851491958987,-42.0841612902042,
0.));
#122058=CARTESIAN_POINT('Ctrl Pts',(57.7851491958987,-42.0841612902042,
12.));
#122059=CARTESIAN_POINT('Ctrl Pts',(57.7719162912744,-42.0653526578588,
0.));
#122060=CARTESIAN_POINT('Ctrl Pts',(57.7719162912744,-42.0653526578588,
12.));
#122061=CARTESIAN_POINT('Ctrl Pts',(57.7586904266834,-42.0465938582882,
0.));
#122062=CARTESIAN_POINT('Ctrl Pts',(57.7586904266834,-42.0465938582882,
12.));
#122063=CARTESIAN_POINT('Ctrl Pts',(57.745471733714,-42.0278849619148,0.));
#122064=CARTESIAN_POINT('Ctrl Pts',(57.745471733714,-42.0278849619148,12.));
#122065=CARTESIAN_POINT('Ctrl Pts',(57.7322603446066,-42.0092260393897,
0.));
#122066=CARTESIAN_POINT('Ctrl Pts',(57.7322603446066,-42.0092260393897,
12.));
#122067=CARTESIAN_POINT('Ctrl Pts',(57.7190563922593,-41.990617161596,0.));
#122068=CARTESIAN_POINT('Ctrl Pts',(57.7190563922593,-41.990617161596,12.));
#122069=CARTESIAN_POINT('Ctrl Pts',(57.7058600102351,-41.9720583996592,
0.));
#122070=CARTESIAN_POINT('Ctrl Pts',(57.7058600102351,-41.9720583996592,
12.));
#122071=CARTESIAN_POINT('Ctrl Pts',(57.6926713327672,-41.9535498249488,
0.));
#122072=CARTESIAN_POINT('Ctrl Pts',(57.6926713327672,-41.9535498249488,
12.));
#122073=CARTESIAN_POINT('Ctrl Pts',(57.6794904947649,-41.9350915090797,
0.));
#122074=CARTESIAN_POINT('Ctrl Pts',(57.6794904947649,-41.9350915090797,
12.));
#122075=CARTESIAN_POINT('Ctrl Pts',(57.6663176318189,-41.9166835239054,
0.));
#122076=CARTESIAN_POINT('Ctrl Pts',(57.6663176318189,-41.9166835239054,
12.));
#122077=CARTESIAN_POINT('Ctrl Pts',(57.6531528802072,-41.8983259415253,
0.));
#122078=CARTESIAN_POINT('Ctrl Pts',(57.6531528802072,-41.8983259415253,
12.));
#122079=CARTESIAN_POINT('Ctrl Pts',(57.6399963769009,-41.8800188342912,
0.));
#122080=CARTESIAN_POINT('Ctrl Pts',(57.6399963769009,-41.8800188342912,
12.));
#122081=CARTESIAN_POINT('Ctrl Pts',(57.6268482595701,-41.8617622748107,
0.));
#122082=CARTESIAN_POINT('Ctrl Pts',(57.6268482595701,-41.8617622748107,
12.));
#122083=CARTESIAN_POINT('Ctrl Pts',(57.613708666588,-41.8435563359456,0.));
#122084=CARTESIAN_POINT('Ctrl Pts',(57.613708666588,-41.8435563359456,12.));
#122085=CARTESIAN_POINT('Ctrl Pts',(57.6005777370347,-41.8254010908051,
0.));
#122086=CARTESIAN_POINT('Ctrl Pts',(57.6005777370347,-41.8254010908051,
12.));
#122087=CARTESIAN_POINT('Ctrl Pts',(57.5874556107054,-41.8072966127559,
0.));
#122088=CARTESIAN_POINT('Ctrl Pts',(57.5874556107054,-41.8072966127559,
12.));
#122089=CARTESIAN_POINT('Ctrl Pts',(57.5743424281204,-41.7892429754298,
0.));
#122090=CARTESIAN_POINT('Ctrl Pts',(57.5743424281204,-41.7892429754298,
12.));
#122091=CARTESIAN_POINT('Ctrl Pts',(57.561238330532,-41.7712402527273,0.));
#122092=CARTESIAN_POINT('Ctrl Pts',(57.561238330532,-41.7712402527273,12.));
#122093=CARTESIAN_POINT('Ctrl Pts',(57.5481434599334,-41.7532885188174,
0.));
#122094=CARTESIAN_POINT('Ctrl Pts',(57.5481434599334,-41.7532885188174,
12.));
#122095=CARTESIAN_POINT('Ctrl Pts',(57.5350579590648,-41.7353878481336,
0.));
#122096=CARTESIAN_POINT('Ctrl Pts',(57.5350579590648,-41.7353878481336,
12.));
#122097=CARTESIAN_POINT('Ctrl Pts',(57.5219819714169,-41.7175383153819,
0.));
#122098=CARTESIAN_POINT('Ctrl Pts',(57.5219819714169,-41.7175383153819,
12.));
#122099=CARTESIAN_POINT('Ctrl Pts',(57.5089156412341,-41.6997399955445,
0.));
#122100=CARTESIAN_POINT('Ctrl Pts',(57.5089156412341,-41.6997399955445,
12.));
#122101=CARTESIAN_POINT('Ctrl Pts',(57.4958591135165,-41.6819929638797,
0.));
#122102=CARTESIAN_POINT('Ctrl Pts',(57.4958591135165,-41.6819929638797,
12.));
#122103=CARTESIAN_POINT('Ctrl Pts',(57.4828125340222,-41.6642972959168,
0.));
#122104=CARTESIAN_POINT('Ctrl Pts',(57.4828125340222,-41.6642972959168,
12.));
#122105=CARTESIAN_POINT('Ctrl Pts',(57.4697760492693,-41.6466530674522,
0.));
#122106=CARTESIAN_POINT('Ctrl Pts',(57.4697760492693,-41.6466530674522,
12.));
#122107=CARTESIAN_POINT('Ctrl Pts',(57.4567498065573,-41.6290603545674,
0.));
#122108=CARTESIAN_POINT('Ctrl Pts',(57.4567498065573,-41.6290603545674,
12.));
#122109=CARTESIAN_POINT('Ctrl Pts',(57.4437339539848,-41.6115192336394,
0.));
#122110=CARTESIAN_POINT('Ctrl Pts',(57.4437339539848,-41.6115192336394,
12.));
#122111=CARTESIAN_POINT('Ctrl Pts',(57.4307286404656,-41.5940297813474,
0.));
#122112=CARTESIAN_POINT('Ctrl Pts',(57.4307286404656,-41.5940297813474,
12.));
#122113=CARTESIAN_POINT('Ctrl Pts',(57.417734015749,-41.5765920746764,0.));
#122114=CARTESIAN_POINT('Ctrl Pts',(57.417734015749,-41.5765920746764,12.));
#122115=CARTESIAN_POINT('Ctrl Pts',(57.4047502304207,-41.5592061909159,
0.));
#122116=CARTESIAN_POINT('Ctrl Pts',(57.4047502304207,-41.5592061909159,
12.));
#122117=CARTESIAN_POINT('Ctrl Pts',(57.3917774358844,-41.5418722076558,
0.));
#122118=CARTESIAN_POINT('Ctrl Pts',(57.3917774358844,-41.5418722076558,
12.));
#122119=CARTESIAN_POINT('Ctrl Pts',(57.378815784345,-41.5245902027767,0.));
#122120=CARTESIAN_POINT('Ctrl Pts',(57.378815784345,-41.5245902027767,12.));
#122121=CARTESIAN_POINT('Ctrl Pts',(57.3658654287948,-41.5073602544404,
0.));
#122122=CARTESIAN_POINT('Ctrl Pts',(57.3658654287948,-41.5073602544404,
12.));
#122123=CARTESIAN_POINT('Ctrl Pts',(57.3529265229858,-41.4901824410654,
0.));
#122124=CARTESIAN_POINT('Ctrl Pts',(57.3529265229858,-41.4901824410654,
12.));
#122125=CARTESIAN_POINT('Ctrl Pts',(57.339999221474,-41.4730568413535,0.));
#122126=CARTESIAN_POINT('Ctrl Pts',(57.339999221474,-41.4730568413535,12.));
#122127=CARTESIAN_POINT('Ctrl Pts',(57.3270836796925,-41.4559835343339,
0.));
#122128=CARTESIAN_POINT('Ctrl Pts',(57.3270836796925,-41.4559835343339,
12.));
#122129=CARTESIAN_POINT('Ctrl Pts',(57.3141800540137,-41.4389625993948,
0.));
#122130=CARTESIAN_POINT('Ctrl Pts',(57.3141800540137,-41.4389625993948,
12.));
#122131=CARTESIAN_POINT('Ctrl Pts',(57.3012885018139,-41.4219941163155,
0.));
#122132=CARTESIAN_POINT('Ctrl Pts',(57.3012885018139,-41.4219941163155,
12.));
#122133=CARTESIAN_POINT('Ctrl Pts',(57.2884091815384,-41.4050781652923,
0.));
#122134=CARTESIAN_POINT('Ctrl Pts',(57.2884091815384,-41.4050781652923,
12.));
#122135=CARTESIAN_POINT('Ctrl Pts',(57.2755422525822,-41.3882148268798,
0.));
#122136=CARTESIAN_POINT('Ctrl Pts',(57.2755422525822,-41.3882148268798,
12.));
#122137=CARTESIAN_POINT('Ctrl Pts',(57.2626878751584,-41.3714041819215,
0.));
#122138=CARTESIAN_POINT('Ctrl Pts',(57.2626878751584,-41.3714041819215,
12.));
#122139=CARTESIAN_POINT('Ctrl Pts',(57.2498462101883,-41.3546463114889,
0.));
#122140=CARTESIAN_POINT('Ctrl Pts',(57.2498462101883,-41.3546463114889,
12.));
#122141=CARTESIAN_POINT('Ctrl Pts',(57.237017419142,-41.3379412967889,0.));
#122142=CARTESIAN_POINT('Ctrl Pts',(57.237017419142,-41.3379412967889,12.));
#122143=CARTESIAN_POINT('Ctrl Pts',(57.2242016640226,-41.321289219151,0.));
#122144=CARTESIAN_POINT('Ctrl Pts',(57.2242016640226,-41.321289219151,12.));
#122145=CARTESIAN_POINT('Ctrl Pts',(57.2113991077325,-41.304690160231,0.));
#122146=CARTESIAN_POINT('Ctrl Pts',(57.2113991077325,-41.304690160231,12.));
#122147=CARTESIAN_POINT('Ctrl Pts',(57.1986099143992,-41.288144202187,0.));
#122148=CARTESIAN_POINT('Ctrl Pts',(57.1986099143992,-41.288144202187,12.));
#122149=CARTESIAN_POINT('Ctrl Pts',(57.1858342496526,-41.2716514278268,
0.));
#122150=CARTESIAN_POINT('Ctrl Pts',(57.1858342496526,-41.2716514278268,
12.));
#122151=CARTESIAN_POINT('Ctrl Pts',(57.1730722810771,-41.2552119208445,
0.));
#122152=CARTESIAN_POINT('Ctrl Pts',(57.1730722810771,-41.2552119208445,
12.));
#122153=CARTESIAN_POINT('Ctrl Pts',(57.1603241779042,-41.2388257656534,
0.));
#122154=CARTESIAN_POINT('Ctrl Pts',(57.1603241779042,-41.2388257656534,
12.));
#122155=CARTESIAN_POINT('Ctrl Pts',(57.1475901101794,-41.2224930469412,
0.));
#122156=CARTESIAN_POINT('Ctrl Pts',(57.1475901101794,-41.2224930469412,
12.));
#122157=CARTESIAN_POINT('Ctrl Pts',(57.1348702480644,-41.2062138492913,
0.));
#122158=CARTESIAN_POINT('Ctrl Pts',(57.1348702480644,-41.2062138492913,
12.));
#122159=CARTESIAN_POINT('Ctrl Pts',(57.1221647611231,-41.1899882567941,
0.));
#122160=CARTESIAN_POINT('Ctrl Pts',(57.1221647611231,-41.1899882567941,
12.));
#122161=CARTESIAN_POINT('Ctrl Pts',(57.1094738174998,-41.1738163525932,
0.));
#122162=CARTESIAN_POINT('Ctrl Pts',(57.1094738174998,-41.1738163525932,
12.));
#122163=CARTESIAN_POINT('Ctrl Pts',(57.0967975854912,-41.1576982197403,
0.));
#122164=CARTESIAN_POINT('Ctrl Pts',(57.0967975854912,-41.1576982197403,
12.));
#122165=CARTESIAN_POINT('Ctrl Pts',(57.084136235428,-41.1416339422132,0.));
#122166=CARTESIAN_POINT('Ctrl Pts',(57.084136235428,-41.1416339422132,12.));
#122167=CARTESIAN_POINT('Ctrl Pts',(57.0714899412091,-41.1256236057437,
0.));
#122168=CARTESIAN_POINT('Ctrl Pts',(57.0714899412091,-41.1256236057437,
12.));
#122169=CARTESIAN_POINT('Ctrl Pts',(57.0588588825266,-41.1096672990125,
0.));
#122170=CARTESIAN_POINT('Ctrl Pts',(57.0588588825266,-41.1096672990125,
12.));
#122171=CARTESIAN_POINT('Ctrl Pts',(57.0462432450637,-41.093765113752,0.));
#122172=CARTESIAN_POINT('Ctrl Pts',(57.0462432450637,-41.093765113752,12.));
#122173=CARTESIAN_POINT('Ctrl Pts',(57.0336432158503,-41.0779171422415,
0.));
#122174=CARTESIAN_POINT('Ctrl Pts',(57.0336432158503,-41.0779171422415,
12.));
#122175=CARTESIAN_POINT('Ctrl Pts',(57.0210589791777,-41.0621234751,0.));
#122176=CARTESIAN_POINT('Ctrl Pts',(57.0210589791777,-41.0621234751,12.));
#122177=CARTESIAN_POINT('Ctrl Pts',(57.008490713044,-41.0463841993622,0.));
#122178=CARTESIAN_POINT('Ctrl Pts',(57.008490713044,-41.0463841993622,12.));
#122179=CARTESIAN_POINT('Ctrl Pts',(56.9959385834768,-41.0306993954021,
0.));
#122180=CARTESIAN_POINT('Ctrl Pts',(56.9959385834768,-41.0306993954021,
12.));
#122181=CARTESIAN_POINT('Ctrl Pts',(56.9834027500178,-41.0150691398988,
0.));
#122182=CARTESIAN_POINT('Ctrl Pts',(56.9834027500178,-41.0150691398988,
12.));
#122183=CARTESIAN_POINT('Ctrl Pts',(56.9708833766183,-40.9994935117307,
0.));
#122184=CARTESIAN_POINT('Ctrl Pts',(56.9708833766183,-40.9994935117307,
12.));
#122185=CARTESIAN_POINT('Ctrl Pts',(56.9583806404069,-40.9839725967121,
0.));
#122186=CARTESIAN_POINT('Ctrl Pts',(56.9583806404069,-40.9839725967121,
12.));
#122187=CARTESIAN_POINT('Ctrl Pts',(56.9458947422541,-40.968506493303,0.));
#122188=CARTESIAN_POINT('Ctrl Pts',(56.9458947422541,-40.968506493303,12.));
#122189=CARTESIAN_POINT('Ctrl Pts',(56.9334259139928,-40.9530953164952,
0.));
#122190=CARTESIAN_POINT('Ctrl Pts',(56.9334259139928,-40.9530953164952,
12.));
#122191=CARTESIAN_POINT('Ctrl Pts',(56.9209743960861,-40.9377391857044,
0.));
#122192=CARTESIAN_POINT('Ctrl Pts',(56.9209743960861,-40.9377391857044,
12.));
#122193=CARTESIAN_POINT('Ctrl Pts',(56.9085404164432,-40.9224382132382,
0.));
#122194=CARTESIAN_POINT('Ctrl Pts',(56.9085404164432,-40.9224382132382,
12.));
#122195=CARTESIAN_POINT('Ctrl Pts',(56.8961241708926,-40.9071924937551,
0.));
#122196=CARTESIAN_POINT('Ctrl Pts',(56.8961241708926,-40.9071924937551,
12.));
#122197=CARTESIAN_POINT('Ctrl Pts',(56.8837257978574,-40.8920020903443,
0.));
#122198=CARTESIAN_POINT('Ctrl Pts',(56.8837257978574,-40.8920020903443,
12.));
#122199=CARTESIAN_POINT('Ctrl Pts',(56.8713453765252,-40.8768670342278,
0.));
#122200=CARTESIAN_POINT('Ctrl Pts',(56.8713453765252,-40.8768670342278,
12.));
#122201=CARTESIAN_POINT('Ctrl Pts',(56.8614554317993,-40.8648032759631,
0.));
#122202=CARTESIAN_POINT('Ctrl Pts',(56.8614554317993,-40.8648032759631,
12.));
#122203=CARTESIAN_POINT('Ctrl Pts',(56.8540460739677,-40.8557803680412,
0.));
#122204=CARTESIAN_POINT('Ctrl Pts',(56.8540460739677,-40.8557803680412,
12.));
#122205=CARTESIAN_POINT('Ctrl Pts',(56.8491101022668,-40.8497761671086,
0.));
#122206=CARTESIAN_POINT('Ctrl Pts',(56.8491101022668,-40.8497761671086,
12.));
#122207=CARTESIAN_POINT('Ctrl Pts',(56.8466430164621,-40.8467768343957,
0.));
#122208=CARTESIAN_POINT('Ctrl Pts',(56.8466430164621,-40.8467768343957,
12.));
#122209=CARTESIAN_POINT('',(56.8466430164621,-40.8467768343957,12.));
#122210=CARTESIAN_POINT('Ctrl Pts',(56.8466430164621,-40.8467768343957,
12.));
#122211=CARTESIAN_POINT('Ctrl Pts',(56.8491101022668,-40.8497761671086,
12.));
#122212=CARTESIAN_POINT('Ctrl Pts',(56.8540460739677,-40.8557803680412,
12.));
#122213=CARTESIAN_POINT('Ctrl Pts',(56.8614554317993,-40.8648032759631,
12.));
#122214=CARTESIAN_POINT('Ctrl Pts',(56.8713453765252,-40.8768670342278,
12.));
#122215=CARTESIAN_POINT('Ctrl Pts',(56.8837257978574,-40.8920020903443,
12.));
#122216=CARTESIAN_POINT('Ctrl Pts',(56.8961241708926,-40.9071924937551,
12.));
#122217=CARTESIAN_POINT('Ctrl Pts',(56.9085404164432,-40.9224382132382,
12.));
#122218=CARTESIAN_POINT('Ctrl Pts',(56.9209743960861,-40.9377391857044,
12.));
#122219=CARTESIAN_POINT('Ctrl Pts',(56.9334259139928,-40.9530953164952,
12.));
#122220=CARTESIAN_POINT('Ctrl Pts',(56.9458947422541,-40.968506493303,12.));
#122221=CARTESIAN_POINT('Ctrl Pts',(56.9583806404069,-40.9839725967121,
12.));
#122222=CARTESIAN_POINT('Ctrl Pts',(56.9708833766183,-40.9994935117307,
12.));
#122223=CARTESIAN_POINT('Ctrl Pts',(56.9834027500178,-41.0150691398988,
12.));
#122224=CARTESIAN_POINT('Ctrl Pts',(56.9959385834768,-41.0306993954021,
12.));
#122225=CARTESIAN_POINT('Ctrl Pts',(57.008490713044,-41.0463841993622,12.));
#122226=CARTESIAN_POINT('Ctrl Pts',(57.0210589791777,-41.0621234751,12.));
#122227=CARTESIAN_POINT('Ctrl Pts',(57.0336432158503,-41.0779171422415,
12.));
#122228=CARTESIAN_POINT('Ctrl Pts',(57.0462432450637,-41.093765113752,12.));
#122229=CARTESIAN_POINT('Ctrl Pts',(57.0588588825266,-41.1096672990125,
12.));
#122230=CARTESIAN_POINT('Ctrl Pts',(57.0714899412091,-41.1256236057437,
12.));
#122231=CARTESIAN_POINT('Ctrl Pts',(57.084136235428,-41.1416339422132,12.));
#122232=CARTESIAN_POINT('Ctrl Pts',(57.0967975854912,-41.1576982197403,
12.));
#122233=CARTESIAN_POINT('Ctrl Pts',(57.1094738174998,-41.1738163525932,
12.));
#122234=CARTESIAN_POINT('Ctrl Pts',(57.1221647611231,-41.1899882567941,
12.));
#122235=CARTESIAN_POINT('Ctrl Pts',(57.1348702480644,-41.2062138492913,
12.));
#122236=CARTESIAN_POINT('Ctrl Pts',(57.1475901101794,-41.2224930469412,
12.));
#122237=CARTESIAN_POINT('Ctrl Pts',(57.1603241779042,-41.2388257656534,
12.));
#122238=CARTESIAN_POINT('Ctrl Pts',(57.1730722810771,-41.2552119208445,
12.));
#122239=CARTESIAN_POINT('Ctrl Pts',(57.1858342496526,-41.2716514278268,
12.));
#122240=CARTESIAN_POINT('Ctrl Pts',(57.1986099143992,-41.288144202187,12.));
#122241=CARTESIAN_POINT('Ctrl Pts',(57.2113991077325,-41.304690160231,12.));
#122242=CARTESIAN_POINT('Ctrl Pts',(57.2242016640226,-41.321289219151,12.));
#122243=CARTESIAN_POINT('Ctrl Pts',(57.237017419142,-41.3379412967889,12.));
#122244=CARTESIAN_POINT('Ctrl Pts',(57.2498462101883,-41.3546463114889,
12.));
#122245=CARTESIAN_POINT('Ctrl Pts',(57.2626878751584,-41.3714041819215,
12.));
#122246=CARTESIAN_POINT('Ctrl Pts',(57.2755422525822,-41.3882148268798,
12.));
#122247=CARTESIAN_POINT('Ctrl Pts',(57.2884091815384,-41.4050781652923,
12.));
#122248=CARTESIAN_POINT('Ctrl Pts',(57.3012885018139,-41.4219941163155,
12.));
#122249=CARTESIAN_POINT('Ctrl Pts',(57.3141800540137,-41.4389625993948,
12.));
#122250=CARTESIAN_POINT('Ctrl Pts',(57.3270836796925,-41.4559835343339,
12.));
#122251=CARTESIAN_POINT('Ctrl Pts',(57.339999221474,-41.4730568413535,12.));
#122252=CARTESIAN_POINT('Ctrl Pts',(57.3529265229858,-41.4901824410654,
12.));
#122253=CARTESIAN_POINT('Ctrl Pts',(57.3658654287948,-41.5073602544404,
12.));
#122254=CARTESIAN_POINT('Ctrl Pts',(57.378815784345,-41.5245902027767,12.));
#122255=CARTESIAN_POINT('Ctrl Pts',(57.3917774358844,-41.5418722076558,
12.));
#122256=CARTESIAN_POINT('Ctrl Pts',(57.4047502304207,-41.5592061909159,
12.));
#122257=CARTESIAN_POINT('Ctrl Pts',(57.417734015749,-41.5765920746764,12.));
#122258=CARTESIAN_POINT('Ctrl Pts',(57.4307286404656,-41.5940297813474,
12.));
#122259=CARTESIAN_POINT('Ctrl Pts',(57.4437339539848,-41.6115192336394,
12.));
#122260=CARTESIAN_POINT('Ctrl Pts',(57.4567498065573,-41.6290603545674,
12.));
#122261=CARTESIAN_POINT('Ctrl Pts',(57.4697760492693,-41.6466530674522,
12.));
#122262=CARTESIAN_POINT('Ctrl Pts',(57.4828125340222,-41.6642972959168,
12.));
#122263=CARTESIAN_POINT('Ctrl Pts',(57.4958591135165,-41.6819929638797,
12.));
#122264=CARTESIAN_POINT('Ctrl Pts',(57.5089156412341,-41.6997399955445,
12.));
#122265=CARTESIAN_POINT('Ctrl Pts',(57.5219819714169,-41.7175383153819,
12.));
#122266=CARTESIAN_POINT('Ctrl Pts',(57.5350579590648,-41.7353878481336,
12.));
#122267=CARTESIAN_POINT('Ctrl Pts',(57.5481434599334,-41.7532885188174,
12.));
#122268=CARTESIAN_POINT('Ctrl Pts',(57.561238330532,-41.7712402527273,12.));
#122269=CARTESIAN_POINT('Ctrl Pts',(57.5743424281204,-41.7892429754298,
12.));
#122270=CARTESIAN_POINT('Ctrl Pts',(57.5874556107054,-41.8072966127559,
12.));
#122271=CARTESIAN_POINT('Ctrl Pts',(57.6005777370347,-41.8254010908051,
12.));
#122272=CARTESIAN_POINT('Ctrl Pts',(57.613708666588,-41.8435563359456,12.));
#122273=CARTESIAN_POINT('Ctrl Pts',(57.6268482595701,-41.8617622748107,
12.));
#122274=CARTESIAN_POINT('Ctrl Pts',(57.6399963769009,-41.8800188342912,
12.));
#122275=CARTESIAN_POINT('Ctrl Pts',(57.6531528802072,-41.8983259415253,
12.));
#122276=CARTESIAN_POINT('Ctrl Pts',(57.6663176318189,-41.9166835239054,
12.));
#122277=CARTESIAN_POINT('Ctrl Pts',(57.6794904947649,-41.9350915090797,
12.));
#122278=CARTESIAN_POINT('Ctrl Pts',(57.6926713327672,-41.9535498249488,
12.));
#122279=CARTESIAN_POINT('Ctrl Pts',(57.7058600102351,-41.9720583996592,
12.));
#122280=CARTESIAN_POINT('Ctrl Pts',(57.7190563922593,-41.990617161596,12.));
#122281=CARTESIAN_POINT('Ctrl Pts',(57.7322603446066,-42.0092260393897,
12.));
#122282=CARTESIAN_POINT('Ctrl Pts',(57.745471733714,-42.0278849619148,12.));
#122283=CARTESIAN_POINT('Ctrl Pts',(57.7586904266834,-42.0465938582882,
12.));
#122284=CARTESIAN_POINT('Ctrl Pts',(57.7719162912744,-42.0653526578588,
12.));
#122285=CARTESIAN_POINT('Ctrl Pts',(57.7851491958987,-42.0841612902042,
12.));
#122286=CARTESIAN_POINT('Ctrl Pts',(57.798389009616,-42.1030196851366,12.));
#122287=CARTESIAN_POINT('Ctrl Pts',(57.8116356021288,-42.1219277727021,
12.));
#122288=CARTESIAN_POINT('Ctrl Pts',(57.8248888437775,-42.1408854831783,
12.));
#122289=CARTESIAN_POINT('Ctrl Pts',(57.8381486055342,-42.1598927470646,
12.));
#122290=CARTESIAN_POINT('Ctrl Pts',(57.8514147589972,-42.1789494950794,
12.));
#122291=CARTESIAN_POINT('Ctrl Pts',(57.864687176387,-42.1980556581665,12.));
#122292=CARTESIAN_POINT('Ctrl Pts',(57.8779657305413,-42.2172111674938,
12.));
#122293=CARTESIAN_POINT('Ctrl Pts',(57.8912502949096,-42.2364159544501,
12.));
#122294=CARTESIAN_POINT('Ctrl Pts',(57.9045407435474,-42.2556699506353,
12.));
#122295=CARTESIAN_POINT('Ctrl Pts',(57.9178369511114,-42.2749730878595,
12.));
#122296=CARTESIAN_POINT('Ctrl Pts',(57.9311387928563,-42.2943252981489,
12.));
#122297=CARTESIAN_POINT('Ctrl Pts',(57.9444461446299,-42.3137265137452,
12.));
#122298=CARTESIAN_POINT('Ctrl Pts',(57.9577588828682,-42.333176667102,12.));
#122299=CARTESIAN_POINT('Ctrl Pts',(57.9710768845899,-42.3526756908747,
12.));
#122300=CARTESIAN_POINT('Ctrl Pts',(57.9844000273911,-42.3722235179198,
12.));
#122301=CARTESIAN_POINT('Ctrl Pts',(57.9977281894422,-42.3918200813014,
12.));
#122302=CARTESIAN_POINT('Ctrl Pts',(58.0110612494828,-42.411465314289,12.));
#122303=CARTESIAN_POINT('Ctrl Pts',(58.0243990868181,-42.4311591503555,
12.));
#122304=CARTESIAN_POINT('Ctrl Pts',(58.037741581314,-42.4509015231674,12.));
#122305=CARTESIAN_POINT('Ctrl Pts',(58.0510886133926,-42.4706923665845,
12.));
#122306=CARTESIAN_POINT('Ctrl Pts',(58.0644400640275,-42.4905316146654,
12.));
#122307=CARTESIAN_POINT('Ctrl Pts',(58.0777958147403,-42.5104192016664,
12.));
#122308=CARTESIAN_POINT('Ctrl Pts',(58.0911557475965,-42.5303550620387,
12.));
#122309=CARTESIAN_POINT('Ctrl Pts',(58.1045197452002,-42.5503391304183,
12.));
#122310=CARTESIAN_POINT('Ctrl Pts',(58.1178876906907,-42.5703713416265,
12.));
#122311=CARTESIAN_POINT('Ctrl Pts',(58.1312594677386,-42.5904516306762,
12.));
#122312=CARTESIAN_POINT('Ctrl Pts',(58.1446349605421,-42.6105799327699,
12.));
#122313=CARTESIAN_POINT('Ctrl Pts',(58.1580140538228,-42.6307561832976,
12.));
#122314=CARTESIAN_POINT('Ctrl Pts',(58.171396632821,-42.6509803178265,12.));
#122315=CARTESIAN_POINT('Ctrl Pts',(58.1847825832923,-42.6712522721016,
12.));
#122316=CARTESIAN_POINT('Ctrl Pts',(58.1981717915037,-42.6915719820513,
12.));
#122317=CARTESIAN_POINT('Ctrl Pts',(58.21156414423,-42.7119393837866,12.));
#122318=CARTESIAN_POINT('Ctrl Pts',(58.22495952875,-42.7323544135985,12.));
#122319=CARTESIAN_POINT('Ctrl Pts',(58.2383578328424,-42.7528170079485,
12.));
#122320=CARTESIAN_POINT('Ctrl Pts',(58.251758944782,-42.773327103468,12.));
#122321=CARTESIAN_POINT('Ctrl Pts',(58.2651627533368,-42.7938846369651,
12.));
#122322=CARTESIAN_POINT('Ctrl Pts',(58.2785691477638,-42.8144895454233,
12.));
#122323=CARTESIAN_POINT('Ctrl Pts',(58.2919780178064,-42.8351417659999,
12.));
#122324=CARTESIAN_POINT('Ctrl Pts',(58.3053892536894,-42.8558412360158,
12.));
#122325=CARTESIAN_POINT('Ctrl Pts',(58.3188027461164,-42.8765878929551,
12.));
#122326=CARTESIAN_POINT('Ctrl Pts',(58.3322183862654,-42.8973816744709,
12.));
#122327=CARTESIAN_POINT('Ctrl Pts',(58.3456360657865,-42.9182225183855,
12.));
#122328=CARTESIAN_POINT('Ctrl Pts',(58.3590556767978,-42.9391103626879,
12.));
#122329=CARTESIAN_POINT('Ctrl Pts',(58.3724771118826,-42.960045145526,12.));
#122330=CARTESIAN_POINT('Ctrl Pts',(58.3859002640856,-42.9810268052032,
12.));
#122331=CARTESIAN_POINT('Ctrl Pts',(58.3993250269101,-43.0020552801859,
12.));
#122332=CARTESIAN_POINT('Ctrl Pts',(58.4127512943136,-43.0231305091027,
12.));
#122333=CARTESIAN_POINT('Ctrl Pts',(58.4261789607058,-43.0442524307434,
12.));
#122334=CARTESIAN_POINT('Ctrl Pts',(58.439607920945,-43.0654209840511,12.));
#122335=CARTESIAN_POINT('Ctrl Pts',(58.4530380703348,-43.0866361081177,
12.));
#122336=CARTESIAN_POINT('Ctrl Pts',(58.4664693046217,-43.1078977421916,
12.));
#122337=CARTESIAN_POINT('Ctrl Pts',(58.4799015199907,-43.1292058256777,
12.));
#122338=CARTESIAN_POINT('Ctrl Pts',(58.4933346130636,-43.1505602981365,
12.));
#122339=CARTESIAN_POINT('Ctrl Pts',(58.5067684808944,-43.1719610992771,
12.));
#122340=CARTESIAN_POINT('Ctrl Pts',(58.5202030209669,-43.1934081689505,
12.));
#122341=CARTESIAN_POINT('Ctrl Pts',(58.5336381311917,-43.2149014471574,
12.));
#122342=CARTESIAN_POINT('Ctrl Pts',(58.5470737099032,-43.2364408740493,
12.));
#122343=CARTESIAN_POINT('Ctrl Pts',(58.5605096558578,-43.2580263899278,
12.));
#122344=CARTESIAN_POINT('Ctrl Pts',(58.573945868231,-43.2796579352401,12.));
#122345=CARTESIAN_POINT('Ctrl Pts',(58.5873822466152,-43.3013354505701,
12.));
#122346=CARTESIAN_POINT('Ctrl Pts',(58.6008186910156,-43.3230588766449,
12.));
#122347=CARTESIAN_POINT('Ctrl Pts',(58.6142551018467,-43.3448281543372,
12.));
#122348=CARTESIAN_POINT('Ctrl Pts',(58.627691379929,-43.3666432246635,12.));
#122349=CARTESIAN_POINT('Ctrl Pts',(58.6411274264857,-43.388504028781,12.));
#122350=CARTESIAN_POINT('Ctrl Pts',(58.6545631431393,-43.4104105079768,
12.));
#122351=CARTESIAN_POINT('Ctrl Pts',(58.6679984319097,-43.4323626036737,
12.));
#122352=CARTESIAN_POINT('Ctrl Pts',(58.6814331952138,-43.4543602574351,
12.));
#122353=CARTESIAN_POINT('Ctrl Pts',(58.6948673358638,-43.4764034109654,
12.));
#122354=CARTESIAN_POINT('Ctrl Pts',(58.7083007570661,-43.4984920061073,
12.));
#122355=CARTESIAN_POINT('Ctrl Pts',(58.7217333624209,-43.5206259848338,
12.));
#122356=CARTESIAN_POINT('Ctrl Pts',(58.735165055918,-43.5428052892488,12.));
#122357=CARTESIAN_POINT('Ctrl Pts',(58.74859574193,-43.5650298615917,12.));
#122358=CARTESIAN_POINT('Ctrl Pts',(58.7620253252062,-43.5872996442345,
12.));
#122359=CARTESIAN_POINT('Ctrl Pts',(58.775453710867,-43.6096145796797,12.));
#122360=CARTESIAN_POINT('Ctrl Pts',(58.788880804397,-43.6319746105482,12.));
#122361=CARTESIAN_POINT('Ctrl Pts',(58.8023065116436,-43.6543796795789,
12.));
#122362=CARTESIAN_POINT('Ctrl Pts',(58.8157307388238,-43.6768297296395,
12.));
#122363=CARTESIAN_POINT('Ctrl Pts',(58.8291533925293,-43.6993247037314,
12.));
#122364=CARTESIAN_POINT('Ctrl Pts',(58.8425743797326,-43.7218645449922,
12.));
#122365=CARTESIAN_POINT('Ctrl Pts',(58.855993607794,-43.7444491966942,12.));
#122366=CARTESIAN_POINT('Ctrl Pts',(58.8694109844647,-43.7670786022402,
12.));
#122367=CARTESIAN_POINT('Ctrl Pts',(58.8828264178621,-43.7897527051609,
12.));
#122368=CARTESIAN_POINT('Ctrl Pts',(58.8962398164493,-43.8124714491077,
12.));
#122369=CARTESIAN_POINT('Ctrl Pts',(58.9096510890129,-43.835234777842,12.));
#122370=CARTESIAN_POINT('Ctrl Pts',(58.9230601446436,-43.858042635223,12.));
#122371=CARTESIAN_POINT('Ctrl Pts',(58.936466892712,-43.8808949651873,12.));
#122372=CARTESIAN_POINT('Ctrl Pts',(58.9498712429054,-43.9037917117739,
12.));
#122373=CARTESIAN_POINT('Ctrl Pts',(58.9632731052696,-43.9267328191501,
12.));
#122374=CARTESIAN_POINT('Ctrl Pts',(58.9766723902529,-43.9497182316331,
12.));
#122375=CARTESIAN_POINT('Ctrl Pts',(58.9900690087408,-43.9727478937056,
12.));
#122376=CARTESIAN_POINT('Ctrl Pts',(59.0034628721167,-43.9958217500369,
12.));
#122377=CARTESIAN_POINT('Ctrl Pts',(59.0168538922095,-44.0189397454599,
12.));
#122378=CARTESIAN_POINT('Ctrl Pts',(59.0302419811777,-44.0421018249223,
12.));
#122379=CARTESIAN_POINT('Ctrl Pts',(59.0436270514086,-44.0653079334385,
12.));
#122380=CARTESIAN_POINT('Ctrl Pts',(59.0570090154242,-44.0885580160433,
12.));
#122381=CARTESIAN_POINT('Ctrl Pts',(59.0703877857525,-44.1118520177221,
12.));
#122382=CARTESIAN_POINT('Ctrl Pts',(59.08376327492,-44.1351898834051,12.));
#122383=CARTESIAN_POINT('Ctrl Pts',(59.0971353957206,-44.1585715581065,
12.));
#122384=CARTESIAN_POINT('Ctrl Pts',(59.1105040614275,-44.1819969870307,
12.));
#122385=CARTESIAN_POINT('Ctrl Pts',(59.1238691860306,-44.2054661156875,
12.));
#122386=CARTESIAN_POINT('Ctrl Pts',(59.1372306844585,-44.228978889997,12.));
#122387=CARTESIAN_POINT('Ctrl Pts',(59.1505884728215,-44.2525352563996,
12.));
#122388=CARTESIAN_POINT('Ctrl Pts',(59.1639424678793,-44.2761351616048,
12.));
#122389=CARTESIAN_POINT('Ctrl Pts',(59.1772925865213,-44.2997785523431,
12.));
#122390=CARTESIAN_POINT('Ctrl Pts',(59.1906387451979,-44.3234653750884,
12.));
#122391=CARTESIAN_POINT('Ctrl Pts',(59.2039808594752,-44.3471955758403,
12.));
#122392=CARTESIAN_POINT('Ctrl Pts',(59.2173188432798,-44.370969099747,12.));
#122393=CARTESIAN_POINT('Ctrl Pts',(59.2306526095131,-44.3947858914074,
12.));
#122394=CARTESIAN_POINT('Ctrl Pts',(59.2439820714187,-44.4186458955451,
12.));
#122395=CARTESIAN_POINT('Ctrl Pts',(59.2573071437774,-44.4425490575911,
12.));
#122396=CARTESIAN_POINT('Ctrl Pts',(59.2706277440445,-44.4664953242379,
12.));
#122397=CARTESIAN_POINT('Ctrl Pts',(59.2839437938237,-44.490484644151,12.));
#122398=CARTESIAN_POINT('Ctrl Pts',(59.2972552192156,-44.5145169681349,
12.));
#122399=CARTESIAN_POINT('Ctrl Pts',(59.3086616639523,-44.5351541478479,
12.));
#122400=CARTESIAN_POINT('Ctrl Pts',(59.3174041872347,-44.5509994358154,
12.));
#122401=CARTESIAN_POINT('Ctrl Pts',(59.3234848865455,-44.5620338188738,
12.));
#122402=CARTESIAN_POINT('Ctrl Pts',(59.3269051738423,-44.5682447396021,
12.));
#122403=CARTESIAN_POINT('Ctrl Pts',(59.3276657444392,-44.5696260757792,
12.));
#122404=CARTESIAN_POINT('',(56.8466430164621,-40.8467768343957,0.));
#122405=CARTESIAN_POINT('',(56.8466430164621,-40.8467768343957,0.));
#122406=CARTESIAN_POINT('Ctrl Pts',(59.3276657444391,-44.569626075779,0.));
#122407=CARTESIAN_POINT('Ctrl Pts',(59.3269051738422,-44.568244739602,0.));
#122408=CARTESIAN_POINT('Ctrl Pts',(59.3234848865455,-44.5620338188737,
0.));
#122409=CARTESIAN_POINT('Ctrl Pts',(59.3174041872347,-44.5509994358153,
0.));
#122410=CARTESIAN_POINT('Ctrl Pts',(59.3086616639523,-44.5351541478479,
0.));
#122411=CARTESIAN_POINT('Ctrl Pts',(59.2972552192156,-44.5145169681349,
0.));
#122412=CARTESIAN_POINT('Ctrl Pts',(59.2839437938237,-44.490484644151,0.));
#122413=CARTESIAN_POINT('Ctrl Pts',(59.2706277440445,-44.4664953242379,
0.));
#122414=CARTESIAN_POINT('Ctrl Pts',(59.2573071437774,-44.4425490575911,
0.));
#122415=CARTESIAN_POINT('Ctrl Pts',(59.2439820714187,-44.4186458955451,
0.));
#122416=CARTESIAN_POINT('Ctrl Pts',(59.2306526095131,-44.3947858914074,
0.));
#122417=CARTESIAN_POINT('Ctrl Pts',(59.2173188432798,-44.370969099747,0.));
#122418=CARTESIAN_POINT('Ctrl Pts',(59.2039808594752,-44.3471955758403,
0.));
#122419=CARTESIAN_POINT('Ctrl Pts',(59.1906387451979,-44.3234653750884,
0.));
#122420=CARTESIAN_POINT('Ctrl Pts',(59.1772925865213,-44.2997785523431,
0.));
#122421=CARTESIAN_POINT('Ctrl Pts',(59.1639424678793,-44.2761351616048,
0.));
#122422=CARTESIAN_POINT('Ctrl Pts',(59.1505884728215,-44.2525352563996,
0.));
#122423=CARTESIAN_POINT('Ctrl Pts',(59.1372306844585,-44.228978889997,0.));
#122424=CARTESIAN_POINT('Ctrl Pts',(59.1238691860306,-44.2054661156875,
0.));
#122425=CARTESIAN_POINT('Ctrl Pts',(59.1105040614275,-44.1819969870307,
0.));
#122426=CARTESIAN_POINT('Ctrl Pts',(59.0971353957206,-44.1585715581065,
0.));
#122427=CARTESIAN_POINT('Ctrl Pts',(59.08376327492,-44.1351898834051,0.));
#122428=CARTESIAN_POINT('Ctrl Pts',(59.0703877857525,-44.1118520177221,
0.));
#122429=CARTESIAN_POINT('Ctrl Pts',(59.0570090154242,-44.0885580160433,
0.));
#122430=CARTESIAN_POINT('Ctrl Pts',(59.0436270514086,-44.0653079334385,
0.));
#122431=CARTESIAN_POINT('Ctrl Pts',(59.0302419811777,-44.0421018249223,
0.));
#122432=CARTESIAN_POINT('Ctrl Pts',(59.0168538922095,-44.0189397454599,
0.));
#122433=CARTESIAN_POINT('Ctrl Pts',(59.0034628721167,-43.9958217500369,
0.));
#122434=CARTESIAN_POINT('Ctrl Pts',(58.9900690087408,-43.9727478937056,
0.));
#122435=CARTESIAN_POINT('Ctrl Pts',(58.9766723902529,-43.9497182316331,
0.));
#122436=CARTESIAN_POINT('Ctrl Pts',(58.9632731052696,-43.9267328191501,
0.));
#122437=CARTESIAN_POINT('Ctrl Pts',(58.9498712429054,-43.9037917117739,
0.));
#122438=CARTESIAN_POINT('Ctrl Pts',(58.936466892712,-43.8808949651873,0.));
#122439=CARTESIAN_POINT('Ctrl Pts',(58.9230601446436,-43.858042635223,0.));
#122440=CARTESIAN_POINT('Ctrl Pts',(58.9096510890129,-43.835234777842,0.));
#122441=CARTESIAN_POINT('Ctrl Pts',(58.8962398164493,-43.8124714491077,
0.));
#122442=CARTESIAN_POINT('Ctrl Pts',(58.8828264178621,-43.7897527051609,
0.));
#122443=CARTESIAN_POINT('Ctrl Pts',(58.8694109844647,-43.7670786022402,
0.));
#122444=CARTESIAN_POINT('Ctrl Pts',(58.855993607794,-43.7444491966942,0.));
#122445=CARTESIAN_POINT('Ctrl Pts',(58.8425743797326,-43.7218645449922,
0.));
#122446=CARTESIAN_POINT('Ctrl Pts',(58.8291533925293,-43.6993247037314,
0.));
#122447=CARTESIAN_POINT('Ctrl Pts',(58.8157307388238,-43.6768297296395,
0.));
#122448=CARTESIAN_POINT('Ctrl Pts',(58.8023065116436,-43.6543796795789,
0.));
#122449=CARTESIAN_POINT('Ctrl Pts',(58.788880804397,-43.6319746105482,0.));
#122450=CARTESIAN_POINT('Ctrl Pts',(58.775453710867,-43.6096145796797,0.));
#122451=CARTESIAN_POINT('Ctrl Pts',(58.7620253252062,-43.5872996442345,
0.));
#122452=CARTESIAN_POINT('Ctrl Pts',(58.74859574193,-43.5650298615917,0.));
#122453=CARTESIAN_POINT('Ctrl Pts',(58.735165055918,-43.5428052892488,0.));
#122454=CARTESIAN_POINT('Ctrl Pts',(58.7217333624209,-43.5206259848338,
0.));
#122455=CARTESIAN_POINT('Ctrl Pts',(58.7083007570661,-43.4984920061073,
0.));
#122456=CARTESIAN_POINT('Ctrl Pts',(58.6948673358638,-43.4764034109654,
0.));
#122457=CARTESIAN_POINT('Ctrl Pts',(58.6814331952138,-43.4543602574351,
0.));
#122458=CARTESIAN_POINT('Ctrl Pts',(58.6679984319097,-43.4323626036737,
0.));
#122459=CARTESIAN_POINT('Ctrl Pts',(58.6545631431393,-43.4104105079768,
0.));
#122460=CARTESIAN_POINT('Ctrl Pts',(58.6411274264857,-43.388504028781,0.));
#122461=CARTESIAN_POINT('Ctrl Pts',(58.627691379929,-43.3666432246635,0.));
#122462=CARTESIAN_POINT('Ctrl Pts',(58.6142551018467,-43.3448281543372,
0.));
#122463=CARTESIAN_POINT('Ctrl Pts',(58.6008186910156,-43.3230588766449,
0.));
#122464=CARTESIAN_POINT('Ctrl Pts',(58.5873822466152,-43.3013354505701,
0.));
#122465=CARTESIAN_POINT('Ctrl Pts',(58.573945868231,-43.2796579352401,0.));
#122466=CARTESIAN_POINT('Ctrl Pts',(58.5605096558578,-43.2580263899278,
0.));
#122467=CARTESIAN_POINT('Ctrl Pts',(58.5470737099032,-43.2364408740493,
0.));
#122468=CARTESIAN_POINT('Ctrl Pts',(58.5336381311917,-43.2149014471574,
0.));
#122469=CARTESIAN_POINT('Ctrl Pts',(58.5202030209669,-43.1934081689505,
0.));
#122470=CARTESIAN_POINT('Ctrl Pts',(58.5067684808944,-43.1719610992771,
0.));
#122471=CARTESIAN_POINT('Ctrl Pts',(58.4933346130636,-43.1505602981365,
0.));
#122472=CARTESIAN_POINT('Ctrl Pts',(58.4799015199907,-43.1292058256777,
0.));
#122473=CARTESIAN_POINT('Ctrl Pts',(58.4664693046217,-43.1078977421916,
0.));
#122474=CARTESIAN_POINT('Ctrl Pts',(58.4530380703348,-43.0866361081177,
0.));
#122475=CARTESIAN_POINT('Ctrl Pts',(58.439607920945,-43.0654209840511,0.));
#122476=CARTESIAN_POINT('Ctrl Pts',(58.4261789607058,-43.0442524307434,
0.));
#122477=CARTESIAN_POINT('Ctrl Pts',(58.4127512943136,-43.0231305091027,
0.));
#122478=CARTESIAN_POINT('Ctrl Pts',(58.3993250269101,-43.0020552801859,
0.));
#122479=CARTESIAN_POINT('Ctrl Pts',(58.3859002640856,-42.9810268052032,
0.));
#122480=CARTESIAN_POINT('Ctrl Pts',(58.3724771118826,-42.960045145526,0.));
#122481=CARTESIAN_POINT('Ctrl Pts',(58.3590556767978,-42.9391103626879,
0.));
#122482=CARTESIAN_POINT('Ctrl Pts',(58.3456360657865,-42.9182225183855,
0.));
#122483=CARTESIAN_POINT('Ctrl Pts',(58.3322183862654,-42.8973816744709,
0.));
#122484=CARTESIAN_POINT('Ctrl Pts',(58.3188027461164,-42.8765878929551,
0.));
#122485=CARTESIAN_POINT('Ctrl Pts',(58.3053892536894,-42.8558412360158,
0.));
#122486=CARTESIAN_POINT('Ctrl Pts',(58.2919780178064,-42.8351417659999,
0.));
#122487=CARTESIAN_POINT('Ctrl Pts',(58.2785691477638,-42.8144895454233,
0.));
#122488=CARTESIAN_POINT('Ctrl Pts',(58.2651627533368,-42.7938846369651,
0.));
#122489=CARTESIAN_POINT('Ctrl Pts',(58.251758944782,-42.773327103468,0.));
#122490=CARTESIAN_POINT('Ctrl Pts',(58.2383578328424,-42.7528170079485,
0.));
#122491=CARTESIAN_POINT('Ctrl Pts',(58.22495952875,-42.7323544135985,0.));
#122492=CARTESIAN_POINT('Ctrl Pts',(58.21156414423,-42.7119393837866,0.));
#122493=CARTESIAN_POINT('Ctrl Pts',(58.1981717915037,-42.6915719820513,
0.));
#122494=CARTESIAN_POINT('Ctrl Pts',(58.1847825832923,-42.6712522721016,
0.));
#122495=CARTESIAN_POINT('Ctrl Pts',(58.171396632821,-42.6509803178265,0.));
#122496=CARTESIAN_POINT('Ctrl Pts',(58.1580140538228,-42.6307561832976,
0.));
#122497=CARTESIAN_POINT('Ctrl Pts',(58.1446349605421,-42.6105799327699,
0.));
#122498=CARTESIAN_POINT('Ctrl Pts',(58.1312594677386,-42.5904516306762,
0.));
#122499=CARTESIAN_POINT('Ctrl Pts',(58.1178876906907,-42.5703713416265,
0.));
#122500=CARTESIAN_POINT('Ctrl Pts',(58.1045197452002,-42.5503391304183,
0.));
#122501=CARTESIAN_POINT('Ctrl Pts',(58.0911557475965,-42.5303550620387,
0.));
#122502=CARTESIAN_POINT('Ctrl Pts',(58.0777958147403,-42.5104192016664,
0.));
#122503=CARTESIAN_POINT('Ctrl Pts',(58.0644400640275,-42.4905316146654,
0.));
#122504=CARTESIAN_POINT('Ctrl Pts',(58.0510886133926,-42.4706923665845,
0.));
#122505=CARTESIAN_POINT('Ctrl Pts',(58.037741581314,-42.4509015231674,0.));
#122506=CARTESIAN_POINT('Ctrl Pts',(58.0243990868181,-42.4311591503555,
0.));
#122507=CARTESIAN_POINT('Ctrl Pts',(58.0110612494828,-42.411465314289,0.));
#122508=CARTESIAN_POINT('Ctrl Pts',(57.9977281894422,-42.3918200813014,
0.));
#122509=CARTESIAN_POINT('Ctrl Pts',(57.9844000273911,-42.3722235179198,
0.));
#122510=CARTESIAN_POINT('Ctrl Pts',(57.9710768845899,-42.3526756908747,
0.));
#122511=CARTESIAN_POINT('Ctrl Pts',(57.9577588828682,-42.333176667102,0.));
#122512=CARTESIAN_POINT('Ctrl Pts',(57.9444461446299,-42.3137265137452,
0.));
#122513=CARTESIAN_POINT('Ctrl Pts',(57.9311387928563,-42.2943252981489,
0.));
#122514=CARTESIAN_POINT('Ctrl Pts',(57.9178369511114,-42.2749730878595,
0.));
#122515=CARTESIAN_POINT('Ctrl Pts',(57.9045407435474,-42.2556699506353,
0.));
#122516=CARTESIAN_POINT('Ctrl Pts',(57.8912502949096,-42.2364159544501,
0.));
#122517=CARTESIAN_POINT('Ctrl Pts',(57.8779657305413,-42.2172111674938,
0.));
#122518=CARTESIAN_POINT('Ctrl Pts',(57.864687176387,-42.1980556581665,0.));
#122519=CARTESIAN_POINT('Ctrl Pts',(57.8514147589972,-42.1789494950794,
0.));
#122520=CARTESIAN_POINT('Ctrl Pts',(57.8381486055342,-42.1598927470646,
0.));
#122521=CARTESIAN_POINT('Ctrl Pts',(57.8248888437775,-42.1408854831783,
0.));
#122522=CARTESIAN_POINT('Ctrl Pts',(57.8116356021288,-42.1219277727021,
0.));
#122523=CARTESIAN_POINT('Ctrl Pts',(57.798389009616,-42.1030196851366,0.));
#122524=CARTESIAN_POINT('Ctrl Pts',(57.7851491958987,-42.0841612902042,
0.));
#122525=CARTESIAN_POINT('Ctrl Pts',(57.7719162912744,-42.0653526578588,
0.));
#122526=CARTESIAN_POINT('Ctrl Pts',(57.7586904266834,-42.0465938582882,
0.));
#122527=CARTESIAN_POINT('Ctrl Pts',(57.745471733714,-42.0278849619148,0.));
#122528=CARTESIAN_POINT('Ctrl Pts',(57.7322603446066,-42.0092260393897,
0.));
#122529=CARTESIAN_POINT('Ctrl Pts',(57.7190563922593,-41.990617161596,0.));
#122530=CARTESIAN_POINT('Ctrl Pts',(57.7058600102351,-41.9720583996592,
0.));
#122531=CARTESIAN_POINT('Ctrl Pts',(57.6926713327672,-41.9535498249488,
0.));
#122532=CARTESIAN_POINT('Ctrl Pts',(57.6794904947649,-41.9350915090797,
0.));
#122533=CARTESIAN_POINT('Ctrl Pts',(57.6663176318189,-41.9166835239054,
0.));
#122534=CARTESIAN_POINT('Ctrl Pts',(57.6531528802072,-41.8983259415253,
0.));
#122535=CARTESIAN_POINT('Ctrl Pts',(57.6399963769009,-41.8800188342912,
0.));
#122536=CARTESIAN_POINT('Ctrl Pts',(57.6268482595701,-41.8617622748107,
0.));
#122537=CARTESIAN_POINT('Ctrl Pts',(57.613708666588,-41.8435563359456,0.));
#122538=CARTESIAN_POINT('Ctrl Pts',(57.6005777370347,-41.8254010908051,
0.));
#122539=CARTESIAN_POINT('Ctrl Pts',(57.5874556107054,-41.8072966127559,
0.));
#122540=CARTESIAN_POINT('Ctrl Pts',(57.5743424281204,-41.7892429754298,
0.));
#122541=CARTESIAN_POINT('Ctrl Pts',(57.561238330532,-41.7712402527273,0.));
#122542=CARTESIAN_POINT('Ctrl Pts',(57.5481434599334,-41.7532885188174,
0.));
#122543=CARTESIAN_POINT('Ctrl Pts',(57.5350579590648,-41.7353878481336,
0.));
#122544=CARTESIAN_POINT('Ctrl Pts',(57.5219819714169,-41.7175383153819,
0.));
#122545=CARTESIAN_POINT('Ctrl Pts',(57.5089156412341,-41.6997399955445,
0.));
#122546=CARTESIAN_POINT('Ctrl Pts',(57.4958591135165,-41.6819929638797,
0.));
#122547=CARTESIAN_POINT('Ctrl Pts',(57.4828125340222,-41.6642972959168,
0.));
#122548=CARTESIAN_POINT('Ctrl Pts',(57.4697760492693,-41.6466530674522,
0.));
#122549=CARTESIAN_POINT('Ctrl Pts',(57.4567498065573,-41.6290603545674,
0.));
#122550=CARTESIAN_POINT('Ctrl Pts',(57.4437339539848,-41.6115192336394,
0.));
#122551=CARTESIAN_POINT('Ctrl Pts',(57.4307286404656,-41.5940297813474,
0.));
#122552=CARTESIAN_POINT('Ctrl Pts',(57.417734015749,-41.5765920746764,0.));
#122553=CARTESIAN_POINT('Ctrl Pts',(57.4047502304207,-41.5592061909159,
0.));
#122554=CARTESIAN_POINT('Ctrl Pts',(57.3917774358844,-41.5418722076558,
0.));
#122555=CARTESIAN_POINT('Ctrl Pts',(57.378815784345,-41.5245902027767,0.));
#122556=CARTESIAN_POINT('Ctrl Pts',(57.3658654287948,-41.5073602544404,
0.));
#122557=CARTESIAN_POINT('Ctrl Pts',(57.3529265229858,-41.4901824410654,
0.));
#122558=CARTESIAN_POINT('Ctrl Pts',(57.339999221474,-41.4730568413535,0.));
#122559=CARTESIAN_POINT('Ctrl Pts',(57.3270836796925,-41.4559835343339,
0.));
#122560=CARTESIAN_POINT('Ctrl Pts',(57.3141800540137,-41.4389625993948,
0.));
#122561=CARTESIAN_POINT('Ctrl Pts',(57.3012885018139,-41.4219941163155,
0.));
#122562=CARTESIAN_POINT('Ctrl Pts',(57.2884091815384,-41.4050781652923,
0.));
#122563=CARTESIAN_POINT('Ctrl Pts',(57.2755422525822,-41.3882148268798,
0.));
#122564=CARTESIAN_POINT('Ctrl Pts',(57.2626878751584,-41.3714041819215,
0.));
#122565=CARTESIAN_POINT('Ctrl Pts',(57.2498462101883,-41.3546463114889,
0.));
#122566=CARTESIAN_POINT('Ctrl Pts',(57.237017419142,-41.3379412967889,0.));
#122567=CARTESIAN_POINT('Ctrl Pts',(57.2242016640226,-41.321289219151,0.));
#122568=CARTESIAN_POINT('Ctrl Pts',(57.2113991077325,-41.304690160231,0.));
#122569=CARTESIAN_POINT('Ctrl Pts',(57.1986099143992,-41.288144202187,0.));
#122570=CARTESIAN_POINT('Ctrl Pts',(57.1858342496526,-41.2716514278268,
0.));
#122571=CARTESIAN_POINT('Ctrl Pts',(57.1730722810771,-41.2552119208445,
0.));
#122572=CARTESIAN_POINT('Ctrl Pts',(57.1603241779042,-41.2388257656534,
0.));
#122573=CARTESIAN_POINT('Ctrl Pts',(57.1475901101794,-41.2224930469412,
0.));
#122574=CARTESIAN_POINT('Ctrl Pts',(57.1348702480644,-41.2062138492913,
0.));
#122575=CARTESIAN_POINT('Ctrl Pts',(57.1221647611231,-41.1899882567941,
0.));
#122576=CARTESIAN_POINT('Ctrl Pts',(57.1094738174998,-41.1738163525932,
0.));
#122577=CARTESIAN_POINT('Ctrl Pts',(57.0967975854912,-41.1576982197403,
0.));
#122578=CARTESIAN_POINT('Ctrl Pts',(57.084136235428,-41.1416339422132,0.));
#122579=CARTESIAN_POINT('Ctrl Pts',(57.0714899412091,-41.1256236057437,
0.));
#122580=CARTESIAN_POINT('Ctrl Pts',(57.0588588825266,-41.1096672990125,
0.));
#122581=CARTESIAN_POINT('Ctrl Pts',(57.0462432450637,-41.093765113752,0.));
#122582=CARTESIAN_POINT('Ctrl Pts',(57.0336432158503,-41.0779171422415,
0.));
#122583=CARTESIAN_POINT('Ctrl Pts',(57.0210589791777,-41.0621234751,0.));
#122584=CARTESIAN_POINT('Ctrl Pts',(57.008490713044,-41.0463841993622,0.));
#122585=CARTESIAN_POINT('Ctrl Pts',(56.9959385834768,-41.0306993954021,
0.));
#122586=CARTESIAN_POINT('Ctrl Pts',(56.9834027500178,-41.0150691398988,
0.));
#122587=CARTESIAN_POINT('Ctrl Pts',(56.9708833766183,-40.9994935117307,
0.));
#122588=CARTESIAN_POINT('Ctrl Pts',(56.9583806404069,-40.9839725967121,
0.));
#122589=CARTESIAN_POINT('Ctrl Pts',(56.9458947422541,-40.968506493303,0.));
#122590=CARTESIAN_POINT('Ctrl Pts',(56.9334259139928,-40.9530953164952,
0.));
#122591=CARTESIAN_POINT('Ctrl Pts',(56.9209743960861,-40.9377391857044,
0.));
#122592=CARTESIAN_POINT('Ctrl Pts',(56.9085404164432,-40.9224382132382,
0.));
#122593=CARTESIAN_POINT('Ctrl Pts',(56.8961241708926,-40.9071924937551,
0.));
#122594=CARTESIAN_POINT('Ctrl Pts',(56.8837257978574,-40.8920020903443,
0.));
#122595=CARTESIAN_POINT('Ctrl Pts',(56.8713453765252,-40.8768670342278,
0.));
#122596=CARTESIAN_POINT('Ctrl Pts',(56.8614554317993,-40.8648032759631,
0.));
#122597=CARTESIAN_POINT('Ctrl Pts',(56.8540460739677,-40.8557803680412,
0.));
#122598=CARTESIAN_POINT('Ctrl Pts',(56.8491101022668,-40.8497761671086,
0.));
#122599=CARTESIAN_POINT('Ctrl Pts',(56.8466430164621,-40.8467768343957,
0.));
#122600=CARTESIAN_POINT('Ctrl Pts',(55.3473204966403,-49.8690697110161,
0.));
#122601=CARTESIAN_POINT('Ctrl Pts',(55.3473204966403,-49.8690697110161,
12.));
#122602=CARTESIAN_POINT('Ctrl Pts',(55.3451131058826,-49.8639277221566,
0.));
#122603=CARTESIAN_POINT('Ctrl Pts',(55.3451131058826,-49.8639277221566,
12.));
#122604=CARTESIAN_POINT('Ctrl Pts',(55.34069740326,-49.8536479176833,0.));
#122605=CARTESIAN_POINT('Ctrl Pts',(55.34069740326,-49.8536479176833,12.));
#122606=CARTESIAN_POINT('Ctrl Pts',(55.3340710860055,-49.8382407307107,
0.));
#122607=CARTESIAN_POINT('Ctrl Pts',(55.3340710860055,-49.8382407307107,
12.));
#122608=CARTESIAN_POINT('Ctrl Pts',(55.3252304694602,-49.8177228552377,
0.));
#122609=CARTESIAN_POINT('Ctrl Pts',(55.3252304694602,-49.8177228552377,
12.));
#122610=CARTESIAN_POINT('Ctrl Pts',(55.3141704897766,-49.7921172540628,
0.));
#122611=CARTESIAN_POINT('Ctrl Pts',(55.3141704897766,-49.7921172540628,
12.));
#122612=CARTESIAN_POINT('Ctrl Pts',(55.3031013105853,-49.7665534128535,
0.));
#122613=CARTESIAN_POINT('Ctrl Pts',(55.3031013105853,-49.7665534128535,
12.));
#122614=CARTESIAN_POINT('Ctrl Pts',(55.2920229527546,-49.7410313576508,
0.));
#122615=CARTESIAN_POINT('Ctrl Pts',(55.2920229527546,-49.7410313576508,
12.));
#122616=CARTESIAN_POINT('Ctrl Pts',(55.2809354521515,-49.7155511248531,
0.));
#122617=CARTESIAN_POINT('Ctrl Pts',(55.2809354521515,-49.7155511248531,
12.));
#122618=CARTESIAN_POINT('Ctrl Pts',(55.2698388650025,-49.6901127631627,
0.));
#122619=CARTESIAN_POINT('Ctrl Pts',(55.2698388650025,-49.6901127631627,
12.));
#122620=CARTESIAN_POINT('Ctrl Pts',(55.2587332663783,-49.6647163322266,
0.));
#122621=CARTESIAN_POINT('Ctrl Pts',(55.2587332663783,-49.6647163322266,
12.));
#122622=CARTESIAN_POINT('Ctrl Pts',(55.2476187434057,-49.6393618987473,
0.));
#122623=CARTESIAN_POINT('Ctrl Pts',(55.2476187434057,-49.6393618987473,
12.));
#122624=CARTESIAN_POINT('Ctrl Pts',(55.2364953899358,-49.6140495332804,
0.));
#122625=CARTESIAN_POINT('Ctrl Pts',(55.2364953899358,-49.6140495332804,
12.));
#122626=CARTESIAN_POINT('Ctrl Pts',(55.2253633007666,-49.5887793068352,
0.));
#122627=CARTESIAN_POINT('Ctrl Pts',(55.2253633007666,-49.5887793068352,
12.));
#122628=CARTESIAN_POINT('Ctrl Pts',(55.2142225657013,-49.5635512873435,
0.));
#122629=CARTESIAN_POINT('Ctrl Pts',(55.2142225657013,-49.5635512873435,
12.));
#122630=CARTESIAN_POINT('Ctrl Pts',(55.2030732647312,-49.5383655368074,
0.));
#122631=CARTESIAN_POINT('Ctrl Pts',(55.2030732647312,-49.5383655368074,
12.));
#122632=CARTESIAN_POINT('Ctrl Pts',(55.1919154713647,-49.5132221132992,
0.));
#122633=CARTESIAN_POINT('Ctrl Pts',(55.1919154713647,-49.5132221132992,
12.));
#122634=CARTESIAN_POINT('Ctrl Pts',(55.1807492550119,-49.4881210723966,
0.));
#122635=CARTESIAN_POINT('Ctrl Pts',(55.1807492550119,-49.4881210723966,
12.));
#122636=CARTESIAN_POINT('Ctrl Pts',(55.1695746838174,-49.4630624688793,
0.));
#122637=CARTESIAN_POINT('Ctrl Pts',(55.1695746838174,-49.4630624688793,
12.));
#122638=CARTESIAN_POINT('Ctrl Pts',(55.1583918271116,-49.4380463581965,
0.));
#122639=CARTESIAN_POINT('Ctrl Pts',(55.1583918271116,-49.4380463581965,
12.));
#122640=CARTESIAN_POINT('Ctrl Pts',(55.1472007585183,-49.4130727983201,
0.));
#122641=CARTESIAN_POINT('Ctrl Pts',(55.1472007585183,-49.4130727983201,
12.));
#122642=CARTESIAN_POINT('Ctrl Pts',(55.136001555622,-49.3881418495489,0.));
#122643=CARTESIAN_POINT('Ctrl Pts',(55.136001555622,-49.3881418495489,12.));
#122644=CARTESIAN_POINT('Ctrl Pts',(55.1247942985619,-49.3632535736715,
0.));
#122645=CARTESIAN_POINT('Ctrl Pts',(55.1247942985619,-49.3632535736715,
12.));
#122646=CARTESIAN_POINT('Ctrl Pts',(55.1135790689464,-49.3384080333155,
0.));
#122647=CARTESIAN_POINT('Ctrl Pts',(55.1135790689464,-49.3384080333155,
12.));
#122648=CARTESIAN_POINT('Ctrl Pts',(55.102355948714,-49.3136052912622,0.));
#122649=CARTESIAN_POINT('Ctrl Pts',(55.102355948714,-49.3136052912622,12.));
#122650=CARTESIAN_POINT('Ctrl Pts',(55.0911250188302,-49.2888454096563,
0.));
#122651=CARTESIAN_POINT('Ctrl Pts',(55.0911250188302,-49.2888454096563,
12.));
#122652=CARTESIAN_POINT('Ctrl Pts',(55.079886358701,-49.264128449652,0.));
#122653=CARTESIAN_POINT('Ctrl Pts',(55.079886358701,-49.264128449652,12.));
#122654=CARTESIAN_POINT('Ctrl Pts',(55.0686400468931,-49.2394544718531,
0.));
#122655=CARTESIAN_POINT('Ctrl Pts',(55.0686400468931,-49.2394544718531,
12.));
#122656=CARTESIAN_POINT('Ctrl Pts',(55.0573861615579,-49.2148235365704,
0.));
#122657=CARTESIAN_POINT('Ctrl Pts',(55.0573861615579,-49.2148235365704,
12.));
#122658=CARTESIAN_POINT('Ctrl Pts',(55.0461247809744,-49.1902357041461,
0.));
#122659=CARTESIAN_POINT('Ctrl Pts',(55.0461247809744,-49.1902357041461,
12.));
#122660=CARTESIAN_POINT('Ctrl Pts',(55.0348559840453,-49.1656910352476,
0.));
#122661=CARTESIAN_POINT('Ctrl Pts',(55.0348559840453,-49.1656910352476,
12.));
#122662=CARTESIAN_POINT('Ctrl Pts',(55.0235798508045,-49.1411895911635,
0.));
#122663=CARTESIAN_POINT('Ctrl Pts',(55.0235798508045,-49.1411895911635,
12.));
#122664=CARTESIAN_POINT('Ctrl Pts',(55.012296462186,-49.116731433673,0.));
#122665=CARTESIAN_POINT('Ctrl Pts',(55.012296462186,-49.116731433673,12.));
#122666=CARTESIAN_POINT('Ctrl Pts',(55.0010058998107,-49.0923166249219,
0.));
#122667=CARTESIAN_POINT('Ctrl Pts',(55.0010058998107,-49.0923166249219,
12.));
#122668=CARTESIAN_POINT('Ctrl Pts',(54.9897082457606,-49.067945227287,0.));
#122669=CARTESIAN_POINT('Ctrl Pts',(54.9897082457606,-49.067945227287,12.));
#122670=CARTESIAN_POINT('Ctrl Pts',(54.9784035823765,-49.0436173032528,
0.));
#122671=CARTESIAN_POINT('Ctrl Pts',(54.9784035823765,-49.0436173032528,
12.));
#122672=CARTESIAN_POINT('Ctrl Pts',(54.9670919920029,-49.0193329152479,
0.));
#122673=CARTESIAN_POINT('Ctrl Pts',(54.9670919920029,-49.0193329152479,
12.));
#122674=CARTESIAN_POINT('Ctrl Pts',(54.9557735569943,-48.9950921256527,
0.));
#122675=CARTESIAN_POINT('Ctrl Pts',(54.9557735569943,-48.9950921256527,
12.));
#122676=CARTESIAN_POINT('Ctrl Pts',(54.9444483598378,-48.9708949968795,
0.));
#122677=CARTESIAN_POINT('Ctrl Pts',(54.9444483598378,-48.9708949968795,
12.));
#122678=CARTESIAN_POINT('Ctrl Pts',(54.9331164832423,-48.9467415914269,
0.));
#122679=CARTESIAN_POINT('Ctrl Pts',(54.9331164832423,-48.9467415914269,
12.));
#122680=CARTESIAN_POINT('Ctrl Pts',(54.9217780102355,-48.9226319719369,
0.));
#122681=CARTESIAN_POINT('Ctrl Pts',(54.9217780102355,-48.9226319719369,
12.));
#122682=CARTESIAN_POINT('Ctrl Pts',(54.9104330242742,-48.8985662012528,
0.));
#122683=CARTESIAN_POINT('Ctrl Pts',(54.9104330242742,-48.8985662012528,
12.));
#122684=CARTESIAN_POINT('Ctrl Pts',(54.8990816092953,-48.8745443424477,
0.));
#122685=CARTESIAN_POINT('Ctrl Pts',(54.8990816092953,-48.8745443424477,
12.));
#122686=CARTESIAN_POINT('Ctrl Pts',(54.8877238496565,-48.8505664587974,
0.));
#122687=CARTESIAN_POINT('Ctrl Pts',(54.8877238496565,-48.8505664587974,
12.));
#122688=CARTESIAN_POINT('Ctrl Pts',(54.8763598301037,-48.8266326137622,
0.));
#122689=CARTESIAN_POINT('Ctrl Pts',(54.8763598301037,-48.8266326137622,
12.));
#122690=CARTESIAN_POINT('Ctrl Pts',(54.8649896357285,-48.8027428709614,
0.));
#122691=CARTESIAN_POINT('Ctrl Pts',(54.8649896357285,-48.8027428709614,
12.));
#122692=CARTESIAN_POINT('Ctrl Pts',(54.8536133519292,-48.7788972941438,
0.));
#122693=CARTESIAN_POINT('Ctrl Pts',(54.8536133519292,-48.7788972941438,
12.));
#122694=CARTESIAN_POINT('Ctrl Pts',(54.8422310643763,-48.7550959471601,
0.));
#122695=CARTESIAN_POINT('Ctrl Pts',(54.8422310643763,-48.7550959471601,
12.));
#122696=CARTESIAN_POINT('Ctrl Pts',(54.8308428590344,-48.7313388939845,
0.));
#122697=CARTESIAN_POINT('Ctrl Pts',(54.8308428590344,-48.7313388939845,
12.));
#122698=CARTESIAN_POINT('Ctrl Pts',(54.819448822181,-48.7076261987292,0.));
#122699=CARTESIAN_POINT('Ctrl Pts',(54.819448822181,-48.7076261987292,12.));
#122700=CARTESIAN_POINT('Ctrl Pts',(54.8080490404275,-48.6839579256566,
0.));
#122701=CARTESIAN_POINT('Ctrl Pts',(54.8080490404275,-48.6839579256566,
12.));
#122702=CARTESIAN_POINT('Ctrl Pts',(54.7966436007389,-48.6603341391886,
0.));
#122703=CARTESIAN_POINT('Ctrl Pts',(54.7966436007389,-48.6603341391886,
12.));
#122704=CARTESIAN_POINT('Ctrl Pts',(54.7852325904583,-48.6367549039112,
0.));
#122705=CARTESIAN_POINT('Ctrl Pts',(54.7852325904583,-48.6367549039112,
12.));
#122706=CARTESIAN_POINT('Ctrl Pts',(54.7738160973031,-48.6132202845783,
0.));
#122707=CARTESIAN_POINT('Ctrl Pts',(54.7738160973031,-48.6132202845783,
12.));
#122708=CARTESIAN_POINT('Ctrl Pts',(54.7623942093586,-48.5897303461125,
0.));
#122709=CARTESIAN_POINT('Ctrl Pts',(54.7623942093586,-48.5897303461125,
12.));
#122710=CARTESIAN_POINT('Ctrl Pts',(54.7509670150714,-48.5662851536026,
0.));
#122711=CARTESIAN_POINT('Ctrl Pts',(54.7509670150714,-48.5662851536026,
12.));
#122712=CARTESIAN_POINT('Ctrl Pts',(54.7395346032453,-48.5428847722977,
0.));
#122713=CARTESIAN_POINT('Ctrl Pts',(54.7395346032453,-48.5428847722977,
12.));
#122714=CARTESIAN_POINT('Ctrl Pts',(54.7280970630351,-48.519529267596,0.));
#122715=CARTESIAN_POINT('Ctrl Pts',(54.7280970630351,-48.519529267596,12.));
#122716=CARTESIAN_POINT('Ctrl Pts',(54.716654483948,-48.4962187050457,0.));
#122717=CARTESIAN_POINT('Ctrl Pts',(54.716654483948,-48.4962187050457,12.));
#122718=CARTESIAN_POINT('Ctrl Pts',(54.7052069558497,-48.472953150357,0.));
#122719=CARTESIAN_POINT('Ctrl Pts',(54.7052069558497,-48.472953150357,12.));
#122720=CARTESIAN_POINT('Ctrl Pts',(54.6937545689695,-48.4497326694052,
0.));
#122721=CARTESIAN_POINT('Ctrl Pts',(54.6937545689695,-48.4497326694052,
12.));
#122722=CARTESIAN_POINT('Ctrl Pts',(54.6822974139063,-48.426557328234,0.));
#122723=CARTESIAN_POINT('Ctrl Pts',(54.6822974139063,-48.426557328234,12.));
#122724=CARTESIAN_POINT('Ctrl Pts',(54.6708355816358,-48.4034271930514,
0.));
#122725=CARTESIAN_POINT('Ctrl Pts',(54.6708355816358,-48.4034271930514,
12.));
#122726=CARTESIAN_POINT('Ctrl Pts',(54.6593691635145,-48.3803423302294,
0.));
#122727=CARTESIAN_POINT('Ctrl Pts',(54.6593691635145,-48.3803423302294,
12.));
#122728=CARTESIAN_POINT('Ctrl Pts',(54.6478982512794,-48.3573028063124,
0.));
#122729=CARTESIAN_POINT('Ctrl Pts',(54.6478982512794,-48.3573028063124,
12.));
#122730=CARTESIAN_POINT('Ctrl Pts',(54.6364229370494,-48.3343086880194,
0.));
#122731=CARTESIAN_POINT('Ctrl Pts',(54.6364229370494,-48.3343086880194,
12.));
#122732=CARTESIAN_POINT('Ctrl Pts',(54.6249433133261,-48.3113600422443,
0.));
#122733=CARTESIAN_POINT('Ctrl Pts',(54.6249433133261,-48.3113600422443,
12.));
#122734=CARTESIAN_POINT('Ctrl Pts',(54.6134594729959,-48.2884569360506,
0.));
#122735=CARTESIAN_POINT('Ctrl Pts',(54.6134594729959,-48.2884569360506,
12.));
#122736=CARTESIAN_POINT('Ctrl Pts',(54.6019715093309,-48.2655994366665,
0.));
#122737=CARTESIAN_POINT('Ctrl Pts',(54.6019715093309,-48.2655994366665,
12.));
#122738=CARTESIAN_POINT('Ctrl Pts',(54.5904795159926,-48.2427876114947,
0.));
#122739=CARTESIAN_POINT('Ctrl Pts',(54.5904795159926,-48.2427876114947,
12.));
#122740=CARTESIAN_POINT('Ctrl Pts',(54.5789835870342,-48.2200215281173,
0.));
#122741=CARTESIAN_POINT('Ctrl Pts',(54.5789835870342,-48.2200215281173,
12.));
#122742=CARTESIAN_POINT('Ctrl Pts',(54.5674838169041,-48.1973012542966,
0.));
#122743=CARTESIAN_POINT('Ctrl Pts',(54.5674838169041,-48.1973012542966,
12.));
#122744=CARTESIAN_POINT('Ctrl Pts',(54.5559803004492,-48.1746268579736,
0.));
#122745=CARTESIAN_POINT('Ctrl Pts',(54.5559803004492,-48.1746268579736,
12.));
#122746=CARTESIAN_POINT('Ctrl Pts',(54.5444731329201,-48.1519984072622,
0.));
#122747=CARTESIAN_POINT('Ctrl Pts',(54.5444731329201,-48.1519984072622,
12.));
#122748=CARTESIAN_POINT('Ctrl Pts',(54.5329624099721,-48.1294159704573,
0.));
#122749=CARTESIAN_POINT('Ctrl Pts',(54.5329624099721,-48.1294159704573,
12.));
#122750=CARTESIAN_POINT('Ctrl Pts',(54.5214482276678,-48.1068796160405,
0.));
#122751=CARTESIAN_POINT('Ctrl Pts',(54.5214482276678,-48.1068796160405,
12.));
#122752=CARTESIAN_POINT('Ctrl Pts',(54.5099306824786,-48.0843894126806,
0.));
#122753=CARTESIAN_POINT('Ctrl Pts',(54.5099306824786,-48.0843894126806,
12.));
#122754=CARTESIAN_POINT('Ctrl Pts',(54.4984098712886,-48.0619454292324,
0.));
#122755=CARTESIAN_POINT('Ctrl Pts',(54.4984098712886,-48.0619454292324,
12.));
#122756=CARTESIAN_POINT('Ctrl Pts',(54.4868858913971,-48.0395477347298,
0.));
#122757=CARTESIAN_POINT('Ctrl Pts',(54.4868858913971,-48.0395477347298,
12.));
#122758=CARTESIAN_POINT('Ctrl Pts',(54.4753588405215,-48.0171963983924,
0.));
#122759=CARTESIAN_POINT('Ctrl Pts',(54.4753588405215,-48.0171963983924,
12.));
#122760=CARTESIAN_POINT('Ctrl Pts',(54.4638288168003,-47.9948914896326,
0.));
#122761=CARTESIAN_POINT('Ctrl Pts',(54.4638288168003,-47.9948914896326,
12.));
#122762=CARTESIAN_POINT('Ctrl Pts',(54.4522959187955,-47.9726330780572,
0.));
#122763=CARTESIAN_POINT('Ctrl Pts',(54.4522959187955,-47.9726330780572,
12.));
#122764=CARTESIAN_POINT('Ctrl Pts',(54.4407602454967,-47.9504212334675,
0.));
#122765=CARTESIAN_POINT('Ctrl Pts',(54.4407602454967,-47.9504212334675,
12.));
#122766=CARTESIAN_POINT('Ctrl Pts',(54.429221896324,-47.9282560258516,0.));
#122767=CARTESIAN_POINT('Ctrl Pts',(54.429221896324,-47.9282560258516,12.));
#122768=CARTESIAN_POINT('Ctrl Pts',(54.4176809711311,-47.9061375253897,
0.));
#122769=CARTESIAN_POINT('Ctrl Pts',(54.4176809711311,-47.9061375253897,
12.));
#122770=CARTESIAN_POINT('Ctrl Pts',(54.4061375702079,-47.8840658024618,
0.));
#122771=CARTESIAN_POINT('Ctrl Pts',(54.4061375702079,-47.8840658024618,
12.));
#122772=CARTESIAN_POINT('Ctrl Pts',(54.3945917942832,-47.8620409276493,
0.));
#122773=CARTESIAN_POINT('Ctrl Pts',(54.3945917942832,-47.8620409276493,
12.));
#122774=CARTESIAN_POINT('Ctrl Pts',(54.3830437445278,-47.8400629717355,
0.));
#122775=CARTESIAN_POINT('Ctrl Pts',(54.3830437445278,-47.8400629717355,
12.));
#122776=CARTESIAN_POINT('Ctrl Pts',(54.3714935225591,-47.8181320056995,
0.));
#122777=CARTESIAN_POINT('Ctrl Pts',(54.3714935225591,-47.8181320056995,
12.));
#122778=CARTESIAN_POINT('Ctrl Pts',(54.3599412304437,-47.7962481007185,
0.));
#122779=CARTESIAN_POINT('Ctrl Pts',(54.3599412304437,-47.7962481007185,
12.));
#122780=CARTESIAN_POINT('Ctrl Pts',(54.3483869707002,-47.7744113281771,
0.));
#122781=CARTESIAN_POINT('Ctrl Pts',(54.3483869707002,-47.7744113281771,
12.));
#122782=CARTESIAN_POINT('Ctrl Pts',(54.3368308463023,-47.7526217596694,
0.));
#122783=CARTESIAN_POINT('Ctrl Pts',(54.3368308463023,-47.7526217596694,
12.));
#122784=CARTESIAN_POINT('Ctrl Pts',(54.3252729606823,-47.7308794669993,
0.));
#122785=CARTESIAN_POINT('Ctrl Pts',(54.3252729606823,-47.7308794669993,
12.));
#122786=CARTESIAN_POINT('Ctrl Pts',(54.3137134177345,-47.7091845221747,
0.));
#122787=CARTESIAN_POINT('Ctrl Pts',(54.3137134177345,-47.7091845221747,
12.));
#122788=CARTESIAN_POINT('Ctrl Pts',(54.302152321819,-47.6875369974087,0.));
#122789=CARTESIAN_POINT('Ctrl Pts',(54.302152321819,-47.6875369974087,12.));
#122790=CARTESIAN_POINT('Ctrl Pts',(54.290589777765,-47.6659369651301,0.));
#122791=CARTESIAN_POINT('Ctrl Pts',(54.290589777765,-47.6659369651301,12.));
#122792=CARTESIAN_POINT('Ctrl Pts',(54.2790258908738,-47.6443844979848,
0.));
#122793=CARTESIAN_POINT('Ctrl Pts',(54.2790258908738,-47.6443844979848,
12.));
#122794=CARTESIAN_POINT('Ctrl Pts',(54.2674607669226,-47.6228796688375,
0.));
#122795=CARTESIAN_POINT('Ctrl Pts',(54.2674607669226,-47.6228796688375,
12.));
#122796=CARTESIAN_POINT('Ctrl Pts',(54.2558945121678,-47.6014225507659,
0.));
#122797=CARTESIAN_POINT('Ctrl Pts',(54.2558945121678,-47.6014225507659,
12.));
#122798=CARTESIAN_POINT('Ctrl Pts',(54.244327233349,-47.5800132170608,0.));
#122799=CARTESIAN_POINT('Ctrl Pts',(54.244327233349,-47.5800132170608,12.));
#122800=CARTESIAN_POINT('Ctrl Pts',(54.2327590376924,-47.5586517412363,
0.));
#122801=CARTESIAN_POINT('Ctrl Pts',(54.2327590376924,-47.5586517412363,
12.));
#122802=CARTESIAN_POINT('Ctrl Pts',(54.2211900329138,-47.5373381970326,
0.));
#122803=CARTESIAN_POINT('Ctrl Pts',(54.2211900329138,-47.5373381970326,
12.));
#122804=CARTESIAN_POINT('Ctrl Pts',(54.209620327223,-47.5160726584174,0.));
#122805=CARTESIAN_POINT('Ctrl Pts',(54.209620327223,-47.5160726584174,12.));
#122806=CARTESIAN_POINT('Ctrl Pts',(54.198050029327,-47.4948551995801,0.));
#122807=CARTESIAN_POINT('Ctrl Pts',(54.198050029327,-47.4948551995801,12.));
#122808=CARTESIAN_POINT('Ctrl Pts',(54.1864792484345,-47.4736858949322,
0.));
#122809=CARTESIAN_POINT('Ctrl Pts',(54.1864792484345,-47.4736858949322,
12.));
#122810=CARTESIAN_POINT('Ctrl Pts',(54.1749080942593,-47.4525648191173,
0.));
#122811=CARTESIAN_POINT('Ctrl Pts',(54.1749080942593,-47.4525648191173,
12.));
#122812=CARTESIAN_POINT('Ctrl Pts',(54.1633366770239,-47.4314920470141,
0.));
#122813=CARTESIAN_POINT('Ctrl Pts',(54.1633366770239,-47.4314920470141,
12.));
#122814=CARTESIAN_POINT('Ctrl Pts',(54.1517651074637,-47.4104676537381,
0.));
#122815=CARTESIAN_POINT('Ctrl Pts',(54.1517651074637,-47.4104676537381,
12.));
#122816=CARTESIAN_POINT('Ctrl Pts',(54.1401934968311,-47.3894917146365,
0.));
#122817=CARTESIAN_POINT('Ctrl Pts',(54.1401934968311,-47.3894917146365,
12.));
#122818=CARTESIAN_POINT('Ctrl Pts',(54.1286219568989,-47.3685643052874,
0.));
#122819=CARTESIAN_POINT('Ctrl Pts',(54.1286219568989,-47.3685643052874,
12.));
#122820=CARTESIAN_POINT('Ctrl Pts',(54.1170505999645,-47.3476855015102,
0.));
#122821=CARTESIAN_POINT('Ctrl Pts',(54.1170505999645,-47.3476855015102,
12.));
#122822=CARTESIAN_POINT('Ctrl Pts',(54.1054795388543,-47.3268553793694,
0.));
#122823=CARTESIAN_POINT('Ctrl Pts',(54.1054795388543,-47.3268553793694,
12.));
#122824=CARTESIAN_POINT('Ctrl Pts',(54.0939088869268,-47.3060740151752,
0.));
#122825=CARTESIAN_POINT('Ctrl Pts',(54.0939088869268,-47.3060740151752,
12.));
#122826=CARTESIAN_POINT('Ctrl Pts',(54.0823387580776,-47.2853414854793,
0.));
#122827=CARTESIAN_POINT('Ctrl Pts',(54.0823387580776,-47.2853414854793,
12.));
#122828=CARTESIAN_POINT('Ctrl Pts',(54.0707692667438,-47.2646578670746,
0.));
#122829=CARTESIAN_POINT('Ctrl Pts',(54.0707692667438,-47.2646578670746,
12.));
#122830=CARTESIAN_POINT('Ctrl Pts',(54.0592005279086,-47.2440232370065,
0.));
#122831=CARTESIAN_POINT('Ctrl Pts',(54.0592005279086,-47.2440232370065,
12.));
#122832=CARTESIAN_POINT('Ctrl Pts',(54.047632657104,-47.2234376725743,0.));
#122833=CARTESIAN_POINT('Ctrl Pts',(54.047632657104,-47.2234376725743,12.));
#122834=CARTESIAN_POINT('Ctrl Pts',(54.0360657704163,-47.202901251334,0.));
#122835=CARTESIAN_POINT('Ctrl Pts',(54.0360657704163,-47.202901251334,12.));
#122836=CARTESIAN_POINT('Ctrl Pts',(54.0244999844893,-47.1824140510926,
0.));
#122837=CARTESIAN_POINT('Ctrl Pts',(54.0244999844893,-47.1824140510926,
12.));
#122838=CARTESIAN_POINT('Ctrl Pts',(54.0129354165297,-47.1619761499087,
0.));
#122839=CARTESIAN_POINT('Ctrl Pts',(54.0129354165297,-47.1619761499087,
12.));
#122840=CARTESIAN_POINT('Ctrl Pts',(54.0013721843118,-47.1415876261035,
0.));
#122841=CARTESIAN_POINT('Ctrl Pts',(54.0013721843118,-47.1415876261035,
12.));
#122842=CARTESIAN_POINT('Ctrl Pts',(53.989810406182,-47.1212485582643,0.));
#122843=CARTESIAN_POINT('Ctrl Pts',(53.989810406182,-47.1212485582643,12.));
#122844=CARTESIAN_POINT('Ctrl Pts',(53.9782502010634,-47.1009590252458,
0.));
#122845=CARTESIAN_POINT('Ctrl Pts',(53.9782502010634,-47.1009590252458,
12.));
#122846=CARTESIAN_POINT('Ctrl Pts',(53.9666916884596,-47.0807191061648,
0.));
#122847=CARTESIAN_POINT('Ctrl Pts',(53.9666916884596,-47.0807191061648,
12.));
#122848=CARTESIAN_POINT('Ctrl Pts',(53.9551349884599,-47.0605288804008,
0.));
#122849=CARTESIAN_POINT('Ctrl Pts',(53.9551349884599,-47.0605288804008,
12.));
#122850=CARTESIAN_POINT('Ctrl Pts',(53.9435802217436,-47.0403884276072,
0.));
#122851=CARTESIAN_POINT('Ctrl Pts',(53.9435802217436,-47.0403884276072,
12.));
#122852=CARTESIAN_POINT('Ctrl Pts',(53.9320275095853,-47.0202978277138,
0.));
#122853=CARTESIAN_POINT('Ctrl Pts',(53.9320275095853,-47.0202978277138,
12.));
#122854=CARTESIAN_POINT('Ctrl Pts',(53.9204769738596,-47.0002571609297,
0.));
#122855=CARTESIAN_POINT('Ctrl Pts',(53.9204769738596,-47.0002571609297,
12.));
#122856=CARTESIAN_POINT('Ctrl Pts',(53.9089287370463,-46.9802665077366,
0.));
#122857=CARTESIAN_POINT('Ctrl Pts',(53.9089287370463,-46.9802665077366,
12.));
#122858=CARTESIAN_POINT('Ctrl Pts',(53.8973829222347,-46.9603259488921,
0.));
#122859=CARTESIAN_POINT('Ctrl Pts',(53.8973829222347,-46.9603259488921,
12.));
#122860=CARTESIAN_POINT('Ctrl Pts',(53.8858396531298,-46.9404355654401,
0.));
#122861=CARTESIAN_POINT('Ctrl Pts',(53.8858396531298,-46.9404355654401,
12.));
#122862=CARTESIAN_POINT('Ctrl Pts',(53.8742990540563,-46.9205954387133,
0.));
#122863=CARTESIAN_POINT('Ctrl Pts',(53.8742990540563,-46.9205954387133,
12.));
#122864=CARTESIAN_POINT('Ctrl Pts',(53.8627612499638,-46.9008056503351,
0.));
#122865=CARTESIAN_POINT('Ctrl Pts',(53.8627612499638,-46.9008056503351,
12.));
#122866=CARTESIAN_POINT('Ctrl Pts',(53.8512263664321,-46.881066282213,0.));
#122867=CARTESIAN_POINT('Ctrl Pts',(53.8512263664321,-46.881066282213,12.));
#122868=CARTESIAN_POINT('Ctrl Pts',(53.8396945296757,-46.8613774165435,
0.));
#122869=CARTESIAN_POINT('Ctrl Pts',(53.8396945296757,-46.8613774165435,
12.));
#122870=CARTESIAN_POINT('Ctrl Pts',(53.8281658665503,-46.841739135822,0.));
#122871=CARTESIAN_POINT('Ctrl Pts',(53.8281658665503,-46.841739135822,12.));
#122872=CARTESIAN_POINT('Ctrl Pts',(53.816640504558,-46.8221515228457,0.));
#122873=CARTESIAN_POINT('Ctrl Pts',(53.816640504558,-46.8221515228457,12.));
#122874=CARTESIAN_POINT('Ctrl Pts',(53.8051185718532,-46.802614660715,0.));
#122875=CARTESIAN_POINT('Ctrl Pts',(53.8051185718532,-46.802614660715,12.));
#122876=CARTESIAN_POINT('Ctrl Pts',(53.793600197248,-46.7831286328278,0.));
#122877=CARTESIAN_POINT('Ctrl Pts',(53.793600197248,-46.7831286328278,12.));
#122878=CARTESIAN_POINT('Ctrl Pts',(53.7820855102182,-46.7636935228861,
0.));
#122879=CARTESIAN_POINT('Ctrl Pts',(53.7820855102182,-46.7636935228861,
12.));
#122880=CARTESIAN_POINT('Ctrl Pts',(53.7705746409075,-46.7443094149045,
0.));
#122881=CARTESIAN_POINT('Ctrl Pts',(53.7705746409075,-46.7443094149045,
12.));
#122882=CARTESIAN_POINT('Ctrl Pts',(53.7590677201342,-46.7249763932129,
0.));
#122883=CARTESIAN_POINT('Ctrl Pts',(53.7590677201342,-46.7249763932129,
12.));
#122884=CARTESIAN_POINT('Ctrl Pts',(53.7475648793946,-46.7056945424559,
0.));
#122885=CARTESIAN_POINT('Ctrl Pts',(53.7475648793946,-46.7056945424559,
12.));
#122886=CARTESIAN_POINT('Ctrl Pts',(53.7360662508675,-46.6864639475862,
0.));
#122887=CARTESIAN_POINT('Ctrl Pts',(53.7360662508675,-46.6864639475862,
12.));
#122888=CARTESIAN_POINT('Ctrl Pts',(53.7245719674221,-46.6672846938752,
0.));
#122889=CARTESIAN_POINT('Ctrl Pts',(53.7245719674221,-46.6672846938752,
12.));
#122890=CARTESIAN_POINT('Ctrl Pts',(53.7130821626262,-46.6481568669217,
0.));
#122891=CARTESIAN_POINT('Ctrl Pts',(53.7130821626262,-46.6481568669217,
12.));
#122892=CARTESIAN_POINT('Ctrl Pts',(53.7015969707541,-46.6290805526559,
0.));
#122893=CARTESIAN_POINT('Ctrl Pts',(53.7015969707541,-46.6290805526559,
12.));
#122894=CARTESIAN_POINT('Ctrl Pts',(53.690116526794,-46.6100558373401,0.));
#122895=CARTESIAN_POINT('Ctrl Pts',(53.690116526794,-46.6100558373401,12.));
#122896=CARTESIAN_POINT('Ctrl Pts',(53.678640966456,-46.5910828075652,0.));
#122897=CARTESIAN_POINT('Ctrl Pts',(53.678640966456,-46.5910828075652,12.));
#122898=CARTESIAN_POINT('Ctrl Pts',(53.6671704261735,-46.572161550259,0.));
#122899=CARTESIAN_POINT('Ctrl Pts',(53.6671704261735,-46.572161550259,12.));
#122900=CARTESIAN_POINT('Ctrl Pts',(53.6557050431069,-46.5532921526899,
0.));
#122901=CARTESIAN_POINT('Ctrl Pts',(53.6557050431069,-46.5532921526899,
12.));
#122902=CARTESIAN_POINT('Ctrl Pts',(53.6442449551455,-46.5344747024677,
0.));
#122903=CARTESIAN_POINT('Ctrl Pts',(53.6442449551455,-46.5344747024677,
12.));
#122904=CARTESIAN_POINT('Ctrl Pts',(53.6327903009097,-46.5157092875377,
0.));
#122905=CARTESIAN_POINT('Ctrl Pts',(53.6327903009097,-46.5157092875377,
12.));
#122906=CARTESIAN_POINT('Ctrl Pts',(53.6213412197542,-46.4969959961779,
0.));
#122907=CARTESIAN_POINT('Ctrl Pts',(53.6213412197542,-46.4969959961779,
12.));
#122908=CARTESIAN_POINT('Ctrl Pts',(53.6098978517869,-46.4783349170182,
0.));
#122909=CARTESIAN_POINT('Ctrl Pts',(53.6098978517869,-46.4783349170182,
12.));
#122910=CARTESIAN_POINT('Ctrl Pts',(53.5984603378861,-46.4597261390526,
0.));
#122911=CARTESIAN_POINT('Ctrl Pts',(53.5984603378861,-46.4597261390526,
12.));
#122912=CARTESIAN_POINT('Ctrl Pts',(53.5870288197161,-46.4411697516474,
0.));
#122913=CARTESIAN_POINT('Ctrl Pts',(53.5870288197161,-46.4411697516474,
12.));
#122914=CARTESIAN_POINT('Ctrl Pts',(53.5756034397464,-46.422665844546,0.));
#122915=CARTESIAN_POINT('Ctrl Pts',(53.5756034397464,-46.422665844546,12.));
#122916=CARTESIAN_POINT('Ctrl Pts',(53.5641843412537,-46.4042145078682,
0.));
#122917=CARTESIAN_POINT('Ctrl Pts',(53.5641843412537,-46.4042145078682,
12.));
#122918=CARTESIAN_POINT('Ctrl Pts',(53.5527716683029,-46.3858158321044,
0.));
#122919=CARTESIAN_POINT('Ctrl Pts',(53.5527716683029,-46.3858158321044,
12.));
#122920=CARTESIAN_POINT('Ctrl Pts',(53.5413655657323,-46.3674699081043,
0.));
#122921=CARTESIAN_POINT('Ctrl Pts',(53.5413655657323,-46.3674699081043,
12.));
#122922=CARTESIAN_POINT('Ctrl Pts',(53.5299661791396,-46.3491768270664,
0.));
#122923=CARTESIAN_POINT('Ctrl Pts',(53.5299661791396,-46.3491768270664,
12.));
#122924=CARTESIAN_POINT('Ctrl Pts',(53.518573654857,-46.3309366805112,0.));
#122925=CARTESIAN_POINT('Ctrl Pts',(53.518573654857,-46.3309366805112,12.));
#122926=CARTESIAN_POINT('Ctrl Pts',(53.5071881399932,-46.3127495603117,
0.));
#122927=CARTESIAN_POINT('Ctrl Pts',(53.5071881399932,-46.3127495603117,
12.));
#122928=CARTESIAN_POINT('Ctrl Pts',(53.4958097825019,-46.2946155587428,
0.));
#122929=CARTESIAN_POINT('Ctrl Pts',(53.4958097825019,-46.2946155587428,
12.));
#122930=CARTESIAN_POINT('Ctrl Pts',(53.4844387312414,-46.2765347685198,
0.));
#122931=CARTESIAN_POINT('Ctrl Pts',(53.4844387312414,-46.2765347685198,
12.));
#122932=CARTESIAN_POINT('Ctrl Pts',(53.4730751360359,-46.2585072828343,
0.));
#122933=CARTESIAN_POINT('Ctrl Pts',(53.4730751360359,-46.2585072828343,
12.));
#122934=CARTESIAN_POINT('Ctrl Pts',(53.4617191477382,-46.2405331953872,
0.));
#122935=CARTESIAN_POINT('Ctrl Pts',(53.4617191477382,-46.2405331953872,
12.));
#122936=CARTESIAN_POINT('Ctrl Pts',(53.4503709181158,-46.2226126003185,
0.));
#122937=CARTESIAN_POINT('Ctrl Pts',(53.4503709181158,-46.2226126003185,
12.));
#122938=CARTESIAN_POINT('Ctrl Pts',(53.4390305997263,-46.2047455921276,
0.));
#122939=CARTESIAN_POINT('Ctrl Pts',(53.4390305997263,-46.2047455921276,
12.));
#122940=CARTESIAN_POINT('Ctrl Pts',(53.4276983458129,-46.1869322656027,
0.));
#122941=CARTESIAN_POINT('Ctrl Pts',(53.4276983458129,-46.1869322656027,
12.));
#122942=CARTESIAN_POINT('Ctrl Pts',(53.4163743101534,-46.1691727157149,
0.));
#122943=CARTESIAN_POINT('Ctrl Pts',(53.4163743101534,-46.1691727157149,
12.));
#122944=CARTESIAN_POINT('Ctrl Pts',(53.4050586470463,-46.1514670376035,
0.));
#122945=CARTESIAN_POINT('Ctrl Pts',(53.4050586470463,-46.1514670376035,
12.));
#122946=CARTESIAN_POINT('Ctrl Pts',(53.3937515116572,-46.1338153268116,
0.));
#122947=CARTESIAN_POINT('Ctrl Pts',(53.3937515116572,-46.1338153268116,
12.));
#122948=CARTESIAN_POINT('Ctrl Pts',(53.3824530603284,-46.1162176794891,
0.));
#122949=CARTESIAN_POINT('Ctrl Pts',(53.3824530603284,-46.1162176794891,
12.));
#122950=CARTESIAN_POINT('Ctrl Pts',(53.3711634508426,-46.0986741925646,
0.));
#122951=CARTESIAN_POINT('Ctrl Pts',(53.3711634508426,-46.0986741925646,
12.));
#122952=CARTESIAN_POINT('Ctrl Pts',(53.3598828428519,-46.0811849640195,
0.));
#122953=CARTESIAN_POINT('Ctrl Pts',(53.3598828428519,-46.0811849640195,
12.));
#122954=CARTESIAN_POINT('Ctrl Pts',(53.3486113975868,-46.0637500926954,
0.));
#122955=CARTESIAN_POINT('Ctrl Pts',(53.3486113975868,-46.0637500926954,
12.));
#122956=CARTESIAN_POINT('Ctrl Pts',(53.3373492770647,-46.046369677778,0.));
#122957=CARTESIAN_POINT('Ctrl Pts',(53.3373492770647,-46.046369677778,12.));
#122958=CARTESIAN_POINT('Ctrl Pts',(53.3260966434277,-46.0290438183598,
0.));
#122959=CARTESIAN_POINT('Ctrl Pts',(53.3260966434277,-46.0290438183598,
12.));
#122960=CARTESIAN_POINT('Ctrl Pts',(53.3148536582658,-46.0117726129893,
0.));
#122961=CARTESIAN_POINT('Ctrl Pts',(53.3148536582658,-46.0117726129893,
12.));
#122962=CARTESIAN_POINT('Ctrl Pts',(53.3036204818367,-45.9945561591486,
0.));
#122963=CARTESIAN_POINT('Ctrl Pts',(53.3036204818367,-45.9945561591486,
12.));
#122964=CARTESIAN_POINT('Ctrl Pts',(53.2923972745585,-45.9773945542415,
0.));
#122965=CARTESIAN_POINT('Ctrl Pts',(53.2923972745585,-45.9773945542415,
12.));
#122966=CARTESIAN_POINT('Ctrl Pts',(53.2811841987945,-45.9602878967715,
0.));
#122967=CARTESIAN_POINT('Ctrl Pts',(53.2811841987945,-45.9602878967715,
12.));
#122968=CARTESIAN_POINT('Ctrl Pts',(53.2699814203097,-45.9432362873001,
0.));
#122969=CARTESIAN_POINT('Ctrl Pts',(53.2699814203097,-45.9432362873001,
12.));
#122970=CARTESIAN_POINT('Ctrl Pts',(53.2587891103835,-45.9262398298323,
0.));
#122971=CARTESIAN_POINT('Ctrl Pts',(53.2587891103835,-45.9262398298323,
12.));
#122972=CARTESIAN_POINT('Ctrl Pts',(53.2476074459977,-45.9092986319343,
0.));
#122973=CARTESIAN_POINT('Ctrl Pts',(53.2476074459977,-45.9092986319343,
12.));
#122974=CARTESIAN_POINT('Ctrl Pts',(53.2364366054276,-45.8924128018354,
0.));
#122975=CARTESIAN_POINT('Ctrl Pts',(53.2364366054276,-45.8924128018354,
12.));
#122976=CARTESIAN_POINT('Ctrl Pts',(53.2252767643652,-45.8755824458715,
0.));
#122977=CARTESIAN_POINT('Ctrl Pts',(53.2252767643652,-45.8755824458715,
12.));
#122978=CARTESIAN_POINT('Ctrl Pts',(53.2141280925458,-45.8588076662598,
0.));
#122979=CARTESIAN_POINT('Ctrl Pts',(53.2141280925458,-45.8588076662598,
12.));
#122980=CARTESIAN_POINT('Ctrl Pts',(53.2029907483602,-45.8420885575386,
0.));
#122981=CARTESIAN_POINT('Ctrl Pts',(53.2029907483602,-45.8420885575386,
12.));
#122982=CARTESIAN_POINT('Ctrl Pts',(53.1918648840598,-45.8254252100003,
0.));
#122983=CARTESIAN_POINT('Ctrl Pts',(53.1918648840598,-45.8254252100003,
12.));
#122984=CARTESIAN_POINT('Ctrl Pts',(53.1807506560977,-45.8088177165124,
0.));
#122985=CARTESIAN_POINT('Ctrl Pts',(53.1807506560977,-45.8088177165124,
12.));
#122986=CARTESIAN_POINT('Ctrl Pts',(53.1696482334487,-45.7922661780005,
0.));
#122987=CARTESIAN_POINT('Ctrl Pts',(53.1696482334487,-45.7922661780005,
12.));
#122988=CARTESIAN_POINT('Ctrl Pts',(53.158557807638,-45.7757707100568,0.));
#122989=CARTESIAN_POINT('Ctrl Pts',(53.158557807638,-45.7757707100568,12.));
#122990=CARTESIAN_POINT('Ctrl Pts',(53.147479599594,-45.7593314474413,0.));
#122991=CARTESIAN_POINT('Ctrl Pts',(53.147479599594,-45.7593314474413,12.));
#122992=CARTESIAN_POINT('Ctrl Pts',(53.136413838457,-45.7429485300727,0.));
#122993=CARTESIAN_POINT('Ctrl Pts',(53.136413838457,-45.7429485300727,12.));
#122994=CARTESIAN_POINT('Ctrl Pts',(53.1253607414806,-45.7266220896951,
0.));
#122995=CARTESIAN_POINT('Ctrl Pts',(53.1253607414806,-45.7266220896951,
12.));
#122996=CARTESIAN_POINT('Ctrl Pts',(53.1143204954981,-45.7103522376744,
0.));
#122997=CARTESIAN_POINT('Ctrl Pts',(53.1143204954981,-45.7103522376744,
12.));
#122998=CARTESIAN_POINT('Ctrl Pts',(53.1032932329074,-45.6941390489239,
0.));
#122999=CARTESIAN_POINT('Ctrl Pts',(53.1032932329074,-45.6941390489239,
12.));
#123000=CARTESIAN_POINT('Ctrl Pts',(53.0922790298736,-45.6779825614486,
0.));
#123001=CARTESIAN_POINT('Ctrl Pts',(53.0922790298736,-45.6779825614486,
12.));
#123002=CARTESIAN_POINT('Ctrl Pts',(53.083478145185,-45.665102743948,0.));
#123003=CARTESIAN_POINT('Ctrl Pts',(53.083478145185,-45.665102743948,12.));
#123004=CARTESIAN_POINT('Ctrl Pts',(53.0768833804386,-45.6554684028296,
0.));
#123005=CARTESIAN_POINT('Ctrl Pts',(53.0768833804386,-45.6554684028296,
12.));
#123006=CARTESIAN_POINT('Ctrl Pts',(53.0724894921921,-45.6490568514146,
0.));
#123007=CARTESIAN_POINT('Ctrl Pts',(53.0724894921921,-45.6490568514146,
12.));
#123008=CARTESIAN_POINT('Ctrl Pts',(53.0702932034641,-45.6458539113724,
0.));
#123009=CARTESIAN_POINT('Ctrl Pts',(53.0702932034641,-45.6458539113724,
12.));
#123010=CARTESIAN_POINT('',(53.0702932034641,-45.6458539113724,12.));
#123011=CARTESIAN_POINT('Ctrl Pts',(53.0702932034641,-45.6458539113724,
12.));
#123012=CARTESIAN_POINT('Ctrl Pts',(53.0724894921921,-45.6490568514146,
12.));
#123013=CARTESIAN_POINT('Ctrl Pts',(53.0768833804386,-45.6554684028296,
12.));
#123014=CARTESIAN_POINT('Ctrl Pts',(53.083478145185,-45.665102743948,12.));
#123015=CARTESIAN_POINT('Ctrl Pts',(53.0922790298736,-45.6779825614486,
12.));
#123016=CARTESIAN_POINT('Ctrl Pts',(53.1032932329074,-45.6941390489239,
12.));
#123017=CARTESIAN_POINT('Ctrl Pts',(53.1143204954981,-45.7103522376744,
12.));
#123018=CARTESIAN_POINT('Ctrl Pts',(53.1253607414806,-45.7266220896951,
12.));
#123019=CARTESIAN_POINT('Ctrl Pts',(53.136413838457,-45.7429485300727,12.));
#123020=CARTESIAN_POINT('Ctrl Pts',(53.147479599594,-45.7593314474413,12.));
#123021=CARTESIAN_POINT('Ctrl Pts',(53.158557807638,-45.7757707100568,12.));
#123022=CARTESIAN_POINT('Ctrl Pts',(53.1696482334487,-45.7922661780005,
12.));
#123023=CARTESIAN_POINT('Ctrl Pts',(53.1807506560977,-45.8088177165124,
12.));
#123024=CARTESIAN_POINT('Ctrl Pts',(53.1918648840598,-45.8254252100003,
12.));
#123025=CARTESIAN_POINT('Ctrl Pts',(53.2029907483602,-45.8420885575386,
12.));
#123026=CARTESIAN_POINT('Ctrl Pts',(53.2141280925458,-45.8588076662598,
12.));
#123027=CARTESIAN_POINT('Ctrl Pts',(53.2252767643652,-45.8755824458715,
12.));
#123028=CARTESIAN_POINT('Ctrl Pts',(53.2364366054276,-45.8924128018354,
12.));
#123029=CARTESIAN_POINT('Ctrl Pts',(53.2476074459977,-45.9092986319343,
12.));
#123030=CARTESIAN_POINT('Ctrl Pts',(53.2587891103835,-45.9262398298323,
12.));
#123031=CARTESIAN_POINT('Ctrl Pts',(53.2699814203097,-45.9432362873001,
12.));
#123032=CARTESIAN_POINT('Ctrl Pts',(53.2811841987945,-45.9602878967715,
12.));
#123033=CARTESIAN_POINT('Ctrl Pts',(53.2923972745585,-45.9773945542415,
12.));
#123034=CARTESIAN_POINT('Ctrl Pts',(53.3036204818367,-45.9945561591486,
12.));
#123035=CARTESIAN_POINT('Ctrl Pts',(53.3148536582658,-46.0117726129893,
12.));
#123036=CARTESIAN_POINT('Ctrl Pts',(53.3260966434277,-46.0290438183598,
12.));
#123037=CARTESIAN_POINT('Ctrl Pts',(53.3373492770647,-46.046369677778,12.));
#123038=CARTESIAN_POINT('Ctrl Pts',(53.3486113975868,-46.0637500926954,
12.));
#123039=CARTESIAN_POINT('Ctrl Pts',(53.3598828428519,-46.0811849640195,
12.));
#123040=CARTESIAN_POINT('Ctrl Pts',(53.3711634508426,-46.0986741925646,
12.));
#123041=CARTESIAN_POINT('Ctrl Pts',(53.3824530603284,-46.1162176794891,
12.));
#123042=CARTESIAN_POINT('Ctrl Pts',(53.3937515116572,-46.1338153268116,
12.));
#123043=CARTESIAN_POINT('Ctrl Pts',(53.4050586470463,-46.1514670376035,
12.));
#123044=CARTESIAN_POINT('Ctrl Pts',(53.4163743101534,-46.1691727157149,
12.));
#123045=CARTESIAN_POINT('Ctrl Pts',(53.4276983458129,-46.1869322656027,
12.));
#123046=CARTESIAN_POINT('Ctrl Pts',(53.4390305997263,-46.2047455921276,
12.));
#123047=CARTESIAN_POINT('Ctrl Pts',(53.4503709181158,-46.2226126003185,
12.));
#123048=CARTESIAN_POINT('Ctrl Pts',(53.4617191477382,-46.2405331953872,
12.));
#123049=CARTESIAN_POINT('Ctrl Pts',(53.4730751360359,-46.2585072828343,
12.));
#123050=CARTESIAN_POINT('Ctrl Pts',(53.4844387312414,-46.2765347685198,
12.));
#123051=CARTESIAN_POINT('Ctrl Pts',(53.4958097825019,-46.2946155587428,
12.));
#123052=CARTESIAN_POINT('Ctrl Pts',(53.5071881399932,-46.3127495603117,
12.));
#123053=CARTESIAN_POINT('Ctrl Pts',(53.518573654857,-46.3309366805112,12.));
#123054=CARTESIAN_POINT('Ctrl Pts',(53.5299661791396,-46.3491768270664,
12.));
#123055=CARTESIAN_POINT('Ctrl Pts',(53.5413655657323,-46.3674699081043,
12.));
#123056=CARTESIAN_POINT('Ctrl Pts',(53.5527716683029,-46.3858158321044,
12.));
#123057=CARTESIAN_POINT('Ctrl Pts',(53.5641843412537,-46.4042145078682,
12.));
#123058=CARTESIAN_POINT('Ctrl Pts',(53.5756034397464,-46.422665844546,12.));
#123059=CARTESIAN_POINT('Ctrl Pts',(53.5870288197161,-46.4411697516474,
12.));
#123060=CARTESIAN_POINT('Ctrl Pts',(53.5984603378861,-46.4597261390526,
12.));
#123061=CARTESIAN_POINT('Ctrl Pts',(53.6098978517869,-46.4783349170182,
12.));
#123062=CARTESIAN_POINT('Ctrl Pts',(53.6213412197542,-46.4969959961779,
12.));
#123063=CARTESIAN_POINT('Ctrl Pts',(53.6327903009097,-46.5157092875377,
12.));
#123064=CARTESIAN_POINT('Ctrl Pts',(53.6442449551455,-46.5344747024677,
12.));
#123065=CARTESIAN_POINT('Ctrl Pts',(53.6557050431069,-46.5532921526899,
12.));
#123066=CARTESIAN_POINT('Ctrl Pts',(53.6671704261735,-46.572161550259,12.));
#123067=CARTESIAN_POINT('Ctrl Pts',(53.678640966456,-46.5910828075652,12.));
#123068=CARTESIAN_POINT('Ctrl Pts',(53.690116526794,-46.6100558373401,12.));
#123069=CARTESIAN_POINT('Ctrl Pts',(53.7015969707541,-46.6290805526559,
12.));
#123070=CARTESIAN_POINT('Ctrl Pts',(53.7130821626262,-46.6481568669217,
12.));
#123071=CARTESIAN_POINT('Ctrl Pts',(53.7245719674221,-46.6672846938752,
12.));
#123072=CARTESIAN_POINT('Ctrl Pts',(53.7360662508675,-46.6864639475862,
12.));
#123073=CARTESIAN_POINT('Ctrl Pts',(53.7475648793946,-46.7056945424559,
12.));
#123074=CARTESIAN_POINT('Ctrl Pts',(53.7590677201342,-46.7249763932129,
12.));
#123075=CARTESIAN_POINT('Ctrl Pts',(53.7705746409075,-46.7443094149045,
12.));
#123076=CARTESIAN_POINT('Ctrl Pts',(53.7820855102182,-46.7636935228861,
12.));
#123077=CARTESIAN_POINT('Ctrl Pts',(53.793600197248,-46.7831286328278,12.));
#123078=CARTESIAN_POINT('Ctrl Pts',(53.8051185718532,-46.802614660715,12.));
#123079=CARTESIAN_POINT('Ctrl Pts',(53.816640504558,-46.8221515228457,12.));
#123080=CARTESIAN_POINT('Ctrl Pts',(53.8281658665503,-46.841739135822,12.));
#123081=CARTESIAN_POINT('Ctrl Pts',(53.8396945296757,-46.8613774165435,
12.));
#123082=CARTESIAN_POINT('Ctrl Pts',(53.8512263664321,-46.881066282213,12.));
#123083=CARTESIAN_POINT('Ctrl Pts',(53.8627612499638,-46.9008056503351,
12.));
#123084=CARTESIAN_POINT('Ctrl Pts',(53.8742990540563,-46.9205954387133,
12.));
#123085=CARTESIAN_POINT('Ctrl Pts',(53.8858396531298,-46.9404355654401,
12.));
#123086=CARTESIAN_POINT('Ctrl Pts',(53.8973829222347,-46.9603259488921,
12.));
#123087=CARTESIAN_POINT('Ctrl Pts',(53.9089287370463,-46.9802665077366,
12.));
#123088=CARTESIAN_POINT('Ctrl Pts',(53.9204769738596,-47.0002571609297,
12.));
#123089=CARTESIAN_POINT('Ctrl Pts',(53.9320275095853,-47.0202978277138,
12.));
#123090=CARTESIAN_POINT('Ctrl Pts',(53.9435802217436,-47.0403884276072,
12.));
#123091=CARTESIAN_POINT('Ctrl Pts',(53.9551349884599,-47.0605288804008,
12.));
#123092=CARTESIAN_POINT('Ctrl Pts',(53.9666916884596,-47.0807191061648,
12.));
#123093=CARTESIAN_POINT('Ctrl Pts',(53.9782502010634,-47.1009590252458,
12.));
#123094=CARTESIAN_POINT('Ctrl Pts',(53.989810406182,-47.1212485582643,12.));
#123095=CARTESIAN_POINT('Ctrl Pts',(54.0013721843118,-47.1415876261035,
12.));
#123096=CARTESIAN_POINT('Ctrl Pts',(54.0129354165297,-47.1619761499087,
12.));
#123097=CARTESIAN_POINT('Ctrl Pts',(54.0244999844893,-47.1824140510926,
12.));
#123098=CARTESIAN_POINT('Ctrl Pts',(54.0360657704163,-47.202901251334,12.));
#123099=CARTESIAN_POINT('Ctrl Pts',(54.047632657104,-47.2234376725743,12.));
#123100=CARTESIAN_POINT('Ctrl Pts',(54.0592005279086,-47.2440232370065,
12.));
#123101=CARTESIAN_POINT('Ctrl Pts',(54.0707692667438,-47.2646578670746,
12.));
#123102=CARTESIAN_POINT('Ctrl Pts',(54.0823387580776,-47.2853414854793,
12.));
#123103=CARTESIAN_POINT('Ctrl Pts',(54.0939088869268,-47.3060740151752,
12.));
#123104=CARTESIAN_POINT('Ctrl Pts',(54.1054795388543,-47.3268553793694,
12.));
#123105=CARTESIAN_POINT('Ctrl Pts',(54.1170505999645,-47.3476855015102,
12.));
#123106=CARTESIAN_POINT('Ctrl Pts',(54.1286219568989,-47.3685643052874,
12.));
#123107=CARTESIAN_POINT('Ctrl Pts',(54.1401934968311,-47.3894917146365,
12.));
#123108=CARTESIAN_POINT('Ctrl Pts',(54.1517651074637,-47.4104676537381,
12.));
#123109=CARTESIAN_POINT('Ctrl Pts',(54.1633366770239,-47.4314920470141,
12.));
#123110=CARTESIAN_POINT('Ctrl Pts',(54.1749080942593,-47.4525648191173,
12.));
#123111=CARTESIAN_POINT('Ctrl Pts',(54.1864792484345,-47.4736858949322,
12.));
#123112=CARTESIAN_POINT('Ctrl Pts',(54.198050029327,-47.4948551995801,12.));
#123113=CARTESIAN_POINT('Ctrl Pts',(54.209620327223,-47.5160726584174,12.));
#123114=CARTESIAN_POINT('Ctrl Pts',(54.2211900329138,-47.5373381970326,
12.));
#123115=CARTESIAN_POINT('Ctrl Pts',(54.2327590376924,-47.5586517412363,
12.));
#123116=CARTESIAN_POINT('Ctrl Pts',(54.244327233349,-47.5800132170608,12.));
#123117=CARTESIAN_POINT('Ctrl Pts',(54.2558945121678,-47.6014225507659,
12.));
#123118=CARTESIAN_POINT('Ctrl Pts',(54.2674607669226,-47.6228796688375,
12.));
#123119=CARTESIAN_POINT('Ctrl Pts',(54.2790258908738,-47.6443844979848,
12.));
#123120=CARTESIAN_POINT('Ctrl Pts',(54.290589777765,-47.6659369651301,12.));
#123121=CARTESIAN_POINT('Ctrl Pts',(54.302152321819,-47.6875369974087,12.));
#123122=CARTESIAN_POINT('Ctrl Pts',(54.3137134177345,-47.7091845221747,
12.));
#123123=CARTESIAN_POINT('Ctrl Pts',(54.3252729606823,-47.7308794669993,
12.));
#123124=CARTESIAN_POINT('Ctrl Pts',(54.3368308463023,-47.7526217596694,
12.));
#123125=CARTESIAN_POINT('Ctrl Pts',(54.3483869707002,-47.7744113281771,
12.));
#123126=CARTESIAN_POINT('Ctrl Pts',(54.3599412304437,-47.7962481007185,
12.));
#123127=CARTESIAN_POINT('Ctrl Pts',(54.3714935225591,-47.8181320056995,
12.));
#123128=CARTESIAN_POINT('Ctrl Pts',(54.3830437445278,-47.8400629717355,
12.));
#123129=CARTESIAN_POINT('Ctrl Pts',(54.3945917942832,-47.8620409276493,
12.));
#123130=CARTESIAN_POINT('Ctrl Pts',(54.4061375702079,-47.8840658024618,
12.));
#123131=CARTESIAN_POINT('Ctrl Pts',(54.4176809711311,-47.9061375253897,
12.));
#123132=CARTESIAN_POINT('Ctrl Pts',(54.429221896324,-47.9282560258516,12.));
#123133=CARTESIAN_POINT('Ctrl Pts',(54.4407602454967,-47.9504212334675,
12.));
#123134=CARTESIAN_POINT('Ctrl Pts',(54.4522959187955,-47.9726330780572,
12.));
#123135=CARTESIAN_POINT('Ctrl Pts',(54.4638288168003,-47.9948914896326,
12.));
#123136=CARTESIAN_POINT('Ctrl Pts',(54.4753588405215,-48.0171963983924,
12.));
#123137=CARTESIAN_POINT('Ctrl Pts',(54.4868858913971,-48.0395477347298,
12.));
#123138=CARTESIAN_POINT('Ctrl Pts',(54.4984098712886,-48.0619454292324,
12.));
#123139=CARTESIAN_POINT('Ctrl Pts',(54.5099306824786,-48.0843894126806,
12.));
#123140=CARTESIAN_POINT('Ctrl Pts',(54.5214482276678,-48.1068796160405,
12.));
#123141=CARTESIAN_POINT('Ctrl Pts',(54.5329624099721,-48.1294159704573,
12.));
#123142=CARTESIAN_POINT('Ctrl Pts',(54.5444731329201,-48.1519984072622,
12.));
#123143=CARTESIAN_POINT('Ctrl Pts',(54.5559803004492,-48.1746268579736,
12.));
#123144=CARTESIAN_POINT('Ctrl Pts',(54.5674838169041,-48.1973012542966,
12.));
#123145=CARTESIAN_POINT('Ctrl Pts',(54.5789835870342,-48.2200215281173,
12.));
#123146=CARTESIAN_POINT('Ctrl Pts',(54.5904795159926,-48.2427876114947,
12.));
#123147=CARTESIAN_POINT('Ctrl Pts',(54.6019715093309,-48.2655994366665,
12.));
#123148=CARTESIAN_POINT('Ctrl Pts',(54.6134594729959,-48.2884569360506,
12.));
#123149=CARTESIAN_POINT('Ctrl Pts',(54.6249433133261,-48.3113600422443,
12.));
#123150=CARTESIAN_POINT('Ctrl Pts',(54.6364229370494,-48.3343086880194,
12.));
#123151=CARTESIAN_POINT('Ctrl Pts',(54.6478982512794,-48.3573028063124,
12.));
#123152=CARTESIAN_POINT('Ctrl Pts',(54.6593691635145,-48.3803423302294,
12.));
#123153=CARTESIAN_POINT('Ctrl Pts',(54.6708355816358,-48.4034271930514,
12.));
#123154=CARTESIAN_POINT('Ctrl Pts',(54.6822974139063,-48.426557328234,12.));
#123155=CARTESIAN_POINT('Ctrl Pts',(54.6937545689695,-48.4497326694052,
12.));
#123156=CARTESIAN_POINT('Ctrl Pts',(54.7052069558497,-48.472953150357,12.));
#123157=CARTESIAN_POINT('Ctrl Pts',(54.716654483948,-48.4962187050457,12.));
#123158=CARTESIAN_POINT('Ctrl Pts',(54.7280970630351,-48.519529267596,12.));
#123159=CARTESIAN_POINT('Ctrl Pts',(54.7395346032453,-48.5428847722977,
12.));
#123160=CARTESIAN_POINT('Ctrl Pts',(54.7509670150714,-48.5662851536026,
12.));
#123161=CARTESIAN_POINT('Ctrl Pts',(54.7623942093586,-48.5897303461125,
12.));
#123162=CARTESIAN_POINT('Ctrl Pts',(54.7738160973031,-48.6132202845783,
12.));
#123163=CARTESIAN_POINT('Ctrl Pts',(54.7852325904583,-48.6367549039112,
12.));
#123164=CARTESIAN_POINT('Ctrl Pts',(54.7966436007389,-48.6603341391886,
12.));
#123165=CARTESIAN_POINT('Ctrl Pts',(54.8080490404275,-48.6839579256566,
12.));
#123166=CARTESIAN_POINT('Ctrl Pts',(54.819448822181,-48.7076261987292,12.));
#123167=CARTESIAN_POINT('Ctrl Pts',(54.8308428590344,-48.7313388939845,
12.));
#123168=CARTESIAN_POINT('Ctrl Pts',(54.8422310643763,-48.7550959471601,
12.));
#123169=CARTESIAN_POINT('Ctrl Pts',(54.8536133519292,-48.7788972941438,
12.));
#123170=CARTESIAN_POINT('Ctrl Pts',(54.8649896357285,-48.8027428709614,
12.));
#123171=CARTESIAN_POINT('Ctrl Pts',(54.8763598301037,-48.8266326137622,
12.));
#123172=CARTESIAN_POINT('Ctrl Pts',(54.8877238496565,-48.8505664587974,
12.));
#123173=CARTESIAN_POINT('Ctrl Pts',(54.8990816092953,-48.8745443424477,
12.));
#123174=CARTESIAN_POINT('Ctrl Pts',(54.9104330242742,-48.8985662012528,
12.));
#123175=CARTESIAN_POINT('Ctrl Pts',(54.9217780102355,-48.9226319719369,
12.));
#123176=CARTESIAN_POINT('Ctrl Pts',(54.9331164832423,-48.9467415914269,
12.));
#123177=CARTESIAN_POINT('Ctrl Pts',(54.9444483598378,-48.9708949968795,
12.));
#123178=CARTESIAN_POINT('Ctrl Pts',(54.9557735569943,-48.9950921256527,
12.));
#123179=CARTESIAN_POINT('Ctrl Pts',(54.9670919920029,-49.0193329152479,
12.));
#123180=CARTESIAN_POINT('Ctrl Pts',(54.9784035823765,-49.0436173032528,
12.));
#123181=CARTESIAN_POINT('Ctrl Pts',(54.9897082457606,-49.067945227287,12.));
#123182=CARTESIAN_POINT('Ctrl Pts',(55.0010058998107,-49.0923166249219,
12.));
#123183=CARTESIAN_POINT('Ctrl Pts',(55.012296462186,-49.116731433673,12.));
#123184=CARTESIAN_POINT('Ctrl Pts',(55.0235798508045,-49.1411895911635,
12.));
#123185=CARTESIAN_POINT('Ctrl Pts',(55.0348559840453,-49.1656910352476,
12.));
#123186=CARTESIAN_POINT('Ctrl Pts',(55.0461247809744,-49.1902357041461,
12.));
#123187=CARTESIAN_POINT('Ctrl Pts',(55.0573861615579,-49.2148235365704,
12.));
#123188=CARTESIAN_POINT('Ctrl Pts',(55.0686400468931,-49.2394544718531,
12.));
#123189=CARTESIAN_POINT('Ctrl Pts',(55.079886358701,-49.264128449652,12.));
#123190=CARTESIAN_POINT('Ctrl Pts',(55.0911250188302,-49.2888454096563,
12.));
#123191=CARTESIAN_POINT('Ctrl Pts',(55.102355948714,-49.3136052912622,12.));
#123192=CARTESIAN_POINT('Ctrl Pts',(55.1135790689464,-49.3384080333155,
12.));
#123193=CARTESIAN_POINT('Ctrl Pts',(55.1247942985619,-49.3632535736715,
12.));
#123194=CARTESIAN_POINT('Ctrl Pts',(55.136001555622,-49.3881418495489,12.));
#123195=CARTESIAN_POINT('Ctrl Pts',(55.1472007585183,-49.4130727983201,
12.));
#123196=CARTESIAN_POINT('Ctrl Pts',(55.1583918271116,-49.4380463581965,
12.));
#123197=CARTESIAN_POINT('Ctrl Pts',(55.1695746838174,-49.4630624688793,
12.));
#123198=CARTESIAN_POINT('Ctrl Pts',(55.1807492550119,-49.4881210723966,
12.));
#123199=CARTESIAN_POINT('Ctrl Pts',(55.1919154713647,-49.5132221132992,
12.));
#123200=CARTESIAN_POINT('Ctrl Pts',(55.2014798624094,-49.534774899476,12.));
#123201=CARTESIAN_POINT('Ctrl Pts',(55.2088081099093,-49.5513218524491,
12.));
#123202=CARTESIAN_POINT('Ctrl Pts',(55.2139039604723,-49.5628442142135,
12.));
#123203=CARTESIAN_POINT('Ctrl Pts',(55.216769915134,-49.5693295981931,12.));
#123204=CARTESIAN_POINT('Ctrl Pts',(55.2174072001497,-49.5707719660643,
12.));
#123205=CARTESIAN_POINT('',(53.0702932034641,-45.6458539113724,0.));
#123206=CARTESIAN_POINT('',(53.0702932034641,-45.6458539113724,0.));
#123207=CARTESIAN_POINT('Ctrl Pts',(55.2174072001497,-49.5707719660643,
0.));
#123208=CARTESIAN_POINT('Ctrl Pts',(55.216769915134,-49.5693295981931,0.));
#123209=CARTESIAN_POINT('Ctrl Pts',(55.2139039604723,-49.5628442142135,
0.));
#123210=CARTESIAN_POINT('Ctrl Pts',(55.2088081099093,-49.5513218524491,
0.));
#123211=CARTESIAN_POINT('Ctrl Pts',(55.2014798624094,-49.534774899476,0.));
#123212=CARTESIAN_POINT('Ctrl Pts',(55.1919154713647,-49.5132221132992,
0.));
#123213=CARTESIAN_POINT('Ctrl Pts',(55.1807492550119,-49.4881210723966,
0.));
#123214=CARTESIAN_POINT('Ctrl Pts',(55.1695746838174,-49.4630624688793,
0.));
#123215=CARTESIAN_POINT('Ctrl Pts',(55.1583918271116,-49.4380463581965,
0.));
#123216=CARTESIAN_POINT('Ctrl Pts',(55.1472007585183,-49.4130727983201,
0.));
#123217=CARTESIAN_POINT('Ctrl Pts',(55.136001555622,-49.3881418495489,0.));
#123218=CARTESIAN_POINT('Ctrl Pts',(55.1247942985619,-49.3632535736715,
0.));
#123219=CARTESIAN_POINT('Ctrl Pts',(55.1135790689464,-49.3384080333155,
0.));
#123220=CARTESIAN_POINT('Ctrl Pts',(55.102355948714,-49.3136052912622,0.));
#123221=CARTESIAN_POINT('Ctrl Pts',(55.0911250188302,-49.2888454096563,
0.));
#123222=CARTESIAN_POINT('Ctrl Pts',(55.079886358701,-49.264128449652,0.));
#123223=CARTESIAN_POINT('Ctrl Pts',(55.0686400468931,-49.2394544718531,
0.));
#123224=CARTESIAN_POINT('Ctrl Pts',(55.0573861615579,-49.2148235365704,
0.));
#123225=CARTESIAN_POINT('Ctrl Pts',(55.0461247809744,-49.1902357041461,
0.));
#123226=CARTESIAN_POINT('Ctrl Pts',(55.0348559840453,-49.1656910352476,
0.));
#123227=CARTESIAN_POINT('Ctrl Pts',(55.0235798508045,-49.1411895911635,
0.));
#123228=CARTESIAN_POINT('Ctrl Pts',(55.012296462186,-49.116731433673,0.));
#123229=CARTESIAN_POINT('Ctrl Pts',(55.0010058998107,-49.0923166249219,
0.));
#123230=CARTESIAN_POINT('Ctrl Pts',(54.9897082457606,-49.067945227287,0.));
#123231=CARTESIAN_POINT('Ctrl Pts',(54.9784035823765,-49.0436173032528,
0.));
#123232=CARTESIAN_POINT('Ctrl Pts',(54.9670919920029,-49.0193329152479,
0.));
#123233=CARTESIAN_POINT('Ctrl Pts',(54.9557735569943,-48.9950921256527,
0.));
#123234=CARTESIAN_POINT('Ctrl Pts',(54.9444483598378,-48.9708949968795,
0.));
#123235=CARTESIAN_POINT('Ctrl Pts',(54.9331164832423,-48.9467415914269,
0.));
#123236=CARTESIAN_POINT('Ctrl Pts',(54.9217780102355,-48.9226319719369,
0.));
#123237=CARTESIAN_POINT('Ctrl Pts',(54.9104330242742,-48.8985662012528,
0.));
#123238=CARTESIAN_POINT('Ctrl Pts',(54.8990816092953,-48.8745443424477,
0.));
#123239=CARTESIAN_POINT('Ctrl Pts',(54.8877238496565,-48.8505664587974,
0.));
#123240=CARTESIAN_POINT('Ctrl Pts',(54.8763598301037,-48.8266326137622,
0.));
#123241=CARTESIAN_POINT('Ctrl Pts',(54.8649896357285,-48.8027428709614,
0.));
#123242=CARTESIAN_POINT('Ctrl Pts',(54.8536133519292,-48.7788972941438,
0.));
#123243=CARTESIAN_POINT('Ctrl Pts',(54.8422310643763,-48.7550959471601,
0.));
#123244=CARTESIAN_POINT('Ctrl Pts',(54.8308428590344,-48.7313388939845,
0.));
#123245=CARTESIAN_POINT('Ctrl Pts',(54.819448822181,-48.7076261987292,0.));
#123246=CARTESIAN_POINT('Ctrl Pts',(54.8080490404275,-48.6839579256566,
0.));
#123247=CARTESIAN_POINT('Ctrl Pts',(54.7966436007389,-48.6603341391886,
0.));
#123248=CARTESIAN_POINT('Ctrl Pts',(54.7852325904583,-48.6367549039112,
0.));
#123249=CARTESIAN_POINT('Ctrl Pts',(54.7738160973031,-48.6132202845783,
0.));
#123250=CARTESIAN_POINT('Ctrl Pts',(54.7623942093586,-48.5897303461125,
0.));
#123251=CARTESIAN_POINT('Ctrl Pts',(54.7509670150714,-48.5662851536026,
0.));
#123252=CARTESIAN_POINT('Ctrl Pts',(54.7395346032453,-48.5428847722977,
0.));
#123253=CARTESIAN_POINT('Ctrl Pts',(54.7280970630351,-48.519529267596,0.));
#123254=CARTESIAN_POINT('Ctrl Pts',(54.716654483948,-48.4962187050457,0.));
#123255=CARTESIAN_POINT('Ctrl Pts',(54.7052069558497,-48.472953150357,0.));
#123256=CARTESIAN_POINT('Ctrl Pts',(54.6937545689695,-48.4497326694052,
0.));
#123257=CARTESIAN_POINT('Ctrl Pts',(54.6822974139063,-48.426557328234,0.));
#123258=CARTESIAN_POINT('Ctrl Pts',(54.6708355816358,-48.4034271930514,
0.));
#123259=CARTESIAN_POINT('Ctrl Pts',(54.6593691635145,-48.3803423302294,
0.));
#123260=CARTESIAN_POINT('Ctrl Pts',(54.6478982512794,-48.3573028063124,
0.));
#123261=CARTESIAN_POINT('Ctrl Pts',(54.6364229370494,-48.3343086880194,
0.));
#123262=CARTESIAN_POINT('Ctrl Pts',(54.6249433133261,-48.3113600422443,
0.));
#123263=CARTESIAN_POINT('Ctrl Pts',(54.6134594729959,-48.2884569360506,
0.));
#123264=CARTESIAN_POINT('Ctrl Pts',(54.6019715093309,-48.2655994366665,
0.));
#123265=CARTESIAN_POINT('Ctrl Pts',(54.5904795159926,-48.2427876114947,
0.));
#123266=CARTESIAN_POINT('Ctrl Pts',(54.5789835870342,-48.2200215281173,
0.));
#123267=CARTESIAN_POINT('Ctrl Pts',(54.5674838169041,-48.1973012542966,
0.));
#123268=CARTESIAN_POINT('Ctrl Pts',(54.5559803004492,-48.1746268579736,
0.));
#123269=CARTESIAN_POINT('Ctrl Pts',(54.5444731329201,-48.1519984072622,
0.));
#123270=CARTESIAN_POINT('Ctrl Pts',(54.5329624099721,-48.1294159704573,
0.));
#123271=CARTESIAN_POINT('Ctrl Pts',(54.5214482276678,-48.1068796160405,
0.));
#123272=CARTESIAN_POINT('Ctrl Pts',(54.5099306824786,-48.0843894126806,
0.));
#123273=CARTESIAN_POINT('Ctrl Pts',(54.4984098712886,-48.0619454292324,
0.));
#123274=CARTESIAN_POINT('Ctrl Pts',(54.4868858913971,-48.0395477347298,
0.));
#123275=CARTESIAN_POINT('Ctrl Pts',(54.4753588405215,-48.0171963983924,
0.));
#123276=CARTESIAN_POINT('Ctrl Pts',(54.4638288168003,-47.9948914896326,
0.));
#123277=CARTESIAN_POINT('Ctrl Pts',(54.4522959187955,-47.9726330780572,
0.));
#123278=CARTESIAN_POINT('Ctrl Pts',(54.4407602454967,-47.9504212334675,
0.));
#123279=CARTESIAN_POINT('Ctrl Pts',(54.429221896324,-47.9282560258516,0.));
#123280=CARTESIAN_POINT('Ctrl Pts',(54.4176809711311,-47.9061375253897,
0.));
#123281=CARTESIAN_POINT('Ctrl Pts',(54.4061375702079,-47.8840658024618,
0.));
#123282=CARTESIAN_POINT('Ctrl Pts',(54.3945917942832,-47.8620409276493,
0.));
#123283=CARTESIAN_POINT('Ctrl Pts',(54.3830437445278,-47.8400629717355,
0.));
#123284=CARTESIAN_POINT('Ctrl Pts',(54.3714935225591,-47.8181320056995,
0.));
#123285=CARTESIAN_POINT('Ctrl Pts',(54.3599412304437,-47.7962481007185,
0.));
#123286=CARTESIAN_POINT('Ctrl Pts',(54.3483869707002,-47.7744113281771,
0.));
#123287=CARTESIAN_POINT('Ctrl Pts',(54.3368308463023,-47.7526217596694,
0.));
#123288=CARTESIAN_POINT('Ctrl Pts',(54.3252729606823,-47.7308794669993,
0.));
#123289=CARTESIAN_POINT('Ctrl Pts',(54.3137134177345,-47.7091845221747,
0.));
#123290=CARTESIAN_POINT('Ctrl Pts',(54.302152321819,-47.6875369974087,0.));
#123291=CARTESIAN_POINT('Ctrl Pts',(54.290589777765,-47.6659369651301,0.));
#123292=CARTESIAN_POINT('Ctrl Pts',(54.2790258908738,-47.6443844979848,
0.));
#123293=CARTESIAN_POINT('Ctrl Pts',(54.2674607669226,-47.6228796688375,
0.));
#123294=CARTESIAN_POINT('Ctrl Pts',(54.2558945121678,-47.6014225507659,
0.));
#123295=CARTESIAN_POINT('Ctrl Pts',(54.244327233349,-47.5800132170608,0.));
#123296=CARTESIAN_POINT('Ctrl Pts',(54.2327590376924,-47.5586517412363,
0.));
#123297=CARTESIAN_POINT('Ctrl Pts',(54.2211900329138,-47.5373381970326,
0.));
#123298=CARTESIAN_POINT('Ctrl Pts',(54.209620327223,-47.5160726584174,0.));
#123299=CARTESIAN_POINT('Ctrl Pts',(54.198050029327,-47.4948551995801,0.));
#123300=CARTESIAN_POINT('Ctrl Pts',(54.1864792484345,-47.4736858949322,
0.));
#123301=CARTESIAN_POINT('Ctrl Pts',(54.1749080942593,-47.4525648191173,
0.));
#123302=CARTESIAN_POINT('Ctrl Pts',(54.1633366770239,-47.4314920470141,
0.));
#123303=CARTESIAN_POINT('Ctrl Pts',(54.1517651074637,-47.4104676537381,
0.));
#123304=CARTESIAN_POINT('Ctrl Pts',(54.1401934968311,-47.3894917146365,
0.));
#123305=CARTESIAN_POINT('Ctrl Pts',(54.1286219568989,-47.3685643052874,
0.));
#123306=CARTESIAN_POINT('Ctrl Pts',(54.1170505999645,-47.3476855015102,
0.));
#123307=CARTESIAN_POINT('Ctrl Pts',(54.1054795388543,-47.3268553793694,
0.));
#123308=CARTESIAN_POINT('Ctrl Pts',(54.0939088869268,-47.3060740151752,
0.));
#123309=CARTESIAN_POINT('Ctrl Pts',(54.0823387580776,-47.2853414854793,
0.));
#123310=CARTESIAN_POINT('Ctrl Pts',(54.0707692667438,-47.2646578670746,
0.));
#123311=CARTESIAN_POINT('Ctrl Pts',(54.0592005279086,-47.2440232370065,
0.));
#123312=CARTESIAN_POINT('Ctrl Pts',(54.047632657104,-47.2234376725743,0.));
#123313=CARTESIAN_POINT('Ctrl Pts',(54.0360657704163,-47.202901251334,0.));
#123314=CARTESIAN_POINT('Ctrl Pts',(54.0244999844893,-47.1824140510926,
0.));
#123315=CARTESIAN_POINT('Ctrl Pts',(54.0129354165297,-47.1619761499087,
0.));
#123316=CARTESIAN_POINT('Ctrl Pts',(54.0013721843118,-47.1415876261035,
0.));
#123317=CARTESIAN_POINT('Ctrl Pts',(53.989810406182,-47.1212485582643,0.));
#123318=CARTESIAN_POINT('Ctrl Pts',(53.9782502010634,-47.1009590252458,
0.));
#123319=CARTESIAN_POINT('Ctrl Pts',(53.9666916884596,-47.0807191061648,
0.));
#123320=CARTESIAN_POINT('Ctrl Pts',(53.9551349884599,-47.0605288804008,
0.));
#123321=CARTESIAN_POINT('Ctrl Pts',(53.9435802217436,-47.0403884276072,
0.));
#123322=CARTESIAN_POINT('Ctrl Pts',(53.9320275095853,-47.0202978277138,
0.));
#123323=CARTESIAN_POINT('Ctrl Pts',(53.9204769738596,-47.0002571609297,
0.));
#123324=CARTESIAN_POINT('Ctrl Pts',(53.9089287370463,-46.9802665077366,
0.));
#123325=CARTESIAN_POINT('Ctrl Pts',(53.8973829222347,-46.9603259488921,
0.));
#123326=CARTESIAN_POINT('Ctrl Pts',(53.8858396531298,-46.9404355654401,
0.));
#123327=CARTESIAN_POINT('Ctrl Pts',(53.8742990540563,-46.9205954387133,
0.));
#123328=CARTESIAN_POINT('Ctrl Pts',(53.8627612499638,-46.9008056503351,
0.));
#123329=CARTESIAN_POINT('Ctrl Pts',(53.8512263664321,-46.881066282213,0.));
#123330=CARTESIAN_POINT('Ctrl Pts',(53.8396945296757,-46.8613774165435,
0.));
#123331=CARTESIAN_POINT('Ctrl Pts',(53.8281658665503,-46.841739135822,0.));
#123332=CARTESIAN_POINT('Ctrl Pts',(53.816640504558,-46.8221515228457,0.));
#123333=CARTESIAN_POINT('Ctrl Pts',(53.8051185718532,-46.802614660715,0.));
#123334=CARTESIAN_POINT('Ctrl Pts',(53.793600197248,-46.7831286328278,0.));
#123335=CARTESIAN_POINT('Ctrl Pts',(53.7820855102182,-46.7636935228861,
0.));
#123336=CARTESIAN_POINT('Ctrl Pts',(53.7705746409075,-46.7443094149045,
0.));
#123337=CARTESIAN_POINT('Ctrl Pts',(53.7590677201342,-46.7249763932129,
0.));
#123338=CARTESIAN_POINT('Ctrl Pts',(53.7475648793946,-46.7056945424559,
0.));
#123339=CARTESIAN_POINT('Ctrl Pts',(53.7360662508675,-46.6864639475862,
0.));
#123340=CARTESIAN_POINT('Ctrl Pts',(53.7245719674221,-46.6672846938752,
0.));
#123341=CARTESIAN_POINT('Ctrl Pts',(53.7130821626262,-46.6481568669217,
0.));
#123342=CARTESIAN_POINT('Ctrl Pts',(53.7015969707541,-46.6290805526559,
0.));
#123343=CARTESIAN_POINT('Ctrl Pts',(53.690116526794,-46.6100558373401,0.));
#123344=CARTESIAN_POINT('Ctrl Pts',(53.678640966456,-46.5910828075652,0.));
#123345=CARTESIAN_POINT('Ctrl Pts',(53.6671704261735,-46.572161550259,0.));
#123346=CARTESIAN_POINT('Ctrl Pts',(53.6557050431069,-46.5532921526899,
0.));
#123347=CARTESIAN_POINT('Ctrl Pts',(53.6442449551455,-46.5344747024677,
0.));
#123348=CARTESIAN_POINT('Ctrl Pts',(53.6327903009097,-46.5157092875377,
0.));
#123349=CARTESIAN_POINT('Ctrl Pts',(53.6213412197542,-46.4969959961779,
0.));
#123350=CARTESIAN_POINT('Ctrl Pts',(53.6098978517869,-46.4783349170182,
0.));
#123351=CARTESIAN_POINT('Ctrl Pts',(53.5984603378861,-46.4597261390526,
0.));
#123352=CARTESIAN_POINT('Ctrl Pts',(53.5870288197161,-46.4411697516474,
0.));
#123353=CARTESIAN_POINT('Ctrl Pts',(53.5756034397464,-46.422665844546,0.));
#123354=CARTESIAN_POINT('Ctrl Pts',(53.5641843412537,-46.4042145078682,
0.));
#123355=CARTESIAN_POINT('Ctrl Pts',(53.5527716683029,-46.3858158321044,
0.));
#123356=CARTESIAN_POINT('Ctrl Pts',(53.5413655657323,-46.3674699081043,
0.));
#123357=CARTESIAN_POINT('Ctrl Pts',(53.5299661791396,-46.3491768270664,
0.));
#123358=CARTESIAN_POINT('Ctrl Pts',(53.518573654857,-46.3309366805112,0.));
#123359=CARTESIAN_POINT('Ctrl Pts',(53.5071881399932,-46.3127495603117,
0.));
#123360=CARTESIAN_POINT('Ctrl Pts',(53.4958097825019,-46.2946155587428,
0.));
#123361=CARTESIAN_POINT('Ctrl Pts',(53.4844387312414,-46.2765347685198,
0.));
#123362=CARTESIAN_POINT('Ctrl Pts',(53.4730751360359,-46.2585072828343,
0.));
#123363=CARTESIAN_POINT('Ctrl Pts',(53.4617191477382,-46.2405331953872,
0.));
#123364=CARTESIAN_POINT('Ctrl Pts',(53.4503709181158,-46.2226126003185,
0.));
#123365=CARTESIAN_POINT('Ctrl Pts',(53.4390305997263,-46.2047455921276,
0.));
#123366=CARTESIAN_POINT('Ctrl Pts',(53.4276983458129,-46.1869322656027,
0.));
#123367=CARTESIAN_POINT('Ctrl Pts',(53.4163743101534,-46.1691727157149,
0.));
#123368=CARTESIAN_POINT('Ctrl Pts',(53.4050586470463,-46.1514670376035,
0.));
#123369=CARTESIAN_POINT('Ctrl Pts',(53.3937515116572,-46.1338153268116,
0.));
#123370=CARTESIAN_POINT('Ctrl Pts',(53.3824530603284,-46.1162176794891,
0.));
#123371=CARTESIAN_POINT('Ctrl Pts',(53.3711634508426,-46.0986741925646,
0.));
#123372=CARTESIAN_POINT('Ctrl Pts',(53.3598828428519,-46.0811849640195,
0.));
#123373=CARTESIAN_POINT('Ctrl Pts',(53.3486113975868,-46.0637500926954,
0.));
#123374=CARTESIAN_POINT('Ctrl Pts',(53.3373492770647,-46.046369677778,0.));
#123375=CARTESIAN_POINT('Ctrl Pts',(53.3260966434277,-46.0290438183598,
0.));
#123376=CARTESIAN_POINT('Ctrl Pts',(53.3148536582658,-46.0117726129893,
0.));
#123377=CARTESIAN_POINT('Ctrl Pts',(53.3036204818367,-45.9945561591486,
0.));
#123378=CARTESIAN_POINT('Ctrl Pts',(53.2923972745585,-45.9773945542415,
0.));
#123379=CARTESIAN_POINT('Ctrl Pts',(53.2811841987945,-45.9602878967715,
0.));
#123380=CARTESIAN_POINT('Ctrl Pts',(53.2699814203097,-45.9432362873001,
0.));
#123381=CARTESIAN_POINT('Ctrl Pts',(53.2587891103835,-45.9262398298323,
0.));
#123382=CARTESIAN_POINT('Ctrl Pts',(53.2476074459977,-45.9092986319343,
0.));
#123383=CARTESIAN_POINT('Ctrl Pts',(53.2364366054276,-45.8924128018354,
0.));
#123384=CARTESIAN_POINT('Ctrl Pts',(53.2252767643652,-45.8755824458715,
0.));
#123385=CARTESIAN_POINT('Ctrl Pts',(53.2141280925458,-45.8588076662598,
0.));
#123386=CARTESIAN_POINT('Ctrl Pts',(53.2029907483602,-45.8420885575386,
0.));
#123387=CARTESIAN_POINT('Ctrl Pts',(53.1918648840598,-45.8254252100003,
0.));
#123388=CARTESIAN_POINT('Ctrl Pts',(53.1807506560977,-45.8088177165124,
0.));
#123389=CARTESIAN_POINT('Ctrl Pts',(53.1696482334487,-45.7922661780005,
0.));
#123390=CARTESIAN_POINT('Ctrl Pts',(53.158557807638,-45.7757707100568,0.));
#123391=CARTESIAN_POINT('Ctrl Pts',(53.147479599594,-45.7593314474413,0.));
#123392=CARTESIAN_POINT('Ctrl Pts',(53.136413838457,-45.7429485300727,0.));
#123393=CARTESIAN_POINT('Ctrl Pts',(53.1253607414806,-45.7266220896951,
0.));
#123394=CARTESIAN_POINT('Ctrl Pts',(53.1143204954981,-45.7103522376744,
0.));
#123395=CARTESIAN_POINT('Ctrl Pts',(53.1032932329074,-45.6941390489239,
0.));
#123396=CARTESIAN_POINT('Ctrl Pts',(53.0922790298736,-45.6779825614486,
0.));
#123397=CARTESIAN_POINT('Ctrl Pts',(53.083478145185,-45.665102743948,0.));
#123398=CARTESIAN_POINT('Ctrl Pts',(53.0768833804386,-45.6554684028296,
0.));
#123399=CARTESIAN_POINT('Ctrl Pts',(53.0724894921921,-45.6490568514146,
0.));
#123400=CARTESIAN_POINT('Ctrl Pts',(53.0702932034641,-45.6458539113724,
0.));
#123401=CARTESIAN_POINT('Ctrl Pts',(50.7903314215393,-54.5031396718592,
0.));
#123402=CARTESIAN_POINT('Ctrl Pts',(50.7903314215393,-54.5031396718592,
12.));
#123403=CARTESIAN_POINT('Ctrl Pts',(50.7885805844281,-54.4978248630387,
0.));
#123404=CARTESIAN_POINT('Ctrl Pts',(50.7885805844281,-54.4978248630387,
12.));
#123405=CARTESIAN_POINT('Ctrl Pts',(50.7850776288813,-54.4871993224832,
0.));
#123406=CARTESIAN_POINT('Ctrl Pts',(50.7850776288813,-54.4871993224832,
12.));
#123407=CARTESIAN_POINT('Ctrl Pts',(50.7798193515888,-54.4712732429066,
0.));
#123408=CARTESIAN_POINT('Ctrl Pts',(50.7798193515888,-54.4712732429066,
12.));
#123409=CARTESIAN_POINT('Ctrl Pts',(50.7728006269349,-54.4500629336429,
0.));
#123410=CARTESIAN_POINT('Ctrl Pts',(50.7728006269349,-54.4500629336429,
12.));
#123411=CARTESIAN_POINT('Ctrl Pts',(50.764014409002,-54.423590828767,0.));
#123412=CARTESIAN_POINT('Ctrl Pts',(50.764014409002,-54.423590828767,12.));
#123413=CARTESIAN_POINT('Ctrl Pts',(50.7552153869475,-54.3971595231574,
0.));
#123414=CARTESIAN_POINT('Ctrl Pts',(50.7552153869475,-54.3971595231574,
12.));
#123415=CARTESIAN_POINT('Ctrl Pts',(50.7464035792906,-54.3707690445749,
0.));
#123416=CARTESIAN_POINT('Ctrl Pts',(50.7464035792906,-54.3707690445749,
12.));
#123417=CARTESIAN_POINT('Ctrl Pts',(50.7375790185896,-54.3444194324054,
0.));
#123418=CARTESIAN_POINT('Ctrl Pts',(50.7375790185896,-54.3444194324054,
12.));
#123419=CARTESIAN_POINT('Ctrl Pts',(50.7287417566123,-54.3181107400663,
0.));
#123420=CARTESIAN_POINT('Ctrl Pts',(50.7287417566123,-54.3181107400663,
12.));
#123421=CARTESIAN_POINT('Ctrl Pts',(50.7198918629451,-54.2918430335206,
0.));
#123422=CARTESIAN_POINT('Ctrl Pts',(50.7198918629451,-54.2918430335206,
12.));
#123423=CARTESIAN_POINT('Ctrl Pts',(50.7110294185698,-54.2656163868104,
0.));
#123424=CARTESIAN_POINT('Ctrl Pts',(50.7110294185698,-54.2656163868104,
12.));
#123425=CARTESIAN_POINT('Ctrl Pts',(50.7021545108311,-54.2394308784026,
0.));
#123426=CARTESIAN_POINT('Ctrl Pts',(50.7021545108311,-54.2394308784026,
12.));
#123427=CARTESIAN_POINT('Ctrl Pts',(50.6932672279772,-54.2132865872985,
0.));
#123428=CARTESIAN_POINT('Ctrl Pts',(50.6932672279772,-54.2132865872985,
12.));
#123429=CARTESIAN_POINT('Ctrl Pts',(50.6843676535492,-54.1871835889981,
0.));
#123430=CARTESIAN_POINT('Ctrl Pts',(50.6843676535492,-54.1871835889981,
12.));
#123431=CARTESIAN_POINT('Ctrl Pts',(50.67545586183,-54.1611219522394,0.));
#123432=CARTESIAN_POINT('Ctrl Pts',(50.67545586183,-54.1611219522394,12.));
#123433=CARTESIAN_POINT('Ctrl Pts',(50.6665319209869,-54.1351017412804,
0.));
#123434=CARTESIAN_POINT('Ctrl Pts',(50.6665319209869,-54.1351017412804,
12.));
#123435=CARTESIAN_POINT('Ctrl Pts',(50.6575958953221,-54.1091230175367,
0.));
#123436=CARTESIAN_POINT('Ctrl Pts',(50.6575958953221,-54.1091230175367,
12.));
#123437=CARTESIAN_POINT('Ctrl Pts',(50.6486478479465,-54.0831858415189,
0.));
#123438=CARTESIAN_POINT('Ctrl Pts',(50.6486478479465,-54.0831858415189,
12.));
#123439=CARTESIAN_POINT('Ctrl Pts',(50.6396878430939,-54.0572902745076,
0.));
#123440=CARTESIAN_POINT('Ctrl Pts',(50.6396878430939,-54.0572902745076,
12.));
#123441=CARTESIAN_POINT('Ctrl Pts',(50.6307159490553,-54.0314363806708,
0.));
#123442=CARTESIAN_POINT('Ctrl Pts',(50.6307159490553,-54.0314363806708,
12.));
#123443=CARTESIAN_POINT('Ctrl Pts',(50.6217322378648,-54.0056242268399,
0.));
#123444=CARTESIAN_POINT('Ctrl Pts',(50.6217322378648,-54.0056242268399,
12.));
#123445=CARTESIAN_POINT('Ctrl Pts',(50.6127367839711,-53.979853881553,0.));
#123446=CARTESIAN_POINT('Ctrl Pts',(50.6127367839711,-53.979853881553,12.));
#123447=CARTESIAN_POINT('Ctrl Pts',(50.6037296632139,-53.9541254143119,
0.));
#123448=CARTESIAN_POINT('Ctrl Pts',(50.6037296632139,-53.9541254143119,
12.));
#123449=CARTESIAN_POINT('Ctrl Pts',(50.5947109517483,-53.9284388948004,
0.));
#123450=CARTESIAN_POINT('Ctrl Pts',(50.5947109517483,-53.9284388948004,
12.));
#123451=CARTESIAN_POINT('Ctrl Pts',(50.5856807248151,-53.9027943919836,
0.));
#123452=CARTESIAN_POINT('Ctrl Pts',(50.5856807248151,-53.9027943919836,
12.));
#123453=CARTESIAN_POINT('Ctrl Pts',(50.5766390561884,-53.8771919737032,
0.));
#123454=CARTESIAN_POINT('Ctrl Pts',(50.5766390561884,-53.8771919737032,
12.));
#123455=CARTESIAN_POINT('Ctrl Pts',(50.5675860188538,-53.8516317071804,
0.));
#123456=CARTESIAN_POINT('Ctrl Pts',(50.5675860188538,-53.8516317071804,
12.));
#123457=CARTESIAN_POINT('Ctrl Pts',(50.5585216854091,-53.8261136593075,
0.));
#123458=CARTESIAN_POINT('Ctrl Pts',(50.5585216854091,-53.8261136593075,
12.));
#123459=CARTESIAN_POINT('Ctrl Pts',(50.5494461285761,-53.8006378970197,
0.));
#123460=CARTESIAN_POINT('Ctrl Pts',(50.5494461285761,-53.8006378970197,
12.));
#123461=CARTESIAN_POINT('Ctrl Pts',(50.5403594216698,-53.7752044876304,
0.));
#123462=CARTESIAN_POINT('Ctrl Pts',(50.5403594216698,-53.7752044876304,
12.));
#123463=CARTESIAN_POINT('Ctrl Pts',(50.5312616390779,-53.7498134991703,
0.));
#123464=CARTESIAN_POINT('Ctrl Pts',(50.5312616390779,-53.7498134991703,
12.));
#123465=CARTESIAN_POINT('Ctrl Pts',(50.522152856042,-53.7244650002374,0.));
#123466=CARTESIAN_POINT('Ctrl Pts',(50.522152856042,-53.7244650002374,12.));
#123467=CARTESIAN_POINT('Ctrl Pts',(50.513033148456,-53.6991590598548,0.));
#123468=CARTESIAN_POINT('Ctrl Pts',(50.513033148456,-53.6991590598548,12.));
#123469=CARTESIAN_POINT('Ctrl Pts',(50.503902592653,-53.6738957473158,0.));
#123470=CARTESIAN_POINT('Ctrl Pts',(50.503902592653,-53.6738957473158,12.));
#123471=CARTESIAN_POINT('Ctrl Pts',(50.4947612652148,-53.6486751320436,
0.));
#123472=CARTESIAN_POINT('Ctrl Pts',(50.4947612652148,-53.6486751320436,
12.));
#123473=CARTESIAN_POINT('Ctrl Pts',(50.4856092427314,-53.623497283406,0.));
#123474=CARTESIAN_POINT('Ctrl Pts',(50.4856092427314,-53.623497283406,12.));
#123475=CARTESIAN_POINT('Ctrl Pts',(50.4764466018071,-53.5983622707238,
0.));
#123476=CARTESIAN_POINT('Ctrl Pts',(50.4764466018071,-53.5983622707238,
12.));
#123477=CARTESIAN_POINT('Ctrl Pts',(50.4672734191756,-53.5732701633609,
0.));
#123478=CARTESIAN_POINT('Ctrl Pts',(50.4672734191756,-53.5732701633609,
12.));
#123479=CARTESIAN_POINT('Ctrl Pts',(50.4580897717838,-53.5482210307868,
0.));
#123480=CARTESIAN_POINT('Ctrl Pts',(50.4580897717838,-53.5482210307868,
12.));
#123481=CARTESIAN_POINT('Ctrl Pts',(50.4488957368839,-53.5232149426413,
0.));
#123482=CARTESIAN_POINT('Ctrl Pts',(50.4488957368839,-53.5232149426413,
12.));
#123483=CARTESIAN_POINT('Ctrl Pts',(50.4396913921381,-53.4982519688024,
0.));
#123484=CARTESIAN_POINT('Ctrl Pts',(50.4396913921381,-53.4982519688024,
12.));
#123485=CARTESIAN_POINT('Ctrl Pts',(50.4304768156666,-53.4733321794188,
0.));
#123486=CARTESIAN_POINT('Ctrl Pts',(50.4304768156666,-53.4733321794188,
12.));
#123487=CARTESIAN_POINT('Ctrl Pts',(50.4212520859914,-53.4484556448776,
0.));
#123488=CARTESIAN_POINT('Ctrl Pts',(50.4212520859914,-53.4484556448776,
12.));
#123489=CARTESIAN_POINT('Ctrl Pts',(50.4120172820047,-53.4236224357838,
0.));
#123490=CARTESIAN_POINT('Ctrl Pts',(50.4120172820047,-53.4236224357838,
12.));
#123491=CARTESIAN_POINT('Ctrl Pts',(50.4027724829297,-53.398832622931,0.));
#123492=CARTESIAN_POINT('Ctrl Pts',(50.4027724829297,-53.398832622931,12.));
#123493=CARTESIAN_POINT('Ctrl Pts',(50.3935177682837,-53.3740862772681,
0.));
#123494=CARTESIAN_POINT('Ctrl Pts',(50.3935177682837,-53.3740862772681,
12.));
#123495=CARTESIAN_POINT('Ctrl Pts',(50.384253217846,-53.3493834698697,0.));
#123496=CARTESIAN_POINT('Ctrl Pts',(50.384253217846,-53.3493834698697,12.));
#123497=CARTESIAN_POINT('Ctrl Pts',(50.3749789116786,-53.3247242719587,
0.));
#123498=CARTESIAN_POINT('Ctrl Pts',(50.3749789116786,-53.3247242719587,
12.));
#123499=CARTESIAN_POINT('Ctrl Pts',(50.365694930143,-53.300108754923,0.));
#123500=CARTESIAN_POINT('Ctrl Pts',(50.365694930143,-53.300108754923,12.));
#123501=CARTESIAN_POINT('Ctrl Pts',(50.3564013539199,-53.2755369903293,
0.));
#123502=CARTESIAN_POINT('Ctrl Pts',(50.3564013539199,-53.2755369903293,
12.));
#123503=CARTESIAN_POINT('Ctrl Pts',(50.3470982640289,-53.2510090499336,
0.));
#123504=CARTESIAN_POINT('Ctrl Pts',(50.3470982640289,-53.2510090499336,
12.));
#123505=CARTESIAN_POINT('Ctrl Pts',(50.3377857418514,-53.2265250056887,
0.));
#123506=CARTESIAN_POINT('Ctrl Pts',(50.3377857418514,-53.2265250056887,
12.));
#123507=CARTESIAN_POINT('Ctrl Pts',(50.3284638691278,-53.2020849297471,
0.));
#123508=CARTESIAN_POINT('Ctrl Pts',(50.3284638691278,-53.2020849297471,
12.));
#123509=CARTESIAN_POINT('Ctrl Pts',(50.3191327279492,-53.1776888944616,
0.));
#123510=CARTESIAN_POINT('Ctrl Pts',(50.3191327279492,-53.1776888944616,
12.));
#123511=CARTESIAN_POINT('Ctrl Pts',(50.3097924007534,-53.1533369723818,
0.));
#123512=CARTESIAN_POINT('Ctrl Pts',(50.3097924007534,-53.1533369723818,
12.));
#123513=CARTESIAN_POINT('Ctrl Pts',(50.300442970319,-53.1290292362485,0.));
#123514=CARTESIAN_POINT('Ctrl Pts',(50.300442970319,-53.1290292362485,12.));
#123515=CARTESIAN_POINT('Ctrl Pts',(50.2910845197619,-53.1047657589812,
0.));
#123516=CARTESIAN_POINT('Ctrl Pts',(50.2910845197619,-53.1047657589812,
12.));
#123517=CARTESIAN_POINT('Ctrl Pts',(50.2817171325358,-53.0805466136798,
0.));
#123518=CARTESIAN_POINT('Ctrl Pts',(50.2817171325358,-53.0805466136798,
12.));
#123519=CARTESIAN_POINT('Ctrl Pts',(50.2723408924373,-53.0563718736366,
0.));
#123520=CARTESIAN_POINT('Ctrl Pts',(50.2723408924373,-53.0563718736366,
12.));
#123521=CARTESIAN_POINT('Ctrl Pts',(50.2629558836111,-53.0322416123406,
0.));
#123522=CARTESIAN_POINT('Ctrl Pts',(50.2629558836111,-53.0322416123406,
12.));
#123523=CARTESIAN_POINT('Ctrl Pts',(50.2535621905552,-53.0081559034801,
0.));
#123524=CARTESIAN_POINT('Ctrl Pts',(50.2535621905552,-53.0081559034801,
12.));
#123525=CARTESIAN_POINT('Ctrl Pts',(50.2441598981286,-52.9841148209402,
0.));
#123526=CARTESIAN_POINT('Ctrl Pts',(50.2441598981286,-52.9841148209402,
12.));
#123527=CARTESIAN_POINT('Ctrl Pts',(50.2347490915555,-52.9601184388028,
0.));
#123528=CARTESIAN_POINT('Ctrl Pts',(50.2347490915555,-52.9601184388028,
12.));
#123529=CARTESIAN_POINT('Ctrl Pts',(50.2253298564241,-52.9361668313542,
0.));
#123530=CARTESIAN_POINT('Ctrl Pts',(50.2253298564241,-52.9361668313542,
12.));
#123531=CARTESIAN_POINT('Ctrl Pts',(50.2159022786879,-52.9122600730884,
0.));
#123532=CARTESIAN_POINT('Ctrl Pts',(50.2159022786879,-52.9122600730884,
12.));
#123533=CARTESIAN_POINT('Ctrl Pts',(50.2064664446663,-52.8883982387068,
0.));
#123534=CARTESIAN_POINT('Ctrl Pts',(50.2064664446663,-52.8883982387068,
12.));
#123535=CARTESIAN_POINT('Ctrl Pts',(50.1970224410471,-52.8645814031133,
0.));
#123536=CARTESIAN_POINT('Ctrl Pts',(50.1970224410471,-52.8645814031133,
12.));
#123537=CARTESIAN_POINT('Ctrl Pts',(50.1875703548884,-52.8408096414093,
0.));
#123538=CARTESIAN_POINT('Ctrl Pts',(50.1875703548884,-52.8408096414093,
12.));
#123539=CARTESIAN_POINT('Ctrl Pts',(50.1781102736205,-52.8170830289044,
0.));
#123540=CARTESIAN_POINT('Ctrl Pts',(50.1781102736205,-52.8170830289044,
12.));
#123541=CARTESIAN_POINT('Ctrl Pts',(50.1686422850487,-52.7934016411205,
0.));
#123542=CARTESIAN_POINT('Ctrl Pts',(50.1686422850487,-52.7934016411205,
12.));
#123543=CARTESIAN_POINT('Ctrl Pts',(50.1591664773561,-52.769765553794,0.));
#123544=CARTESIAN_POINT('Ctrl Pts',(50.1591664773561,-52.769765553794,12.));
#123545=CARTESIAN_POINT('Ctrl Pts',(50.1496829391073,-52.7461748428738,
0.));
#123546=CARTESIAN_POINT('Ctrl Pts',(50.1496829391073,-52.7461748428738,
12.));
#123547=CARTESIAN_POINT('Ctrl Pts',(50.1401917592537,-52.7226295845161,
0.));
#123548=CARTESIAN_POINT('Ctrl Pts',(50.1401917592537,-52.7226295845161,
12.));
#123549=CARTESIAN_POINT('Ctrl Pts',(50.1306930271345,-52.699129855093,0.));
#123550=CARTESIAN_POINT('Ctrl Pts',(50.1306930271345,-52.699129855093,12.));
#123551=CARTESIAN_POINT('Ctrl Pts',(50.121186832478,-52.6756757311978,0.));
#123552=CARTESIAN_POINT('Ctrl Pts',(50.121186832478,-52.6756757311978,12.));
#123553=CARTESIAN_POINT('Ctrl Pts',(50.111673265404,-52.652267289646,0.));
#123554=CARTESIAN_POINT('Ctrl Pts',(50.111673265404,-52.652267289646,12.));
#123555=CARTESIAN_POINT('Ctrl Pts',(50.1021524164264,-52.6289046074746,
0.));
#123556=CARTESIAN_POINT('Ctrl Pts',(50.1021524164264,-52.6289046074746,
12.));
#123557=CARTESIAN_POINT('Ctrl Pts',(50.0926243764578,-52.6055877619348,
0.));
#123558=CARTESIAN_POINT('Ctrl Pts',(50.0926243764578,-52.6055877619348,
12.));
#123559=CARTESIAN_POINT('Ctrl Pts',(50.0830892368107,-52.5823168304994,
0.));
#123560=CARTESIAN_POINT('Ctrl Pts',(50.0830892368107,-52.5823168304994,
12.));
#123561=CARTESIAN_POINT('Ctrl Pts',(50.0735470892007,-52.5590918908702,
0.));
#123562=CARTESIAN_POINT('Ctrl Pts',(50.0735470892007,-52.5590918908702,
12.));
#123563=CARTESIAN_POINT('Ctrl Pts',(50.0639980257479,-52.5359130209792,
0.));
#123564=CARTESIAN_POINT('Ctrl Pts',(50.0639980257479,-52.5359130209792,
12.));
#123565=CARTESIAN_POINT('Ctrl Pts',(50.0544421389817,-52.5127802989896,
0.));
#123566=CARTESIAN_POINT('Ctrl Pts',(50.0544421389817,-52.5127802989896,
12.));
#123567=CARTESIAN_POINT('Ctrl Pts',(50.0448795218441,-52.4896938032884,
0.));
#123568=CARTESIAN_POINT('Ctrl Pts',(50.0448795218441,-52.4896938032884,
12.));
#123569=CARTESIAN_POINT('Ctrl Pts',(50.0353102676921,-52.4666536124913,
0.));
#123570=CARTESIAN_POINT('Ctrl Pts',(50.0353102676921,-52.4666536124913,
12.));
#123571=CARTESIAN_POINT('Ctrl Pts',(50.0257344703,-52.4436598054515,0.));
#123572=CARTESIAN_POINT('Ctrl Pts',(50.0257344703,-52.4436598054515,12.));
#123573=CARTESIAN_POINT('Ctrl Pts',(50.0161522238616,-52.4207124612608,
0.));
#123574=CARTESIAN_POINT('Ctrl Pts',(50.0161522238616,-52.4207124612608,
12.));
#123575=CARTESIAN_POINT('Ctrl Pts',(50.0065636229938,-52.3978116592509,
0.));
#123576=CARTESIAN_POINT('Ctrl Pts',(50.0065636229938,-52.3978116592509,
12.));
#123577=CARTESIAN_POINT('Ctrl Pts',(49.9969687627408,-52.3749574789871,
0.));
#123578=CARTESIAN_POINT('Ctrl Pts',(49.9969687627408,-52.3749574789871,
12.));
#123579=CARTESIAN_POINT('Ctrl Pts',(49.9873677385775,-52.3521500002718,
0.));
#123580=CARTESIAN_POINT('Ctrl Pts',(49.9873677385775,-52.3521500002718,
12.));
#123581=CARTESIAN_POINT('Ctrl Pts',(49.9777606464106,-52.3293893031528,
0.));
#123582=CARTESIAN_POINT('Ctrl Pts',(49.9777606464106,-52.3293893031528,
12.));
#123583=CARTESIAN_POINT('Ctrl Pts',(49.9681475825824,-52.3066754679265,
0.));
#123584=CARTESIAN_POINT('Ctrl Pts',(49.9681475825824,-52.3066754679265,
12.));
#123585=CARTESIAN_POINT('Ctrl Pts',(49.9585286438733,-52.2840085751384,
0.));
#123586=CARTESIAN_POINT('Ctrl Pts',(49.9585286438733,-52.2840085751384,
12.));
#123587=CARTESIAN_POINT('Ctrl Pts',(49.9489039275064,-52.2613887055773,
0.));
#123588=CARTESIAN_POINT('Ctrl Pts',(49.9489039275064,-52.2613887055773,
12.));
#123589=CARTESIAN_POINT('Ctrl Pts',(49.9392735311509,-52.2388159402771,
0.));
#123590=CARTESIAN_POINT('Ctrl Pts',(49.9392735311509,-52.2388159402771,
12.));
#123591=CARTESIAN_POINT('Ctrl Pts',(49.9296375529245,-52.2162903605275,
0.));
#123592=CARTESIAN_POINT('Ctrl Pts',(49.9296375529245,-52.2162903605275,
12.));
#123593=CARTESIAN_POINT('Ctrl Pts',(49.9199960913962,-52.1938120478754,
0.));
#123594=CARTESIAN_POINT('Ctrl Pts',(49.9199960913962,-52.1938120478754,
12.));
#123595=CARTESIAN_POINT('Ctrl Pts',(49.9103492455902,-52.1713810841276,
0.));
#123596=CARTESIAN_POINT('Ctrl Pts',(49.9103492455902,-52.1713810841276,
12.));
#123597=CARTESIAN_POINT('Ctrl Pts',(49.9006971149894,-52.1489975513445,
0.));
#123598=CARTESIAN_POINT('Ctrl Pts',(49.9006971149894,-52.1489975513445,
12.));
#123599=CARTESIAN_POINT('Ctrl Pts',(49.8910397995397,-52.1266615318407,
0.));
#123600=CARTESIAN_POINT('Ctrl Pts',(49.8910397995397,-52.1266615318407,
12.));
#123601=CARTESIAN_POINT('Ctrl Pts',(49.8813773996517,-52.1043731081962,
0.));
#123602=CARTESIAN_POINT('Ctrl Pts',(49.8813773996517,-52.1043731081962,
12.));
#123603=CARTESIAN_POINT('Ctrl Pts',(49.8717100162048,-52.0821323632587,
0.));
#123604=CARTESIAN_POINT('Ctrl Pts',(49.8717100162048,-52.0821323632587,
12.));
#123605=CARTESIAN_POINT('Ctrl Pts',(49.86203775055,-52.0599393801452,0.));
#123606=CARTESIAN_POINT('Ctrl Pts',(49.86203775055,-52.0599393801452,12.));
#123607=CARTESIAN_POINT('Ctrl Pts',(49.8523607045149,-52.0377942422376,
0.));
#123608=CARTESIAN_POINT('Ctrl Pts',(49.8523607045149,-52.0377942422376,
12.));
#123609=CARTESIAN_POINT('Ctrl Pts',(49.8426789804071,-52.0156970331823,
0.));
#123610=CARTESIAN_POINT('Ctrl Pts',(49.8426789804071,-52.0156970331823,
12.));
#123611=CARTESIAN_POINT('Ctrl Pts',(49.8329926810171,-51.9936478369008,
0.));
#123612=CARTESIAN_POINT('Ctrl Pts',(49.8329926810171,-51.9936478369008,
12.));
#123613=CARTESIAN_POINT('Ctrl Pts',(49.8233019096222,-51.9716467375937,
0.));
#123614=CARTESIAN_POINT('Ctrl Pts',(49.8233019096222,-51.9716467375937,
12.));
#123615=CARTESIAN_POINT('Ctrl Pts',(49.8136067699896,-51.9496938197418,
0.));
#123616=CARTESIAN_POINT('Ctrl Pts',(49.8136067699896,-51.9496938197418,
12.));
#123617=CARTESIAN_POINT('Ctrl Pts',(49.8039073663812,-51.9277891681018,
0.));
#123618=CARTESIAN_POINT('Ctrl Pts',(49.8039073663812,-51.9277891681018,
12.));
#123619=CARTESIAN_POINT('Ctrl Pts',(49.7942038035576,-51.9059328677059,
0.));
#123620=CARTESIAN_POINT('Ctrl Pts',(49.7942038035576,-51.9059328677059,
12.));
#123621=CARTESIAN_POINT('Ctrl Pts',(49.7844961867807,-51.8841250038724,
0.));
#123622=CARTESIAN_POINT('Ctrl Pts',(49.7844961867807,-51.8841250038724,
12.));
#123623=CARTESIAN_POINT('Ctrl Pts',(49.7747846218182,-51.8623656622097,
0.));
#123624=CARTESIAN_POINT('Ctrl Pts',(49.7747846218182,-51.8623656622097,
12.));
#123625=CARTESIAN_POINT('Ctrl Pts',(49.7650692149462,-51.8406549286175,
0.));
#123626=CARTESIAN_POINT('Ctrl Pts',(49.7650692149462,-51.8406549286175,
12.));
#123627=CARTESIAN_POINT('Ctrl Pts',(49.755350072955,-51.8189928892828,0.));
#123628=CARTESIAN_POINT('Ctrl Pts',(49.755350072955,-51.8189928892828,12.));
#123629=CARTESIAN_POINT('Ctrl Pts',(49.7456273031534,-51.7973796306803,
0.));
#123630=CARTESIAN_POINT('Ctrl Pts',(49.7456273031534,-51.7973796306803,
12.));
#123631=CARTESIAN_POINT('Ctrl Pts',(49.7359010133721,-51.7758152395836,
0.));
#123632=CARTESIAN_POINT('Ctrl Pts',(49.7359010133721,-51.7758152395836,
12.));
#123633=CARTESIAN_POINT('Ctrl Pts',(49.7261713119663,-51.754299803067,0.));
#123634=CARTESIAN_POINT('Ctrl Pts',(49.7261713119663,-51.754299803067,12.));
#123635=CARTESIAN_POINT('Ctrl Pts',(49.7164383078212,-51.7328334085091,
0.));
#123636=CARTESIAN_POINT('Ctrl Pts',(49.7164383078212,-51.7328334085091,
12.));
#123637=CARTESIAN_POINT('Ctrl Pts',(49.7067021103553,-51.7114161435869,
0.));
#123638=CARTESIAN_POINT('Ctrl Pts',(49.7067021103553,-51.7114161435869,
12.));
#123639=CARTESIAN_POINT('Ctrl Pts',(49.6969628295262,-51.6900480962773,
0.));
#123640=CARTESIAN_POINT('Ctrl Pts',(49.6969628295262,-51.6900480962773,
12.));
#123641=CARTESIAN_POINT('Ctrl Pts',(49.6872205758336,-51.6687293548682,
0.));
#123642=CARTESIAN_POINT('Ctrl Pts',(49.6872205758336,-51.6687293548682,
12.));
#123643=CARTESIAN_POINT('Ctrl Pts',(49.6774754603245,-51.6474600079622,
0.));
#123644=CARTESIAN_POINT('Ctrl Pts',(49.6774754603245,-51.6474600079622,
12.));
#123645=CARTESIAN_POINT('Ctrl Pts',(49.6677275945967,-51.6262401444791,
0.));
#123646=CARTESIAN_POINT('Ctrl Pts',(49.6677275945967,-51.6262401444791,
12.));
#123647=CARTESIAN_POINT('Ctrl Pts',(49.6579770908037,-51.6050698536496,
0.));
#123648=CARTESIAN_POINT('Ctrl Pts',(49.6579770908037,-51.6050698536496,
12.));
#123649=CARTESIAN_POINT('Ctrl Pts',(49.6482240616593,-51.5839492250181,
0.));
#123650=CARTESIAN_POINT('Ctrl Pts',(49.6482240616593,-51.5839492250181,
12.));
#123651=CARTESIAN_POINT('Ctrl Pts',(49.6384686204413,-51.5628783484525,
0.));
#123652=CARTESIAN_POINT('Ctrl Pts',(49.6384686204413,-51.5628783484525,
12.));
#123653=CARTESIAN_POINT('Ctrl Pts',(49.6287108809965,-51.5418573141484,
0.));
#123654=CARTESIAN_POINT('Ctrl Pts',(49.6287108809965,-51.5418573141484,
12.));
#123655=CARTESIAN_POINT('Ctrl Pts',(49.6189509577452,-51.5208862126315,
0.));
#123656=CARTESIAN_POINT('Ctrl Pts',(49.6189509577452,-51.5208862126315,
12.));
#123657=CARTESIAN_POINT('Ctrl Pts',(49.6091889656866,-51.4999651347523,
0.));
#123658=CARTESIAN_POINT('Ctrl Pts',(49.6091889656866,-51.4999651347523,
12.));
#123659=CARTESIAN_POINT('Ctrl Pts',(49.5994250204031,-51.4790941716888,
0.));
#123660=CARTESIAN_POINT('Ctrl Pts',(49.5994250204031,-51.4790941716888,
12.));
#123661=CARTESIAN_POINT('Ctrl Pts',(49.5896592380654,-51.4582734149583,
0.));
#123662=CARTESIAN_POINT('Ctrl Pts',(49.5896592380654,-51.4582734149583,
12.));
#123663=CARTESIAN_POINT('Ctrl Pts',(49.5798917354365,-51.4375029564197,
0.));
#123664=CARTESIAN_POINT('Ctrl Pts',(49.5798917354365,-51.4375029564197,
12.));
#123665=CARTESIAN_POINT('Ctrl Pts',(49.5701226298769,-51.4167828882756,
0.));
#123666=CARTESIAN_POINT('Ctrl Pts',(49.5701226298769,-51.4167828882756,
12.));
#123667=CARTESIAN_POINT('Ctrl Pts',(49.5603520393496,-51.396113303067,0.));
#123668=CARTESIAN_POINT('Ctrl Pts',(49.5603520393496,-51.396113303067,12.));
#123669=CARTESIAN_POINT('Ctrl Pts',(49.550580082425,-51.3754942936778,0.));
#123670=CARTESIAN_POINT('Ctrl Pts',(49.550580082425,-51.3754942936778,12.));
#123671=CARTESIAN_POINT('Ctrl Pts',(49.5408068782859,-51.3549259533458,
0.));
#123672=CARTESIAN_POINT('Ctrl Pts',(49.5408068782859,-51.3549259533458,
12.));
#123673=CARTESIAN_POINT('Ctrl Pts',(49.5310325467332,-51.3344083756657,
0.));
#123674=CARTESIAN_POINT('Ctrl Pts',(49.5310325467332,-51.3344083756657,
12.));
#123675=CARTESIAN_POINT('Ctrl Pts',(49.5212572081908,-51.313941654591,0.));
#123676=CARTESIAN_POINT('Ctrl Pts',(49.5212572081908,-51.313941654591,12.));
#123677=CARTESIAN_POINT('Ctrl Pts',(49.5114809837122,-51.2935258844289,
0.));
#123678=CARTESIAN_POINT('Ctrl Pts',(49.5114809837122,-51.2935258844289,
12.));
#123679=CARTESIAN_POINT('Ctrl Pts',(49.5017039949852,-51.2731611598475,
0.));
#123680=CARTESIAN_POINT('Ctrl Pts',(49.5017039949852,-51.2731611598475,
12.));
#123681=CARTESIAN_POINT('Ctrl Pts',(49.4919263643362,-51.2528475758846,
0.));
#123682=CARTESIAN_POINT('Ctrl Pts',(49.4919263643362,-51.2528475758846,
12.));
#123683=CARTESIAN_POINT('Ctrl Pts',(49.4821482147356,-51.2325852279506,
0.));
#123684=CARTESIAN_POINT('Ctrl Pts',(49.4821482147356,-51.2325852279506,
12.));
#123685=CARTESIAN_POINT('Ctrl Pts',(49.4723696698021,-51.2123742118287,
0.));
#123686=CARTESIAN_POINT('Ctrl Pts',(49.4723696698021,-51.2123742118287,
12.));
#123687=CARTESIAN_POINT('Ctrl Pts',(49.4625908538074,-51.1922146236686,
0.));
#123688=CARTESIAN_POINT('Ctrl Pts',(49.4625908538074,-51.1922146236686,
12.));
#123689=CARTESIAN_POINT('Ctrl Pts',(49.4528118916832,-51.1721065599973,
0.));
#123690=CARTESIAN_POINT('Ctrl Pts',(49.4528118916832,-51.1721065599973,
12.));
#123691=CARTESIAN_POINT('Ctrl Pts',(49.4430329090287,-51.1520501177291,
0.));
#123692=CARTESIAN_POINT('Ctrl Pts',(49.4430329090287,-51.1520501177291,
12.));
#123693=CARTESIAN_POINT('Ctrl Pts',(49.4332540321178,-51.1320453941702,
0.));
#123694=CARTESIAN_POINT('Ctrl Pts',(49.4332540321178,-51.1320453941702,
12.));
#123695=CARTESIAN_POINT('Ctrl Pts',(49.423475387907,-51.1120924870195,0.));
#123696=CARTESIAN_POINT('Ctrl Pts',(49.423475387907,-51.1120924870195,12.));
#123697=CARTESIAN_POINT('Ctrl Pts',(49.4136971040428,-51.0921914943662,
0.));
#123698=CARTESIAN_POINT('Ctrl Pts',(49.4136971040428,-51.0921914943662,
12.));
#123699=CARTESIAN_POINT('Ctrl Pts',(49.4039193088634,-51.0723425146985,
0.));
#123700=CARTESIAN_POINT('Ctrl Pts',(49.4039193088634,-51.0723425146985,
12.));
#123701=CARTESIAN_POINT('Ctrl Pts',(49.3941421314012,-51.052545646907,0.));
#123702=CARTESIAN_POINT('Ctrl Pts',(49.3941421314012,-51.052545646907,12.));
#123703=CARTESIAN_POINT('Ctrl Pts',(49.3843657013852,-51.0328009902858,
0.));
#123704=CARTESIAN_POINT('Ctrl Pts',(49.3843657013852,-51.0328009902858,
12.));
#123705=CARTESIAN_POINT('Ctrl Pts',(49.3745901492432,-51.0131086445272,
0.));
#123706=CARTESIAN_POINT('Ctrl Pts',(49.3745901492432,-51.0131086445272,
12.));
#123707=CARTESIAN_POINT('Ctrl Pts',(49.3648156061058,-50.9934687097188,
0.));
#123708=CARTESIAN_POINT('Ctrl Pts',(49.3648156061058,-50.9934687097188,
12.));
#123709=CARTESIAN_POINT('Ctrl Pts',(49.355042203823,-50.9738812863646,0.));
#123710=CARTESIAN_POINT('Ctrl Pts',(49.355042203823,-50.9738812863646,12.));
#123711=CARTESIAN_POINT('Ctrl Pts',(49.345270074981,-50.9543464753981,0.));
#123712=CARTESIAN_POINT('Ctrl Pts',(49.345270074981,-50.9543464753981,12.));
#123713=CARTESIAN_POINT('Ctrl Pts',(49.3354993529158,-50.9348643781924,
0.));
#123714=CARTESIAN_POINT('Ctrl Pts',(49.3354993529158,-50.9348643781924,
12.));
#123715=CARTESIAN_POINT('Ctrl Pts',(49.3257301717335,-50.9154350965666,
0.));
#123716=CARTESIAN_POINT('Ctrl Pts',(49.3257301717335,-50.9154350965666,
12.));
#123717=CARTESIAN_POINT('Ctrl Pts',(49.3159626663109,-50.8960587327848,
0.));
#123718=CARTESIAN_POINT('Ctrl Pts',(49.3159626663109,-50.8960587327848,
12.));
#123719=CARTESIAN_POINT('Ctrl Pts',(49.3061969722781,-50.8767353895492,
0.));
#123720=CARTESIAN_POINT('Ctrl Pts',(49.3061969722781,-50.8767353895492,
12.));
#123721=CARTESIAN_POINT('Ctrl Pts',(49.2964332260039,-50.8574651699873,
0.));
#123722=CARTESIAN_POINT('Ctrl Pts',(49.2964332260039,-50.8574651699873,
12.));
#123723=CARTESIAN_POINT('Ctrl Pts',(49.2866715645838,-50.8382481776403,
0.));
#123724=CARTESIAN_POINT('Ctrl Pts',(49.2866715645838,-50.8382481776403,
12.));
#123725=CARTESIAN_POINT('Ctrl Pts',(49.2769121258164,-50.819084516434,0.));
#123726=CARTESIAN_POINT('Ctrl Pts',(49.2769121258164,-50.819084516434,12.));
#123727=CARTESIAN_POINT('Ctrl Pts',(49.2671550482435,-50.7999742907131,
0.));
#123728=CARTESIAN_POINT('Ctrl Pts',(49.2671550482435,-50.7999742907131,
12.));
#123729=CARTESIAN_POINT('Ctrl Pts',(49.2574004712134,-50.7809176052966,
0.));
#123730=CARTESIAN_POINT('Ctrl Pts',(49.2574004712134,-50.7809176052966,
12.));
#123731=CARTESIAN_POINT('Ctrl Pts',(49.2476485349373,-50.7619145655207,
0.));
#123732=CARTESIAN_POINT('Ctrl Pts',(49.2476485349373,-50.7619145655207,
12.));
#123733=CARTESIAN_POINT('Ctrl Pts',(49.2378993805471,-50.7429652772805,
0.));
#123734=CARTESIAN_POINT('Ctrl Pts',(49.2378993805471,-50.7429652772805,
12.));
#123735=CARTESIAN_POINT('Ctrl Pts',(49.228153150155,-50.7240698470679,0.));
#123736=CARTESIAN_POINT('Ctrl Pts',(49.228153150155,-50.7240698470679,12.));
#123737=CARTESIAN_POINT('Ctrl Pts',(49.2184099867461,-50.7052283818922,
0.));
#123738=CARTESIAN_POINT('Ctrl Pts',(49.2184099867461,-50.7052283818922,
12.));
#123739=CARTESIAN_POINT('Ctrl Pts',(49.2086700340614,-50.6864409891895,
0.));
#123740=CARTESIAN_POINT('Ctrl Pts',(49.2086700340614,-50.6864409891895,
12.));
#123741=CARTESIAN_POINT('Ctrl Pts',(49.1989334364995,-50.6677077767432,
0.));
#123742=CARTESIAN_POINT('Ctrl Pts',(49.1989334364995,-50.6677077767432,
12.));
#123743=CARTESIAN_POINT('Ctrl Pts',(49.189200338976,-50.6490288525656,0.));
#123744=CARTESIAN_POINT('Ctrl Pts',(49.189200338976,-50.6490288525656,12.));
#123745=CARTESIAN_POINT('Ctrl Pts',(49.1794708869099,-50.6304043248821,
0.));
#123746=CARTESIAN_POINT('Ctrl Pts',(49.1794708869099,-50.6304043248821,
12.));
#123747=CARTESIAN_POINT('Ctrl Pts',(49.1697452265494,-50.6118343023958,
0.));
#123748=CARTESIAN_POINT('Ctrl Pts',(49.1697452265494,-50.6118343023958,
12.));
#123749=CARTESIAN_POINT('Ctrl Pts',(49.1600235052621,-50.5933188945168,
0.));
#123750=CARTESIAN_POINT('Ctrl Pts',(49.1600235052621,-50.5933188945168,
12.));
#123751=CARTESIAN_POINT('Ctrl Pts',(49.1503058717821,-50.5748582115565,
0.));
#123752=CARTESIAN_POINT('Ctrl Pts',(49.1503058717821,-50.5748582115565,
12.));
#123753=CARTESIAN_POINT('Ctrl Pts',(49.1405924766144,-50.556452365038,0.));
#123754=CARTESIAN_POINT('Ctrl Pts',(49.1405924766144,-50.556452365038,12.));
#123755=CARTESIAN_POINT('Ctrl Pts',(49.1308834717615,-50.5381014674791,
0.));
#123756=CARTESIAN_POINT('Ctrl Pts',(49.1308834717615,-50.5381014674791,
12.));
#123757=CARTESIAN_POINT('Ctrl Pts',(49.1211790099795,-50.5198056318089,
0.));
#123758=CARTESIAN_POINT('Ctrl Pts',(49.1211790099795,-50.5198056318089,
12.));
#123759=CARTESIAN_POINT('Ctrl Pts',(49.1114792441571,-50.501564970874,0.));
#123760=CARTESIAN_POINT('Ctrl Pts',(49.1114792441571,-50.501564970874,12.));
#123761=CARTESIAN_POINT('Ctrl Pts',(49.1017843266803,-50.4833795969318,
0.));
#123762=CARTESIAN_POINT('Ctrl Pts',(49.1017843266803,-50.4833795969318,
12.));
#123763=CARTESIAN_POINT('Ctrl Pts',(49.0920944087008,-50.4652496210607,
0.));
#123764=CARTESIAN_POINT('Ctrl Pts',(49.0920944087008,-50.4652496210607,
12.));
#123765=CARTESIAN_POINT('Ctrl Pts',(49.0824096415371,-50.4471751542751,
0.));
#123766=CARTESIAN_POINT('Ctrl Pts',(49.0824096415371,-50.4471751542751,
12.));
#123767=CARTESIAN_POINT('Ctrl Pts',(49.0727301783494,-50.4291563088547,
0.));
#123768=CARTESIAN_POINT('Ctrl Pts',(49.0727301783494,-50.4291563088547,
12.));
#123769=CARTESIAN_POINT('Ctrl Pts',(49.0630561755075,-50.4111931994257,
0.));
#123770=CARTESIAN_POINT('Ctrl Pts',(49.0630561755075,-50.4111931994257,
12.));
#123771=CARTESIAN_POINT('Ctrl Pts',(49.0533877945744,-50.3932859445252,
0.));
#123772=CARTESIAN_POINT('Ctrl Pts',(49.0533877945744,-50.3932859445252,
12.));
#123773=CARTESIAN_POINT('Ctrl Pts',(49.0437252024832,-50.3754346667353,
0.));
#123774=CARTESIAN_POINT('Ctrl Pts',(49.0437252024832,-50.3754346667353,
12.));
#123775=CARTESIAN_POINT('Ctrl Pts',(49.0340685673982,-50.3576394894108,
0.));
#123776=CARTESIAN_POINT('Ctrl Pts',(49.0340685673982,-50.3576394894108,
12.));
#123777=CARTESIAN_POINT('Ctrl Pts',(49.024418055075,-50.3399005337958,0.));
#123778=CARTESIAN_POINT('Ctrl Pts',(49.024418055075,-50.3399005337958,12.));
#123779=CARTESIAN_POINT('Ctrl Pts',(49.0147738256942,-50.3222179165119,
0.));
#123780=CARTESIAN_POINT('Ctrl Pts',(49.0147738256942,-50.3222179165119,
12.));
#123781=CARTESIAN_POINT('Ctrl Pts',(49.0051360288044,-50.3045917455424,
0.));
#123782=CARTESIAN_POINT('Ctrl Pts',(49.0051360288044,-50.3045917455424,
12.));
#123783=CARTESIAN_POINT('Ctrl Pts',(48.9955048082081,-50.2870221241054,
0.));
#123784=CARTESIAN_POINT('Ctrl Pts',(48.9955048082081,-50.2870221241054,
12.));
#123785=CARTESIAN_POINT('Ctrl Pts',(48.9858803116689,-50.2695091583511,
0.));
#123786=CARTESIAN_POINT('Ctrl Pts',(48.9858803116689,-50.2695091583511,
12.));
#123787=CARTESIAN_POINT('Ctrl Pts',(48.9762626987227,-50.252052963548,0.));
#123788=CARTESIAN_POINT('Ctrl Pts',(48.9762626987227,-50.252052963548,12.));
#123789=CARTESIAN_POINT('Ctrl Pts',(48.9666521500911,-50.234653671541,0.));
#123790=CARTESIAN_POINT('Ctrl Pts',(48.9666521500911,-50.234653671541,12.));
#123791=CARTESIAN_POINT('Ctrl Pts',(48.9570488741167,-50.2173114358325,
0.));
#123792=CARTESIAN_POINT('Ctrl Pts',(48.9570488741167,-50.2173114358325,
12.));
#123793=CARTESIAN_POINT('Ctrl Pts',(48.9474530868733,-50.2000264157797,
0.));
#123794=CARTESIAN_POINT('Ctrl Pts',(48.9474530868733,-50.2000264157797,
12.));
#123795=CARTESIAN_POINT('Ctrl Pts',(48.9378649933055,-50.1827987615602,
0.));
#123796=CARTESIAN_POINT('Ctrl Pts',(48.9378649933055,-50.1827987615602,
12.));
#123797=CARTESIAN_POINT('Ctrl Pts',(48.9282847698294,-50.1656286003997,
0.));
#123798=CARTESIAN_POINT('Ctrl Pts',(48.9282847698294,-50.1656286003997,
12.));
#123799=CARTESIAN_POINT('Ctrl Pts',(48.9187125418099,-50.1485160184657,
0.));
#123800=CARTESIAN_POINT('Ctrl Pts',(48.9187125418099,-50.1485160184657,
12.));
#123801=CARTESIAN_POINT('Ctrl Pts',(48.90914838181,-50.1314610602569,0.));
#123802=CARTESIAN_POINT('Ctrl Pts',(48.90914838181,-50.1314610602569,12.));
#123803=CARTESIAN_POINT('Ctrl Pts',(48.9015035372055,-50.1178632067084,
0.));
#123804=CARTESIAN_POINT('Ctrl Pts',(48.9015035372055,-50.1178632067084,
12.));
#123805=CARTESIAN_POINT('Ctrl Pts',(48.895773555686,-50.1076907555471,0.));
#123806=CARTESIAN_POINT('Ctrl Pts',(48.895773555686,-50.1076907555471,12.));
#123807=CARTESIAN_POINT('Ctrl Pts',(48.8919551910366,-50.1009206494272,
0.));
#123808=CARTESIAN_POINT('Ctrl Pts',(48.8919551910366,-50.1009206494272,
12.));
#123809=CARTESIAN_POINT('Ctrl Pts',(48.8900464144686,-50.0975384783635,
0.));
#123810=CARTESIAN_POINT('Ctrl Pts',(48.8900464144686,-50.0975384783635,
12.));
#123811=CARTESIAN_POINT('',(48.8900464144686,-50.0975384783635,12.));
#123812=CARTESIAN_POINT('Ctrl Pts',(48.8900464144686,-50.0975384783635,
12.));
#123813=CARTESIAN_POINT('Ctrl Pts',(48.8919551910366,-50.1009206494272,
12.));
#123814=CARTESIAN_POINT('Ctrl Pts',(48.895773555686,-50.1076907555471,12.));
#123815=CARTESIAN_POINT('Ctrl Pts',(48.9015035372055,-50.1178632067084,
12.));
#123816=CARTESIAN_POINT('Ctrl Pts',(48.90914838181,-50.1314610602569,12.));
#123817=CARTESIAN_POINT('Ctrl Pts',(48.9187125418099,-50.1485160184657,
12.));
#123818=CARTESIAN_POINT('Ctrl Pts',(48.9282847698294,-50.1656286003997,
12.));
#123819=CARTESIAN_POINT('Ctrl Pts',(48.9378649933055,-50.1827987615602,
12.));
#123820=CARTESIAN_POINT('Ctrl Pts',(48.9474530868733,-50.2000264157797,
12.));
#123821=CARTESIAN_POINT('Ctrl Pts',(48.9570488741167,-50.2173114358325,
12.));
#123822=CARTESIAN_POINT('Ctrl Pts',(48.9666521500911,-50.234653671541,12.));
#123823=CARTESIAN_POINT('Ctrl Pts',(48.9762626987227,-50.252052963548,12.));
#123824=CARTESIAN_POINT('Ctrl Pts',(48.9858803116689,-50.2695091583511,
12.));
#123825=CARTESIAN_POINT('Ctrl Pts',(48.9955048082081,-50.2870221241054,
12.));
#123826=CARTESIAN_POINT('Ctrl Pts',(49.0051360288044,-50.3045917455424,
12.));
#123827=CARTESIAN_POINT('Ctrl Pts',(49.0147738256942,-50.3222179165119,
12.));
#123828=CARTESIAN_POINT('Ctrl Pts',(49.024418055075,-50.3399005337958,12.));
#123829=CARTESIAN_POINT('Ctrl Pts',(49.0340685673982,-50.3576394894108,
12.));
#123830=CARTESIAN_POINT('Ctrl Pts',(49.0437252024832,-50.3754346667353,
12.));
#123831=CARTESIAN_POINT('Ctrl Pts',(49.0533877945744,-50.3932859445252,
12.));
#123832=CARTESIAN_POINT('Ctrl Pts',(49.0630561755075,-50.4111931994257,
12.));
#123833=CARTESIAN_POINT('Ctrl Pts',(49.0727301783494,-50.4291563088547,
12.));
#123834=CARTESIAN_POINT('Ctrl Pts',(49.0824096415371,-50.4471751542751,
12.));
#123835=CARTESIAN_POINT('Ctrl Pts',(49.0920944087008,-50.4652496210607,
12.));
#123836=CARTESIAN_POINT('Ctrl Pts',(49.1017843266803,-50.4833795969318,
12.));
#123837=CARTESIAN_POINT('Ctrl Pts',(49.1114792441571,-50.501564970874,12.));
#123838=CARTESIAN_POINT('Ctrl Pts',(49.1211790099795,-50.5198056318089,
12.));
#123839=CARTESIAN_POINT('Ctrl Pts',(49.1308834717615,-50.5381014674791,
12.));
#123840=CARTESIAN_POINT('Ctrl Pts',(49.1405924766144,-50.556452365038,12.));
#123841=CARTESIAN_POINT('Ctrl Pts',(49.1503058717821,-50.5748582115565,
12.));
#123842=CARTESIAN_POINT('Ctrl Pts',(49.1600235052621,-50.5933188945168,
12.));
#123843=CARTESIAN_POINT('Ctrl Pts',(49.1697452265494,-50.6118343023958,
12.));
#123844=CARTESIAN_POINT('Ctrl Pts',(49.1794708869099,-50.6304043248821,
12.));
#123845=CARTESIAN_POINT('Ctrl Pts',(49.189200338976,-50.6490288525656,12.));
#123846=CARTESIAN_POINT('Ctrl Pts',(49.1989334364995,-50.6677077767432,
12.));
#123847=CARTESIAN_POINT('Ctrl Pts',(49.2086700340614,-50.6864409891895,
12.));
#123848=CARTESIAN_POINT('Ctrl Pts',(49.2184099867461,-50.7052283818922,
12.));
#123849=CARTESIAN_POINT('Ctrl Pts',(49.228153150155,-50.7240698470679,12.));
#123850=CARTESIAN_POINT('Ctrl Pts',(49.2378993805471,-50.7429652772805,
12.));
#123851=CARTESIAN_POINT('Ctrl Pts',(49.2476485349373,-50.7619145655207,
12.));
#123852=CARTESIAN_POINT('Ctrl Pts',(49.2574004712134,-50.7809176052966,
12.));
#123853=CARTESIAN_POINT('Ctrl Pts',(49.2671550482435,-50.7999742907131,
12.));
#123854=CARTESIAN_POINT('Ctrl Pts',(49.2769121258164,-50.819084516434,12.));
#123855=CARTESIAN_POINT('Ctrl Pts',(49.2866715645838,-50.8382481776403,
12.));
#123856=CARTESIAN_POINT('Ctrl Pts',(49.2964332260039,-50.8574651699873,
12.));
#123857=CARTESIAN_POINT('Ctrl Pts',(49.3061969722781,-50.8767353895492,
12.));
#123858=CARTESIAN_POINT('Ctrl Pts',(49.3159626663109,-50.8960587327848,
12.));
#123859=CARTESIAN_POINT('Ctrl Pts',(49.3257301717335,-50.9154350965666,
12.));
#123860=CARTESIAN_POINT('Ctrl Pts',(49.3354993529158,-50.9348643781924,
12.));
#123861=CARTESIAN_POINT('Ctrl Pts',(49.345270074981,-50.9543464753981,12.));
#123862=CARTESIAN_POINT('Ctrl Pts',(49.355042203823,-50.9738812863646,12.));
#123863=CARTESIAN_POINT('Ctrl Pts',(49.3648156061058,-50.9934687097188,
12.));
#123864=CARTESIAN_POINT('Ctrl Pts',(49.3745901492432,-51.0131086445272,
12.));
#123865=CARTESIAN_POINT('Ctrl Pts',(49.3843657013852,-51.0328009902858,
12.));
#123866=CARTESIAN_POINT('Ctrl Pts',(49.3941421314012,-51.052545646907,12.));
#123867=CARTESIAN_POINT('Ctrl Pts',(49.4039193088634,-51.0723425146985,
12.));
#123868=CARTESIAN_POINT('Ctrl Pts',(49.4136971040428,-51.0921914943662,
12.));
#123869=CARTESIAN_POINT('Ctrl Pts',(49.423475387907,-51.1120924870195,12.));
#123870=CARTESIAN_POINT('Ctrl Pts',(49.4332540321178,-51.1320453941702,
12.));
#123871=CARTESIAN_POINT('Ctrl Pts',(49.4430329090287,-51.1520501177291,
12.));
#123872=CARTESIAN_POINT('Ctrl Pts',(49.4528118916832,-51.1721065599973,
12.));
#123873=CARTESIAN_POINT('Ctrl Pts',(49.4625908538074,-51.1922146236686,
12.));
#123874=CARTESIAN_POINT('Ctrl Pts',(49.4723696698021,-51.2123742118287,
12.));
#123875=CARTESIAN_POINT('Ctrl Pts',(49.4821482147356,-51.2325852279506,
12.));
#123876=CARTESIAN_POINT('Ctrl Pts',(49.4919263643362,-51.2528475758846,
12.));
#123877=CARTESIAN_POINT('Ctrl Pts',(49.5017039949852,-51.2731611598475,
12.));
#123878=CARTESIAN_POINT('Ctrl Pts',(49.5114809837122,-51.2935258844289,
12.));
#123879=CARTESIAN_POINT('Ctrl Pts',(49.5212572081908,-51.313941654591,12.));
#123880=CARTESIAN_POINT('Ctrl Pts',(49.5310325467332,-51.3344083756657,
12.));
#123881=CARTESIAN_POINT('Ctrl Pts',(49.5408068782859,-51.3549259533458,
12.));
#123882=CARTESIAN_POINT('Ctrl Pts',(49.550580082425,-51.3754942936778,12.));
#123883=CARTESIAN_POINT('Ctrl Pts',(49.5603520393496,-51.396113303067,12.));
#123884=CARTESIAN_POINT('Ctrl Pts',(49.5701226298769,-51.4167828882756,
12.));
#123885=CARTESIAN_POINT('Ctrl Pts',(49.5798917354365,-51.4375029564197,
12.));
#123886=CARTESIAN_POINT('Ctrl Pts',(49.5896592380654,-51.4582734149583,
12.));
#123887=CARTESIAN_POINT('Ctrl Pts',(49.5994250204031,-51.4790941716888,
12.));
#123888=CARTESIAN_POINT('Ctrl Pts',(49.6091889656866,-51.4999651347523,
12.));
#123889=CARTESIAN_POINT('Ctrl Pts',(49.6189509577452,-51.5208862126315,
12.));
#123890=CARTESIAN_POINT('Ctrl Pts',(49.6287108809965,-51.5418573141484,
12.));
#123891=CARTESIAN_POINT('Ctrl Pts',(49.6384686204413,-51.5628783484525,
12.));
#123892=CARTESIAN_POINT('Ctrl Pts',(49.6482240616593,-51.5839492250181,
12.));
#123893=CARTESIAN_POINT('Ctrl Pts',(49.6579770908037,-51.6050698536496,
12.));
#123894=CARTESIAN_POINT('Ctrl Pts',(49.6677275945967,-51.6262401444791,
12.));
#123895=CARTESIAN_POINT('Ctrl Pts',(49.6774754603245,-51.6474600079622,
12.));
#123896=CARTESIAN_POINT('Ctrl Pts',(49.6872205758336,-51.6687293548682,
12.));
#123897=CARTESIAN_POINT('Ctrl Pts',(49.6969628295262,-51.6900480962773,
12.));
#123898=CARTESIAN_POINT('Ctrl Pts',(49.7067021103553,-51.7114161435869,
12.));
#123899=CARTESIAN_POINT('Ctrl Pts',(49.7164383078212,-51.7328334085091,
12.));
#123900=CARTESIAN_POINT('Ctrl Pts',(49.7261713119663,-51.754299803067,12.));
#123901=CARTESIAN_POINT('Ctrl Pts',(49.7359010133721,-51.7758152395836,
12.));
#123902=CARTESIAN_POINT('Ctrl Pts',(49.7456273031534,-51.7973796306803,
12.));
#123903=CARTESIAN_POINT('Ctrl Pts',(49.755350072955,-51.8189928892828,12.));
#123904=CARTESIAN_POINT('Ctrl Pts',(49.7650692149462,-51.8406549286175,
12.));
#123905=CARTESIAN_POINT('Ctrl Pts',(49.7747846218182,-51.8623656622097,
12.));
#123906=CARTESIAN_POINT('Ctrl Pts',(49.7844961867807,-51.8841250038724,
12.));
#123907=CARTESIAN_POINT('Ctrl Pts',(49.7942038035576,-51.9059328677059,
12.));
#123908=CARTESIAN_POINT('Ctrl Pts',(49.8039073663812,-51.9277891681018,
12.));
#123909=CARTESIAN_POINT('Ctrl Pts',(49.8136067699896,-51.9496938197418,
12.));
#123910=CARTESIAN_POINT('Ctrl Pts',(49.8233019096222,-51.9716467375937,
12.));
#123911=CARTESIAN_POINT('Ctrl Pts',(49.8329926810171,-51.9936478369008,
12.));
#123912=CARTESIAN_POINT('Ctrl Pts',(49.8426789804071,-52.0156970331823,
12.));
#123913=CARTESIAN_POINT('Ctrl Pts',(49.8523607045149,-52.0377942422376,
12.));
#123914=CARTESIAN_POINT('Ctrl Pts',(49.86203775055,-52.0599393801452,12.));
#123915=CARTESIAN_POINT('Ctrl Pts',(49.8717100162048,-52.0821323632587,
12.));
#123916=CARTESIAN_POINT('Ctrl Pts',(49.8813773996517,-52.1043731081962,
12.));
#123917=CARTESIAN_POINT('Ctrl Pts',(49.8910397995397,-52.1266615318407,
12.));
#123918=CARTESIAN_POINT('Ctrl Pts',(49.9006971149894,-52.1489975513445,
12.));
#123919=CARTESIAN_POINT('Ctrl Pts',(49.9103492455902,-52.1713810841276,
12.));
#123920=CARTESIAN_POINT('Ctrl Pts',(49.9199960913962,-52.1938120478754,
12.));
#123921=CARTESIAN_POINT('Ctrl Pts',(49.9296375529245,-52.2162903605275,
12.));
#123922=CARTESIAN_POINT('Ctrl Pts',(49.9392735311509,-52.2388159402771,
12.));
#123923=CARTESIAN_POINT('Ctrl Pts',(49.9489039275064,-52.2613887055773,
12.));
#123924=CARTESIAN_POINT('Ctrl Pts',(49.9585286438733,-52.2840085751384,
12.));
#123925=CARTESIAN_POINT('Ctrl Pts',(49.9681475825824,-52.3066754679265,
12.));
#123926=CARTESIAN_POINT('Ctrl Pts',(49.9777606464106,-52.3293893031528,
12.));
#123927=CARTESIAN_POINT('Ctrl Pts',(49.9873677385775,-52.3521500002718,
12.));
#123928=CARTESIAN_POINT('Ctrl Pts',(49.9969687627408,-52.3749574789871,
12.));
#123929=CARTESIAN_POINT('Ctrl Pts',(50.0065636229938,-52.3978116592509,
12.));
#123930=CARTESIAN_POINT('Ctrl Pts',(50.0161522238616,-52.4207124612608,
12.));
#123931=CARTESIAN_POINT('Ctrl Pts',(50.0257344703,-52.4436598054515,12.));
#123932=CARTESIAN_POINT('Ctrl Pts',(50.0353102676921,-52.4666536124913,
12.));
#123933=CARTESIAN_POINT('Ctrl Pts',(50.0448795218441,-52.4896938032884,
12.));
#123934=CARTESIAN_POINT('Ctrl Pts',(50.0544421389817,-52.5127802989896,
12.));
#123935=CARTESIAN_POINT('Ctrl Pts',(50.0639980257479,-52.5359130209792,
12.));
#123936=CARTESIAN_POINT('Ctrl Pts',(50.0735470892007,-52.5590918908702,
12.));
#123937=CARTESIAN_POINT('Ctrl Pts',(50.0830892368107,-52.5823168304994,
12.));
#123938=CARTESIAN_POINT('Ctrl Pts',(50.0926243764578,-52.6055877619348,
12.));
#123939=CARTESIAN_POINT('Ctrl Pts',(50.1021524164264,-52.6289046074746,
12.));
#123940=CARTESIAN_POINT('Ctrl Pts',(50.111673265404,-52.652267289646,12.));
#123941=CARTESIAN_POINT('Ctrl Pts',(50.121186832478,-52.6756757311978,12.));
#123942=CARTESIAN_POINT('Ctrl Pts',(50.1306930271345,-52.699129855093,12.));
#123943=CARTESIAN_POINT('Ctrl Pts',(50.1401917592537,-52.7226295845161,
12.));
#123944=CARTESIAN_POINT('Ctrl Pts',(50.1496829391073,-52.7461748428738,
12.));
#123945=CARTESIAN_POINT('Ctrl Pts',(50.1591664773561,-52.769765553794,12.));
#123946=CARTESIAN_POINT('Ctrl Pts',(50.1686422850487,-52.7934016411205,
12.));
#123947=CARTESIAN_POINT('Ctrl Pts',(50.1781102736205,-52.8170830289044,
12.));
#123948=CARTESIAN_POINT('Ctrl Pts',(50.1875703548884,-52.8408096414093,
12.));
#123949=CARTESIAN_POINT('Ctrl Pts',(50.1970224410471,-52.8645814031133,
12.));
#123950=CARTESIAN_POINT('Ctrl Pts',(50.2064664446663,-52.8883982387068,
12.));
#123951=CARTESIAN_POINT('Ctrl Pts',(50.2159022786879,-52.9122600730884,
12.));
#123952=CARTESIAN_POINT('Ctrl Pts',(50.2253298564241,-52.9361668313542,
12.));
#123953=CARTESIAN_POINT('Ctrl Pts',(50.2347490915555,-52.9601184388028,
12.));
#123954=CARTESIAN_POINT('Ctrl Pts',(50.2441598981286,-52.9841148209402,
12.));
#123955=CARTESIAN_POINT('Ctrl Pts',(50.2535621905552,-53.0081559034801,
12.));
#123956=CARTESIAN_POINT('Ctrl Pts',(50.2629558836111,-53.0322416123406,
12.));
#123957=CARTESIAN_POINT('Ctrl Pts',(50.2723408924373,-53.0563718736366,
12.));
#123958=CARTESIAN_POINT('Ctrl Pts',(50.2817171325358,-53.0805466136798,
12.));
#123959=CARTESIAN_POINT('Ctrl Pts',(50.2910845197619,-53.1047657589812,
12.));
#123960=CARTESIAN_POINT('Ctrl Pts',(50.300442970319,-53.1290292362485,12.));
#123961=CARTESIAN_POINT('Ctrl Pts',(50.3097924007534,-53.1533369723818,
12.));
#123962=CARTESIAN_POINT('Ctrl Pts',(50.3191327279492,-53.1776888944616,
12.));
#123963=CARTESIAN_POINT('Ctrl Pts',(50.3284638691278,-53.2020849297471,
12.));
#123964=CARTESIAN_POINT('Ctrl Pts',(50.3377857418514,-53.2265250056887,
12.));
#123965=CARTESIAN_POINT('Ctrl Pts',(50.3470982640289,-53.2510090499336,
12.));
#123966=CARTESIAN_POINT('Ctrl Pts',(50.3564013539199,-53.2755369903293,
12.));
#123967=CARTESIAN_POINT('Ctrl Pts',(50.365694930143,-53.300108754923,12.));
#123968=CARTESIAN_POINT('Ctrl Pts',(50.3749789116786,-53.3247242719587,
12.));
#123969=CARTESIAN_POINT('Ctrl Pts',(50.384253217846,-53.3493834698697,12.));
#123970=CARTESIAN_POINT('Ctrl Pts',(50.3935177682837,-53.3740862772681,
12.));
#123971=CARTESIAN_POINT('Ctrl Pts',(50.4027724829297,-53.398832622931,12.));
#123972=CARTESIAN_POINT('Ctrl Pts',(50.4120172820047,-53.4236224357838,
12.));
#123973=CARTESIAN_POINT('Ctrl Pts',(50.4212520859914,-53.4484556448776,
12.));
#123974=CARTESIAN_POINT('Ctrl Pts',(50.4304768156666,-53.4733321794188,
12.));
#123975=CARTESIAN_POINT('Ctrl Pts',(50.4396913921381,-53.4982519688024,
12.));
#123976=CARTESIAN_POINT('Ctrl Pts',(50.4488957368839,-53.5232149426413,
12.));
#123977=CARTESIAN_POINT('Ctrl Pts',(50.4580897717838,-53.5482210307868,
12.));
#123978=CARTESIAN_POINT('Ctrl Pts',(50.4672734191756,-53.5732701633609,
12.));
#123979=CARTESIAN_POINT('Ctrl Pts',(50.4764466018071,-53.5983622707238,
12.));
#123980=CARTESIAN_POINT('Ctrl Pts',(50.4856092427314,-53.623497283406,12.));
#123981=CARTESIAN_POINT('Ctrl Pts',(50.4947612652148,-53.6486751320436,
12.));
#123982=CARTESIAN_POINT('Ctrl Pts',(50.503902592653,-53.6738957473158,12.));
#123983=CARTESIAN_POINT('Ctrl Pts',(50.513033148456,-53.6991590598548,12.));
#123984=CARTESIAN_POINT('Ctrl Pts',(50.522152856042,-53.7244650002374,12.));
#123985=CARTESIAN_POINT('Ctrl Pts',(50.5312616390779,-53.7498134991703,
12.));
#123986=CARTESIAN_POINT('Ctrl Pts',(50.5403594216698,-53.7752044876304,
12.));
#123987=CARTESIAN_POINT('Ctrl Pts',(50.5494461285761,-53.8006378970197,
12.));
#123988=CARTESIAN_POINT('Ctrl Pts',(50.5585216854091,-53.8261136593075,
12.));
#123989=CARTESIAN_POINT('Ctrl Pts',(50.5675860188538,-53.8516317071804,
12.));
#123990=CARTESIAN_POINT('Ctrl Pts',(50.5766390561884,-53.8771919737032,
12.));
#123991=CARTESIAN_POINT('Ctrl Pts',(50.5856807248151,-53.9027943919836,
12.));
#123992=CARTESIAN_POINT('Ctrl Pts',(50.5947109517483,-53.9284388948004,
12.));
#123993=CARTESIAN_POINT('Ctrl Pts',(50.6037296632139,-53.9541254143119,
12.));
#123994=CARTESIAN_POINT('Ctrl Pts',(50.6127367839711,-53.979853881553,12.));
#123995=CARTESIAN_POINT('Ctrl Pts',(50.6217322378648,-54.0056242268399,
12.));
#123996=CARTESIAN_POINT('Ctrl Pts',(50.6307159490553,-54.0314363806708,
12.));
#123997=CARTESIAN_POINT('Ctrl Pts',(50.6396878430939,-54.0572902745076,
12.));
#123998=CARTESIAN_POINT('Ctrl Pts',(50.6486478479465,-54.0831858415189,
12.));
#123999=CARTESIAN_POINT('Ctrl Pts',(50.6575958953221,-54.1091230175367,
12.));
#124000=CARTESIAN_POINT('Ctrl Pts',(50.6665319209869,-54.1351017412804,
12.));
#124001=CARTESIAN_POINT('Ctrl Pts',(50.6741814675485,-54.1574061042042,
12.));
#124002=CARTESIAN_POINT('Ctrl Pts',(50.6800396668777,-54.1745287898794,
12.));
#124003=CARTESIAN_POINT('Ctrl Pts',(50.684111886193,-54.1864514382193,12.));
#124004=CARTESIAN_POINT('Ctrl Pts',(50.6864016965742,-54.1931619277619,
12.));
#124005=CARTESIAN_POINT('Ctrl Pts',(50.6869108458849,-54.1946543500368,
12.));
#124006=CARTESIAN_POINT('',(48.8900464144686,-50.0975384783635,0.));
#124007=CARTESIAN_POINT('',(48.8900464144686,-50.0975384783634,0.));
#124008=CARTESIAN_POINT('Ctrl Pts',(50.6869108458849,-54.1946543500368,
0.));
#124009=CARTESIAN_POINT('Ctrl Pts',(50.6864016965742,-54.1931619277619,
0.));
#124010=CARTESIAN_POINT('Ctrl Pts',(50.684111886193,-54.1864514382193,0.));
#124011=CARTESIAN_POINT('Ctrl Pts',(50.6800396668777,-54.1745287898794,
0.));
#124012=CARTESIAN_POINT('Ctrl Pts',(50.6741814675486,-54.1574061042042,
0.));
#124013=CARTESIAN_POINT('Ctrl Pts',(50.6665319209869,-54.1351017412804,
0.));
#124014=CARTESIAN_POINT('Ctrl Pts',(50.6575958953221,-54.1091230175367,
0.));
#124015=CARTESIAN_POINT('Ctrl Pts',(50.6486478479465,-54.0831858415189,
0.));
#124016=CARTESIAN_POINT('Ctrl Pts',(50.6396878430939,-54.0572902745076,
0.));
#124017=CARTESIAN_POINT('Ctrl Pts',(50.6307159490553,-54.0314363806708,
0.));
#124018=CARTESIAN_POINT('Ctrl Pts',(50.6217322378648,-54.0056242268399,
0.));
#124019=CARTESIAN_POINT('Ctrl Pts',(50.6127367839711,-53.979853881553,0.));
#124020=CARTESIAN_POINT('Ctrl Pts',(50.6037296632139,-53.9541254143119,
0.));
#124021=CARTESIAN_POINT('Ctrl Pts',(50.5947109517483,-53.9284388948004,
0.));
#124022=CARTESIAN_POINT('Ctrl Pts',(50.5856807248151,-53.9027943919836,
0.));
#124023=CARTESIAN_POINT('Ctrl Pts',(50.5766390561884,-53.8771919737032,
0.));
#124024=CARTESIAN_POINT('Ctrl Pts',(50.5675860188538,-53.8516317071804,
0.));
#124025=CARTESIAN_POINT('Ctrl Pts',(50.5585216854091,-53.8261136593075,
0.));
#124026=CARTESIAN_POINT('Ctrl Pts',(50.5494461285761,-53.8006378970197,
0.));
#124027=CARTESIAN_POINT('Ctrl Pts',(50.5403594216698,-53.7752044876304,
0.));
#124028=CARTESIAN_POINT('Ctrl Pts',(50.5312616390779,-53.7498134991703,
0.));
#124029=CARTESIAN_POINT('Ctrl Pts',(50.522152856042,-53.7244650002374,0.));
#124030=CARTESIAN_POINT('Ctrl Pts',(50.513033148456,-53.6991590598548,0.));
#124031=CARTESIAN_POINT('Ctrl Pts',(50.503902592653,-53.6738957473158,0.));
#124032=CARTESIAN_POINT('Ctrl Pts',(50.4947612652148,-53.6486751320436,
0.));
#124033=CARTESIAN_POINT('Ctrl Pts',(50.4856092427314,-53.623497283406,0.));
#124034=CARTESIAN_POINT('Ctrl Pts',(50.4764466018071,-53.5983622707238,
0.));
#124035=CARTESIAN_POINT('Ctrl Pts',(50.4672734191756,-53.5732701633609,
0.));
#124036=CARTESIAN_POINT('Ctrl Pts',(50.4580897717838,-53.5482210307868,
0.));
#124037=CARTESIAN_POINT('Ctrl Pts',(50.4488957368839,-53.5232149426413,
0.));
#124038=CARTESIAN_POINT('Ctrl Pts',(50.4396913921381,-53.4982519688024,
0.));
#124039=CARTESIAN_POINT('Ctrl Pts',(50.4304768156666,-53.4733321794188,
0.));
#124040=CARTESIAN_POINT('Ctrl Pts',(50.4212520859914,-53.4484556448776,
0.));
#124041=CARTESIAN_POINT('Ctrl Pts',(50.4120172820047,-53.4236224357838,
0.));
#124042=CARTESIAN_POINT('Ctrl Pts',(50.4027724829297,-53.398832622931,0.));
#124043=CARTESIAN_POINT('Ctrl Pts',(50.3935177682837,-53.3740862772681,
0.));
#124044=CARTESIAN_POINT('Ctrl Pts',(50.384253217846,-53.3493834698697,0.));
#124045=CARTESIAN_POINT('Ctrl Pts',(50.3749789116786,-53.3247242719587,
0.));
#124046=CARTESIAN_POINT('Ctrl Pts',(50.365694930143,-53.300108754923,0.));
#124047=CARTESIAN_POINT('Ctrl Pts',(50.3564013539199,-53.2755369903293,
0.));
#124048=CARTESIAN_POINT('Ctrl Pts',(50.3470982640289,-53.2510090499336,
0.));
#124049=CARTESIAN_POINT('Ctrl Pts',(50.3377857418514,-53.2265250056887,
0.));
#124050=CARTESIAN_POINT('Ctrl Pts',(50.3284638691278,-53.2020849297471,
0.));
#124051=CARTESIAN_POINT('Ctrl Pts',(50.3191327279492,-53.1776888944616,
0.));
#124052=CARTESIAN_POINT('Ctrl Pts',(50.3097924007534,-53.1533369723818,
0.));
#124053=CARTESIAN_POINT('Ctrl Pts',(50.300442970319,-53.1290292362485,0.));
#124054=CARTESIAN_POINT('Ctrl Pts',(50.2910845197619,-53.1047657589812,
0.));
#124055=CARTESIAN_POINT('Ctrl Pts',(50.2817171325358,-53.0805466136798,
0.));
#124056=CARTESIAN_POINT('Ctrl Pts',(50.2723408924373,-53.0563718736366,
0.));
#124057=CARTESIAN_POINT('Ctrl Pts',(50.2629558836111,-53.0322416123406,
0.));
#124058=CARTESIAN_POINT('Ctrl Pts',(50.2535621905552,-53.0081559034801,
0.));
#124059=CARTESIAN_POINT('Ctrl Pts',(50.2441598981286,-52.9841148209402,
0.));
#124060=CARTESIAN_POINT('Ctrl Pts',(50.2347490915555,-52.9601184388028,
0.));
#124061=CARTESIAN_POINT('Ctrl Pts',(50.2253298564241,-52.9361668313542,
0.));
#124062=CARTESIAN_POINT('Ctrl Pts',(50.2159022786879,-52.9122600730884,
0.));
#124063=CARTESIAN_POINT('Ctrl Pts',(50.2064664446663,-52.8883982387068,
0.));
#124064=CARTESIAN_POINT('Ctrl Pts',(50.1970224410471,-52.8645814031133,
0.));
#124065=CARTESIAN_POINT('Ctrl Pts',(50.1875703548884,-52.8408096414093,
0.));
#124066=CARTESIAN_POINT('Ctrl Pts',(50.1781102736205,-52.8170830289044,
0.));
#124067=CARTESIAN_POINT('Ctrl Pts',(50.1686422850487,-52.7934016411205,
0.));
#124068=CARTESIAN_POINT('Ctrl Pts',(50.1591664773561,-52.769765553794,0.));
#124069=CARTESIAN_POINT('Ctrl Pts',(50.1496829391073,-52.7461748428738,
0.));
#124070=CARTESIAN_POINT('Ctrl Pts',(50.1401917592537,-52.7226295845161,
0.));
#124071=CARTESIAN_POINT('Ctrl Pts',(50.1306930271345,-52.699129855093,0.));
#124072=CARTESIAN_POINT('Ctrl Pts',(50.121186832478,-52.6756757311978,0.));
#124073=CARTESIAN_POINT('Ctrl Pts',(50.111673265404,-52.652267289646,0.));
#124074=CARTESIAN_POINT('Ctrl Pts',(50.1021524164264,-52.6289046074746,
0.));
#124075=CARTESIAN_POINT('Ctrl Pts',(50.0926243764578,-52.6055877619348,
0.));
#124076=CARTESIAN_POINT('Ctrl Pts',(50.0830892368107,-52.5823168304994,
0.));
#124077=CARTESIAN_POINT('Ctrl Pts',(50.0735470892007,-52.5590918908702,
0.));
#124078=CARTESIAN_POINT('Ctrl Pts',(50.0639980257479,-52.5359130209792,
0.));
#124079=CARTESIAN_POINT('Ctrl Pts',(50.0544421389817,-52.5127802989896,
0.));
#124080=CARTESIAN_POINT('Ctrl Pts',(50.0448795218441,-52.4896938032884,
0.));
#124081=CARTESIAN_POINT('Ctrl Pts',(50.0353102676921,-52.4666536124913,
0.));
#124082=CARTESIAN_POINT('Ctrl Pts',(50.0257344703,-52.4436598054515,0.));
#124083=CARTESIAN_POINT('Ctrl Pts',(50.0161522238616,-52.4207124612608,
0.));
#124084=CARTESIAN_POINT('Ctrl Pts',(50.0065636229938,-52.3978116592509,
0.));
#124085=CARTESIAN_POINT('Ctrl Pts',(49.9969687627408,-52.3749574789871,
0.));
#124086=CARTESIAN_POINT('Ctrl Pts',(49.9873677385775,-52.3521500002718,
0.));
#124087=CARTESIAN_POINT('Ctrl Pts',(49.9777606464106,-52.3293893031528,
0.));
#124088=CARTESIAN_POINT('Ctrl Pts',(49.9681475825824,-52.3066754679265,
0.));
#124089=CARTESIAN_POINT('Ctrl Pts',(49.9585286438733,-52.2840085751384,
0.));
#124090=CARTESIAN_POINT('Ctrl Pts',(49.9489039275064,-52.2613887055773,
0.));
#124091=CARTESIAN_POINT('Ctrl Pts',(49.9392735311509,-52.2388159402771,
0.));
#124092=CARTESIAN_POINT('Ctrl Pts',(49.9296375529245,-52.2162903605275,
0.));
#124093=CARTESIAN_POINT('Ctrl Pts',(49.9199960913962,-52.1938120478754,
0.));
#124094=CARTESIAN_POINT('Ctrl Pts',(49.9103492455902,-52.1713810841276,
0.));
#124095=CARTESIAN_POINT('Ctrl Pts',(49.9006971149894,-52.1489975513445,
0.));
#124096=CARTESIAN_POINT('Ctrl Pts',(49.8910397995397,-52.1266615318407,
0.));
#124097=CARTESIAN_POINT('Ctrl Pts',(49.8813773996517,-52.1043731081962,
0.));
#124098=CARTESIAN_POINT('Ctrl Pts',(49.8717100162048,-52.0821323632587,
0.));
#124099=CARTESIAN_POINT('Ctrl Pts',(49.86203775055,-52.0599393801452,0.));
#124100=CARTESIAN_POINT('Ctrl Pts',(49.8523607045149,-52.0377942422376,
0.));
#124101=CARTESIAN_POINT('Ctrl Pts',(49.8426789804071,-52.0156970331823,
0.));
#124102=CARTESIAN_POINT('Ctrl Pts',(49.8329926810171,-51.9936478369008,
0.));
#124103=CARTESIAN_POINT('Ctrl Pts',(49.8233019096222,-51.9716467375937,
0.));
#124104=CARTESIAN_POINT('Ctrl Pts',(49.8136067699896,-51.9496938197418,
0.));
#124105=CARTESIAN_POINT('Ctrl Pts',(49.8039073663812,-51.9277891681018,
0.));
#124106=CARTESIAN_POINT('Ctrl Pts',(49.7942038035576,-51.9059328677059,
0.));
#124107=CARTESIAN_POINT('Ctrl Pts',(49.7844961867807,-51.8841250038724,
0.));
#124108=CARTESIAN_POINT('Ctrl Pts',(49.7747846218182,-51.8623656622097,
0.));
#124109=CARTESIAN_POINT('Ctrl Pts',(49.7650692149462,-51.8406549286175,
0.));
#124110=CARTESIAN_POINT('Ctrl Pts',(49.755350072955,-51.8189928892828,0.));
#124111=CARTESIAN_POINT('Ctrl Pts',(49.7456273031534,-51.7973796306803,
0.));
#124112=CARTESIAN_POINT('Ctrl Pts',(49.7359010133721,-51.7758152395836,
0.));
#124113=CARTESIAN_POINT('Ctrl Pts',(49.7261713119663,-51.754299803067,0.));
#124114=CARTESIAN_POINT('Ctrl Pts',(49.7164383078212,-51.7328334085091,
0.));
#124115=CARTESIAN_POINT('Ctrl Pts',(49.7067021103553,-51.7114161435869,
0.));
#124116=CARTESIAN_POINT('Ctrl Pts',(49.6969628295262,-51.6900480962773,
0.));
#124117=CARTESIAN_POINT('Ctrl Pts',(49.6872205758336,-51.6687293548682,
0.));
#124118=CARTESIAN_POINT('Ctrl Pts',(49.6774754603245,-51.6474600079622,
0.));
#124119=CARTESIAN_POINT('Ctrl Pts',(49.6677275945967,-51.6262401444791,
0.));
#124120=CARTESIAN_POINT('Ctrl Pts',(49.6579770908037,-51.6050698536496,
0.));
#124121=CARTESIAN_POINT('Ctrl Pts',(49.6482240616593,-51.5839492250181,
0.));
#124122=CARTESIAN_POINT('Ctrl Pts',(49.6384686204413,-51.5628783484525,
0.));
#124123=CARTESIAN_POINT('Ctrl Pts',(49.6287108809965,-51.5418573141484,
0.));
#124124=CARTESIAN_POINT('Ctrl Pts',(49.6189509577452,-51.5208862126315,
0.));
#124125=CARTESIAN_POINT('Ctrl Pts',(49.6091889656866,-51.4999651347523,
0.));
#124126=CARTESIAN_POINT('Ctrl Pts',(49.5994250204031,-51.4790941716888,
0.));
#124127=CARTESIAN_POINT('Ctrl Pts',(49.5896592380654,-51.4582734149583,
0.));
#124128=CARTESIAN_POINT('Ctrl Pts',(49.5798917354365,-51.4375029564197,
0.));
#124129=CARTESIAN_POINT('Ctrl Pts',(49.5701226298769,-51.4167828882756,
0.));
#124130=CARTESIAN_POINT('Ctrl Pts',(49.5603520393496,-51.396113303067,0.));
#124131=CARTESIAN_POINT('Ctrl Pts',(49.550580082425,-51.3754942936778,0.));
#124132=CARTESIAN_POINT('Ctrl Pts',(49.5408068782859,-51.3549259533458,
0.));
#124133=CARTESIAN_POINT('Ctrl Pts',(49.5310325467332,-51.3344083756657,
0.));
#124134=CARTESIAN_POINT('Ctrl Pts',(49.5212572081908,-51.313941654591,0.));
#124135=CARTESIAN_POINT('Ctrl Pts',(49.5114809837122,-51.2935258844289,
0.));
#124136=CARTESIAN_POINT('Ctrl Pts',(49.5017039949852,-51.2731611598475,
0.));
#124137=CARTESIAN_POINT('Ctrl Pts',(49.4919263643362,-51.2528475758846,
0.));
#124138=CARTESIAN_POINT('Ctrl Pts',(49.4821482147356,-51.2325852279506,
0.));
#124139=CARTESIAN_POINT('Ctrl Pts',(49.4723696698021,-51.2123742118287,
0.));
#124140=CARTESIAN_POINT('Ctrl Pts',(49.4625908538074,-51.1922146236686,
0.));
#124141=CARTESIAN_POINT('Ctrl Pts',(49.4528118916832,-51.1721065599973,
0.));
#124142=CARTESIAN_POINT('Ctrl Pts',(49.4430329090287,-51.1520501177291,
0.));
#124143=CARTESIAN_POINT('Ctrl Pts',(49.4332540321178,-51.1320453941702,
0.));
#124144=CARTESIAN_POINT('Ctrl Pts',(49.423475387907,-51.1120924870195,0.));
#124145=CARTESIAN_POINT('Ctrl Pts',(49.4136971040428,-51.0921914943662,
0.));
#124146=CARTESIAN_POINT('Ctrl Pts',(49.4039193088634,-51.0723425146985,
0.));
#124147=CARTESIAN_POINT('Ctrl Pts',(49.3941421314012,-51.052545646907,0.));
#124148=CARTESIAN_POINT('Ctrl Pts',(49.3843657013852,-51.0328009902858,
0.));
#124149=CARTESIAN_POINT('Ctrl Pts',(49.3745901492432,-51.0131086445272,
0.));
#124150=CARTESIAN_POINT('Ctrl Pts',(49.3648156061058,-50.9934687097188,
0.));
#124151=CARTESIAN_POINT('Ctrl Pts',(49.355042203823,-50.9738812863646,0.));
#124152=CARTESIAN_POINT('Ctrl Pts',(49.345270074981,-50.9543464753981,0.));
#124153=CARTESIAN_POINT('Ctrl Pts',(49.3354993529158,-50.9348643781924,
0.));
#124154=CARTESIAN_POINT('Ctrl Pts',(49.3257301717335,-50.9154350965666,
0.));
#124155=CARTESIAN_POINT('Ctrl Pts',(49.3159626663109,-50.8960587327848,
0.));
#124156=CARTESIAN_POINT('Ctrl Pts',(49.3061969722781,-50.8767353895492,
0.));
#124157=CARTESIAN_POINT('Ctrl Pts',(49.2964332260039,-50.8574651699873,
0.));
#124158=CARTESIAN_POINT('Ctrl Pts',(49.2866715645838,-50.8382481776403,
0.));
#124159=CARTESIAN_POINT('Ctrl Pts',(49.2769121258164,-50.819084516434,0.));
#124160=CARTESIAN_POINT('Ctrl Pts',(49.2671550482435,-50.7999742907131,
0.));
#124161=CARTESIAN_POINT('Ctrl Pts',(49.2574004712134,-50.7809176052966,
0.));
#124162=CARTESIAN_POINT('Ctrl Pts',(49.2476485349373,-50.7619145655207,
0.));
#124163=CARTESIAN_POINT('Ctrl Pts',(49.2378993805471,-50.7429652772805,
0.));
#124164=CARTESIAN_POINT('Ctrl Pts',(49.228153150155,-50.7240698470679,0.));
#124165=CARTESIAN_POINT('Ctrl Pts',(49.2184099867461,-50.7052283818922,
0.));
#124166=CARTESIAN_POINT('Ctrl Pts',(49.2086700340614,-50.6864409891895,
0.));
#124167=CARTESIAN_POINT('Ctrl Pts',(49.1989334364995,-50.6677077767432,
0.));
#124168=CARTESIAN_POINT('Ctrl Pts',(49.189200338976,-50.6490288525656,0.));
#124169=CARTESIAN_POINT('Ctrl Pts',(49.1794708869099,-50.6304043248821,
0.));
#124170=CARTESIAN_POINT('Ctrl Pts',(49.1697452265494,-50.6118343023958,
0.));
#124171=CARTESIAN_POINT('Ctrl Pts',(49.1600235052621,-50.5933188945168,
0.));
#124172=CARTESIAN_POINT('Ctrl Pts',(49.1503058717821,-50.5748582115565,
0.));
#124173=CARTESIAN_POINT('Ctrl Pts',(49.1405924766144,-50.556452365038,0.));
#124174=CARTESIAN_POINT('Ctrl Pts',(49.1308834717615,-50.5381014674791,
0.));
#124175=CARTESIAN_POINT('Ctrl Pts',(49.1211790099795,-50.5198056318089,
0.));
#124176=CARTESIAN_POINT('Ctrl Pts',(49.1114792441571,-50.501564970874,0.));
#124177=CARTESIAN_POINT('Ctrl Pts',(49.1017843266803,-50.4833795969318,
0.));
#124178=CARTESIAN_POINT('Ctrl Pts',(49.0920944087008,-50.4652496210607,
0.));
#124179=CARTESIAN_POINT('Ctrl Pts',(49.0824096415371,-50.4471751542751,
0.));
#124180=CARTESIAN_POINT('Ctrl Pts',(49.0727301783494,-50.4291563088547,
0.));
#124181=CARTESIAN_POINT('Ctrl Pts',(49.0630561755075,-50.4111931994257,
0.));
#124182=CARTESIAN_POINT('Ctrl Pts',(49.0533877945744,-50.3932859445252,
0.));
#124183=CARTESIAN_POINT('Ctrl Pts',(49.0437252024832,-50.3754346667353,
0.));
#124184=CARTESIAN_POINT('Ctrl Pts',(49.0340685673982,-50.3576394894108,
0.));
#124185=CARTESIAN_POINT('Ctrl Pts',(49.024418055075,-50.3399005337958,0.));
#124186=CARTESIAN_POINT('Ctrl Pts',(49.0147738256942,-50.3222179165119,
0.));
#124187=CARTESIAN_POINT('Ctrl Pts',(49.0051360288044,-50.3045917455424,
0.));
#124188=CARTESIAN_POINT('Ctrl Pts',(48.9955048082081,-50.2870221241054,
0.));
#124189=CARTESIAN_POINT('Ctrl Pts',(48.9858803116689,-50.2695091583511,
0.));
#124190=CARTESIAN_POINT('Ctrl Pts',(48.9762626987227,-50.252052963548,0.));
#124191=CARTESIAN_POINT('Ctrl Pts',(48.9666521500911,-50.234653671541,0.));
#124192=CARTESIAN_POINT('Ctrl Pts',(48.9570488741167,-50.2173114358325,
0.));
#124193=CARTESIAN_POINT('Ctrl Pts',(48.9474530868733,-50.2000264157797,
0.));
#124194=CARTESIAN_POINT('Ctrl Pts',(48.9378649933055,-50.1827987615602,
0.));
#124195=CARTESIAN_POINT('Ctrl Pts',(48.9282847698294,-50.1656286003997,
0.));
#124196=CARTESIAN_POINT('Ctrl Pts',(48.9187125418099,-50.1485160184657,
0.));
#124197=CARTESIAN_POINT('Ctrl Pts',(48.90914838181,-50.1314610602569,0.));
#124198=CARTESIAN_POINT('Ctrl Pts',(48.9015035372055,-50.1178632067084,
0.));
#124199=CARTESIAN_POINT('Ctrl Pts',(48.895773555686,-50.1076907555471,0.));
#124200=CARTESIAN_POINT('Ctrl Pts',(48.8919551910366,-50.1009206494272,
0.));
#124201=CARTESIAN_POINT('Ctrl Pts',(48.8900464144686,-50.0975384783635,
0.));
#124202=CARTESIAN_POINT('Ctrl Pts',(45.8467972562798,-58.722407829904,0.));
#124203=CARTESIAN_POINT('Ctrl Pts',(45.8467972562798,-58.722407829904,12.));
#124204=CARTESIAN_POINT('Ctrl Pts',(45.8455162977427,-58.7169606500268,
0.));
#124205=CARTESIAN_POINT('Ctrl Pts',(45.8455162977427,-58.7169606500268,
12.));
#124206=CARTESIAN_POINT('Ctrl Pts',(45.8429527488786,-58.7060702401686,
0.));
#124207=CARTESIAN_POINT('Ctrl Pts',(45.8429527488786,-58.7060702401686,
12.));
#124208=CARTESIAN_POINT('Ctrl Pts',(45.8391025302132,-58.6897464750699,
0.));
#124209=CARTESIAN_POINT('Ctrl Pts',(45.8391025302132,-58.6897464750699,
12.));
#124210=CARTESIAN_POINT('Ctrl Pts',(45.8339591141834,-58.6680051552762,
0.));
#124211=CARTESIAN_POINT('Ctrl Pts',(45.8339591141834,-58.6680051552762,
12.));
#124212=CARTESIAN_POINT('Ctrl Pts',(45.827513526425,-58.6408680154016,0.));
#124213=CARTESIAN_POINT('Ctrl Pts',(45.827513526425,-58.6408680154016,12.));
#124214=CARTESIAN_POINT('Ctrl Pts',(45.8210516273781,-58.6137704035871,
0.));
#124215=CARTESIAN_POINT('Ctrl Pts',(45.8210516273781,-58.6137704035871,
12.));
#124216=CARTESIAN_POINT('Ctrl Pts',(45.814573433072,-58.5867123491018,0.));
#124217=CARTESIAN_POINT('Ctrl Pts',(45.814573433072,-58.5867123491018,12.));
#124218=CARTESIAN_POINT('Ctrl Pts',(45.8080789725084,-58.5596938940195,
0.));
#124219=CARTESIAN_POINT('Ctrl Pts',(45.8080789725084,-58.5596938940195,
12.));
#124220=CARTESIAN_POINT('Ctrl Pts',(45.8015682926025,-58.5327150960661,
0.));
#124221=CARTESIAN_POINT('Ctrl Pts',(45.8015682926025,-58.5327150960661,
12.));
#124222=CARTESIAN_POINT('Ctrl Pts',(45.7950414569268,-58.5057760270184,
0.));
#124223=CARTESIAN_POINT('Ctrl Pts',(45.7950414569268,-58.5057760270184,
12.));
#124224=CARTESIAN_POINT('Ctrl Pts',(45.7884985397018,-58.4788767676949,
0.));
#124225=CARTESIAN_POINT('Ctrl Pts',(45.7884985397018,-58.4788767676949,
12.));
#124226=CARTESIAN_POINT('Ctrl Pts',(45.7819396211009,-58.4520174038764,
0.));
#124227=CARTESIAN_POINT('Ctrl Pts',(45.7819396211009,-58.4520174038764,
12.));
#124228=CARTESIAN_POINT('Ctrl Pts',(45.7753647821513,-58.425198021955,0.));
#124229=CARTESIAN_POINT('Ctrl Pts',(45.7753647821513,-58.425198021955,12.));
#124230=CARTESIAN_POINT('Ctrl Pts',(45.7687740994957,-58.3984187044245,
0.));
#124231=CARTESIAN_POINT('Ctrl Pts',(45.7687740994957,-58.3984187044245,
12.));
#124232=CARTESIAN_POINT('Ctrl Pts',(45.7621676411434,-58.3716795262353,
0.));
#124233=CARTESIAN_POINT('Ctrl Pts',(45.7621676411434,-58.3716795262353,
12.));
#124234=CARTESIAN_POINT('Ctrl Pts',(45.755545469402,-58.3449805573423,0.));
#124235=CARTESIAN_POINT('Ctrl Pts',(45.755545469402,-58.3449805573423,12.));
#124236=CARTESIAN_POINT('Ctrl Pts',(45.7489076429763,-58.3183218645316,
0.));
#124237=CARTESIAN_POINT('Ctrl Pts',(45.7489076429763,-58.3183218645316,
12.));
#124238=CARTESIAN_POINT('Ctrl Pts',(45.742254219463,-58.291703513584,0.));
#124239=CARTESIAN_POINT('Ctrl Pts',(45.742254219463,-58.291703513584,12.));
#124240=CARTESIAN_POINT('Ctrl Pts',(45.7355852575107,-58.2651255711453,
0.));
#124241=CARTESIAN_POINT('Ctrl Pts',(45.7355852575107,-58.2651255711453,
12.));
#124242=CARTESIAN_POINT('Ctrl Pts',(45.7289008195579,-58.2385881070913,
0.));
#124243=CARTESIAN_POINT('Ctrl Pts',(45.7289008195579,-58.2385881070913,
12.));
#124244=CARTESIAN_POINT('Ctrl Pts',(45.7222009715397,-58.2120911942772,
0.));
#124245=CARTESIAN_POINT('Ctrl Pts',(45.7222009715397,-58.2120911942772,
12.));
#124246=CARTESIAN_POINT('Ctrl Pts',(45.7154857816483,-58.185634907469,0.));
#124247=CARTESIAN_POINT('Ctrl Pts',(45.7154857816483,-58.185634907469,12.));
#124248=CARTESIAN_POINT('Ctrl Pts',(45.7087553193771,-58.1592193225137,
0.));
#124249=CARTESIAN_POINT('Ctrl Pts',(45.7087553193771,-58.1592193225137,
12.));
#124250=CARTESIAN_POINT('Ctrl Pts',(45.702009654518,-58.1328445154676,0.));
#124251=CARTESIAN_POINT('Ctrl Pts',(45.702009654518,-58.1328445154676,12.));
#124252=CARTESIAN_POINT('Ctrl Pts',(45.695248856015,-58.1065105615907,0.));
#124253=CARTESIAN_POINT('Ctrl Pts',(45.695248856015,-58.1065105615907,12.));
#124254=CARTESIAN_POINT('Ctrl Pts',(45.6884729914485,-58.0802175348966,
0.));
#124255=CARTESIAN_POINT('Ctrl Pts',(45.6884729914485,-58.0802175348966,
12.));
#124256=CARTESIAN_POINT('Ctrl Pts',(45.6816821276678,-58.0539655087117,
0.));
#124257=CARTESIAN_POINT('Ctrl Pts',(45.6816821276678,-58.0539655087117,
12.));
#124258=CARTESIAN_POINT('Ctrl Pts',(45.6748763311643,-58.0277545560012,
0.));
#124259=CARTESIAN_POINT('Ctrl Pts',(45.6748763311643,-58.0277545560012,
12.));
#124260=CARTESIAN_POINT('Ctrl Pts',(45.6680556685493,-58.0015847497837,
0.));
#124261=CARTESIAN_POINT('Ctrl Pts',(45.6680556685493,-58.0015847497837,
12.));
#124262=CARTESIAN_POINT('Ctrl Pts',(45.661220206992,-57.9754561635061,0.));
#124263=CARTESIAN_POINT('Ctrl Pts',(45.661220206992,-57.9754561635061,12.));
#124264=CARTESIAN_POINT('Ctrl Pts',(45.6543700146679,-57.9493688714237,
0.));
#124265=CARTESIAN_POINT('Ctrl Pts',(45.6543700146679,-57.9493688714237,
12.));
#124266=CARTESIAN_POINT('Ctrl Pts',(45.6475051605535,-57.9233229484311,
0.));
#124267=CARTESIAN_POINT('Ctrl Pts',(45.6475051605535,-57.9233229484311,
12.));
#124268=CARTESIAN_POINT('Ctrl Pts',(45.6406257142382,-57.8973184699034,
0.));
#124269=CARTESIAN_POINT('Ctrl Pts',(45.6406257142382,-57.8973184699034,
12.));
#124270=CARTESIAN_POINT('Ctrl Pts',(45.6337317457252,-57.8713555115232,
0.));
#124271=CARTESIAN_POINT('Ctrl Pts',(45.6337317457252,-57.8713555115232,
12.));
#124272=CARTESIAN_POINT('Ctrl Pts',(45.6268233252544,-57.8454341491238,
0.));
#124273=CARTESIAN_POINT('Ctrl Pts',(45.6268233252544,-57.8454341491238,
12.));
#124274=CARTESIAN_POINT('Ctrl Pts',(45.6199005230784,-57.8195544584845,
0.));
#124275=CARTESIAN_POINT('Ctrl Pts',(45.6199005230784,-57.8195544584845,
12.));
#124276=CARTESIAN_POINT('Ctrl Pts',(45.6129634094683,-57.7937165153387,
0.));
#124277=CARTESIAN_POINT('Ctrl Pts',(45.6129634094683,-57.7937165153387,
12.));
#124278=CARTESIAN_POINT('Ctrl Pts',(45.6060120548205,-57.7679203954742,
0.));
#124279=CARTESIAN_POINT('Ctrl Pts',(45.6060120548205,-57.7679203954742,
12.));
#124280=CARTESIAN_POINT('Ctrl Pts',(45.5990465297344,-57.7421661748026,
0.));
#124281=CARTESIAN_POINT('Ctrl Pts',(45.5990465297344,-57.7421661748026,
12.));
#124282=CARTESIAN_POINT('Ctrl Pts',(45.5920669050986,-57.7164539294314,
0.));
#124283=CARTESIAN_POINT('Ctrl Pts',(45.5920669050986,-57.7164539294314,
12.));
#124284=CARTESIAN_POINT('Ctrl Pts',(45.5850732521896,-57.6907837357417,
0.));
#124285=CARTESIAN_POINT('Ctrl Pts',(45.5850732521896,-57.6907837357417,
12.));
#124286=CARTESIAN_POINT('Ctrl Pts',(45.5780656427163,-57.6651556704237,
0.));
#124287=CARTESIAN_POINT('Ctrl Pts',(45.5780656427163,-57.6651556704237,
12.));
#124288=CARTESIAN_POINT('Ctrl Pts',(45.5710441487674,-57.6395698104404,
0.));
#124289=CARTESIAN_POINT('Ctrl Pts',(45.5710441487674,-57.6395698104404,
12.));
#124290=CARTESIAN_POINT('Ctrl Pts',(45.5640088427813,-57.614026233004,0.));
#124291=CARTESIAN_POINT('Ctrl Pts',(45.5640088427813,-57.614026233004,12.));
#124292=CARTESIAN_POINT('Ctrl Pts',(45.5569597975096,-57.5885250155433,
0.));
#124293=CARTESIAN_POINT('Ctrl Pts',(45.5569597975096,-57.5885250155433,
12.));
#124294=CARTESIAN_POINT('Ctrl Pts',(45.5498970859835,-57.563066235668,0.));
#124295=CARTESIAN_POINT('Ctrl Pts',(45.5498970859835,-57.563066235668,12.));
#124296=CARTESIAN_POINT('Ctrl Pts',(45.542820781484,-57.537649971135,0.));
#124297=CARTESIAN_POINT('Ctrl Pts',(45.542820781484,-57.537649971135,12.));
#124298=CARTESIAN_POINT('Ctrl Pts',(45.5357309575611,-57.5122762998745,
0.));
#124299=CARTESIAN_POINT('Ctrl Pts',(45.5357309575611,-57.5122762998745,
12.));
#124300=CARTESIAN_POINT('Ctrl Pts',(45.5286276880485,-57.4869453000063,
0.));
#124301=CARTESIAN_POINT('Ctrl Pts',(45.5286276880485,-57.4869453000063,
12.));
#124302=CARTESIAN_POINT('Ctrl Pts',(45.5215110470825,-57.4616570498568,
0.));
#124303=CARTESIAN_POINT('Ctrl Pts',(45.5215110470825,-57.4616570498568,
12.));
#124304=CARTESIAN_POINT('Ctrl Pts',(45.5143811091205,-57.4364116279702,
0.));
#124305=CARTESIAN_POINT('Ctrl Pts',(45.5143811091205,-57.4364116279702,
12.));
#124306=CARTESIAN_POINT('Ctrl Pts',(45.5072379489631,-57.4112091131183,
0.));
#124307=CARTESIAN_POINT('Ctrl Pts',(45.5072379489631,-57.4112091131183,
12.));
#124308=CARTESIAN_POINT('Ctrl Pts',(45.500081641751,-57.3860495843033,0.));
#124309=CARTESIAN_POINT('Ctrl Pts',(45.500081641751,-57.3860495843033,12.));
#124310=CARTESIAN_POINT('Ctrl Pts',(45.4929122629572,-57.3609331207574,
0.));
#124311=CARTESIAN_POINT('Ctrl Pts',(45.4929122629572,-57.3609331207574,
12.));
#124312=CARTESIAN_POINT('Ctrl Pts',(45.4857298883824,-57.3358598019389,
0.));
#124313=CARTESIAN_POINT('Ctrl Pts',(45.4857298883824,-57.3358598019389,
12.));
#124314=CARTESIAN_POINT('Ctrl Pts',(45.4785345941507,-57.3108297075265,
0.));
#124315=CARTESIAN_POINT('Ctrl Pts',(45.4785345941507,-57.3108297075265,
12.));
#124316=CARTESIAN_POINT('Ctrl Pts',(45.4713264567063,-57.2858429174062,
0.));
#124317=CARTESIAN_POINT('Ctrl Pts',(45.4713264567063,-57.2858429174062,
12.));
#124318=CARTESIAN_POINT('Ctrl Pts',(45.4641055528141,-57.2608995116733,
0.));
#124319=CARTESIAN_POINT('Ctrl Pts',(45.4641055528141,-57.2608995116733,
12.));
#124320=CARTESIAN_POINT('Ctrl Pts',(45.4568719595642,-57.2359995706447,
0.));
#124321=CARTESIAN_POINT('Ctrl Pts',(45.4568719595642,-57.2359995706447,
12.));
#124322=CARTESIAN_POINT('Ctrl Pts',(45.4496257543759,-57.2111431748631,
0.));
#124323=CARTESIAN_POINT('Ctrl Pts',(45.4496257543759,-57.2111431748631,
12.));
#124324=CARTESIAN_POINT('Ctrl Pts',(45.4423670150034,-57.186330405101,0.));
#124325=CARTESIAN_POINT('Ctrl Pts',(45.4423670150034,-57.186330405101,12.));
#124326=CARTESIAN_POINT('Ctrl Pts',(45.4350958195434,-57.1615613423584,
0.));
#124327=CARTESIAN_POINT('Ctrl Pts',(45.4350958195434,-57.1615613423584,
12.));
#124328=CARTESIAN_POINT('Ctrl Pts',(45.4278122464389,-57.136836067863,0.));
#124329=CARTESIAN_POINT('Ctrl Pts',(45.4278122464389,-57.136836067863,12.));
#124330=CARTESIAN_POINT('Ctrl Pts',(45.4205163744782,-57.112154663078,0.));
#124331=CARTESIAN_POINT('Ctrl Pts',(45.4205163744782,-57.112154663078,12.));
#124332=CARTESIAN_POINT('Ctrl Pts',(45.4132082827948,-57.0875172097051,
0.));
#124333=CARTESIAN_POINT('Ctrl Pts',(45.4132082827948,-57.0875172097051,
12.));
#124334=CARTESIAN_POINT('Ctrl Pts',(45.4058880508693,-57.0629237896848,
0.));
#124335=CARTESIAN_POINT('Ctrl Pts',(45.4058880508693,-57.0629237896848,
12.));
#124336=CARTESIAN_POINT('Ctrl Pts',(45.3985557585311,-57.0383744851913,
0.));
#124337=CARTESIAN_POINT('Ctrl Pts',(45.3985557585311,-57.0383744851913,
12.));
#124338=CARTESIAN_POINT('Ctrl Pts',(45.3912114859616,-57.0138693786278,
0.));
#124339=CARTESIAN_POINT('Ctrl Pts',(45.3912114859616,-57.0138693786278,
12.));
#124340=CARTESIAN_POINT('Ctrl Pts',(45.3838553136948,-56.9894085526373,
0.));
#124341=CARTESIAN_POINT('Ctrl Pts',(45.3838553136948,-56.9894085526373,
12.));
#124342=CARTESIAN_POINT('Ctrl Pts',(45.3764873226196,-56.9649920901073,
0.));
#124343=CARTESIAN_POINT('Ctrl Pts',(45.3764873226196,-56.9649920901073,
12.));
#124344=CARTESIAN_POINT('Ctrl Pts',(45.3691075939827,-56.9406200741714,
0.));
#124345=CARTESIAN_POINT('Ctrl Pts',(45.3691075939827,-56.9406200741714,
12.));
#124346=CARTESIAN_POINT('Ctrl Pts',(45.3617162093923,-56.9162925882085,
0.));
#124347=CARTESIAN_POINT('Ctrl Pts',(45.3617162093923,-56.9162925882085,
12.));
#124348=CARTESIAN_POINT('Ctrl Pts',(45.3543132508239,-56.8920097158377,
0.));
#124349=CARTESIAN_POINT('Ctrl Pts',(45.3543132508239,-56.8920097158377,
12.));
#124350=CARTESIAN_POINT('Ctrl Pts',(45.3468988006203,-56.8677715409268,
0.));
#124351=CARTESIAN_POINT('Ctrl Pts',(45.3468988006203,-56.8677715409268,
12.));
#124352=CARTESIAN_POINT('Ctrl Pts',(45.3394729414931,-56.8435781475981,
0.));
#124353=CARTESIAN_POINT('Ctrl Pts',(45.3394729414931,-56.8435781475981,
12.));
#124354=CARTESIAN_POINT('Ctrl Pts',(45.332035756524,-56.8194296202291,0.));
#124355=CARTESIAN_POINT('Ctrl Pts',(45.332035756524,-56.8194296202291,12.));
#124356=CARTESIAN_POINT('Ctrl Pts',(45.3245873291684,-56.7953260434524,
0.));
#124357=CARTESIAN_POINT('Ctrl Pts',(45.3245873291684,-56.7953260434524,
12.));
#124358=CARTESIAN_POINT('Ctrl Pts',(45.31712774326,-56.7712675021491,0.));
#124359=CARTESIAN_POINT('Ctrl Pts',(45.31712774326,-56.7712675021491,12.));
#124360=CARTESIAN_POINT('Ctrl Pts',(45.3096570830118,-56.7472540814553,
0.));
#124361=CARTESIAN_POINT('Ctrl Pts',(45.3096570830118,-56.7472540814553,
12.));
#124362=CARTESIAN_POINT('Ctrl Pts',(45.3021754330179,-56.7232858667709,
0.));
#124363=CARTESIAN_POINT('Ctrl Pts',(45.3021754330179,-56.7232858667709,
12.));
#124364=CARTESIAN_POINT('Ctrl Pts',(45.2946828782559,-56.69936294376,0.));
#124365=CARTESIAN_POINT('Ctrl Pts',(45.2946828782559,-56.69936294376,12.));
#124366=CARTESIAN_POINT('Ctrl Pts',(45.2871795040906,-56.6754853983528,
0.));
#124367=CARTESIAN_POINT('Ctrl Pts',(45.2871795040906,-56.6754853983528,
12.));
#124368=CARTESIAN_POINT('Ctrl Pts',(45.2796653962785,-56.6516533167384,
0.));
#124369=CARTESIAN_POINT('Ctrl Pts',(45.2796653962785,-56.6516533167384,
12.));
#124370=CARTESIAN_POINT('Ctrl Pts',(45.2721406409695,-56.6278667853702,
0.));
#124371=CARTESIAN_POINT('Ctrl Pts',(45.2721406409695,-56.6278667853702,
12.));
#124372=CARTESIAN_POINT('Ctrl Pts',(45.2646053247087,-56.6041258909741,
0.));
#124373=CARTESIAN_POINT('Ctrl Pts',(45.2646053247087,-56.6041258909741,
12.));
#124374=CARTESIAN_POINT('Ctrl Pts',(45.257059534438,-56.5804307205505,0.));
#124375=CARTESIAN_POINT('Ctrl Pts',(45.257059534438,-56.5804307205505,12.));
#124376=CARTESIAN_POINT('Ctrl Pts',(45.2495033575,-56.5567813613756,0.));
#124377=CARTESIAN_POINT('Ctrl Pts',(45.2495033575,-56.5567813613756,12.));
#124378=CARTESIAN_POINT('Ctrl Pts',(45.2419368816429,-56.5331779009958,
0.));
#124379=CARTESIAN_POINT('Ctrl Pts',(45.2419368816429,-56.5331779009958,
12.));
#124380=CARTESIAN_POINT('Ctrl Pts',(45.2343601950228,-56.5096204272306,
0.));
#124381=CARTESIAN_POINT('Ctrl Pts',(45.2343601950228,-56.5096204272306,
12.));
#124382=CARTESIAN_POINT('Ctrl Pts',(45.2267733862049,-56.4861090281823,
0.));
#124383=CARTESIAN_POINT('Ctrl Pts',(45.2267733862049,-56.4861090281823,
12.));
#124384=CARTESIAN_POINT('Ctrl Pts',(45.2191765441667,-56.4626437922386,
0.));
#124385=CARTESIAN_POINT('Ctrl Pts',(45.2191765441667,-56.4626437922386,
12.));
#124386=CARTESIAN_POINT('Ctrl Pts',(45.2115697583001,-56.4392248080732,
0.));
#124387=CARTESIAN_POINT('Ctrl Pts',(45.2115697583001,-56.4392248080732,
12.));
#124388=CARTESIAN_POINT('Ctrl Pts',(45.2039531184172,-56.4158521646411,
0.));
#124389=CARTESIAN_POINT('Ctrl Pts',(45.2039531184172,-56.4158521646411,
12.));
#124390=CARTESIAN_POINT('Ctrl Pts',(45.1963267147529,-56.3925259511806,
0.));
#124391=CARTESIAN_POINT('Ctrl Pts',(45.1963267147529,-56.3925259511806,
12.));
#124392=CARTESIAN_POINT('Ctrl Pts',(45.1886906379667,-56.3692462572231,
0.));
#124393=CARTESIAN_POINT('Ctrl Pts',(45.1886906379667,-56.3692462572231,
12.));
#124394=CARTESIAN_POINT('Ctrl Pts',(45.1810449791453,-56.3460131725964,
0.));
#124395=CARTESIAN_POINT('Ctrl Pts',(45.1810449791453,-56.3460131725964,
12.));
#124396=CARTESIAN_POINT('Ctrl Pts',(45.1733898298061,-56.3228267874264,
0.));
#124397=CARTESIAN_POINT('Ctrl Pts',(45.1733898298061,-56.3228267874264,
12.));
#124398=CARTESIAN_POINT('Ctrl Pts',(45.1657252819013,-56.2996871921316,
0.));
#124399=CARTESIAN_POINT('Ctrl Pts',(45.1657252819013,-56.2996871921316,
12.));
#124400=CARTESIAN_POINT('Ctrl Pts',(45.1580514278223,-56.2765944774245,
0.));
#124401=CARTESIAN_POINT('Ctrl Pts',(45.1580514278223,-56.2765944774245,
12.));
#124402=CARTESIAN_POINT('Ctrl Pts',(45.1503683604005,-56.2535487343221,
0.));
#124403=CARTESIAN_POINT('Ctrl Pts',(45.1503683604005,-56.2535487343221,
12.));
#124404=CARTESIAN_POINT('Ctrl Pts',(45.1426761729105,-56.2305500541489,
0.));
#124405=CARTESIAN_POINT('Ctrl Pts',(45.1426761729105,-56.2305500541489,
12.));
#124406=CARTESIAN_POINT('Ctrl Pts',(45.1349749590738,-56.2075985285393,
0.));
#124407=CARTESIAN_POINT('Ctrl Pts',(45.1349749590738,-56.2075985285393,
12.));
#124408=CARTESIAN_POINT('Ctrl Pts',(45.127264813063,-56.1846942494325,0.));
#124409=CARTESIAN_POINT('Ctrl Pts',(45.127264813063,-56.1846942494325,12.));
#124410=CARTESIAN_POINT('Ctrl Pts',(45.1195458295063,-56.1618373090732,
0.));
#124411=CARTESIAN_POINT('Ctrl Pts',(45.1195458295063,-56.1618373090732,
12.));
#124412=CARTESIAN_POINT('Ctrl Pts',(45.1118181034888,-56.1390278000226,
0.));
#124413=CARTESIAN_POINT('Ctrl Pts',(45.1118181034888,-56.1390278000226,
12.));
#124414=CARTESIAN_POINT('Ctrl Pts',(45.1040817305561,-56.116265815162,0.));
#124415=CARTESIAN_POINT('Ctrl Pts',(45.1040817305561,-56.116265815162,12.));
#124416=CARTESIAN_POINT('Ctrl Pts',(45.0963368067177,-56.0935514476945,
0.));
#124417=CARTESIAN_POINT('Ctrl Pts',(45.0963368067177,-56.0935514476945,
12.));
#124418=CARTESIAN_POINT('Ctrl Pts',(45.0885834284517,-56.0708847911416,
0.));
#124419=CARTESIAN_POINT('Ctrl Pts',(45.0885834284517,-56.0708847911416,
12.));
#124420=CARTESIAN_POINT('Ctrl Pts',(45.0808216927089,-56.048265939342,0.));
#124421=CARTESIAN_POINT('Ctrl Pts',(45.0808216927089,-56.048265939342,12.));
#124422=CARTESIAN_POINT('Ctrl Pts',(45.0730516969149,-56.0256949864639,
0.));
#124423=CARTESIAN_POINT('Ctrl Pts',(45.0730516969149,-56.0256949864639,
12.));
#124424=CARTESIAN_POINT('Ctrl Pts',(45.0652735389733,-56.003172027008,0.));
#124425=CARTESIAN_POINT('Ctrl Pts',(45.0652735389733,-56.003172027008,12.));
#124426=CARTESIAN_POINT('Ctrl Pts',(45.0574873172695,-55.9806971558097,
0.));
#124427=CARTESIAN_POINT('Ctrl Pts',(45.0574873172695,-55.9806971558097,
12.));
#124428=CARTESIAN_POINT('Ctrl Pts',(45.0496931306755,-55.9582704680356,
0.));
#124429=CARTESIAN_POINT('Ctrl Pts',(45.0496931306755,-55.9582704680356,
12.));
#124430=CARTESIAN_POINT('Ctrl Pts',(45.0418910785551,-55.9358920591837,
0.));
#124431=CARTESIAN_POINT('Ctrl Pts',(45.0418910785551,-55.9358920591837,
12.));
#124432=CARTESIAN_POINT('Ctrl Pts',(45.0340812607657,-55.9135620250954,
0.));
#124433=CARTESIAN_POINT('Ctrl Pts',(45.0340812607657,-55.9135620250954,
12.));
#124434=CARTESIAN_POINT('Ctrl Pts',(45.0262637776615,-55.8912804619577,
0.));
#124435=CARTESIAN_POINT('Ctrl Pts',(45.0262637776615,-55.8912804619577,
12.));
#124436=CARTESIAN_POINT('Ctrl Pts',(45.0184387300973,-55.8690474663065,
0.));
#124437=CARTESIAN_POINT('Ctrl Pts',(45.0184387300973,-55.8690474663065,
12.));
#124438=CARTESIAN_POINT('Ctrl Pts',(45.0106062194342,-55.8468631350218,
0.));
#124439=CARTESIAN_POINT('Ctrl Pts',(45.0106062194342,-55.8468631350218,
12.));
#124440=CARTESIAN_POINT('Ctrl Pts',(45.0027663475433,-55.8247275653289,
0.));
#124441=CARTESIAN_POINT('Ctrl Pts',(45.0027663475433,-55.8247275653289,
12.));
#124442=CARTESIAN_POINT('Ctrl Pts',(44.9949192168093,-55.8026408548105,
0.));
#124443=CARTESIAN_POINT('Ctrl Pts',(44.9949192168093,-55.8026408548105,
12.));
#124444=CARTESIAN_POINT('Ctrl Pts',(44.9870649301342,-55.7806031014106,
0.));
#124445=CARTESIAN_POINT('Ctrl Pts',(44.9870649301342,-55.7806031014106,
12.));
#124446=CARTESIAN_POINT('Ctrl Pts',(44.9792035909413,-55.7586144034367,
0.));
#124447=CARTESIAN_POINT('Ctrl Pts',(44.9792035909413,-55.7586144034367,
12.));
#124448=CARTESIAN_POINT('Ctrl Pts',(44.9713353031804,-55.7366748595551,
0.));
#124449=CARTESIAN_POINT('Ctrl Pts',(44.9713353031804,-55.7366748595551,
12.));
#124450=CARTESIAN_POINT('Ctrl Pts',(44.9634601713321,-55.714784568793,0.));
#124451=CARTESIAN_POINT('Ctrl Pts',(44.9634601713321,-55.714784568793,12.));
#124452=CARTESIAN_POINT('Ctrl Pts',(44.9555783004106,-55.6929436305489,
0.));
#124453=CARTESIAN_POINT('Ctrl Pts',(44.9555783004106,-55.6929436305489,
12.));
#124454=CARTESIAN_POINT('Ctrl Pts',(44.9476897959685,-55.6711521445979,
0.));
#124455=CARTESIAN_POINT('Ctrl Pts',(44.9476897959685,-55.6711521445979,
12.));
#124456=CARTESIAN_POINT('Ctrl Pts',(44.9397947641007,-55.6494102110935,
0.));
#124457=CARTESIAN_POINT('Ctrl Pts',(44.9397947641007,-55.6494102110935,
12.));
#124458=CARTESIAN_POINT('Ctrl Pts',(44.9318933114507,-55.6277179305633,
0.));
#124459=CARTESIAN_POINT('Ctrl Pts',(44.9318933114507,-55.6277179305633,
12.));
#124460=CARTESIAN_POINT('Ctrl Pts',(44.9239855452144,-55.6060754039121,
0.));
#124461=CARTESIAN_POINT('Ctrl Pts',(44.9239855452144,-55.6060754039121,
12.));
#124462=CARTESIAN_POINT('Ctrl Pts',(44.9160715731443,-55.5844827324338,
0.));
#124463=CARTESIAN_POINT('Ctrl Pts',(44.9160715731443,-55.5844827324338,
12.));
#124464=CARTESIAN_POINT('Ctrl Pts',(44.908151503553,-55.5629400178142,0.));
#124465=CARTESIAN_POINT('Ctrl Pts',(44.908151503553,-55.5629400178142,12.));
#124466=CARTESIAN_POINT('Ctrl Pts',(44.9002254453183,-55.541447362134,0.));
#124467=CARTESIAN_POINT('Ctrl Pts',(44.9002254453183,-55.541447362134,12.));
#124468=CARTESIAN_POINT('Ctrl Pts',(44.8922935078889,-55.5200048678629,
0.));
#124469=CARTESIAN_POINT('Ctrl Pts',(44.8922935078889,-55.5200048678629,
12.));
#124470=CARTESIAN_POINT('Ctrl Pts',(44.8843558012886,-55.4986126378656,
0.));
#124471=CARTESIAN_POINT('Ctrl Pts',(44.8843558012886,-55.4986126378656,
12.));
#124472=CARTESIAN_POINT('Ctrl Pts',(44.8764124361207,-55.4772707754126,
0.));
#124473=CARTESIAN_POINT('Ctrl Pts',(44.8764124361207,-55.4772707754126,
12.));
#124474=CARTESIAN_POINT('Ctrl Pts',(44.8684635235725,-55.4559793841836,
0.));
#124475=CARTESIAN_POINT('Ctrl Pts',(44.8684635235725,-55.4559793841836,
12.));
#124476=CARTESIAN_POINT('Ctrl Pts',(44.8605091754214,-55.4347385682704,
0.));
#124477=CARTESIAN_POINT('Ctrl Pts',(44.8605091754214,-55.4347385682704,
12.));
#124478=CARTESIAN_POINT('Ctrl Pts',(44.8525495040408,-55.4135484321718,
0.));
#124479=CARTESIAN_POINT('Ctrl Pts',(44.8525495040408,-55.4135484321718,
12.));
#124480=CARTESIAN_POINT('Ctrl Pts',(44.8445846224044,-55.3924090808014,
0.));
#124481=CARTESIAN_POINT('Ctrl Pts',(44.8445846224044,-55.3924090808014,
12.));
#124482=CARTESIAN_POINT('Ctrl Pts',(44.8366146440901,-55.3713206194967,
0.));
#124483=CARTESIAN_POINT('Ctrl Pts',(44.8366146440901,-55.3713206194967,
12.));
#124484=CARTESIAN_POINT('Ctrl Pts',(44.8286396832848,-55.3502831540228,
0.));
#124485=CARTESIAN_POINT('Ctrl Pts',(44.8286396832848,-55.3502831540228,
12.));
#124486=CARTESIAN_POINT('Ctrl Pts',(44.8206598547888,-55.3292967905725,
0.));
#124487=CARTESIAN_POINT('Ctrl Pts',(44.8206598547888,-55.3292967905725,
12.));
#124488=CARTESIAN_POINT('Ctrl Pts',(44.8126752740208,-55.3083616357605,
0.));
#124489=CARTESIAN_POINT('Ctrl Pts',(44.8126752740208,-55.3083616357605,
12.));
#124490=CARTESIAN_POINT('Ctrl Pts',(44.8046860570244,-55.287477796635,0.));
#124491=CARTESIAN_POINT('Ctrl Pts',(44.8046860570244,-55.287477796635,12.));
#124492=CARTESIAN_POINT('Ctrl Pts',(44.796692320474,-55.2666453806883,0.));
#124493=CARTESIAN_POINT('Ctrl Pts',(44.796692320474,-55.2666453806883,12.));
#124494=CARTESIAN_POINT('Ctrl Pts',(44.7886941816823,-55.2458644958617,
0.));
#124495=CARTESIAN_POINT('Ctrl Pts',(44.7886941816823,-55.2458644958617,
12.));
#124496=CARTESIAN_POINT('Ctrl Pts',(44.7806917586077,-55.2251352505474,
0.));
#124497=CARTESIAN_POINT('Ctrl Pts',(44.7806917586077,-55.2251352505474,
12.));
#124498=CARTESIAN_POINT('Ctrl Pts',(44.7726851698618,-55.2044577535865,
0.));
#124499=CARTESIAN_POINT('Ctrl Pts',(44.7726851698618,-55.2044577535865,
12.));
#124500=CARTESIAN_POINT('Ctrl Pts',(44.7646745347108,-55.1838321142777,
0.));
#124501=CARTESIAN_POINT('Ctrl Pts',(44.7646745347108,-55.1838321142777,
12.));
#124502=CARTESIAN_POINT('Ctrl Pts',(44.7566599730771,-55.1632584423813,
0.));
#124503=CARTESIAN_POINT('Ctrl Pts',(44.7566599730771,-55.1632584423813,
12.));
#124504=CARTESIAN_POINT('Ctrl Pts',(44.748641605542,-55.1427368481201,0.));
#124505=CARTESIAN_POINT('Ctrl Pts',(44.748641605542,-55.1427368481201,12.));
#124506=CARTESIAN_POINT('Ctrl Pts',(44.7406195533483,-55.1222674421747,
0.));
#124507=CARTESIAN_POINT('Ctrl Pts',(44.7406195533483,-55.1222674421747,
12.));
#124508=CARTESIAN_POINT('Ctrl Pts',(44.7325939384042,-55.1018503356806,
0.));
#124509=CARTESIAN_POINT('Ctrl Pts',(44.7325939384042,-55.1018503356806,
12.));
#124510=CARTESIAN_POINT('Ctrl Pts',(44.7245648832988,-55.0814856402507,
0.));
#124511=CARTESIAN_POINT('Ctrl Pts',(44.7245648832988,-55.0814856402507,
12.));
#124512=CARTESIAN_POINT('Ctrl Pts',(44.7165325113165,-55.0611734679902,
0.));
#124513=CARTESIAN_POINT('Ctrl Pts',(44.7165325113165,-55.0611734679902,
12.));
#124514=CARTESIAN_POINT('Ctrl Pts',(44.7084969464509,-55.0409139315074,
0.));
#124515=CARTESIAN_POINT('Ctrl Pts',(44.7084969464509,-55.0409139315074,
12.));
#124516=CARTESIAN_POINT('Ctrl Pts',(44.7004583134235,-55.020707143922,0.));
#124517=CARTESIAN_POINT('Ctrl Pts',(44.7004583134235,-55.020707143922,12.));
#124518=CARTESIAN_POINT('Ctrl Pts',(44.6924167376851,-55.0005532188644,
0.));
#124519=CARTESIAN_POINT('Ctrl Pts',(44.6924167376851,-55.0005532188644,
12.));
#124520=CARTESIAN_POINT('Ctrl Pts',(44.6843723453985,-54.9804522704668,
0.));
#124521=CARTESIAN_POINT('Ctrl Pts',(44.6843723453985,-54.9804522704668,
12.));
#124522=CARTESIAN_POINT('Ctrl Pts',(44.6763252634255,-54.9604044133497,
0.));
#124523=CARTESIAN_POINT('Ctrl Pts',(44.6763252634255,-54.9604044133497,
12.));
#124524=CARTESIAN_POINT('Ctrl Pts',(44.6682756193156,-54.9404097626088,
0.));
#124525=CARTESIAN_POINT('Ctrl Pts',(44.6682756193156,-54.9404097626088,
12.));
#124526=CARTESIAN_POINT('Ctrl Pts',(44.6602235412854,-54.9204684337845,
0.));
#124527=CARTESIAN_POINT('Ctrl Pts',(44.6602235412854,-54.9204684337845,
12.));
#124528=CARTESIAN_POINT('Ctrl Pts',(44.6521691582551,-54.9005805428991,
0.));
#124529=CARTESIAN_POINT('Ctrl Pts',(44.6521691582551,-54.9005805428991,
12.));
#124530=CARTESIAN_POINT('Ctrl Pts',(44.6441125999074,-54.8807462065177,
0.));
#124531=CARTESIAN_POINT('Ctrl Pts',(44.6441125999074,-54.8807462065177,
12.));
#124532=CARTESIAN_POINT('Ctrl Pts',(44.6360539967392,-54.860965541796,0.));
#124533=CARTESIAN_POINT('Ctrl Pts',(44.6360539967392,-54.860965541796,12.));
#124534=CARTESIAN_POINT('Ctrl Pts',(44.6279934801159,-54.8412386665264,
0.));
#124535=CARTESIAN_POINT('Ctrl Pts',(44.6279934801159,-54.8412386665264,
12.));
#124536=CARTESIAN_POINT('Ctrl Pts',(44.6199311823276,-54.8215656991817,
0.));
#124537=CARTESIAN_POINT('Ctrl Pts',(44.6199311823276,-54.8215656991817,
12.));
#124538=CARTESIAN_POINT('Ctrl Pts',(44.6118672364889,-54.8019467588257,
0.));
#124539=CARTESIAN_POINT('Ctrl Pts',(44.6118672364889,-54.8019467588257,
12.));
#124540=CARTESIAN_POINT('Ctrl Pts',(44.60380177643,-54.7823819650137,0.));
#124541=CARTESIAN_POINT('Ctrl Pts',(44.60380177643,-54.7823819650137,12.));
#124542=CARTESIAN_POINT('Ctrl Pts',(44.5957349366062,-54.7628714377041,
0.));
#124543=CARTESIAN_POINT('Ctrl Pts',(44.5957349366062,-54.7628714377041,
12.));
#124544=CARTESIAN_POINT('Ctrl Pts',(44.5876668519676,-54.7434152971285,
0.));
#124545=CARTESIAN_POINT('Ctrl Pts',(44.5876668519676,-54.7434152971285,
12.));
#124546=CARTESIAN_POINT('Ctrl Pts',(44.5795976579476,-54.7240136637744,
0.));
#124547=CARTESIAN_POINT('Ctrl Pts',(44.5795976579476,-54.7240136637744,
12.));
#124548=CARTESIAN_POINT('Ctrl Pts',(44.5715274907637,-54.7046666586776,
0.));
#124549=CARTESIAN_POINT('Ctrl Pts',(44.5715274907637,-54.7046666586776,
12.));
#124550=CARTESIAN_POINT('Ctrl Pts',(44.563456487687,-54.685374403676,0.));
#124551=CARTESIAN_POINT('Ctrl Pts',(44.563456487687,-54.685374403676,12.));
#124552=CARTESIAN_POINT('Ctrl Pts',(44.5553847872712,-54.6661370216242,
0.));
#124553=CARTESIAN_POINT('Ctrl Pts',(44.5553847872712,-54.6661370216242,
12.));
#124554=CARTESIAN_POINT('Ctrl Pts',(44.5473125297289,-54.6469546367381,
0.));
#124555=CARTESIAN_POINT('Ctrl Pts',(44.5473125297289,-54.6469546367381,
12.));
#124556=CARTESIAN_POINT('Ctrl Pts',(44.5392398566775,-54.6278273743554,
0.));
#124557=CARTESIAN_POINT('Ctrl Pts',(44.5392398566775,-54.6278273743554,
12.));
#124558=CARTESIAN_POINT('Ctrl Pts',(44.5311669104495,-54.6087553602889,
0.));
#124559=CARTESIAN_POINT('Ctrl Pts',(44.5311669104495,-54.6087553602889,
12.));
#124560=CARTESIAN_POINT('Ctrl Pts',(44.5230938335165,-54.5897387202812,
0.));
#124561=CARTESIAN_POINT('Ctrl Pts',(44.5230938335165,-54.5897387202812,
12.));
#124562=CARTESIAN_POINT('Ctrl Pts',(44.5150207679007,-54.5707775794436,
0.));
#124563=CARTESIAN_POINT('Ctrl Pts',(44.5150207679007,-54.5707775794436,
12.));
#124564=CARTESIAN_POINT('Ctrl Pts',(44.5069478544977,-54.5518720616056,
0.));
#124565=CARTESIAN_POINT('Ctrl Pts',(44.5069478544977,-54.5518720616056,
12.));
#124566=CARTESIAN_POINT('Ctrl Pts',(44.4988752343744,-54.5330222905475,
0.));
#124567=CARTESIAN_POINT('Ctrl Pts',(44.4988752343744,-54.5330222905475,
12.));
#124568=CARTESIAN_POINT('Ctrl Pts',(44.4908030503225,-54.5142283914704,
0.));
#124569=CARTESIAN_POINT('Ctrl Pts',(44.4908030503225,-54.5142283914704,
12.));
#124570=CARTESIAN_POINT('Ctrl Pts',(44.4827314481264,-54.495490492193,0.));
#124571=CARTESIAN_POINT('Ctrl Pts',(44.4827314481264,-54.495490492193,12.));
#124572=CARTESIAN_POINT('Ctrl Pts',(44.4746605784031,-54.4768087248824,
0.));
#124573=CARTESIAN_POINT('Ctrl Pts',(44.4746605784031,-54.4768087248824,
12.));
#124574=CARTESIAN_POINT('Ctrl Pts',(44.4665905967668,-54.4581832262033,
0.));
#124575=CARTESIAN_POINT('Ctrl Pts',(44.4665905967668,-54.4581832262033,
12.));
#124576=CARTESIAN_POINT('Ctrl Pts',(44.4585216599908,-54.4396141336978,
0.));
#124577=CARTESIAN_POINT('Ctrl Pts',(44.4585216599908,-54.4396141336978,
12.));
#124578=CARTESIAN_POINT('Ctrl Pts',(44.4504539226328,-54.421101582595,0.));
#124579=CARTESIAN_POINT('Ctrl Pts',(44.4504539226328,-54.421101582595,12.));
#124580=CARTESIAN_POINT('Ctrl Pts',(44.4423875340996,-54.4026457030335,
0.));
#124581=CARTESIAN_POINT('Ctrl Pts',(44.4423875340996,-54.4026457030335,
12.));
#124582=CARTESIAN_POINT('Ctrl Pts',(44.4343226339593,-54.3842466156196,
0.));
#124583=CARTESIAN_POINT('Ctrl Pts',(44.4343226339593,-54.3842466156196,
12.));
#124584=CARTESIAN_POINT('Ctrl Pts',(44.4262593564712,-54.3659044357119,
0.));
#124585=CARTESIAN_POINT('Ctrl Pts',(44.4262593564712,-54.3659044357119,
12.));
#124586=CARTESIAN_POINT('Ctrl Pts',(44.4181978395851,-54.3476192819352,
0.));
#124587=CARTESIAN_POINT('Ctrl Pts',(44.4181978395851,-54.3476192819352,
12.));
#124588=CARTESIAN_POINT('Ctrl Pts',(44.4101382321834,-54.3293912830237,
0.));
#124589=CARTESIAN_POINT('Ctrl Pts',(44.4101382321834,-54.3293912830237,
12.));
#124590=CARTESIAN_POINT('Ctrl Pts',(44.402080702809,-54.3112205860716,0.));
#124591=CARTESIAN_POINT('Ctrl Pts',(44.402080702809,-54.3112205860716,12.));
#124592=CARTESIAN_POINT('Ctrl Pts',(44.3940254456331,-54.2931073621553,
0.));
#124593=CARTESIAN_POINT('Ctrl Pts',(44.3940254456331,-54.2931073621553,
12.));
#124594=CARTESIAN_POINT('Ctrl Pts',(44.3859726620183,-54.2750517888579,
0.));
#124595=CARTESIAN_POINT('Ctrl Pts',(44.3859726620183,-54.2750517888579,
12.));
#124596=CARTESIAN_POINT('Ctrl Pts',(44.3779225430406,-54.2570540336475,
0.));
#124597=CARTESIAN_POINT('Ctrl Pts',(44.3779225430406,-54.2570540336475,
12.));
#124598=CARTESIAN_POINT('Ctrl Pts',(44.3698752533562,-54.2391142386412,
0.));
#124599=CARTESIAN_POINT('Ctrl Pts',(44.3698752533562,-54.2391142386412,
12.));
#124600=CARTESIAN_POINT('Ctrl Pts',(44.361830910343,-54.2212325006052,0.));
#124601=CARTESIAN_POINT('Ctrl Pts',(44.361830910343,-54.2212325006052,12.));
#124602=CARTESIAN_POINT('Ctrl Pts',(44.3537895824096,-54.2034088701928,
0.));
#124603=CARTESIAN_POINT('Ctrl Pts',(44.3537895824096,-54.2034088701928,
12.));
#124604=CARTESIAN_POINT('Ctrl Pts',(44.3473589597726,-54.1891964684727,
0.));
#124605=CARTESIAN_POINT('Ctrl Pts',(44.3473589597726,-54.1891964684727,
12.));
#124606=CARTESIAN_POINT('Ctrl Pts',(44.3425373700993,-54.1785633257639,
0.));
#124607=CARTESIAN_POINT('Ctrl Pts',(44.3425373700993,-54.1785633257639,
12.));
#124608=CARTESIAN_POINT('Ctrl Pts',(44.3393235891075,-54.1714861895346,
0.));
#124609=CARTESIAN_POINT('Ctrl Pts',(44.3393235891075,-54.1714861895346,
12.));
#124610=CARTESIAN_POINT('Ctrl Pts',(44.3377168516418,-54.1679505278134,
0.));
#124611=CARTESIAN_POINT('Ctrl Pts',(44.3377168516418,-54.1679505278134,
12.));
#124612=CARTESIAN_POINT('',(44.3377168516418,-54.1679505278134,12.));
#124613=CARTESIAN_POINT('Ctrl Pts',(44.3377168516418,-54.1679505278134,
12.));
#124614=CARTESIAN_POINT('Ctrl Pts',(44.3393235891075,-54.1714861895346,
12.));
#124615=CARTESIAN_POINT('Ctrl Pts',(44.3425373700993,-54.1785633257639,
12.));
#124616=CARTESIAN_POINT('Ctrl Pts',(44.3473589597726,-54.1891964684727,
12.));
#124617=CARTESIAN_POINT('Ctrl Pts',(44.3537895824096,-54.2034088701928,
12.));
#124618=CARTESIAN_POINT('Ctrl Pts',(44.361830910343,-54.2212325006052,12.));
#124619=CARTESIAN_POINT('Ctrl Pts',(44.3698752533562,-54.2391142386412,
12.));
#124620=CARTESIAN_POINT('Ctrl Pts',(44.3779225430406,-54.2570540336475,
12.));
#124621=CARTESIAN_POINT('Ctrl Pts',(44.3859726620183,-54.2750517888579,
12.));
#124622=CARTESIAN_POINT('Ctrl Pts',(44.3940254456331,-54.2931073621553,
12.));
#124623=CARTESIAN_POINT('Ctrl Pts',(44.402080702809,-54.3112205860716,12.));
#124624=CARTESIAN_POINT('Ctrl Pts',(44.4101382321834,-54.3293912830237,
12.));
#124625=CARTESIAN_POINT('Ctrl Pts',(44.4181978395851,-54.3476192819352,
12.));
#124626=CARTESIAN_POINT('Ctrl Pts',(44.4262593564712,-54.3659044357119,
12.));
#124627=CARTESIAN_POINT('Ctrl Pts',(44.4343226339593,-54.3842466156196,
12.));
#124628=CARTESIAN_POINT('Ctrl Pts',(44.4423875340996,-54.4026457030335,
12.));
#124629=CARTESIAN_POINT('Ctrl Pts',(44.4504539226328,-54.421101582595,12.));
#124630=CARTESIAN_POINT('Ctrl Pts',(44.4585216599908,-54.4396141336978,
12.));
#124631=CARTESIAN_POINT('Ctrl Pts',(44.4665905967668,-54.4581832262033,
12.));
#124632=CARTESIAN_POINT('Ctrl Pts',(44.4746605784031,-54.4768087248824,
12.));
#124633=CARTESIAN_POINT('Ctrl Pts',(44.4827314481264,-54.495490492193,12.));
#124634=CARTESIAN_POINT('Ctrl Pts',(44.4908030503225,-54.5142283914704,
12.));
#124635=CARTESIAN_POINT('Ctrl Pts',(44.4988752343744,-54.5330222905475,
12.));
#124636=CARTESIAN_POINT('Ctrl Pts',(44.5069478544977,-54.5518720616056,
12.));
#124637=CARTESIAN_POINT('Ctrl Pts',(44.5150207679007,-54.5707775794436,
12.));
#124638=CARTESIAN_POINT('Ctrl Pts',(44.5230938335165,-54.5897387202812,
12.));
#124639=CARTESIAN_POINT('Ctrl Pts',(44.5311669104495,-54.6087553602889,
12.));
#124640=CARTESIAN_POINT('Ctrl Pts',(44.5392398566775,-54.6278273743554,
12.));
#124641=CARTESIAN_POINT('Ctrl Pts',(44.5473125297289,-54.6469546367381,
12.));
#124642=CARTESIAN_POINT('Ctrl Pts',(44.5553847872712,-54.6661370216242,
12.));
#124643=CARTESIAN_POINT('Ctrl Pts',(44.563456487687,-54.685374403676,12.));
#124644=CARTESIAN_POINT('Ctrl Pts',(44.5715274907637,-54.7046666586776,
12.));
#124645=CARTESIAN_POINT('Ctrl Pts',(44.5795976579476,-54.7240136637744,
12.));
#124646=CARTESIAN_POINT('Ctrl Pts',(44.5876668519676,-54.7434152971285,
12.));
#124647=CARTESIAN_POINT('Ctrl Pts',(44.5957349366062,-54.7628714377041,
12.));
#124648=CARTESIAN_POINT('Ctrl Pts',(44.60380177643,-54.7823819650137,12.));
#124649=CARTESIAN_POINT('Ctrl Pts',(44.6118672364889,-54.8019467588257,
12.));
#124650=CARTESIAN_POINT('Ctrl Pts',(44.6199311823276,-54.8215656991817,
12.));
#124651=CARTESIAN_POINT('Ctrl Pts',(44.6279934801159,-54.8412386665264,
12.));
#124652=CARTESIAN_POINT('Ctrl Pts',(44.6360539967392,-54.860965541796,12.));
#124653=CARTESIAN_POINT('Ctrl Pts',(44.6441125999074,-54.8807462065177,
12.));
#124654=CARTESIAN_POINT('Ctrl Pts',(44.6521691582551,-54.9005805428991,
12.));
#124655=CARTESIAN_POINT('Ctrl Pts',(44.6602235412854,-54.9204684337845,
12.));
#124656=CARTESIAN_POINT('Ctrl Pts',(44.6682756193156,-54.9404097626088,
12.));
#124657=CARTESIAN_POINT('Ctrl Pts',(44.6763252634255,-54.9604044133497,
12.));
#124658=CARTESIAN_POINT('Ctrl Pts',(44.6843723453985,-54.9804522704668,
12.));
#124659=CARTESIAN_POINT('Ctrl Pts',(44.6924167376851,-55.0005532188644,
12.));
#124660=CARTESIAN_POINT('Ctrl Pts',(44.7004583134235,-55.020707143922,12.));
#124661=CARTESIAN_POINT('Ctrl Pts',(44.7084969464509,-55.0409139315074,
12.));
#124662=CARTESIAN_POINT('Ctrl Pts',(44.7165325113165,-55.0611734679902,
12.));
#124663=CARTESIAN_POINT('Ctrl Pts',(44.7245648832988,-55.0814856402507,
12.));
#124664=CARTESIAN_POINT('Ctrl Pts',(44.7325939384042,-55.1018503356806,
12.));
#124665=CARTESIAN_POINT('Ctrl Pts',(44.7406195533483,-55.1222674421747,
12.));
#124666=CARTESIAN_POINT('Ctrl Pts',(44.748641605542,-55.1427368481201,12.));
#124667=CARTESIAN_POINT('Ctrl Pts',(44.7566599730771,-55.1632584423813,
12.));
#124668=CARTESIAN_POINT('Ctrl Pts',(44.7646745347108,-55.1838321142777,
12.));
#124669=CARTESIAN_POINT('Ctrl Pts',(44.7726851698618,-55.2044577535865,
12.));
#124670=CARTESIAN_POINT('Ctrl Pts',(44.7806917586077,-55.2251352505474,
12.));
#124671=CARTESIAN_POINT('Ctrl Pts',(44.7886941816823,-55.2458644958617,
12.));
#124672=CARTESIAN_POINT('Ctrl Pts',(44.796692320474,-55.2666453806883,12.));
#124673=CARTESIAN_POINT('Ctrl Pts',(44.8046860570244,-55.287477796635,12.));
#124674=CARTESIAN_POINT('Ctrl Pts',(44.8126752740208,-55.3083616357605,
12.));
#124675=CARTESIAN_POINT('Ctrl Pts',(44.8206598547888,-55.3292967905725,
12.));
#124676=CARTESIAN_POINT('Ctrl Pts',(44.8286396832848,-55.3502831540228,
12.));
#124677=CARTESIAN_POINT('Ctrl Pts',(44.8366146440901,-55.3713206194967,
12.));
#124678=CARTESIAN_POINT('Ctrl Pts',(44.8445846224044,-55.3924090808014,
12.));
#124679=CARTESIAN_POINT('Ctrl Pts',(44.8525495040408,-55.4135484321718,
12.));
#124680=CARTESIAN_POINT('Ctrl Pts',(44.8605091754214,-55.4347385682704,
12.));
#124681=CARTESIAN_POINT('Ctrl Pts',(44.8684635235725,-55.4559793841836,
12.));
#124682=CARTESIAN_POINT('Ctrl Pts',(44.8764124361207,-55.4772707754126,
12.));
#124683=CARTESIAN_POINT('Ctrl Pts',(44.8843558012886,-55.4986126378656,
12.));
#124684=CARTESIAN_POINT('Ctrl Pts',(44.8922935078889,-55.5200048678629,
12.));
#124685=CARTESIAN_POINT('Ctrl Pts',(44.9002254453183,-55.541447362134,12.));
#124686=CARTESIAN_POINT('Ctrl Pts',(44.908151503553,-55.5629400178142,12.));
#124687=CARTESIAN_POINT('Ctrl Pts',(44.9160715731443,-55.5844827324338,
12.));
#124688=CARTESIAN_POINT('Ctrl Pts',(44.9239855452144,-55.6060754039121,
12.));
#124689=CARTESIAN_POINT('Ctrl Pts',(44.9318933114507,-55.6277179305633,
12.));
#124690=CARTESIAN_POINT('Ctrl Pts',(44.9397947641007,-55.6494102110935,
12.));
#124691=CARTESIAN_POINT('Ctrl Pts',(44.9476897959685,-55.6711521445979,
12.));
#124692=CARTESIAN_POINT('Ctrl Pts',(44.9555783004106,-55.6929436305489,
12.));
#124693=CARTESIAN_POINT('Ctrl Pts',(44.9634601713321,-55.714784568793,12.));
#124694=CARTESIAN_POINT('Ctrl Pts',(44.9713353031804,-55.7366748595551,
12.));
#124695=CARTESIAN_POINT('Ctrl Pts',(44.9792035909413,-55.7586144034367,
12.));
#124696=CARTESIAN_POINT('Ctrl Pts',(44.9870649301342,-55.7806031014106,
12.));
#124697=CARTESIAN_POINT('Ctrl Pts',(44.9949192168093,-55.8026408548105,
12.));
#124698=CARTESIAN_POINT('Ctrl Pts',(45.0027663475433,-55.8247275653289,
12.));
#124699=CARTESIAN_POINT('Ctrl Pts',(45.0106062194342,-55.8468631350218,
12.));
#124700=CARTESIAN_POINT('Ctrl Pts',(45.0184387300973,-55.8690474663065,
12.));
#124701=CARTESIAN_POINT('Ctrl Pts',(45.0262637776615,-55.8912804619577,
12.));
#124702=CARTESIAN_POINT('Ctrl Pts',(45.0340812607657,-55.9135620250954,
12.));
#124703=CARTESIAN_POINT('Ctrl Pts',(45.0418910785551,-55.9358920591837,
12.));
#124704=CARTESIAN_POINT('Ctrl Pts',(45.0496931306755,-55.9582704680356,
12.));
#124705=CARTESIAN_POINT('Ctrl Pts',(45.0574873172695,-55.9806971558097,
12.));
#124706=CARTESIAN_POINT('Ctrl Pts',(45.0652735389733,-56.003172027008,12.));
#124707=CARTESIAN_POINT('Ctrl Pts',(45.0730516969149,-56.0256949864639,
12.));
#124708=CARTESIAN_POINT('Ctrl Pts',(45.0808216927089,-56.048265939342,12.));
#124709=CARTESIAN_POINT('Ctrl Pts',(45.0885834284517,-56.0708847911416,
12.));
#124710=CARTESIAN_POINT('Ctrl Pts',(45.0963368067177,-56.0935514476945,
12.));
#124711=CARTESIAN_POINT('Ctrl Pts',(45.1040817305561,-56.116265815162,12.));
#124712=CARTESIAN_POINT('Ctrl Pts',(45.1118181034888,-56.1390278000226,
12.));
#124713=CARTESIAN_POINT('Ctrl Pts',(45.1195458295063,-56.1618373090732,
12.));
#124714=CARTESIAN_POINT('Ctrl Pts',(45.127264813063,-56.1846942494325,12.));
#124715=CARTESIAN_POINT('Ctrl Pts',(45.1349749590738,-56.2075985285393,
12.));
#124716=CARTESIAN_POINT('Ctrl Pts',(45.1426761729105,-56.2305500541489,
12.));
#124717=CARTESIAN_POINT('Ctrl Pts',(45.1503683604005,-56.2535487343221,
12.));
#124718=CARTESIAN_POINT('Ctrl Pts',(45.1580514278223,-56.2765944774245,
12.));
#124719=CARTESIAN_POINT('Ctrl Pts',(45.1657252819013,-56.2996871921316,
12.));
#124720=CARTESIAN_POINT('Ctrl Pts',(45.1733898298061,-56.3228267874264,
12.));
#124721=CARTESIAN_POINT('Ctrl Pts',(45.1810449791453,-56.3460131725964,
12.));
#124722=CARTESIAN_POINT('Ctrl Pts',(45.1886906379667,-56.3692462572231,
12.));
#124723=CARTESIAN_POINT('Ctrl Pts',(45.1963267147529,-56.3925259511806,
12.));
#124724=CARTESIAN_POINT('Ctrl Pts',(45.2039531184172,-56.4158521646411,
12.));
#124725=CARTESIAN_POINT('Ctrl Pts',(45.2115697583001,-56.4392248080732,
12.));
#124726=CARTESIAN_POINT('Ctrl Pts',(45.2191765441667,-56.4626437922386,
12.));
#124727=CARTESIAN_POINT('Ctrl Pts',(45.2267733862049,-56.4861090281823,
12.));
#124728=CARTESIAN_POINT('Ctrl Pts',(45.2343601950228,-56.5096204272306,
12.));
#124729=CARTESIAN_POINT('Ctrl Pts',(45.2419368816429,-56.5331779009958,
12.));
#124730=CARTESIAN_POINT('Ctrl Pts',(45.2495033575,-56.5567813613756,12.));
#124731=CARTESIAN_POINT('Ctrl Pts',(45.257059534438,-56.5804307205505,12.));
#124732=CARTESIAN_POINT('Ctrl Pts',(45.2646053247087,-56.6041258909741,
12.));
#124733=CARTESIAN_POINT('Ctrl Pts',(45.2721406409695,-56.6278667853702,
12.));
#124734=CARTESIAN_POINT('Ctrl Pts',(45.2796653962785,-56.6516533167384,
12.));
#124735=CARTESIAN_POINT('Ctrl Pts',(45.2871795040906,-56.6754853983528,
12.));
#124736=CARTESIAN_POINT('Ctrl Pts',(45.2946828782559,-56.69936294376,12.));
#124737=CARTESIAN_POINT('Ctrl Pts',(45.3021754330179,-56.7232858667709,
12.));
#124738=CARTESIAN_POINT('Ctrl Pts',(45.3096570830118,-56.7472540814553,
12.));
#124739=CARTESIAN_POINT('Ctrl Pts',(45.31712774326,-56.7712675021491,12.));
#124740=CARTESIAN_POINT('Ctrl Pts',(45.3245873291684,-56.7953260434524,
12.));
#124741=CARTESIAN_POINT('Ctrl Pts',(45.332035756524,-56.8194296202291,12.));
#124742=CARTESIAN_POINT('Ctrl Pts',(45.3394729414931,-56.8435781475981,
12.));
#124743=CARTESIAN_POINT('Ctrl Pts',(45.3468988006203,-56.8677715409268,
12.));
#124744=CARTESIAN_POINT('Ctrl Pts',(45.3543132508239,-56.8920097158377,
12.));
#124745=CARTESIAN_POINT('Ctrl Pts',(45.3617162093923,-56.9162925882085,
12.));
#124746=CARTESIAN_POINT('Ctrl Pts',(45.3691075939827,-56.9406200741714,
12.));
#124747=CARTESIAN_POINT('Ctrl Pts',(45.3764873226196,-56.9649920901073,
12.));
#124748=CARTESIAN_POINT('Ctrl Pts',(45.3838553136948,-56.9894085526373,
12.));
#124749=CARTESIAN_POINT('Ctrl Pts',(45.3912114859616,-57.0138693786278,
12.));
#124750=CARTESIAN_POINT('Ctrl Pts',(45.3985557585311,-57.0383744851913,
12.));
#124751=CARTESIAN_POINT('Ctrl Pts',(45.4058880508693,-57.0629237896848,
12.));
#124752=CARTESIAN_POINT('Ctrl Pts',(45.4132082827948,-57.0875172097051,
12.));
#124753=CARTESIAN_POINT('Ctrl Pts',(45.4205163744782,-57.112154663078,12.));
#124754=CARTESIAN_POINT('Ctrl Pts',(45.4278122464389,-57.136836067863,12.));
#124755=CARTESIAN_POINT('Ctrl Pts',(45.4350958195434,-57.1615613423584,
12.));
#124756=CARTESIAN_POINT('Ctrl Pts',(45.4423670150034,-57.186330405101,12.));
#124757=CARTESIAN_POINT('Ctrl Pts',(45.4496257543759,-57.2111431748631,
12.));
#124758=CARTESIAN_POINT('Ctrl Pts',(45.4568719595642,-57.2359995706447,
12.));
#124759=CARTESIAN_POINT('Ctrl Pts',(45.4641055528141,-57.2608995116733,
12.));
#124760=CARTESIAN_POINT('Ctrl Pts',(45.4713264567063,-57.2858429174062,
12.));
#124761=CARTESIAN_POINT('Ctrl Pts',(45.4785345941507,-57.3108297075265,
12.));
#124762=CARTESIAN_POINT('Ctrl Pts',(45.4857298883824,-57.3358598019389,
12.));
#124763=CARTESIAN_POINT('Ctrl Pts',(45.4929122629572,-57.3609331207574,
12.));
#124764=CARTESIAN_POINT('Ctrl Pts',(45.500081641751,-57.3860495843033,12.));
#124765=CARTESIAN_POINT('Ctrl Pts',(45.5072379489631,-57.4112091131183,
12.));
#124766=CARTESIAN_POINT('Ctrl Pts',(45.5143811091205,-57.4364116279702,
12.));
#124767=CARTESIAN_POINT('Ctrl Pts',(45.5215110470825,-57.4616570498568,
12.));
#124768=CARTESIAN_POINT('Ctrl Pts',(45.5286276880485,-57.4869453000063,
12.));
#124769=CARTESIAN_POINT('Ctrl Pts',(45.5357309575611,-57.5122762998745,
12.));
#124770=CARTESIAN_POINT('Ctrl Pts',(45.542820781484,-57.537649971135,12.));
#124771=CARTESIAN_POINT('Ctrl Pts',(45.5498970859835,-57.563066235668,12.));
#124772=CARTESIAN_POINT('Ctrl Pts',(45.5569597975096,-57.5885250155433,
12.));
#124773=CARTESIAN_POINT('Ctrl Pts',(45.5640088427813,-57.614026233004,12.));
#124774=CARTESIAN_POINT('Ctrl Pts',(45.5710441487674,-57.6395698104404,
12.));
#124775=CARTESIAN_POINT('Ctrl Pts',(45.5780656427163,-57.6651556704237,
12.));
#124776=CARTESIAN_POINT('Ctrl Pts',(45.5850732521896,-57.6907837357417,
12.));
#124777=CARTESIAN_POINT('Ctrl Pts',(45.5920669050986,-57.7164539294314,
12.));
#124778=CARTESIAN_POINT('Ctrl Pts',(45.5990465297344,-57.7421661748026,
12.));
#124779=CARTESIAN_POINT('Ctrl Pts',(45.6060120548205,-57.7679203954742,
12.));
#124780=CARTESIAN_POINT('Ctrl Pts',(45.6129634094683,-57.7937165153387,
12.));
#124781=CARTESIAN_POINT('Ctrl Pts',(45.6199005230784,-57.8195544584845,
12.));
#124782=CARTESIAN_POINT('Ctrl Pts',(45.6268233252544,-57.8454341491238,
12.));
#124783=CARTESIAN_POINT('Ctrl Pts',(45.6337317457252,-57.8713555115232,
12.));
#124784=CARTESIAN_POINT('Ctrl Pts',(45.6406257142382,-57.8973184699034,
12.));
#124785=CARTESIAN_POINT('Ctrl Pts',(45.6475051605535,-57.9233229484311,
12.));
#124786=CARTESIAN_POINT('Ctrl Pts',(45.6543700146679,-57.9493688714237,
12.));
#124787=CARTESIAN_POINT('Ctrl Pts',(45.661220206992,-57.9754561635061,12.));
#124788=CARTESIAN_POINT('Ctrl Pts',(45.6680556685493,-58.0015847497837,
12.));
#124789=CARTESIAN_POINT('Ctrl Pts',(45.6748763311643,-58.0277545560012,
12.));
#124790=CARTESIAN_POINT('Ctrl Pts',(45.6816821276678,-58.0539655087117,
12.));
#124791=CARTESIAN_POINT('Ctrl Pts',(45.6884729914485,-58.0802175348966,
12.));
#124792=CARTESIAN_POINT('Ctrl Pts',(45.695248856015,-58.1065105615907,12.));
#124793=CARTESIAN_POINT('Ctrl Pts',(45.702009654518,-58.1328445154676,12.));
#124794=CARTESIAN_POINT('Ctrl Pts',(45.7087553193771,-58.1592193225137,
12.));
#124795=CARTESIAN_POINT('Ctrl Pts',(45.7154857816483,-58.185634907469,12.));
#124796=CARTESIAN_POINT('Ctrl Pts',(45.7222009715397,-58.2120911942772,
12.));
#124797=CARTESIAN_POINT('Ctrl Pts',(45.7289008195579,-58.2385881070913,
12.));
#124798=CARTESIAN_POINT('Ctrl Pts',(45.7355852575107,-58.2651255711453,
12.));
#124799=CARTESIAN_POINT('Ctrl Pts',(45.742254219463,-58.291703513584,12.));
#124800=CARTESIAN_POINT('Ctrl Pts',(45.7489076429763,-58.3183218645316,
12.));
#124801=CARTESIAN_POINT('Ctrl Pts',(45.755545469402,-58.3449805573423,12.));
#124802=CARTESIAN_POINT('Ctrl Pts',(45.7612219538124,-58.3678667473437,
12.));
#124803=CARTESIAN_POINT('Ctrl Pts',(45.7655655205367,-58.3854348517442,
12.));
#124804=CARTESIAN_POINT('Ctrl Pts',(45.7685831165564,-58.3976670481067,
12.));
#124805=CARTESIAN_POINT('Ctrl Pts',(45.7702793558176,-58.4045515723353,
12.));
#124806=CARTESIAN_POINT('Ctrl Pts',(45.7706564944895,-58.4060826907792,
12.));
#124807=CARTESIAN_POINT('',(44.3377168516418,-54.1679505278134,0.));
#124808=CARTESIAN_POINT('',(44.3377168516418,-54.1679505278134,0.));
#124809=CARTESIAN_POINT('Ctrl Pts',(45.7706564944895,-58.4060826907792,
0.));
#124810=CARTESIAN_POINT('Ctrl Pts',(45.7702793558176,-58.4045515723353,
0.));
#124811=CARTESIAN_POINT('Ctrl Pts',(45.7685831165564,-58.3976670481067,
0.));
#124812=CARTESIAN_POINT('Ctrl Pts',(45.7655655205367,-58.3854348517442,
0.));
#124813=CARTESIAN_POINT('Ctrl Pts',(45.7612219538124,-58.3678667473437,
0.));
#124814=CARTESIAN_POINT('Ctrl Pts',(45.755545469402,-58.3449805573423,0.));
#124815=CARTESIAN_POINT('Ctrl Pts',(45.7489076429763,-58.3183218645316,
0.));
#124816=CARTESIAN_POINT('Ctrl Pts',(45.742254219463,-58.291703513584,0.));
#124817=CARTESIAN_POINT('Ctrl Pts',(45.7355852575107,-58.2651255711453,
0.));
#124818=CARTESIAN_POINT('Ctrl Pts',(45.7289008195579,-58.2385881070913,
0.));
#124819=CARTESIAN_POINT('Ctrl Pts',(45.7222009715397,-58.2120911942772,
0.));
#124820=CARTESIAN_POINT('Ctrl Pts',(45.7154857816483,-58.185634907469,0.));
#124821=CARTESIAN_POINT('Ctrl Pts',(45.7087553193771,-58.1592193225137,
0.));
#124822=CARTESIAN_POINT('Ctrl Pts',(45.702009654518,-58.1328445154676,0.));
#124823=CARTESIAN_POINT('Ctrl Pts',(45.695248856015,-58.1065105615907,0.));
#124824=CARTESIAN_POINT('Ctrl Pts',(45.6884729914485,-58.0802175348966,
0.));
#124825=CARTESIAN_POINT('Ctrl Pts',(45.6816821276678,-58.0539655087117,
0.));
#124826=CARTESIAN_POINT('Ctrl Pts',(45.6748763311643,-58.0277545560012,
0.));
#124827=CARTESIAN_POINT('Ctrl Pts',(45.6680556685493,-58.0015847497837,
0.));
#124828=CARTESIAN_POINT('Ctrl Pts',(45.661220206992,-57.9754561635061,0.));
#124829=CARTESIAN_POINT('Ctrl Pts',(45.6543700146679,-57.9493688714237,
0.));
#124830=CARTESIAN_POINT('Ctrl Pts',(45.6475051605535,-57.9233229484311,
0.));
#124831=CARTESIAN_POINT('Ctrl Pts',(45.6406257142382,-57.8973184699034,
0.));
#124832=CARTESIAN_POINT('Ctrl Pts',(45.6337317457252,-57.8713555115232,
0.));
#124833=CARTESIAN_POINT('Ctrl Pts',(45.6268233252544,-57.8454341491238,
0.));
#124834=CARTESIAN_POINT('Ctrl Pts',(45.6199005230784,-57.8195544584845,
0.));
#124835=CARTESIAN_POINT('Ctrl Pts',(45.6129634094683,-57.7937165153387,
0.));
#124836=CARTESIAN_POINT('Ctrl Pts',(45.6060120548205,-57.7679203954742,
0.));
#124837=CARTESIAN_POINT('Ctrl Pts',(45.5990465297344,-57.7421661748026,
0.));
#124838=CARTESIAN_POINT('Ctrl Pts',(45.5920669050986,-57.7164539294314,
0.));
#124839=CARTESIAN_POINT('Ctrl Pts',(45.5850732521896,-57.6907837357417,
0.));
#124840=CARTESIAN_POINT('Ctrl Pts',(45.5780656427163,-57.6651556704237,
0.));
#124841=CARTESIAN_POINT('Ctrl Pts',(45.5710441487674,-57.6395698104404,
0.));
#124842=CARTESIAN_POINT('Ctrl Pts',(45.5640088427813,-57.614026233004,0.));
#124843=CARTESIAN_POINT('Ctrl Pts',(45.5569597975096,-57.5885250155433,
0.));
#124844=CARTESIAN_POINT('Ctrl Pts',(45.5498970859835,-57.563066235668,0.));
#124845=CARTESIAN_POINT('Ctrl Pts',(45.542820781484,-57.537649971135,0.));
#124846=CARTESIAN_POINT('Ctrl Pts',(45.5357309575611,-57.5122762998745,
0.));
#124847=CARTESIAN_POINT('Ctrl Pts',(45.5286276880485,-57.4869453000063,
0.));
#124848=CARTESIAN_POINT('Ctrl Pts',(45.5215110470825,-57.4616570498568,
0.));
#124849=CARTESIAN_POINT('Ctrl Pts',(45.5143811091205,-57.4364116279702,
0.));
#124850=CARTESIAN_POINT('Ctrl Pts',(45.5072379489631,-57.4112091131183,
0.));
#124851=CARTESIAN_POINT('Ctrl Pts',(45.500081641751,-57.3860495843033,0.));
#124852=CARTESIAN_POINT('Ctrl Pts',(45.4929122629572,-57.3609331207574,
0.));
#124853=CARTESIAN_POINT('Ctrl Pts',(45.4857298883824,-57.3358598019389,
0.));
#124854=CARTESIAN_POINT('Ctrl Pts',(45.4785345941507,-57.3108297075265,
0.));
#124855=CARTESIAN_POINT('Ctrl Pts',(45.4713264567063,-57.2858429174062,
0.));
#124856=CARTESIAN_POINT('Ctrl Pts',(45.4641055528141,-57.2608995116733,
0.));
#124857=CARTESIAN_POINT('Ctrl Pts',(45.4568719595642,-57.2359995706447,
0.));
#124858=CARTESIAN_POINT('Ctrl Pts',(45.4496257543759,-57.2111431748631,
0.));
#124859=CARTESIAN_POINT('Ctrl Pts',(45.4423670150034,-57.186330405101,0.));
#124860=CARTESIAN_POINT('Ctrl Pts',(45.4350958195434,-57.1615613423584,
0.));
#124861=CARTESIAN_POINT('Ctrl Pts',(45.4278122464389,-57.136836067863,0.));
#124862=CARTESIAN_POINT('Ctrl Pts',(45.4205163744782,-57.112154663078,0.));
#124863=CARTESIAN_POINT('Ctrl Pts',(45.4132082827948,-57.0875172097051,
0.));
#124864=CARTESIAN_POINT('Ctrl Pts',(45.4058880508693,-57.0629237896848,
0.));
#124865=CARTESIAN_POINT('Ctrl Pts',(45.3985557585311,-57.0383744851913,
0.));
#124866=CARTESIAN_POINT('Ctrl Pts',(45.3912114859616,-57.0138693786278,
0.));
#124867=CARTESIAN_POINT('Ctrl Pts',(45.3838553136948,-56.9894085526373,
0.));
#124868=CARTESIAN_POINT('Ctrl Pts',(45.3764873226196,-56.9649920901073,
0.));
#124869=CARTESIAN_POINT('Ctrl Pts',(45.3691075939827,-56.9406200741714,
0.));
#124870=CARTESIAN_POINT('Ctrl Pts',(45.3617162093923,-56.9162925882085,
0.));
#124871=CARTESIAN_POINT('Ctrl Pts',(45.3543132508239,-56.8920097158377,
0.));
#124872=CARTESIAN_POINT('Ctrl Pts',(45.3468988006203,-56.8677715409268,
0.));
#124873=CARTESIAN_POINT('Ctrl Pts',(45.3394729414931,-56.8435781475981,
0.));
#124874=CARTESIAN_POINT('Ctrl Pts',(45.332035756524,-56.8194296202291,0.));
#124875=CARTESIAN_POINT('Ctrl Pts',(45.3245873291684,-56.7953260434524,
0.));
#124876=CARTESIAN_POINT('Ctrl Pts',(45.31712774326,-56.7712675021491,0.));
#124877=CARTESIAN_POINT('Ctrl Pts',(45.3096570830118,-56.7472540814553,
0.));
#124878=CARTESIAN_POINT('Ctrl Pts',(45.3021754330179,-56.7232858667709,
0.));
#124879=CARTESIAN_POINT('Ctrl Pts',(45.2946828782559,-56.69936294376,0.));
#124880=CARTESIAN_POINT('Ctrl Pts',(45.2871795040906,-56.6754853983528,
0.));
#124881=CARTESIAN_POINT('Ctrl Pts',(45.2796653962785,-56.6516533167384,
0.));
#124882=CARTESIAN_POINT('Ctrl Pts',(45.2721406409695,-56.6278667853702,
0.));
#124883=CARTESIAN_POINT('Ctrl Pts',(45.2646053247087,-56.6041258909741,
0.));
#124884=CARTESIAN_POINT('Ctrl Pts',(45.257059534438,-56.5804307205505,0.));
#124885=CARTESIAN_POINT('Ctrl Pts',(45.2495033575,-56.5567813613756,0.));
#124886=CARTESIAN_POINT('Ctrl Pts',(45.2419368816429,-56.5331779009958,
0.));
#124887=CARTESIAN_POINT('Ctrl Pts',(45.2343601950228,-56.5096204272306,
0.));
#124888=CARTESIAN_POINT('Ctrl Pts',(45.2267733862049,-56.4861090281823,
0.));
#124889=CARTESIAN_POINT('Ctrl Pts',(45.2191765441667,-56.4626437922386,
0.));
#124890=CARTESIAN_POINT('Ctrl Pts',(45.2115697583001,-56.4392248080732,
0.));
#124891=CARTESIAN_POINT('Ctrl Pts',(45.2039531184172,-56.4158521646411,
0.));
#124892=CARTESIAN_POINT('Ctrl Pts',(45.1963267147529,-56.3925259511806,
0.));
#124893=CARTESIAN_POINT('Ctrl Pts',(45.1886906379667,-56.3692462572231,
0.));
#124894=CARTESIAN_POINT('Ctrl Pts',(45.1810449791453,-56.3460131725964,
0.));
#124895=CARTESIAN_POINT('Ctrl Pts',(45.1733898298061,-56.3228267874264,
0.));
#124896=CARTESIAN_POINT('Ctrl Pts',(45.1657252819013,-56.2996871921316,
0.));
#124897=CARTESIAN_POINT('Ctrl Pts',(45.1580514278223,-56.2765944774245,
0.));
#124898=CARTESIAN_POINT('Ctrl Pts',(45.1503683604005,-56.2535487343221,
0.));
#124899=CARTESIAN_POINT('Ctrl Pts',(45.1426761729105,-56.2305500541489,
0.));
#124900=CARTESIAN_POINT('Ctrl Pts',(45.1349749590738,-56.2075985285393,
0.));
#124901=CARTESIAN_POINT('Ctrl Pts',(45.127264813063,-56.1846942494325,0.));
#124902=CARTESIAN_POINT('Ctrl Pts',(45.1195458295063,-56.1618373090732,
0.));
#124903=CARTESIAN_POINT('Ctrl Pts',(45.1118181034888,-56.1390278000226,
0.));
#124904=CARTESIAN_POINT('Ctrl Pts',(45.1040817305561,-56.116265815162,0.));
#124905=CARTESIAN_POINT('Ctrl Pts',(45.0963368067177,-56.0935514476945,
0.));
#124906=CARTESIAN_POINT('Ctrl Pts',(45.0885834284517,-56.0708847911416,
0.));
#124907=CARTESIAN_POINT('Ctrl Pts',(45.0808216927089,-56.048265939342,0.));
#124908=CARTESIAN_POINT('Ctrl Pts',(45.0730516969149,-56.0256949864639,
0.));
#124909=CARTESIAN_POINT('Ctrl Pts',(45.0652735389733,-56.003172027008,0.));
#124910=CARTESIAN_POINT('Ctrl Pts',(45.0574873172695,-55.9806971558097,
0.));
#124911=CARTESIAN_POINT('Ctrl Pts',(45.0496931306755,-55.9582704680356,
0.));
#124912=CARTESIAN_POINT('Ctrl Pts',(45.0418910785551,-55.9358920591837,
0.));
#124913=CARTESIAN_POINT('Ctrl Pts',(45.0340812607657,-55.9135620250954,
0.));
#124914=CARTESIAN_POINT('Ctrl Pts',(45.0262637776615,-55.8912804619577,
0.));
#124915=CARTESIAN_POINT('Ctrl Pts',(45.0184387300973,-55.8690474663065,
0.));
#124916=CARTESIAN_POINT('Ctrl Pts',(45.0106062194342,-55.8468631350218,
0.));
#124917=CARTESIAN_POINT('Ctrl Pts',(45.0027663475433,-55.8247275653289,
0.));
#124918=CARTESIAN_POINT('Ctrl Pts',(44.9949192168093,-55.8026408548105,
0.));
#124919=CARTESIAN_POINT('Ctrl Pts',(44.9870649301342,-55.7806031014106,
0.));
#124920=CARTESIAN_POINT('Ctrl Pts',(44.9792035909413,-55.7586144034367,
0.));
#124921=CARTESIAN_POINT('Ctrl Pts',(44.9713353031804,-55.7366748595551,
0.));
#124922=CARTESIAN_POINT('Ctrl Pts',(44.9634601713321,-55.714784568793,0.));
#124923=CARTESIAN_POINT('Ctrl Pts',(44.9555783004106,-55.6929436305489,
0.));
#124924=CARTESIAN_POINT('Ctrl Pts',(44.9476897959685,-55.6711521445979,
0.));
#124925=CARTESIAN_POINT('Ctrl Pts',(44.9397947641007,-55.6494102110935,
0.));
#124926=CARTESIAN_POINT('Ctrl Pts',(44.9318933114507,-55.6277179305633,
0.));
#124927=CARTESIAN_POINT('Ctrl Pts',(44.9239855452144,-55.6060754039121,
0.));
#124928=CARTESIAN_POINT('Ctrl Pts',(44.9160715731443,-55.5844827324338,
0.));
#124929=CARTESIAN_POINT('Ctrl Pts',(44.908151503553,-55.5629400178142,0.));
#124930=CARTESIAN_POINT('Ctrl Pts',(44.9002254453183,-55.541447362134,0.));
#124931=CARTESIAN_POINT('Ctrl Pts',(44.8922935078889,-55.5200048678629,
0.));
#124932=CARTESIAN_POINT('Ctrl Pts',(44.8843558012886,-55.4986126378656,
0.));
#124933=CARTESIAN_POINT('Ctrl Pts',(44.8764124361207,-55.4772707754126,
0.));
#124934=CARTESIAN_POINT('Ctrl Pts',(44.8684635235725,-55.4559793841836,
0.));
#124935=CARTESIAN_POINT('Ctrl Pts',(44.8605091754214,-55.4347385682704,
0.));
#124936=CARTESIAN_POINT('Ctrl Pts',(44.8525495040408,-55.4135484321718,
0.));
#124937=CARTESIAN_POINT('Ctrl Pts',(44.8445846224044,-55.3924090808014,
0.));
#124938=CARTESIAN_POINT('Ctrl Pts',(44.8366146440901,-55.3713206194967,
0.));
#124939=CARTESIAN_POINT('Ctrl Pts',(44.8286396832848,-55.3502831540228,
0.));
#124940=CARTESIAN_POINT('Ctrl Pts',(44.8206598547888,-55.3292967905725,
0.));
#124941=CARTESIAN_POINT('Ctrl Pts',(44.8126752740208,-55.3083616357605,
0.));
#124942=CARTESIAN_POINT('Ctrl Pts',(44.8046860570244,-55.287477796635,0.));
#124943=CARTESIAN_POINT('Ctrl Pts',(44.796692320474,-55.2666453806883,0.));
#124944=CARTESIAN_POINT('Ctrl Pts',(44.7886941816823,-55.2458644958617,
0.));
#124945=CARTESIAN_POINT('Ctrl Pts',(44.7806917586077,-55.2251352505474,
0.));
#124946=CARTESIAN_POINT('Ctrl Pts',(44.7726851698618,-55.2044577535865,
0.));
#124947=CARTESIAN_POINT('Ctrl Pts',(44.7646745347108,-55.1838321142777,
0.));
#124948=CARTESIAN_POINT('Ctrl Pts',(44.7566599730771,-55.1632584423813,
0.));
#124949=CARTESIAN_POINT('Ctrl Pts',(44.748641605542,-55.1427368481201,0.));
#124950=CARTESIAN_POINT('Ctrl Pts',(44.7406195533483,-55.1222674421747,
0.));
#124951=CARTESIAN_POINT('Ctrl Pts',(44.7325939384042,-55.1018503356806,
0.));
#124952=CARTESIAN_POINT('Ctrl Pts',(44.7245648832988,-55.0814856402507,
0.));
#124953=CARTESIAN_POINT('Ctrl Pts',(44.7165325113165,-55.0611734679902,
0.));
#124954=CARTESIAN_POINT('Ctrl Pts',(44.7084969464509,-55.0409139315074,
0.));
#124955=CARTESIAN_POINT('Ctrl Pts',(44.7004583134235,-55.020707143922,0.));
#124956=CARTESIAN_POINT('Ctrl Pts',(44.6924167376851,-55.0005532188644,
0.));
#124957=CARTESIAN_POINT('Ctrl Pts',(44.6843723453985,-54.9804522704668,
0.));
#124958=CARTESIAN_POINT('Ctrl Pts',(44.6763252634255,-54.9604044133497,
0.));
#124959=CARTESIAN_POINT('Ctrl Pts',(44.6682756193156,-54.9404097626088,
0.));
#124960=CARTESIAN_POINT('Ctrl Pts',(44.6602235412854,-54.9204684337845,
0.));
#124961=CARTESIAN_POINT('Ctrl Pts',(44.6521691582551,-54.9005805428991,
0.));
#124962=CARTESIAN_POINT('Ctrl Pts',(44.6441125999074,-54.8807462065177,
0.));
#124963=CARTESIAN_POINT('Ctrl Pts',(44.6360539967392,-54.860965541796,0.));
#124964=CARTESIAN_POINT('Ctrl Pts',(44.6279934801159,-54.8412386665264,
0.));
#124965=CARTESIAN_POINT('Ctrl Pts',(44.6199311823276,-54.8215656991817,
0.));
#124966=CARTESIAN_POINT('Ctrl Pts',(44.6118672364889,-54.8019467588257,
0.));
#124967=CARTESIAN_POINT('Ctrl Pts',(44.60380177643,-54.7823819650137,0.));
#124968=CARTESIAN_POINT('Ctrl Pts',(44.5957349366062,-54.7628714377041,
0.));
#124969=CARTESIAN_POINT('Ctrl Pts',(44.5876668519676,-54.7434152971285,
0.));
#124970=CARTESIAN_POINT('Ctrl Pts',(44.5795976579476,-54.7240136637744,
0.));
#124971=CARTESIAN_POINT('Ctrl Pts',(44.5715274907637,-54.7046666586776,
0.));
#124972=CARTESIAN_POINT('Ctrl Pts',(44.563456487687,-54.685374403676,0.));
#124973=CARTESIAN_POINT('Ctrl Pts',(44.5553847872712,-54.6661370216242,
0.));
#124974=CARTESIAN_POINT('Ctrl Pts',(44.5473125297289,-54.6469546367381,
0.));
#124975=CARTESIAN_POINT('Ctrl Pts',(44.5392398566775,-54.6278273743554,
0.));
#124976=CARTESIAN_POINT('Ctrl Pts',(44.5311669104495,-54.6087553602889,
0.));
#124977=CARTESIAN_POINT('Ctrl Pts',(44.5230938335165,-54.5897387202812,
0.));
#124978=CARTESIAN_POINT('Ctrl Pts',(44.5150207679007,-54.5707775794436,
0.));
#124979=CARTESIAN_POINT('Ctrl Pts',(44.5069478544977,-54.5518720616056,
0.));
#124980=CARTESIAN_POINT('Ctrl Pts',(44.4988752343744,-54.5330222905475,
0.));
#124981=CARTESIAN_POINT('Ctrl Pts',(44.4908030503225,-54.5142283914704,
0.));
#124982=CARTESIAN_POINT('Ctrl Pts',(44.4827314481264,-54.495490492193,0.));
#124983=CARTESIAN_POINT('Ctrl Pts',(44.4746605784031,-54.4768087248824,
0.));
#124984=CARTESIAN_POINT('Ctrl Pts',(44.4665905967668,-54.4581832262033,
0.));
#124985=CARTESIAN_POINT('Ctrl Pts',(44.4585216599908,-54.4396141336978,
0.));
#124986=CARTESIAN_POINT('Ctrl Pts',(44.4504539226328,-54.421101582595,0.));
#124987=CARTESIAN_POINT('Ctrl Pts',(44.4423875340996,-54.4026457030335,
0.));
#124988=CARTESIAN_POINT('Ctrl Pts',(44.4343226339593,-54.3842466156196,
0.));
#124989=CARTESIAN_POINT('Ctrl Pts',(44.4262593564712,-54.3659044357119,
0.));
#124990=CARTESIAN_POINT('Ctrl Pts',(44.4181978395851,-54.3476192819352,
0.));
#124991=CARTESIAN_POINT('Ctrl Pts',(44.4101382321834,-54.3293912830237,
0.));
#124992=CARTESIAN_POINT('Ctrl Pts',(44.402080702809,-54.3112205860716,0.));
#124993=CARTESIAN_POINT('Ctrl Pts',(44.3940254456331,-54.2931073621553,
0.));
#124994=CARTESIAN_POINT('Ctrl Pts',(44.3859726620183,-54.2750517888579,
0.));
#124995=CARTESIAN_POINT('Ctrl Pts',(44.3779225430406,-54.2570540336475,
0.));
#124996=CARTESIAN_POINT('Ctrl Pts',(44.3698752533562,-54.2391142386412,
0.));
#124997=CARTESIAN_POINT('Ctrl Pts',(44.361830910343,-54.2212325006052,0.));
#124998=CARTESIAN_POINT('Ctrl Pts',(44.3537895824096,-54.2034088701928,
0.));
#124999=CARTESIAN_POINT('Ctrl Pts',(44.3473589597726,-54.1891964684727,
0.));
#125000=CARTESIAN_POINT('Ctrl Pts',(44.3425373700993,-54.1785633257639,
0.));
#125001=CARTESIAN_POINT('Ctrl Pts',(44.3393235891075,-54.1714861895346,
0.));
#125002=CARTESIAN_POINT('Ctrl Pts',(44.3377168516418,-54.1679505278134,
0.));
#125003=CARTESIAN_POINT('Ctrl Pts',(40.554341280847,-62.494763006804,0.));
#125004=CARTESIAN_POINT('Ctrl Pts',(40.554341280847,-62.494763006804,12.));
#125005=CARTESIAN_POINT('Ctrl Pts',(40.5535399497519,-62.489224912198,0.));
#125006=CARTESIAN_POINT('Ctrl Pts',(40.5535399497519,-62.489224912198,12.));
#125007=CARTESIAN_POINT('Ctrl Pts',(40.5519353177252,-62.4781525156318,
0.));
#125008=CARTESIAN_POINT('Ctrl Pts',(40.5519353177252,-62.4781525156318,
12.));
#125009=CARTESIAN_POINT('Ctrl Pts',(40.5495224601758,-62.4615552987202,
0.));
#125010=CARTESIAN_POINT('Ctrl Pts',(40.5495224601758,-62.4615552987202,
12.));
#125011=CARTESIAN_POINT('Ctrl Pts',(40.5462934972718,-62.4394484329678,
0.));
#125012=CARTESIAN_POINT('Ctrl Pts',(40.5462934972718,-62.4394484329678,
12.));
#125013=CARTESIAN_POINT('Ctrl Pts',(40.5422375945026,-62.4118527881148,
0.));
#125014=CARTESIAN_POINT('Ctrl Pts',(40.5422375945026,-62.4118527881148,
12.));
#125015=CARTESIAN_POINT('Ctrl Pts',(40.5381619974169,-62.3842950992832,
0.));
#125016=CARTESIAN_POINT('Ctrl Pts',(40.5381619974169,-62.3842950992832,
12.));
#125017=CARTESIAN_POINT('Ctrl Pts',(40.5340667194319,-62.3567753970279,
0.));
#125018=CARTESIAN_POINT('Ctrl Pts',(40.5340667194319,-62.3567753970279,
12.));
#125019=CARTESIAN_POINT('Ctrl Pts',(40.5299517857721,-62.3292937257901,
0.));
#125020=CARTESIAN_POINT('Ctrl Pts',(40.5299517857721,-62.3292937257901,
12.));
#125021=CARTESIAN_POINT('Ctrl Pts',(40.5258172381429,-62.301850147165,0.));
#125022=CARTESIAN_POINT('Ctrl Pts',(40.5258172381429,-62.301850147165,12.));
#125023=CARTESIAN_POINT('Ctrl Pts',(40.5216631336193,-62.2744447381971,
0.));
#125024=CARTESIAN_POINT('Ctrl Pts',(40.5216631336193,-62.2744447381971,
12.));
#125025=CARTESIAN_POINT('Ctrl Pts',(40.5174895390954,-62.247077585866,0.));
#125026=CARTESIAN_POINT('Ctrl Pts',(40.5174895390954,-62.247077585866,12.));
#125027=CARTESIAN_POINT('Ctrl Pts',(40.5132965269633,-62.2197487826136,
0.));
#125028=CARTESIAN_POINT('Ctrl Pts',(40.5132965269633,-62.2197487826136,
12.));
#125029=CARTESIAN_POINT('Ctrl Pts',(40.5090841704122,-62.1924584215653,
0.));
#125030=CARTESIAN_POINT('Ctrl Pts',(40.5090841704122,-62.1924584215653,
12.));
#125031=CARTESIAN_POINT('Ctrl Pts',(40.5048525386035,-62.1652065915808,
0.));
#125032=CARTESIAN_POINT('Ctrl Pts',(40.5048525386035,-62.1652065915808,
12.));
#125033=CARTESIAN_POINT('Ctrl Pts',(40.5006016927554,-62.1379933732528,
0.));
#125034=CARTESIAN_POINT('Ctrl Pts',(40.5006016927554,-62.1379933732528,
12.));
#125035=CARTESIAN_POINT('Ctrl Pts',(40.4963316888412,-62.1108188417003,
0.));
#125036=CARTESIAN_POINT('Ctrl Pts',(40.4963316888412,-62.1108188417003,
12.));
#125037=CARTESIAN_POINT('Ctrl Pts',(40.4920425795217,-62.0836830685719,
0.));
#125038=CARTESIAN_POINT('Ctrl Pts',(40.4920425795217,-62.0836830685719,
12.));
#125039=CARTESIAN_POINT('Ctrl Pts',(40.4877344164411,-62.0565861244178,
0.));
#125040=CARTESIAN_POINT('Ctrl Pts',(40.4877344164411,-62.0565861244178,
12.));
#125041=CARTESIAN_POINT('Ctrl Pts',(40.4834072522164,-62.029528080742,0.));
#125042=CARTESIAN_POINT('Ctrl Pts',(40.4834072522164,-62.029528080742,12.));
#125043=CARTESIAN_POINT('Ctrl Pts',(40.4790611429584,-62.0025090125959,
0.));
#125044=CARTESIAN_POINT('Ctrl Pts',(40.4790611429584,-62.0025090125959,
12.));
#125045=CARTESIAN_POINT('Ctrl Pts',(40.4746961480015,-61.9755289983044,
0.));
#125046=CARTESIAN_POINT('Ctrl Pts',(40.4746961480015,-61.9755289983044,
12.));
#125047=CARTESIAN_POINT('Ctrl Pts',(40.4703123287621,-61.9485881182921,
0.));
#125048=CARTESIAN_POINT('Ctrl Pts',(40.4703123287621,-61.9485881182921,
12.));
#125049=CARTESIAN_POINT('Ctrl Pts',(40.4659097478587,-61.9216864541744,
0.));
#125050=CARTESIAN_POINT('Ctrl Pts',(40.4659097478587,-61.9216864541744,
12.));
#125051=CARTESIAN_POINT('Ctrl Pts',(40.4614884681889,-61.8948240878007,
0.));
#125052=CARTESIAN_POINT('Ctrl Pts',(40.4614884681889,-61.8948240878007,
12.));
#125053=CARTESIAN_POINT('Ctrl Pts',(40.457048551875,-61.8680011001537,0.));
#125054=CARTESIAN_POINT('Ctrl Pts',(40.457048551875,-61.8680011001537,12.));
#125055=CARTESIAN_POINT('Ctrl Pts',(40.4525900597894,-61.8412175708552,
0.));
#125056=CARTESIAN_POINT('Ctrl Pts',(40.4525900597894,-61.8412175708552,
12.));
#125057=CARTESIAN_POINT('Ctrl Pts',(40.4481130521364,-61.814473578779,0.));
#125058=CARTESIAN_POINT('Ctrl Pts',(40.4481130521364,-61.814473578779,12.));
#125059=CARTESIAN_POINT('Ctrl Pts',(40.443617588795,-61.7877692024076,0.));
#125060=CARTESIAN_POINT('Ctrl Pts',(40.443617588795,-61.7877692024076,12.));
#125061=CARTESIAN_POINT('Ctrl Pts',(40.4391037297589,-61.7611045202874,
0.));
#125062=CARTESIAN_POINT('Ctrl Pts',(40.4391037297589,-61.7611045202874,
12.));
#125063=CARTESIAN_POINT('Ctrl Pts',(40.4345715355405,-61.7344796114399,
0.));
#125064=CARTESIAN_POINT('Ctrl Pts',(40.4345715355405,-61.7344796114399,
12.));
#125065=CARTESIAN_POINT('Ctrl Pts',(40.430021067584,-61.7078945557799,0.));
#125066=CARTESIAN_POINT('Ctrl Pts',(40.430021067584,-61.7078945557799,12.));
#125067=CARTESIAN_POINT('Ctrl Pts',(40.425452388076,-61.6813494339286,0.));
#125068=CARTESIAN_POINT('Ctrl Pts',(40.425452388076,-61.6813494339286,12.));
#125069=CARTESIAN_POINT('Ctrl Pts',(40.4208655597717,-61.6548443270394,
0.));
#125070=CARTESIAN_POINT('Ctrl Pts',(40.4208655597717,-61.6548443270394,
12.));
#125071=CARTESIAN_POINT('Ctrl Pts',(40.4162606458119,-61.6283793166079,
0.));
#125072=CARTESIAN_POINT('Ctrl Pts',(40.4162606458119,-61.6283793166079,
12.));
#125073=CARTESIAN_POINT('Ctrl Pts',(40.4116377095596,-61.601954484301,0.));
#125074=CARTESIAN_POINT('Ctrl Pts',(40.4116377095596,-61.601954484301,12.));
#125075=CARTESIAN_POINT('Ctrl Pts',(40.4069968143956,-61.5755699117324,
0.));
#125076=CARTESIAN_POINT('Ctrl Pts',(40.4069968143956,-61.5755699117324,
12.));
#125077=CARTESIAN_POINT('Ctrl Pts',(40.4023380237232,-61.5492256804717,
0.));
#125078=CARTESIAN_POINT('Ctrl Pts',(40.4023380237232,-61.5492256804717,
12.));
#125079=CARTESIAN_POINT('Ctrl Pts',(40.3976614010653,-61.522921872154,0.));
#125080=CARTESIAN_POINT('Ctrl Pts',(40.3976614010653,-61.522921872154,12.));
#125081=CARTESIAN_POINT('Ctrl Pts',(40.3929670101366,-61.4966585685549,
0.));
#125082=CARTESIAN_POINT('Ctrl Pts',(40.3929670101366,-61.4966585685549,
12.));
#125083=CARTESIAN_POINT('Ctrl Pts',(40.3882549149228,-61.4704358516709,
0.));
#125084=CARTESIAN_POINT('Ctrl Pts',(40.3882549149228,-61.4704358516709,
12.));
#125085=CARTESIAN_POINT('Ctrl Pts',(40.383525179772,-61.4442538038044,0.));
#125086=CARTESIAN_POINT('Ctrl Pts',(40.383525179772,-61.4442538038044,12.));
#125087=CARTESIAN_POINT('Ctrl Pts',(40.3787778694364,-61.4181125076037,
0.));
#125088=CARTESIAN_POINT('Ctrl Pts',(40.3787778694364,-61.4181125076037,
12.));
#125089=CARTESIAN_POINT('Ctrl Pts',(40.3740130490225,-61.3920120460219,
0.));
#125090=CARTESIAN_POINT('Ctrl Pts',(40.3740130490225,-61.3920120460219,
12.));
#125091=CARTESIAN_POINT('Ctrl Pts',(40.3692307839636,-61.3659525022908,
0.));
#125092=CARTESIAN_POINT('Ctrl Pts',(40.3692307839636,-61.3659525022908,
12.));
#125093=CARTESIAN_POINT('Ctrl Pts',(40.3644311399861,-61.3399339598853,
0.));
#125094=CARTESIAN_POINT('Ctrl Pts',(40.3644311399861,-61.3399339598853,
12.));
#125095=CARTESIAN_POINT('Ctrl Pts',(40.3596141830791,-61.3139565024847,
0.));
#125096=CARTESIAN_POINT('Ctrl Pts',(40.3596141830791,-61.3139565024847,
12.));
#125097=CARTESIAN_POINT('Ctrl Pts',(40.3547799794679,-61.2880202139371,
0.));
#125098=CARTESIAN_POINT('Ctrl Pts',(40.3547799794679,-61.2880202139371,
12.));
#125099=CARTESIAN_POINT('Ctrl Pts',(40.3499285956304,-61.2621251782863,
0.));
#125100=CARTESIAN_POINT('Ctrl Pts',(40.3499285956304,-61.2621251782863,
12.));
#125101=CARTESIAN_POINT('Ctrl Pts',(40.3450600983109,-61.2362714797899,
0.));
#125102=CARTESIAN_POINT('Ctrl Pts',(40.3450600983109,-61.2362714797899,
12.));
#125103=CARTESIAN_POINT('Ctrl Pts',(40.340174554537,-61.2104592029377,0.));
#125104=CARTESIAN_POINT('Ctrl Pts',(40.340174554537,-61.2104592029377,12.));
#125105=CARTESIAN_POINT('Ctrl Pts',(40.335272031637,-61.1846884324643,0.));
#125106=CARTESIAN_POINT('Ctrl Pts',(40.335272031637,-61.1846884324643,12.));
#125107=CARTESIAN_POINT('Ctrl Pts',(40.3303525972616,-61.1589592533613,
0.));
#125108=CARTESIAN_POINT('Ctrl Pts',(40.3303525972616,-61.1589592533613,
12.));
#125109=CARTESIAN_POINT('Ctrl Pts',(40.32541631938,-61.1332717508789,0.));
#125110=CARTESIAN_POINT('Ctrl Pts',(40.32541631938,-61.1332717508789,12.));
#125111=CARTESIAN_POINT('Ctrl Pts',(40.3204632662726,-61.1076260105258,
0.));
#125112=CARTESIAN_POINT('Ctrl Pts',(40.3204632662726,-61.1076260105258,
12.));
#125113=CARTESIAN_POINT('Ctrl Pts',(40.3154935065262,-61.0820221180645,
0.));
#125114=CARTESIAN_POINT('Ctrl Pts',(40.3154935065262,-61.0820221180645,
12.));
#125115=CARTESIAN_POINT('Ctrl Pts',(40.310507109031,-61.056460159505,0.));
#125116=CARTESIAN_POINT('Ctrl Pts',(40.310507109031,-61.056460159505,12.));
#125117=CARTESIAN_POINT('Ctrl Pts',(40.3055041429775,-61.0309402210921,
0.));
#125118=CARTESIAN_POINT('Ctrl Pts',(40.3055041429775,-61.0309402210921,
12.));
#125119=CARTESIAN_POINT('Ctrl Pts',(40.300484677858,-61.0054623893066,0.));
#125120=CARTESIAN_POINT('Ctrl Pts',(40.300484677858,-61.0054623893066,12.));
#125121=CARTESIAN_POINT('Ctrl Pts',(40.295448783469,-60.9800267508786,0.));
#125122=CARTESIAN_POINT('Ctrl Pts',(40.295448783469,-60.9800267508786,12.));
#125123=CARTESIAN_POINT('Ctrl Pts',(40.2903965299155,-60.954633392792,0.));
#125124=CARTESIAN_POINT('Ctrl Pts',(40.2903965299155,-60.954633392792,12.));
#125125=CARTESIAN_POINT('Ctrl Pts',(40.2853279876161,-60.9292824022887,
0.));
#125126=CARTESIAN_POINT('Ctrl Pts',(40.2853279876161,-60.9292824022887,
12.));
#125127=CARTESIAN_POINT('Ctrl Pts',(40.2802432273105,-60.9039738668668,
0.));
#125128=CARTESIAN_POINT('Ctrl Pts',(40.2802432273105,-60.9039738668668,
12.));
#125129=CARTESIAN_POINT('Ctrl Pts',(40.2751423200639,-60.8787078742818,
0.));
#125130=CARTESIAN_POINT('Ctrl Pts',(40.2751423200639,-60.8787078742818,
12.));
#125131=CARTESIAN_POINT('Ctrl Pts',(40.2700253372648,-60.8534845125538,
0.));
#125132=CARTESIAN_POINT('Ctrl Pts',(40.2700253372648,-60.8534845125538,
12.));
#125133=CARTESIAN_POINT('Ctrl Pts',(40.2648923506248,-60.8283038699706,
0.));
#125134=CARTESIAN_POINT('Ctrl Pts',(40.2648923506248,-60.8283038699706,
12.));
#125135=CARTESIAN_POINT('Ctrl Pts',(40.2597434321803,-60.8031660350879,
0.));
#125136=CARTESIAN_POINT('Ctrl Pts',(40.2597434321803,-60.8031660350879,
12.));
#125137=CARTESIAN_POINT('Ctrl Pts',(40.2545786542953,-60.7780710967248,
0.));
#125138=CARTESIAN_POINT('Ctrl Pts',(40.2545786542953,-60.7780710967248,
12.));
#125139=CARTESIAN_POINT('Ctrl Pts',(40.2493980896638,-60.7530191439593,
0.));
#125140=CARTESIAN_POINT('Ctrl Pts',(40.2493980896638,-60.7530191439593,
12.));
#125141=CARTESIAN_POINT('Ctrl Pts',(40.2442018113108,-60.728010266139,0.));
#125142=CARTESIAN_POINT('Ctrl Pts',(40.2442018113108,-60.728010266139,12.));
#125143=CARTESIAN_POINT('Ctrl Pts',(40.2389898925932,-60.7030445528857,
0.));
#125144=CARTESIAN_POINT('Ctrl Pts',(40.2389898925932,-60.7030445528857,
12.));
#125145=CARTESIAN_POINT('Ctrl Pts',(40.2337624072029,-60.678122094098,0.));
#125146=CARTESIAN_POINT('Ctrl Pts',(40.2337624072029,-60.678122094098,12.));
#125147=CARTESIAN_POINT('Ctrl Pts',(40.2285194291706,-60.6532429799499,
0.));
#125148=CARTESIAN_POINT('Ctrl Pts',(40.2285194291706,-60.6532429799499,
12.));
#125149=CARTESIAN_POINT('Ctrl Pts',(40.2232610328721,-60.6284073008871,
0.));
#125150=CARTESIAN_POINT('Ctrl Pts',(40.2232610328721,-60.6284073008871,
12.));
#125151=CARTESIAN_POINT('Ctrl Pts',(40.2179872930273,-60.6036151476349,
0.));
#125152=CARTESIAN_POINT('Ctrl Pts',(40.2179872930273,-60.6036151476349,
12.));
#125153=CARTESIAN_POINT('Ctrl Pts',(40.2126982847011,-60.5788666112042,
0.));
#125154=CARTESIAN_POINT('Ctrl Pts',(40.2126982847011,-60.5788666112042,
12.));
#125155=CARTESIAN_POINT('Ctrl Pts',(40.2073940833053,-60.5541617828925,
0.));
#125156=CARTESIAN_POINT('Ctrl Pts',(40.2073940833053,-60.5541617828925,
12.));
#125157=CARTESIAN_POINT('Ctrl Pts',(40.2020747646014,-60.5295007542841,
0.));
#125158=CARTESIAN_POINT('Ctrl Pts',(40.2020747646014,-60.5295007542841,
12.));
#125159=CARTESIAN_POINT('Ctrl Pts',(40.1967404047062,-60.5048836172435,
0.));
#125160=CARTESIAN_POINT('Ctrl Pts',(40.1967404047062,-60.5048836172435,
12.));
#125161=CARTESIAN_POINT('Ctrl Pts',(40.1913910800921,-60.4803104639225,
0.));
#125162=CARTESIAN_POINT('Ctrl Pts',(40.1913910800921,-60.4803104639225,
12.));
#125163=CARTESIAN_POINT('Ctrl Pts',(40.1860268675884,-60.455781386769,0.));
#125164=CARTESIAN_POINT('Ctrl Pts',(40.1860268675884,-60.455781386769,12.));
#125165=CARTESIAN_POINT('Ctrl Pts',(40.180647844383,-60.4312964785273,0.));
#125166=CARTESIAN_POINT('Ctrl Pts',(40.180647844383,-60.4312964785273,12.));
#125167=CARTESIAN_POINT('Ctrl Pts',(40.1752540880268,-60.4068558322407,
0.));
#125168=CARTESIAN_POINT('Ctrl Pts',(40.1752540880268,-60.4068558322407,
12.));
#125169=CARTESIAN_POINT('Ctrl Pts',(40.1698456764377,-60.3824595412445,
0.));
#125170=CARTESIAN_POINT('Ctrl Pts',(40.1698456764377,-60.3824595412445,
12.));
#125171=CARTESIAN_POINT('Ctrl Pts',(40.1644226879033,-60.3581076991716,
0.));
#125172=CARTESIAN_POINT('Ctrl Pts',(40.1644226879033,-60.3581076991716,
12.));
#125173=CARTESIAN_POINT('Ctrl Pts',(40.1589852010804,-60.3338003999606,
0.));
#125174=CARTESIAN_POINT('Ctrl Pts',(40.1589852010804,-60.3338003999606,
12.));
#125175=CARTESIAN_POINT('Ctrl Pts',(40.1535332949976,-60.3095377378586,
0.));
#125176=CARTESIAN_POINT('Ctrl Pts',(40.1535332949976,-60.3095377378586,
12.));
#125177=CARTESIAN_POINT('Ctrl Pts',(40.1480670490586,-60.285319807422,0.));
#125178=CARTESIAN_POINT('Ctrl Pts',(40.1480670490586,-60.285319807422,12.));
#125179=CARTESIAN_POINT('Ctrl Pts',(40.1425865430472,-60.2611467035116,
0.));
#125180=CARTESIAN_POINT('Ctrl Pts',(40.1425865430472,-60.2611467035116,
12.));
#125181=CARTESIAN_POINT('Ctrl Pts',(40.1370918571305,-60.2370185212964,
0.));
#125182=CARTESIAN_POINT('Ctrl Pts',(40.1370918571305,-60.2370185212964,
12.));
#125183=CARTESIAN_POINT('Ctrl Pts',(40.1315830718577,-60.2129353562622,
0.));
#125184=CARTESIAN_POINT('Ctrl Pts',(40.1315830718577,-60.2129353562622,
12.));
#125185=CARTESIAN_POINT('Ctrl Pts',(40.1260602681644,-60.1888973042152,
0.));
#125186=CARTESIAN_POINT('Ctrl Pts',(40.1260602681644,-60.1888973042152,
12.));
#125187=CARTESIAN_POINT('Ctrl Pts',(40.120523527374,-60.1649044612828,0.));
#125188=CARTESIAN_POINT('Ctrl Pts',(40.120523527374,-60.1649044612828,12.));
#125189=CARTESIAN_POINT('Ctrl Pts',(40.1149729312036,-60.1409569239092,
0.));
#125190=CARTESIAN_POINT('Ctrl Pts',(40.1149729312036,-60.1409569239092,
12.));
#125191=CARTESIAN_POINT('Ctrl Pts',(40.1094085617674,-60.1170547888574,
0.));
#125192=CARTESIAN_POINT('Ctrl Pts',(40.1094085617674,-60.1170547888574,
12.));
#125193=CARTESIAN_POINT('Ctrl Pts',(40.1038305015766,-60.0931981532197,
0.));
#125194=CARTESIAN_POINT('Ctrl Pts',(40.1038305015766,-60.0931981532197,
12.));
#125195=CARTESIAN_POINT('Ctrl Pts',(40.0982388335423,-60.069387114421,0.));
#125196=CARTESIAN_POINT('Ctrl Pts',(40.0982388335423,-60.069387114421,12.));
#125197=CARTESIAN_POINT('Ctrl Pts',(40.0926336409785,-60.0456217702201,
0.));
#125198=CARTESIAN_POINT('Ctrl Pts',(40.0926336409785,-60.0456217702201,
12.));
#125199=CARTESIAN_POINT('Ctrl Pts',(40.0870150076074,-60.021902218706,0.));
#125200=CARTESIAN_POINT('Ctrl Pts',(40.0870150076074,-60.021902218706,12.));
#125201=CARTESIAN_POINT('Ctrl Pts',(40.0813830175623,-59.9982285582983,
0.));
#125202=CARTESIAN_POINT('Ctrl Pts',(40.0813830175623,-59.9982285582983,
12.));
#125203=CARTESIAN_POINT('Ctrl Pts',(40.0757377553888,-59.9746008877584,
0.));
#125204=CARTESIAN_POINT('Ctrl Pts',(40.0757377553888,-59.9746008877584,
12.));
#125205=CARTESIAN_POINT('Ctrl Pts',(40.0700793060473,-59.9510193061927,
0.));
#125206=CARTESIAN_POINT('Ctrl Pts',(40.0700793060473,-59.9510193061927,
12.));
#125207=CARTESIAN_POINT('Ctrl Pts',(40.064407754916,-59.9274839130553,0.));
#125208=CARTESIAN_POINT('Ctrl Pts',(40.064407754916,-59.9274839130553,12.));
#125209=CARTESIAN_POINT('Ctrl Pts',(40.0587231877962,-59.9039948081432,
0.));
#125210=CARTESIAN_POINT('Ctrl Pts',(40.0587231877962,-59.9039948081432,
12.));
#125211=CARTESIAN_POINT('Ctrl Pts',(40.0530256909162,-59.8805520915975,
0.));
#125212=CARTESIAN_POINT('Ctrl Pts',(40.0530256909162,-59.8805520915975,
12.));
#125213=CARTESIAN_POINT('Ctrl Pts',(40.0473153509323,-59.8571558639144,
0.));
#125214=CARTESIAN_POINT('Ctrl Pts',(40.0473153509323,-59.8571558639144,
12.));
#125215=CARTESIAN_POINT('Ctrl Pts',(40.0415922549313,-59.8338062259491,
0.));
#125216=CARTESIAN_POINT('Ctrl Pts',(40.0415922549313,-59.8338062259491,
12.));
#125217=CARTESIAN_POINT('Ctrl Pts',(40.035856490434,-59.8105032789179,0.));
#125218=CARTESIAN_POINT('Ctrl Pts',(40.035856490434,-59.8105032789179,12.));
#125219=CARTESIAN_POINT('Ctrl Pts',(40.0301081454006,-59.7872471243948,
0.));
#125220=CARTESIAN_POINT('Ctrl Pts',(40.0301081454006,-59.7872471243948,
12.));
#125221=CARTESIAN_POINT('Ctrl Pts',(40.0243473082343,-59.7640378643114,
0.));
#125222=CARTESIAN_POINT('Ctrl Pts',(40.0243473082343,-59.7640378643114,
12.));
#125223=CARTESIAN_POINT('Ctrl Pts',(40.0185740677827,-59.7408756009688,
0.));
#125224=CARTESIAN_POINT('Ctrl Pts',(40.0185740677827,-59.7408756009688,
12.));
#125225=CARTESIAN_POINT('Ctrl Pts',(40.0127885133407,-59.7177604370409,
0.));
#125226=CARTESIAN_POINT('Ctrl Pts',(40.0127885133407,-59.7177604370409,
12.));
#125227=CARTESIAN_POINT('Ctrl Pts',(40.0069907346536,-59.6946924755771,
0.));
#125228=CARTESIAN_POINT('Ctrl Pts',(40.0069907346536,-59.6946924755771,
12.));
#125229=CARTESIAN_POINT('Ctrl Pts',(40.0011808219231,-59.671671819999,0.));
#125230=CARTESIAN_POINT('Ctrl Pts',(40.0011808219231,-59.671671819999,12.));
#125231=CARTESIAN_POINT('Ctrl Pts',(39.9953588658115,-59.6486985741015,
0.));
#125232=CARTESIAN_POINT('Ctrl Pts',(39.9953588658115,-59.6486985741015,
12.));
#125233=CARTESIAN_POINT('Ctrl Pts',(39.9895249574432,-59.6257728420644,
0.));
#125234=CARTESIAN_POINT('Ctrl Pts',(39.9895249574432,-59.6257728420644,
12.));
#125235=CARTESIAN_POINT('Ctrl Pts',(39.9836791884072,-59.6028947284551,
0.));
#125236=CARTESIAN_POINT('Ctrl Pts',(39.9836791884072,-59.6028947284551,
12.));
#125237=CARTESIAN_POINT('Ctrl Pts',(39.9778216507609,-59.5800643382322,
0.));
#125238=CARTESIAN_POINT('Ctrl Pts',(39.9778216507609,-59.5800643382322,
12.));
#125239=CARTESIAN_POINT('Ctrl Pts',(39.971952437036,-59.5572817767412,0.));
#125240=CARTESIAN_POINT('Ctrl Pts',(39.971952437036,-59.5572817767412,12.));
#125241=CARTESIAN_POINT('Ctrl Pts',(39.9660716402423,-59.5345471497162,
0.));
#125242=CARTESIAN_POINT('Ctrl Pts',(39.9660716402423,-59.5345471497162,
12.));
#125243=CARTESIAN_POINT('Ctrl Pts',(39.96017935387,-59.5118605632919,0.));
#125244=CARTESIAN_POINT('Ctrl Pts',(39.96017935387,-59.5118605632919,12.));
#125245=CARTESIAN_POINT('Ctrl Pts',(39.954275671893,-59.4892221240081,0.));
#125246=CARTESIAN_POINT('Ctrl Pts',(39.954275671893,-59.4892221240081,12.));
#125247=CARTESIAN_POINT('Ctrl Pts',(39.9483606887731,-59.4666319388123,
0.));
#125248=CARTESIAN_POINT('Ctrl Pts',(39.9483606887731,-59.4666319388123,
12.));
#125249=CARTESIAN_POINT('Ctrl Pts',(39.9424344994652,-59.444090115055,0.));
#125250=CARTESIAN_POINT('Ctrl Pts',(39.9424344994652,-59.444090115055,12.));
#125251=CARTESIAN_POINT('Ctrl Pts',(39.9364971994215,-59.4215967604925,
0.));
#125252=CARTESIAN_POINT('Ctrl Pts',(39.9364971994215,-59.4215967604925,
12.));
#125253=CARTESIAN_POINT('Ctrl Pts',(39.9305488845934,-59.3991519832981,
0.));
#125254=CARTESIAN_POINT('Ctrl Pts',(39.9305488845934,-59.3991519832981,
12.));
#125255=CARTESIAN_POINT('Ctrl Pts',(39.9245896514359,-59.3767558920663,
0.));
#125256=CARTESIAN_POINT('Ctrl Pts',(39.9245896514359,-59.3767558920663,
12.));
#125257=CARTESIAN_POINT('Ctrl Pts',(39.9186195969113,-59.3544085958165,
0.));
#125258=CARTESIAN_POINT('Ctrl Pts',(39.9186195969113,-59.3544085958165,
12.));
#125259=CARTESIAN_POINT('Ctrl Pts',(39.9126388184956,-59.3321102039883,
0.));
#125260=CARTESIAN_POINT('Ctrl Pts',(39.9126388184956,-59.3321102039883,
12.));
#125261=CARTESIAN_POINT('Ctrl Pts',(39.9066474141826,-59.3098608264452,
0.));
#125262=CARTESIAN_POINT('Ctrl Pts',(39.9066474141826,-59.3098608264452,
12.));
#125263=CARTESIAN_POINT('Ctrl Pts',(39.9006454824861,-59.287660573487,0.));
#125264=CARTESIAN_POINT('Ctrl Pts',(39.9006454824861,-59.287660573487,12.));
#125265=CARTESIAN_POINT('Ctrl Pts',(39.8946331224442,-59.2655095558527,
0.));
#125266=CARTESIAN_POINT('Ctrl Pts',(39.8946331224442,-59.2655095558527,
12.));
#125267=CARTESIAN_POINT('Ctrl Pts',(39.8886104336234,-59.2434078847236,
0.));
#125268=CARTESIAN_POINT('Ctrl Pts',(39.8886104336234,-59.2434078847236,
12.));
#125269=CARTESIAN_POINT('Ctrl Pts',(39.8825775161253,-59.2213556717188,
0.));
#125270=CARTESIAN_POINT('Ctrl Pts',(39.8825775161253,-59.2213556717188,
12.));
#125271=CARTESIAN_POINT('Ctrl Pts',(39.8765344705895,-59.1993530289008,
0.));
#125272=CARTESIAN_POINT('Ctrl Pts',(39.8765344705895,-59.1993530289008,
12.));
#125273=CARTESIAN_POINT('Ctrl Pts',(39.8704813981978,-59.1774000687865,
0.));
#125274=CARTESIAN_POINT('Ctrl Pts',(39.8704813981978,-59.1774000687865,
12.));
#125275=CARTESIAN_POINT('Ctrl Pts',(39.8644184006785,-59.155496904352,0.));
#125276=CARTESIAN_POINT('Ctrl Pts',(39.8644184006785,-59.155496904352,12.));
#125277=CARTESIAN_POINT('Ctrl Pts',(39.8583455803111,-59.133643649035,0.));
#125278=CARTESIAN_POINT('Ctrl Pts',(39.8583455803111,-59.133643649035,12.));
#125279=CARTESIAN_POINT('Ctrl Pts',(39.8522630399337,-59.1118404167304,
0.));
#125280=CARTESIAN_POINT('Ctrl Pts',(39.8522630399337,-59.1118404167304,
12.));
#125281=CARTESIAN_POINT('Ctrl Pts',(39.8461708829465,-59.0900873217992,
0.));
#125282=CARTESIAN_POINT('Ctrl Pts',(39.8461708829465,-59.0900873217992,
12.));
#125283=CARTESIAN_POINT('Ctrl Pts',(39.8400692133143,-59.068384479077,0.));
#125284=CARTESIAN_POINT('Ctrl Pts',(39.8400692133143,-59.068384479077,12.));
#125285=CARTESIAN_POINT('Ctrl Pts',(39.8339581355715,-59.0467320038782,
0.));
#125286=CARTESIAN_POINT('Ctrl Pts',(39.8339581355715,-59.0467320038782,
12.));
#125287=CARTESIAN_POINT('Ctrl Pts',(39.8278377548261,-59.0251300119972,
0.));
#125288=CARTESIAN_POINT('Ctrl Pts',(39.8278377548261,-59.0251300119972,
12.));
#125289=CARTESIAN_POINT('Ctrl Pts',(39.8217081767658,-59.0035786197024,
0.));
#125290=CARTESIAN_POINT('Ctrl Pts',(39.8217081767658,-59.0035786197024,
12.));
#125291=CARTESIAN_POINT('Ctrl Pts',(39.8155695076625,-58.9820779437485,
0.));
#125292=CARTESIAN_POINT('Ctrl Pts',(39.8155695076625,-58.9820779437485,
12.));
#125293=CARTESIAN_POINT('Ctrl Pts',(39.8094218543781,-58.9606281013875,
0.));
#125294=CARTESIAN_POINT('Ctrl Pts',(39.8094218543781,-58.9606281013875,
12.));
#125295=CARTESIAN_POINT('Ctrl Pts',(39.8032653243712,-58.9392292103747,
0.));
#125296=CARTESIAN_POINT('Ctrl Pts',(39.8032653243712,-58.9392292103747,
12.));
#125297=CARTESIAN_POINT('Ctrl Pts',(39.7971000257044,-58.9178813889703,
0.));
#125298=CARTESIAN_POINT('Ctrl Pts',(39.7971000257044,-58.9178813889703,
12.));
#125299=CARTESIAN_POINT('Ctrl Pts',(39.7909260670517,-58.8965847559389,
0.));
#125300=CARTESIAN_POINT('Ctrl Pts',(39.7909260670517,-58.8965847559389,
12.));
#125301=CARTESIAN_POINT('Ctrl Pts',(39.7847435576996,-58.8753394305583,
0.));
#125302=CARTESIAN_POINT('Ctrl Pts',(39.7847435576996,-58.8753394305583,
12.));
#125303=CARTESIAN_POINT('Ctrl Pts',(39.7785526075477,-58.8541455326229,
0.));
#125304=CARTESIAN_POINT('Ctrl Pts',(39.7785526075477,-58.8541455326229,
12.));
#125305=CARTESIAN_POINT('Ctrl Pts',(39.772353327112,-58.8330031824453,0.));
#125306=CARTESIAN_POINT('Ctrl Pts',(39.772353327112,-58.8330031824453,12.));
#125307=CARTESIAN_POINT('Ctrl Pts',(39.7661458275276,-58.8119125008521,
0.));
#125308=CARTESIAN_POINT('Ctrl Pts',(39.7661458275276,-58.8119125008521,
12.));
#125309=CARTESIAN_POINT('Ctrl Pts',(39.7599302205527,-58.7908736091808,
0.));
#125310=CARTESIAN_POINT('Ctrl Pts',(39.7599302205527,-58.7908736091808,
12.));
#125311=CARTESIAN_POINT('Ctrl Pts',(39.753706618582,-58.769886629304,0.));
#125312=CARTESIAN_POINT('Ctrl Pts',(39.753706618582,-58.769886629304,12.));
#125313=CARTESIAN_POINT('Ctrl Pts',(39.7474751346603,-58.7489516836452,
0.));
#125314=CARTESIAN_POINT('Ctrl Pts',(39.7474751346603,-58.7489516836452,
12.));
#125315=CARTESIAN_POINT('Ctrl Pts',(39.741235882495,-58.7280688951911,0.));
#125316=CARTESIAN_POINT('Ctrl Pts',(39.741235882495,-58.7280688951911,12.));
#125317=CARTESIAN_POINT('Ctrl Pts',(39.7349889764737,-58.7072383875009,
0.));
#125318=CARTESIAN_POINT('Ctrl Pts',(39.7349889764737,-58.7072383875009,
12.));
#125319=CARTESIAN_POINT('Ctrl Pts',(39.7287345316664,-58.6864602847064,
0.));
#125320=CARTESIAN_POINT('Ctrl Pts',(39.7287345316664,-58.6864602847064,
12.));
#125321=CARTESIAN_POINT('Ctrl Pts',(39.7224726638087,-58.6657347115014,
0.));
#125322=CARTESIAN_POINT('Ctrl Pts',(39.7224726638087,-58.6657347115014,
12.));
#125323=CARTESIAN_POINT('Ctrl Pts',(39.7162034892896,-58.6450617931269,
0.));
#125324=CARTESIAN_POINT('Ctrl Pts',(39.7162034892896,-58.6450617931269,
12.));
#125325=CARTESIAN_POINT('Ctrl Pts',(39.7099271251421,-58.6244416553574,
0.));
#125326=CARTESIAN_POINT('Ctrl Pts',(39.7099271251421,-58.6244416553574,
12.));
#125327=CARTESIAN_POINT('Ctrl Pts',(39.7036436890248,-58.6038744244683,
0.));
#125328=CARTESIAN_POINT('Ctrl Pts',(39.7036436890248,-58.6038744244683,
12.));
#125329=CARTESIAN_POINT('Ctrl Pts',(39.6973532992555,-58.5833602272767,
0.));
#125330=CARTESIAN_POINT('Ctrl Pts',(39.6973532992555,-58.5833602272767,
12.));
#125331=CARTESIAN_POINT('Ctrl Pts',(39.6910560748639,-58.5628991912067,
0.));
#125332=CARTESIAN_POINT('Ctrl Pts',(39.6910560748639,-58.5628991912067,
12.));
#125333=CARTESIAN_POINT('Ctrl Pts',(39.6847521356395,-58.5424914443415,
0.));
#125334=CARTESIAN_POINT('Ctrl Pts',(39.6847521356395,-58.5424914443415,
12.));
#125335=CARTESIAN_POINT('Ctrl Pts',(39.6784416021817,-58.5221371154748,
0.));
#125336=CARTESIAN_POINT('Ctrl Pts',(39.6784416021817,-58.5221371154748,
12.));
#125337=CARTESIAN_POINT('Ctrl Pts',(39.6721245959516,-58.5018363341582,
0.));
#125338=CARTESIAN_POINT('Ctrl Pts',(39.6721245959516,-58.5018363341582,
12.));
#125339=CARTESIAN_POINT('Ctrl Pts',(39.66580123918,-58.4815892306044,0.));
#125340=CARTESIAN_POINT('Ctrl Pts',(39.66580123918,-58.4815892306044,12.));
#125341=CARTESIAN_POINT('Ctrl Pts',(39.6594716547681,-58.4613959355776,
0.));
#125342=CARTESIAN_POINT('Ctrl Pts',(39.6594716547681,-58.4613959355776,
12.));
#125343=CARTESIAN_POINT('Ctrl Pts',(39.6531359662043,-58.4412565802984,
0.));
#125344=CARTESIAN_POINT('Ctrl Pts',(39.6531359662043,-58.4412565802984,
12.));
#125345=CARTESIAN_POINT('Ctrl Pts',(39.6467942974465,-58.4211712963023,
0.));
#125346=CARTESIAN_POINT('Ctrl Pts',(39.6467942974465,-58.4211712963023,
12.));
#125347=CARTESIAN_POINT('Ctrl Pts',(39.6404467729114,-58.4011402154225,
0.));
#125348=CARTESIAN_POINT('Ctrl Pts',(39.6404467729114,-58.4011402154225,
12.));
#125349=CARTESIAN_POINT('Ctrl Pts',(39.6340935177492,-58.3811634701061,
0.));
#125350=CARTESIAN_POINT('Ctrl Pts',(39.6340935177492,-58.3811634701061,
12.));
#125351=CARTESIAN_POINT('Ctrl Pts',(39.6277346580898,-58.3612411936914,
0.));
#125352=CARTESIAN_POINT('Ctrl Pts',(39.6277346580898,-58.3612411936914,
12.));
#125353=CARTESIAN_POINT('Ctrl Pts',(39.6213703212523,-58.3413735206412,
0.));
#125354=CARTESIAN_POINT('Ctrl Pts',(39.6213703212523,-58.3413735206412,
12.));
#125355=CARTESIAN_POINT('Ctrl Pts',(39.6150006360894,-58.3215605869192,
0.));
#125356=CARTESIAN_POINT('Ctrl Pts',(39.6150006360894,-58.3215605869192,
12.));
#125357=CARTESIAN_POINT('Ctrl Pts',(39.6086257327559,-58.3018025297288,
0.));
#125358=CARTESIAN_POINT('Ctrl Pts',(39.6086257327559,-58.3018025297288,
12.));
#125359=CARTESIAN_POINT('Ctrl Pts',(39.6022457420772,-58.2820994868092,
0.));
#125360=CARTESIAN_POINT('Ctrl Pts',(39.6022457420772,-58.2820994868092,
12.));
#125361=CARTESIAN_POINT('Ctrl Pts',(39.5958607950237,-58.2624515958416,
0.));
#125362=CARTESIAN_POINT('Ctrl Pts',(39.5958607950237,-58.2624515958416,
12.));
#125363=CARTESIAN_POINT('Ctrl Pts',(39.589471022173,-58.2428589938394,0.));
#125364=CARTESIAN_POINT('Ctrl Pts',(39.589471022173,-58.2428589938394,12.));
#125365=CARTESIAN_POINT('Ctrl Pts',(39.5830765530919,-58.2233218164407,
0.));
#125366=CARTESIAN_POINT('Ctrl Pts',(39.5830765530919,-58.2233218164407,
12.));
#125367=CARTESIAN_POINT('Ctrl Pts',(39.5766775175226,-58.2038401992496,
0.));
#125368=CARTESIAN_POINT('Ctrl Pts',(39.5766775175226,-58.2038401992496,
12.));
#125369=CARTESIAN_POINT('Ctrl Pts',(39.5702740468013,-58.1844142794359,
0.));
#125370=CARTESIAN_POINT('Ctrl Pts',(39.5702740468013,-58.1844142794359,
12.));
#125371=CARTESIAN_POINT('Ctrl Pts',(39.5638662750174,-58.1650441970378,
0.));
#125372=CARTESIAN_POINT('Ctrl Pts',(39.5638662750174,-58.1650441970378,
12.));
#125373=CARTESIAN_POINT('Ctrl Pts',(39.5574543406959,-58.1457300968466,
0.));
#125374=CARTESIAN_POINT('Ctrl Pts',(39.5574543406959,-58.1457300968466,
12.));
#125375=CARTESIAN_POINT('Ctrl Pts',(39.5510383869476,-58.1264721285697,
0.));
#125376=CARTESIAN_POINT('Ctrl Pts',(39.5510383869476,-58.1264721285697,
12.));
#125377=CARTESIAN_POINT('Ctrl Pts',(39.5446185579615,-58.1072704428895,
0.));
#125378=CARTESIAN_POINT('Ctrl Pts',(39.5446185579615,-58.1072704428895,
12.));
#125379=CARTESIAN_POINT('Ctrl Pts',(39.5381949959214,-58.088125187991,0.));
#125380=CARTESIAN_POINT('Ctrl Pts',(39.5381949959214,-58.088125187991,12.));
#125381=CARTESIAN_POINT('Ctrl Pts',(39.5317678383231,-58.0690365065393,
0.));
#125382=CARTESIAN_POINT('Ctrl Pts',(39.5317678383231,-58.0690365065393,
12.));
#125383=CARTESIAN_POINT('Ctrl Pts',(39.5253372136921,-58.0500045308459,
0.));
#125384=CARTESIAN_POINT('Ctrl Pts',(39.5253372136921,-58.0500045308459,
12.));
#125385=CARTESIAN_POINT('Ctrl Pts',(39.5189032457227,-58.0310293875321,
0.));
#125386=CARTESIAN_POINT('Ctrl Pts',(39.5189032457227,-58.0310293875321,
12.));
#125387=CARTESIAN_POINT('Ctrl Pts',(39.5124660615009,-58.012111206794,0.));
#125388=CARTESIAN_POINT('Ctrl Pts',(39.5124660615009,-58.012111206794,12.));
#125389=CARTESIAN_POINT('Ctrl Pts',(39.5060257981225,-57.9932501298522,
0.));
#125390=CARTESIAN_POINT('Ctrl Pts',(39.5060257981225,-57.9932501298522,
12.));
#125391=CARTESIAN_POINT('Ctrl Pts',(39.4995826106692,-57.9744463179305,
0.));
#125392=CARTESIAN_POINT('Ctrl Pts',(39.4995826106692,-57.9744463179305,
12.));
#125393=CARTESIAN_POINT('Ctrl Pts',(39.4931366776628,-57.9556999583777,
0.));
#125394=CARTESIAN_POINT('Ctrl Pts',(39.4931366776628,-57.9556999583777,
12.));
#125395=CARTESIAN_POINT('Ctrl Pts',(39.4866881842223,-57.9370112456506,
0.));
#125396=CARTESIAN_POINT('Ctrl Pts',(39.4866881842223,-57.9370112456506,
12.));
#125397=CARTESIAN_POINT('Ctrl Pts',(39.4802373061008,-57.9183803632337,
0.));
#125398=CARTESIAN_POINT('Ctrl Pts',(39.4802373061008,-57.9183803632337,
12.));
#125399=CARTESIAN_POINT('Ctrl Pts',(39.4737841949417,-57.899807467054,0.));
#125400=CARTESIAN_POINT('Ctrl Pts',(39.4737841949417,-57.899807467054,12.));
#125401=CARTESIAN_POINT('Ctrl Pts',(39.4673289592425,-57.8812926637397,
0.));
#125402=CARTESIAN_POINT('Ctrl Pts',(39.4673289592425,-57.8812926637397,
12.));
#125403=CARTESIAN_POINT('Ctrl Pts',(39.4608716627367,-57.8628360097134,
0.));
#125404=CARTESIAN_POINT('Ctrl Pts',(39.4608716627367,-57.8628360097134,
12.));
#125405=CARTESIAN_POINT('Ctrl Pts',(39.4557042029884,-57.8481172247804,
0.));
#125406=CARTESIAN_POINT('Ctrl Pts',(39.4557042029884,-57.8481172247804,
12.));
#125407=CARTESIAN_POINT('Ctrl Pts',(39.45182770037,-57.8371043151606,0.));
#125408=CARTESIAN_POINT('Ctrl Pts',(39.45182770037,-57.8371043151606,12.));
#125409=CARTESIAN_POINT('Ctrl Pts',(39.4492429618498,-57.829774010102,0.));
#125410=CARTESIAN_POINT('Ctrl Pts',(39.4492429618498,-57.829774010102,12.));
#125411=CARTESIAN_POINT('Ctrl Pts',(39.4479504917287,-57.8261117662439,
0.));
#125412=CARTESIAN_POINT('Ctrl Pts',(39.4479504917287,-57.8261117662439,
12.));
#125413=CARTESIAN_POINT('',(39.4479504917287,-57.8261117662439,12.));
#125414=CARTESIAN_POINT('Ctrl Pts',(39.4479504917287,-57.8261117662439,
12.));
#125415=CARTESIAN_POINT('Ctrl Pts',(39.4492429618498,-57.829774010102,12.));
#125416=CARTESIAN_POINT('Ctrl Pts',(39.45182770037,-57.8371043151606,12.));
#125417=CARTESIAN_POINT('Ctrl Pts',(39.4557042029884,-57.8481172247804,
12.));
#125418=CARTESIAN_POINT('Ctrl Pts',(39.4608716627367,-57.8628360097134,
12.));
#125419=CARTESIAN_POINT('Ctrl Pts',(39.4673289592425,-57.8812926637397,
12.));
#125420=CARTESIAN_POINT('Ctrl Pts',(39.4737841949417,-57.899807467054,12.));
#125421=CARTESIAN_POINT('Ctrl Pts',(39.4802373061008,-57.9183803632337,
12.));
#125422=CARTESIAN_POINT('Ctrl Pts',(39.4866881842223,-57.9370112456506,
12.));
#125423=CARTESIAN_POINT('Ctrl Pts',(39.4931366776628,-57.9556999583777,
12.));
#125424=CARTESIAN_POINT('Ctrl Pts',(39.4995826106692,-57.9744463179305,
12.));
#125425=CARTESIAN_POINT('Ctrl Pts',(39.5060257981225,-57.9932501298522,
12.));
#125426=CARTESIAN_POINT('Ctrl Pts',(39.5124660615009,-58.012111206794,12.));
#125427=CARTESIAN_POINT('Ctrl Pts',(39.5189032457227,-58.0310293875321,
12.));
#125428=CARTESIAN_POINT('Ctrl Pts',(39.5253372136921,-58.0500045308459,
12.));
#125429=CARTESIAN_POINT('Ctrl Pts',(39.5317678383231,-58.0690365065393,
12.));
#125430=CARTESIAN_POINT('Ctrl Pts',(39.5381949959214,-58.088125187991,12.));
#125431=CARTESIAN_POINT('Ctrl Pts',(39.5446185579615,-58.1072704428895,
12.));
#125432=CARTESIAN_POINT('Ctrl Pts',(39.5510383869476,-58.1264721285697,
12.));
#125433=CARTESIAN_POINT('Ctrl Pts',(39.5574543406959,-58.1457300968466,
12.));
#125434=CARTESIAN_POINT('Ctrl Pts',(39.5638662750174,-58.1650441970378,
12.));
#125435=CARTESIAN_POINT('Ctrl Pts',(39.5702740468013,-58.1844142794359,
12.));
#125436=CARTESIAN_POINT('Ctrl Pts',(39.5766775175226,-58.2038401992496,
12.));
#125437=CARTESIAN_POINT('Ctrl Pts',(39.5830765530919,-58.2233218164407,
12.));
#125438=CARTESIAN_POINT('Ctrl Pts',(39.589471022173,-58.2428589938394,12.));
#125439=CARTESIAN_POINT('Ctrl Pts',(39.5958607950237,-58.2624515958416,
12.));
#125440=CARTESIAN_POINT('Ctrl Pts',(39.6022457420772,-58.2820994868092,
12.));
#125441=CARTESIAN_POINT('Ctrl Pts',(39.6086257327559,-58.3018025297288,
12.));
#125442=CARTESIAN_POINT('Ctrl Pts',(39.6150006360894,-58.3215605869192,
12.));
#125443=CARTESIAN_POINT('Ctrl Pts',(39.6213703212523,-58.3413735206412,
12.));
#125444=CARTESIAN_POINT('Ctrl Pts',(39.6277346580898,-58.3612411936914,
12.));
#125445=CARTESIAN_POINT('Ctrl Pts',(39.6340935177492,-58.3811634701061,
12.));
#125446=CARTESIAN_POINT('Ctrl Pts',(39.6404467729114,-58.4011402154225,
12.));
#125447=CARTESIAN_POINT('Ctrl Pts',(39.6467942974465,-58.4211712963023,
12.));
#125448=CARTESIAN_POINT('Ctrl Pts',(39.6531359662043,-58.4412565802984,
12.));
#125449=CARTESIAN_POINT('Ctrl Pts',(39.6594716547681,-58.4613959355776,
12.));
#125450=CARTESIAN_POINT('Ctrl Pts',(39.66580123918,-58.4815892306044,12.));
#125451=CARTESIAN_POINT('Ctrl Pts',(39.6721245959516,-58.5018363341582,
12.));
#125452=CARTESIAN_POINT('Ctrl Pts',(39.6784416021817,-58.5221371154748,
12.));
#125453=CARTESIAN_POINT('Ctrl Pts',(39.6847521356395,-58.5424914443415,
12.));
#125454=CARTESIAN_POINT('Ctrl Pts',(39.6910560748639,-58.5628991912067,
12.));
#125455=CARTESIAN_POINT('Ctrl Pts',(39.6973532992555,-58.5833602272767,
12.));
#125456=CARTESIAN_POINT('Ctrl Pts',(39.7036436890248,-58.6038744244683,
12.));
#125457=CARTESIAN_POINT('Ctrl Pts',(39.7099271251421,-58.6244416553574,
12.));
#125458=CARTESIAN_POINT('Ctrl Pts',(39.7162034892896,-58.6450617931269,
12.));
#125459=CARTESIAN_POINT('Ctrl Pts',(39.7224726638087,-58.6657347115014,
12.));
#125460=CARTESIAN_POINT('Ctrl Pts',(39.7287345316664,-58.6864602847064,
12.));
#125461=CARTESIAN_POINT('Ctrl Pts',(39.7349889764737,-58.7072383875009,
12.));
#125462=CARTESIAN_POINT('Ctrl Pts',(39.741235882495,-58.7280688951911,12.));
#125463=CARTESIAN_POINT('Ctrl Pts',(39.7474751346603,-58.7489516836452,
12.));
#125464=CARTESIAN_POINT('Ctrl Pts',(39.753706618582,-58.769886629304,12.));
#125465=CARTESIAN_POINT('Ctrl Pts',(39.7599302205527,-58.7908736091808,
12.));
#125466=CARTESIAN_POINT('Ctrl Pts',(39.7661458275276,-58.8119125008521,
12.));
#125467=CARTESIAN_POINT('Ctrl Pts',(39.772353327112,-58.8330031824453,12.));
#125468=CARTESIAN_POINT('Ctrl Pts',(39.7785526075477,-58.8541455326229,
12.));
#125469=CARTESIAN_POINT('Ctrl Pts',(39.7847435576996,-58.8753394305583,
12.));
#125470=CARTESIAN_POINT('Ctrl Pts',(39.7909260670517,-58.8965847559389,
12.));
#125471=CARTESIAN_POINT('Ctrl Pts',(39.7971000257044,-58.9178813889703,
12.));
#125472=CARTESIAN_POINT('Ctrl Pts',(39.8032653243712,-58.9392292103747,
12.));
#125473=CARTESIAN_POINT('Ctrl Pts',(39.8094218543781,-58.9606281013875,
12.));
#125474=CARTESIAN_POINT('Ctrl Pts',(39.8155695076625,-58.9820779437485,
12.));
#125475=CARTESIAN_POINT('Ctrl Pts',(39.8217081767658,-59.0035786197024,
12.));
#125476=CARTESIAN_POINT('Ctrl Pts',(39.8278377548261,-59.0251300119972,
12.));
#125477=CARTESIAN_POINT('Ctrl Pts',(39.8339581355715,-59.0467320038782,
12.));
#125478=CARTESIAN_POINT('Ctrl Pts',(39.8400692133143,-59.068384479077,12.));
#125479=CARTESIAN_POINT('Ctrl Pts',(39.8461708829465,-59.0900873217992,
12.));
#125480=CARTESIAN_POINT('Ctrl Pts',(39.8522630399337,-59.1118404167304,
12.));
#125481=CARTESIAN_POINT('Ctrl Pts',(39.8583455803111,-59.133643649035,12.));
#125482=CARTESIAN_POINT('Ctrl Pts',(39.8644184006785,-59.155496904352,12.));
#125483=CARTESIAN_POINT('Ctrl Pts',(39.8704813981978,-59.1774000687865,
12.));
#125484=CARTESIAN_POINT('Ctrl Pts',(39.8765344705895,-59.1993530289008,
12.));
#125485=CARTESIAN_POINT('Ctrl Pts',(39.8825775161253,-59.2213556717188,
12.));
#125486=CARTESIAN_POINT('Ctrl Pts',(39.8886104336234,-59.2434078847236,
12.));
#125487=CARTESIAN_POINT('Ctrl Pts',(39.8946331224442,-59.2655095558527,
12.));
#125488=CARTESIAN_POINT('Ctrl Pts',(39.9006454824861,-59.287660573487,12.));
#125489=CARTESIAN_POINT('Ctrl Pts',(39.9066474141826,-59.3098608264452,
12.));
#125490=CARTESIAN_POINT('Ctrl Pts',(39.9126388184956,-59.3321102039883,
12.));
#125491=CARTESIAN_POINT('Ctrl Pts',(39.9186195969113,-59.3544085958165,
12.));
#125492=CARTESIAN_POINT('Ctrl Pts',(39.9245896514359,-59.3767558920663,
12.));
#125493=CARTESIAN_POINT('Ctrl Pts',(39.9305488845934,-59.3991519832981,
12.));
#125494=CARTESIAN_POINT('Ctrl Pts',(39.9364971994215,-59.4215967604925,
12.));
#125495=CARTESIAN_POINT('Ctrl Pts',(39.9424344994652,-59.444090115055,12.));
#125496=CARTESIAN_POINT('Ctrl Pts',(39.9483606887731,-59.4666319388123,
12.));
#125497=CARTESIAN_POINT('Ctrl Pts',(39.954275671893,-59.4892221240081,12.));
#125498=CARTESIAN_POINT('Ctrl Pts',(39.96017935387,-59.5118605632919,12.));
#125499=CARTESIAN_POINT('Ctrl Pts',(39.9660716402423,-59.5345471497162,
12.));
#125500=CARTESIAN_POINT('Ctrl Pts',(39.971952437036,-59.5572817767412,12.));
#125501=CARTESIAN_POINT('Ctrl Pts',(39.9778216507609,-59.5800643382322,
12.));
#125502=CARTESIAN_POINT('Ctrl Pts',(39.9836791884072,-59.6028947284551,
12.));
#125503=CARTESIAN_POINT('Ctrl Pts',(39.9895249574432,-59.6257728420644,
12.));
#125504=CARTESIAN_POINT('Ctrl Pts',(39.9953588658115,-59.6486985741015,
12.));
#125505=CARTESIAN_POINT('Ctrl Pts',(40.0011808219231,-59.671671819999,12.));
#125506=CARTESIAN_POINT('Ctrl Pts',(40.0069907346536,-59.6946924755771,
12.));
#125507=CARTESIAN_POINT('Ctrl Pts',(40.0127885133407,-59.7177604370409,
12.));
#125508=CARTESIAN_POINT('Ctrl Pts',(40.0185740677827,-59.7408756009688,
12.));
#125509=CARTESIAN_POINT('Ctrl Pts',(40.0243473082343,-59.7640378643114,
12.));
#125510=CARTESIAN_POINT('Ctrl Pts',(40.0301081454006,-59.7872471243948,
12.));
#125511=CARTESIAN_POINT('Ctrl Pts',(40.035856490434,-59.8105032789179,12.));
#125512=CARTESIAN_POINT('Ctrl Pts',(40.0415922549313,-59.8338062259491,
12.));
#125513=CARTESIAN_POINT('Ctrl Pts',(40.0473153509323,-59.8571558639144,
12.));
#125514=CARTESIAN_POINT('Ctrl Pts',(40.0530256909162,-59.8805520915975,
12.));
#125515=CARTESIAN_POINT('Ctrl Pts',(40.0587231877962,-59.9039948081432,
12.));
#125516=CARTESIAN_POINT('Ctrl Pts',(40.064407754916,-59.9274839130553,12.));
#125517=CARTESIAN_POINT('Ctrl Pts',(40.0700793060473,-59.9510193061927,
12.));
#125518=CARTESIAN_POINT('Ctrl Pts',(40.0757377553888,-59.9746008877584,
12.));
#125519=CARTESIAN_POINT('Ctrl Pts',(40.0813830175623,-59.9982285582983,
12.));
#125520=CARTESIAN_POINT('Ctrl Pts',(40.0870150076074,-60.021902218706,12.));
#125521=CARTESIAN_POINT('Ctrl Pts',(40.0926336409785,-60.0456217702201,
12.));
#125522=CARTESIAN_POINT('Ctrl Pts',(40.0982388335423,-60.069387114421,12.));
#125523=CARTESIAN_POINT('Ctrl Pts',(40.1038305015766,-60.0931981532197,
12.));
#125524=CARTESIAN_POINT('Ctrl Pts',(40.1094085617674,-60.1170547888574,
12.));
#125525=CARTESIAN_POINT('Ctrl Pts',(40.1149729312036,-60.1409569239092,
12.));
#125526=CARTESIAN_POINT('Ctrl Pts',(40.120523527374,-60.1649044612828,12.));
#125527=CARTESIAN_POINT('Ctrl Pts',(40.1260602681644,-60.1888973042152,
12.));
#125528=CARTESIAN_POINT('Ctrl Pts',(40.1315830718577,-60.2129353562622,
12.));
#125529=CARTESIAN_POINT('Ctrl Pts',(40.1370918571305,-60.2370185212964,
12.));
#125530=CARTESIAN_POINT('Ctrl Pts',(40.1425865430472,-60.2611467035116,
12.));
#125531=CARTESIAN_POINT('Ctrl Pts',(40.1480670490586,-60.285319807422,12.));
#125532=CARTESIAN_POINT('Ctrl Pts',(40.1535332949976,-60.3095377378586,
12.));
#125533=CARTESIAN_POINT('Ctrl Pts',(40.1589852010804,-60.3338003999606,
12.));
#125534=CARTESIAN_POINT('Ctrl Pts',(40.1644226879033,-60.3581076991716,
12.));
#125535=CARTESIAN_POINT('Ctrl Pts',(40.1698456764377,-60.3824595412445,
12.));
#125536=CARTESIAN_POINT('Ctrl Pts',(40.1752540880268,-60.4068558322407,
12.));
#125537=CARTESIAN_POINT('Ctrl Pts',(40.180647844383,-60.4312964785273,12.));
#125538=CARTESIAN_POINT('Ctrl Pts',(40.1860268675884,-60.455781386769,12.));
#125539=CARTESIAN_POINT('Ctrl Pts',(40.1913910800921,-60.4803104639225,
12.));
#125540=CARTESIAN_POINT('Ctrl Pts',(40.1967404047062,-60.5048836172435,
12.));
#125541=CARTESIAN_POINT('Ctrl Pts',(40.2020747646014,-60.5295007542841,
12.));
#125542=CARTESIAN_POINT('Ctrl Pts',(40.2073940833053,-60.5541617828925,
12.));
#125543=CARTESIAN_POINT('Ctrl Pts',(40.2126982847011,-60.5788666112042,
12.));
#125544=CARTESIAN_POINT('Ctrl Pts',(40.2179872930273,-60.6036151476349,
12.));
#125545=CARTESIAN_POINT('Ctrl Pts',(40.2232610328721,-60.6284073008871,
12.));
#125546=CARTESIAN_POINT('Ctrl Pts',(40.2285194291706,-60.6532429799499,
12.));
#125547=CARTESIAN_POINT('Ctrl Pts',(40.2337624072029,-60.678122094098,12.));
#125548=CARTESIAN_POINT('Ctrl Pts',(40.2389898925932,-60.7030445528857,
12.));
#125549=CARTESIAN_POINT('Ctrl Pts',(40.2442018113108,-60.728010266139,12.));
#125550=CARTESIAN_POINT('Ctrl Pts',(40.2493980896638,-60.7530191439593,
12.));
#125551=CARTESIAN_POINT('Ctrl Pts',(40.2545786542953,-60.7780710967248,
12.));
#125552=CARTESIAN_POINT('Ctrl Pts',(40.2597434321803,-60.8031660350879,
12.));
#125553=CARTESIAN_POINT('Ctrl Pts',(40.2648923506248,-60.8283038699706,
12.));
#125554=CARTESIAN_POINT('Ctrl Pts',(40.2700253372648,-60.8534845125538,
12.));
#125555=CARTESIAN_POINT('Ctrl Pts',(40.2751423200639,-60.8787078742818,
12.));
#125556=CARTESIAN_POINT('Ctrl Pts',(40.2802432273105,-60.9039738668668,
12.));
#125557=CARTESIAN_POINT('Ctrl Pts',(40.2853279876161,-60.9292824022887,
12.));
#125558=CARTESIAN_POINT('Ctrl Pts',(40.2903965299155,-60.954633392792,12.));
#125559=CARTESIAN_POINT('Ctrl Pts',(40.295448783469,-60.9800267508786,12.));
#125560=CARTESIAN_POINT('Ctrl Pts',(40.300484677858,-61.0054623893066,12.));
#125561=CARTESIAN_POINT('Ctrl Pts',(40.3055041429775,-61.0309402210921,
12.));
#125562=CARTESIAN_POINT('Ctrl Pts',(40.310507109031,-61.056460159505,12.));
#125563=CARTESIAN_POINT('Ctrl Pts',(40.3154935065262,-61.0820221180645,
12.));
#125564=CARTESIAN_POINT('Ctrl Pts',(40.3204632662726,-61.1076260105258,
12.));
#125565=CARTESIAN_POINT('Ctrl Pts',(40.32541631938,-61.1332717508789,12.));
#125566=CARTESIAN_POINT('Ctrl Pts',(40.3303525972616,-61.1589592533613,
12.));
#125567=CARTESIAN_POINT('Ctrl Pts',(40.335272031637,-61.1846884324643,12.));
#125568=CARTESIAN_POINT('Ctrl Pts',(40.340174554537,-61.2104592029377,12.));
#125569=CARTESIAN_POINT('Ctrl Pts',(40.3450600983109,-61.2362714797899,
12.));
#125570=CARTESIAN_POINT('Ctrl Pts',(40.3499285956304,-61.2621251782863,
12.));
#125571=CARTESIAN_POINT('Ctrl Pts',(40.3547799794679,-61.2880202139371,
12.));
#125572=CARTESIAN_POINT('Ctrl Pts',(40.3596141830791,-61.3139565024847,
12.));
#125573=CARTESIAN_POINT('Ctrl Pts',(40.3644311399861,-61.3399339598853,
12.));
#125574=CARTESIAN_POINT('Ctrl Pts',(40.3692307839636,-61.3659525022908,
12.));
#125575=CARTESIAN_POINT('Ctrl Pts',(40.3740130490225,-61.3920120460219,
12.));
#125576=CARTESIAN_POINT('Ctrl Pts',(40.3787778694364,-61.4181125076037,
12.));
#125577=CARTESIAN_POINT('Ctrl Pts',(40.383525179772,-61.4442538038044,12.));
#125578=CARTESIAN_POINT('Ctrl Pts',(40.3882549149228,-61.4704358516709,
12.));
#125579=CARTESIAN_POINT('Ctrl Pts',(40.3929670101366,-61.4966585685549,
12.));
#125580=CARTESIAN_POINT('Ctrl Pts',(40.3976614010653,-61.522921872154,12.));
#125581=CARTESIAN_POINT('Ctrl Pts',(40.4023380237232,-61.5492256804717,
12.));
#125582=CARTESIAN_POINT('Ctrl Pts',(40.4069968143956,-61.5755699117324,
12.));
#125583=CARTESIAN_POINT('Ctrl Pts',(40.4116377095596,-61.601954484301,12.));
#125584=CARTESIAN_POINT('Ctrl Pts',(40.4162606458119,-61.6283793166079,
12.));
#125585=CARTESIAN_POINT('Ctrl Pts',(40.4208655597717,-61.6548443270394,
12.));
#125586=CARTESIAN_POINT('Ctrl Pts',(40.425452388076,-61.6813494339286,12.));
#125587=CARTESIAN_POINT('Ctrl Pts',(40.430021067584,-61.7078945557799,12.));
#125588=CARTESIAN_POINT('Ctrl Pts',(40.4345715355405,-61.7344796114399,
12.));
#125589=CARTESIAN_POINT('Ctrl Pts',(40.4391037297589,-61.7611045202874,
12.));
#125590=CARTESIAN_POINT('Ctrl Pts',(40.443617588795,-61.7877692024076,12.));
#125591=CARTESIAN_POINT('Ctrl Pts',(40.4481130521364,-61.814473578779,12.));
#125592=CARTESIAN_POINT('Ctrl Pts',(40.4525900597894,-61.8412175708552,
12.));
#125593=CARTESIAN_POINT('Ctrl Pts',(40.457048551875,-61.8680011001537,12.));
#125594=CARTESIAN_POINT('Ctrl Pts',(40.4614884681889,-61.8948240878007,
12.));
#125595=CARTESIAN_POINT('Ctrl Pts',(40.4659097478587,-61.9216864541744,
12.));
#125596=CARTESIAN_POINT('Ctrl Pts',(40.4703123287621,-61.9485881182921,
12.));
#125597=CARTESIAN_POINT('Ctrl Pts',(40.4746961480015,-61.9755289983044,
12.));
#125598=CARTESIAN_POINT('Ctrl Pts',(40.4790611429584,-62.0025090125959,
12.));
#125599=CARTESIAN_POINT('Ctrl Pts',(40.4834072522164,-62.029528080742,12.));
#125600=CARTESIAN_POINT('Ctrl Pts',(40.4877344164411,-62.0565861244178,
12.));
#125601=CARTESIAN_POINT('Ctrl Pts',(40.4920425795217,-62.0836830685719,
12.));
#125602=CARTESIAN_POINT('Ctrl Pts',(40.4963316888412,-62.1108188417003,
12.));
#125603=CARTESIAN_POINT('Ctrl Pts',(40.4999919096264,-62.1341126810542,
12.));
#125604=CARTESIAN_POINT('Ctrl Pts',(40.5027877865803,-62.1519925002976,
12.));
#125605=CARTESIAN_POINT('Ctrl Pts',(40.5047277935767,-62.1644411502823,
12.));
#125606=CARTESIAN_POINT('Ctrl Pts',(40.5058175523128,-62.1714473138104,
12.));
#125607=CARTESIAN_POINT('Ctrl Pts',(40.506059810093,-62.1730054756875,12.));
#125608=CARTESIAN_POINT('',(39.4479504917287,-57.8261117662439,0.));
#125609=CARTESIAN_POINT('',(39.4479504917286,-57.8261117662438,0.));
#125610=CARTESIAN_POINT('Ctrl Pts',(40.506059810093,-62.1730054756875,0.));
#125611=CARTESIAN_POINT('Ctrl Pts',(40.5058175523128,-62.1714473138104,
0.));
#125612=CARTESIAN_POINT('Ctrl Pts',(40.5047277935767,-62.1644411502823,
0.));
#125613=CARTESIAN_POINT('Ctrl Pts',(40.5027877865803,-62.1519925002976,
0.));
#125614=CARTESIAN_POINT('Ctrl Pts',(40.4999919096264,-62.1341126810542,
0.));
#125615=CARTESIAN_POINT('Ctrl Pts',(40.4963316888412,-62.1108188417003,
0.));
#125616=CARTESIAN_POINT('Ctrl Pts',(40.4920425795217,-62.0836830685719,
0.));
#125617=CARTESIAN_POINT('Ctrl Pts',(40.4877344164411,-62.0565861244178,
0.));
#125618=CARTESIAN_POINT('Ctrl Pts',(40.4834072522164,-62.029528080742,0.));
#125619=CARTESIAN_POINT('Ctrl Pts',(40.4790611429584,-62.0025090125959,
0.));
#125620=CARTESIAN_POINT('Ctrl Pts',(40.4746961480015,-61.9755289983044,
0.));
#125621=CARTESIAN_POINT('Ctrl Pts',(40.4703123287621,-61.9485881182921,
0.));
#125622=CARTESIAN_POINT('Ctrl Pts',(40.4659097478587,-61.9216864541744,
0.));
#125623=CARTESIAN_POINT('Ctrl Pts',(40.4614884681889,-61.8948240878007,
0.));
#125624=CARTESIAN_POINT('Ctrl Pts',(40.457048551875,-61.8680011001537,0.));
#125625=CARTESIAN_POINT('Ctrl Pts',(40.4525900597894,-61.8412175708552,
0.));
#125626=CARTESIAN_POINT('Ctrl Pts',(40.4481130521364,-61.814473578779,0.));
#125627=CARTESIAN_POINT('Ctrl Pts',(40.443617588795,-61.7877692024076,0.));
#125628=CARTESIAN_POINT('Ctrl Pts',(40.4391037297589,-61.7611045202874,
0.));
#125629=CARTESIAN_POINT('Ctrl Pts',(40.4345715355405,-61.7344796114399,
0.));
#125630=CARTESIAN_POINT('Ctrl Pts',(40.430021067584,-61.7078945557799,0.));
#125631=CARTESIAN_POINT('Ctrl Pts',(40.425452388076,-61.6813494339286,0.));
#125632=CARTESIAN_POINT('Ctrl Pts',(40.4208655597717,-61.6548443270394,
0.));
#125633=CARTESIAN_POINT('Ctrl Pts',(40.4162606458119,-61.6283793166079,
0.));
#125634=CARTESIAN_POINT('Ctrl Pts',(40.4116377095596,-61.601954484301,0.));
#125635=CARTESIAN_POINT('Ctrl Pts',(40.4069968143956,-61.5755699117324,
0.));
#125636=CARTESIAN_POINT('Ctrl Pts',(40.4023380237232,-61.5492256804717,
0.));
#125637=CARTESIAN_POINT('Ctrl Pts',(40.3976614010653,-61.522921872154,0.));
#125638=CARTESIAN_POINT('Ctrl Pts',(40.3929670101366,-61.4966585685549,
0.));
#125639=CARTESIAN_POINT('Ctrl Pts',(40.3882549149228,-61.4704358516709,
0.));
#125640=CARTESIAN_POINT('Ctrl Pts',(40.383525179772,-61.4442538038044,0.));
#125641=CARTESIAN_POINT('Ctrl Pts',(40.3787778694364,-61.4181125076037,
0.));
#125642=CARTESIAN_POINT('Ctrl Pts',(40.3740130490225,-61.3920120460219,
0.));
#125643=CARTESIAN_POINT('Ctrl Pts',(40.3692307839636,-61.3659525022908,
0.));
#125644=CARTESIAN_POINT('Ctrl Pts',(40.3644311399861,-61.3399339598853,
0.));
#125645=CARTESIAN_POINT('Ctrl Pts',(40.3596141830791,-61.3139565024847,
0.));
#125646=CARTESIAN_POINT('Ctrl Pts',(40.3547799794679,-61.2880202139371,
0.));
#125647=CARTESIAN_POINT('Ctrl Pts',(40.3499285956304,-61.2621251782863,
0.));
#125648=CARTESIAN_POINT('Ctrl Pts',(40.3450600983109,-61.2362714797899,
0.));
#125649=CARTESIAN_POINT('Ctrl Pts',(40.340174554537,-61.2104592029377,0.));
#125650=CARTESIAN_POINT('Ctrl Pts',(40.335272031637,-61.1846884324643,0.));
#125651=CARTESIAN_POINT('Ctrl Pts',(40.3303525972616,-61.1589592533613,
0.));
#125652=CARTESIAN_POINT('Ctrl Pts',(40.32541631938,-61.1332717508789,0.));
#125653=CARTESIAN_POINT('Ctrl Pts',(40.3204632662726,-61.1076260105258,
0.));
#125654=CARTESIAN_POINT('Ctrl Pts',(40.3154935065262,-61.0820221180645,
0.));
#125655=CARTESIAN_POINT('Ctrl Pts',(40.310507109031,-61.056460159505,0.));
#125656=CARTESIAN_POINT('Ctrl Pts',(40.3055041429775,-61.0309402210921,
0.));
#125657=CARTESIAN_POINT('Ctrl Pts',(40.300484677858,-61.0054623893066,0.));
#125658=CARTESIAN_POINT('Ctrl Pts',(40.295448783469,-60.9800267508786,0.));
#125659=CARTESIAN_POINT('Ctrl Pts',(40.2903965299155,-60.954633392792,0.));
#125660=CARTESIAN_POINT('Ctrl Pts',(40.2853279876161,-60.9292824022887,
0.));
#125661=CARTESIAN_POINT('Ctrl Pts',(40.2802432273105,-60.9039738668668,
0.));
#125662=CARTESIAN_POINT('Ctrl Pts',(40.2751423200639,-60.8787078742818,
0.));
#125663=CARTESIAN_POINT('Ctrl Pts',(40.2700253372648,-60.8534845125538,
0.));
#125664=CARTESIAN_POINT('Ctrl Pts',(40.2648923506248,-60.8283038699706,
0.));
#125665=CARTESIAN_POINT('Ctrl Pts',(40.2597434321803,-60.8031660350879,
0.));
#125666=CARTESIAN_POINT('Ctrl Pts',(40.2545786542953,-60.7780710967248,
0.));
#125667=CARTESIAN_POINT('Ctrl Pts',(40.2493980896638,-60.7530191439593,
0.));
#125668=CARTESIAN_POINT('Ctrl Pts',(40.2442018113108,-60.728010266139,0.));
#125669=CARTESIAN_POINT('Ctrl Pts',(40.2389898925932,-60.7030445528857,
0.));
#125670=CARTESIAN_POINT('Ctrl Pts',(40.2337624072029,-60.678122094098,0.));
#125671=CARTESIAN_POINT('Ctrl Pts',(40.2285194291706,-60.6532429799499,
0.));
#125672=CARTESIAN_POINT('Ctrl Pts',(40.2232610328721,-60.6284073008871,
0.));
#125673=CARTESIAN_POINT('Ctrl Pts',(40.2179872930273,-60.6036151476349,
0.));
#125674=CARTESIAN_POINT('Ctrl Pts',(40.2126982847011,-60.5788666112042,
0.));
#125675=CARTESIAN_POINT('Ctrl Pts',(40.2073940833053,-60.5541617828925,
0.));
#125676=CARTESIAN_POINT('Ctrl Pts',(40.2020747646014,-60.5295007542841,
0.));
#125677=CARTESIAN_POINT('Ctrl Pts',(40.1967404047062,-60.5048836172435,
0.));
#125678=CARTESIAN_POINT('Ctrl Pts',(40.1913910800921,-60.4803104639225,
0.));
#125679=CARTESIAN_POINT('Ctrl Pts',(40.1860268675884,-60.455781386769,0.));
#125680=CARTESIAN_POINT('Ctrl Pts',(40.180647844383,-60.4312964785273,0.));
#125681=CARTESIAN_POINT('Ctrl Pts',(40.1752540880268,-60.4068558322407,
0.));
#125682=CARTESIAN_POINT('Ctrl Pts',(40.1698456764377,-60.3824595412445,
0.));
#125683=CARTESIAN_POINT('Ctrl Pts',(40.1644226879033,-60.3581076991716,
0.));
#125684=CARTESIAN_POINT('Ctrl Pts',(40.1589852010804,-60.3338003999606,
0.));
#125685=CARTESIAN_POINT('Ctrl Pts',(40.1535332949976,-60.3095377378586,
0.));
#125686=CARTESIAN_POINT('Ctrl Pts',(40.1480670490586,-60.285319807422,0.));
#125687=CARTESIAN_POINT('Ctrl Pts',(40.1425865430472,-60.2611467035116,
0.));
#125688=CARTESIAN_POINT('Ctrl Pts',(40.1370918571305,-60.2370185212964,
0.));
#125689=CARTESIAN_POINT('Ctrl Pts',(40.1315830718577,-60.2129353562622,
0.));
#125690=CARTESIAN_POINT('Ctrl Pts',(40.1260602681644,-60.1888973042152,
0.));
#125691=CARTESIAN_POINT('Ctrl Pts',(40.120523527374,-60.1649044612828,0.));
#125692=CARTESIAN_POINT('Ctrl Pts',(40.1149729312036,-60.1409569239092,
0.));
#125693=CARTESIAN_POINT('Ctrl Pts',(40.1094085617674,-60.1170547888574,
0.));
#125694=CARTESIAN_POINT('Ctrl Pts',(40.1038305015766,-60.0931981532197,
0.));
#125695=CARTESIAN_POINT('Ctrl Pts',(40.0982388335423,-60.069387114421,0.));
#125696=CARTESIAN_POINT('Ctrl Pts',(40.0926336409785,-60.0456217702201,
0.));
#125697=CARTESIAN_POINT('Ctrl Pts',(40.0870150076074,-60.021902218706,0.));
#125698=CARTESIAN_POINT('Ctrl Pts',(40.0813830175623,-59.9982285582983,
0.));
#125699=CARTESIAN_POINT('Ctrl Pts',(40.0757377553888,-59.9746008877584,
0.));
#125700=CARTESIAN_POINT('Ctrl Pts',(40.0700793060473,-59.9510193061927,
0.));
#125701=CARTESIAN_POINT('Ctrl Pts',(40.064407754916,-59.9274839130553,0.));
#125702=CARTESIAN_POINT('Ctrl Pts',(40.0587231877962,-59.9039948081432,
0.));
#125703=CARTESIAN_POINT('Ctrl Pts',(40.0530256909162,-59.8805520915975,
0.));
#125704=CARTESIAN_POINT('Ctrl Pts',(40.0473153509323,-59.8571558639144,
0.));
#125705=CARTESIAN_POINT('Ctrl Pts',(40.0415922549313,-59.8338062259491,
0.));
#125706=CARTESIAN_POINT('Ctrl Pts',(40.035856490434,-59.8105032789179,0.));
#125707=CARTESIAN_POINT('Ctrl Pts',(40.0301081454006,-59.7872471243948,
0.));
#125708=CARTESIAN_POINT('Ctrl Pts',(40.0243473082343,-59.7640378643114,
0.));
#125709=CARTESIAN_POINT('Ctrl Pts',(40.0185740677827,-59.7408756009688,
0.));
#125710=CARTESIAN_POINT('Ctrl Pts',(40.0127885133407,-59.7177604370409,
0.));
#125711=CARTESIAN_POINT('Ctrl Pts',(40.0069907346536,-59.6946924755771,
0.));
#125712=CARTESIAN_POINT('Ctrl Pts',(40.0011808219231,-59.671671819999,0.));
#125713=CARTESIAN_POINT('Ctrl Pts',(39.9953588658115,-59.6486985741015,
0.));
#125714=CARTESIAN_POINT('Ctrl Pts',(39.9895249574432,-59.6257728420644,
0.));
#125715=CARTESIAN_POINT('Ctrl Pts',(39.9836791884072,-59.6028947284551,
0.));
#125716=CARTESIAN_POINT('Ctrl Pts',(39.9778216507609,-59.5800643382322,
0.));
#125717=CARTESIAN_POINT('Ctrl Pts',(39.971952437036,-59.5572817767412,0.));
#125718=CARTESIAN_POINT('Ctrl Pts',(39.9660716402423,-59.5345471497162,
0.));
#125719=CARTESIAN_POINT('Ctrl Pts',(39.96017935387,-59.5118605632919,0.));
#125720=CARTESIAN_POINT('Ctrl Pts',(39.954275671893,-59.4892221240081,0.));
#125721=CARTESIAN_POINT('Ctrl Pts',(39.9483606887731,-59.4666319388123,
0.));
#125722=CARTESIAN_POINT('Ctrl Pts',(39.9424344994652,-59.444090115055,0.));
#125723=CARTESIAN_POINT('Ctrl Pts',(39.9364971994215,-59.4215967604925,
0.));
#125724=CARTESIAN_POINT('Ctrl Pts',(39.9305488845934,-59.3991519832981,
0.));
#125725=CARTESIAN_POINT('Ctrl Pts',(39.9245896514359,-59.3767558920663,
0.));
#125726=CARTESIAN_POINT('Ctrl Pts',(39.9186195969113,-59.3544085958165,
0.));
#125727=CARTESIAN_POINT('Ctrl Pts',(39.9126388184956,-59.3321102039883,
0.));
#125728=CARTESIAN_POINT('Ctrl Pts',(39.9066474141826,-59.3098608264452,
0.));
#125729=CARTESIAN_POINT('Ctrl Pts',(39.9006454824861,-59.287660573487,0.));
#125730=CARTESIAN_POINT('Ctrl Pts',(39.8946331224442,-59.2655095558527,
0.));
#125731=CARTESIAN_POINT('Ctrl Pts',(39.8886104336234,-59.2434078847236,
0.));
#125732=CARTESIAN_POINT('Ctrl Pts',(39.8825775161253,-59.2213556717188,
0.));
#125733=CARTESIAN_POINT('Ctrl Pts',(39.8765344705895,-59.1993530289008,
0.));
#125734=CARTESIAN_POINT('Ctrl Pts',(39.8704813981978,-59.1774000687865,
0.));
#125735=CARTESIAN_POINT('Ctrl Pts',(39.8644184006785,-59.155496904352,0.));
#125736=CARTESIAN_POINT('Ctrl Pts',(39.8583455803111,-59.133643649035,0.));
#125737=CARTESIAN_POINT('Ctrl Pts',(39.8522630399337,-59.1118404167304,
0.));
#125738=CARTESIAN_POINT('Ctrl Pts',(39.8461708829465,-59.0900873217992,
0.));
#125739=CARTESIAN_POINT('Ctrl Pts',(39.8400692133143,-59.068384479077,0.));
#125740=CARTESIAN_POINT('Ctrl Pts',(39.8339581355715,-59.0467320038782,
0.));
#125741=CARTESIAN_POINT('Ctrl Pts',(39.8278377548261,-59.0251300119972,
0.));
#125742=CARTESIAN_POINT('Ctrl Pts',(39.8217081767658,-59.0035786197024,
0.));
#125743=CARTESIAN_POINT('Ctrl Pts',(39.8155695076625,-58.9820779437485,
0.));
#125744=CARTESIAN_POINT('Ctrl Pts',(39.8094218543781,-58.9606281013875,
0.));
#125745=CARTESIAN_POINT('Ctrl Pts',(39.8032653243712,-58.9392292103747,
0.));
#125746=CARTESIAN_POINT('Ctrl Pts',(39.7971000257044,-58.9178813889703,
0.));
#125747=CARTESIAN_POINT('Ctrl Pts',(39.7909260670517,-58.8965847559389,
0.));
#125748=CARTESIAN_POINT('Ctrl Pts',(39.7847435576996,-58.8753394305583,
0.));
#125749=CARTESIAN_POINT('Ctrl Pts',(39.7785526075477,-58.8541455326229,
0.));
#125750=CARTESIAN_POINT('Ctrl Pts',(39.772353327112,-58.8330031824453,0.));
#125751=CARTESIAN_POINT('Ctrl Pts',(39.7661458275276,-58.8119125008521,
0.));
#125752=CARTESIAN_POINT('Ctrl Pts',(39.7599302205527,-58.7908736091808,
0.));
#125753=CARTESIAN_POINT('Ctrl Pts',(39.753706618582,-58.769886629304,0.));
#125754=CARTESIAN_POINT('Ctrl Pts',(39.7474751346603,-58.7489516836452,
0.));
#125755=CARTESIAN_POINT('Ctrl Pts',(39.741235882495,-58.7280688951911,0.));
#125756=CARTESIAN_POINT('Ctrl Pts',(39.7349889764737,-58.7072383875009,
0.));
#125757=CARTESIAN_POINT('Ctrl Pts',(39.7287345316664,-58.6864602847064,
0.));
#125758=CARTESIAN_POINT('Ctrl Pts',(39.7224726638087,-58.6657347115014,
0.));
#125759=CARTESIAN_POINT('Ctrl Pts',(39.7162034892896,-58.6450617931269,
0.));
#125760=CARTESIAN_POINT('Ctrl Pts',(39.7099271251421,-58.6244416553574,
0.));
#125761=CARTESIAN_POINT('Ctrl Pts',(39.7036436890248,-58.6038744244683,
0.));
#125762=CARTESIAN_POINT('Ctrl Pts',(39.6973532992555,-58.5833602272767,
0.));
#125763=CARTESIAN_POINT('Ctrl Pts',(39.6910560748639,-58.5628991912067,
0.));
#125764=CARTESIAN_POINT('Ctrl Pts',(39.6847521356395,-58.5424914443415,
0.));
#125765=CARTESIAN_POINT('Ctrl Pts',(39.6784416021817,-58.5221371154748,
0.));
#125766=CARTESIAN_POINT('Ctrl Pts',(39.6721245959516,-58.5018363341582,
0.));
#125767=CARTESIAN_POINT('Ctrl Pts',(39.66580123918,-58.4815892306044,0.));
#125768=CARTESIAN_POINT('Ctrl Pts',(39.6594716547681,-58.4613959355776,
0.));
#125769=CARTESIAN_POINT('Ctrl Pts',(39.6531359662043,-58.4412565802984,
0.));
#125770=CARTESIAN_POINT('Ctrl Pts',(39.6467942974465,-58.4211712963023,
0.));
#125771=CARTESIAN_POINT('Ctrl Pts',(39.6404467729114,-58.4011402154225,
0.));
#125772=CARTESIAN_POINT('Ctrl Pts',(39.6340935177492,-58.3811634701061,
0.));
#125773=CARTESIAN_POINT('Ctrl Pts',(39.6277346580898,-58.3612411936914,
0.));
#125774=CARTESIAN_POINT('Ctrl Pts',(39.6213703212523,-58.3413735206412,
0.));
#125775=CARTESIAN_POINT('Ctrl Pts',(39.6150006360894,-58.3215605869192,
0.));
#125776=CARTESIAN_POINT('Ctrl Pts',(39.6086257327559,-58.3018025297288,
0.));
#125777=CARTESIAN_POINT('Ctrl Pts',(39.6022457420772,-58.2820994868092,
0.));
#125778=CARTESIAN_POINT('Ctrl Pts',(39.5958607950237,-58.2624515958416,
0.));
#125779=CARTESIAN_POINT('Ctrl Pts',(39.589471022173,-58.2428589938394,0.));
#125780=CARTESIAN_POINT('Ctrl Pts',(39.5830765530919,-58.2233218164407,
0.));
#125781=CARTESIAN_POINT('Ctrl Pts',(39.5766775175226,-58.2038401992496,
0.));
#125782=CARTESIAN_POINT('Ctrl Pts',(39.5702740468013,-58.1844142794359,
0.));
#125783=CARTESIAN_POINT('Ctrl Pts',(39.5638662750174,-58.1650441970378,
0.));
#125784=CARTESIAN_POINT('Ctrl Pts',(39.5574543406959,-58.1457300968466,
0.));
#125785=CARTESIAN_POINT('Ctrl Pts',(39.5510383869476,-58.1264721285697,
0.));
#125786=CARTESIAN_POINT('Ctrl Pts',(39.5446185579615,-58.1072704428895,
0.));
#125787=CARTESIAN_POINT('Ctrl Pts',(39.5381949959214,-58.088125187991,0.));
#125788=CARTESIAN_POINT('Ctrl Pts',(39.5317678383231,-58.0690365065393,
0.));
#125789=CARTESIAN_POINT('Ctrl Pts',(39.5253372136921,-58.0500045308459,
0.));
#125790=CARTESIAN_POINT('Ctrl Pts',(39.5189032457227,-58.0310293875321,
0.));
#125791=CARTESIAN_POINT('Ctrl Pts',(39.5124660615009,-58.012111206794,0.));
#125792=CARTESIAN_POINT('Ctrl Pts',(39.5060257981225,-57.9932501298522,
0.));
#125793=CARTESIAN_POINT('Ctrl Pts',(39.4995826106692,-57.9744463179305,
0.));
#125794=CARTESIAN_POINT('Ctrl Pts',(39.4931366776628,-57.9556999583777,
0.));
#125795=CARTESIAN_POINT('Ctrl Pts',(39.4866881842223,-57.9370112456506,
0.));
#125796=CARTESIAN_POINT('Ctrl Pts',(39.4802373061008,-57.9183803632337,
0.));
#125797=CARTESIAN_POINT('Ctrl Pts',(39.4737841949417,-57.899807467054,0.));
#125798=CARTESIAN_POINT('Ctrl Pts',(39.4673289592425,-57.8812926637397,
0.));
#125799=CARTESIAN_POINT('Ctrl Pts',(39.4608716627367,-57.8628360097134,
0.));
#125800=CARTESIAN_POINT('Ctrl Pts',(39.4557042029884,-57.8481172247804,
0.));
#125801=CARTESIAN_POINT('Ctrl Pts',(39.45182770037,-57.8371043151606,0.));
#125802=CARTESIAN_POINT('Ctrl Pts',(39.4492429618498,-57.829774010102,0.));
#125803=CARTESIAN_POINT('Ctrl Pts',(39.4479504917287,-57.8261117662439,
0.));
#125804=CARTESIAN_POINT('Ctrl Pts',(34.953242280886,-65.7914953018525,0.));
#125805=CARTESIAN_POINT('Ctrl Pts',(34.953242280886,-65.7914953018525,12.));
#125806=CARTESIAN_POINT('Ctrl Pts',(34.9529266758465,-65.7859084407618,
0.));
#125807=CARTESIAN_POINT('Ctrl Pts',(34.9529266758465,-65.7859084407618,
12.));
#125808=CARTESIAN_POINT('Ctrl Pts',(34.9522931728758,-65.7747383251112,
0.));
#125809=CARTESIAN_POINT('Ctrl Pts',(34.9522931728758,-65.7747383251112,
12.));
#125810=CARTESIAN_POINT('Ctrl Pts',(34.9513360397454,-65.7579939712289,
0.));
#125811=CARTESIAN_POINT('Ctrl Pts',(34.9513360397454,-65.7579939712289,
12.));
#125812=CARTESIAN_POINT('Ctrl Pts',(34.9500461043246,-65.7356898061148,
0.));
#125813=CARTESIAN_POINT('Ctrl Pts',(34.9500461043246,-65.7356898061148,
12.));
#125814=CARTESIAN_POINT('Ctrl Pts',(34.9484107544136,-65.7078456758034,
0.));
#125815=CARTESIAN_POINT('Ctrl Pts',(34.9484107544136,-65.7078456758034,
12.));
#125816=CARTESIAN_POINT('Ctrl Pts',(34.9467524770438,-65.6800376406066,
0.));
#125817=CARTESIAN_POINT('Ctrl Pts',(34.9467524770438,-65.6800376406066,
12.));
#125818=CARTESIAN_POINT('Ctrl Pts',(34.9450712829182,-65.6522657321322,
0.));
#125819=CARTESIAN_POINT('Ctrl Pts',(34.9450712829182,-65.6522657321322,
12.));
#125820=CARTESIAN_POINT('Ctrl Pts',(34.943367193292,-65.624529996851,0.));
#125821=CARTESIAN_POINT('Ctrl Pts',(34.943367193292,-65.624529996851,12.));
#125822=CARTESIAN_POINT('Ctrl Pts',(34.9416402443435,-65.5968304997585,
0.));
#125823=CARTESIAN_POINT('Ctrl Pts',(34.9416402443435,-65.5968304997585,
12.));
#125824=CARTESIAN_POINT('Ctrl Pts',(34.9398904862157,-65.5691673225803,
0.));
#125825=CARTESIAN_POINT('Ctrl Pts',(34.9398904862157,-65.5691673225803,
12.));
#125826=CARTESIAN_POINT('Ctrl Pts',(34.9381179779673,-65.5415405577955,
0.));
#125827=CARTESIAN_POINT('Ctrl Pts',(34.9381179779673,-65.5415405577955,
12.));
#125828=CARTESIAN_POINT('Ctrl Pts',(34.9363227836581,-65.5139503038036,
0.));
#125829=CARTESIAN_POINT('Ctrl Pts',(34.9363227836581,-65.5139503038036,
12.));
#125830=CARTESIAN_POINT('Ctrl Pts',(34.9345049680825,-65.4863966597544,
0.));
#125831=CARTESIAN_POINT('Ctrl Pts',(34.9345049680825,-65.4863966597544,
12.));
#125832=CARTESIAN_POINT('Ctrl Pts',(34.9326645923939,-65.4588797201972,
0.));
#125833=CARTESIAN_POINT('Ctrl Pts',(34.9326645923939,-65.4588797201972,
12.));
#125834=CARTESIAN_POINT('Ctrl Pts',(34.9308017105535,-65.4313995707536,
0.));
#125835=CARTESIAN_POINT('Ctrl Pts',(34.9308017105535,-65.4313995707536,
12.));
#125836=CARTESIAN_POINT('Ctrl Pts',(34.9289163717747,-65.4039562911353,
0.));
#125837=CARTESIAN_POINT('Ctrl Pts',(34.9289163717747,-65.4039562911353,
12.));
#125838=CARTESIAN_POINT('Ctrl Pts',(34.927008622273,-65.3765499573077,0.));
#125839=CARTESIAN_POINT('Ctrl Pts',(34.927008622273,-65.3765499573077,12.));
#125840=CARTESIAN_POINT('Ctrl Pts',(34.9250785073476,-65.3491806440537,
0.));
#125841=CARTESIAN_POINT('Ctrl Pts',(34.9250785073476,-65.3491806440537,
12.));
#125842=CARTESIAN_POINT('Ctrl Pts',(34.923126073183,-65.3218484271911,0.));
#125843=CARTESIAN_POINT('Ctrl Pts',(34.923126073183,-65.3218484271911,12.));
#125844=CARTESIAN_POINT('Ctrl Pts',(34.9211513691355,-65.2945533863762,
0.));
#125845=CARTESIAN_POINT('Ctrl Pts',(34.9211513691355,-65.2945533863762,
12.));
#125846=CARTESIAN_POINT('Ctrl Pts',(34.9191544474872,-65.267295604807,0.));
#125847=CARTESIAN_POINT('Ctrl Pts',(34.9191544474872,-65.267295604807,12.));
#125848=CARTESIAN_POINT('Ctrl Pts',(34.9171353624112,-65.2400751679549,
0.));
#125849=CARTESIAN_POINT('Ctrl Pts',(34.9171353624112,-65.2400751679549,
12.));
#125850=CARTESIAN_POINT('Ctrl Pts',(34.9150941691747,-65.2128921625824,
0.));
#125851=CARTESIAN_POINT('Ctrl Pts',(34.9150941691747,-65.2128921625824,
12.));
#125852=CARTESIAN_POINT('Ctrl Pts',(34.9130309233021,-65.1857466757092,
0.));
#125853=CARTESIAN_POINT('Ctrl Pts',(34.9130309233021,-65.1857466757092,
12.));
#125854=CARTESIAN_POINT('Ctrl Pts',(34.9109456796213,-65.1586387934241,
0.));
#125855=CARTESIAN_POINT('Ctrl Pts',(34.9109456796213,-65.1586387934241,
12.));
#125856=CARTESIAN_POINT('Ctrl Pts',(34.9088384918336,-65.1315686003516,
0.));
#125857=CARTESIAN_POINT('Ctrl Pts',(34.9088384918336,-65.1315686003516,
12.));
#125858=CARTESIAN_POINT('Ctrl Pts',(34.9067094130398,-65.1045361803122,
0.));
#125859=CARTESIAN_POINT('Ctrl Pts',(34.9067094130398,-65.1045361803122,
12.));
#125860=CARTESIAN_POINT('Ctrl Pts',(34.9045584960508,-65.0775416167086,
0.));
#125861=CARTESIAN_POINT('Ctrl Pts',(34.9045584960508,-65.0775416167086,
12.));
#125862=CARTESIAN_POINT('Ctrl Pts',(34.9023857937865,-65.0505849930172,
0.));
#125863=CARTESIAN_POINT('Ctrl Pts',(34.9023857937865,-65.0505849930172,
12.));
#125864=CARTESIAN_POINT('Ctrl Pts',(34.9001913596416,-65.0236663932328,
0.));
#125865=CARTESIAN_POINT('Ctrl Pts',(34.9001913596416,-65.0236663932328,
12.));
#125866=CARTESIAN_POINT('Ctrl Pts',(34.8979752478615,-64.9967859023212,
0.));
#125867=CARTESIAN_POINT('Ctrl Pts',(34.8979752478615,-64.9967859023212,
12.));
#125868=CARTESIAN_POINT('Ctrl Pts',(34.8957375133697,-64.9699436060169,
0.));
#125869=CARTESIAN_POINT('Ctrl Pts',(34.8957375133697,-64.9699436060169,
12.));
#125870=CARTESIAN_POINT('Ctrl Pts',(34.8934782116094,-64.9431395906337,
0.));
#125871=CARTESIAN_POINT('Ctrl Pts',(34.8934782116094,-64.9431395906337,
12.));
#125872=CARTESIAN_POINT('Ctrl Pts',(34.8911973983784,-64.9163739428605,
0.));
#125873=CARTESIAN_POINT('Ctrl Pts',(34.8911973983784,-64.9163739428605,
12.));
#125874=CARTESIAN_POINT('Ctrl Pts',(34.888895129681,-64.8896467495757,0.));
#125875=CARTESIAN_POINT('Ctrl Pts',(34.888895129681,-64.8896467495757,12.));
#125876=CARTESIAN_POINT('Ctrl Pts',(34.8865714615435,-64.8629580976063,
0.));
#125877=CARTESIAN_POINT('Ctrl Pts',(34.8865714615435,-64.8629580976063,
12.));
#125878=CARTESIAN_POINT('Ctrl Pts',(34.8842264500188,-64.8363080737378,
0.));
#125879=CARTESIAN_POINT('Ctrl Pts',(34.8842264500188,-64.8363080737378,
12.));
#125880=CARTESIAN_POINT('Ctrl Pts',(34.881860151273,-64.8096967648308,0.));
#125881=CARTESIAN_POINT('Ctrl Pts',(34.881860151273,-64.8096967648308,12.));
#125882=CARTESIAN_POINT('Ctrl Pts',(34.8794726216512,-64.7831242579028,
0.));
#125883=CARTESIAN_POINT('Ctrl Pts',(34.8794726216512,-64.7831242579028,
12.));
#125884=CARTESIAN_POINT('Ctrl Pts',(34.8770639177492,-64.7565906402151,
0.));
#125885=CARTESIAN_POINT('Ctrl Pts',(34.8770639177492,-64.7565906402151,
12.));
#125886=CARTESIAN_POINT('Ctrl Pts',(34.8746340964971,-64.7300959993653,
0.));
#125887=CARTESIAN_POINT('Ctrl Pts',(34.8746340964971,-64.7300959993653,
12.));
#125888=CARTESIAN_POINT('Ctrl Pts',(34.8721832151974,-64.7036404233306,
0.));
#125889=CARTESIAN_POINT('Ctrl Pts',(34.8721832151974,-64.7036404233306,
12.));
#125890=CARTESIAN_POINT('Ctrl Pts',(34.8697113314789,-64.6772240004228,
0.));
#125891=CARTESIAN_POINT('Ctrl Pts',(34.8697113314789,-64.6772240004228,
12.));
#125892=CARTESIAN_POINT('Ctrl Pts',(34.8672185032719,-64.65084681926,0.));
#125893=CARTESIAN_POINT('Ctrl Pts',(34.8672185032719,-64.65084681926,12.));
#125894=CARTESIAN_POINT('Ctrl Pts',(34.8647047887774,-64.6245089687277,
0.));
#125895=CARTESIAN_POINT('Ctrl Pts',(34.8647047887774,-64.6245089687277,
12.));
#125896=CARTESIAN_POINT('Ctrl Pts',(34.8621702464401,-64.5982105379384,
0.));
#125897=CARTESIAN_POINT('Ctrl Pts',(34.8621702464401,-64.5982105379384,
12.));
#125898=CARTESIAN_POINT('Ctrl Pts',(34.8596149349256,-64.5719516161927,
0.));
#125899=CARTESIAN_POINT('Ctrl Pts',(34.8596149349256,-64.5719516161927,
12.));
#125900=CARTESIAN_POINT('Ctrl Pts',(34.857038913134,-64.5457322930088,0.));
#125901=CARTESIAN_POINT('Ctrl Pts',(34.857038913134,-64.5457322930088,12.));
#125902=CARTESIAN_POINT('Ctrl Pts',(34.8544422402118,-64.5195526581407,
0.));
#125903=CARTESIAN_POINT('Ctrl Pts',(34.8544422402118,-64.5195526581407,
12.));
#125904=CARTESIAN_POINT('Ctrl Pts',(34.851824975568,-64.4934128015985,0.));
#125905=CARTESIAN_POINT('Ctrl Pts',(34.851824975568,-64.4934128015985,12.));
#125906=CARTESIAN_POINT('Ctrl Pts',(34.8491871788895,-64.4673128136625,
0.));
#125907=CARTESIAN_POINT('Ctrl Pts',(34.8491871788895,-64.4673128136625,
12.));
#125908=CARTESIAN_POINT('Ctrl Pts',(34.8465289101621,-64.4412527848969,
0.));
#125909=CARTESIAN_POINT('Ctrl Pts',(34.8465289101621,-64.4412527848969,
12.));
#125910=CARTESIAN_POINT('Ctrl Pts',(34.8438502296664,-64.4152328061515,
0.));
#125911=CARTESIAN_POINT('Ctrl Pts',(34.8438502296664,-64.4152328061515,
12.));
#125912=CARTESIAN_POINT('Ctrl Pts',(34.8411511979702,-64.3892529685607,
0.));
#125913=CARTESIAN_POINT('Ctrl Pts',(34.8411511979702,-64.3892529685607,
12.));
#125914=CARTESIAN_POINT('Ctrl Pts',(34.8384318759248,-64.3633133635383,
0.));
#125915=CARTESIAN_POINT('Ctrl Pts',(34.8384318759248,-64.3633133635383,
12.));
#125916=CARTESIAN_POINT('Ctrl Pts',(34.8356923246617,-64.3374140827712,
0.));
#125917=CARTESIAN_POINT('Ctrl Pts',(34.8356923246617,-64.3374140827712,
12.));
#125918=CARTESIAN_POINT('Ctrl Pts',(34.8329326055918,-64.3115552182063,
0.));
#125919=CARTESIAN_POINT('Ctrl Pts',(34.8329326055918,-64.3115552182063,
12.));
#125920=CARTESIAN_POINT('Ctrl Pts',(34.8301527804054,-64.285736862052,0.));
#125921=CARTESIAN_POINT('Ctrl Pts',(34.8301527804054,-64.285736862052,12.));
#125922=CARTESIAN_POINT('Ctrl Pts',(34.8273529110743,-64.2599591067916,
0.));
#125923=CARTESIAN_POINT('Ctrl Pts',(34.8273529110743,-64.2599591067916,
12.));
#125924=CARTESIAN_POINT('Ctrl Pts',(34.8245330598559,-64.234222045188,0.));
#125925=CARTESIAN_POINT('Ctrl Pts',(34.8245330598559,-64.234222045188,12.));
#125926=CARTESIAN_POINT('Ctrl Pts',(34.8216932892968,-64.2085257702884,
0.));
#125927=CARTESIAN_POINT('Ctrl Pts',(34.8216932892968,-64.2085257702884,
12.));
#125928=CARTESIAN_POINT('Ctrl Pts',(34.8188336622418,-64.1828703754236,
0.));
#125929=CARTESIAN_POINT('Ctrl Pts',(34.8188336622418,-64.1828703754236,
12.));
#125930=CARTESIAN_POINT('Ctrl Pts',(34.8159542418374,-64.1572559542086,
0.));
#125931=CARTESIAN_POINT('Ctrl Pts',(34.8159542418374,-64.1572559542086,
12.));
#125932=CARTESIAN_POINT('Ctrl Pts',(34.8130550915286,-64.1316826005506,
0.));
#125933=CARTESIAN_POINT('Ctrl Pts',(34.8130550915286,-64.1316826005506,
12.));
#125934=CARTESIAN_POINT('Ctrl Pts',(34.8101362750597,-64.1061504086516,
0.));
#125935=CARTESIAN_POINT('Ctrl Pts',(34.8101362750597,-64.1061504086516,
12.));
#125936=CARTESIAN_POINT('Ctrl Pts',(34.8071978564747,-64.0806594730085,
0.));
#125937=CARTESIAN_POINT('Ctrl Pts',(34.8071978564747,-64.0806594730085,
12.));
#125938=CARTESIAN_POINT('Ctrl Pts',(34.804239900121,-64.0552098884096,0.));
#125939=CARTESIAN_POINT('Ctrl Pts',(34.804239900121,-64.0552098884096,12.));
#125940=CARTESIAN_POINT('Ctrl Pts',(34.8012624706526,-64.0298017499294,
0.));
#125941=CARTESIAN_POINT('Ctrl Pts',(34.8012624706526,-64.0298017499294,
12.));
#125942=CARTESIAN_POINT('Ctrl Pts',(34.7982656330293,-64.0044351529402,
0.));
#125943=CARTESIAN_POINT('Ctrl Pts',(34.7982656330293,-64.0044351529402,
12.));
#125944=CARTESIAN_POINT('Ctrl Pts',(34.7952494525177,-63.9791101931162,
0.));
#125945=CARTESIAN_POINT('Ctrl Pts',(34.7952494525177,-63.9791101931162,
12.));
#125946=CARTESIAN_POINT('Ctrl Pts',(34.7922139946942,-63.9538269664366,
0.));
#125947=CARTESIAN_POINT('Ctrl Pts',(34.7922139946942,-63.9538269664366,
12.));
#125948=CARTESIAN_POINT('Ctrl Pts',(34.7891593254488,-63.9285855691845,
0.));
#125949=CARTESIAN_POINT('Ctrl Pts',(34.7891593254488,-63.9285855691845,
12.));
#125950=CARTESIAN_POINT('Ctrl Pts',(34.7860855109911,-63.9033860979435,
0.));
#125951=CARTESIAN_POINT('Ctrl Pts',(34.7860855109911,-63.9033860979435,
12.));
#125952=CARTESIAN_POINT('Ctrl Pts',(34.7829926178496,-63.8782286496062,
0.));
#125953=CARTESIAN_POINT('Ctrl Pts',(34.7829926178496,-63.8782286496062,
12.));
#125954=CARTESIAN_POINT('Ctrl Pts',(34.7798807128714,-63.8531133213793,
0.));
#125955=CARTESIAN_POINT('Ctrl Pts',(34.7798807128714,-63.8531133213793,
12.));
#125956=CARTESIAN_POINT('Ctrl Pts',(34.7767498632242,-63.8280402107856,
0.));
#125957=CARTESIAN_POINT('Ctrl Pts',(34.7767498632242,-63.8280402107856,
12.));
#125958=CARTESIAN_POINT('Ctrl Pts',(34.7736001363992,-63.8030094156639,
0.));
#125959=CARTESIAN_POINT('Ctrl Pts',(34.7736001363992,-63.8030094156639,
12.));
#125960=CARTESIAN_POINT('Ctrl Pts',(34.7704316002171,-63.778021034163,0.));
#125961=CARTESIAN_POINT('Ctrl Pts',(34.7704316002171,-63.778021034163,12.));
#125962=CARTESIAN_POINT('Ctrl Pts',(34.7672443228274,-63.7530751647494,
0.));
#125963=CARTESIAN_POINT('Ctrl Pts',(34.7672443228274,-63.7530751647494,
12.));
#125964=CARTESIAN_POINT('Ctrl Pts',(34.76403837271,-63.7281719062149,0.));
#125965=CARTESIAN_POINT('Ctrl Pts',(34.76403837271,-63.7281719062149,12.));
#125966=CARTESIAN_POINT('Ctrl Pts',(34.7608138186759,-63.7033113576786,
0.));
#125967=CARTESIAN_POINT('Ctrl Pts',(34.7608138186759,-63.7033113576786,
12.));
#125968=CARTESIAN_POINT('Ctrl Pts',(34.7575707298713,-63.6784936185885,
0.));
#125969=CARTESIAN_POINT('Ctrl Pts',(34.7575707298713,-63.6784936185885,
12.));
#125970=CARTESIAN_POINT('Ctrl Pts',(34.7543091757833,-63.6537187887159,
0.));
#125971=CARTESIAN_POINT('Ctrl Pts',(34.7543091757833,-63.6537187887159,
12.));
#125972=CARTESIAN_POINT('Ctrl Pts',(34.7510292262406,-63.6289869681604,
0.));
#125973=CARTESIAN_POINT('Ctrl Pts',(34.7510292262406,-63.6289869681604,
12.));
#125974=CARTESIAN_POINT('Ctrl Pts',(34.7477309514136,-63.6042982573588,
0.));
#125975=CARTESIAN_POINT('Ctrl Pts',(34.7477309514136,-63.6042982573588,
12.));
#125976=CARTESIAN_POINT('Ctrl Pts',(34.744414421816,-63.5796527570872,0.));
#125977=CARTESIAN_POINT('Ctrl Pts',(34.744414421816,-63.5796527570872,12.));
#125978=CARTESIAN_POINT('Ctrl Pts',(34.741079708308,-63.5550505684626,0.));
#125979=CARTESIAN_POINT('Ctrl Pts',(34.741079708308,-63.5550505684626,12.));
#125980=CARTESIAN_POINT('Ctrl Pts',(34.7377268821025,-63.5304917929386,
0.));
#125981=CARTESIAN_POINT('Ctrl Pts',(34.7377268821025,-63.5304917929386,
12.));
#125982=CARTESIAN_POINT('Ctrl Pts',(34.7343560147667,-63.505976532309,0.));
#125983=CARTESIAN_POINT('Ctrl Pts',(34.7343560147667,-63.505976532309,12.));
#125984=CARTESIAN_POINT('Ctrl Pts',(34.7309671782213,-63.4815048887166,
0.));
#125985=CARTESIAN_POINT('Ctrl Pts',(34.7309671782213,-63.4815048887166,
12.));
#125986=CARTESIAN_POINT('Ctrl Pts',(34.7275604447438,-63.4570769646569,
0.));
#125987=CARTESIAN_POINT('Ctrl Pts',(34.7275604447438,-63.4570769646569,
12.));
#125988=CARTESIAN_POINT('Ctrl Pts',(34.72413588697,-63.4326928629795,0.));
#125989=CARTESIAN_POINT('Ctrl Pts',(34.72413588697,-63.4326928629795,12.));
#125990=CARTESIAN_POINT('Ctrl Pts',(34.7206935779007,-63.4083526868837,
0.));
#125991=CARTESIAN_POINT('Ctrl Pts',(34.7206935779007,-63.4083526868837,
12.));
#125992=CARTESIAN_POINT('Ctrl Pts',(34.7172335909038,-63.3840565399208,
0.));
#125993=CARTESIAN_POINT('Ctrl Pts',(34.7172335909038,-63.3840565399208,
12.));
#125994=CARTESIAN_POINT('Ctrl Pts',(34.7137559997145,-63.3598045260053,
0.));
#125995=CARTESIAN_POINT('Ctrl Pts',(34.7137559997145,-63.3598045260053,
12.));
#125996=CARTESIAN_POINT('Ctrl Pts',(34.7102608784374,-63.3355967494172,
0.));
#125997=CARTESIAN_POINT('Ctrl Pts',(34.7102608784374,-63.3355967494172,
12.));
#125998=CARTESIAN_POINT('Ctrl Pts',(34.706748301549,-63.3114333148048,0.));
#125999=CARTESIAN_POINT('Ctrl Pts',(34.706748301549,-63.3114333148048,12.));
#126000=CARTESIAN_POINT('Ctrl Pts',(34.703218343904,-63.2873143271807,0.));
#126001=CARTESIAN_POINT('Ctrl Pts',(34.703218343904,-63.2873143271807,12.));
#126002=CARTESIAN_POINT('Ctrl Pts',(34.6996710807378,-63.2632398919225,
0.));
#126003=CARTESIAN_POINT('Ctrl Pts',(34.6996710807378,-63.2632398919225,
12.));
#126004=CARTESIAN_POINT('Ctrl Pts',(34.6961065876666,-63.2392101147847,
0.));
#126005=CARTESIAN_POINT('Ctrl Pts',(34.6961065876666,-63.2392101147847,
12.));
#126006=CARTESIAN_POINT('Ctrl Pts',(34.6925249406896,-63.2152251019012,
0.));
#126007=CARTESIAN_POINT('Ctrl Pts',(34.6925249406896,-63.2152251019012,
12.));
#126008=CARTESIAN_POINT('Ctrl Pts',(34.6889262161924,-63.1912849597888,
0.));
#126009=CARTESIAN_POINT('Ctrl Pts',(34.6889262161924,-63.1912849597888,
12.));
#126010=CARTESIAN_POINT('Ctrl Pts',(34.6853104909518,-63.1673897953429,
0.));
#126011=CARTESIAN_POINT('Ctrl Pts',(34.6853104909518,-63.1673897953429,
12.));
#126012=CARTESIAN_POINT('Ctrl Pts',(34.6816778421402,-63.1435397158389,
0.));
#126013=CARTESIAN_POINT('Ctrl Pts',(34.6816778421402,-63.1435397158389,
12.));
#126014=CARTESIAN_POINT('Ctrl Pts',(34.6780283473251,-63.119734828943,0.));
#126015=CARTESIAN_POINT('Ctrl Pts',(34.6780283473251,-63.119734828943,12.));
#126016=CARTESIAN_POINT('Ctrl Pts',(34.674362084472,-63.0959752427168,0.));
#126017=CARTESIAN_POINT('Ctrl Pts',(34.674362084472,-63.0959752427168,12.));
#126018=CARTESIAN_POINT('Ctrl Pts',(34.670679131947,-63.0722610656194,0.));
#126019=CARTESIAN_POINT('Ctrl Pts',(34.670679131947,-63.0722610656194,12.));
#126020=CARTESIAN_POINT('Ctrl Pts',(34.6669795685228,-63.0485924065045,
0.));
#126021=CARTESIAN_POINT('Ctrl Pts',(34.6669795685228,-63.0485924065045,
12.));
#126022=CARTESIAN_POINT('Ctrl Pts',(34.6632634733824,-63.0249693746208,
0.));
#126023=CARTESIAN_POINT('Ctrl Pts',(34.6632634733824,-63.0249693746208,
12.));
#126024=CARTESIAN_POINT('Ctrl Pts',(34.659530926119,-63.0013920796235,0.));
#126025=CARTESIAN_POINT('Ctrl Pts',(34.659530926119,-63.0013920796235,12.));
#126026=CARTESIAN_POINT('Ctrl Pts',(34.6557820067392,-62.9778606315783,
0.));
#126027=CARTESIAN_POINT('Ctrl Pts',(34.6557820067392,-62.9778606315783,
12.));
#126028=CARTESIAN_POINT('Ctrl Pts',(34.6520167956655,-62.9543751409646,
0.));
#126029=CARTESIAN_POINT('Ctrl Pts',(34.6520167956655,-62.9543751409646,
12.));
#126030=CARTESIAN_POINT('Ctrl Pts',(34.6482353737424,-62.9309357186717,
0.));
#126031=CARTESIAN_POINT('Ctrl Pts',(34.6482353737424,-62.9309357186717,
12.));
#126032=CARTESIAN_POINT('Ctrl Pts',(34.644437822241,-62.9075424760015,0.));
#126033=CARTESIAN_POINT('Ctrl Pts',(34.644437822241,-62.9075424760015,12.));
#126034=CARTESIAN_POINT('Ctrl Pts',(34.6406242228591,-62.8841955246794,
0.));
#126035=CARTESIAN_POINT('Ctrl Pts',(34.6406242228591,-62.8841955246794,
12.));
#126036=CARTESIAN_POINT('Ctrl Pts',(34.6367946577234,-62.8608949768571,
0.));
#126037=CARTESIAN_POINT('Ctrl Pts',(34.6367946577234,-62.8608949768571,
12.));
#126038=CARTESIAN_POINT('Ctrl Pts',(34.6329492093935,-62.8376409451175,
0.));
#126039=CARTESIAN_POINT('Ctrl Pts',(34.6329492093935,-62.8376409451175,
12.));
#126040=CARTESIAN_POINT('Ctrl Pts',(34.6290879608672,-62.8144335424697,
0.));
#126041=CARTESIAN_POINT('Ctrl Pts',(34.6290879608672,-62.8144335424697,
12.));
#126042=CARTESIAN_POINT('Ctrl Pts',(34.6252109955852,-62.7912728823518,
0.));
#126043=CARTESIAN_POINT('Ctrl Pts',(34.6252109955852,-62.7912728823518,
12.));
#126044=CARTESIAN_POINT('Ctrl Pts',(34.6213183974317,-62.7681590786429,
0.));
#126045=CARTESIAN_POINT('Ctrl Pts',(34.6213183974317,-62.7681590786429,
12.));
#126046=CARTESIAN_POINT('Ctrl Pts',(34.6174102507374,-62.7450922456676,
0.));
#126047=CARTESIAN_POINT('Ctrl Pts',(34.6174102507374,-62.7450922456676,
12.));
#126048=CARTESIAN_POINT('Ctrl Pts',(34.6134866402836,-62.7220724981995,
0.));
#126049=CARTESIAN_POINT('Ctrl Pts',(34.6134866402836,-62.7220724981995,
12.));
#126050=CARTESIAN_POINT('Ctrl Pts',(34.6095476513076,-62.6990999514563,
0.));
#126051=CARTESIAN_POINT('Ctrl Pts',(34.6095476513076,-62.6990999514563,
12.));
#126052=CARTESIAN_POINT('Ctrl Pts',(34.6055933695069,-62.6761747211037,
0.));
#126053=CARTESIAN_POINT('Ctrl Pts',(34.6055933695069,-62.6761747211037,
12.));
#126054=CARTESIAN_POINT('Ctrl Pts',(34.6016238810398,-62.6532969232658,
0.));
#126055=CARTESIAN_POINT('Ctrl Pts',(34.6016238810398,-62.6532969232658,
12.));
#126056=CARTESIAN_POINT('Ctrl Pts',(34.5976392725296,-62.6304666745307,
0.));
#126057=CARTESIAN_POINT('Ctrl Pts',(34.5976392725296,-62.6304666745307,
12.));
#126058=CARTESIAN_POINT('Ctrl Pts',(34.5936396310679,-62.6076840919536,
0.));
#126059=CARTESIAN_POINT('Ctrl Pts',(34.5936396310679,-62.6076840919536,
12.));
#126060=CARTESIAN_POINT('Ctrl Pts',(34.5896250442216,-62.5849492930533,
0.));
#126061=CARTESIAN_POINT('Ctrl Pts',(34.5896250442216,-62.5849492930533,
12.));
#126062=CARTESIAN_POINT('Ctrl Pts',(34.5855956000362,-62.5622623958161,
0.));
#126063=CARTESIAN_POINT('Ctrl Pts',(34.5855956000362,-62.5622623958161,
12.));
#126064=CARTESIAN_POINT('Ctrl Pts',(34.5815513870376,-62.5396235187079,
0.));
#126065=CARTESIAN_POINT('Ctrl Pts',(34.5815513870376,-62.5396235187079,
12.));
#126066=CARTESIAN_POINT('Ctrl Pts',(34.5774924942354,-62.5170327806781,
0.));
#126067=CARTESIAN_POINT('Ctrl Pts',(34.5774924942354,-62.5170327806781,
12.));
#126068=CARTESIAN_POINT('Ctrl Pts',(34.5734190111272,-62.4944903011628,
0.));
#126069=CARTESIAN_POINT('Ctrl Pts',(34.5734190111272,-62.4944903011628,
12.));
#126070=CARTESIAN_POINT('Ctrl Pts',(34.5693310277051,-62.4719962000808,
0.));
#126071=CARTESIAN_POINT('Ctrl Pts',(34.5693310277051,-62.4719962000808,
12.));
#126072=CARTESIAN_POINT('Ctrl Pts',(34.5652286344592,-62.4495505978393,
0.));
#126073=CARTESIAN_POINT('Ctrl Pts',(34.5652286344592,-62.4495505978393,
12.));
#126074=CARTESIAN_POINT('Ctrl Pts',(34.5611119223798,-62.4271536153459,
0.));
#126075=CARTESIAN_POINT('Ctrl Pts',(34.5611119223798,-62.4271536153459,
12.));
#126076=CARTESIAN_POINT('Ctrl Pts',(34.5569809829613,-62.4048053740127,
0.));
#126077=CARTESIAN_POINT('Ctrl Pts',(34.5569809829613,-62.4048053740127,
12.));
#126078=CARTESIAN_POINT('Ctrl Pts',(34.5528359082074,-62.3825059957601,
0.));
#126079=CARTESIAN_POINT('Ctrl Pts',(34.5528359082074,-62.3825059957601,
12.));
#126080=CARTESIAN_POINT('Ctrl Pts',(34.5486767906384,-62.3602556030127,
0.));
#126081=CARTESIAN_POINT('Ctrl Pts',(34.5486767906384,-62.3602556030127,
12.));
#126082=CARTESIAN_POINT('Ctrl Pts',(34.5445037232936,-62.338054318708,0.));
#126083=CARTESIAN_POINT('Ctrl Pts',(34.5445037232936,-62.338054318708,12.));
#126084=CARTESIAN_POINT('Ctrl Pts',(34.5403167997337,-62.3159022663058,
0.));
#126085=CARTESIAN_POINT('Ctrl Pts',(34.5403167997337,-62.3159022663058,
12.));
#126086=CARTESIAN_POINT('Ctrl Pts',(34.5361161140449,-62.2937995697926,
0.));
#126087=CARTESIAN_POINT('Ctrl Pts',(34.5361161140449,-62.2937995697926,
12.));
#126088=CARTESIAN_POINT('Ctrl Pts',(34.5319017608433,-62.2717463536828,
0.));
#126089=CARTESIAN_POINT('Ctrl Pts',(34.5319017608433,-62.2717463536828,
12.));
#126090=CARTESIAN_POINT('Ctrl Pts',(34.5276738352808,-62.2497427430135,
0.));
#126091=CARTESIAN_POINT('Ctrl Pts',(34.5276738352808,-62.2497427430135,
12.));
#126092=CARTESIAN_POINT('Ctrl Pts',(34.523432433049,-62.2277888633577,0.));
#126093=CARTESIAN_POINT('Ctrl Pts',(34.523432433049,-62.2277888633577,12.));
#126094=CARTESIAN_POINT('Ctrl Pts',(34.5191776503842,-62.2058848408347,
0.));
#126095=CARTESIAN_POINT('Ctrl Pts',(34.5191776503842,-62.2058848408347,
12.));
#126096=CARTESIAN_POINT('Ctrl Pts',(34.5149095840729,-62.1840308021171,
0.));
#126097=CARTESIAN_POINT('Ctrl Pts',(34.5149095840729,-62.1840308021171,
12.));
#126098=CARTESIAN_POINT('Ctrl Pts',(34.5106283314594,-62.1622268744336,
0.));
#126099=CARTESIAN_POINT('Ctrl Pts',(34.5106283314594,-62.1622268744336,
12.));
#126100=CARTESIAN_POINT('Ctrl Pts',(34.5063339904533,-62.1404731855686,
0.));
#126101=CARTESIAN_POINT('Ctrl Pts',(34.5063339904533,-62.1404731855686,
12.));
#126102=CARTESIAN_POINT('Ctrl Pts',(34.5020266595292,-62.1187698638705,
0.));
#126103=CARTESIAN_POINT('Ctrl Pts',(34.5020266595292,-62.1187698638705,
12.));
#126104=CARTESIAN_POINT('Ctrl Pts',(34.4977064377281,-62.0971170382565,
0.));
#126105=CARTESIAN_POINT('Ctrl Pts',(34.4977064377281,-62.0971170382565,
12.));
#126106=CARTESIAN_POINT('Ctrl Pts',(34.4933734246592,-62.0755148382136,
0.));
#126107=CARTESIAN_POINT('Ctrl Pts',(34.4933734246592,-62.0755148382136,
12.));
#126108=CARTESIAN_POINT('Ctrl Pts',(34.4890277205041,-62.0539633937944,
0.));
#126109=CARTESIAN_POINT('Ctrl Pts',(34.4890277205041,-62.0539633937944,
12.));
#126110=CARTESIAN_POINT('Ctrl Pts',(34.4846694260205,-62.0324628356152,
0.));
#126111=CARTESIAN_POINT('Ctrl Pts',(34.4846694260205,-62.0324628356152,
12.));
#126112=CARTESIAN_POINT('Ctrl Pts',(34.4802986425534,-62.0110132948807,
0.));
#126113=CARTESIAN_POINT('Ctrl Pts',(34.4802986425534,-62.0110132948807,
12.));
#126114=CARTESIAN_POINT('Ctrl Pts',(34.4759154720477,-61.9896149034009,
0.));
#126115=CARTESIAN_POINT('Ctrl Pts',(34.4759154720477,-61.9896149034009,
12.));
#126116=CARTESIAN_POINT('Ctrl Pts',(34.4715200170588,-61.9682677936048,
0.));
#126117=CARTESIAN_POINT('Ctrl Pts',(34.4715200170588,-61.9682677936048,
12.));
#126118=CARTESIAN_POINT('Ctrl Pts',(34.4671123807705,-61.9469720985512,
0.));
#126119=CARTESIAN_POINT('Ctrl Pts',(34.4671123807705,-61.9469720985512,
12.));
#126120=CARTESIAN_POINT('Ctrl Pts',(34.462692666996,-61.9257279519283,0.));
#126121=CARTESIAN_POINT('Ctrl Pts',(34.462692666996,-61.9257279519283,12.));
#126122=CARTESIAN_POINT('Ctrl Pts',(34.4582609801625,-61.9045354880424,
0.));
#126123=CARTESIAN_POINT('Ctrl Pts',(34.4582609801625,-61.9045354880424,
12.));
#126124=CARTESIAN_POINT('Ctrl Pts',(34.4538174253009,-61.883394841802,0.));
#126125=CARTESIAN_POINT('Ctrl Pts',(34.4538174253009,-61.883394841802,12.));
#126126=CARTESIAN_POINT('Ctrl Pts',(34.4493621080367,-61.8623061487031,
0.));
#126127=CARTESIAN_POINT('Ctrl Pts',(34.4493621080367,-61.8623061487031,
12.));
#126128=CARTESIAN_POINT('Ctrl Pts',(34.4448951345753,-61.8412695447951,
0.));
#126129=CARTESIAN_POINT('Ctrl Pts',(34.4448951345753,-61.8412695447951,
12.));
#126130=CARTESIAN_POINT('Ctrl Pts',(34.4404166117312,-61.8202851667247,
0.));
#126131=CARTESIAN_POINT('Ctrl Pts',(34.4404166117312,-61.8202851667247,
12.));
#126132=CARTESIAN_POINT('Ctrl Pts',(34.4359266469757,-61.7993531518052,
0.));
#126133=CARTESIAN_POINT('Ctrl Pts',(34.4359266469757,-61.7993531518052,
12.));
#126134=CARTESIAN_POINT('Ctrl Pts',(34.4314253484791,-61.7784736380728,
0.));
#126135=CARTESIAN_POINT('Ctrl Pts',(34.4314253484791,-61.7784736380728,
12.));
#126136=CARTESIAN_POINT('Ctrl Pts',(34.4269128251568,-61.7576467643419,
0.));
#126137=CARTESIAN_POINT('Ctrl Pts',(34.4269128251568,-61.7576467643419,
12.));
#126138=CARTESIAN_POINT('Ctrl Pts',(34.4223891867166,-61.7368726702573,
0.));
#126139=CARTESIAN_POINT('Ctrl Pts',(34.4223891867166,-61.7368726702573,
12.));
#126140=CARTESIAN_POINT('Ctrl Pts',(34.4178545435753,-61.7161514961892,
0.));
#126141=CARTESIAN_POINT('Ctrl Pts',(34.4178545435753,-61.7161514961892,
12.));
#126142=CARTESIAN_POINT('Ctrl Pts',(34.4133090067696,-61.6954833831158,
0.));
#126143=CARTESIAN_POINT('Ctrl Pts',(34.4133090067696,-61.6954833831158,
12.));
#126144=CARTESIAN_POINT('Ctrl Pts',(34.4087526878814,-61.674868472521,0.));
#126145=CARTESIAN_POINT('Ctrl Pts',(34.4087526878814,-61.674868472521,12.));
#126146=CARTESIAN_POINT('Ctrl Pts',(34.4041856989328,-61.6543069062436,
0.));
#126147=CARTESIAN_POINT('Ctrl Pts',(34.4041856989328,-61.6543069062436,
12.));
#126148=CARTESIAN_POINT('Ctrl Pts',(34.399608152377,-61.6337988264586,0.));
#126149=CARTESIAN_POINT('Ctrl Pts',(34.399608152377,-61.6337988264586,12.));
#126150=CARTESIAN_POINT('Ctrl Pts',(34.3950201613446,-61.6133443760168,
0.));
#126151=CARTESIAN_POINT('Ctrl Pts',(34.3950201613446,-61.6133443760168,
12.));
#126152=CARTESIAN_POINT('Ctrl Pts',(34.3904218398641,-61.5929436987419,
0.));
#126153=CARTESIAN_POINT('Ctrl Pts',(34.3904218398641,-61.5929436987419,
12.));
#126154=CARTESIAN_POINT('Ctrl Pts',(34.3858133030511,-61.5725969396817,
0.));
#126155=CARTESIAN_POINT('Ctrl Pts',(34.3858133030511,-61.5725969396817,
12.));
#126156=CARTESIAN_POINT('Ctrl Pts',(34.3811946674179,-61.5523042455128,
0.));
#126157=CARTESIAN_POINT('Ctrl Pts',(34.3811946674179,-61.5523042455128,
12.));
#126158=CARTESIAN_POINT('Ctrl Pts',(34.3765660506659,-61.5320657642601,
0.));
#126159=CARTESIAN_POINT('Ctrl Pts',(34.3765660506659,-61.5320657642601,
12.));
#126160=CARTESIAN_POINT('Ctrl Pts',(34.3719275711179,-61.511881644541,0.));
#126161=CARTESIAN_POINT('Ctrl Pts',(34.3719275711179,-61.511881644541,12.));
#126162=CARTESIAN_POINT('Ctrl Pts',(34.3672793472463,-61.4917520349276,
0.));
#126163=CARTESIAN_POINT('Ctrl Pts',(34.3672793472463,-61.4917520349276,
12.));
#126164=CARTESIAN_POINT('Ctrl Pts',(34.3626214971903,-61.4716770832924,
0.));
#126165=CARTESIAN_POINT('Ctrl Pts',(34.3626214971903,-61.4716770832924,
12.));
#126166=CARTESIAN_POINT('Ctrl Pts',(34.357954138202,-61.4516569360499,0.));
#126167=CARTESIAN_POINT('Ctrl Pts',(34.357954138202,-61.4516569360499,12.));
#126168=CARTESIAN_POINT('Ctrl Pts',(34.3532773877111,-61.4316917395959,
0.));
#126169=CARTESIAN_POINT('Ctrl Pts',(34.3532773877111,-61.4316917395959,
12.));
#126170=CARTESIAN_POINT('Ctrl Pts',(34.3485913645991,-61.4117816420251,
0.));
#126171=CARTESIAN_POINT('Ctrl Pts',(34.3485913645991,-61.4117816420251,
12.));
#126172=CARTESIAN_POINT('Ctrl Pts',(34.34389619024,-61.3919267945294,0.));
#126173=CARTESIAN_POINT('Ctrl Pts',(34.34389619024,-61.3919267945294,12.));
#126174=CARTESIAN_POINT('Ctrl Pts',(34.339191990012,-61.3721273534222,0.));
#126175=CARTESIAN_POINT('Ctrl Pts',(34.339191990012,-61.3721273534222,12.));
#126176=CARTESIAN_POINT('Ctrl Pts',(34.3344788934337,-61.3523834803144,
0.));
#126177=CARTESIAN_POINT('Ctrl Pts',(34.3344788934337,-61.3523834803144,
12.));
#126178=CARTESIAN_POINT('Ctrl Pts',(34.3297570310126,-61.3326953378817,
0.));
#126179=CARTESIAN_POINT('Ctrl Pts',(34.3297570310126,-61.3326953378817,
12.));
#126180=CARTESIAN_POINT('Ctrl Pts',(34.3250265314761,-61.3130630861375,
0.));
#126181=CARTESIAN_POINT('Ctrl Pts',(34.3250265314761,-61.3130630861375,
12.));
#126182=CARTESIAN_POINT('Ctrl Pts',(34.3202875193629,-61.2934868791876,
0.));
#126183=CARTESIAN_POINT('Ctrl Pts',(34.3202875193629,-61.2934868791876,
12.));
#126184=CARTESIAN_POINT('Ctrl Pts',(34.3155401111776,-61.2739668600416,
0.));
#126185=CARTESIAN_POINT('Ctrl Pts',(34.3155401111776,-61.2739668600416,
12.));
#126186=CARTESIAN_POINT('Ctrl Pts',(34.3107844191081,-61.2545031656196,
0.));
#126187=CARTESIAN_POINT('Ctrl Pts',(34.3107844191081,-61.2545031656196,
12.));
#126188=CARTESIAN_POINT('Ctrl Pts',(34.3060205584093,-61.2350959366987,
0.));
#126189=CARTESIAN_POINT('Ctrl Pts',(34.3060205584093,-61.2350959366987,
12.));
#126190=CARTESIAN_POINT('Ctrl Pts',(34.3012486533473,-61.2157453259108,
0.));
#126191=CARTESIAN_POINT('Ctrl Pts',(34.3012486533473,-61.2157453259108,
12.));
#126192=CARTESIAN_POINT('Ctrl Pts',(34.296468844362,-61.1964515073823,0.));
#126193=CARTESIAN_POINT('Ctrl Pts',(34.296468844362,-61.1964515073823,12.));
#126194=CARTESIAN_POINT('Ctrl Pts',(34.2916812929674,-61.1772146833083,
0.));
#126195=CARTESIAN_POINT('Ctrl Pts',(34.2916812929674,-61.1772146833083,
12.));
#126196=CARTESIAN_POINT('Ctrl Pts',(34.2868861666301,-61.15803506354,0.));
#126197=CARTESIAN_POINT('Ctrl Pts',(34.2868861666301,-61.15803506354,12.));
#126198=CARTESIAN_POINT('Ctrl Pts',(34.2820836244425,-61.1389128461815,
0.));
#126199=CARTESIAN_POINT('Ctrl Pts',(34.2820836244425,-61.1389128461815,
12.));
#126200=CARTESIAN_POINT('Ctrl Pts',(34.2772738038811,-61.119848199783,0.));
#126201=CARTESIAN_POINT('Ctrl Pts',(34.2772738038811,-61.119848199783,12.));
#126202=CARTESIAN_POINT('Ctrl Pts',(34.2724568037373,-61.1008412400231,
0.));
#126203=CARTESIAN_POINT('Ctrl Pts',(34.2724568037373,-61.1008412400231,
12.));
#126204=CARTESIAN_POINT('Ctrl Pts',(34.2676326825845,-61.0818920286645,
0.));
#126205=CARTESIAN_POINT('Ctrl Pts',(34.2676326825845,-61.0818920286645,
12.));
#126206=CARTESIAN_POINT('Ctrl Pts',(34.2637677132139,-61.0667788793594,
0.));
#126207=CARTESIAN_POINT('Ctrl Pts',(34.2637677132139,-61.0667788793594,
12.));
#126208=CARTESIAN_POINT('Ctrl Pts',(34.260865800176,-61.0554700177207,0.));
#126209=CARTESIAN_POINT('Ctrl Pts',(34.260865800176,-61.0554700177207,12.));
#126210=CARTESIAN_POINT('Ctrl Pts',(34.2589297755482,-61.0479423318803,
0.));
#126211=CARTESIAN_POINT('Ctrl Pts',(34.2589297755482,-61.0479423318803,
12.));
#126212=CARTESIAN_POINT('Ctrl Pts',(34.2579614092496,-61.0441813777723,
0.));
#126213=CARTESIAN_POINT('Ctrl Pts',(34.2579614092496,-61.0441813777723,
12.));
#126214=CARTESIAN_POINT('',(34.2579614092496,-61.0441813777723,12.));
#126215=CARTESIAN_POINT('Ctrl Pts',(34.2579614092496,-61.0441813777723,
12.));
#126216=CARTESIAN_POINT('Ctrl Pts',(34.2589297755482,-61.0479423318803,
12.));
#126217=CARTESIAN_POINT('Ctrl Pts',(34.260865800176,-61.0554700177207,12.));
#126218=CARTESIAN_POINT('Ctrl Pts',(34.2637677132139,-61.0667788793594,
12.));
#126219=CARTESIAN_POINT('Ctrl Pts',(34.2676326825845,-61.0818920286645,
12.));
#126220=CARTESIAN_POINT('Ctrl Pts',(34.2724568037373,-61.1008412400231,
12.));
#126221=CARTESIAN_POINT('Ctrl Pts',(34.2772738038811,-61.119848199783,12.));
#126222=CARTESIAN_POINT('Ctrl Pts',(34.2820836244425,-61.1389128461815,
12.));
#126223=CARTESIAN_POINT('Ctrl Pts',(34.2868861666301,-61.15803506354,12.));
#126224=CARTESIAN_POINT('Ctrl Pts',(34.2916812929674,-61.1772146833083,
12.));
#126225=CARTESIAN_POINT('Ctrl Pts',(34.296468844362,-61.1964515073823,12.));
#126226=CARTESIAN_POINT('Ctrl Pts',(34.3012486533473,-61.2157453259108,
12.));
#126227=CARTESIAN_POINT('Ctrl Pts',(34.3060205584093,-61.2350959366987,
12.));
#126228=CARTESIAN_POINT('Ctrl Pts',(34.3107844191081,-61.2545031656196,
12.));
#126229=CARTESIAN_POINT('Ctrl Pts',(34.3155401111776,-61.2739668600416,
12.));
#126230=CARTESIAN_POINT('Ctrl Pts',(34.3202875193629,-61.2934868791876,
12.));
#126231=CARTESIAN_POINT('Ctrl Pts',(34.3250265314761,-61.3130630861375,
12.));
#126232=CARTESIAN_POINT('Ctrl Pts',(34.3297570310126,-61.3326953378817,
12.));
#126233=CARTESIAN_POINT('Ctrl Pts',(34.3344788934337,-61.3523834803144,
12.));
#126234=CARTESIAN_POINT('Ctrl Pts',(34.339191990012,-61.3721273534222,12.));
#126235=CARTESIAN_POINT('Ctrl Pts',(34.34389619024,-61.3919267945294,12.));
#126236=CARTESIAN_POINT('Ctrl Pts',(34.3485913645991,-61.4117816420251,
12.));
#126237=CARTESIAN_POINT('Ctrl Pts',(34.3532773877111,-61.4316917395959,
12.));
#126238=CARTESIAN_POINT('Ctrl Pts',(34.357954138202,-61.4516569360499,12.));
#126239=CARTESIAN_POINT('Ctrl Pts',(34.3626214971903,-61.4716770832924,
12.));
#126240=CARTESIAN_POINT('Ctrl Pts',(34.3672793472463,-61.4917520349276,
12.));
#126241=CARTESIAN_POINT('Ctrl Pts',(34.3719275711179,-61.511881644541,12.));
#126242=CARTESIAN_POINT('Ctrl Pts',(34.3765660506659,-61.5320657642601,
12.));
#126243=CARTESIAN_POINT('Ctrl Pts',(34.3811946674179,-61.5523042455128,
12.));
#126244=CARTESIAN_POINT('Ctrl Pts',(34.3858133030511,-61.5725969396817,
12.));
#126245=CARTESIAN_POINT('Ctrl Pts',(34.3904218398641,-61.5929436987419,
12.));
#126246=CARTESIAN_POINT('Ctrl Pts',(34.3950201613446,-61.6133443760168,
12.));
#126247=CARTESIAN_POINT('Ctrl Pts',(34.399608152377,-61.6337988264586,12.));
#126248=CARTESIAN_POINT('Ctrl Pts',(34.4041856989328,-61.6543069062436,
12.));
#126249=CARTESIAN_POINT('Ctrl Pts',(34.4087526878814,-61.674868472521,12.));
#126250=CARTESIAN_POINT('Ctrl Pts',(34.4133090067696,-61.6954833831158,
12.));
#126251=CARTESIAN_POINT('Ctrl Pts',(34.4178545435753,-61.7161514961892,
12.));
#126252=CARTESIAN_POINT('Ctrl Pts',(34.4223891867166,-61.7368726702573,
12.));
#126253=CARTESIAN_POINT('Ctrl Pts',(34.4269128251568,-61.7576467643419,
12.));
#126254=CARTESIAN_POINT('Ctrl Pts',(34.4314253484791,-61.7784736380728,
12.));
#126255=CARTESIAN_POINT('Ctrl Pts',(34.4359266469757,-61.7993531518052,
12.));
#126256=CARTESIAN_POINT('Ctrl Pts',(34.4404166117312,-61.8202851667247,
12.));
#126257=CARTESIAN_POINT('Ctrl Pts',(34.4448951345753,-61.8412695447951,
12.));
#126258=CARTESIAN_POINT('Ctrl Pts',(34.4493621080367,-61.8623061487031,
12.));
#126259=CARTESIAN_POINT('Ctrl Pts',(34.4538174253009,-61.883394841802,12.));
#126260=CARTESIAN_POINT('Ctrl Pts',(34.4582609801625,-61.9045354880424,
12.));
#126261=CARTESIAN_POINT('Ctrl Pts',(34.462692666996,-61.9257279519283,12.));
#126262=CARTESIAN_POINT('Ctrl Pts',(34.4671123807705,-61.9469720985512,
12.));
#126263=CARTESIAN_POINT('Ctrl Pts',(34.4715200170588,-61.9682677936048,
12.));
#126264=CARTESIAN_POINT('Ctrl Pts',(34.4759154720477,-61.9896149034009,
12.));
#126265=CARTESIAN_POINT('Ctrl Pts',(34.4802986425534,-62.0110132948807,
12.));
#126266=CARTESIAN_POINT('Ctrl Pts',(34.4846694260205,-62.0324628356152,
12.));
#126267=CARTESIAN_POINT('Ctrl Pts',(34.4890277205041,-62.0539633937944,
12.));
#126268=CARTESIAN_POINT('Ctrl Pts',(34.4933734246592,-62.0755148382136,
12.));
#126269=CARTESIAN_POINT('Ctrl Pts',(34.4977064377281,-62.0971170382565,
12.));
#126270=CARTESIAN_POINT('Ctrl Pts',(34.5020266595292,-62.1187698638705,
12.));
#126271=CARTESIAN_POINT('Ctrl Pts',(34.5063339904533,-62.1404731855686,
12.));
#126272=CARTESIAN_POINT('Ctrl Pts',(34.5106283314594,-62.1622268744336,
12.));
#126273=CARTESIAN_POINT('Ctrl Pts',(34.5149095840729,-62.1840308021171,
12.));
#126274=CARTESIAN_POINT('Ctrl Pts',(34.5191776503842,-62.2058848408347,
12.));
#126275=CARTESIAN_POINT('Ctrl Pts',(34.523432433049,-62.2277888633577,12.));
#126276=CARTESIAN_POINT('Ctrl Pts',(34.5276738352808,-62.2497427430135,
12.));
#126277=CARTESIAN_POINT('Ctrl Pts',(34.5319017608433,-62.2717463536828,
12.));
#126278=CARTESIAN_POINT('Ctrl Pts',(34.5361161140449,-62.2937995697926,
12.));
#126279=CARTESIAN_POINT('Ctrl Pts',(34.5403167997337,-62.3159022663058,
12.));
#126280=CARTESIAN_POINT('Ctrl Pts',(34.5445037232936,-62.338054318708,12.));
#126281=CARTESIAN_POINT('Ctrl Pts',(34.5486767906384,-62.3602556030127,
12.));
#126282=CARTESIAN_POINT('Ctrl Pts',(34.5528359082074,-62.3825059957601,
12.));
#126283=CARTESIAN_POINT('Ctrl Pts',(34.5569809829613,-62.4048053740127,
12.));
#126284=CARTESIAN_POINT('Ctrl Pts',(34.5611119223798,-62.4271536153459,
12.));
#126285=CARTESIAN_POINT('Ctrl Pts',(34.5652286344592,-62.4495505978393,
12.));
#126286=CARTESIAN_POINT('Ctrl Pts',(34.5693310277051,-62.4719962000808,
12.));
#126287=CARTESIAN_POINT('Ctrl Pts',(34.5734190111272,-62.4944903011628,
12.));
#126288=CARTESIAN_POINT('Ctrl Pts',(34.5774924942354,-62.5170327806781,
12.));
#126289=CARTESIAN_POINT('Ctrl Pts',(34.5815513870376,-62.5396235187079,
12.));
#126290=CARTESIAN_POINT('Ctrl Pts',(34.5855956000362,-62.5622623958161,
12.));
#126291=CARTESIAN_POINT('Ctrl Pts',(34.5896250442216,-62.5849492930533,
12.));
#126292=CARTESIAN_POINT('Ctrl Pts',(34.5936396310679,-62.6076840919536,
12.));
#126293=CARTESIAN_POINT('Ctrl Pts',(34.5976392725296,-62.6304666745307,
12.));
#126294=CARTESIAN_POINT('Ctrl Pts',(34.6016238810398,-62.6532969232658,
12.));
#126295=CARTESIAN_POINT('Ctrl Pts',(34.6055933695069,-62.6761747211037,
12.));
#126296=CARTESIAN_POINT('Ctrl Pts',(34.6095476513076,-62.6990999514563,
12.));
#126297=CARTESIAN_POINT('Ctrl Pts',(34.6134866402836,-62.7220724981995,
12.));
#126298=CARTESIAN_POINT('Ctrl Pts',(34.6174102507374,-62.7450922456676,
12.));
#126299=CARTESIAN_POINT('Ctrl Pts',(34.6213183974317,-62.7681590786429,
12.));
#126300=CARTESIAN_POINT('Ctrl Pts',(34.6252109955852,-62.7912728823518,
12.));
#126301=CARTESIAN_POINT('Ctrl Pts',(34.6290879608672,-62.8144335424697,
12.));
#126302=CARTESIAN_POINT('Ctrl Pts',(34.6329492093935,-62.8376409451175,
12.));
#126303=CARTESIAN_POINT('Ctrl Pts',(34.6367946577234,-62.8608949768571,
12.));
#126304=CARTESIAN_POINT('Ctrl Pts',(34.6406242228591,-62.8841955246794,
12.));
#126305=CARTESIAN_POINT('Ctrl Pts',(34.644437822241,-62.9075424760015,12.));
#126306=CARTESIAN_POINT('Ctrl Pts',(34.6482353737424,-62.9309357186717,
12.));
#126307=CARTESIAN_POINT('Ctrl Pts',(34.6520167956655,-62.9543751409646,
12.));
#126308=CARTESIAN_POINT('Ctrl Pts',(34.6557820067392,-62.9778606315783,
12.));
#126309=CARTESIAN_POINT('Ctrl Pts',(34.659530926119,-63.0013920796235,12.));
#126310=CARTESIAN_POINT('Ctrl Pts',(34.6632634733824,-63.0249693746208,
12.));
#126311=CARTESIAN_POINT('Ctrl Pts',(34.6669795685228,-63.0485924065045,
12.));
#126312=CARTESIAN_POINT('Ctrl Pts',(34.670679131947,-63.0722610656194,12.));
#126313=CARTESIAN_POINT('Ctrl Pts',(34.674362084472,-63.0959752427168,12.));
#126314=CARTESIAN_POINT('Ctrl Pts',(34.6780283473251,-63.119734828943,12.));
#126315=CARTESIAN_POINT('Ctrl Pts',(34.6816778421402,-63.1435397158389,
12.));
#126316=CARTESIAN_POINT('Ctrl Pts',(34.6853104909518,-63.1673897953429,
12.));
#126317=CARTESIAN_POINT('Ctrl Pts',(34.6889262161924,-63.1912849597888,
12.));
#126318=CARTESIAN_POINT('Ctrl Pts',(34.6925249406896,-63.2152251019012,
12.));
#126319=CARTESIAN_POINT('Ctrl Pts',(34.6961065876666,-63.2392101147847,
12.));
#126320=CARTESIAN_POINT('Ctrl Pts',(34.6996710807378,-63.2632398919225,
12.));
#126321=CARTESIAN_POINT('Ctrl Pts',(34.703218343904,-63.2873143271807,12.));
#126322=CARTESIAN_POINT('Ctrl Pts',(34.706748301549,-63.3114333148048,12.));
#126323=CARTESIAN_POINT('Ctrl Pts',(34.7102608784374,-63.3355967494172,
12.));
#126324=CARTESIAN_POINT('Ctrl Pts',(34.7137559997145,-63.3598045260053,
12.));
#126325=CARTESIAN_POINT('Ctrl Pts',(34.7172335909038,-63.3840565399208,
12.));
#126326=CARTESIAN_POINT('Ctrl Pts',(34.7206935779007,-63.4083526868837,
12.));
#126327=CARTESIAN_POINT('Ctrl Pts',(34.72413588697,-63.4326928629795,12.));
#126328=CARTESIAN_POINT('Ctrl Pts',(34.7275604447438,-63.4570769646569,
12.));
#126329=CARTESIAN_POINT('Ctrl Pts',(34.7309671782213,-63.4815048887166,
12.));
#126330=CARTESIAN_POINT('Ctrl Pts',(34.7343560147667,-63.505976532309,12.));
#126331=CARTESIAN_POINT('Ctrl Pts',(34.7377268821025,-63.5304917929386,
12.));
#126332=CARTESIAN_POINT('Ctrl Pts',(34.741079708308,-63.5550505684626,12.));
#126333=CARTESIAN_POINT('Ctrl Pts',(34.744414421816,-63.5796527570872,12.));
#126334=CARTESIAN_POINT('Ctrl Pts',(34.7477309514136,-63.6042982573588,
12.));
#126335=CARTESIAN_POINT('Ctrl Pts',(34.7510292262406,-63.6289869681604,
12.));
#126336=CARTESIAN_POINT('Ctrl Pts',(34.7543091757833,-63.6537187887159,
12.));
#126337=CARTESIAN_POINT('Ctrl Pts',(34.7575707298713,-63.6784936185885,
12.));
#126338=CARTESIAN_POINT('Ctrl Pts',(34.7608138186759,-63.7033113576786,
12.));
#126339=CARTESIAN_POINT('Ctrl Pts',(34.76403837271,-63.7281719062149,12.));
#126340=CARTESIAN_POINT('Ctrl Pts',(34.7672443228274,-63.7530751647494,
12.));
#126341=CARTESIAN_POINT('Ctrl Pts',(34.7704316002171,-63.778021034163,12.));
#126342=CARTESIAN_POINT('Ctrl Pts',(34.7736001363992,-63.8030094156639,
12.));
#126343=CARTESIAN_POINT('Ctrl Pts',(34.7767498632242,-63.8280402107856,
12.));
#126344=CARTESIAN_POINT('Ctrl Pts',(34.7798807128714,-63.8531133213793,
12.));
#126345=CARTESIAN_POINT('Ctrl Pts',(34.7829926178496,-63.8782286496062,
12.));
#126346=CARTESIAN_POINT('Ctrl Pts',(34.7860855109911,-63.9033860979435,
12.));
#126347=CARTESIAN_POINT('Ctrl Pts',(34.7891593254488,-63.9285855691845,
12.));
#126348=CARTESIAN_POINT('Ctrl Pts',(34.7922139946942,-63.9538269664366,
12.));
#126349=CARTESIAN_POINT('Ctrl Pts',(34.7952494525177,-63.9791101931162,
12.));
#126350=CARTESIAN_POINT('Ctrl Pts',(34.7982656330293,-64.0044351529402,
12.));
#126351=CARTESIAN_POINT('Ctrl Pts',(34.8012624706526,-64.0298017499294,
12.));
#126352=CARTESIAN_POINT('Ctrl Pts',(34.804239900121,-64.0552098884096,12.));
#126353=CARTESIAN_POINT('Ctrl Pts',(34.8071978564747,-64.0806594730085,
12.));
#126354=CARTESIAN_POINT('Ctrl Pts',(34.8101362750597,-64.1061504086516,
12.));
#126355=CARTESIAN_POINT('Ctrl Pts',(34.8130550915286,-64.1316826005506,
12.));
#126356=CARTESIAN_POINT('Ctrl Pts',(34.8159542418374,-64.1572559542086,
12.));
#126357=CARTESIAN_POINT('Ctrl Pts',(34.8188336622418,-64.1828703754236,
12.));
#126358=CARTESIAN_POINT('Ctrl Pts',(34.8216932892968,-64.2085257702884,
12.));
#126359=CARTESIAN_POINT('Ctrl Pts',(34.8245330598559,-64.234222045188,12.));
#126360=CARTESIAN_POINT('Ctrl Pts',(34.8273529110743,-64.2599591067916,
12.));
#126361=CARTESIAN_POINT('Ctrl Pts',(34.8301527804054,-64.285736862052,12.));
#126362=CARTESIAN_POINT('Ctrl Pts',(34.8329326055918,-64.3115552182063,
12.));
#126363=CARTESIAN_POINT('Ctrl Pts',(34.8356923246617,-64.3374140827712,
12.));
#126364=CARTESIAN_POINT('Ctrl Pts',(34.8384318759248,-64.3633133635383,
12.));
#126365=CARTESIAN_POINT('Ctrl Pts',(34.8411511979702,-64.3892529685607,
12.));
#126366=CARTESIAN_POINT('Ctrl Pts',(34.8438502296664,-64.4152328061515,
12.));
#126367=CARTESIAN_POINT('Ctrl Pts',(34.8465289101621,-64.4412527848969,
12.));
#126368=CARTESIAN_POINT('Ctrl Pts',(34.8491871788895,-64.4673128136625,
12.));
#126369=CARTESIAN_POINT('Ctrl Pts',(34.851824975568,-64.4934128015985,12.));
#126370=CARTESIAN_POINT('Ctrl Pts',(34.8544422402118,-64.5195526581407,
12.));
#126371=CARTESIAN_POINT('Ctrl Pts',(34.857038913134,-64.5457322930088,12.));
#126372=CARTESIAN_POINT('Ctrl Pts',(34.8596149349256,-64.5719516161927,
12.));
#126373=CARTESIAN_POINT('Ctrl Pts',(34.8621702464401,-64.5982105379384,
12.));
#126374=CARTESIAN_POINT('Ctrl Pts',(34.8647047887774,-64.6245089687277,
12.));
#126375=CARTESIAN_POINT('Ctrl Pts',(34.8672185032719,-64.65084681926,12.));
#126376=CARTESIAN_POINT('Ctrl Pts',(34.8697113314789,-64.6772240004228,
12.));
#126377=CARTESIAN_POINT('Ctrl Pts',(34.8721832151974,-64.7036404233306,
12.));
#126378=CARTESIAN_POINT('Ctrl Pts',(34.8746340964971,-64.7300959993653,
12.));
#126379=CARTESIAN_POINT('Ctrl Pts',(34.8770639177492,-64.7565906402151,
12.));
#126380=CARTESIAN_POINT('Ctrl Pts',(34.8794726216512,-64.7831242579028,
12.));
#126381=CARTESIAN_POINT('Ctrl Pts',(34.881860151273,-64.8096967648308,12.));
#126382=CARTESIAN_POINT('Ctrl Pts',(34.8842264500188,-64.8363080737378,
12.));
#126383=CARTESIAN_POINT('Ctrl Pts',(34.8865714615435,-64.8629580976063,
12.));
#126384=CARTESIAN_POINT('Ctrl Pts',(34.888895129681,-64.8896467495757,12.));
#126385=CARTESIAN_POINT('Ctrl Pts',(34.8911973983784,-64.9163739428605,
12.));
#126386=CARTESIAN_POINT('Ctrl Pts',(34.8934782116094,-64.9431395906337,
12.));
#126387=CARTESIAN_POINT('Ctrl Pts',(34.8957375133697,-64.9699436060169,
12.));
#126388=CARTESIAN_POINT('Ctrl Pts',(34.8979752478615,-64.9967859023212,
12.));
#126389=CARTESIAN_POINT('Ctrl Pts',(34.9001913596416,-65.0236663932328,
12.));
#126390=CARTESIAN_POINT('Ctrl Pts',(34.9023857937865,-65.0505849930172,
12.));
#126391=CARTESIAN_POINT('Ctrl Pts',(34.9045584960508,-65.0775416167086,
12.));
#126392=CARTESIAN_POINT('Ctrl Pts',(34.9067094130398,-65.1045361803122,
12.));
#126393=CARTESIAN_POINT('Ctrl Pts',(34.9088384918336,-65.1315686003516,
12.));
#126394=CARTESIAN_POINT('Ctrl Pts',(34.9109456796213,-65.1586387934241,
12.));
#126395=CARTESIAN_POINT('Ctrl Pts',(34.9130309233021,-65.1857466757092,
12.));
#126396=CARTESIAN_POINT('Ctrl Pts',(34.9150941691747,-65.2128921625824,
12.));
#126397=CARTESIAN_POINT('Ctrl Pts',(34.9171353624112,-65.2400751679549,
12.));
#126398=CARTESIAN_POINT('Ctrl Pts',(34.9191544474872,-65.267295604807,12.));
#126399=CARTESIAN_POINT('Ctrl Pts',(34.9211513691355,-65.2945533863762,
12.));
#126400=CARTESIAN_POINT('Ctrl Pts',(34.923126073183,-65.3218484271911,12.));
#126401=CARTESIAN_POINT('Ctrl Pts',(34.9250785073476,-65.3491806440537,
12.));
#126402=CARTESIAN_POINT('Ctrl Pts',(34.927008622273,-65.3765499573077,12.));
#126403=CARTESIAN_POINT('Ctrl Pts',(34.9289163717747,-65.4039562911353,
12.));
#126404=CARTESIAN_POINT('Ctrl Pts',(34.9305324724444,-65.4274804996591,
12.));
#126405=CARTESIAN_POINT('Ctrl Pts',(34.931759381316,-65.4455359575249,12.));
#126406=CARTESIAN_POINT('Ctrl Pts',(34.9326070346645,-65.4581063193889,
12.));
#126407=CARTESIAN_POINT('Ctrl Pts',(34.9330820191535,-65.4651808010818,
12.));
#126408=CARTESIAN_POINT('Ctrl Pts',(34.933187552314,-65.4667541478394,12.));
#126409=CARTESIAN_POINT('',(34.2579614092496,-61.0441813777723,0.));
#126410=CARTESIAN_POINT('',(34.2579614092496,-61.0441813777723,0.));
#126411=CARTESIAN_POINT('Ctrl Pts',(34.933187552314,-65.4667541478395,0.));
#126412=CARTESIAN_POINT('Ctrl Pts',(34.9330820191535,-65.4651808010819,
0.));
#126413=CARTESIAN_POINT('Ctrl Pts',(34.9326070346645,-65.458106319389,0.));
#126414=CARTESIAN_POINT('Ctrl Pts',(34.931759381316,-65.4455359575249,0.));
#126415=CARTESIAN_POINT('Ctrl Pts',(34.9305324724444,-65.4274804996591,
0.));
#126416=CARTESIAN_POINT('Ctrl Pts',(34.9289163717747,-65.4039562911353,
0.));
#126417=CARTESIAN_POINT('Ctrl Pts',(34.927008622273,-65.3765499573077,0.));
#126418=CARTESIAN_POINT('Ctrl Pts',(34.9250785073476,-65.3491806440537,
0.));
#126419=CARTESIAN_POINT('Ctrl Pts',(34.923126073183,-65.3218484271911,0.));
#126420=CARTESIAN_POINT('Ctrl Pts',(34.9211513691355,-65.2945533863762,
0.));
#126421=CARTESIAN_POINT('Ctrl Pts',(34.9191544474872,-65.267295604807,0.));
#126422=CARTESIAN_POINT('Ctrl Pts',(34.9171353624112,-65.2400751679549,
0.));
#126423=CARTESIAN_POINT('Ctrl Pts',(34.9150941691747,-65.2128921625824,
0.));
#126424=CARTESIAN_POINT('Ctrl Pts',(34.9130309233021,-65.1857466757092,
0.));
#126425=CARTESIAN_POINT('Ctrl Pts',(34.9109456796213,-65.1586387934241,
0.));
#126426=CARTESIAN_POINT('Ctrl Pts',(34.9088384918336,-65.1315686003516,
0.));
#126427=CARTESIAN_POINT('Ctrl Pts',(34.9067094130398,-65.1045361803122,
0.));
#126428=CARTESIAN_POINT('Ctrl Pts',(34.9045584960508,-65.0775416167086,
0.));
#126429=CARTESIAN_POINT('Ctrl Pts',(34.9023857937865,-65.0505849930172,
0.));
#126430=CARTESIAN_POINT('Ctrl Pts',(34.9001913596416,-65.0236663932328,
0.));
#126431=CARTESIAN_POINT('Ctrl Pts',(34.8979752478615,-64.9967859023212,
0.));
#126432=CARTESIAN_POINT('Ctrl Pts',(34.8957375133697,-64.9699436060169,
0.));
#126433=CARTESIAN_POINT('Ctrl Pts',(34.8934782116094,-64.9431395906337,
0.));
#126434=CARTESIAN_POINT('Ctrl Pts',(34.8911973983784,-64.9163739428605,
0.));
#126435=CARTESIAN_POINT('Ctrl Pts',(34.888895129681,-64.8896467495757,0.));
#126436=CARTESIAN_POINT('Ctrl Pts',(34.8865714615435,-64.8629580976063,
0.));
#126437=CARTESIAN_POINT('Ctrl Pts',(34.8842264500188,-64.8363080737378,
0.));
#126438=CARTESIAN_POINT('Ctrl Pts',(34.881860151273,-64.8096967648308,0.));
#126439=CARTESIAN_POINT('Ctrl Pts',(34.8794726216512,-64.7831242579028,
0.));
#126440=CARTESIAN_POINT('Ctrl Pts',(34.8770639177492,-64.7565906402151,
0.));
#126441=CARTESIAN_POINT('Ctrl Pts',(34.8746340964971,-64.7300959993653,
0.));
#126442=CARTESIAN_POINT('Ctrl Pts',(34.8721832151974,-64.7036404233306,
0.));
#126443=CARTESIAN_POINT('Ctrl Pts',(34.8697113314789,-64.6772240004228,
0.));
#126444=CARTESIAN_POINT('Ctrl Pts',(34.8672185032719,-64.65084681926,0.));
#126445=CARTESIAN_POINT('Ctrl Pts',(34.8647047887774,-64.6245089687277,
0.));
#126446=CARTESIAN_POINT('Ctrl Pts',(34.8621702464401,-64.5982105379384,
0.));
#126447=CARTESIAN_POINT('Ctrl Pts',(34.8596149349256,-64.5719516161927,
0.));
#126448=CARTESIAN_POINT('Ctrl Pts',(34.857038913134,-64.5457322930088,0.));
#126449=CARTESIAN_POINT('Ctrl Pts',(34.8544422402118,-64.5195526581407,
0.));
#126450=CARTESIAN_POINT('Ctrl Pts',(34.851824975568,-64.4934128015985,0.));
#126451=CARTESIAN_POINT('Ctrl Pts',(34.8491871788895,-64.4673128136625,
0.));
#126452=CARTESIAN_POINT('Ctrl Pts',(34.8465289101621,-64.4412527848969,
0.));
#126453=CARTESIAN_POINT('Ctrl Pts',(34.8438502296664,-64.4152328061515,
0.));
#126454=CARTESIAN_POINT('Ctrl Pts',(34.8411511979702,-64.3892529685607,
0.));
#126455=CARTESIAN_POINT('Ctrl Pts',(34.8384318759248,-64.3633133635383,
0.));
#126456=CARTESIAN_POINT('Ctrl Pts',(34.8356923246617,-64.3374140827712,
0.));
#126457=CARTESIAN_POINT('Ctrl Pts',(34.8329326055918,-64.3115552182063,
0.));
#126458=CARTESIAN_POINT('Ctrl Pts',(34.8301527804054,-64.285736862052,0.));
#126459=CARTESIAN_POINT('Ctrl Pts',(34.8273529110743,-64.2599591067916,
0.));
#126460=CARTESIAN_POINT('Ctrl Pts',(34.8245330598559,-64.234222045188,0.));
#126461=CARTESIAN_POINT('Ctrl Pts',(34.8216932892968,-64.2085257702884,
0.));
#126462=CARTESIAN_POINT('Ctrl Pts',(34.8188336622418,-64.1828703754236,
0.));
#126463=CARTESIAN_POINT('Ctrl Pts',(34.8159542418374,-64.1572559542086,
0.));
#126464=CARTESIAN_POINT('Ctrl Pts',(34.8130550915286,-64.1316826005506,
0.));
#126465=CARTESIAN_POINT('Ctrl Pts',(34.8101362750597,-64.1061504086516,
0.));
#126466=CARTESIAN_POINT('Ctrl Pts',(34.8071978564747,-64.0806594730085,
0.));
#126467=CARTESIAN_POINT('Ctrl Pts',(34.804239900121,-64.0552098884096,0.));
#126468=CARTESIAN_POINT('Ctrl Pts',(34.8012624706526,-64.0298017499294,
0.));
#126469=CARTESIAN_POINT('Ctrl Pts',(34.7982656330293,-64.0044351529402,
0.));
#126470=CARTESIAN_POINT('Ctrl Pts',(34.7952494525177,-63.9791101931162,
0.));
#126471=CARTESIAN_POINT('Ctrl Pts',(34.7922139946942,-63.9538269664366,
0.));
#126472=CARTESIAN_POINT('Ctrl Pts',(34.7891593254488,-63.9285855691845,
0.));
#126473=CARTESIAN_POINT('Ctrl Pts',(34.7860855109911,-63.9033860979435,
0.));
#126474=CARTESIAN_POINT('Ctrl Pts',(34.7829926178496,-63.8782286496062,
0.));
#126475=CARTESIAN_POINT('Ctrl Pts',(34.7798807128714,-63.8531133213793,
0.));
#126476=CARTESIAN_POINT('Ctrl Pts',(34.7767498632242,-63.8280402107856,
0.));
#126477=CARTESIAN_POINT('Ctrl Pts',(34.7736001363992,-63.8030094156639,
0.));
#126478=CARTESIAN_POINT('Ctrl Pts',(34.7704316002171,-63.778021034163,0.));
#126479=CARTESIAN_POINT('Ctrl Pts',(34.7672443228274,-63.7530751647494,
0.));
#126480=CARTESIAN_POINT('Ctrl Pts',(34.76403837271,-63.7281719062149,0.));
#126481=CARTESIAN_POINT('Ctrl Pts',(34.7608138186759,-63.7033113576786,
0.));
#126482=CARTESIAN_POINT('Ctrl Pts',(34.7575707298713,-63.6784936185885,
0.));
#126483=CARTESIAN_POINT('Ctrl Pts',(34.7543091757833,-63.6537187887159,
0.));
#126484=CARTESIAN_POINT('Ctrl Pts',(34.7510292262406,-63.6289869681604,
0.));
#126485=CARTESIAN_POINT('Ctrl Pts',(34.7477309514136,-63.6042982573588,
0.));
#126486=CARTESIAN_POINT('Ctrl Pts',(34.744414421816,-63.5796527570872,0.));
#126487=CARTESIAN_POINT('Ctrl Pts',(34.741079708308,-63.5550505684626,0.));
#126488=CARTESIAN_POINT('Ctrl Pts',(34.7377268821025,-63.5304917929386,
0.));
#126489=CARTESIAN_POINT('Ctrl Pts',(34.7343560147667,-63.505976532309,0.));
#126490=CARTESIAN_POINT('Ctrl Pts',(34.7309671782213,-63.4815048887166,
0.));
#126491=CARTESIAN_POINT('Ctrl Pts',(34.7275604447438,-63.4570769646569,
0.));
#126492=CARTESIAN_POINT('Ctrl Pts',(34.72413588697,-63.4326928629795,0.));
#126493=CARTESIAN_POINT('Ctrl Pts',(34.7206935779007,-63.4083526868837,
0.));
#126494=CARTESIAN_POINT('Ctrl Pts',(34.7172335909038,-63.3840565399208,
0.));
#126495=CARTESIAN_POINT('Ctrl Pts',(34.7137559997145,-63.3598045260053,
0.));
#126496=CARTESIAN_POINT('Ctrl Pts',(34.7102608784374,-63.3355967494172,
0.));
#126497=CARTESIAN_POINT('Ctrl Pts',(34.706748301549,-63.3114333148048,0.));
#126498=CARTESIAN_POINT('Ctrl Pts',(34.703218343904,-63.2873143271807,0.));
#126499=CARTESIAN_POINT('Ctrl Pts',(34.6996710807378,-63.2632398919225,
0.));
#126500=CARTESIAN_POINT('Ctrl Pts',(34.6961065876666,-63.2392101147847,
0.));
#126501=CARTESIAN_POINT('Ctrl Pts',(34.6925249406896,-63.2152251019012,
0.));
#126502=CARTESIAN_POINT('Ctrl Pts',(34.6889262161924,-63.1912849597888,
0.));
#126503=CARTESIAN_POINT('Ctrl Pts',(34.6853104909518,-63.1673897953429,
0.));
#126504=CARTESIAN_POINT('Ctrl Pts',(34.6816778421402,-63.1435397158389,
0.));
#126505=CARTESIAN_POINT('Ctrl Pts',(34.6780283473251,-63.119734828943,0.));
#126506=CARTESIAN_POINT('Ctrl Pts',(34.674362084472,-63.0959752427168,0.));
#126507=CARTESIAN_POINT('Ctrl Pts',(34.670679131947,-63.0722610656194,0.));
#126508=CARTESIAN_POINT('Ctrl Pts',(34.6669795685228,-63.0485924065045,
0.));
#126509=CARTESIAN_POINT('Ctrl Pts',(34.6632634733824,-63.0249693746208,
0.));
#126510=CARTESIAN_POINT('Ctrl Pts',(34.659530926119,-63.0013920796235,0.));
#126511=CARTESIAN_POINT('Ctrl Pts',(34.6557820067392,-62.9778606315783,
0.));
#126512=CARTESIAN_POINT('Ctrl Pts',(34.6520167956655,-62.9543751409646,
0.));
#126513=CARTESIAN_POINT('Ctrl Pts',(34.6482353737424,-62.9309357186717,
0.));
#126514=CARTESIAN_POINT('Ctrl Pts',(34.644437822241,-62.9075424760015,0.));
#126515=CARTESIAN_POINT('Ctrl Pts',(34.6406242228591,-62.8841955246794,
0.));
#126516=CARTESIAN_POINT('Ctrl Pts',(34.6367946577234,-62.8608949768571,
0.));
#126517=CARTESIAN_POINT('Ctrl Pts',(34.6329492093935,-62.8376409451175,
0.));
#126518=CARTESIAN_POINT('Ctrl Pts',(34.6290879608672,-62.8144335424697,
0.));
#126519=CARTESIAN_POINT('Ctrl Pts',(34.6252109955852,-62.7912728823518,
0.));
#126520=CARTESIAN_POINT('Ctrl Pts',(34.6213183974317,-62.7681590786429,
0.));
#126521=CARTESIAN_POINT('Ctrl Pts',(34.6174102507374,-62.7450922456676,
0.));
#126522=CARTESIAN_POINT('Ctrl Pts',(34.6134866402836,-62.7220724981995,
0.));
#126523=CARTESIAN_POINT('Ctrl Pts',(34.6095476513076,-62.6990999514563,
0.));
#126524=CARTESIAN_POINT('Ctrl Pts',(34.6055933695069,-62.6761747211037,
0.));
#126525=CARTESIAN_POINT('Ctrl Pts',(34.6016238810398,-62.6532969232658,
0.));
#126526=CARTESIAN_POINT('Ctrl Pts',(34.5976392725296,-62.6304666745307,
0.));
#126527=CARTESIAN_POINT('Ctrl Pts',(34.5936396310679,-62.6076840919536,
0.));
#126528=CARTESIAN_POINT('Ctrl Pts',(34.5896250442216,-62.5849492930533,
0.));
#126529=CARTESIAN_POINT('Ctrl Pts',(34.5855956000362,-62.5622623958161,
0.));
#126530=CARTESIAN_POINT('Ctrl Pts',(34.5815513870376,-62.5396235187079,
0.));
#126531=CARTESIAN_POINT('Ctrl Pts',(34.5774924942354,-62.5170327806781,
0.));
#126532=CARTESIAN_POINT('Ctrl Pts',(34.5734190111272,-62.4944903011628,
0.));
#126533=CARTESIAN_POINT('Ctrl Pts',(34.5693310277051,-62.4719962000808,
0.));
#126534=CARTESIAN_POINT('Ctrl Pts',(34.5652286344592,-62.4495505978393,
0.));
#126535=CARTESIAN_POINT('Ctrl Pts',(34.5611119223798,-62.4271536153459,
0.));
#126536=CARTESIAN_POINT('Ctrl Pts',(34.5569809829613,-62.4048053740127,
0.));
#126537=CARTESIAN_POINT('Ctrl Pts',(34.5528359082074,-62.3825059957601,
0.));
#126538=CARTESIAN_POINT('Ctrl Pts',(34.5486767906384,-62.3602556030127,
0.));
#126539=CARTESIAN_POINT('Ctrl Pts',(34.5445037232936,-62.338054318708,0.));
#126540=CARTESIAN_POINT('Ctrl Pts',(34.5403167997337,-62.3159022663058,
0.));
#126541=CARTESIAN_POINT('Ctrl Pts',(34.5361161140449,-62.2937995697926,
0.));
#126542=CARTESIAN_POINT('Ctrl Pts',(34.5319017608433,-62.2717463536828,
0.));
#126543=CARTESIAN_POINT('Ctrl Pts',(34.5276738352808,-62.2497427430135,
0.));
#126544=CARTESIAN_POINT('Ctrl Pts',(34.523432433049,-62.2277888633577,0.));
#126545=CARTESIAN_POINT('Ctrl Pts',(34.5191776503842,-62.2058848408347,
0.));
#126546=CARTESIAN_POINT('Ctrl Pts',(34.5149095840729,-62.1840308021171,
0.));
#126547=CARTESIAN_POINT('Ctrl Pts',(34.5106283314594,-62.1622268744336,
0.));
#126548=CARTESIAN_POINT('Ctrl Pts',(34.5063339904533,-62.1404731855686,
0.));
#126549=CARTESIAN_POINT('Ctrl Pts',(34.5020266595292,-62.1187698638705,
0.));
#126550=CARTESIAN_POINT('Ctrl Pts',(34.4977064377281,-62.0971170382565,
0.));
#126551=CARTESIAN_POINT('Ctrl Pts',(34.4933734246592,-62.0755148382136,
0.));
#126552=CARTESIAN_POINT('Ctrl Pts',(34.4890277205041,-62.0539633937944,
0.));
#126553=CARTESIAN_POINT('Ctrl Pts',(34.4846694260205,-62.0324628356152,
0.));
#126554=CARTESIAN_POINT('Ctrl Pts',(34.4802986425534,-62.0110132948807,
0.));
#126555=CARTESIAN_POINT('Ctrl Pts',(34.4759154720477,-61.9896149034009,
0.));
#126556=CARTESIAN_POINT('Ctrl Pts',(34.4715200170588,-61.9682677936048,
0.));
#126557=CARTESIAN_POINT('Ctrl Pts',(34.4671123807705,-61.9469720985512,
0.));
#126558=CARTESIAN_POINT('Ctrl Pts',(34.462692666996,-61.9257279519283,0.));
#126559=CARTESIAN_POINT('Ctrl Pts',(34.4582609801625,-61.9045354880424,
0.));
#126560=CARTESIAN_POINT('Ctrl Pts',(34.4538174253009,-61.883394841802,0.));
#126561=CARTESIAN_POINT('Ctrl Pts',(34.4493621080367,-61.8623061487031,
0.));
#126562=CARTESIAN_POINT('Ctrl Pts',(34.4448951345753,-61.8412695447951,
0.));
#126563=CARTESIAN_POINT('Ctrl Pts',(34.4404166117312,-61.8202851667247,
0.));
#126564=CARTESIAN_POINT('Ctrl Pts',(34.4359266469757,-61.7993531518052,
0.));
#126565=CARTESIAN_POINT('Ctrl Pts',(34.4314253484791,-61.7784736380728,
0.));
#126566=CARTESIAN_POINT('Ctrl Pts',(34.4269128251568,-61.7576467643419,
0.));
#126567=CARTESIAN_POINT('Ctrl Pts',(34.4223891867166,-61.7368726702573,
0.));
#126568=CARTESIAN_POINT('Ctrl Pts',(34.4178545435753,-61.7161514961892,
0.));
#126569=CARTESIAN_POINT('Ctrl Pts',(34.4133090067696,-61.6954833831158,
0.));
#126570=CARTESIAN_POINT('Ctrl Pts',(34.4087526878814,-61.674868472521,0.));
#126571=CARTESIAN_POINT('Ctrl Pts',(34.4041856989328,-61.6543069062436,
0.));
#126572=CARTESIAN_POINT('Ctrl Pts',(34.399608152377,-61.6337988264586,0.));
#126573=CARTESIAN_POINT('Ctrl Pts',(34.3950201613446,-61.6133443760168,
0.));
#126574=CARTESIAN_POINT('Ctrl Pts',(34.3904218398641,-61.5929436987419,
0.));
#126575=CARTESIAN_POINT('Ctrl Pts',(34.3858133030511,-61.5725969396817,
0.));
#126576=CARTESIAN_POINT('Ctrl Pts',(34.3811946674179,-61.5523042455128,
0.));
#126577=CARTESIAN_POINT('Ctrl Pts',(34.3765660506659,-61.5320657642601,
0.));
#126578=CARTESIAN_POINT('Ctrl Pts',(34.3719275711179,-61.511881644541,0.));
#126579=CARTESIAN_POINT('Ctrl Pts',(34.3672793472463,-61.4917520349276,
0.));
#126580=CARTESIAN_POINT('Ctrl Pts',(34.3626214971903,-61.4716770832924,
0.));
#126581=CARTESIAN_POINT('Ctrl Pts',(34.357954138202,-61.4516569360499,0.));
#126582=CARTESIAN_POINT('Ctrl Pts',(34.3532773877111,-61.4316917395959,
0.));
#126583=CARTESIAN_POINT('Ctrl Pts',(34.3485913645991,-61.4117816420251,
0.));
#126584=CARTESIAN_POINT('Ctrl Pts',(34.34389619024,-61.3919267945294,0.));
#126585=CARTESIAN_POINT('Ctrl Pts',(34.339191990012,-61.3721273534222,0.));
#126586=CARTESIAN_POINT('Ctrl Pts',(34.3344788934337,-61.3523834803144,
0.));
#126587=CARTESIAN_POINT('Ctrl Pts',(34.3297570310126,-61.3326953378817,
0.));
#126588=CARTESIAN_POINT('Ctrl Pts',(34.3250265314761,-61.3130630861375,
0.));
#126589=CARTESIAN_POINT('Ctrl Pts',(34.3202875193629,-61.2934868791876,
0.));
#126590=CARTESIAN_POINT('Ctrl Pts',(34.3155401111776,-61.2739668600416,
0.));
#126591=CARTESIAN_POINT('Ctrl Pts',(34.3107844191081,-61.2545031656196,
0.));
#126592=CARTESIAN_POINT('Ctrl Pts',(34.3060205584093,-61.2350959366987,
0.));
#126593=CARTESIAN_POINT('Ctrl Pts',(34.3012486533473,-61.2157453259108,
0.));
#126594=CARTESIAN_POINT('Ctrl Pts',(34.296468844362,-61.1964515073823,0.));
#126595=CARTESIAN_POINT('Ctrl Pts',(34.2916812929674,-61.1772146833083,
0.));
#126596=CARTESIAN_POINT('Ctrl Pts',(34.2868861666301,-61.15803506354,0.));
#126597=CARTESIAN_POINT('Ctrl Pts',(34.2820836244425,-61.1389128461815,
0.));
#126598=CARTESIAN_POINT('Ctrl Pts',(34.2772738038811,-61.119848199783,0.));
#126599=CARTESIAN_POINT('Ctrl Pts',(34.2724568037373,-61.1008412400231,
0.));
#126600=CARTESIAN_POINT('Ctrl Pts',(34.2676326825845,-61.0818920286645,
0.));
#126601=CARTESIAN_POINT('Ctrl Pts',(34.2637677132139,-61.0667788793594,
0.));
#126602=CARTESIAN_POINT('Ctrl Pts',(34.260865800176,-61.0554700177207,0.));
#126603=CARTESIAN_POINT('Ctrl Pts',(34.2589297755482,-61.0479423318803,
0.));
#126604=CARTESIAN_POINT('Ctrl Pts',(34.2579614092496,-61.0441813777723,
0.));
#126605=CARTESIAN_POINT('Ctrl Pts',(29.0861280018229,-68.5875145916629,
0.));
#126606=CARTESIAN_POINT('Ctrl Pts',(29.0861280018229,-68.5875145916629,
12.));
#126607=CARTESIAN_POINT('Ctrl Pts',(29.0863005247838,-68.5819214834737,
0.));
#126608=CARTESIAN_POINT('Ctrl Pts',(29.0863005247838,-68.5819214834737,
12.));
#126609=CARTESIAN_POINT('Ctrl Pts',(29.0866429722093,-68.5707386600636,
0.));
#126610=CARTESIAN_POINT('Ctrl Pts',(29.0866429722093,-68.5707386600636,
12.));
#126611=CARTESIAN_POINT('Ctrl Pts',(29.0871488478588,-68.5539746038542,
0.));
#126612=CARTESIAN_POINT('Ctrl Pts',(29.0871488478588,-68.5539746038542,
12.));
#126613=CARTESIAN_POINT('Ctrl Pts',(29.0878077571086,-68.5316428875424,
0.));
#126614=CARTESIAN_POINT('Ctrl Pts',(29.0878077571086,-68.5316428875424,
12.));
#126615=CARTESIAN_POINT('Ctrl Pts',(29.0886054060562,-68.5037621824171,
0.));
#126616=CARTESIAN_POINT('Ctrl Pts',(29.0886054060562,-68.5037621824171,
12.));
#126617=CARTESIAN_POINT('Ctrl Pts',(29.0893770688944,-68.4759154367939,
0.));
#126618=CARTESIAN_POINT('Ctrl Pts',(29.0893770688944,-68.4759154367939,
12.));
#126619=CARTESIAN_POINT('Ctrl Pts',(29.0901227535306,-68.4481026830931,
0.));
#126620=CARTESIAN_POINT('Ctrl Pts',(29.0901227535306,-68.4481026830931,
12.));
#126621=CARTESIAN_POINT('Ctrl Pts',(29.090842477089,-68.4203239694612,0.));
#126622=CARTESIAN_POINT('Ctrl Pts',(29.090842477089,-68.4203239694612,12.));
#126623=CARTESIAN_POINT('Ctrl Pts',(29.0915362699455,-68.3925793637995,
0.));
#126624=CARTESIAN_POINT('Ctrl Pts',(29.0915362699455,-68.3925793637995,
12.));
#126625=CARTESIAN_POINT('Ctrl Pts',(29.0922041749293,-68.364868951893,0.));
#126626=CARTESIAN_POINT('Ctrl Pts',(29.0922041749293,-68.364868951893,12.));
#126627=CARTESIAN_POINT('Ctrl Pts',(29.0928462428145,-68.3371928310161,
0.));
#126628=CARTESIAN_POINT('Ctrl Pts',(29.0928462428145,-68.3371928310161,
12.));
#126629=CARTESIAN_POINT('Ctrl Pts',(29.0934625288409,-68.3095511047769,
0.));
#126630=CARTESIAN_POINT('Ctrl Pts',(29.0934625288409,-68.3095511047769,
12.));
#126631=CARTESIAN_POINT('Ctrl Pts',(29.0940530889149,-68.2819438775953,
0.));
#126632=CARTESIAN_POINT('Ctrl Pts',(29.0940530889149,-68.2819438775953,
12.));
#126633=CARTESIAN_POINT('Ctrl Pts',(29.0946179757167,-68.2543712489906,
0.));
#126634=CARTESIAN_POINT('Ctrl Pts',(29.0946179757167,-68.2543712489906,
12.));
#126635=CARTESIAN_POINT('Ctrl Pts',(29.0951572355397,-68.2268333089617,
0.));
#126636=CARTESIAN_POINT('Ctrl Pts',(29.0951572355397,-68.2268333089617,
12.));
#126637=CARTESIAN_POINT('Ctrl Pts',(29.0956709104627,-68.1993301412061,
0.));
#126638=CARTESIAN_POINT('Ctrl Pts',(29.0956709104627,-68.1993301412061,
12.));
#126639=CARTESIAN_POINT('Ctrl Pts',(29.0961590399046,-68.1718618254281,
0.));
#126640=CARTESIAN_POINT('Ctrl Pts',(29.0961590399046,-68.1718618254281,
12.));
#126641=CARTESIAN_POINT('Ctrl Pts',(29.0966216624743,-68.1444284400742,
0.));
#126642=CARTESIAN_POINT('Ctrl Pts',(29.0966216624743,-68.1444284400742,
12.));
#126643=CARTESIAN_POINT('Ctrl Pts',(29.0970588175728,-68.1170300646987,
0.));
#126644=CARTESIAN_POINT('Ctrl Pts',(29.0970588175728,-68.1170300646987,
12.));
#126645=CARTESIAN_POINT('Ctrl Pts',(29.0974705474258,-68.0896667829568,
0.));
#126646=CARTESIAN_POINT('Ctrl Pts',(29.0974705474258,-68.0896667829568,
12.));
#126647=CARTESIAN_POINT('Ctrl Pts',(29.0978568968656,-68.0623386822863,
0.));
#126648=CARTESIAN_POINT('Ctrl Pts',(29.0978568968656,-68.0623386822863,
12.));
#126649=CARTESIAN_POINT('Ctrl Pts',(29.0982179124097,-68.0350458525551,
0.));
#126650=CARTESIAN_POINT('Ctrl Pts',(29.0982179124097,-68.0350458525551,
12.));
#126651=CARTESIAN_POINT('Ctrl Pts',(29.098553641553,-68.0077883850121,0.));
#126652=CARTESIAN_POINT('Ctrl Pts',(29.098553641553,-68.0077883850121,12.));
#126653=CARTESIAN_POINT('Ctrl Pts',(29.0988641320246,-67.9805663711855,
0.));
#126654=CARTESIAN_POINT('Ctrl Pts',(29.0988641320246,-67.9805663711855,
12.));
#126655=CARTESIAN_POINT('Ctrl Pts',(29.0991494309404,-67.9533799016148,
0.));
#126656=CARTESIAN_POINT('Ctrl Pts',(29.0991494309404,-67.9533799016148,
12.));
#126657=CARTESIAN_POINT('Ctrl Pts',(29.099409584422,-67.9262290652829,0.));
#126658=CARTESIAN_POINT('Ctrl Pts',(29.099409584422,-67.9262290652829,12.));
#126659=CARTESIAN_POINT('Ctrl Pts',(29.0996446380626,-67.8991139503193,
0.));
#126660=CARTESIAN_POINT('Ctrl Pts',(29.0996446380626,-67.8991139503193,
12.));
#126661=CARTESIAN_POINT('Ctrl Pts',(29.0998546372032,-67.8720346444124,
0.));
#126662=CARTESIAN_POINT('Ctrl Pts',(29.0998546372032,-67.8720346444124,
12.));
#126663=CARTESIAN_POINT('Ctrl Pts',(29.1000396272867,-67.8449912353329,
0.));
#126664=CARTESIAN_POINT('Ctrl Pts',(29.1000396272867,-67.8449912353329,
12.));
#126665=CARTESIAN_POINT('Ctrl Pts',(29.1001996541841,-67.8179838114099,
0.));
#126666=CARTESIAN_POINT('Ctrl Pts',(29.1001996541841,-67.8179838114099,
12.));
#126667=CARTESIAN_POINT('Ctrl Pts',(29.1003347645293,-67.7910124620135,
0.));
#126668=CARTESIAN_POINT('Ctrl Pts',(29.1003347645293,-67.7910124620135,
12.));
#126669=CARTESIAN_POINT('Ctrl Pts',(29.1004450055642,-67.7640772773388,
0.));
#126670=CARTESIAN_POINT('Ctrl Pts',(29.1004450055642,-67.7640772773388,
12.));
#126671=CARTESIAN_POINT('Ctrl Pts',(29.1005304249986,-67.7371783482035,
0.));
#126672=CARTESIAN_POINT('Ctrl Pts',(29.1005304249986,-67.7371783482035,
12.));
#126673=CARTESIAN_POINT('Ctrl Pts',(29.1005910708624,-67.7103157658296,
0.));
#126674=CARTESIAN_POINT('Ctrl Pts',(29.1005910708624,-67.7103157658296,
12.));
#126675=CARTESIAN_POINT('Ctrl Pts',(29.1006269913747,-67.6834896216461,
0.));
#126676=CARTESIAN_POINT('Ctrl Pts',(29.1006269913747,-67.6834896216461,
12.));
#126677=CARTESIAN_POINT('Ctrl Pts',(29.1006382347814,-67.6567000070326,
0.));
#126678=CARTESIAN_POINT('Ctrl Pts',(29.1006382347814,-67.6567000070326,
12.));
#126679=CARTESIAN_POINT('Ctrl Pts',(29.100624849358,-67.6299470133295,0.));
#126680=CARTESIAN_POINT('Ctrl Pts',(29.100624849358,-67.6299470133295,12.));
#126681=CARTESIAN_POINT('Ctrl Pts',(29.1005868834866,-67.6032307319623,
0.));
#126682=CARTESIAN_POINT('Ctrl Pts',(29.1005868834866,-67.6032307319623,
12.));
#126683=CARTESIAN_POINT('Ctrl Pts',(29.1005243857138,-67.5765512545282,
0.));
#126684=CARTESIAN_POINT('Ctrl Pts',(29.1005243857138,-67.5765512545282,
12.));
#126685=CARTESIAN_POINT('Ctrl Pts',(29.1004374048147,-67.5499086728889,
0.));
#126686=CARTESIAN_POINT('Ctrl Pts',(29.1004374048147,-67.5499086728889,
12.));
#126687=CARTESIAN_POINT('Ctrl Pts',(29.1003259898681,-67.5233030792704,
0.));
#126688=CARTESIAN_POINT('Ctrl Pts',(29.1003259898681,-67.5233030792704,
12.));
#126689=CARTESIAN_POINT('Ctrl Pts',(29.1001901902908,-67.4967345663096,
0.));
#126690=CARTESIAN_POINT('Ctrl Pts',(29.1001901902908,-67.4967345663096,
12.));
#126691=CARTESIAN_POINT('Ctrl Pts',(29.1000300557955,-67.4702032270049,
0.));
#126692=CARTESIAN_POINT('Ctrl Pts',(29.1000300557955,-67.4702032270049,
12.));
#126693=CARTESIAN_POINT('Ctrl Pts',(29.0998456363682,-67.4437091546859,
0.));
#126694=CARTESIAN_POINT('Ctrl Pts',(29.0998456363682,-67.4437091546859,
12.));
#126695=CARTESIAN_POINT('Ctrl Pts',(29.0996369822418,-67.4172524429728,
0.));
#126696=CARTESIAN_POINT('Ctrl Pts',(29.0996369822418,-67.4172524429728,
12.));
#126697=CARTESIAN_POINT('Ctrl Pts',(29.0994041438718,-67.3908331857323,
0.));
#126698=CARTESIAN_POINT('Ctrl Pts',(29.0994041438718,-67.3908331857323,
12.));
#126699=CARTESIAN_POINT('Ctrl Pts',(29.0991471719176,-67.3644514770387,
0.));
#126700=CARTESIAN_POINT('Ctrl Pts',(29.0991471719176,-67.3644514770387,
12.));
#126701=CARTESIAN_POINT('Ctrl Pts',(29.098866117253,-67.3381074112027,0.));
#126702=CARTESIAN_POINT('Ctrl Pts',(29.098866117253,-67.3381074112027,12.));
#126703=CARTESIAN_POINT('Ctrl Pts',(29.098561030977,-67.311801082792,0.));
#126704=CARTESIAN_POINT('Ctrl Pts',(29.098561030977,-67.311801082792,12.));
#126705=CARTESIAN_POINT('Ctrl Pts',(29.0982319644276,-67.2855325866517,
0.));
#126706=CARTESIAN_POINT('Ctrl Pts',(29.0982319644276,-67.2855325866517,
12.));
#126707=CARTESIAN_POINT('Ctrl Pts',(29.0978789691962,-67.2593020179209,
0.));
#126708=CARTESIAN_POINT('Ctrl Pts',(29.0978789691962,-67.2593020179209,
12.));
#126709=CARTESIAN_POINT('Ctrl Pts',(29.0975020971469,-67.2331094720471,
0.));
#126710=CARTESIAN_POINT('Ctrl Pts',(29.0975020971469,-67.2331094720471,
12.));
#126711=CARTESIAN_POINT('Ctrl Pts',(29.097101400413,-67.2069550447884,0.));
#126712=CARTESIAN_POINT('Ctrl Pts',(29.097101400413,-67.2069550447884,12.));
#126713=CARTESIAN_POINT('Ctrl Pts',(29.096676931389,-67.1808388322109,0.));
#126714=CARTESIAN_POINT('Ctrl Pts',(29.096676931389,-67.1808388322109,12.));
#126715=CARTESIAN_POINT('Ctrl Pts',(29.0962287427273,-67.1547609306843,
0.));
#126716=CARTESIAN_POINT('Ctrl Pts',(29.0962287427273,-67.1547609306843,
12.));
#126717=CARTESIAN_POINT('Ctrl Pts',(29.0957568873358,-67.1287214368746,
0.));
#126718=CARTESIAN_POINT('Ctrl Pts',(29.0957568873358,-67.1287214368746,
12.));
#126719=CARTESIAN_POINT('Ctrl Pts',(29.0952614183779,-67.1027204477311,
0.));
#126720=CARTESIAN_POINT('Ctrl Pts',(29.0952614183779,-67.1027204477311,
12.));
#126721=CARTESIAN_POINT('Ctrl Pts',(29.0947423892726,-67.0767580604879,
0.));
#126722=CARTESIAN_POINT('Ctrl Pts',(29.0947423892726,-67.0767580604879,
12.));
#126723=CARTESIAN_POINT('Ctrl Pts',(29.0941998536958,-67.0508343726777,
0.));
#126724=CARTESIAN_POINT('Ctrl Pts',(29.0941998536958,-67.0508343726777,
12.));
#126725=CARTESIAN_POINT('Ctrl Pts',(29.0936338655828,-67.0249494821363,
0.));
#126726=CARTESIAN_POINT('Ctrl Pts',(29.0936338655828,-67.0249494821363,
12.));
#126727=CARTESIAN_POINT('Ctrl Pts',(29.0930444791328,-66.9991034870083,
0.));
#126728=CARTESIAN_POINT('Ctrl Pts',(29.0930444791328,-66.9991034870083,
12.));
#126729=CARTESIAN_POINT('Ctrl Pts',(29.092431748817,-66.9732964857466,0.));
#126730=CARTESIAN_POINT('Ctrl Pts',(29.092431748817,-66.9732964857466,12.));
#126731=CARTESIAN_POINT('Ctrl Pts',(29.0917957293826,-66.9475285771135,
0.));
#126732=CARTESIAN_POINT('Ctrl Pts',(29.0917957293826,-66.9475285771135,
12.));
#126733=CARTESIAN_POINT('Ctrl Pts',(29.0911364758486,-66.9217998601885,
0.));
#126734=CARTESIAN_POINT('Ctrl Pts',(29.0911364758486,-66.9217998601885,
12.));
#126735=CARTESIAN_POINT('Ctrl Pts',(29.0904540435065,-66.8961104343707,
0.));
#126736=CARTESIAN_POINT('Ctrl Pts',(29.0904540435065,-66.8961104343707,
12.));
#126737=CARTESIAN_POINT('Ctrl Pts',(29.0897484879207,-66.8704603993794,
0.));
#126738=CARTESIAN_POINT('Ctrl Pts',(29.0897484879207,-66.8704603993794,
12.));
#126739=CARTESIAN_POINT('Ctrl Pts',(29.0890198649323,-66.8448498552503,
0.));
#126740=CARTESIAN_POINT('Ctrl Pts',(29.0890198649323,-66.8448498552503,
12.));
#126741=CARTESIAN_POINT('Ctrl Pts',(29.088268230663,-66.8192789023312,0.));
#126742=CARTESIAN_POINT('Ctrl Pts',(29.088268230663,-66.8192789023312,12.));
#126743=CARTESIAN_POINT('Ctrl Pts',(29.0874936415131,-66.793747641293,0.));
#126744=CARTESIAN_POINT('Ctrl Pts',(29.0874936415131,-66.793747641293,12.));
#126745=CARTESIAN_POINT('Ctrl Pts',(29.0866961541625,-66.7682561731342,
0.));
#126746=CARTESIAN_POINT('Ctrl Pts',(29.0866961541625,-66.7682561731342,
12.));
#126747=CARTESIAN_POINT('Ctrl Pts',(29.0858758255728,-66.7428045991841,
0.));
#126748=CARTESIAN_POINT('Ctrl Pts',(29.0858758255728,-66.7428045991841,
12.));
#126749=CARTESIAN_POINT('Ctrl Pts',(29.0850327129916,-66.7173930211022,
0.));
#126750=CARTESIAN_POINT('Ctrl Pts',(29.0850327129916,-66.7173930211022,
12.));
#126751=CARTESIAN_POINT('Ctrl Pts',(29.0841668739588,-66.6920215408751,
0.));
#126752=CARTESIAN_POINT('Ctrl Pts',(29.0841668739588,-66.6920215408751,
12.));
#126753=CARTESIAN_POINT('Ctrl Pts',(29.0832783663049,-66.6666902608249,
0.));
#126754=CARTESIAN_POINT('Ctrl Pts',(29.0832783663049,-66.6666902608249,
12.));
#126755=CARTESIAN_POINT('Ctrl Pts',(29.0823672481507,-66.6413992836147,
0.));
#126756=CARTESIAN_POINT('Ctrl Pts',(29.0823672481507,-66.6413992836147,
12.));
#126757=CARTESIAN_POINT('Ctrl Pts',(29.0814335779084,-66.6161487122502,
0.));
#126758=CARTESIAN_POINT('Ctrl Pts',(29.0814335779084,-66.6161487122502,
12.));
#126759=CARTESIAN_POINT('Ctrl Pts',(29.0804774142853,-66.59093865008,0.));
#126760=CARTESIAN_POINT('Ctrl Pts',(29.0804774142853,-66.59093865008,12.));
#126761=CARTESIAN_POINT('Ctrl Pts',(29.0794988162897,-66.5657692007906,
0.));
#126762=CARTESIAN_POINT('Ctrl Pts',(29.0794988162897,-66.5657692007906,
12.));
#126763=CARTESIAN_POINT('Ctrl Pts',(29.07849784323,-66.5406404684132,0.));
#126764=CARTESIAN_POINT('Ctrl Pts',(29.07849784323,-66.5406404684132,12.));
#126765=CARTESIAN_POINT('Ctrl Pts',(29.0774745547151,-66.5155525573323,
0.));
#126766=CARTESIAN_POINT('Ctrl Pts',(29.0774745547151,-66.5155525573323,
12.));
#126767=CARTESIAN_POINT('Ctrl Pts',(29.0764290106554,-66.4905055722868,
0.));
#126768=CARTESIAN_POINT('Ctrl Pts',(29.0764290106554,-66.4905055722868,
12.));
#126769=CARTESIAN_POINT('Ctrl Pts',(29.0753612712665,-66.4654996183731,
0.));
#126770=CARTESIAN_POINT('Ctrl Pts',(29.0753612712665,-66.4654996183731,
12.));
#126771=CARTESIAN_POINT('Ctrl Pts',(29.0742713970755,-66.4405348010388,
0.));
#126772=CARTESIAN_POINT('Ctrl Pts',(29.0742713970755,-66.4405348010388,
12.));
#126773=CARTESIAN_POINT('Ctrl Pts',(29.0731594489211,-66.4156112260887,
0.));
#126774=CARTESIAN_POINT('Ctrl Pts',(29.0731594489211,-66.4156112260887,
12.));
#126775=CARTESIAN_POINT('Ctrl Pts',(29.072025487953,-66.3907289996932,0.));
#126776=CARTESIAN_POINT('Ctrl Pts',(29.072025487953,-66.3907289996932,12.));
#126777=CARTESIAN_POINT('Ctrl Pts',(29.0708695756334,-66.3658882283903,
0.));
#126778=CARTESIAN_POINT('Ctrl Pts',(29.0708695756334,-66.3658882283903,
12.));
#126779=CARTESIAN_POINT('Ctrl Pts',(29.0696917737399,-66.3410890190884,
0.));
#126780=CARTESIAN_POINT('Ctrl Pts',(29.0696917737399,-66.3410890190884,
12.));
#126781=CARTESIAN_POINT('Ctrl Pts',(29.0684921443721,-66.3163314790615,
0.));
#126782=CARTESIAN_POINT('Ctrl Pts',(29.0684921443721,-66.3163314790615,
12.));
#126783=CARTESIAN_POINT('Ctrl Pts',(29.0672707499529,-66.2916157159536,
0.));
#126784=CARTESIAN_POINT('Ctrl Pts',(29.0672707499529,-66.2916157159536,
12.));
#126785=CARTESIAN_POINT('Ctrl Pts',(29.0660276532273,-66.2669418377871,
0.));
#126786=CARTESIAN_POINT('Ctrl Pts',(29.0660276532273,-66.2669418377871,
12.));
#126787=CARTESIAN_POINT('Ctrl Pts',(29.0647629172644,-66.2423099529669,
0.));
#126788=CARTESIAN_POINT('Ctrl Pts',(29.0647629172644,-66.2423099529669,
12.));
#126789=CARTESIAN_POINT('Ctrl Pts',(29.0634766054598,-66.2177201702818,
0.));
#126790=CARTESIAN_POINT('Ctrl Pts',(29.0634766054598,-66.2177201702818,
12.));
#126791=CARTESIAN_POINT('Ctrl Pts',(29.062168781542,-66.1931725989008,0.));
#126792=CARTESIAN_POINT('Ctrl Pts',(29.062168781542,-66.1931725989008,12.));
#126793=CARTESIAN_POINT('Ctrl Pts',(29.0608395095746,-66.1686673483757,
0.));
#126794=CARTESIAN_POINT('Ctrl Pts',(29.0608395095746,-66.1686673483757,
12.));
#126795=CARTESIAN_POINT('Ctrl Pts',(29.0594888539557,-66.144204528652,0.));
#126796=CARTESIAN_POINT('Ctrl Pts',(29.0594888539557,-66.144204528652,12.));
#126797=CARTESIAN_POINT('Ctrl Pts',(29.058116879419,-66.1197842500714,0.));
#126798=CARTESIAN_POINT('Ctrl Pts',(29.058116879419,-66.1197842500714,12.));
#126799=CARTESIAN_POINT('Ctrl Pts',(29.0567236510372,-66.0954066233752,
0.));
#126800=CARTESIAN_POINT('Ctrl Pts',(29.0567236510372,-66.0954066233752,
12.));
#126801=CARTESIAN_POINT('Ctrl Pts',(29.0553092342274,-66.0710717597003,
0.));
#126802=CARTESIAN_POINT('Ctrl Pts',(29.0553092342274,-66.0710717597003,
12.));
#126803=CARTESIAN_POINT('Ctrl Pts',(29.0538736947547,-66.0467797705806,
0.));
#126804=CARTESIAN_POINT('Ctrl Pts',(29.0538736947547,-66.0467797705806,
12.));
#126805=CARTESIAN_POINT('Ctrl Pts',(29.0524170987302,-66.0225307679584,
0.));
#126806=CARTESIAN_POINT('Ctrl Pts',(29.0524170987302,-66.0225307679584,
12.));
#126807=CARTESIAN_POINT('Ctrl Pts',(29.0509395126141,-65.9983248641877,
0.));
#126808=CARTESIAN_POINT('Ctrl Pts',(29.0509395126141,-65.9983248641877,
12.));
#126809=CARTESIAN_POINT('Ctrl Pts',(29.0494410032173,-65.9741621720372,
0.));
#126810=CARTESIAN_POINT('Ctrl Pts',(29.0494410032173,-65.9741621720372,
12.));
#126811=CARTESIAN_POINT('Ctrl Pts',(29.0479216377082,-65.9500428046873,
0.));
#126812=CARTESIAN_POINT('Ctrl Pts',(29.0479216377082,-65.9500428046873,
12.));
#126813=CARTESIAN_POINT('Ctrl Pts',(29.0463814836158,-65.925966875731,0.));
#126814=CARTESIAN_POINT('Ctrl Pts',(29.0463814836158,-65.925966875731,12.));
#126815=CARTESIAN_POINT('Ctrl Pts',(29.0448206088288,-65.9019344991854,
0.));
#126816=CARTESIAN_POINT('Ctrl Pts',(29.0448206088288,-65.9019344991854,
12.));
#126817=CARTESIAN_POINT('Ctrl Pts',(29.0432390815976,-65.8779457894959,
0.));
#126818=CARTESIAN_POINT('Ctrl Pts',(29.0432390815976,-65.8779457894959,
12.));
#126819=CARTESIAN_POINT('Ctrl Pts',(29.0416369705375,-65.854000861539,0.));
#126820=CARTESIAN_POINT('Ctrl Pts',(29.0416369705375,-65.854000861539,12.));
#126821=CARTESIAN_POINT('Ctrl Pts',(29.040014344634,-65.8300998306198,0.));
#126822=CARTESIAN_POINT('Ctrl Pts',(29.040014344634,-65.8300998306198,12.));
#126823=CARTESIAN_POINT('Ctrl Pts',(29.0383712732473,-65.8062428124723,
0.));
#126824=CARTESIAN_POINT('Ctrl Pts',(29.0383712732473,-65.8062428124723,
12.));
#126825=CARTESIAN_POINT('Ctrl Pts',(29.0367078261107,-65.7824299232715,
0.));
#126826=CARTESIAN_POINT('Ctrl Pts',(29.0367078261107,-65.7824299232715,
12.));
#126827=CARTESIAN_POINT('Ctrl Pts',(29.0350240733332,-65.7586612796375,
0.));
#126828=CARTESIAN_POINT('Ctrl Pts',(29.0350240733332,-65.7586612796375,
12.));
#126829=CARTESIAN_POINT('Ctrl Pts',(29.0333200854026,-65.7349369986382,
0.));
#126830=CARTESIAN_POINT('Ctrl Pts',(29.0333200854026,-65.7349369986382,
12.));
#126831=CARTESIAN_POINT('Ctrl Pts',(29.0315959331911,-65.7112571977874,
0.));
#126832=CARTESIAN_POINT('Ctrl Pts',(29.0315959331911,-65.7112571977874,
12.));
#126833=CARTESIAN_POINT('Ctrl Pts',(29.0298516879599,-65.6876219950465,
0.));
#126834=CARTESIAN_POINT('Ctrl Pts',(29.0298516879599,-65.6876219950465,
12.));
#126835=CARTESIAN_POINT('Ctrl Pts',(29.0280874213584,-65.6640315088361,
0.));
#126836=CARTESIAN_POINT('Ctrl Pts',(29.0280874213584,-65.6640315088361,
12.));
#126837=CARTESIAN_POINT('Ctrl Pts',(29.0263032054261,-65.6404858580391,
0.));
#126838=CARTESIAN_POINT('Ctrl Pts',(29.0263032054261,-65.6404858580391,
12.));
#126839=CARTESIAN_POINT('Ctrl Pts',(29.0244991125961,-65.6169851620054,
0.));
#126840=CARTESIAN_POINT('Ctrl Pts',(29.0244991125961,-65.6169851620054,
12.));
#126841=CARTESIAN_POINT('Ctrl Pts',(29.0226752157013,-65.593529540548,0.));
#126842=CARTESIAN_POINT('Ctrl Pts',(29.0226752157013,-65.593529540548,12.));
#126843=CARTESIAN_POINT('Ctrl Pts',(29.0208315879778,-65.5701191139455,
0.));
#126844=CARTESIAN_POINT('Ctrl Pts',(29.0208315879778,-65.5701191139455,
12.));
#126845=CARTESIAN_POINT('Ctrl Pts',(29.0189683030654,-65.5467540029546,
0.));
#126846=CARTESIAN_POINT('Ctrl Pts',(29.0189683030654,-65.5467540029546,
12.));
#126847=CARTESIAN_POINT('Ctrl Pts',(29.01708543501,-65.523434328815,0.));
#126848=CARTESIAN_POINT('Ctrl Pts',(29.01708543501,-65.523434328815,12.));
#126849=CARTESIAN_POINT('Ctrl Pts',(29.015183058267,-65.5001602132524,0.));
#126850=CARTESIAN_POINT('Ctrl Pts',(29.015183058267,-65.5001602132524,12.));
#126851=CARTESIAN_POINT('Ctrl Pts',(29.0132612477075,-65.4769317784754,
0.));
#126852=CARTESIAN_POINT('Ctrl Pts',(29.0132612477075,-65.4769317784754,
12.));
#126853=CARTESIAN_POINT('Ctrl Pts',(29.0113200786218,-65.4537491471782,
0.));
#126854=CARTESIAN_POINT('Ctrl Pts',(29.0113200786218,-65.4537491471782,
12.));
#126855=CARTESIAN_POINT('Ctrl Pts',(29.0093596267198,-65.4306124425524,
0.));
#126856=CARTESIAN_POINT('Ctrl Pts',(29.0093596267198,-65.4306124425524,
12.));
#126857=CARTESIAN_POINT('Ctrl Pts',(29.0073799681335,-65.4075217882921,
0.));
#126858=CARTESIAN_POINT('Ctrl Pts',(29.0073799681335,-65.4075217882921,
12.));
#126859=CARTESIAN_POINT('Ctrl Pts',(29.0053811794213,-65.3844773085977,
0.));
#126860=CARTESIAN_POINT('Ctrl Pts',(29.0053811794213,-65.3844773085977,
12.));
#126861=CARTESIAN_POINT('Ctrl Pts',(29.0033633375744,-65.3614791281726,
0.));
#126862=CARTESIAN_POINT('Ctrl Pts',(29.0033633375744,-65.3614791281726,
12.));
#126863=CARTESIAN_POINT('Ctrl Pts',(29.0013265200201,-65.3385273722279,
0.));
#126864=CARTESIAN_POINT('Ctrl Pts',(29.0013265200201,-65.3385273722279,
12.));
#126865=CARTESIAN_POINT('Ctrl Pts',(28.9992708046223,-65.3156221664942,
0.));
#126866=CARTESIAN_POINT('Ctrl Pts',(28.9992708046223,-65.3156221664942,
12.));
#126867=CARTESIAN_POINT('Ctrl Pts',(28.9971962696848,-65.2927636372261,
0.));
#126868=CARTESIAN_POINT('Ctrl Pts',(28.9971962696848,-65.2927636372261,
12.));
#126869=CARTESIAN_POINT('Ctrl Pts',(28.9951029939551,-65.2699519112052,
0.));
#126870=CARTESIAN_POINT('Ctrl Pts',(28.9951029939551,-65.2699519112052,
12.));
#126871=CARTESIAN_POINT('Ctrl Pts',(28.9929910566314,-65.2471871157375,
0.));
#126872=CARTESIAN_POINT('Ctrl Pts',(28.9929910566314,-65.2471871157375,
12.));
#126873=CARTESIAN_POINT('Ctrl Pts',(28.9908605373651,-65.2244693786586,
0.));
#126874=CARTESIAN_POINT('Ctrl Pts',(28.9908605373651,-65.2244693786586,
12.));
#126875=CARTESIAN_POINT('Ctrl Pts',(28.9887115162626,-65.2017988283465,
0.));
#126876=CARTESIAN_POINT('Ctrl Pts',(28.9887115162626,-65.2017988283465,
12.));
#126877=CARTESIAN_POINT('Ctrl Pts',(28.9865440738882,-65.1791755937254,
0.));
#126878=CARTESIAN_POINT('Ctrl Pts',(28.9865440738882,-65.1791755937254,
12.));
#126879=CARTESIAN_POINT('Ctrl Pts',(28.9843582912696,-65.1565998042706,
0.));
#126880=CARTESIAN_POINT('Ctrl Pts',(28.9843582912696,-65.1565998042706,
12.));
#126881=CARTESIAN_POINT('Ctrl Pts',(28.9821542499049,-65.1340715900042,
0.));
#126882=CARTESIAN_POINT('Ctrl Pts',(28.9821542499049,-65.1340715900042,
12.));
#126883=CARTESIAN_POINT('Ctrl Pts',(28.9799320317648,-65.1115910815051,
0.));
#126884=CARTESIAN_POINT('Ctrl Pts',(28.9799320317648,-65.1115910815051,
12.));
#126885=CARTESIAN_POINT('Ctrl Pts',(28.9776917192936,-65.0891584099174,
0.));
#126886=CARTESIAN_POINT('Ctrl Pts',(28.9776917192936,-65.0891584099174,
12.));
#126887=CARTESIAN_POINT('Ctrl Pts',(28.9754333954134,-65.0667737069562,
0.));
#126888=CARTESIAN_POINT('Ctrl Pts',(28.9754333954134,-65.0667737069562,
12.));
#126889=CARTESIAN_POINT('Ctrl Pts',(28.9731571435281,-65.0444371049082,
0.));
#126890=CARTESIAN_POINT('Ctrl Pts',(28.9731571435281,-65.0444371049082,
12.));
#126891=CARTESIAN_POINT('Ctrl Pts',(28.9708630475298,-65.022148736628,0.));
#126892=CARTESIAN_POINT('Ctrl Pts',(28.9708630475298,-65.022148736628,12.));
#126893=CARTESIAN_POINT('Ctrl Pts',(28.9685511918016,-64.9999087355504,
0.));
#126894=CARTESIAN_POINT('Ctrl Pts',(28.9685511918016,-64.9999087355504,
12.));
#126895=CARTESIAN_POINT('Ctrl Pts',(28.9662216612216,-64.9777172357028,
0.));
#126896=CARTESIAN_POINT('Ctrl Pts',(28.9662216612216,-64.9777172357028,
12.));
#126897=CARTESIAN_POINT('Ctrl Pts',(28.9638745411676,-64.955574371711,0.));
#126898=CARTESIAN_POINT('Ctrl Pts',(28.9638745411676,-64.955574371711,12.));
#126899=CARTESIAN_POINT('Ctrl Pts',(28.9615099175249,-64.9334802788037,
0.));
#126900=CARTESIAN_POINT('Ctrl Pts',(28.9615099175249,-64.9334802788037,
12.));
#126901=CARTESIAN_POINT('Ctrl Pts',(28.9591278766934,-64.9114350928124,
0.));
#126902=CARTESIAN_POINT('Ctrl Pts',(28.9591278766934,-64.9114350928124,
12.));
#126903=CARTESIAN_POINT('Ctrl Pts',(28.9567285055865,-64.8894389501799,
0.));
#126904=CARTESIAN_POINT('Ctrl Pts',(28.9567285055865,-64.8894389501799,
12.));
#126905=CARTESIAN_POINT('Ctrl Pts',(28.9543118916327,-64.8674919879646,
0.));
#126906=CARTESIAN_POINT('Ctrl Pts',(28.9543118916327,-64.8674919879646,
12.));
#126907=CARTESIAN_POINT('Ctrl Pts',(28.9518781227764,-64.8455943438424,
0.));
#126908=CARTESIAN_POINT('Ctrl Pts',(28.9518781227764,-64.8455943438424,
12.));
#126909=CARTESIAN_POINT('Ctrl Pts',(28.9494272874833,-64.8237461561024,
0.));
#126910=CARTESIAN_POINT('Ctrl Pts',(28.9494272874833,-64.8237461561024,
12.));
#126911=CARTESIAN_POINT('Ctrl Pts',(28.9469594747436,-64.8019475636454,
0.));
#126912=CARTESIAN_POINT('Ctrl Pts',(28.9469594747436,-64.8019475636454,
12.));
#126913=CARTESIAN_POINT('Ctrl Pts',(28.9444747740815,-64.7801987060097,
0.));
#126914=CARTESIAN_POINT('Ctrl Pts',(28.9444747740815,-64.7801987060097,
12.));
#126915=CARTESIAN_POINT('Ctrl Pts',(28.9419732755659,-64.7584997233889,
0.));
#126916=CARTESIAN_POINT('Ctrl Pts',(28.9419732755659,-64.7584997233889,
12.));
#126917=CARTESIAN_POINT('Ctrl Pts',(28.9394550698201,-64.7368507566462,
0.));
#126918=CARTESIAN_POINT('Ctrl Pts',(28.9394550698201,-64.7368507566462,
12.));
#126919=CARTESIAN_POINT('Ctrl Pts',(28.9369202480383,-64.715251947327,0.));
#126920=CARTESIAN_POINT('Ctrl Pts',(28.9369202480383,-64.715251947327,12.));
#126921=CARTESIAN_POINT('Ctrl Pts',(28.9343689019869,-64.6937034376591,
0.));
#126922=CARTESIAN_POINT('Ctrl Pts',(28.9343689019869,-64.6937034376591,
12.));
#126923=CARTESIAN_POINT('Ctrl Pts',(28.9318011239905,-64.6722053705389,
0.));
#126924=CARTESIAN_POINT('Ctrl Pts',(28.9318011239905,-64.6722053705389,
12.));
#126925=CARTESIAN_POINT('Ctrl Pts',(28.9292170069219,-64.6507578895155,
0.));
#126926=CARTESIAN_POINT('Ctrl Pts',(28.9292170069219,-64.6507578895155,
12.));
#126927=CARTESIAN_POINT('Ctrl Pts',(28.9266166441956,-64.6293611387754,
0.));
#126928=CARTESIAN_POINT('Ctrl Pts',(28.9266166441956,-64.6293611387754,
12.));
#126929=CARTESIAN_POINT('Ctrl Pts',(28.9240001297553,-64.6080152631066,
0.));
#126930=CARTESIAN_POINT('Ctrl Pts',(28.9240001297553,-64.6080152631066,
12.));
#126931=CARTESIAN_POINT('Ctrl Pts',(28.9213675580996,-64.5867204079452,
0.));
#126932=CARTESIAN_POINT('Ctrl Pts',(28.9213675580996,-64.5867204079452,
12.));
#126933=CARTESIAN_POINT('Ctrl Pts',(28.918719024323,-64.5654767194488,0.));
#126934=CARTESIAN_POINT('Ctrl Pts',(28.918719024323,-64.5654767194488,12.));
#126935=CARTESIAN_POINT('Ctrl Pts',(28.9160546241538,-64.544284344556,0.));
#126936=CARTESIAN_POINT('Ctrl Pts',(28.9160546241538,-64.544284344556,12.));
#126937=CARTESIAN_POINT('Ctrl Pts',(28.9133744539942,-64.5231434310457,
0.));
#126938=CARTESIAN_POINT('Ctrl Pts',(28.9133744539942,-64.5231434310457,
12.));
#126939=CARTESIAN_POINT('Ctrl Pts',(28.9106786109638,-64.5020541275927,
0.));
#126940=CARTESIAN_POINT('Ctrl Pts',(28.9106786109638,-64.5020541275927,
12.));
#126941=CARTESIAN_POINT('Ctrl Pts',(28.9079671928252,-64.4810165836568,
0.));
#126942=CARTESIAN_POINT('Ctrl Pts',(28.9079671928252,-64.4810165836568,
12.));
#126943=CARTESIAN_POINT('Ctrl Pts',(28.9052402979055,-64.460030949357,0.));
#126944=CARTESIAN_POINT('Ctrl Pts',(28.9052402979055,-64.460030949357,12.));
#126945=CARTESIAN_POINT('Ctrl Pts',(28.9024980250309,-64.439097375364,0.));
#126946=CARTESIAN_POINT('Ctrl Pts',(28.9024980250309,-64.439097375364,12.));
#126947=CARTESIAN_POINT('Ctrl Pts',(28.8997404734349,-64.4182160127401,
0.));
#126948=CARTESIAN_POINT('Ctrl Pts',(28.8997404734349,-64.4182160127401,
12.));
#126949=CARTESIAN_POINT('Ctrl Pts',(28.8969677427518,-64.3973870129201,
0.));
#126950=CARTESIAN_POINT('Ctrl Pts',(28.8969677427518,-64.3973870129201,
12.));
#126951=CARTESIAN_POINT('Ctrl Pts',(28.8941799332312,-64.3766105280715,
0.));
#126952=CARTESIAN_POINT('Ctrl Pts',(28.8941799332312,-64.3766105280715,
12.));
#126953=CARTESIAN_POINT('Ctrl Pts',(28.8913771459327,-64.3558867114087,
0.));
#126954=CARTESIAN_POINT('Ctrl Pts',(28.8913771459327,-64.3558867114087,
12.));
#126955=CARTESIAN_POINT('Ctrl Pts',(28.8885594828919,-64.3352157174607,
0.));
#126956=CARTESIAN_POINT('Ctrl Pts',(28.8885594828919,-64.3352157174607,
12.));
#126957=CARTESIAN_POINT('Ctrl Pts',(28.8857270473944,-64.3145977025005,
0.));
#126958=CARTESIAN_POINT('Ctrl Pts',(28.8857270473944,-64.3145977025005,
12.));
#126959=CARTESIAN_POINT('Ctrl Pts',(28.8828799437922,-64.2940328242483,
0.));
#126960=CARTESIAN_POINT('Ctrl Pts',(28.8828799437922,-64.2940328242483,
12.));
#126961=CARTESIAN_POINT('Ctrl Pts',(28.8800182770051,-64.2735212410682,
0.));
#126962=CARTESIAN_POINT('Ctrl Pts',(28.8800182770051,-64.2735212410682,
12.));
#126963=CARTESIAN_POINT('Ctrl Pts',(28.8771421521058,-64.2530631112927,
0.));
#126964=CARTESIAN_POINT('Ctrl Pts',(28.8771421521058,-64.2530631112927,
12.));
#126965=CARTESIAN_POINT('Ctrl Pts',(28.8742516738958,-64.232658592528,0.));
#126966=CARTESIAN_POINT('Ctrl Pts',(28.8742516738958,-64.232658592528,12.));
#126967=CARTESIAN_POINT('Ctrl Pts',(28.8713469464205,-64.2123078408507,
0.));
#126968=CARTESIAN_POINT('Ctrl Pts',(28.8713469464205,-64.2123078408507,
12.));
#126969=CARTESIAN_POINT('Ctrl Pts',(28.8684280739032,-64.1920110123342,
0.));
#126970=CARTESIAN_POINT('Ctrl Pts',(28.8684280739032,-64.1920110123342,
12.));
#126971=CARTESIAN_POINT('Ctrl Pts',(28.8654951618658,-64.1717682648708,
0.));
#126972=CARTESIAN_POINT('Ctrl Pts',(28.8654951618658,-64.1717682648708,
12.));
#126973=CARTESIAN_POINT('Ctrl Pts',(28.8625483180433,-64.1515797596555,
0.));
#126974=CARTESIAN_POINT('Ctrl Pts',(28.8625483180433,-64.1515797596555,
12.));
#126975=CARTESIAN_POINT('Ctrl Pts',(28.8595876537131,-64.1314456633345,
0.));
#126976=CARTESIAN_POINT('Ctrl Pts',(28.8595876537131,-64.1314456633345,
12.));
#126977=CARTESIAN_POINT('Ctrl Pts',(28.8566132838156,-64.1113661481918,
0.));
#126978=CARTESIAN_POINT('Ctrl Pts',(28.8566132838156,-64.1113661481918,
12.));
#126979=CARTESIAN_POINT('Ctrl Pts',(28.8536253241836,-64.0913413876586,
0.));
#126980=CARTESIAN_POINT('Ctrl Pts',(28.8536253241836,-64.0913413876586,
12.));
#126981=CARTESIAN_POINT('Ctrl Pts',(28.8506238891086,-64.0713715523588,
0.));
#126982=CARTESIAN_POINT('Ctrl Pts',(28.8506238891086,-64.0713715523588,
12.));
#126983=CARTESIAN_POINT('Ctrl Pts',(28.8476090892242,-64.0514568066659,
0.));
#126984=CARTESIAN_POINT('Ctrl Pts',(28.8476090892242,-64.0514568066659,
12.));
#126985=CARTESIAN_POINT('Ctrl Pts',(28.8445810281275,-64.0315973031995,
0.));
#126986=CARTESIAN_POINT('Ctrl Pts',(28.8445810281275,-64.0315973031995,
12.));
#126987=CARTESIAN_POINT('Ctrl Pts',(28.841539805646,-64.0117931881364,0.));
#126988=CARTESIAN_POINT('Ctrl Pts',(28.841539805646,-64.0117931881364,12.));
#126989=CARTESIAN_POINT('Ctrl Pts',(28.8384855243267,-63.9920446117632,
0.));
#126990=CARTESIAN_POINT('Ctrl Pts',(28.8384855243267,-63.9920446117632,
12.));
#126991=CARTESIAN_POINT('Ctrl Pts',(28.83541829466,-63.9723517369614,0.));
#126992=CARTESIAN_POINT('Ctrl Pts',(28.83541829466,-63.9723517369614,12.));
#126993=CARTESIAN_POINT('Ctrl Pts',(28.8323382413752,-63.9527147494351,
0.));
#126994=CARTESIAN_POINT('Ctrl Pts',(28.8323382413752,-63.9527147494351,
12.));
#126995=CARTESIAN_POINT('Ctrl Pts',(28.8292455077494,-63.9331338646868,
0.));
#126996=CARTESIAN_POINT('Ctrl Pts',(28.8292455077494,-63.9331338646868,
12.));
#126997=CARTESIAN_POINT('Ctrl Pts',(28.8261402423219,-63.9136093063647,
0.));
#126998=CARTESIAN_POINT('Ctrl Pts',(28.8261402423219,-63.9136093063647,
12.));
#126999=CARTESIAN_POINT('Ctrl Pts',(28.8230225863142,-63.894141285685,0.));
#127000=CARTESIAN_POINT('Ctrl Pts',(28.8230225863142,-63.894141285685,12.));
#127001=CARTESIAN_POINT('Ctrl Pts',(28.8198926619892,-63.8747299825383,
0.));
#127002=CARTESIAN_POINT('Ctrl Pts',(28.8198926619892,-63.8747299825383,
12.));
#127003=CARTESIAN_POINT('Ctrl Pts',(28.8167505576805,-63.8553755207732,
0.));
#127004=CARTESIAN_POINT('Ctrl Pts',(28.8167505576805,-63.8553755207732,
12.));
#127005=CARTESIAN_POINT('Ctrl Pts',(28.8135963263556,-63.8360779670226,
0.));
#127006=CARTESIAN_POINT('Ctrl Pts',(28.8135963263556,-63.8360779670226,
12.));
#127007=CARTESIAN_POINT('Ctrl Pts',(28.8110632621132,-63.8206854735372,
0.));
#127008=CARTESIAN_POINT('Ctrl Pts',(28.8110632621132,-63.8206854735372,
12.));
#127009=CARTESIAN_POINT('Ctrl Pts',(28.8091580239664,-63.8091667271451,
0.));
#127010=CARTESIAN_POINT('Ctrl Pts',(28.8091580239664,-63.8091667271451,
12.));
#127011=CARTESIAN_POINT('Ctrl Pts',(28.8078854475473,-63.8014989507576,
0.));
#127012=CARTESIAN_POINT('Ctrl Pts',(28.8078854475473,-63.8014989507576,
12.));
#127013=CARTESIAN_POINT('Ctrl Pts',(28.8072485549236,-63.7976679095314,
0.));
#127014=CARTESIAN_POINT('Ctrl Pts',(28.8072485549236,-63.7976679095314,
12.));
#127015=CARTESIAN_POINT('',(28.8072485549236,-63.7976679095314,12.));
#127016=CARTESIAN_POINT('Ctrl Pts',(28.8072485549236,-63.7976679095314,
12.));
#127017=CARTESIAN_POINT('Ctrl Pts',(28.8078854475473,-63.8014989507576,
12.));
#127018=CARTESIAN_POINT('Ctrl Pts',(28.8091580239664,-63.8091667271451,
12.));
#127019=CARTESIAN_POINT('Ctrl Pts',(28.8110632621132,-63.8206854735372,
12.));
#127020=CARTESIAN_POINT('Ctrl Pts',(28.8135963263556,-63.8360779670226,
12.));
#127021=CARTESIAN_POINT('Ctrl Pts',(28.8167505576805,-63.8553755207732,
12.));
#127022=CARTESIAN_POINT('Ctrl Pts',(28.8198926619892,-63.8747299825383,
12.));
#127023=CARTESIAN_POINT('Ctrl Pts',(28.8230225863142,-63.894141285685,12.));
#127024=CARTESIAN_POINT('Ctrl Pts',(28.8261402423219,-63.9136093063647,
12.));
#127025=CARTESIAN_POINT('Ctrl Pts',(28.8292455077494,-63.9331338646868,
12.));
#127026=CARTESIAN_POINT('Ctrl Pts',(28.8323382413752,-63.9527147494351,
12.));
#127027=CARTESIAN_POINT('Ctrl Pts',(28.83541829466,-63.9723517369614,12.));
#127028=CARTESIAN_POINT('Ctrl Pts',(28.8384855243267,-63.9920446117632,
12.));
#127029=CARTESIAN_POINT('Ctrl Pts',(28.841539805646,-64.0117931881364,12.));
#127030=CARTESIAN_POINT('Ctrl Pts',(28.8445810281275,-64.0315973031995,
12.));
#127031=CARTESIAN_POINT('Ctrl Pts',(28.8476090892242,-64.0514568066659,
12.));
#127032=CARTESIAN_POINT('Ctrl Pts',(28.8506238891086,-64.0713715523588,
12.));
#127033=CARTESIAN_POINT('Ctrl Pts',(28.8536253241836,-64.0913413876586,
12.));
#127034=CARTESIAN_POINT('Ctrl Pts',(28.8566132838156,-64.1113661481918,
12.));
#127035=CARTESIAN_POINT('Ctrl Pts',(28.8595876537131,-64.1314456633345,
12.));
#127036=CARTESIAN_POINT('Ctrl Pts',(28.8625483180433,-64.1515797596555,
12.));
#127037=CARTESIAN_POINT('Ctrl Pts',(28.8654951618658,-64.1717682648708,
12.));
#127038=CARTESIAN_POINT('Ctrl Pts',(28.8684280739032,-64.1920110123342,
12.));
#127039=CARTESIAN_POINT('Ctrl Pts',(28.8713469464205,-64.2123078408507,
12.));
#127040=CARTESIAN_POINT('Ctrl Pts',(28.8742516738958,-64.232658592528,12.));
#127041=CARTESIAN_POINT('Ctrl Pts',(28.8771421521058,-64.2530631112927,
12.));
#127042=CARTESIAN_POINT('Ctrl Pts',(28.8800182770051,-64.2735212410682,
12.));
#127043=CARTESIAN_POINT('Ctrl Pts',(28.8828799437922,-64.2940328242483,
12.));
#127044=CARTESIAN_POINT('Ctrl Pts',(28.8857270473944,-64.3145977025005,
12.));
#127045=CARTESIAN_POINT('Ctrl Pts',(28.8885594828919,-64.3352157174607,
12.));
#127046=CARTESIAN_POINT('Ctrl Pts',(28.8913771459327,-64.3558867114087,
12.));
#127047=CARTESIAN_POINT('Ctrl Pts',(28.8941799332312,-64.3766105280715,
12.));
#127048=CARTESIAN_POINT('Ctrl Pts',(28.8969677427518,-64.3973870129201,
12.));
#127049=CARTESIAN_POINT('Ctrl Pts',(28.8997404734349,-64.4182160127401,
12.));
#127050=CARTESIAN_POINT('Ctrl Pts',(28.9024980250309,-64.439097375364,12.));
#127051=CARTESIAN_POINT('Ctrl Pts',(28.9052402979055,-64.460030949357,12.));
#127052=CARTESIAN_POINT('Ctrl Pts',(28.9079671928252,-64.4810165836568,
12.));
#127053=CARTESIAN_POINT('Ctrl Pts',(28.9106786109638,-64.5020541275927,
12.));
#127054=CARTESIAN_POINT('Ctrl Pts',(28.9133744539942,-64.5231434310457,
12.));
#127055=CARTESIAN_POINT('Ctrl Pts',(28.9160546241538,-64.544284344556,12.));
#127056=CARTESIAN_POINT('Ctrl Pts',(28.918719024323,-64.5654767194488,12.));
#127057=CARTESIAN_POINT('Ctrl Pts',(28.9213675580996,-64.5867204079452,
12.));
#127058=CARTESIAN_POINT('Ctrl Pts',(28.9240001297553,-64.6080152631066,
12.));
#127059=CARTESIAN_POINT('Ctrl Pts',(28.9266166441956,-64.6293611387754,
12.));
#127060=CARTESIAN_POINT('Ctrl Pts',(28.9292170069219,-64.6507578895155,
12.));
#127061=CARTESIAN_POINT('Ctrl Pts',(28.9318011239905,-64.6722053705389,
12.));
#127062=CARTESIAN_POINT('Ctrl Pts',(28.9343689019869,-64.6937034376591,
12.));
#127063=CARTESIAN_POINT('Ctrl Pts',(28.9369202480383,-64.715251947327,12.));
#127064=CARTESIAN_POINT('Ctrl Pts',(28.9394550698201,-64.7368507566462,
12.));
#127065=CARTESIAN_POINT('Ctrl Pts',(28.9419732755659,-64.7584997233889,
12.));
#127066=CARTESIAN_POINT('Ctrl Pts',(28.9444747740815,-64.7801987060097,
12.));
#127067=CARTESIAN_POINT('Ctrl Pts',(28.9469594747436,-64.8019475636454,
12.));
#127068=CARTESIAN_POINT('Ctrl Pts',(28.9494272874833,-64.8237461561024,
12.));
#127069=CARTESIAN_POINT('Ctrl Pts',(28.9518781227764,-64.8455943438424,
12.));
#127070=CARTESIAN_POINT('Ctrl Pts',(28.9543118916327,-64.8674919879646,
12.));
#127071=CARTESIAN_POINT('Ctrl Pts',(28.9567285055865,-64.8894389501799,
12.));
#127072=CARTESIAN_POINT('Ctrl Pts',(28.9591278766934,-64.9114350928124,
12.));
#127073=CARTESIAN_POINT('Ctrl Pts',(28.9615099175249,-64.9334802788037,
12.));
#127074=CARTESIAN_POINT('Ctrl Pts',(28.9638745411676,-64.955574371711,12.));
#127075=CARTESIAN_POINT('Ctrl Pts',(28.9662216612216,-64.9777172357028,
12.));
#127076=CARTESIAN_POINT('Ctrl Pts',(28.9685511918016,-64.9999087355504,
12.));
#127077=CARTESIAN_POINT('Ctrl Pts',(28.9708630475298,-65.022148736628,12.));
#127078=CARTESIAN_POINT('Ctrl Pts',(28.9731571435281,-65.0444371049082,
12.));
#127079=CARTESIAN_POINT('Ctrl Pts',(28.9754333954134,-65.0667737069562,
12.));
#127080=CARTESIAN_POINT('Ctrl Pts',(28.9776917192936,-65.0891584099174,
12.));
#127081=CARTESIAN_POINT('Ctrl Pts',(28.9799320317648,-65.1115910815051,
12.));
#127082=CARTESIAN_POINT('Ctrl Pts',(28.9821542499049,-65.1340715900042,
12.));
#127083=CARTESIAN_POINT('Ctrl Pts',(28.9843582912696,-65.1565998042706,
12.));
#127084=CARTESIAN_POINT('Ctrl Pts',(28.9865440738882,-65.1791755937254,
12.));
#127085=CARTESIAN_POINT('Ctrl Pts',(28.9887115162626,-65.2017988283465,
12.));
#127086=CARTESIAN_POINT('Ctrl Pts',(28.9908605373651,-65.2244693786586,
12.));
#127087=CARTESIAN_POINT('Ctrl Pts',(28.9929910566314,-65.2471871157375,
12.));
#127088=CARTESIAN_POINT('Ctrl Pts',(28.9951029939551,-65.2699519112052,
12.));
#127089=CARTESIAN_POINT('Ctrl Pts',(28.9971962696848,-65.2927636372261,
12.));
#127090=CARTESIAN_POINT('Ctrl Pts',(28.9992708046223,-65.3156221664942,
12.));
#127091=CARTESIAN_POINT('Ctrl Pts',(29.0013265200201,-65.3385273722279,
12.));
#127092=CARTESIAN_POINT('Ctrl Pts',(29.0033633375744,-65.3614791281726,
12.));
#127093=CARTESIAN_POINT('Ctrl Pts',(29.0053811794213,-65.3844773085977,
12.));
#127094=CARTESIAN_POINT('Ctrl Pts',(29.0073799681335,-65.4075217882921,
12.));
#127095=CARTESIAN_POINT('Ctrl Pts',(29.0093596267198,-65.4306124425524,
12.));
#127096=CARTESIAN_POINT('Ctrl Pts',(29.0113200786218,-65.4537491471782,
12.));
#127097=CARTESIAN_POINT('Ctrl Pts',(29.0132612477075,-65.4769317784754,
12.));
#127098=CARTESIAN_POINT('Ctrl Pts',(29.015183058267,-65.5001602132524,12.));
#127099=CARTESIAN_POINT('Ctrl Pts',(29.01708543501,-65.523434328815,12.));
#127100=CARTESIAN_POINT('Ctrl Pts',(29.0189683030654,-65.5467540029546,
12.));
#127101=CARTESIAN_POINT('Ctrl Pts',(29.0208315879778,-65.5701191139455,
12.));
#127102=CARTESIAN_POINT('Ctrl Pts',(29.0226752157013,-65.593529540548,12.));
#127103=CARTESIAN_POINT('Ctrl Pts',(29.0244991125961,-65.6169851620054,
12.));
#127104=CARTESIAN_POINT('Ctrl Pts',(29.0263032054261,-65.6404858580391,
12.));
#127105=CARTESIAN_POINT('Ctrl Pts',(29.0280874213584,-65.6640315088361,
12.));
#127106=CARTESIAN_POINT('Ctrl Pts',(29.0298516879599,-65.6876219950465,
12.));
#127107=CARTESIAN_POINT('Ctrl Pts',(29.0315959331911,-65.7112571977874,
12.));
#127108=CARTESIAN_POINT('Ctrl Pts',(29.0333200854026,-65.7349369986382,
12.));
#127109=CARTESIAN_POINT('Ctrl Pts',(29.0350240733332,-65.7586612796375,
12.));
#127110=CARTESIAN_POINT('Ctrl Pts',(29.0367078261107,-65.7824299232715,
12.));
#127111=CARTESIAN_POINT('Ctrl Pts',(29.0383712732473,-65.8062428124723,
12.));
#127112=CARTESIAN_POINT('Ctrl Pts',(29.040014344634,-65.8300998306198,12.));
#127113=CARTESIAN_POINT('Ctrl Pts',(29.0416369705375,-65.854000861539,12.));
#127114=CARTESIAN_POINT('Ctrl Pts',(29.0432390815976,-65.8779457894959,
12.));
#127115=CARTESIAN_POINT('Ctrl Pts',(29.0448206088288,-65.9019344991854,
12.));
#127116=CARTESIAN_POINT('Ctrl Pts',(29.0463814836158,-65.925966875731,12.));
#127117=CARTESIAN_POINT('Ctrl Pts',(29.0479216377082,-65.9500428046873,
12.));
#127118=CARTESIAN_POINT('Ctrl Pts',(29.0494410032173,-65.9741621720372,
12.));
#127119=CARTESIAN_POINT('Ctrl Pts',(29.0509395126141,-65.9983248641877,
12.));
#127120=CARTESIAN_POINT('Ctrl Pts',(29.0524170987302,-66.0225307679584,
12.));
#127121=CARTESIAN_POINT('Ctrl Pts',(29.0538736947547,-66.0467797705806,
12.));
#127122=CARTESIAN_POINT('Ctrl Pts',(29.0553092342274,-66.0710717597003,
12.));
#127123=CARTESIAN_POINT('Ctrl Pts',(29.0567236510372,-66.0954066233752,
12.));
#127124=CARTESIAN_POINT('Ctrl Pts',(29.058116879419,-66.1197842500714,12.));
#127125=CARTESIAN_POINT('Ctrl Pts',(29.0594888539557,-66.144204528652,12.));
#127126=CARTESIAN_POINT('Ctrl Pts',(29.0608395095746,-66.1686673483757,
12.));
#127127=CARTESIAN_POINT('Ctrl Pts',(29.062168781542,-66.1931725989008,12.));
#127128=CARTESIAN_POINT('Ctrl Pts',(29.0634766054598,-66.2177201702818,
12.));
#127129=CARTESIAN_POINT('Ctrl Pts',(29.0647629172644,-66.2423099529669,
12.));
#127130=CARTESIAN_POINT('Ctrl Pts',(29.0660276532273,-66.2669418377871,
12.));
#127131=CARTESIAN_POINT('Ctrl Pts',(29.0672707499529,-66.2916157159536,
12.));
#127132=CARTESIAN_POINT('Ctrl Pts',(29.0684921443721,-66.3163314790615,
12.));
#127133=CARTESIAN_POINT('Ctrl Pts',(29.0696917737399,-66.3410890190884,
12.));
#127134=CARTESIAN_POINT('Ctrl Pts',(29.0708695756334,-66.3658882283903,
12.));
#127135=CARTESIAN_POINT('Ctrl Pts',(29.072025487953,-66.3907289996932,12.));
#127136=CARTESIAN_POINT('Ctrl Pts',(29.0731594489211,-66.4156112260887,
12.));
#127137=CARTESIAN_POINT('Ctrl Pts',(29.0742713970755,-66.4405348010388,
12.));
#127138=CARTESIAN_POINT('Ctrl Pts',(29.0753612712665,-66.4654996183731,
12.));
#127139=CARTESIAN_POINT('Ctrl Pts',(29.0764290106554,-66.4905055722868,
12.));
#127140=CARTESIAN_POINT('Ctrl Pts',(29.0774745547151,-66.5155525573323,
12.));
#127141=CARTESIAN_POINT('Ctrl Pts',(29.07849784323,-66.5406404684132,12.));
#127142=CARTESIAN_POINT('Ctrl Pts',(29.0794988162897,-66.5657692007906,
12.));
#127143=CARTESIAN_POINT('Ctrl Pts',(29.0804774142853,-66.59093865008,12.));
#127144=CARTESIAN_POINT('Ctrl Pts',(29.0814335779084,-66.6161487122502,
12.));
#127145=CARTESIAN_POINT('Ctrl Pts',(29.0823672481507,-66.6413992836147,
12.));
#127146=CARTESIAN_POINT('Ctrl Pts',(29.0832783663049,-66.6666902608249,
12.));
#127147=CARTESIAN_POINT('Ctrl Pts',(29.0841668739588,-66.6920215408751,
12.));
#127148=CARTESIAN_POINT('Ctrl Pts',(29.0850327129916,-66.7173930211022,
12.));
#127149=CARTESIAN_POINT('Ctrl Pts',(29.0858758255728,-66.7428045991841,
12.));
#127150=CARTESIAN_POINT('Ctrl Pts',(29.0866961541625,-66.7682561731342,
12.));
#127151=CARTESIAN_POINT('Ctrl Pts',(29.0874936415131,-66.793747641293,12.));
#127152=CARTESIAN_POINT('Ctrl Pts',(29.088268230663,-66.8192789023312,12.));
#127153=CARTESIAN_POINT('Ctrl Pts',(29.0890198649323,-66.8448498552503,
12.));
#127154=CARTESIAN_POINT('Ctrl Pts',(29.0897484879207,-66.8704603993794,
12.));
#127155=CARTESIAN_POINT('Ctrl Pts',(29.0904540435065,-66.8961104343707,
12.));
#127156=CARTESIAN_POINT('Ctrl Pts',(29.0911364758486,-66.9217998601885,
12.));
#127157=CARTESIAN_POINT('Ctrl Pts',(29.0917957293826,-66.9475285771135,
12.));
#127158=CARTESIAN_POINT('Ctrl Pts',(29.092431748817,-66.9732964857466,12.));
#127159=CARTESIAN_POINT('Ctrl Pts',(29.0930444791328,-66.9991034870083,
12.));
#127160=CARTESIAN_POINT('Ctrl Pts',(29.0936338655828,-67.0249494821363,
12.));
#127161=CARTESIAN_POINT('Ctrl Pts',(29.0941998536958,-67.0508343726777,
12.));
#127162=CARTESIAN_POINT('Ctrl Pts',(29.0947423892726,-67.0767580604879,
12.));
#127163=CARTESIAN_POINT('Ctrl Pts',(29.0952614183779,-67.1027204477311,
12.));
#127164=CARTESIAN_POINT('Ctrl Pts',(29.0957568873358,-67.1287214368746,
12.));
#127165=CARTESIAN_POINT('Ctrl Pts',(29.0962287427273,-67.1547609306843,
12.));
#127166=CARTESIAN_POINT('Ctrl Pts',(29.096676931389,-67.1808388322109,12.));
#127167=CARTESIAN_POINT('Ctrl Pts',(29.097101400413,-67.2069550447884,12.));
#127168=CARTESIAN_POINT('Ctrl Pts',(29.0975020971469,-67.2331094720471,
12.));
#127169=CARTESIAN_POINT('Ctrl Pts',(29.0978789691962,-67.2593020179209,
12.));
#127170=CARTESIAN_POINT('Ctrl Pts',(29.0982319644276,-67.2855325866517,
12.));
#127171=CARTESIAN_POINT('Ctrl Pts',(29.098561030977,-67.311801082792,12.));
#127172=CARTESIAN_POINT('Ctrl Pts',(29.098866117253,-67.3381074112027,12.));
#127173=CARTESIAN_POINT('Ctrl Pts',(29.0991471719176,-67.3644514770387,
12.));
#127174=CARTESIAN_POINT('Ctrl Pts',(29.0994041438718,-67.3908331857323,
12.));
#127175=CARTESIAN_POINT('Ctrl Pts',(29.0996369822418,-67.4172524429728,
12.));
#127176=CARTESIAN_POINT('Ctrl Pts',(29.0998456363682,-67.4437091546859,
12.));
#127177=CARTESIAN_POINT('Ctrl Pts',(29.1000300557955,-67.4702032270049,
12.));
#127178=CARTESIAN_POINT('Ctrl Pts',(29.1001901902908,-67.4967345663096,
12.));
#127179=CARTESIAN_POINT('Ctrl Pts',(29.1003259898681,-67.5233030792704,
12.));
#127180=CARTESIAN_POINT('Ctrl Pts',(29.1004374048147,-67.5499086728889,
12.));
#127181=CARTESIAN_POINT('Ctrl Pts',(29.1005243857138,-67.5765512545282,
12.));
#127182=CARTESIAN_POINT('Ctrl Pts',(29.1005868834866,-67.6032307319623,
12.));
#127183=CARTESIAN_POINT('Ctrl Pts',(29.100624849358,-67.6299470133295,12.));
#127184=CARTESIAN_POINT('Ctrl Pts',(29.1006382347814,-67.6567000070326,
12.));
#127185=CARTESIAN_POINT('Ctrl Pts',(29.1006269913747,-67.6834896216461,
12.));
#127186=CARTESIAN_POINT('Ctrl Pts',(29.1005910708624,-67.7103157658296,
12.));
#127187=CARTESIAN_POINT('Ctrl Pts',(29.1005304249986,-67.7371783482035,
12.));
#127188=CARTESIAN_POINT('Ctrl Pts',(29.1004450055642,-67.7640772773388,
12.));
#127189=CARTESIAN_POINT('Ctrl Pts',(29.1003347645293,-67.7910124620135,
12.));
#127190=CARTESIAN_POINT('Ctrl Pts',(29.1001996541841,-67.8179838114099,
12.));
#127191=CARTESIAN_POINT('Ctrl Pts',(29.1000396272867,-67.8449912353329,
12.));
#127192=CARTESIAN_POINT('Ctrl Pts',(29.0998546372032,-67.8720346444124,
12.));
#127193=CARTESIAN_POINT('Ctrl Pts',(29.0996446380626,-67.8991139503193,
12.));
#127194=CARTESIAN_POINT('Ctrl Pts',(29.099409584422,-67.9262290652829,12.));
#127195=CARTESIAN_POINT('Ctrl Pts',(29.0991494309404,-67.9533799016148,
12.));
#127196=CARTESIAN_POINT('Ctrl Pts',(29.0988641320246,-67.9805663711855,
12.));
#127197=CARTESIAN_POINT('Ctrl Pts',(29.098553641553,-68.0077883850121,12.));
#127198=CARTESIAN_POINT('Ctrl Pts',(29.0982179124097,-68.0350458525551,
12.));
#127199=CARTESIAN_POINT('Ctrl Pts',(29.0978568968656,-68.0623386822863,
12.));
#127200=CARTESIAN_POINT('Ctrl Pts',(29.0974705474258,-68.0896667829568,
12.));
#127201=CARTESIAN_POINT('Ctrl Pts',(29.0970588175728,-68.1170300646987,
12.));
#127202=CARTESIAN_POINT('Ctrl Pts',(29.0966216624743,-68.1444284400742,
12.));
#127203=CARTESIAN_POINT('Ctrl Pts',(29.0961590399046,-68.1718618254281,
12.));
#127204=CARTESIAN_POINT('Ctrl Pts',(29.0956709104627,-68.1993301412061,
12.));
#127205=CARTESIAN_POINT('Ctrl Pts',(29.095230591515,-68.2229056854684,12.));
#127206=CARTESIAN_POINT('Ctrl Pts',(29.094879194787,-68.2409993690197,12.));
#127207=CARTESIAN_POINT('Ctrl Pts',(29.0946280433337,-68.2535957747188,
12.));
#127208=CARTESIAN_POINT('Ctrl Pts',(29.0944846386568,-68.2606847334988,
12.));
#127209=CARTESIAN_POINT('Ctrl Pts',(29.0944526440265,-68.2622612910179,
12.));
#127210=CARTESIAN_POINT('',(28.8072485549236,-63.7976679095314,0.));
#127211=CARTESIAN_POINT('',(28.8072485549236,-63.7976679095314,0.));
#127212=CARTESIAN_POINT('Ctrl Pts',(29.0944526440265,-68.2622612910179,
0.));
#127213=CARTESIAN_POINT('Ctrl Pts',(29.0944846386568,-68.2606847334988,
0.));
#127214=CARTESIAN_POINT('Ctrl Pts',(29.0946280433337,-68.2535957747188,
0.));
#127215=CARTESIAN_POINT('Ctrl Pts',(29.094879194787,-68.2409993690197,0.));
#127216=CARTESIAN_POINT('Ctrl Pts',(29.095230591515,-68.2229056854684,0.));
#127217=CARTESIAN_POINT('Ctrl Pts',(29.0956709104627,-68.1993301412061,
0.));
#127218=CARTESIAN_POINT('Ctrl Pts',(29.0961590399046,-68.1718618254281,
0.));
#127219=CARTESIAN_POINT('Ctrl Pts',(29.0966216624743,-68.1444284400742,
0.));
#127220=CARTESIAN_POINT('Ctrl Pts',(29.0970588175728,-68.1170300646987,
0.));
#127221=CARTESIAN_POINT('Ctrl Pts',(29.0974705474258,-68.0896667829568,
0.));
#127222=CARTESIAN_POINT('Ctrl Pts',(29.0978568968656,-68.0623386822863,
0.));
#127223=CARTESIAN_POINT('Ctrl Pts',(29.0982179124097,-68.0350458525551,
0.));
#127224=CARTESIAN_POINT('Ctrl Pts',(29.098553641553,-68.0077883850121,0.));
#127225=CARTESIAN_POINT('Ctrl Pts',(29.0988641320246,-67.9805663711855,
0.));
#127226=CARTESIAN_POINT('Ctrl Pts',(29.0991494309404,-67.9533799016148,
0.));
#127227=CARTESIAN_POINT('Ctrl Pts',(29.099409584422,-67.9262290652829,0.));
#127228=CARTESIAN_POINT('Ctrl Pts',(29.0996446380626,-67.8991139503193,
0.));
#127229=CARTESIAN_POINT('Ctrl Pts',(29.0998546372032,-67.8720346444124,
0.));
#127230=CARTESIAN_POINT('Ctrl Pts',(29.1000396272867,-67.8449912353329,
0.));
#127231=CARTESIAN_POINT('Ctrl Pts',(29.1001996541841,-67.8179838114099,
0.));
#127232=CARTESIAN_POINT('Ctrl Pts',(29.1003347645293,-67.7910124620135,
0.));
#127233=CARTESIAN_POINT('Ctrl Pts',(29.1004450055642,-67.7640772773388,
0.));
#127234=CARTESIAN_POINT('Ctrl Pts',(29.1005304249986,-67.7371783482035,
0.));
#127235=CARTESIAN_POINT('Ctrl Pts',(29.1005910708624,-67.7103157658296,
0.));
#127236=CARTESIAN_POINT('Ctrl Pts',(29.1006269913747,-67.6834896216461,
0.));
#127237=CARTESIAN_POINT('Ctrl Pts',(29.1006382347814,-67.6567000070326,
0.));
#127238=CARTESIAN_POINT('Ctrl Pts',(29.100624849358,-67.6299470133295,0.));
#127239=CARTESIAN_POINT('Ctrl Pts',(29.1005868834866,-67.6032307319623,
0.));
#127240=CARTESIAN_POINT('Ctrl Pts',(29.1005243857138,-67.5765512545282,
0.));
#127241=CARTESIAN_POINT('Ctrl Pts',(29.1004374048147,-67.5499086728889,
0.));
#127242=CARTESIAN_POINT('Ctrl Pts',(29.1003259898681,-67.5233030792704,
0.));
#127243=CARTESIAN_POINT('Ctrl Pts',(29.1001901902908,-67.4967345663096,
0.));
#127244=CARTESIAN_POINT('Ctrl Pts',(29.1000300557955,-67.4702032270049,
0.));
#127245=CARTESIAN_POINT('Ctrl Pts',(29.0998456363682,-67.4437091546859,
0.));
#127246=CARTESIAN_POINT('Ctrl Pts',(29.0996369822418,-67.4172524429728,
0.));
#127247=CARTESIAN_POINT('Ctrl Pts',(29.0994041438718,-67.3908331857323,
0.));
#127248=CARTESIAN_POINT('Ctrl Pts',(29.0991471719176,-67.3644514770387,
0.));
#127249=CARTESIAN_POINT('Ctrl Pts',(29.098866117253,-67.3381074112027,0.));
#127250=CARTESIAN_POINT('Ctrl Pts',(29.098561030977,-67.311801082792,0.));
#127251=CARTESIAN_POINT('Ctrl Pts',(29.0982319644276,-67.2855325866517,
0.));
#127252=CARTESIAN_POINT('Ctrl Pts',(29.0978789691962,-67.2593020179209,
0.));
#127253=CARTESIAN_POINT('Ctrl Pts',(29.0975020971469,-67.2331094720471,
0.));
#127254=CARTESIAN_POINT('Ctrl Pts',(29.097101400413,-67.2069550447884,0.));
#127255=CARTESIAN_POINT('Ctrl Pts',(29.096676931389,-67.1808388322109,0.));
#127256=CARTESIAN_POINT('Ctrl Pts',(29.0962287427273,-67.1547609306843,
0.));
#127257=CARTESIAN_POINT('Ctrl Pts',(29.0957568873358,-67.1287214368746,
0.));
#127258=CARTESIAN_POINT('Ctrl Pts',(29.0952614183779,-67.1027204477311,
0.));
#127259=CARTESIAN_POINT('Ctrl Pts',(29.0947423892726,-67.0767580604879,
0.));
#127260=CARTESIAN_POINT('Ctrl Pts',(29.0941998536958,-67.0508343726777,
0.));
#127261=CARTESIAN_POINT('Ctrl Pts',(29.0936338655828,-67.0249494821363,
0.));
#127262=CARTESIAN_POINT('Ctrl Pts',(29.0930444791328,-66.9991034870083,
0.));
#127263=CARTESIAN_POINT('Ctrl Pts',(29.092431748817,-66.9732964857466,0.));
#127264=CARTESIAN_POINT('Ctrl Pts',(29.0917957293826,-66.9475285771135,
0.));
#127265=CARTESIAN_POINT('Ctrl Pts',(29.0911364758486,-66.9217998601885,
0.));
#127266=CARTESIAN_POINT('Ctrl Pts',(29.0904540435065,-66.8961104343707,
0.));
#127267=CARTESIAN_POINT('Ctrl Pts',(29.0897484879207,-66.8704603993794,
0.));
#127268=CARTESIAN_POINT('Ctrl Pts',(29.0890198649323,-66.8448498552503,
0.));
#127269=CARTESIAN_POINT('Ctrl Pts',(29.088268230663,-66.8192789023312,0.));
#127270=CARTESIAN_POINT('Ctrl Pts',(29.0874936415131,-66.793747641293,0.));
#127271=CARTESIAN_POINT('Ctrl Pts',(29.0866961541625,-66.7682561731342,
0.));
#127272=CARTESIAN_POINT('Ctrl Pts',(29.0858758255728,-66.7428045991841,
0.));
#127273=CARTESIAN_POINT('Ctrl Pts',(29.0850327129916,-66.7173930211022,
0.));
#127274=CARTESIAN_POINT('Ctrl Pts',(29.0841668739588,-66.6920215408751,
0.));
#127275=CARTESIAN_POINT('Ctrl Pts',(29.0832783663049,-66.6666902608249,
0.));
#127276=CARTESIAN_POINT('Ctrl Pts',(29.0823672481507,-66.6413992836147,
0.));
#127277=CARTESIAN_POINT('Ctrl Pts',(29.0814335779084,-66.6161487122502,
0.));
#127278=CARTESIAN_POINT('Ctrl Pts',(29.0804774142853,-66.59093865008,0.));
#127279=CARTESIAN_POINT('Ctrl Pts',(29.0794988162897,-66.5657692007906,
0.));
#127280=CARTESIAN_POINT('Ctrl Pts',(29.07849784323,-66.5406404684132,0.));
#127281=CARTESIAN_POINT('Ctrl Pts',(29.0774745547151,-66.5155525573323,
0.));
#127282=CARTESIAN_POINT('Ctrl Pts',(29.0764290106554,-66.4905055722868,
0.));
#127283=CARTESIAN_POINT('Ctrl Pts',(29.0753612712665,-66.4654996183731,
0.));
#127284=CARTESIAN_POINT('Ctrl Pts',(29.0742713970755,-66.4405348010388,
0.));
#127285=CARTESIAN_POINT('Ctrl Pts',(29.0731594489211,-66.4156112260887,
0.));
#127286=CARTESIAN_POINT('Ctrl Pts',(29.072025487953,-66.3907289996932,0.));
#127287=CARTESIAN_POINT('Ctrl Pts',(29.0708695756334,-66.3658882283903,
0.));
#127288=CARTESIAN_POINT('Ctrl Pts',(29.0696917737399,-66.3410890190884,
0.));
#127289=CARTESIAN_POINT('Ctrl Pts',(29.0684921443721,-66.3163314790615,
0.));
#127290=CARTESIAN_POINT('Ctrl Pts',(29.0672707499529,-66.2916157159536,
0.));
#127291=CARTESIAN_POINT('Ctrl Pts',(29.0660276532273,-66.2669418377871,
0.));
#127292=CARTESIAN_POINT('Ctrl Pts',(29.0647629172644,-66.2423099529669,
0.));
#127293=CARTESIAN_POINT('Ctrl Pts',(29.0634766054598,-66.2177201702818,
0.));
#127294=CARTESIAN_POINT('Ctrl Pts',(29.062168781542,-66.1931725989008,0.));
#127295=CARTESIAN_POINT('Ctrl Pts',(29.0608395095746,-66.1686673483757,
0.));
#127296=CARTESIAN_POINT('Ctrl Pts',(29.0594888539557,-66.144204528652,0.));
#127297=CARTESIAN_POINT('Ctrl Pts',(29.058116879419,-66.1197842500714,0.));
#127298=CARTESIAN_POINT('Ctrl Pts',(29.0567236510372,-66.0954066233752,
0.));
#127299=CARTESIAN_POINT('Ctrl Pts',(29.0553092342274,-66.0710717597003,
0.));
#127300=CARTESIAN_POINT('Ctrl Pts',(29.0538736947547,-66.0467797705806,
0.));
#127301=CARTESIAN_POINT('Ctrl Pts',(29.0524170987302,-66.0225307679584,
0.));
#127302=CARTESIAN_POINT('Ctrl Pts',(29.0509395126141,-65.9983248641877,
0.));
#127303=CARTESIAN_POINT('Ctrl Pts',(29.0494410032173,-65.9741621720372,
0.));
#127304=CARTESIAN_POINT('Ctrl Pts',(29.0479216377082,-65.9500428046873,
0.));
#127305=CARTESIAN_POINT('Ctrl Pts',(29.0463814836158,-65.925966875731,0.));
#127306=CARTESIAN_POINT('Ctrl Pts',(29.0448206088288,-65.9019344991854,
0.));
#127307=CARTESIAN_POINT('Ctrl Pts',(29.0432390815976,-65.8779457894959,
0.));
#127308=CARTESIAN_POINT('Ctrl Pts',(29.0416369705375,-65.854000861539,0.));
#127309=CARTESIAN_POINT('Ctrl Pts',(29.040014344634,-65.8300998306198,0.));
#127310=CARTESIAN_POINT('Ctrl Pts',(29.0383712732473,-65.8062428124723,
0.));
#127311=CARTESIAN_POINT('Ctrl Pts',(29.0367078261107,-65.7824299232715,
0.));
#127312=CARTESIAN_POINT('Ctrl Pts',(29.0350240733332,-65.7586612796375,
0.));
#127313=CARTESIAN_POINT('Ctrl Pts',(29.0333200854026,-65.7349369986382,
0.));
#127314=CARTESIAN_POINT('Ctrl Pts',(29.0315959331911,-65.7112571977874,
0.));
#127315=CARTESIAN_POINT('Ctrl Pts',(29.0298516879599,-65.6876219950465,
0.));
#127316=CARTESIAN_POINT('Ctrl Pts',(29.0280874213584,-65.6640315088361,
0.));
#127317=CARTESIAN_POINT('Ctrl Pts',(29.0263032054261,-65.6404858580391,
0.));
#127318=CARTESIAN_POINT('Ctrl Pts',(29.0244991125961,-65.6169851620054,
0.));
#127319=CARTESIAN_POINT('Ctrl Pts',(29.0226752157013,-65.593529540548,0.));
#127320=CARTESIAN_POINT('Ctrl Pts',(29.0208315879778,-65.5701191139455,
0.));
#127321=CARTESIAN_POINT('Ctrl Pts',(29.0189683030654,-65.5467540029546,
0.));
#127322=CARTESIAN_POINT('Ctrl Pts',(29.01708543501,-65.523434328815,0.));
#127323=CARTESIAN_POINT('Ctrl Pts',(29.015183058267,-65.5001602132524,0.));
#127324=CARTESIAN_POINT('Ctrl Pts',(29.0132612477075,-65.4769317784754,
0.));
#127325=CARTESIAN_POINT('Ctrl Pts',(29.0113200786218,-65.4537491471782,
0.));
#127326=CARTESIAN_POINT('Ctrl Pts',(29.0093596267198,-65.4306124425524,
0.));
#127327=CARTESIAN_POINT('Ctrl Pts',(29.0073799681335,-65.4075217882921,
0.));
#127328=CARTESIAN_POINT('Ctrl Pts',(29.0053811794213,-65.3844773085977,
0.));
#127329=CARTESIAN_POINT('Ctrl Pts',(29.0033633375744,-65.3614791281726,
0.));
#127330=CARTESIAN_POINT('Ctrl Pts',(29.0013265200201,-65.3385273722279,
0.));
#127331=CARTESIAN_POINT('Ctrl Pts',(28.9992708046223,-65.3156221664942,
0.));
#127332=CARTESIAN_POINT('Ctrl Pts',(28.9971962696848,-65.2927636372261,
0.));
#127333=CARTESIAN_POINT('Ctrl Pts',(28.9951029939551,-65.2699519112052,
0.));
#127334=CARTESIAN_POINT('Ctrl Pts',(28.9929910566314,-65.2471871157375,
0.));
#127335=CARTESIAN_POINT('Ctrl Pts',(28.9908605373651,-65.2244693786586,
0.));
#127336=CARTESIAN_POINT('Ctrl Pts',(28.9887115162626,-65.2017988283465,
0.));
#127337=CARTESIAN_POINT('Ctrl Pts',(28.9865440738882,-65.1791755937254,
0.));
#127338=CARTESIAN_POINT('Ctrl Pts',(28.9843582912696,-65.1565998042706,
0.));
#127339=CARTESIAN_POINT('Ctrl Pts',(28.9821542499049,-65.1340715900042,
0.));
#127340=CARTESIAN_POINT('Ctrl Pts',(28.9799320317648,-65.1115910815051,
0.));
#127341=CARTESIAN_POINT('Ctrl Pts',(28.9776917192936,-65.0891584099174,
0.));
#127342=CARTESIAN_POINT('Ctrl Pts',(28.9754333954134,-65.0667737069562,
0.));
#127343=CARTESIAN_POINT('Ctrl Pts',(28.9731571435281,-65.0444371049082,
0.));
#127344=CARTESIAN_POINT('Ctrl Pts',(28.9708630475298,-65.022148736628,0.));
#127345=CARTESIAN_POINT('Ctrl Pts',(28.9685511918016,-64.9999087355504,
0.));
#127346=CARTESIAN_POINT('Ctrl Pts',(28.9662216612216,-64.9777172357028,
0.));
#127347=CARTESIAN_POINT('Ctrl Pts',(28.9638745411676,-64.955574371711,0.));
#127348=CARTESIAN_POINT('Ctrl Pts',(28.9615099175249,-64.9334802788037,
0.));
#127349=CARTESIAN_POINT('Ctrl Pts',(28.9591278766934,-64.9114350928124,
0.));
#127350=CARTESIAN_POINT('Ctrl Pts',(28.9567285055865,-64.8894389501799,
0.));
#127351=CARTESIAN_POINT('Ctrl Pts',(28.9543118916327,-64.8674919879646,
0.));
#127352=CARTESIAN_POINT('Ctrl Pts',(28.9518781227764,-64.8455943438424,
0.));
#127353=CARTESIAN_POINT('Ctrl Pts',(28.9494272874833,-64.8237461561024,
0.));
#127354=CARTESIAN_POINT('Ctrl Pts',(28.9469594747436,-64.8019475636454,
0.));
#127355=CARTESIAN_POINT('Ctrl Pts',(28.9444747740815,-64.7801987060097,
0.));
#127356=CARTESIAN_POINT('Ctrl Pts',(28.9419732755659,-64.7584997233889,
0.));
#127357=CARTESIAN_POINT('Ctrl Pts',(28.9394550698201,-64.7368507566462,
0.));
#127358=CARTESIAN_POINT('Ctrl Pts',(28.9369202480383,-64.715251947327,0.));
#127359=CARTESIAN_POINT('Ctrl Pts',(28.9343689019869,-64.6937034376591,
0.));
#127360=CARTESIAN_POINT('Ctrl Pts',(28.9318011239905,-64.6722053705389,
0.));
#127361=CARTESIAN_POINT('Ctrl Pts',(28.9292170069219,-64.6507578895155,
0.));
#127362=CARTESIAN_POINT('Ctrl Pts',(28.9266166441956,-64.6293611387754,
0.));
#127363=CARTESIAN_POINT('Ctrl Pts',(28.9240001297553,-64.6080152631066,
0.));
#127364=CARTESIAN_POINT('Ctrl Pts',(28.9213675580996,-64.5867204079452,
0.));
#127365=CARTESIAN_POINT('Ctrl Pts',(28.918719024323,-64.5654767194488,0.));
#127366=CARTESIAN_POINT('Ctrl Pts',(28.9160546241538,-64.544284344556,0.));
#127367=CARTESIAN_POINT('Ctrl Pts',(28.9133744539942,-64.5231434310457,
0.));
#127368=CARTESIAN_POINT('Ctrl Pts',(28.9106786109638,-64.5020541275927,
0.));
#127369=CARTESIAN_POINT('Ctrl Pts',(28.9079671928252,-64.4810165836568,
0.));
#127370=CARTESIAN_POINT('Ctrl Pts',(28.9052402979055,-64.460030949357,0.));
#127371=CARTESIAN_POINT('Ctrl Pts',(28.9024980250309,-64.439097375364,0.));
#127372=CARTESIAN_POINT('Ctrl Pts',(28.8997404734349,-64.4182160127401,
0.));
#127373=CARTESIAN_POINT('Ctrl Pts',(28.8969677427518,-64.3973870129201,
0.));
#127374=CARTESIAN_POINT('Ctrl Pts',(28.8941799332312,-64.3766105280715,
0.));
#127375=CARTESIAN_POINT('Ctrl Pts',(28.8913771459327,-64.3558867114087,
0.));
#127376=CARTESIAN_POINT('Ctrl Pts',(28.8885594828919,-64.3352157174607,
0.));
#127377=CARTESIAN_POINT('Ctrl Pts',(28.8857270473944,-64.3145977025005,
0.));
#127378=CARTESIAN_POINT('Ctrl Pts',(28.8828799437922,-64.2940328242483,
0.));
#127379=CARTESIAN_POINT('Ctrl Pts',(28.8800182770051,-64.2735212410682,
0.));
#127380=CARTESIAN_POINT('Ctrl Pts',(28.8771421521058,-64.2530631112927,
0.));
#127381=CARTESIAN_POINT('Ctrl Pts',(28.8742516738958,-64.232658592528,0.));
#127382=CARTESIAN_POINT('Ctrl Pts',(28.8713469464205,-64.2123078408507,
0.));
#127383=CARTESIAN_POINT('Ctrl Pts',(28.8684280739032,-64.1920110123342,
0.));
#127384=CARTESIAN_POINT('Ctrl Pts',(28.8654951618658,-64.1717682648708,
0.));
#127385=CARTESIAN_POINT('Ctrl Pts',(28.8625483180433,-64.1515797596555,
0.));
#127386=CARTESIAN_POINT('Ctrl Pts',(28.8595876537131,-64.1314456633345,
0.));
#127387=CARTESIAN_POINT('Ctrl Pts',(28.8566132838156,-64.1113661481918,
0.));
#127388=CARTESIAN_POINT('Ctrl Pts',(28.8536253241836,-64.0913413876586,
0.));
#127389=CARTESIAN_POINT('Ctrl Pts',(28.8506238891086,-64.0713715523588,
0.));
#127390=CARTESIAN_POINT('Ctrl Pts',(28.8476090892242,-64.0514568066659,
0.));
#127391=CARTESIAN_POINT('Ctrl Pts',(28.8445810281275,-64.0315973031995,
0.));
#127392=CARTESIAN_POINT('Ctrl Pts',(28.841539805646,-64.0117931881364,0.));
#127393=CARTESIAN_POINT('Ctrl Pts',(28.8384855243267,-63.9920446117632,
0.));
#127394=CARTESIAN_POINT('Ctrl Pts',(28.83541829466,-63.9723517369614,0.));
#127395=CARTESIAN_POINT('Ctrl Pts',(28.8323382413752,-63.9527147494351,
0.));
#127396=CARTESIAN_POINT('Ctrl Pts',(28.8292455077494,-63.9331338646868,
0.));
#127397=CARTESIAN_POINT('Ctrl Pts',(28.8261402423219,-63.9136093063647,
0.));
#127398=CARTESIAN_POINT('Ctrl Pts',(28.8230225863142,-63.894141285685,0.));
#127399=CARTESIAN_POINT('Ctrl Pts',(28.8198926619892,-63.8747299825383,
0.));
#127400=CARTESIAN_POINT('Ctrl Pts',(28.8167505576805,-63.8553755207732,
0.));
#127401=CARTESIAN_POINT('Ctrl Pts',(28.8135963263556,-63.8360779670226,
0.));
#127402=CARTESIAN_POINT('Ctrl Pts',(28.8110632621132,-63.8206854735372,
0.));
#127403=CARTESIAN_POINT('Ctrl Pts',(28.8091580239664,-63.8091667271451,
0.));
#127404=CARTESIAN_POINT('Ctrl Pts',(28.8078854475473,-63.8014989507576,
0.));
#127405=CARTESIAN_POINT('Ctrl Pts',(28.8072485549236,-63.7976679095314,
0.));
#127406=CARTESIAN_POINT('Ctrl Pts',(22.9976507259816,-70.8615414811572,
0.));
#127407=CARTESIAN_POINT('Ctrl Pts',(22.9976507259816,-70.8615414811572,
12.));
#127408=CARTESIAN_POINT('Ctrl Pts',(22.9983100639391,-70.8559846928,0.));
#127409=CARTESIAN_POINT('Ctrl Pts',(22.9983100639391,-70.8559846928,12.));
#127410=CARTESIAN_POINT('Ctrl Pts',(22.999625855529,-70.8448742696689,0.));
#127411=CARTESIAN_POINT('Ctrl Pts',(22.999625855529,-70.8448742696689,12.));
#127412=CARTESIAN_POINT('Ctrl Pts',(23.0015908899394,-70.8282180957225,
0.));
#127413=CARTESIAN_POINT('Ctrl Pts',(23.0015908899394,-70.8282180957225,
12.));
#127414=CARTESIAN_POINT('Ctrl Pts',(23.0041936291625,-70.8060287860585,
0.));
#127415=CARTESIAN_POINT('Ctrl Pts',(23.0041936291625,-70.8060287860585,
12.));
#127416=CARTESIAN_POINT('Ctrl Pts',(23.0074182063786,-70.7783236951202,
0.));
#127417=CARTESIAN_POINT('Ctrl Pts',(23.0074182063786,-70.7783236951202,
12.));
#127418=CARTESIAN_POINT('Ctrl Pts',(23.0106139366046,-70.750650169619,0.));
#127419=CARTESIAN_POINT('Ctrl Pts',(23.0106139366046,-70.750650169619,12.));
#127420=CARTESIAN_POINT('Ctrl Pts',(23.0137808248923,-70.7230082425413,
0.));
#127421=CARTESIAN_POINT('Ctrl Pts',(23.0137808248923,-70.7230082425413,
12.));
#127422=CARTESIAN_POINT('Ctrl Pts',(23.0169188841044,-70.6953979633426,
0.));
#127423=CARTESIAN_POINT('Ctrl Pts',(23.0169188841044,-70.6953979633426,
12.));
#127424=CARTESIAN_POINT('Ctrl Pts',(23.0200281385833,-70.6678194023135,
0.));
#127425=CARTESIAN_POINT('Ctrl Pts',(23.0200281385833,-70.6678194023135,
12.));
#127426=CARTESIAN_POINT('Ctrl Pts',(23.0231086235186,-70.6402726486453,
0.));
#127427=CARTESIAN_POINT('Ctrl Pts',(23.0231086235186,-70.6402726486453,
12.));
#127428=CARTESIAN_POINT('Ctrl Pts',(23.026160381013,-70.6127578036674,0.));
#127429=CARTESIAN_POINT('Ctrl Pts',(23.026160381013,-70.6127578036674,12.));
#127430=CARTESIAN_POINT('Ctrl Pts',(23.0291834570662,-70.5852749754082,
0.));
#127431=CARTESIAN_POINT('Ctrl Pts',(23.0291834570662,-70.5852749754082,
12.));
#127432=CARTESIAN_POINT('Ctrl Pts',(23.0321778982711,-70.5578242727627,
0.));
#127433=CARTESIAN_POINT('Ctrl Pts',(23.0321778982711,-70.5578242727627,
12.));
#127434=CARTESIAN_POINT('Ctrl Pts',(23.0351437484336,-70.5304057994631,
0.));
#127435=CARTESIAN_POINT('Ctrl Pts',(23.0351437484336,-70.5304057994631,
12.));
#127436=CARTESIAN_POINT('Ctrl Pts',(23.0380810458271,-70.5030196492003,
0.));
#127437=CARTESIAN_POINT('Ctrl Pts',(23.0380810458271,-70.5030196492003,
12.));
#127438=CARTESIAN_POINT('Ctrl Pts',(23.0409898250756,-70.4756659090209,
0.));
#127439=CARTESIAN_POINT('Ctrl Pts',(23.0409898250756,-70.4756659090209,
12.));
#127440=CARTESIAN_POINT('Ctrl Pts',(23.0438701185012,-70.4483446617614,
0.));
#127441=CARTESIAN_POINT('Ctrl Pts',(23.0438701185012,-70.4483446617614,
12.));
#127442=CARTESIAN_POINT('Ctrl Pts',(23.046721957729,-70.4210559889348,0.));
#127443=CARTESIAN_POINT('Ctrl Pts',(23.046721957729,-70.4210559889348,12.));
#127444=CARTESIAN_POINT('Ctrl Pts',(23.0495453750763,-70.3937999732267,
0.));
#127445=CARTESIAN_POINT('Ctrl Pts',(23.0495453750763,-70.3937999732267,
12.));
#127446=CARTESIAN_POINT('Ctrl Pts',(23.0523404053172,-70.3665767016542,
0.));
#127447=CARTESIAN_POINT('Ctrl Pts',(23.0523404053172,-70.3665767016542,
12.));
#127448=CARTESIAN_POINT('Ctrl Pts',(23.0551070854926,-70.3393862652297,
0.));
#127449=CARTESIAN_POINT('Ctrl Pts',(23.0551070854926,-70.3393862652297,
12.));
#127450=CARTESIAN_POINT('Ctrl Pts',(23.0578454541104,-70.3122287575335,
0.));
#127451=CARTESIAN_POINT('Ctrl Pts',(23.0578454541104,-70.3122287575335,
12.));
#127452=CARTESIAN_POINT('Ctrl Pts',(23.0605555505321,-70.2851042736066,
0.));
#127453=CARTESIAN_POINT('Ctrl Pts',(23.0605555505321,-70.2851042736066,
12.));
#127454=CARTESIAN_POINT('Ctrl Pts',(23.0632374143279,-70.2580129087888,
0.));
#127455=CARTESIAN_POINT('Ctrl Pts',(23.0632374143279,-70.2580129087888,
12.));
#127456=CARTESIAN_POINT('Ctrl Pts',(23.0658910845432,-70.2309547573815,
0.));
#127457=CARTESIAN_POINT('Ctrl Pts',(23.0658910845432,-70.2309547573815,
12.));
#127458=CARTESIAN_POINT('Ctrl Pts',(23.068516599369,-70.2039299120488,0.));
#127459=CARTESIAN_POINT('Ctrl Pts',(23.068516599369,-70.2039299120488,12.));
#127460=CARTESIAN_POINT('Ctrl Pts',(23.0711139965439,-70.1769384645587,
0.));
#127461=CARTESIAN_POINT('Ctrl Pts',(23.0711139965439,-70.1769384645587,
12.));
#127462=CARTESIAN_POINT('Ctrl Pts',(23.0736833135938,-70.1499805062172,
0.));
#127463=CARTESIAN_POINT('Ctrl Pts',(23.0736833135938,-70.1499805062172,
12.));
#127464=CARTESIAN_POINT('Ctrl Pts',(23.0762245881389,-70.1230561284221,
0.));
#127465=CARTESIAN_POINT('Ctrl Pts',(23.0762245881389,-70.1230561284221,
12.));
#127466=CARTESIAN_POINT('Ctrl Pts',(23.0787378581774,-70.0961654231639,
0.));
#127467=CARTESIAN_POINT('Ctrl Pts',(23.0787378581774,-70.0961654231639,
12.));
#127468=CARTESIAN_POINT('Ctrl Pts',(23.0812231623765,-70.0693084835373,
0.));
#127469=CARTESIAN_POINT('Ctrl Pts',(23.0812231623765,-70.0693084835373,
12.));
#127470=CARTESIAN_POINT('Ctrl Pts',(23.0836805399374,-70.0424854035115,
0.));
#127471=CARTESIAN_POINT('Ctrl Pts',(23.0836805399374,-70.0424854035115,
12.));
#127472=CARTESIAN_POINT('Ctrl Pts',(23.0861100304729,-70.0156962777169,
0.));
#127473=CARTESIAN_POINT('Ctrl Pts',(23.0861100304729,-70.0156962777169,
12.));
#127474=CARTESIAN_POINT('Ctrl Pts',(23.0885116738797,-69.9889412012143,
0.));
#127475=CARTESIAN_POINT('Ctrl Pts',(23.0885116738797,-69.9889412012143,
12.));
#127476=CARTESIAN_POINT('Ctrl Pts',(23.090885510225,-69.9622202692873,0.));
#127477=CARTESIAN_POINT('Ctrl Pts',(23.090885510225,-69.9622202692873,12.));
#127478=CARTESIAN_POINT('Ctrl Pts',(23.0932315796067,-69.9355335771729,
0.));
#127479=CARTESIAN_POINT('Ctrl Pts',(23.0932315796067,-69.9355335771729,
12.));
#127480=CARTESIAN_POINT('Ctrl Pts',(23.0955499221558,-69.9088812200713,
0.));
#127481=CARTESIAN_POINT('Ctrl Pts',(23.0955499221558,-69.9088812200713,
12.));
#127482=CARTESIAN_POINT('Ctrl Pts',(23.097840578102,-69.8822632932768,0.));
#127483=CARTESIAN_POINT('Ctrl Pts',(23.097840578102,-69.8822632932768,12.));
#127484=CARTESIAN_POINT('Ctrl Pts',(23.1001035878241,-69.8556798922693,
0.));
#127485=CARTESIAN_POINT('Ctrl Pts',(23.1001035878241,-69.8556798922693,
12.));
#127486=CARTESIAN_POINT('Ctrl Pts',(23.1023389919051,-69.8291311128119,
0.));
#127487=CARTESIAN_POINT('Ctrl Pts',(23.1023389919051,-69.8291311128119,
12.));
#127488=CARTESIAN_POINT('Ctrl Pts',(23.104546831199,-69.8026170510572,0.));
#127489=CARTESIAN_POINT('Ctrl Pts',(23.104546831199,-69.8026170510572,12.));
#127490=CARTESIAN_POINT('Ctrl Pts',(23.1067271468609,-69.7761378035964,
0.));
#127491=CARTESIAN_POINT('Ctrl Pts',(23.1067271468609,-69.7761378035964,
12.));
#127492=CARTESIAN_POINT('Ctrl Pts',(23.1088799803089,-69.7496934674069,
0.));
#127493=CARTESIAN_POINT('Ctrl Pts',(23.1088799803089,-69.7496934674069,
12.));
#127494=CARTESIAN_POINT('Ctrl Pts',(23.1110053732046,-69.7232841398197,
0.));
#127495=CARTESIAN_POINT('Ctrl Pts',(23.1110053732046,-69.7232841398197,
12.));
#127496=CARTESIAN_POINT('Ctrl Pts',(23.1131033674301,-69.6969099184767,
0.));
#127497=CARTESIAN_POINT('Ctrl Pts',(23.1131033674301,-69.6969099184767,
12.));
#127498=CARTESIAN_POINT('Ctrl Pts',(23.115174005068,-69.6705709012852,0.));
#127499=CARTESIAN_POINT('Ctrl Pts',(23.115174005068,-69.6705709012852,12.));
#127500=CARTESIAN_POINT('Ctrl Pts',(23.1172173283858,-69.6442671863765,
0.));
#127501=CARTESIAN_POINT('Ctrl Pts',(23.1172173283858,-69.6442671863765,
12.));
#127502=CARTESIAN_POINT('Ctrl Pts',(23.1192333798441,-69.6179988721365,
0.));
#127503=CARTESIAN_POINT('Ctrl Pts',(23.1192333798441,-69.6179988721365,
12.));
#127504=CARTESIAN_POINT('Ctrl Pts',(23.1212222021051,-69.5917660572265,
0.));
#127505=CARTESIAN_POINT('Ctrl Pts',(23.1212222021051,-69.5917660572265,
12.));
#127506=CARTESIAN_POINT('Ctrl Pts',(23.1231838380452,-69.5655688406052,
0.));
#127507=CARTESIAN_POINT('Ctrl Pts',(23.1231838380452,-69.5655688406052,
12.));
#127508=CARTESIAN_POINT('Ctrl Pts',(23.1251183307676,-69.539407321546,0.));
#127509=CARTESIAN_POINT('Ctrl Pts',(23.1251183307676,-69.539407321546,12.));
#127510=CARTESIAN_POINT('Ctrl Pts',(23.1270257236204,-69.5132815996537,
0.));
#127511=CARTESIAN_POINT('Ctrl Pts',(23.1270257236204,-69.5132815996537,
12.));
#127512=CARTESIAN_POINT('Ctrl Pts',(23.1289060601924,-69.4871917748654,
0.));
#127513=CARTESIAN_POINT('Ctrl Pts',(23.1289060601924,-69.4871917748654,
12.));
#127514=CARTESIAN_POINT('Ctrl Pts',(23.1307593843061,-69.4611379474484,
0.));
#127515=CARTESIAN_POINT('Ctrl Pts',(23.1307593843061,-69.4611379474484,
12.));
#127516=CARTESIAN_POINT('Ctrl Pts',(23.1325857400144,-69.4351202179946,
0.));
#127517=CARTESIAN_POINT('Ctrl Pts',(23.1325857400144,-69.4351202179946,
12.));
#127518=CARTESIAN_POINT('Ctrl Pts',(23.1343851715989,-69.4091386874132,
0.));
#127519=CARTESIAN_POINT('Ctrl Pts',(23.1343851715989,-69.4091386874132,
12.));
#127520=CARTESIAN_POINT('Ctrl Pts',(23.1361577235709,-69.3831934569183,
0.));
#127521=CARTESIAN_POINT('Ctrl Pts',(23.1361577235709,-69.3831934569183,
12.));
#127522=CARTESIAN_POINT('Ctrl Pts',(23.1379034406718,-69.3572846280297,
0.));
#127523=CARTESIAN_POINT('Ctrl Pts',(23.1379034406718,-69.3572846280297,
12.));
#127524=CARTESIAN_POINT('Ctrl Pts',(23.1396223678725,-69.3314123025869,
0.));
#127525=CARTESIAN_POINT('Ctrl Pts',(23.1396223678725,-69.3314123025869,
12.));
#127526=CARTESIAN_POINT('Ctrl Pts',(23.1413145503762,-69.3055765827546,
0.));
#127527=CARTESIAN_POINT('Ctrl Pts',(23.1413145503762,-69.3055765827546,
12.));
#127528=CARTESIAN_POINT('Ctrl Pts',(23.142980033622,-69.2797775710273,0.));
#127529=CARTESIAN_POINT('Ctrl Pts',(23.142980033622,-69.2797775710273,12.));
#127530=CARTESIAN_POINT('Ctrl Pts',(23.1446188632931,-69.254015370231,0.));
#127531=CARTESIAN_POINT('Ctrl Pts',(23.1446188632931,-69.254015370231,12.));
#127532=CARTESIAN_POINT('Ctrl Pts',(23.1462310853206,-69.2282900835236,
0.));
#127533=CARTESIAN_POINT('Ctrl Pts',(23.1462310853206,-69.2282900835236,
12.));
#127534=CARTESIAN_POINT('Ctrl Pts',(23.1478167458789,-69.2026018144028,
0.));
#127535=CARTESIAN_POINT('Ctrl Pts',(23.1478167458789,-69.2026018144028,
12.));
#127536=CARTESIAN_POINT('Ctrl Pts',(23.1493758913858,-69.1769506667084,
0.));
#127537=CARTESIAN_POINT('Ctrl Pts',(23.1493758913858,-69.1769506667084,
12.));
#127538=CARTESIAN_POINT('Ctrl Pts',(23.1509085685032,-69.1513367446231,
0.));
#127539=CARTESIAN_POINT('Ctrl Pts',(23.1509085685032,-69.1513367446231,
12.));
#127540=CARTESIAN_POINT('Ctrl Pts',(23.152414824141,-69.1257601526687,0.));
#127541=CARTESIAN_POINT('Ctrl Pts',(23.152414824141,-69.1257601526687,12.));
#127542=CARTESIAN_POINT('Ctrl Pts',(23.1538947054614,-69.1002209957025,
0.));
#127543=CARTESIAN_POINT('Ctrl Pts',(23.1538947054614,-69.1002209957025,
12.));
#127544=CARTESIAN_POINT('Ctrl Pts',(23.1553482598762,-69.074719378928,0.));
#127545=CARTESIAN_POINT('Ctrl Pts',(23.1553482598762,-69.074719378928,12.));
#127546=CARTESIAN_POINT('Ctrl Pts',(23.1567755350469,-69.0492554078992,
0.));
#127547=CARTESIAN_POINT('Ctrl Pts',(23.1567755350469,-69.0492554078992,
12.));
#127548=CARTESIAN_POINT('Ctrl Pts',(23.1581765788868,-69.0238291885245,
0.));
#127549=CARTESIAN_POINT('Ctrl Pts',(23.1581765788868,-69.0238291885245,
12.));
#127550=CARTESIAN_POINT('Ctrl Pts',(23.1595514395656,-68.9984408270659,
0.));
#127551=CARTESIAN_POINT('Ctrl Pts',(23.1595514395656,-68.9984408270659,
12.));
#127552=CARTESIAN_POINT('Ctrl Pts',(23.1609001655155,-68.9730904301369,
0.));
#127553=CARTESIAN_POINT('Ctrl Pts',(23.1609001655155,-68.9730904301369,
12.));
#127554=CARTESIAN_POINT('Ctrl Pts',(23.1622228054291,-68.9477781047106,
0.));
#127555=CARTESIAN_POINT('Ctrl Pts',(23.1622228054291,-68.9477781047106,
12.));
#127556=CARTESIAN_POINT('Ctrl Pts',(23.1635194082581,-68.9225039581248,
0.));
#127557=CARTESIAN_POINT('Ctrl Pts',(23.1635194082581,-68.9225039581248,
12.));
#127558=CARTESIAN_POINT('Ctrl Pts',(23.164790023215,-68.8972680980842,0.));
#127559=CARTESIAN_POINT('Ctrl Pts',(23.164790023215,-68.8972680980842,12.));
#127560=CARTESIAN_POINT('Ctrl Pts',(23.1660346997763,-68.872070632661,0.));
#127561=CARTESIAN_POINT('Ctrl Pts',(23.1660346997763,-68.872070632661,12.));
#127562=CARTESIAN_POINT('Ctrl Pts',(23.1672534876889,-68.8469116702898,
0.));
#127563=CARTESIAN_POINT('Ctrl Pts',(23.1672534876889,-68.8469116702898,
12.));
#127564=CARTESIAN_POINT('Ctrl Pts',(23.1684464369686,-68.8217913197752,
0.));
#127565=CARTESIAN_POINT('Ctrl Pts',(23.1684464369686,-68.8217913197752,
12.));
#127566=CARTESIAN_POINT('Ctrl Pts',(23.1696135978997,-68.7967096902996,
0.));
#127567=CARTESIAN_POINT('Ctrl Pts',(23.1696135978997,-68.7967096902996,
12.));
#127568=CARTESIAN_POINT('Ctrl Pts',(23.170755021036,-68.771666891425,0.));
#127569=CARTESIAN_POINT('Ctrl Pts',(23.170755021036,-68.771666891425,12.));
#127570=CARTESIAN_POINT('Ctrl Pts',(23.1718707572043,-68.746663033096,0.));
#127571=CARTESIAN_POINT('Ctrl Pts',(23.1718707572043,-68.746663033096,12.));
#127572=CARTESIAN_POINT('Ctrl Pts',(23.1729608575109,-68.7216982256341,
0.));
#127573=CARTESIAN_POINT('Ctrl Pts',(23.1729608575109,-68.7216982256341,
12.));
#127574=CARTESIAN_POINT('Ctrl Pts',(23.1740253733417,-68.696772579744,0.));
#127575=CARTESIAN_POINT('Ctrl Pts',(23.1740253733417,-68.696772579744,12.));
#127576=CARTESIAN_POINT('Ctrl Pts',(23.1750643563601,-68.6718862065216,
0.));
#127577=CARTESIAN_POINT('Ctrl Pts',(23.1750643563601,-68.6718862065216,
12.));
#127578=CARTESIAN_POINT('Ctrl Pts',(23.1760778585092,-68.6470392174564,
0.));
#127579=CARTESIAN_POINT('Ctrl Pts',(23.1760778585092,-68.6470392174564,
12.));
#127580=CARTESIAN_POINT('Ctrl Pts',(23.1770659320137,-68.6222317244342,
0.));
#127581=CARTESIAN_POINT('Ctrl Pts',(23.1770659320137,-68.6222317244342,
12.));
#127582=CARTESIAN_POINT('Ctrl Pts',(23.1780286293875,-68.597463839733,0.));
#127583=CARTESIAN_POINT('Ctrl Pts',(23.1780286293875,-68.597463839733,12.));
#127584=CARTESIAN_POINT('Ctrl Pts',(23.1789660034341,-68.5727356760278,
0.));
#127585=CARTESIAN_POINT('Ctrl Pts',(23.1789660034341,-68.5727356760278,
12.));
#127586=CARTESIAN_POINT('Ctrl Pts',(23.1798781072449,-68.5480473463985,
0.));
#127587=CARTESIAN_POINT('Ctrl Pts',(23.1798781072449,-68.5480473463985,
12.));
#127588=CARTESIAN_POINT('Ctrl Pts',(23.180764994201,-68.5233989643345,0.));
#127589=CARTESIAN_POINT('Ctrl Pts',(23.180764994201,-68.5233989643345,12.));
#127590=CARTESIAN_POINT('Ctrl Pts',(23.1816267179751,-68.4987906437356,
0.));
#127591=CARTESIAN_POINT('Ctrl Pts',(23.1816267179751,-68.4987906437356,
12.));
#127592=CARTESIAN_POINT('Ctrl Pts',(23.1824633325384,-68.4742224989099,
0.));
#127593=CARTESIAN_POINT('Ctrl Pts',(23.1824633325384,-68.4742224989099,
12.));
#127594=CARTESIAN_POINT('Ctrl Pts',(23.183274892163,-68.4496946445758,0.));
#127595=CARTESIAN_POINT('Ctrl Pts',(23.183274892163,-68.4496946445758,12.));
#127596=CARTESIAN_POINT('Ctrl Pts',(23.1840614514192,-68.4252071958729,
0.));
#127597=CARTESIAN_POINT('Ctrl Pts',(23.1840614514192,-68.4252071958729,
12.));
#127598=CARTESIAN_POINT('Ctrl Pts',(23.1848230651776,-68.4007602683652,
0.));
#127599=CARTESIAN_POINT('Ctrl Pts',(23.1848230651776,-68.4007602683652,
12.));
#127600=CARTESIAN_POINT('Ctrl Pts',(23.1855597886115,-68.376353978044,0.));
#127601=CARTESIAN_POINT('Ctrl Pts',(23.1855597886115,-68.376353978044,12.));
#127602=CARTESIAN_POINT('Ctrl Pts',(23.186271677203,-68.3519884413246,0.));
#127603=CARTESIAN_POINT('Ctrl Pts',(23.186271677203,-68.3519884413246,12.));
#127604=CARTESIAN_POINT('Ctrl Pts',(23.1869587867459,-68.3276637750485,
0.));
#127605=CARTESIAN_POINT('Ctrl Pts',(23.1869587867459,-68.3276637750485,
12.));
#127606=CARTESIAN_POINT('Ctrl Pts',(23.1876211733435,-68.3033800964939,
0.));
#127607=CARTESIAN_POINT('Ctrl Pts',(23.1876211733435,-68.3033800964939,
12.));
#127608=CARTESIAN_POINT('Ctrl Pts',(23.1882588934106,-68.2791375233795,
0.));
#127609=CARTESIAN_POINT('Ctrl Pts',(23.1882588934106,-68.2791375233795,
12.));
#127610=CARTESIAN_POINT('Ctrl Pts',(23.1888720036757,-68.2549361738681,
0.));
#127611=CARTESIAN_POINT('Ctrl Pts',(23.1888720036757,-68.2549361738681,
12.));
#127612=CARTESIAN_POINT('Ctrl Pts',(23.1894605611871,-68.2307761665633,
0.));
#127613=CARTESIAN_POINT('Ctrl Pts',(23.1894605611871,-68.2307761665633,
12.));
#127614=CARTESIAN_POINT('Ctrl Pts',(23.1900246233165,-68.2066576205116,
0.));
#127615=CARTESIAN_POINT('Ctrl Pts',(23.1900246233165,-68.2066576205116,
12.));
#127616=CARTESIAN_POINT('Ctrl Pts',(23.1905642477571,-68.1825806552129,
0.));
#127617=CARTESIAN_POINT('Ctrl Pts',(23.1905642477571,-68.1825806552129,
12.));
#127618=CARTESIAN_POINT('Ctrl Pts',(23.1910794925251,-68.1585453906257,
0.));
#127619=CARTESIAN_POINT('Ctrl Pts',(23.1910794925251,-68.1585453906257,
12.));
#127620=CARTESIAN_POINT('Ctrl Pts',(23.1915704159623,-68.1345519471695,
0.));
#127621=CARTESIAN_POINT('Ctrl Pts',(23.1915704159623,-68.1345519471695,
12.));
#127622=CARTESIAN_POINT('Ctrl Pts',(23.1920370767425,-68.110600445723,0.));
#127623=CARTESIAN_POINT('Ctrl Pts',(23.1920370767425,-68.110600445723,12.));
#127624=CARTESIAN_POINT('Ctrl Pts',(23.1924795338749,-68.0866910076251,
0.));
#127625=CARTESIAN_POINT('Ctrl Pts',(23.1924795338749,-68.0866910076251,
12.));
#127626=CARTESIAN_POINT('Ctrl Pts',(23.192897846702,-68.0628237546863,0.));
#127627=CARTESIAN_POINT('Ctrl Pts',(23.192897846702,-68.0628237546863,12.));
#127628=CARTESIAN_POINT('Ctrl Pts',(23.1932920749023,-68.0389988091933,
0.));
#127629=CARTESIAN_POINT('Ctrl Pts',(23.1932920749023,-68.0389988091933,
12.));
#127630=CARTESIAN_POINT('Ctrl Pts',(23.1936622784918,-68.0152162939121,
0.));
#127631=CARTESIAN_POINT('Ctrl Pts',(23.1936622784918,-68.0152162939121,
12.));
#127632=CARTESIAN_POINT('Ctrl Pts',(23.1940085178313,-67.991476332086,0.));
#127633=CARTESIAN_POINT('Ctrl Pts',(23.1940085178313,-67.991476332086,12.));
#127634=CARTESIAN_POINT('Ctrl Pts',(23.1943308536297,-67.9677790474385,
0.));
#127635=CARTESIAN_POINT('Ctrl Pts',(23.1943308536297,-67.9677790474385,
12.));
#127636=CARTESIAN_POINT('Ctrl Pts',(23.1946293469427,-67.9441245641842,
0.));
#127637=CARTESIAN_POINT('Ctrl Pts',(23.1946293469427,-67.9441245641842,
12.));
#127638=CARTESIAN_POINT('Ctrl Pts',(23.1949040591744,-67.9205130070324,
0.));
#127639=CARTESIAN_POINT('Ctrl Pts',(23.1949040591744,-67.9205130070324,
12.));
#127640=CARTESIAN_POINT('Ctrl Pts',(23.1951550520802,-67.8969445011916,
0.));
#127641=CARTESIAN_POINT('Ctrl Pts',(23.1951550520802,-67.8969445011916,
12.));
#127642=CARTESIAN_POINT('Ctrl Pts',(23.1953823877734,-67.8734191723667,
0.));
#127643=CARTESIAN_POINT('Ctrl Pts',(23.1953823877734,-67.8734191723667,
12.));
#127644=CARTESIAN_POINT('Ctrl Pts',(23.1955861287286,-67.8499371467616,
0.));
#127645=CARTESIAN_POINT('Ctrl Pts',(23.1955861287286,-67.8499371467616,
12.));
#127646=CARTESIAN_POINT('Ctrl Pts',(23.1957663377806,-67.8264985510917,
0.));
#127647=CARTESIAN_POINT('Ctrl Pts',(23.1957663377806,-67.8264985510917,
12.));
#127648=CARTESIAN_POINT('Ctrl Pts',(23.1959230781269,-67.8031035125887,
0.));
#127649=CARTESIAN_POINT('Ctrl Pts',(23.1959230781269,-67.8031035125887,
12.));
#127650=CARTESIAN_POINT('Ctrl Pts',(23.1960564133304,-67.7797521590045,
0.));
#127651=CARTESIAN_POINT('Ctrl Pts',(23.1960564133304,-67.7797521590045,
12.));
#127652=CARTESIAN_POINT('Ctrl Pts',(23.1961664073261,-67.7564446186079,
0.));
#127653=CARTESIAN_POINT('Ctrl Pts',(23.1961664073261,-67.7564446186079,
12.));
#127654=CARTESIAN_POINT('Ctrl Pts',(23.1962531244245,-67.7331810201883,
0.));
#127655=CARTESIAN_POINT('Ctrl Pts',(23.1962531244245,-67.7331810201883,
12.));
#127656=CARTESIAN_POINT('Ctrl Pts',(23.1963166293102,-67.7099614930671,
0.));
#127657=CARTESIAN_POINT('Ctrl Pts',(23.1963166293102,-67.7099614930671,
12.));
#127658=CARTESIAN_POINT('Ctrl Pts',(23.1963569870451,-67.6867861671031,
0.));
#127659=CARTESIAN_POINT('Ctrl Pts',(23.1963569870451,-67.6867861671031,
12.));
#127660=CARTESIAN_POINT('Ctrl Pts',(23.1963742630714,-67.6636551726964,
0.));
#127661=CARTESIAN_POINT('Ctrl Pts',(23.1963742630714,-67.6636551726964,
12.));
#127662=CARTESIAN_POINT('Ctrl Pts',(23.1963685232187,-67.6405686407863,
0.));
#127663=CARTESIAN_POINT('Ctrl Pts',(23.1963685232187,-67.6405686407863,
12.));
#127664=CARTESIAN_POINT('Ctrl Pts',(23.1963398337068,-67.6175267028555,
0.));
#127665=CARTESIAN_POINT('Ctrl Pts',(23.1963398337068,-67.6175267028555,
12.));
#127666=CARTESIAN_POINT('Ctrl Pts',(23.1962882611452,-67.5945294909426,
0.));
#127667=CARTESIAN_POINT('Ctrl Pts',(23.1962882611452,-67.5945294909426,
12.));
#127668=CARTESIAN_POINT('Ctrl Pts',(23.196213872536,-67.5715771376461,0.));
#127669=CARTESIAN_POINT('Ctrl Pts',(23.196213872536,-67.5715771376461,12.));
#127670=CARTESIAN_POINT('Ctrl Pts',(23.1961167352771,-67.5486697761288,
0.));
#127671=CARTESIAN_POINT('Ctrl Pts',(23.1961167352771,-67.5486697761288,
12.));
#127672=CARTESIAN_POINT('Ctrl Pts',(23.19599691717,-67.5258075401146,0.));
#127673=CARTESIAN_POINT('Ctrl Pts',(23.19599691717,-67.5258075401146,12.));
#127674=CARTESIAN_POINT('Ctrl Pts',(23.1958544864215,-67.502990563895,0.));
#127675=CARTESIAN_POINT('Ctrl Pts',(23.1958544864215,-67.502990563895,12.));
#127676=CARTESIAN_POINT('Ctrl Pts',(23.195689511644,-67.4802189823408,0.));
#127677=CARTESIAN_POINT('Ctrl Pts',(23.195689511644,-67.4802189823408,12.));
#127678=CARTESIAN_POINT('Ctrl Pts',(23.1955020618589,-67.4574929309076,
0.));
#127679=CARTESIAN_POINT('Ctrl Pts',(23.1955020618589,-67.4574929309076,
12.));
#127680=CARTESIAN_POINT('Ctrl Pts',(23.1952922065012,-67.4348125456398,
0.));
#127681=CARTESIAN_POINT('Ctrl Pts',(23.1952922065012,-67.4348125456398,
12.));
#127682=CARTESIAN_POINT('Ctrl Pts',(23.1950600154265,-67.412177963168,0.));
#127683=CARTESIAN_POINT('Ctrl Pts',(23.1950600154265,-67.412177963168,12.));
#127684=CARTESIAN_POINT('Ctrl Pts',(23.1948055589128,-67.3895893207182,
0.));
#127685=CARTESIAN_POINT('Ctrl Pts',(23.1948055589128,-67.3895893207182,
12.));
#127686=CARTESIAN_POINT('Ctrl Pts',(23.194528907661,-67.3670467561212,0.));
#127687=CARTESIAN_POINT('Ctrl Pts',(23.194528907661,-67.3670467561212,12.));
#127688=CARTESIAN_POINT('Ctrl Pts',(23.1942301327978,-67.3445504078176,
0.));
#127689=CARTESIAN_POINT('Ctrl Pts',(23.1942301327978,-67.3445504078176,
12.));
#127690=CARTESIAN_POINT('Ctrl Pts',(23.1939093058801,-67.3221004148604,
0.));
#127691=CARTESIAN_POINT('Ctrl Pts',(23.1939093058801,-67.3221004148604,
12.));
#127692=CARTESIAN_POINT('Ctrl Pts',(23.1935664989018,-67.2996969169098,
0.));
#127693=CARTESIAN_POINT('Ctrl Pts',(23.1935664989018,-67.2996969169098,
12.));
#127694=CARTESIAN_POINT('Ctrl Pts',(23.1932017842952,-67.2773400542477,
0.));
#127695=CARTESIAN_POINT('Ctrl Pts',(23.1932017842952,-67.2773400542477,
12.));
#127696=CARTESIAN_POINT('Ctrl Pts',(23.1928152349342,-67.2550299677888,
0.));
#127697=CARTESIAN_POINT('Ctrl Pts',(23.1928152349342,-67.2550299677888,
12.));
#127698=CARTESIAN_POINT('Ctrl Pts',(23.1924069241385,-67.232766799088,0.));
#127699=CARTESIAN_POINT('Ctrl Pts',(23.1924069241385,-67.232766799088,12.));
#127700=CARTESIAN_POINT('Ctrl Pts',(23.1919769256803,-67.2105506903447,
0.));
#127701=CARTESIAN_POINT('Ctrl Pts',(23.1919769256803,-67.2105506903447,
12.));
#127702=CARTESIAN_POINT('Ctrl Pts',(23.1915253137923,-67.1883817844038,
0.));
#127703=CARTESIAN_POINT('Ctrl Pts',(23.1915253137923,-67.1883817844038,
12.));
#127704=CARTESIAN_POINT('Ctrl Pts',(23.1910521631657,-67.1662602247639,
0.));
#127705=CARTESIAN_POINT('Ctrl Pts',(23.1910521631657,-67.1662602247639,
12.));
#127706=CARTESIAN_POINT('Ctrl Pts',(23.1905575489504,-67.1441861555817,
0.));
#127707=CARTESIAN_POINT('Ctrl Pts',(23.1905575489504,-67.1441861555817,
12.));
#127708=CARTESIAN_POINT('Ctrl Pts',(23.1900415467574,-67.1221597216741,
0.));
#127709=CARTESIAN_POINT('Ctrl Pts',(23.1900415467574,-67.1221597216741,
12.));
#127710=CARTESIAN_POINT('Ctrl Pts',(23.1895042326626,-67.1001810685143,
0.));
#127711=CARTESIAN_POINT('Ctrl Pts',(23.1895042326626,-67.1001810685143,
12.));
#127712=CARTESIAN_POINT('Ctrl Pts',(23.1889456832119,-67.0782503422305,
0.));
#127713=CARTESIAN_POINT('Ctrl Pts',(23.1889456832119,-67.0782503422305,
12.));
#127714=CARTESIAN_POINT('Ctrl Pts',(23.1883659754271,-67.0563676896325,
0.));
#127715=CARTESIAN_POINT('Ctrl Pts',(23.1883659754271,-67.0563676896325,
12.));
#127716=CARTESIAN_POINT('Ctrl Pts',(23.1877651868157,-67.0345332582306,
0.));
#127717=CARTESIAN_POINT('Ctrl Pts',(23.1877651868157,-67.0345332582306,
12.));
#127718=CARTESIAN_POINT('Ctrl Pts',(23.1871433953793,-67.0127471962501,
0.));
#127719=CARTESIAN_POINT('Ctrl Pts',(23.1871433953793,-67.0127471962501,
12.));
#127720=CARTESIAN_POINT('Ctrl Pts',(23.1865006796283,-66.9910096526462,
0.));
#127721=CARTESIAN_POINT('Ctrl Pts',(23.1865006796283,-66.9910096526462,
12.));
#127722=CARTESIAN_POINT('Ctrl Pts',(23.1858371185842,-66.9693207771031,
0.));
#127723=CARTESIAN_POINT('Ctrl Pts',(23.1858371185842,-66.9693207771031,
12.));
#127724=CARTESIAN_POINT('Ctrl Pts',(23.1851527917657,-66.9476807200203,
0.));
#127725=CARTESIAN_POINT('Ctrl Pts',(23.1851527917657,-66.9476807200203,
12.));
#127726=CARTESIAN_POINT('Ctrl Pts',(23.1844477791814,-66.9260896324949,
0.));
#127727=CARTESIAN_POINT('Ctrl Pts',(23.1844477791814,-66.9260896324949,
12.));
#127728=CARTESIAN_POINT('Ctrl Pts',(23.1837221613235,-66.9045476663063,
0.));
#127729=CARTESIAN_POINT('Ctrl Pts',(23.1837221613235,-66.9045476663063,
12.));
#127730=CARTESIAN_POINT('Ctrl Pts',(23.1829760191591,-66.8830549738795,
0.));
#127731=CARTESIAN_POINT('Ctrl Pts',(23.1829760191591,-66.8830549738795,
12.));
#127732=CARTESIAN_POINT('Ctrl Pts',(23.1822094341517,-66.8616117083331,
0.));
#127733=CARTESIAN_POINT('Ctrl Pts',(23.1822094341517,-66.8616117083331,
12.));
#127734=CARTESIAN_POINT('Ctrl Pts',(23.1814224882953,-66.8402180235566,
0.));
#127735=CARTESIAN_POINT('Ctrl Pts',(23.1814224882953,-66.8402180235566,
12.));
#127736=CARTESIAN_POINT('Ctrl Pts',(23.1806152641475,-66.8188740742727,
0.));
#127737=CARTESIAN_POINT('Ctrl Pts',(23.1806152641475,-66.8188740742727,
12.));
#127738=CARTESIAN_POINT('Ctrl Pts',(23.1797878448639,-66.7975800161,0.));
#127739=CARTESIAN_POINT('Ctrl Pts',(23.1797878448639,-66.7975800161,12.));
#127740=CARTESIAN_POINT('Ctrl Pts',(23.1789403142366,-66.7763360056121,
0.));
#127741=CARTESIAN_POINT('Ctrl Pts',(23.1789403142366,-66.7763360056121,
12.));
#127742=CARTESIAN_POINT('Ctrl Pts',(23.17807275663,-66.7551422002204,0.));
#127743=CARTESIAN_POINT('Ctrl Pts',(23.17807275663,-66.7551422002204,12.));
#127744=CARTESIAN_POINT('Ctrl Pts',(23.1771852569131,-66.7339987580427,
0.));
#127745=CARTESIAN_POINT('Ctrl Pts',(23.1771852569131,-66.7339987580427,
12.));
#127746=CARTESIAN_POINT('Ctrl Pts',(23.1762779004044,-66.7129058377896,
0.));
#127747=CARTESIAN_POINT('Ctrl Pts',(23.1762779004044,-66.7129058377896,
12.));
#127748=CARTESIAN_POINT('Ctrl Pts',(23.1753507727939,-66.6918635985972,
0.));
#127749=CARTESIAN_POINT('Ctrl Pts',(23.1753507727939,-66.6918635985972,
12.));
#127750=CARTESIAN_POINT('Ctrl Pts',(23.1744039601381,-66.6708722000079,
0.));
#127751=CARTESIAN_POINT('Ctrl Pts',(23.1744039601381,-66.6708722000079,
12.));
#127752=CARTESIAN_POINT('Ctrl Pts',(23.1734375490431,-66.6499318023473,
0.));
#127753=CARTESIAN_POINT('Ctrl Pts',(23.1734375490431,-66.6499318023473,
12.));
#127754=CARTESIAN_POINT('Ctrl Pts',(23.1724516268302,-66.6290425670549,
0.));
#127755=CARTESIAN_POINT('Ctrl Pts',(23.1724516268302,-66.6290425670549,
12.));
#127756=CARTESIAN_POINT('Ctrl Pts',(23.1714462816789,-66.6082046569644,
0.));
#127757=CARTESIAN_POINT('Ctrl Pts',(23.1714462816789,-66.6082046569644,
12.));
#127758=CARTESIAN_POINT('Ctrl Pts',(23.1704216028614,-66.5874182367563,
0.));
#127759=CARTESIAN_POINT('Ctrl Pts',(23.1704216028614,-66.5874182367563,
12.));
#127760=CARTESIAN_POINT('Ctrl Pts',(23.1693776805865,-66.5666834726454,
0.));
#127761=CARTESIAN_POINT('Ctrl Pts',(23.1693776805865,-66.5666834726454,
12.));
#127762=CARTESIAN_POINT('Ctrl Pts',(23.1683146055726,-66.5460005315376,
0.));
#127763=CARTESIAN_POINT('Ctrl Pts',(23.1683146055726,-66.5460005315376,
12.));
#127764=CARTESIAN_POINT('Ctrl Pts',(23.1672324686926,-66.5253695803206,
0.));
#127765=CARTESIAN_POINT('Ctrl Pts',(23.1672324686926,-66.5253695803206,
12.));
#127766=CARTESIAN_POINT('Ctrl Pts',(23.1661313606132,-66.5047907851348,
0.));
#127767=CARTESIAN_POINT('Ctrl Pts',(23.1661313606132,-66.5047907851348,
12.));
#127768=CARTESIAN_POINT('Ctrl Pts',(23.1650113713808,-66.4842643105311,
0.));
#127769=CARTESIAN_POINT('Ctrl Pts',(23.1650113713808,-66.4842643105311,
12.));
#127770=CARTESIAN_POINT('Ctrl Pts',(23.1638725912195,-66.4637903210727,
0.));
#127771=CARTESIAN_POINT('Ctrl Pts',(23.1638725912195,-66.4637903210727,
12.));
#127772=CARTESIAN_POINT('Ctrl Pts',(23.1627151114883,-66.4433689832478,
0.));
#127773=CARTESIAN_POINT('Ctrl Pts',(23.1627151114883,-66.4433689832478,
12.));
#127774=CARTESIAN_POINT('Ctrl Pts',(23.1615390254631,-66.4230004670278,
0.));
#127775=CARTESIAN_POINT('Ctrl Pts',(23.1615390254631,-66.4230004670278,
12.));
#127776=CARTESIAN_POINT('Ctrl Pts',(23.160344429474,-66.4026849481232,0.));
#127777=CARTESIAN_POINT('Ctrl Pts',(23.160344429474,-66.4026849481232,12.));
#127778=CARTESIAN_POINT('Ctrl Pts',(23.1591314230083,-66.3824226081802,
0.));
#127779=CARTESIAN_POINT('Ctrl Pts',(23.1591314230083,-66.3824226081802,
12.));
#127780=CARTESIAN_POINT('Ctrl Pts',(23.1579001063423,-66.3622136300654,
0.));
#127781=CARTESIAN_POINT('Ctrl Pts',(23.1579001063423,-66.3622136300654,
12.));
#127782=CARTESIAN_POINT('Ctrl Pts',(23.1566505784621,-66.3420581937147,
0.));
#127783=CARTESIAN_POINT('Ctrl Pts',(23.1566505784621,-66.3420581937147,
12.));
#127784=CARTESIAN_POINT('Ctrl Pts',(23.1553829352539,-66.3219564725184,
0.));
#127785=CARTESIAN_POINT('Ctrl Pts',(23.1553829352539,-66.3219564725184,
12.));
#127786=CARTESIAN_POINT('Ctrl Pts',(23.154097266619,-66.3019086275445,0.));
#127787=CARTESIAN_POINT('Ctrl Pts',(23.154097266619,-66.3019086275445,12.));
#127788=CARTESIAN_POINT('Ctrl Pts',(23.1527936592651,-66.281914813114,0.));
#127789=CARTESIAN_POINT('Ctrl Pts',(23.1527936592651,-66.281914813114,12.));
#127790=CARTESIAN_POINT('Ctrl Pts',(23.1514722022503,-66.2619751878793,
0.));
#127791=CARTESIAN_POINT('Ctrl Pts',(23.1514722022503,-66.2619751878793,
12.));
#127792=CARTESIAN_POINT('Ctrl Pts',(23.1501329914487,-66.2420899237318,
0.));
#127793=CARTESIAN_POINT('Ctrl Pts',(23.1501329914487,-66.2420899237318,
12.));
#127794=CARTESIAN_POINT('Ctrl Pts',(23.1487761349297,-66.2222592165398,
0.));
#127795=CARTESIAN_POINT('Ctrl Pts',(23.1487761349297,-66.2222592165398,
12.));
#127796=CARTESIAN_POINT('Ctrl Pts',(23.147401756643,-66.2024832934733,0.));
#127797=CARTESIAN_POINT('Ctrl Pts',(23.147401756643,-66.2024832934733,12.));
#127798=CARTESIAN_POINT('Ctrl Pts',(23.1460099850704,-66.1827623902755,
0.));
#127799=CARTESIAN_POINT('Ctrl Pts',(23.1460099850704,-66.1827623902755,
12.));
#127800=CARTESIAN_POINT('Ctrl Pts',(23.1446009424871,-66.163096729667,0.));
#127801=CARTESIAN_POINT('Ctrl Pts',(23.1446009424871,-66.163096729667,12.));
#127802=CARTESIAN_POINT('Ctrl Pts',(23.1431747350127,-66.14348650151,0.));
#127803=CARTESIAN_POINT('Ctrl Pts',(23.1431747350127,-66.14348650151,12.));
#127804=CARTESIAN_POINT('Ctrl Pts',(23.1417314398501,-66.1239318368803,
0.));
#127805=CARTESIAN_POINT('Ctrl Pts',(23.1417314398501,-66.1239318368803,
12.));
#127806=CARTESIAN_POINT('Ctrl Pts',(23.140271103958,-66.1044328067739,0.));
#127807=CARTESIAN_POINT('Ctrl Pts',(23.140271103958,-66.1044328067739,12.));
#127808=CARTESIAN_POINT('Ctrl Pts',(23.1390892229923,-66.0888781152779,
0.));
#127809=CARTESIAN_POINT('Ctrl Pts',(23.1390892229923,-66.0888781152779,
12.));
#127810=CARTESIAN_POINT('Ctrl Pts',(23.1381951597491,-66.0772371487475,
0.));
#127811=CARTESIAN_POINT('Ctrl Pts',(23.1381951597491,-66.0772371487475,
12.));
#127812=CARTESIAN_POINT('Ctrl Pts',(23.1375957166138,-66.0694876382212,
0.));
#127813=CARTESIAN_POINT('Ctrl Pts',(23.1375957166138,-66.0694876382212,
12.));
#127814=CARTESIAN_POINT('Ctrl Pts',(23.1372951448023,-66.0656156664139,
0.));
#127815=CARTESIAN_POINT('Ctrl Pts',(23.1372951448023,-66.0656156664139,
12.));
#127816=CARTESIAN_POINT('',(23.1372951448023,-66.0656156664139,12.));
#127817=CARTESIAN_POINT('Ctrl Pts',(23.1372951448023,-66.0656156664139,
12.));
#127818=CARTESIAN_POINT('Ctrl Pts',(23.1375957166138,-66.0694876382212,
12.));
#127819=CARTESIAN_POINT('Ctrl Pts',(23.1381951597491,-66.0772371487475,
12.));
#127820=CARTESIAN_POINT('Ctrl Pts',(23.1390892229923,-66.0888781152779,
12.));
#127821=CARTESIAN_POINT('Ctrl Pts',(23.140271103958,-66.1044328067739,12.));
#127822=CARTESIAN_POINT('Ctrl Pts',(23.1417314398501,-66.1239318368803,
12.));
#127823=CARTESIAN_POINT('Ctrl Pts',(23.1431747350127,-66.14348650151,12.));
#127824=CARTESIAN_POINT('Ctrl Pts',(23.1446009424871,-66.163096729667,12.));
#127825=CARTESIAN_POINT('Ctrl Pts',(23.1460099850704,-66.1827623902755,
12.));
#127826=CARTESIAN_POINT('Ctrl Pts',(23.147401756643,-66.2024832934733,12.));
#127827=CARTESIAN_POINT('Ctrl Pts',(23.1487761349297,-66.2222592165398,
12.));
#127828=CARTESIAN_POINT('Ctrl Pts',(23.1501329914487,-66.2420899237318,
12.));
#127829=CARTESIAN_POINT('Ctrl Pts',(23.1514722022503,-66.2619751878793,
12.));
#127830=CARTESIAN_POINT('Ctrl Pts',(23.1527936592651,-66.281914813114,12.));
#127831=CARTESIAN_POINT('Ctrl Pts',(23.154097266619,-66.3019086275445,12.));
#127832=CARTESIAN_POINT('Ctrl Pts',(23.1553829352539,-66.3219564725184,
12.));
#127833=CARTESIAN_POINT('Ctrl Pts',(23.1566505784621,-66.3420581937147,
12.));
#127834=CARTESIAN_POINT('Ctrl Pts',(23.1579001063423,-66.3622136300654,
12.));
#127835=CARTESIAN_POINT('Ctrl Pts',(23.1591314230083,-66.3824226081802,
12.));
#127836=CARTESIAN_POINT('Ctrl Pts',(23.160344429474,-66.4026849481232,12.));
#127837=CARTESIAN_POINT('Ctrl Pts',(23.1615390254631,-66.4230004670278,
12.));
#127838=CARTESIAN_POINT('Ctrl Pts',(23.1627151114883,-66.4433689832478,
12.));
#127839=CARTESIAN_POINT('Ctrl Pts',(23.1638725912195,-66.4637903210727,
12.));
#127840=CARTESIAN_POINT('Ctrl Pts',(23.1650113713808,-66.4842643105311,
12.));
#127841=CARTESIAN_POINT('Ctrl Pts',(23.1661313606132,-66.5047907851348,
12.));
#127842=CARTESIAN_POINT('Ctrl Pts',(23.1672324686926,-66.5253695803206,
12.));
#127843=CARTESIAN_POINT('Ctrl Pts',(23.1683146055726,-66.5460005315376,
12.));
#127844=CARTESIAN_POINT('Ctrl Pts',(23.1693776805865,-66.5666834726454,
12.));
#127845=CARTESIAN_POINT('Ctrl Pts',(23.1704216028614,-66.5874182367563,
12.));
#127846=CARTESIAN_POINT('Ctrl Pts',(23.1714462816789,-66.6082046569644,
12.));
#127847=CARTESIAN_POINT('Ctrl Pts',(23.1724516268302,-66.6290425670549,
12.));
#127848=CARTESIAN_POINT('Ctrl Pts',(23.1734375490431,-66.6499318023473,
12.));
#127849=CARTESIAN_POINT('Ctrl Pts',(23.1744039601381,-66.6708722000079,
12.));
#127850=CARTESIAN_POINT('Ctrl Pts',(23.1753507727939,-66.6918635985972,
12.));
#127851=CARTESIAN_POINT('Ctrl Pts',(23.1762779004044,-66.7129058377896,
12.));
#127852=CARTESIAN_POINT('Ctrl Pts',(23.1771852569131,-66.7339987580427,
12.));
#127853=CARTESIAN_POINT('Ctrl Pts',(23.17807275663,-66.7551422002204,12.));
#127854=CARTESIAN_POINT('Ctrl Pts',(23.1789403142366,-66.7763360056121,
12.));
#127855=CARTESIAN_POINT('Ctrl Pts',(23.1797878448639,-66.7975800161,12.));
#127856=CARTESIAN_POINT('Ctrl Pts',(23.1806152641475,-66.8188740742727,
12.));
#127857=CARTESIAN_POINT('Ctrl Pts',(23.1814224882953,-66.8402180235566,
12.));
#127858=CARTESIAN_POINT('Ctrl Pts',(23.1822094341517,-66.8616117083331,
12.));
#127859=CARTESIAN_POINT('Ctrl Pts',(23.1829760191591,-66.8830549738795,
12.));
#127860=CARTESIAN_POINT('Ctrl Pts',(23.1837221613235,-66.9045476663063,
12.));
#127861=CARTESIAN_POINT('Ctrl Pts',(23.1844477791814,-66.9260896324949,
12.));
#127862=CARTESIAN_POINT('Ctrl Pts',(23.1851527917657,-66.9476807200203,
12.));
#127863=CARTESIAN_POINT('Ctrl Pts',(23.1858371185842,-66.9693207771031,
12.));
#127864=CARTESIAN_POINT('Ctrl Pts',(23.1865006796283,-66.9910096526462,
12.));
#127865=CARTESIAN_POINT('Ctrl Pts',(23.1871433953793,-67.0127471962501,
12.));
#127866=CARTESIAN_POINT('Ctrl Pts',(23.1877651868157,-67.0345332582306,
12.));
#127867=CARTESIAN_POINT('Ctrl Pts',(23.1883659754271,-67.0563676896325,
12.));
#127868=CARTESIAN_POINT('Ctrl Pts',(23.1889456832119,-67.0782503422305,
12.));
#127869=CARTESIAN_POINT('Ctrl Pts',(23.1895042326626,-67.1001810685143,
12.));
#127870=CARTESIAN_POINT('Ctrl Pts',(23.1900415467574,-67.1221597216741,
12.));
#127871=CARTESIAN_POINT('Ctrl Pts',(23.1905575489504,-67.1441861555817,
12.));
#127872=CARTESIAN_POINT('Ctrl Pts',(23.1910521631657,-67.1662602247639,
12.));
#127873=CARTESIAN_POINT('Ctrl Pts',(23.1915253137923,-67.1883817844038,
12.));
#127874=CARTESIAN_POINT('Ctrl Pts',(23.1919769256803,-67.2105506903447,
12.));
#127875=CARTESIAN_POINT('Ctrl Pts',(23.1924069241385,-67.232766799088,12.));
#127876=CARTESIAN_POINT('Ctrl Pts',(23.1928152349342,-67.2550299677888,
12.));
#127877=CARTESIAN_POINT('Ctrl Pts',(23.1932017842952,-67.2773400542477,
12.));
#127878=CARTESIAN_POINT('Ctrl Pts',(23.1935664989018,-67.2996969169098,
12.));
#127879=CARTESIAN_POINT('Ctrl Pts',(23.1939093058801,-67.3221004148604,
12.));
#127880=CARTESIAN_POINT('Ctrl Pts',(23.1942301327978,-67.3445504078176,
12.));
#127881=CARTESIAN_POINT('Ctrl Pts',(23.194528907661,-67.3670467561212,12.));
#127882=CARTESIAN_POINT('Ctrl Pts',(23.1948055589128,-67.3895893207182,
12.));
#127883=CARTESIAN_POINT('Ctrl Pts',(23.1950600154265,-67.412177963168,12.));
#127884=CARTESIAN_POINT('Ctrl Pts',(23.1952922065012,-67.4348125456398,
12.));
#127885=CARTESIAN_POINT('Ctrl Pts',(23.1955020618589,-67.4574929309076,
12.));
#127886=CARTESIAN_POINT('Ctrl Pts',(23.195689511644,-67.4802189823408,12.));
#127887=CARTESIAN_POINT('Ctrl Pts',(23.1958544864215,-67.502990563895,12.));
#127888=CARTESIAN_POINT('Ctrl Pts',(23.19599691717,-67.5258075401146,12.));
#127889=CARTESIAN_POINT('Ctrl Pts',(23.1961167352771,-67.5486697761288,
12.));
#127890=CARTESIAN_POINT('Ctrl Pts',(23.196213872536,-67.5715771376461,12.));
#127891=CARTESIAN_POINT('Ctrl Pts',(23.1962882611452,-67.5945294909426,
12.));
#127892=CARTESIAN_POINT('Ctrl Pts',(23.1963398337068,-67.6175267028555,
12.));
#127893=CARTESIAN_POINT('Ctrl Pts',(23.1963685232187,-67.6405686407863,
12.));
#127894=CARTESIAN_POINT('Ctrl Pts',(23.1963742630714,-67.6636551726964,
12.));
#127895=CARTESIAN_POINT('Ctrl Pts',(23.1963569870451,-67.6867861671031,
12.));
#127896=CARTESIAN_POINT('Ctrl Pts',(23.1963166293102,-67.7099614930671,
12.));
#127897=CARTESIAN_POINT('Ctrl Pts',(23.1962531244245,-67.7331810201883,
12.));
#127898=CARTESIAN_POINT('Ctrl Pts',(23.1961664073261,-67.7564446186079,
12.));
#127899=CARTESIAN_POINT('Ctrl Pts',(23.1960564133304,-67.7797521590045,
12.));
#127900=CARTESIAN_POINT('Ctrl Pts',(23.1959230781269,-67.8031035125887,
12.));
#127901=CARTESIAN_POINT('Ctrl Pts',(23.1957663377806,-67.8264985510917,
12.));
#127902=CARTESIAN_POINT('Ctrl Pts',(23.1955861287286,-67.8499371467616,
12.));
#127903=CARTESIAN_POINT('Ctrl Pts',(23.1953823877734,-67.8734191723667,
12.));
#127904=CARTESIAN_POINT('Ctrl Pts',(23.1951550520802,-67.8969445011916,
12.));
#127905=CARTESIAN_POINT('Ctrl Pts',(23.1949040591744,-67.9205130070324,
12.));
#127906=CARTESIAN_POINT('Ctrl Pts',(23.1946293469427,-67.9441245641842,
12.));
#127907=CARTESIAN_POINT('Ctrl Pts',(23.1943308536297,-67.9677790474385,
12.));
#127908=CARTESIAN_POINT('Ctrl Pts',(23.1940085178313,-67.991476332086,12.));
#127909=CARTESIAN_POINT('Ctrl Pts',(23.1936622784918,-68.0152162939121,
12.));
#127910=CARTESIAN_POINT('Ctrl Pts',(23.1932920749023,-68.0389988091933,
12.));
#127911=CARTESIAN_POINT('Ctrl Pts',(23.192897846702,-68.0628237546863,12.));
#127912=CARTESIAN_POINT('Ctrl Pts',(23.1924795338749,-68.0866910076251,
12.));
#127913=CARTESIAN_POINT('Ctrl Pts',(23.1920370767425,-68.110600445723,12.));
#127914=CARTESIAN_POINT('Ctrl Pts',(23.1915704159623,-68.1345519471695,
12.));
#127915=CARTESIAN_POINT('Ctrl Pts',(23.1910794925251,-68.1585453906257,
12.));
#127916=CARTESIAN_POINT('Ctrl Pts',(23.1905642477571,-68.1825806552129,
12.));
#127917=CARTESIAN_POINT('Ctrl Pts',(23.1900246233165,-68.2066576205116,
12.));
#127918=CARTESIAN_POINT('Ctrl Pts',(23.1894605611871,-68.2307761665633,
12.));
#127919=CARTESIAN_POINT('Ctrl Pts',(23.1888720036757,-68.2549361738681,
12.));
#127920=CARTESIAN_POINT('Ctrl Pts',(23.1882588934106,-68.2791375233795,
12.));
#127921=CARTESIAN_POINT('Ctrl Pts',(23.1876211733435,-68.3033800964939,
12.));
#127922=CARTESIAN_POINT('Ctrl Pts',(23.1869587867459,-68.3276637750485,
12.));
#127923=CARTESIAN_POINT('Ctrl Pts',(23.186271677203,-68.3519884413246,12.));
#127924=CARTESIAN_POINT('Ctrl Pts',(23.1855597886115,-68.376353978044,12.));
#127925=CARTESIAN_POINT('Ctrl Pts',(23.1848230651776,-68.4007602683652,
12.));
#127926=CARTESIAN_POINT('Ctrl Pts',(23.1840614514192,-68.4252071958729,
12.));
#127927=CARTESIAN_POINT('Ctrl Pts',(23.183274892163,-68.4496946445758,12.));
#127928=CARTESIAN_POINT('Ctrl Pts',(23.1824633325384,-68.4742224989099,
12.));
#127929=CARTESIAN_POINT('Ctrl Pts',(23.1816267179751,-68.4987906437356,
12.));
#127930=CARTESIAN_POINT('Ctrl Pts',(23.180764994201,-68.5233989643345,12.));
#127931=CARTESIAN_POINT('Ctrl Pts',(23.1798781072449,-68.5480473463985,
12.));
#127932=CARTESIAN_POINT('Ctrl Pts',(23.1789660034341,-68.5727356760278,
12.));
#127933=CARTESIAN_POINT('Ctrl Pts',(23.1780286293875,-68.597463839733,12.));
#127934=CARTESIAN_POINT('Ctrl Pts',(23.1770659320137,-68.6222317244342,
12.));
#127935=CARTESIAN_POINT('Ctrl Pts',(23.1760778585092,-68.6470392174564,
12.));
#127936=CARTESIAN_POINT('Ctrl Pts',(23.1750643563601,-68.6718862065216,
12.));
#127937=CARTESIAN_POINT('Ctrl Pts',(23.1740253733417,-68.696772579744,12.));
#127938=CARTESIAN_POINT('Ctrl Pts',(23.1729608575109,-68.7216982256341,
12.));
#127939=CARTESIAN_POINT('Ctrl Pts',(23.1718707572043,-68.746663033096,12.));
#127940=CARTESIAN_POINT('Ctrl Pts',(23.170755021036,-68.771666891425,12.));
#127941=CARTESIAN_POINT('Ctrl Pts',(23.1696135978997,-68.7967096902996,
12.));
#127942=CARTESIAN_POINT('Ctrl Pts',(23.1684464369686,-68.8217913197752,
12.));
#127943=CARTESIAN_POINT('Ctrl Pts',(23.1672534876889,-68.8469116702898,
12.));
#127944=CARTESIAN_POINT('Ctrl Pts',(23.1660346997763,-68.872070632661,12.));
#127945=CARTESIAN_POINT('Ctrl Pts',(23.164790023215,-68.8972680980842,12.));
#127946=CARTESIAN_POINT('Ctrl Pts',(23.1635194082581,-68.9225039581248,
12.));
#127947=CARTESIAN_POINT('Ctrl Pts',(23.1622228054291,-68.9477781047106,
12.));
#127948=CARTESIAN_POINT('Ctrl Pts',(23.1609001655155,-68.9730904301369,
12.));
#127949=CARTESIAN_POINT('Ctrl Pts',(23.1595514395656,-68.9984408270659,
12.));
#127950=CARTESIAN_POINT('Ctrl Pts',(23.1581765788868,-69.0238291885245,
12.));
#127951=CARTESIAN_POINT('Ctrl Pts',(23.1567755350469,-69.0492554078992,
12.));
#127952=CARTESIAN_POINT('Ctrl Pts',(23.1553482598762,-69.074719378928,12.));
#127953=CARTESIAN_POINT('Ctrl Pts',(23.1538947054614,-69.1002209957025,
12.));
#127954=CARTESIAN_POINT('Ctrl Pts',(23.152414824141,-69.1257601526687,12.));
#127955=CARTESIAN_POINT('Ctrl Pts',(23.1509085685032,-69.1513367446231,
12.));
#127956=CARTESIAN_POINT('Ctrl Pts',(23.1493758913858,-69.1769506667084,
12.));
#127957=CARTESIAN_POINT('Ctrl Pts',(23.1478167458789,-69.2026018144028,
12.));
#127958=CARTESIAN_POINT('Ctrl Pts',(23.1462310853206,-69.2282900835236,
12.));
#127959=CARTESIAN_POINT('Ctrl Pts',(23.1446188632931,-69.254015370231,12.));
#127960=CARTESIAN_POINT('Ctrl Pts',(23.142980033622,-69.2797775710273,12.));
#127961=CARTESIAN_POINT('Ctrl Pts',(23.1413145503762,-69.3055765827546,
12.));
#127962=CARTESIAN_POINT('Ctrl Pts',(23.1396223678725,-69.3314123025869,
12.));
#127963=CARTESIAN_POINT('Ctrl Pts',(23.1379034406718,-69.3572846280297,
12.));
#127964=CARTESIAN_POINT('Ctrl Pts',(23.1361577235709,-69.3831934569183,
12.));
#127965=CARTESIAN_POINT('Ctrl Pts',(23.1343851715989,-69.4091386874132,
12.));
#127966=CARTESIAN_POINT('Ctrl Pts',(23.1325857400144,-69.4351202179946,
12.));
#127967=CARTESIAN_POINT('Ctrl Pts',(23.1307593843061,-69.4611379474484,
12.));
#127968=CARTESIAN_POINT('Ctrl Pts',(23.1289060601924,-69.4871917748654,
12.));
#127969=CARTESIAN_POINT('Ctrl Pts',(23.1270257236204,-69.5132815996537,
12.));
#127970=CARTESIAN_POINT('Ctrl Pts',(23.1251183307676,-69.539407321546,12.));
#127971=CARTESIAN_POINT('Ctrl Pts',(23.1231838380452,-69.5655688406052,
12.));
#127972=CARTESIAN_POINT('Ctrl Pts',(23.1212222021051,-69.5917660572265,
12.));
#127973=CARTESIAN_POINT('Ctrl Pts',(23.1192333798441,-69.6179988721365,
12.));
#127974=CARTESIAN_POINT('Ctrl Pts',(23.1172173283858,-69.6442671863765,
12.));
#127975=CARTESIAN_POINT('Ctrl Pts',(23.115174005068,-69.6705709012852,12.));
#127976=CARTESIAN_POINT('Ctrl Pts',(23.1131033674301,-69.6969099184767,
12.));
#127977=CARTESIAN_POINT('Ctrl Pts',(23.1110053732046,-69.7232841398197,
12.));
#127978=CARTESIAN_POINT('Ctrl Pts',(23.1088799803089,-69.7496934674069,
12.));
#127979=CARTESIAN_POINT('Ctrl Pts',(23.1067271468609,-69.7761378035964,
12.));
#127980=CARTESIAN_POINT('Ctrl Pts',(23.104546831199,-69.8026170510572,12.));
#127981=CARTESIAN_POINT('Ctrl Pts',(23.1023389919051,-69.8291311128119,
12.));
#127982=CARTESIAN_POINT('Ctrl Pts',(23.1001035878241,-69.8556798922693,
12.));
#127983=CARTESIAN_POINT('Ctrl Pts',(23.097840578102,-69.8822632932768,12.));
#127984=CARTESIAN_POINT('Ctrl Pts',(23.0955499221558,-69.9088812200713,
12.));
#127985=CARTESIAN_POINT('Ctrl Pts',(23.0932315796067,-69.9355335771729,
12.));
#127986=CARTESIAN_POINT('Ctrl Pts',(23.090885510225,-69.9622202692873,12.));
#127987=CARTESIAN_POINT('Ctrl Pts',(23.0885116738797,-69.9889412012143,
12.));
#127988=CARTESIAN_POINT('Ctrl Pts',(23.0861100304729,-70.0156962777169,
12.));
#127989=CARTESIAN_POINT('Ctrl Pts',(23.0836805399374,-70.0424854035115,
12.));
#127990=CARTESIAN_POINT('Ctrl Pts',(23.0812231623765,-70.0693084835373,
12.));
#127991=CARTESIAN_POINT('Ctrl Pts',(23.0787378581774,-70.0961654231639,
12.));
#127992=CARTESIAN_POINT('Ctrl Pts',(23.0762245881389,-70.1230561284221,
12.));
#127993=CARTESIAN_POINT('Ctrl Pts',(23.0736833135938,-70.1499805062172,
12.));
#127994=CARTESIAN_POINT('Ctrl Pts',(23.0711139965439,-70.1769384645587,
12.));
#127995=CARTESIAN_POINT('Ctrl Pts',(23.068516599369,-70.2039299120488,12.));
#127996=CARTESIAN_POINT('Ctrl Pts',(23.0658910845432,-70.2309547573815,
12.));
#127997=CARTESIAN_POINT('Ctrl Pts',(23.0632374143279,-70.2580129087888,
12.));
#127998=CARTESIAN_POINT('Ctrl Pts',(23.0605555505321,-70.2851042736066,
12.));
#127999=CARTESIAN_POINT('Ctrl Pts',(23.0578454541104,-70.3122287575335,
12.));
#128000=CARTESIAN_POINT('Ctrl Pts',(23.0551070854926,-70.3393862652297,
12.));
#128001=CARTESIAN_POINT('Ctrl Pts',(23.0523404053172,-70.3665767016542,
12.));
#128002=CARTESIAN_POINT('Ctrl Pts',(23.0495453750763,-70.3937999732267,
12.));
#128003=CARTESIAN_POINT('Ctrl Pts',(23.046721957729,-70.4210559889348,12.));
#128004=CARTESIAN_POINT('Ctrl Pts',(23.0438701185012,-70.4483446617614,
12.));
#128005=CARTESIAN_POINT('Ctrl Pts',(23.0409898250756,-70.4756659090209,
12.));
#128006=CARTESIAN_POINT('Ctrl Pts',(23.0384964376036,-70.4991133648947,
12.));
#128007=CARTESIAN_POINT('Ctrl Pts',(23.0365694096172,-70.5171075702746,
12.));
#128008=CARTESIAN_POINT('Ctrl Pts',(23.0352213647764,-70.5296341535556,
12.));
#128009=CARTESIAN_POINT('Ctrl Pts',(23.0344606623298,-70.5366836381661,
12.));
#128010=CARTESIAN_POINT('Ctrl Pts',(23.0342913834072,-70.538251407892,12.));
#128011=CARTESIAN_POINT('',(23.1372951448023,-66.0656156664139,0.));
#128012=CARTESIAN_POINT('',(23.1372951448023,-66.0656156664138,0.));
#128013=CARTESIAN_POINT('Ctrl Pts',(23.0342913834072,-70.538251407892,0.));
#128014=CARTESIAN_POINT('Ctrl Pts',(23.0344606623298,-70.5366836381661,
0.));
#128015=CARTESIAN_POINT('Ctrl Pts',(23.0352213647764,-70.5296341535556,
0.));
#128016=CARTESIAN_POINT('Ctrl Pts',(23.0365694096172,-70.5171075702746,
0.));
#128017=CARTESIAN_POINT('Ctrl Pts',(23.0384964376036,-70.4991133648947,
0.));
#128018=CARTESIAN_POINT('Ctrl Pts',(23.0409898250756,-70.4756659090209,
0.));
#128019=CARTESIAN_POINT('Ctrl Pts',(23.0438701185012,-70.4483446617614,
0.));
#128020=CARTESIAN_POINT('Ctrl Pts',(23.046721957729,-70.4210559889348,0.));
#128021=CARTESIAN_POINT('Ctrl Pts',(23.0495453750763,-70.3937999732267,
0.));
#128022=CARTESIAN_POINT('Ctrl Pts',(23.0523404053172,-70.3665767016542,
0.));
#128023=CARTESIAN_POINT('Ctrl Pts',(23.0551070854926,-70.3393862652297,
0.));
#128024=CARTESIAN_POINT('Ctrl Pts',(23.0578454541104,-70.3122287575335,
0.));
#128025=CARTESIAN_POINT('Ctrl Pts',(23.0605555505321,-70.2851042736066,
0.));
#128026=CARTESIAN_POINT('Ctrl Pts',(23.0632374143279,-70.2580129087888,
0.));
#128027=CARTESIAN_POINT('Ctrl Pts',(23.0658910845432,-70.2309547573815,
0.));
#128028=CARTESIAN_POINT('Ctrl Pts',(23.068516599369,-70.2039299120488,0.));
#128029=CARTESIAN_POINT('Ctrl Pts',(23.0711139965439,-70.1769384645587,
0.));
#128030=CARTESIAN_POINT('Ctrl Pts',(23.0736833135938,-70.1499805062172,
0.));
#128031=CARTESIAN_POINT('Ctrl Pts',(23.0762245881389,-70.1230561284221,
0.));
#128032=CARTESIAN_POINT('Ctrl Pts',(23.0787378581774,-70.0961654231639,
0.));
#128033=CARTESIAN_POINT('Ctrl Pts',(23.0812231623765,-70.0693084835373,
0.));
#128034=CARTESIAN_POINT('Ctrl Pts',(23.0836805399374,-70.0424854035115,
0.));
#128035=CARTESIAN_POINT('Ctrl Pts',(23.0861100304729,-70.0156962777169,
0.));
#128036=CARTESIAN_POINT('Ctrl Pts',(23.0885116738797,-69.9889412012143,
0.));
#128037=CARTESIAN_POINT('Ctrl Pts',(23.090885510225,-69.9622202692873,0.));
#128038=CARTESIAN_POINT('Ctrl Pts',(23.0932315796067,-69.9355335771729,
0.));
#128039=CARTESIAN_POINT('Ctrl Pts',(23.0955499221558,-69.9088812200713,
0.));
#128040=CARTESIAN_POINT('Ctrl Pts',(23.097840578102,-69.8822632932768,0.));
#128041=CARTESIAN_POINT('Ctrl Pts',(23.1001035878241,-69.8556798922693,
0.));
#128042=CARTESIAN_POINT('Ctrl Pts',(23.1023389919051,-69.8291311128119,
0.));
#128043=CARTESIAN_POINT('Ctrl Pts',(23.104546831199,-69.8026170510572,0.));
#128044=CARTESIAN_POINT('Ctrl Pts',(23.1067271468609,-69.7761378035964,
0.));
#128045=CARTESIAN_POINT('Ctrl Pts',(23.1088799803089,-69.7496934674069,
0.));
#128046=CARTESIAN_POINT('Ctrl Pts',(23.1110053732046,-69.7232841398197,
0.));
#128047=CARTESIAN_POINT('Ctrl Pts',(23.1131033674301,-69.6969099184767,
0.));
#128048=CARTESIAN_POINT('Ctrl Pts',(23.115174005068,-69.6705709012852,0.));
#128049=CARTESIAN_POINT('Ctrl Pts',(23.1172173283858,-69.6442671863765,
0.));
#128050=CARTESIAN_POINT('Ctrl Pts',(23.1192333798441,-69.6179988721365,
0.));
#128051=CARTESIAN_POINT('Ctrl Pts',(23.1212222021051,-69.5917660572265,
0.));
#128052=CARTESIAN_POINT('Ctrl Pts',(23.1231838380452,-69.5655688406052,
0.));
#128053=CARTESIAN_POINT('Ctrl Pts',(23.1251183307676,-69.539407321546,0.));
#128054=CARTESIAN_POINT('Ctrl Pts',(23.1270257236204,-69.5132815996537,
0.));
#128055=CARTESIAN_POINT('Ctrl Pts',(23.1289060601924,-69.4871917748654,
0.));
#128056=CARTESIAN_POINT('Ctrl Pts',(23.1307593843061,-69.4611379474484,
0.));
#128057=CARTESIAN_POINT('Ctrl Pts',(23.1325857400144,-69.4351202179946,
0.));
#128058=CARTESIAN_POINT('Ctrl Pts',(23.1343851715989,-69.4091386874132,
0.));
#128059=CARTESIAN_POINT('Ctrl Pts',(23.1361577235709,-69.3831934569183,
0.));
#128060=CARTESIAN_POINT('Ctrl Pts',(23.1379034406718,-69.3572846280297,
0.));
#128061=CARTESIAN_POINT('Ctrl Pts',(23.1396223678725,-69.3314123025869,
0.));
#128062=CARTESIAN_POINT('Ctrl Pts',(23.1413145503762,-69.3055765827546,
0.));
#128063=CARTESIAN_POINT('Ctrl Pts',(23.142980033622,-69.2797775710273,0.));
#128064=CARTESIAN_POINT('Ctrl Pts',(23.1446188632931,-69.254015370231,0.));
#128065=CARTESIAN_POINT('Ctrl Pts',(23.1462310853206,-69.2282900835236,
0.));
#128066=CARTESIAN_POINT('Ctrl Pts',(23.1478167458789,-69.2026018144028,
0.));
#128067=CARTESIAN_POINT('Ctrl Pts',(23.1493758913858,-69.1769506667084,
0.));
#128068=CARTESIAN_POINT('Ctrl Pts',(23.1509085685032,-69.1513367446231,
0.));
#128069=CARTESIAN_POINT('Ctrl Pts',(23.152414824141,-69.1257601526687,0.));
#128070=CARTESIAN_POINT('Ctrl Pts',(23.1538947054614,-69.1002209957025,
0.));
#128071=CARTESIAN_POINT('Ctrl Pts',(23.1553482598762,-69.074719378928,0.));
#128072=CARTESIAN_POINT('Ctrl Pts',(23.1567755350469,-69.0492554078992,
0.));
#128073=CARTESIAN_POINT('Ctrl Pts',(23.1581765788868,-69.0238291885245,
0.));
#128074=CARTESIAN_POINT('Ctrl Pts',(23.1595514395656,-68.9984408270659,
0.));
#128075=CARTESIAN_POINT('Ctrl Pts',(23.1609001655155,-68.9730904301369,
0.));
#128076=CARTESIAN_POINT('Ctrl Pts',(23.1622228054291,-68.9477781047106,
0.));
#128077=CARTESIAN_POINT('Ctrl Pts',(23.1635194082581,-68.9225039581248,
0.));
#128078=CARTESIAN_POINT('Ctrl Pts',(23.164790023215,-68.8972680980842,0.));
#128079=CARTESIAN_POINT('Ctrl Pts',(23.1660346997763,-68.872070632661,0.));
#128080=CARTESIAN_POINT('Ctrl Pts',(23.1672534876889,-68.8469116702898,
0.));
#128081=CARTESIAN_POINT('Ctrl Pts',(23.1684464369686,-68.8217913197752,
0.));
#128082=CARTESIAN_POINT('Ctrl Pts',(23.1696135978997,-68.7967096902996,
0.));
#128083=CARTESIAN_POINT('Ctrl Pts',(23.170755021036,-68.771666891425,0.));
#128084=CARTESIAN_POINT('Ctrl Pts',(23.1718707572043,-68.746663033096,0.));
#128085=CARTESIAN_POINT('Ctrl Pts',(23.1729608575109,-68.7216982256341,
0.));
#128086=CARTESIAN_POINT('Ctrl Pts',(23.1740253733417,-68.696772579744,0.));
#128087=CARTESIAN_POINT('Ctrl Pts',(23.1750643563601,-68.6718862065216,
0.));
#128088=CARTESIAN_POINT('Ctrl Pts',(23.1760778585092,-68.6470392174564,
0.));
#128089=CARTESIAN_POINT('Ctrl Pts',(23.1770659320137,-68.6222317244342,
0.));
#128090=CARTESIAN_POINT('Ctrl Pts',(23.1780286293875,-68.597463839733,0.));
#128091=CARTESIAN_POINT('Ctrl Pts',(23.1789660034341,-68.5727356760278,
0.));
#128092=CARTESIAN_POINT('Ctrl Pts',(23.1798781072449,-68.5480473463985,
0.));
#128093=CARTESIAN_POINT('Ctrl Pts',(23.180764994201,-68.5233989643345,0.));
#128094=CARTESIAN_POINT('Ctrl Pts',(23.1816267179751,-68.4987906437356,
0.));
#128095=CARTESIAN_POINT('Ctrl Pts',(23.1824633325384,-68.4742224989099,
0.));
#128096=CARTESIAN_POINT('Ctrl Pts',(23.183274892163,-68.4496946445758,0.));
#128097=CARTESIAN_POINT('Ctrl Pts',(23.1840614514192,-68.4252071958729,
0.));
#128098=CARTESIAN_POINT('Ctrl Pts',(23.1848230651776,-68.4007602683652,
0.));
#128099=CARTESIAN_POINT('Ctrl Pts',(23.1855597886115,-68.376353978044,0.));
#128100=CARTESIAN_POINT('Ctrl Pts',(23.186271677203,-68.3519884413246,0.));
#128101=CARTESIAN_POINT('Ctrl Pts',(23.1869587867459,-68.3276637750485,
0.));
#128102=CARTESIAN_POINT('Ctrl Pts',(23.1876211733435,-68.3033800964939,
0.));
#128103=CARTESIAN_POINT('Ctrl Pts',(23.1882588934106,-68.2791375233795,
0.));
#128104=CARTESIAN_POINT('Ctrl Pts',(23.1888720036757,-68.2549361738681,
0.));
#128105=CARTESIAN_POINT('Ctrl Pts',(23.1894605611871,-68.2307761665633,
0.));
#128106=CARTESIAN_POINT('Ctrl Pts',(23.1900246233165,-68.2066576205116,
0.));
#128107=CARTESIAN_POINT('Ctrl Pts',(23.1905642477571,-68.1825806552129,
0.));
#128108=CARTESIAN_POINT('Ctrl Pts',(23.1910794925251,-68.1585453906257,
0.));
#128109=CARTESIAN_POINT('Ctrl Pts',(23.1915704159623,-68.1345519471695,
0.));
#128110=CARTESIAN_POINT('Ctrl Pts',(23.1920370767425,-68.110600445723,0.));
#128111=CARTESIAN_POINT('Ctrl Pts',(23.1924795338749,-68.0866910076251,
0.));
#128112=CARTESIAN_POINT('Ctrl Pts',(23.192897846702,-68.0628237546863,0.));
#128113=CARTESIAN_POINT('Ctrl Pts',(23.1932920749023,-68.0389988091933,
0.));
#128114=CARTESIAN_POINT('Ctrl Pts',(23.1936622784918,-68.0152162939121,
0.));
#128115=CARTESIAN_POINT('Ctrl Pts',(23.1940085178313,-67.991476332086,0.));
#128116=CARTESIAN_POINT('Ctrl Pts',(23.1943308536297,-67.9677790474385,
0.));
#128117=CARTESIAN_POINT('Ctrl Pts',(23.1946293469427,-67.9441245641842,
0.));
#128118=CARTESIAN_POINT('Ctrl Pts',(23.1949040591744,-67.9205130070324,
0.));
#128119=CARTESIAN_POINT('Ctrl Pts',(23.1951550520802,-67.8969445011916,
0.));
#128120=CARTESIAN_POINT('Ctrl Pts',(23.1953823877734,-67.8734191723667,
0.));
#128121=CARTESIAN_POINT('Ctrl Pts',(23.1955861287286,-67.8499371467616,
0.));
#128122=CARTESIAN_POINT('Ctrl Pts',(23.1957663377806,-67.8264985510917,
0.));
#128123=CARTESIAN_POINT('Ctrl Pts',(23.1959230781269,-67.8031035125887,
0.));
#128124=CARTESIAN_POINT('Ctrl Pts',(23.1960564133304,-67.7797521590045,
0.));
#128125=CARTESIAN_POINT('Ctrl Pts',(23.1961664073261,-67.7564446186079,
0.));
#128126=CARTESIAN_POINT('Ctrl Pts',(23.1962531244245,-67.7331810201883,
0.));
#128127=CARTESIAN_POINT('Ctrl Pts',(23.1963166293102,-67.7099614930671,
0.));
#128128=CARTESIAN_POINT('Ctrl Pts',(23.1963569870451,-67.6867861671031,
0.));
#128129=CARTESIAN_POINT('Ctrl Pts',(23.1963742630714,-67.6636551726964,
0.));
#128130=CARTESIAN_POINT('Ctrl Pts',(23.1963685232187,-67.6405686407863,
0.));
#128131=CARTESIAN_POINT('Ctrl Pts',(23.1963398337068,-67.6175267028555,
0.));
#128132=CARTESIAN_POINT('Ctrl Pts',(23.1962882611452,-67.5945294909426,
0.));
#128133=CARTESIAN_POINT('Ctrl Pts',(23.196213872536,-67.5715771376461,0.));
#128134=CARTESIAN_POINT('Ctrl Pts',(23.1961167352771,-67.5486697761288,
0.));
#128135=CARTESIAN_POINT('Ctrl Pts',(23.19599691717,-67.5258075401146,0.));
#128136=CARTESIAN_POINT('Ctrl Pts',(23.1958544864215,-67.502990563895,0.));
#128137=CARTESIAN_POINT('Ctrl Pts',(23.195689511644,-67.4802189823408,0.));
#128138=CARTESIAN_POINT('Ctrl Pts',(23.1955020618589,-67.4574929309076,
0.));
#128139=CARTESIAN_POINT('Ctrl Pts',(23.1952922065012,-67.4348125456398,
0.));
#128140=CARTESIAN_POINT('Ctrl Pts',(23.1950600154265,-67.412177963168,0.));
#128141=CARTESIAN_POINT('Ctrl Pts',(23.1948055589128,-67.3895893207182,
0.));
#128142=CARTESIAN_POINT('Ctrl Pts',(23.194528907661,-67.3670467561212,0.));
#128143=CARTESIAN_POINT('Ctrl Pts',(23.1942301327978,-67.3445504078176,
0.));
#128144=CARTESIAN_POINT('Ctrl Pts',(23.1939093058801,-67.3221004148604,
0.));
#128145=CARTESIAN_POINT('Ctrl Pts',(23.1935664989018,-67.2996969169098,
0.));
#128146=CARTESIAN_POINT('Ctrl Pts',(23.1932017842952,-67.2773400542477,
0.));
#128147=CARTESIAN_POINT('Ctrl Pts',(23.1928152349342,-67.2550299677888,
0.));
#128148=CARTESIAN_POINT('Ctrl Pts',(23.1924069241385,-67.232766799088,0.));
#128149=CARTESIAN_POINT('Ctrl Pts',(23.1919769256803,-67.2105506903447,
0.));
#128150=CARTESIAN_POINT('Ctrl Pts',(23.1915253137923,-67.1883817844038,
0.));
#128151=CARTESIAN_POINT('Ctrl Pts',(23.1910521631657,-67.1662602247639,
0.));
#128152=CARTESIAN_POINT('Ctrl Pts',(23.1905575489504,-67.1441861555817,
0.));
#128153=CARTESIAN_POINT('Ctrl Pts',(23.1900415467574,-67.1221597216741,
0.));
#128154=CARTESIAN_POINT('Ctrl Pts',(23.1895042326626,-67.1001810685143,
0.));
#128155=CARTESIAN_POINT('Ctrl Pts',(23.1889456832119,-67.0782503422305,
0.));
#128156=CARTESIAN_POINT('Ctrl Pts',(23.1883659754271,-67.0563676896325,
0.));
#128157=CARTESIAN_POINT('Ctrl Pts',(23.1877651868157,-67.0345332582306,
0.));
#128158=CARTESIAN_POINT('Ctrl Pts',(23.1871433953793,-67.0127471962501,
0.));
#128159=CARTESIAN_POINT('Ctrl Pts',(23.1865006796283,-66.9910096526462,
0.));
#128160=CARTESIAN_POINT('Ctrl Pts',(23.1858371185842,-66.9693207771031,
0.));
#128161=CARTESIAN_POINT('Ctrl Pts',(23.1851527917657,-66.9476807200203,
0.));
#128162=CARTESIAN_POINT('Ctrl Pts',(23.1844477791814,-66.9260896324949,
0.));
#128163=CARTESIAN_POINT('Ctrl Pts',(23.1837221613235,-66.9045476663063,
0.));
#128164=CARTESIAN_POINT('Ctrl Pts',(23.1829760191591,-66.8830549738795,
0.));
#128165=CARTESIAN_POINT('Ctrl Pts',(23.1822094341517,-66.8616117083331,
0.));
#128166=CARTESIAN_POINT('Ctrl Pts',(23.1814224882953,-66.8402180235566,
0.));
#128167=CARTESIAN_POINT('Ctrl Pts',(23.1806152641475,-66.8188740742727,
0.));
#128168=CARTESIAN_POINT('Ctrl Pts',(23.1797878448639,-66.7975800161,0.));
#128169=CARTESIAN_POINT('Ctrl Pts',(23.1789403142366,-66.7763360056121,
0.));
#128170=CARTESIAN_POINT('Ctrl Pts',(23.17807275663,-66.7551422002204,0.));
#128171=CARTESIAN_POINT('Ctrl Pts',(23.1771852569131,-66.7339987580427,
0.));
#128172=CARTESIAN_POINT('Ctrl Pts',(23.1762779004044,-66.7129058377896,
0.));
#128173=CARTESIAN_POINT('Ctrl Pts',(23.1753507727939,-66.6918635985972,
0.));
#128174=CARTESIAN_POINT('Ctrl Pts',(23.1744039601381,-66.6708722000079,
0.));
#128175=CARTESIAN_POINT('Ctrl Pts',(23.1734375490431,-66.6499318023473,
0.));
#128176=CARTESIAN_POINT('Ctrl Pts',(23.1724516268302,-66.6290425670549,
0.));
#128177=CARTESIAN_POINT('Ctrl Pts',(23.1714462816789,-66.6082046569644,
0.));
#128178=CARTESIAN_POINT('Ctrl Pts',(23.1704216028614,-66.5874182367563,
0.));
#128179=CARTESIAN_POINT('Ctrl Pts',(23.1693776805865,-66.5666834726454,
0.));
#128180=CARTESIAN_POINT('Ctrl Pts',(23.1683146055726,-66.5460005315376,
0.));
#128181=CARTESIAN_POINT('Ctrl Pts',(23.1672324686926,-66.5253695803206,
0.));
#128182=CARTESIAN_POINT('Ctrl Pts',(23.1661313606132,-66.5047907851348,
0.));
#128183=CARTESIAN_POINT('Ctrl Pts',(23.1650113713808,-66.4842643105311,
0.));
#128184=CARTESIAN_POINT('Ctrl Pts',(23.1638725912195,-66.4637903210727,
0.));
#128185=CARTESIAN_POINT('Ctrl Pts',(23.1627151114883,-66.4433689832478,
0.));
#128186=CARTESIAN_POINT('Ctrl Pts',(23.1615390254631,-66.4230004670278,
0.));
#128187=CARTESIAN_POINT('Ctrl Pts',(23.160344429474,-66.4026849481232,0.));
#128188=CARTESIAN_POINT('Ctrl Pts',(23.1591314230083,-66.3824226081802,
0.));
#128189=CARTESIAN_POINT('Ctrl Pts',(23.1579001063423,-66.3622136300654,
0.));
#128190=CARTESIAN_POINT('Ctrl Pts',(23.1566505784621,-66.3420581937147,
0.));
#128191=CARTESIAN_POINT('Ctrl Pts',(23.1553829352539,-66.3219564725184,
0.));
#128192=CARTESIAN_POINT('Ctrl Pts',(23.154097266619,-66.3019086275445,0.));
#128193=CARTESIAN_POINT('Ctrl Pts',(23.1527936592651,-66.281914813114,0.));
#128194=CARTESIAN_POINT('Ctrl Pts',(23.1514722022503,-66.2619751878793,
0.));
#128195=CARTESIAN_POINT('Ctrl Pts',(23.1501329914487,-66.2420899237318,
0.));
#128196=CARTESIAN_POINT('Ctrl Pts',(23.1487761349297,-66.2222592165398,
0.));
#128197=CARTESIAN_POINT('Ctrl Pts',(23.147401756643,-66.2024832934733,0.));
#128198=CARTESIAN_POINT('Ctrl Pts',(23.1460099850704,-66.1827623902755,
0.));
#128199=CARTESIAN_POINT('Ctrl Pts',(23.1446009424871,-66.163096729667,0.));
#128200=CARTESIAN_POINT('Ctrl Pts',(23.1431747350127,-66.14348650151,0.));
#128201=CARTESIAN_POINT('Ctrl Pts',(23.1417314398501,-66.1239318368803,
0.));
#128202=CARTESIAN_POINT('Ctrl Pts',(23.140271103958,-66.1044328067739,0.));
#128203=CARTESIAN_POINT('Ctrl Pts',(23.1390892229923,-66.0888781152779,
0.));
#128204=CARTESIAN_POINT('Ctrl Pts',(23.1381951597491,-66.0772371487475,
0.));
#128205=CARTESIAN_POINT('Ctrl Pts',(23.1375957166138,-66.0694876382212,
0.));
#128206=CARTESIAN_POINT('Ctrl Pts',(23.1372951448023,-66.0656156664139,
0.));
#128207=CARTESIAN_POINT('Ctrl Pts',(16.7341474417544,-72.5962692526112,
0.));
#128208=CARTESIAN_POINT('Ctrl Pts',(16.7341474417544,-72.5962692526112,
12.));
#128209=CARTESIAN_POINT('Ctrl Pts',(16.7352885767485,-72.5907910746008,
0.));
#128210=CARTESIAN_POINT('Ctrl Pts',(16.7352885767485,-72.5907910746008,
12.));
#128211=CARTESIAN_POINT('Ctrl Pts',(16.7375676985344,-72.5798376087774,
0.));
#128212=CARTESIAN_POINT('Ctrl Pts',(16.7375676985344,-72.5798376087774,
12.));
#128213=CARTESIAN_POINT('Ctrl Pts',(16.7409769366072,-72.5634160806351,
0.));
#128214=CARTESIAN_POINT('Ctrl Pts',(16.7409769366072,-72.5634160806351,
12.));
#128215=CARTESIAN_POINT('Ctrl Pts',(16.7455036973866,-72.5415380516637,
0.));
#128216=CARTESIAN_POINT('Ctrl Pts',(16.7455036973866,-72.5415380516637,
12.));
#128217=CARTESIAN_POINT('Ctrl Pts',(16.7511306618915,-72.514219427383,0.));
#128218=CARTESIAN_POINT('Ctrl Pts',(16.7511306618915,-72.514219427383,12.));
#128219=CARTESIAN_POINT('Ctrl Pts',(16.7567261380687,-72.4869297342427,
0.));
#128220=CARTESIAN_POINT('Ctrl Pts',(16.7567261380687,-72.4869297342427,
12.));
#128221=CARTESIAN_POINT('Ctrl Pts',(16.7622901280758,-72.4596690055437,
0.));
#128222=CARTESIAN_POINT('Ctrl Pts',(16.7622901280758,-72.4596690055437,
12.));
#128223=CARTESIAN_POINT('Ctrl Pts',(16.7678226404162,-72.4324372916746,
0.));
#128224=CARTESIAN_POINT('Ctrl Pts',(16.7678226404162,-72.4324372916746,
12.));
#128225=CARTESIAN_POINT('Ctrl Pts',(16.7733236932135,-72.4052346647799,
0.));
#128226=CARTESIAN_POINT('Ctrl Pts',(16.7733236932135,-72.4052346647799,
12.));
#128227=CARTESIAN_POINT('Ctrl Pts',(16.7787933137498,-72.3780612167786,
0.));
#128228=CARTESIAN_POINT('Ctrl Pts',(16.7787933137498,-72.3780612167786,
12.));
#128229=CARTESIAN_POINT('Ctrl Pts',(16.7842315351362,-72.3509170522838,
0.));
#128230=CARTESIAN_POINT('Ctrl Pts',(16.7842315351362,-72.3509170522838,
12.));
#128231=CARTESIAN_POINT('Ctrl Pts',(16.7896383937821,-72.3238022829223,
0.));
#128232=CARTESIAN_POINT('Ctrl Pts',(16.7896383937821,-72.3238022829223,
12.));
#128233=CARTESIAN_POINT('Ctrl Pts',(16.7950139266121,-72.2967170212353,
0.));
#128234=CARTESIAN_POINT('Ctrl Pts',(16.7950139266121,-72.2967170212353,
12.));
#128235=CARTESIAN_POINT('Ctrl Pts',(16.8003581682248,-72.2696613743782,
0.));
#128236=CARTESIAN_POINT('Ctrl Pts',(16.8003581682248,-72.2696613743782,
12.));
#128237=CARTESIAN_POINT('Ctrl Pts',(16.8056711485821,-72.2426354390213,
0.));
#128238=CARTESIAN_POINT('Ctrl Pts',(16.8056711485821,-72.2426354390213,
12.));
#128239=CARTESIAN_POINT('Ctrl Pts',(16.8109528945896,-72.2156393048975,
0.));
#128240=CARTESIAN_POINT('Ctrl Pts',(16.8109528945896,-72.2156393048975,
12.));
#128241=CARTESIAN_POINT('Ctrl Pts',(16.8162034312269,-72.1886730573452,
0.));
#128242=CARTESIAN_POINT('Ctrl Pts',(16.8162034312269,-72.1886730573452,
12.));
#128243=CARTESIAN_POINT('Ctrl Pts',(16.8214227828942,-72.1617367803235,
0.));
#128244=CARTESIAN_POINT('Ctrl Pts',(16.8214227828942,-72.1617367803235,
12.));
#128245=CARTESIAN_POINT('Ctrl Pts',(16.8266109745795,-72.13483055902,0.));
#128246=CARTESIAN_POINT('Ctrl Pts',(16.8266109745795,-72.13483055902,12.));
#128247=CARTESIAN_POINT('Ctrl Pts',(16.8317680333404,-72.1079544831513,
0.));
#128248=CARTESIAN_POINT('Ctrl Pts',(16.8317680333404,-72.1079544831513,
12.));
#128249=CARTESIAN_POINT('Ctrl Pts',(16.8368939881446,-72.0811086466121,
0.));
#128250=CARTESIAN_POINT('Ctrl Pts',(16.8368939881446,-72.0811086466121,
12.));
#128251=CARTESIAN_POINT('Ctrl Pts',(16.8419888691976,-72.0542931459825,
0.));
#128252=CARTESIAN_POINT('Ctrl Pts',(16.8419888691976,-72.0542931459825,
12.));
#128253=CARTESIAN_POINT('Ctrl Pts',(16.8470527074275,-72.0275080793727,
0.));
#128254=CARTESIAN_POINT('Ctrl Pts',(16.8470527074275,-72.0275080793727,
12.));
#128255=CARTESIAN_POINT('Ctrl Pts',(16.8520855339445,-72.0007535452081,
0.));
#128256=CARTESIAN_POINT('Ctrl Pts',(16.8520855339445,-72.0007535452081,
12.));
#128257=CARTESIAN_POINT('Ctrl Pts',(16.8570873794269,-71.9740296408347,
0.));
#128258=CARTESIAN_POINT('Ctrl Pts',(16.8570873794269,-71.9740296408347,
12.));
#128259=CARTESIAN_POINT('Ctrl Pts',(16.8620582738437,-71.9473364618922,
0.));
#128260=CARTESIAN_POINT('Ctrl Pts',(16.8620582738437,-71.9473364618922,
12.));
#128261=CARTESIAN_POINT('Ctrl Pts',(16.866998246792,-71.9206741030887,0.));
#128262=CARTESIAN_POINT('Ctrl Pts',(16.866998246792,-71.9206741030887,12.));
#128263=CARTESIAN_POINT('Ctrl Pts',(16.871907327697,-71.8940426586534,0.));
#128264=CARTESIAN_POINT('Ctrl Pts',(16.871907327697,-71.8940426586534,12.));
#128265=CARTESIAN_POINT('Ctrl Pts',(16.87678554607,-71.8674422229149,0.));
#128266=CARTESIAN_POINT('Ctrl Pts',(16.87678554607,-71.8674422229149,12.));
#128267=CARTESIAN_POINT('Ctrl Pts',(16.881632931747,-71.8408728908258,0.));
#128268=CARTESIAN_POINT('Ctrl Pts',(16.881632931747,-71.8408728908258,12.));
#128269=CARTESIAN_POINT('Ctrl Pts',(16.8864495151344,-71.8143347584962,
0.));
#128270=CARTESIAN_POINT('Ctrl Pts',(16.8864495151344,-71.8143347584962,
12.));
#128271=CARTESIAN_POINT('Ctrl Pts',(16.8912353270942,-71.7878279229546,
0.));
#128272=CARTESIAN_POINT('Ctrl Pts',(16.8912353270942,-71.7878279229546,
12.));
#128273=CARTESIAN_POINT('Ctrl Pts',(16.8959903988409,-71.7613524819235,
0.));
#128274=CARTESIAN_POINT('Ctrl Pts',(16.8959903988409,-71.7613524819235,
12.));
#128275=CARTESIAN_POINT('Ctrl Pts',(16.9007147618344,-71.7349085335796,
0.));
#128276=CARTESIAN_POINT('Ctrl Pts',(16.9007147618344,-71.7349085335796,
12.));
#128277=CARTESIAN_POINT('Ctrl Pts',(16.9054084476847,-71.7084961763357,
0.));
#128278=CARTESIAN_POINT('Ctrl Pts',(16.9054084476847,-71.7084961763357,
12.));
#128279=CARTESIAN_POINT('Ctrl Pts',(16.9100714880368,-71.6821155085612,
0.));
#128280=CARTESIAN_POINT('Ctrl Pts',(16.9100714880368,-71.6821155085612,
12.));
#128281=CARTESIAN_POINT('Ctrl Pts',(16.9147039145717,-71.6557666285917,
0.));
#128282=CARTESIAN_POINT('Ctrl Pts',(16.9147039145717,-71.6557666285917,
12.));
#128283=CARTESIAN_POINT('Ctrl Pts',(16.9193057590607,-71.6294496348652,
0.));
#128284=CARTESIAN_POINT('Ctrl Pts',(16.9193057590607,-71.6294496348652,
12.));
#128285=CARTESIAN_POINT('Ctrl Pts',(16.9238770534071,-71.6031646260174,
0.));
#128286=CARTESIAN_POINT('Ctrl Pts',(16.9238770534071,-71.6031646260174,
12.));
#128287=CARTESIAN_POINT('Ctrl Pts',(16.9284178296933,-71.5769117009842,
0.));
#128288=CARTESIAN_POINT('Ctrl Pts',(16.9284178296933,-71.5769117009842,
12.));
#128289=CARTESIAN_POINT('Ctrl Pts',(16.9329281202377,-71.5506909591128,
0.));
#128290=CARTESIAN_POINT('Ctrl Pts',(16.9329281202377,-71.5506909591128,
12.));
#128291=CARTESIAN_POINT('Ctrl Pts',(16.9374079576201,-71.5245025002139,
0.));
#128292=CARTESIAN_POINT('Ctrl Pts',(16.9374079576201,-71.5245025002139,
12.));
#128293=CARTESIAN_POINT('Ctrl Pts',(16.9418573746488,-71.4983464245055,
0.));
#128294=CARTESIAN_POINT('Ctrl Pts',(16.9418573746488,-71.4983464245055,
12.));
#128295=CARTESIAN_POINT('Ctrl Pts',(16.9462764043443,-71.4722228325794,
0.));
#128296=CARTESIAN_POINT('Ctrl Pts',(16.9462764043443,-71.4722228325794,
12.));
#128297=CARTESIAN_POINT('Ctrl Pts',(16.9506650799188,-71.4461318253563,
0.));
#128298=CARTESIAN_POINT('Ctrl Pts',(16.9506650799188,-71.4461318253563,
12.));
#128299=CARTESIAN_POINT('Ctrl Pts',(16.955023434762,-71.4200735040384,0.));
#128300=CARTESIAN_POINT('Ctrl Pts',(16.955023434762,-71.4200735040384,12.));
#128301=CARTESIAN_POINT('Ctrl Pts',(16.9593515024276,-71.3940479700677,
0.));
#128302=CARTESIAN_POINT('Ctrl Pts',(16.9593515024276,-71.3940479700677,
12.));
#128303=CARTESIAN_POINT('Ctrl Pts',(16.9636493166397,-71.3680553251562,
0.));
#128304=CARTESIAN_POINT('Ctrl Pts',(16.9636493166397,-71.3680553251562,
12.));
#128305=CARTESIAN_POINT('Ctrl Pts',(16.9679169112994,-71.3420956713082,
0.));
#128306=CARTESIAN_POINT('Ctrl Pts',(16.9679169112994,-71.3420956713082,
12.));
#128307=CARTESIAN_POINT('Ctrl Pts',(16.9721543204951,-71.3161691108427,
0.));
#128308=CARTESIAN_POINT('Ctrl Pts',(16.9721543204951,-71.3161691108427,
12.));
#128309=CARTESIAN_POINT('Ctrl Pts',(16.9763615785136,-71.290275746412,0.));
#128310=CARTESIAN_POINT('Ctrl Pts',(16.9763615785136,-71.290275746412,12.));
#128311=CARTESIAN_POINT('Ctrl Pts',(16.9805387198571,-71.2644156810198,
0.));
#128312=CARTESIAN_POINT('Ctrl Pts',(16.9805387198571,-71.2644156810198,
12.));
#128313=CARTESIAN_POINT('Ctrl Pts',(16.9846857792383,-71.2385890180221,
0.));
#128314=CARTESIAN_POINT('Ctrl Pts',(16.9846857792383,-71.2385890180221,
12.));
#128315=CARTESIAN_POINT('Ctrl Pts',(16.9888027915742,-71.212795861124,0.));
#128316=CARTESIAN_POINT('Ctrl Pts',(16.9888027915742,-71.212795861124,12.));
#128317=CARTESIAN_POINT('Ctrl Pts',(16.9928897919828,-71.187036314374,0.));
#128318=CARTESIAN_POINT('Ctrl Pts',(16.9928897919828,-71.187036314374,12.));
#128319=CARTESIAN_POINT('Ctrl Pts',(16.9969468157824,-71.1613104821568,
0.));
#128320=CARTESIAN_POINT('Ctrl Pts',(16.9969468157824,-71.1613104821568,
12.));
#128321=CARTESIAN_POINT('Ctrl Pts',(17.0009738984935,-71.1356184691806,
0.));
#128322=CARTESIAN_POINT('Ctrl Pts',(17.0009738984935,-71.1356184691806,
12.));
#128323=CARTESIAN_POINT('Ctrl Pts',(17.0049710758393,-71.1099603804786,
0.));
#128324=CARTESIAN_POINT('Ctrl Pts',(17.0049710758393,-71.1099603804786,
12.));
#128325=CARTESIAN_POINT('Ctrl Pts',(17.0089383837437,-71.0843363214221,
0.));
#128326=CARTESIAN_POINT('Ctrl Pts',(17.0089383837437,-71.0843363214221,
12.));
#128327=CARTESIAN_POINT('Ctrl Pts',(17.0128758583334,-71.0587463977268,
0.));
#128328=CARTESIAN_POINT('Ctrl Pts',(17.0128758583334,-71.0587463977268,
12.));
#128329=CARTESIAN_POINT('Ctrl Pts',(17.0167835359419,-71.0331907154574,
0.));
#128330=CARTESIAN_POINT('Ctrl Pts',(17.0167835359419,-71.0331907154574,
12.));
#128331=CARTESIAN_POINT('Ctrl Pts',(17.0206614531166,-71.0076693810301,
0.));
#128332=CARTESIAN_POINT('Ctrl Pts',(17.0206614531166,-71.0076693810301,
12.));
#128333=CARTESIAN_POINT('Ctrl Pts',(17.0245096466229,-70.9821825012136,
0.));
#128334=CARTESIAN_POINT('Ctrl Pts',(17.0245096466229,-70.9821825012136,
12.));
#128335=CARTESIAN_POINT('Ctrl Pts',(17.0283281534392,-70.956730183136,0.));
#128336=CARTESIAN_POINT('Ctrl Pts',(17.0283281534392,-70.956730183136,12.));
#128337=CARTESIAN_POINT('Ctrl Pts',(17.0321170107564,-70.9313125342876,
0.));
#128338=CARTESIAN_POINT('Ctrl Pts',(17.0321170107564,-70.9313125342876,
12.));
#128339=CARTESIAN_POINT('Ctrl Pts',(17.0358762559786,-70.9059296625214,
0.));
#128340=CARTESIAN_POINT('Ctrl Pts',(17.0358762559786,-70.9059296625214,
12.));
#128341=CARTESIAN_POINT('Ctrl Pts',(17.0396059267277,-70.8805816760501,
0.));
#128342=CARTESIAN_POINT('Ctrl Pts',(17.0396059267277,-70.8805816760501,
12.));
#128343=CARTESIAN_POINT('Ctrl Pts',(17.0433060608474,-70.8552686834423,
0.));
#128344=CARTESIAN_POINT('Ctrl Pts',(17.0433060608474,-70.8552686834423,
12.));
#128345=CARTESIAN_POINT('Ctrl Pts',(17.0469766964001,-70.8299907936334,
0.));
#128346=CARTESIAN_POINT('Ctrl Pts',(17.0469766964001,-70.8299907936334,
12.));
#128347=CARTESIAN_POINT('Ctrl Pts',(17.0506178716661,-70.8047481159298,
0.));
#128348=CARTESIAN_POINT('Ctrl Pts',(17.0506178716661,-70.8047481159298,
12.));
#128349=CARTESIAN_POINT('Ctrl Pts',(17.0542296251462,-70.7795407600127,
0.));
#128350=CARTESIAN_POINT('Ctrl Pts',(17.0542296251462,-70.7795407600127,
12.));
#128351=CARTESIAN_POINT('Ctrl Pts',(17.0578119955651,-70.754368835938,0.));
#128352=CARTESIAN_POINT('Ctrl Pts',(17.0578119955651,-70.754368835938,12.));
#128353=CARTESIAN_POINT('Ctrl Pts',(17.0613650218788,-70.7292324541348,
0.));
#128354=CARTESIAN_POINT('Ctrl Pts',(17.0613650218788,-70.7292324541348,
12.));
#128355=CARTESIAN_POINT('Ctrl Pts',(17.0648887432714,-70.7041317254127,
0.));
#128356=CARTESIAN_POINT('Ctrl Pts',(17.0648887432714,-70.7041317254127,
12.));
#128357=CARTESIAN_POINT('Ctrl Pts',(17.0683831991532,-70.6790667609678,
0.));
#128358=CARTESIAN_POINT('Ctrl Pts',(17.0683831991532,-70.6790667609678,
12.));
#128359=CARTESIAN_POINT('Ctrl Pts',(17.0718484291623,-70.6540376723839,
0.));
#128360=CARTESIAN_POINT('Ctrl Pts',(17.0718484291623,-70.6540376723839,
12.));
#128361=CARTESIAN_POINT('Ctrl Pts',(17.0752844731679,-70.6290445716341,
0.));
#128362=CARTESIAN_POINT('Ctrl Pts',(17.0752844731679,-70.6290445716341,
12.));
#128363=CARTESIAN_POINT('Ctrl Pts',(17.0786913712766,-70.6040875710762,
0.));
#128364=CARTESIAN_POINT('Ctrl Pts',(17.0786913712766,-70.6040875710762,
12.));
#128365=CARTESIAN_POINT('Ctrl Pts',(17.0820691638314,-70.5791667834599,
0.));
#128366=CARTESIAN_POINT('Ctrl Pts',(17.0820691638314,-70.5791667834599,
12.));
#128367=CARTESIAN_POINT('Ctrl Pts',(17.085417891409,-70.5542823219346,0.));
#128368=CARTESIAN_POINT('Ctrl Pts',(17.085417891409,-70.5542823219346,12.));
#128369=CARTESIAN_POINT('Ctrl Pts',(17.0887375948221,-70.5294343000516,
0.));
#128370=CARTESIAN_POINT('Ctrl Pts',(17.0887375948221,-70.5294343000516,
12.));
#128371=CARTESIAN_POINT('Ctrl Pts',(17.0920283151217,-70.5046228317669,
0.));
#128372=CARTESIAN_POINT('Ctrl Pts',(17.0920283151217,-70.5046228317669,
12.));
#128373=CARTESIAN_POINT('Ctrl Pts',(17.0952900936044,-70.4798480314364,
0.));
#128374=CARTESIAN_POINT('Ctrl Pts',(17.0952900936044,-70.4798480314364,
12.));
#128375=CARTESIAN_POINT('Ctrl Pts',(17.098522971812,-70.4551100138221,0.));
#128376=CARTESIAN_POINT('Ctrl Pts',(17.098522971812,-70.4551100138221,12.));
#128377=CARTESIAN_POINT('Ctrl Pts',(17.1017269915289,-70.4304088940998,
0.));
#128378=CARTESIAN_POINT('Ctrl Pts',(17.1017269915289,-70.4304088940998,
12.));
#128379=CARTESIAN_POINT('Ctrl Pts',(17.1049021947833,-70.4057447878621,
0.));
#128380=CARTESIAN_POINT('Ctrl Pts',(17.1049021947833,-70.4057447878621,
12.));
#128381=CARTESIAN_POINT('Ctrl Pts',(17.1080486238499,-70.3811178111206,
0.));
#128382=CARTESIAN_POINT('Ctrl Pts',(17.1080486238499,-70.3811178111206,
12.));
#128383=CARTESIAN_POINT('Ctrl Pts',(17.111166321257,-70.356528080303,0.));
#128384=CARTESIAN_POINT('Ctrl Pts',(17.111166321257,-70.356528080303,12.));
#128385=CARTESIAN_POINT('Ctrl Pts',(17.1142553297869,-70.3319757122576,
0.));
#128386=CARTESIAN_POINT('Ctrl Pts',(17.1142553297869,-70.3319757122576,
12.));
#128387=CARTESIAN_POINT('Ctrl Pts',(17.1173156924733,-70.3074608242613,
0.));
#128388=CARTESIAN_POINT('Ctrl Pts',(17.1173156924733,-70.3074608242613,
12.));
#128389=CARTESIAN_POINT('Ctrl Pts',(17.1203474526031,-70.2829835340239,
0.));
#128390=CARTESIAN_POINT('Ctrl Pts',(17.1203474526031,-70.2829835340239,
12.));
#128391=CARTESIAN_POINT('Ctrl Pts',(17.1233506537176,-70.2585439596899,
0.));
#128392=CARTESIAN_POINT('Ctrl Pts',(17.1233506537176,-70.2585439596899,
12.));
#128393=CARTESIAN_POINT('Ctrl Pts',(17.1263253396202,-70.2341422198362,
0.));
#128394=CARTESIAN_POINT('Ctrl Pts',(17.1263253396202,-70.2341422198362,
12.));
#128395=CARTESIAN_POINT('Ctrl Pts',(17.1292715543779,-70.2097784334749,
0.));
#128396=CARTESIAN_POINT('Ctrl Pts',(17.1292715543779,-70.2097784334749,
12.));
#128397=CARTESIAN_POINT('Ctrl Pts',(17.1321893423183,-70.1854527200636,
0.));
#128398=CARTESIAN_POINT('Ctrl Pts',(17.1321893423183,-70.1854527200636,
12.));
#128399=CARTESIAN_POINT('Ctrl Pts',(17.1350787480313,-70.1611651995085,
0.));
#128400=CARTESIAN_POINT('Ctrl Pts',(17.1350787480313,-70.1611651995085,
12.));
#128401=CARTESIAN_POINT('Ctrl Pts',(17.1379398163708,-70.1369159921686,
0.));
#128402=CARTESIAN_POINT('Ctrl Pts',(17.1379398163708,-70.1369159921686,
12.));
#128403=CARTESIAN_POINT('Ctrl Pts',(17.1407725924615,-70.1127052188515,
0.));
#128404=CARTESIAN_POINT('Ctrl Pts',(17.1407725924615,-70.1127052188515,
12.));
#128405=CARTESIAN_POINT('Ctrl Pts',(17.1435771217015,-70.0885330008169,
0.));
#128406=CARTESIAN_POINT('Ctrl Pts',(17.1435771217015,-70.0885330008169,
12.));
#128407=CARTESIAN_POINT('Ctrl Pts',(17.1463534497592,-70.0643994597865,
0.));
#128408=CARTESIAN_POINT('Ctrl Pts',(17.1463534497592,-70.0643994597865,
12.));
#128409=CARTESIAN_POINT('Ctrl Pts',(17.1491016225748,-70.040304717948,0.));
#128410=CARTESIAN_POINT('Ctrl Pts',(17.1491016225748,-70.040304717948,12.));
#128411=CARTESIAN_POINT('Ctrl Pts',(17.1518216863624,-70.0162488979586,
0.));
#128412=CARTESIAN_POINT('Ctrl Pts',(17.1518216863624,-70.0162488979586,
12.));
#128413=CARTESIAN_POINT('Ctrl Pts',(17.1545136876161,-69.9922321229428,
0.));
#128414=CARTESIAN_POINT('Ctrl Pts',(17.1545136876161,-69.9922321229428,
12.));
#128415=CARTESIAN_POINT('Ctrl Pts',(17.157177673114,-69.9682545164942,0.));
#128416=CARTESIAN_POINT('Ctrl Pts',(17.157177673114,-69.9682545164942,12.));
#128417=CARTESIAN_POINT('Ctrl Pts',(17.1598136899144,-69.9443162026865,
0.));
#128418=CARTESIAN_POINT('Ctrl Pts',(17.1598136899144,-69.9443162026865,
12.));
#128419=CARTESIAN_POINT('Ctrl Pts',(17.1624217853577,-69.9204173060779,
0.));
#128420=CARTESIAN_POINT('Ctrl Pts',(17.1624217853577,-69.9204173060779,
12.));
#128421=CARTESIAN_POINT('Ctrl Pts',(17.1650020070686,-69.8965579517147,
0.));
#128422=CARTESIAN_POINT('Ctrl Pts',(17.1650020070686,-69.8965579517147,
12.));
#128423=CARTESIAN_POINT('Ctrl Pts',(17.1675544029621,-69.8727382651292,
0.));
#128424=CARTESIAN_POINT('Ctrl Pts',(17.1675544029621,-69.8727382651292,
12.));
#128425=CARTESIAN_POINT('Ctrl Pts',(17.1700790212476,-69.8489583723417,
0.));
#128426=CARTESIAN_POINT('Ctrl Pts',(17.1700790212476,-69.8489583723417,
12.));
#128427=CARTESIAN_POINT('Ctrl Pts',(17.1725759104254,-69.8252183998713,
0.));
#128428=CARTESIAN_POINT('Ctrl Pts',(17.1725759104254,-69.8252183998713,
12.));
#128429=CARTESIAN_POINT('Ctrl Pts',(17.1750451192887,-69.8015184747404,
0.));
#128430=CARTESIAN_POINT('Ctrl Pts',(17.1750451192887,-69.8015184747404,
12.));
#128431=CARTESIAN_POINT('Ctrl Pts',(17.1774866969255,-69.7778587244788,
0.));
#128432=CARTESIAN_POINT('Ctrl Pts',(17.1774866969255,-69.7778587244788,
12.));
#128433=CARTESIAN_POINT('Ctrl Pts',(17.1799006927255,-69.7542392771216,
0.));
#128434=CARTESIAN_POINT('Ctrl Pts',(17.1799006927255,-69.7542392771216,
12.));
#128435=CARTESIAN_POINT('Ctrl Pts',(17.1822871563834,-69.7306602612125,
0.));
#128436=CARTESIAN_POINT('Ctrl Pts',(17.1822871563834,-69.7306602612125,
12.));
#128437=CARTESIAN_POINT('Ctrl Pts',(17.1846461378966,-69.7071218058149,
0.));
#128438=CARTESIAN_POINT('Ctrl Pts',(17.1846461378966,-69.7071218058149,
12.));
#128439=CARTESIAN_POINT('Ctrl Pts',(17.1869776875663,-69.6836240405151,
0.));
#128440=CARTESIAN_POINT('Ctrl Pts',(17.1869776875663,-69.6836240405151,
12.));
#128441=CARTESIAN_POINT('Ctrl Pts',(17.1892818560004,-69.6601670954277,
0.));
#128442=CARTESIAN_POINT('Ctrl Pts',(17.1892818560004,-69.6601670954277,
12.));
#128443=CARTESIAN_POINT('Ctrl Pts',(17.1915586941198,-69.6367511011927,
0.));
#128444=CARTESIAN_POINT('Ctrl Pts',(17.1915586941198,-69.6367511011927,
12.));
#128445=CARTESIAN_POINT('Ctrl Pts',(17.1938082531619,-69.6133761889787,
0.));
#128446=CARTESIAN_POINT('Ctrl Pts',(17.1938082531619,-69.6133761889787,
12.));
#128447=CARTESIAN_POINT('Ctrl Pts',(17.1960305846787,-69.5900424904954,
0.));
#128448=CARTESIAN_POINT('Ctrl Pts',(17.1960305846787,-69.5900424904954,
12.));
#128449=CARTESIAN_POINT('Ctrl Pts',(17.198225740538,-69.5667501379984,0.));
#128450=CARTESIAN_POINT('Ctrl Pts',(17.198225740538,-69.5667501379984,12.));
#128451=CARTESIAN_POINT('Ctrl Pts',(17.2003937729266,-69.5434992642932,
0.));
#128452=CARTESIAN_POINT('Ctrl Pts',(17.2003937729266,-69.5434992642932,
12.));
#128453=CARTESIAN_POINT('Ctrl Pts',(17.2025347343568,-69.5202900027329,
0.));
#128454=CARTESIAN_POINT('Ctrl Pts',(17.2025347343568,-69.5202900027329,
12.));
#128455=CARTESIAN_POINT('Ctrl Pts',(17.2046486776697,-69.497122487222,0.));
#128456=CARTESIAN_POINT('Ctrl Pts',(17.2046486776697,-69.497122487222,12.));
#128457=CARTESIAN_POINT('Ctrl Pts',(17.2067356560326,-69.4739968522271,
0.));
#128458=CARTESIAN_POINT('Ctrl Pts',(17.2067356560326,-69.4739968522271,
12.));
#128459=CARTESIAN_POINT('Ctrl Pts',(17.208795722942,-69.4509132327836,0.));
#128460=CARTESIAN_POINT('Ctrl Pts',(17.208795722942,-69.4509132327836,12.));
#128461=CARTESIAN_POINT('Ctrl Pts',(17.2108289322258,-69.4278717644989,
0.));
#128462=CARTESIAN_POINT('Ctrl Pts',(17.2108289322258,-69.4278717644989,
12.));
#128463=CARTESIAN_POINT('Ctrl Pts',(17.2128353380511,-69.4048725835516,
0.));
#128464=CARTESIAN_POINT('Ctrl Pts',(17.2128353380511,-69.4048725835516,
12.));
#128465=CARTESIAN_POINT('Ctrl Pts',(17.2148149949261,-69.3819158266955,
0.));
#128466=CARTESIAN_POINT('Ctrl Pts',(17.2148149949261,-69.3819158266955,
12.));
#128467=CARTESIAN_POINT('Ctrl Pts',(17.2167679576991,-69.359001631272,0.));
#128468=CARTESIAN_POINT('Ctrl Pts',(17.2167679576991,-69.359001631272,12.));
#128469=CARTESIAN_POINT('Ctrl Pts',(17.2186942815603,-69.3361301352149,
0.));
#128470=CARTESIAN_POINT('Ctrl Pts',(17.2186942815603,-69.3361301352149,
12.));
#128471=CARTESIAN_POINT('Ctrl Pts',(17.2205940220455,-69.3133014770542,
0.));
#128472=CARTESIAN_POINT('Ctrl Pts',(17.2205940220455,-69.3133014770542,
12.));
#128473=CARTESIAN_POINT('Ctrl Pts',(17.2224672350432,-69.2905157959141,
0.));
#128474=CARTESIAN_POINT('Ctrl Pts',(17.2224672350432,-69.2905157959141,
12.));
#128475=CARTESIAN_POINT('Ctrl Pts',(17.2243139767963,-69.2677732315199,
0.));
#128476=CARTESIAN_POINT('Ctrl Pts',(17.2243139767963,-69.2677732315199,
12.));
#128477=CARTESIAN_POINT('Ctrl Pts',(17.2261343039015,-69.2450739242092,
0.));
#128478=CARTESIAN_POINT('Ctrl Pts',(17.2261343039015,-69.2450739242092,
12.));
#128479=CARTESIAN_POINT('Ctrl Pts',(17.2279282733119,-69.2224180149377,
0.));
#128480=CARTESIAN_POINT('Ctrl Pts',(17.2279282733119,-69.2224180149377,
12.));
#128481=CARTESIAN_POINT('Ctrl Pts',(17.229695942341,-69.1998056452837,0.));
#128482=CARTESIAN_POINT('Ctrl Pts',(17.229695942341,-69.1998056452837,12.));
#128483=CARTESIAN_POINT('Ctrl Pts',(17.2314373686705,-69.1772369574462,
0.));
#128484=CARTESIAN_POINT('Ctrl Pts',(17.2314373686705,-69.1772369574462,
12.));
#128485=CARTESIAN_POINT('Ctrl Pts',(17.2331526103511,-69.1547120942542,
0.));
#128486=CARTESIAN_POINT('Ctrl Pts',(17.2331526103511,-69.1547120942542,
12.));
#128487=CARTESIAN_POINT('Ctrl Pts',(17.2348417258017,-69.1322311991759,
0.));
#128488=CARTESIAN_POINT('Ctrl Pts',(17.2348417258017,-69.1322311991759,
12.));
#128489=CARTESIAN_POINT('Ctrl Pts',(17.2365047738125,-69.1097944163244,
0.));
#128490=CARTESIAN_POINT('Ctrl Pts',(17.2365047738125,-69.1097944163244,
12.));
#128491=CARTESIAN_POINT('Ctrl Pts',(17.2381418135489,-69.0874018904598,
0.));
#128492=CARTESIAN_POINT('Ctrl Pts',(17.2381418135489,-69.0874018904598,
12.));
#128493=CARTESIAN_POINT('Ctrl Pts',(17.2397529045587,-69.0650537669859,
0.));
#128494=CARTESIAN_POINT('Ctrl Pts',(17.2397529045587,-69.0650537669859,
12.));
#128495=CARTESIAN_POINT('Ctrl Pts',(17.2413381067722,-69.0427501919636,
0.));
#128496=CARTESIAN_POINT('Ctrl Pts',(17.2413381067722,-69.0427501919636,
12.));
#128497=CARTESIAN_POINT('Ctrl Pts',(17.2428974805043,-69.0204913121226,
0.));
#128498=CARTESIAN_POINT('Ctrl Pts',(17.2428974805043,-69.0204913121226,
12.));
#128499=CARTESIAN_POINT('Ctrl Pts',(17.2444310864585,-68.9982772748694,
0.));
#128500=CARTESIAN_POINT('Ctrl Pts',(17.2444310864585,-68.9982772748694,
12.));
#128501=CARTESIAN_POINT('Ctrl Pts',(17.2459389857327,-68.9761082282922,
0.));
#128502=CARTESIAN_POINT('Ctrl Pts',(17.2459389857327,-68.9761082282922,
12.));
#128503=CARTESIAN_POINT('Ctrl Pts',(17.2474212398275,-68.9539843211618,
0.));
#128504=CARTESIAN_POINT('Ctrl Pts',(17.2474212398275,-68.9539843211618,
12.));
#128505=CARTESIAN_POINT('Ctrl Pts',(17.248877910643,-68.9319057029407,0.));
#128506=CARTESIAN_POINT('Ctrl Pts',(17.248877910643,-68.9319057029407,12.));
#128507=CARTESIAN_POINT('Ctrl Pts',(17.2503090604792,-68.9098725237868,
0.));
#128508=CARTESIAN_POINT('Ctrl Pts',(17.2503090604792,-68.9098725237868,
12.));
#128509=CARTESIAN_POINT('Ctrl Pts',(17.2517147520376,-68.8878849345557,
0.));
#128510=CARTESIAN_POINT('Ctrl Pts',(17.2517147520376,-68.8878849345557,
12.));
#128511=CARTESIAN_POINT('Ctrl Pts',(17.2530950484259,-68.8659430867977,
0.));
#128512=CARTESIAN_POINT('Ctrl Pts',(17.2530950484259,-68.8659430867977,
12.));
#128513=CARTESIAN_POINT('Ctrl Pts',(17.2544500131627,-68.8440471327563,
0.));
#128514=CARTESIAN_POINT('Ctrl Pts',(17.2544500131627,-68.8440471327563,
12.));
#128515=CARTESIAN_POINT('Ctrl Pts',(17.2557797101815,-68.8221972253954,
0.));
#128516=CARTESIAN_POINT('Ctrl Pts',(17.2557797101815,-68.8221972253954,
12.));
#128517=CARTESIAN_POINT('Ctrl Pts',(17.2570842038385,-68.8003935184193,
0.));
#128518=CARTESIAN_POINT('Ctrl Pts',(17.2570842038385,-68.8003935184193,
12.));
#128519=CARTESIAN_POINT('Ctrl Pts',(17.2583635589196,-68.7786361662876,
0.));
#128520=CARTESIAN_POINT('Ctrl Pts',(17.2583635589196,-68.7786361662876,
12.));
#128521=CARTESIAN_POINT('Ctrl Pts',(17.2596178406545,-68.7569253242312,
0.));
#128522=CARTESIAN_POINT('Ctrl Pts',(17.2596178406545,-68.7569253242312,
12.));
#128523=CARTESIAN_POINT('Ctrl Pts',(17.2608471147178,-68.7352611482519,
0.));
#128524=CARTESIAN_POINT('Ctrl Pts',(17.2608471147178,-68.7352611482519,
12.));
#128525=CARTESIAN_POINT('Ctrl Pts',(17.2620514472176,-68.7136437951074,
0.));
#128526=CARTESIAN_POINT('Ctrl Pts',(17.2620514472176,-68.7136437951074,
12.));
#128527=CARTESIAN_POINT('Ctrl Pts',(17.263230904689,-68.6920734222932,0.));
#128528=CARTESIAN_POINT('Ctrl Pts',(17.263230904689,-68.6920734222932,12.));
#128529=CARTESIAN_POINT('Ctrl Pts',(17.2643855540895,-68.6705501880263,
0.));
#128530=CARTESIAN_POINT('Ctrl Pts',(17.2643855540895,-68.6705501880263,
12.));
#128531=CARTESIAN_POINT('Ctrl Pts',(17.2655154627935,-68.6490742512085,
0.));
#128532=CARTESIAN_POINT('Ctrl Pts',(17.2655154627935,-68.6490742512085,
12.));
#128533=CARTESIAN_POINT('Ctrl Pts',(17.266620698609,-68.6276457714757,0.));
#128534=CARTESIAN_POINT('Ctrl Pts',(17.266620698609,-68.6276457714757,12.));
#128535=CARTESIAN_POINT('Ctrl Pts',(17.2677013298061,-68.606264909278,0.));
#128536=CARTESIAN_POINT('Ctrl Pts',(17.2677013298061,-68.606264909278,12.));
#128537=CARTESIAN_POINT('Ctrl Pts',(17.2687574251428,-68.5849318259449,
0.));
#128538=CARTESIAN_POINT('Ctrl Pts',(17.2687574251428,-68.5849318259449,
12.));
#128539=CARTESIAN_POINT('Ctrl Pts',(17.2697890538956,-68.5636466837502,
0.));
#128540=CARTESIAN_POINT('Ctrl Pts',(17.2697890538956,-68.5636466837502,
12.));
#128541=CARTESIAN_POINT('Ctrl Pts',(17.2707962858912,-68.5424096459746,
0.));
#128542=CARTESIAN_POINT('Ctrl Pts',(17.2707962858912,-68.5424096459746,
12.));
#128543=CARTESIAN_POINT('Ctrl Pts',(17.2717791914537,-68.5212208767835,
0.));
#128544=CARTESIAN_POINT('Ctrl Pts',(17.2717791914537,-68.5212208767835,
12.));
#128545=CARTESIAN_POINT('Ctrl Pts',(17.2727378413485,-68.5000805410896,
0.));
#128546=CARTESIAN_POINT('Ctrl Pts',(17.2727378413485,-68.5000805410896,
12.));
#128547=CARTESIAN_POINT('Ctrl Pts',(17.2736723067366,-68.4789888044357,
0.));
#128548=CARTESIAN_POINT('Ctrl Pts',(17.2736723067366,-68.4789888044357,
12.));
#128549=CARTESIAN_POINT('Ctrl Pts',(17.2745826591125,-68.4579458328208,
0.));
#128550=CARTESIAN_POINT('Ctrl Pts',(17.2745826591125,-68.4579458328208,
12.));
#128551=CARTESIAN_POINT('Ctrl Pts',(17.2754689703001,-68.4369517926803,
0.));
#128552=CARTESIAN_POINT('Ctrl Pts',(17.2754689703001,-68.4369517926803,
12.));
#128553=CARTESIAN_POINT('Ctrl Pts',(17.2763313126025,-68.4160068512781,
0.));
#128554=CARTESIAN_POINT('Ctrl Pts',(17.2763313126025,-68.4160068512781,
12.));
#128555=CARTESIAN_POINT('Ctrl Pts',(17.2771697589387,-68.3951111770498,
0.));
#128556=CARTESIAN_POINT('Ctrl Pts',(17.2771697589387,-68.3951111770498,
12.));
#128557=CARTESIAN_POINT('Ctrl Pts',(17.2779843829605,-68.374264939895,0.));
#128558=CARTESIAN_POINT('Ctrl Pts',(17.2779843829605,-68.374264939895,12.));
#128559=CARTESIAN_POINT('Ctrl Pts',(17.2787752592475,-68.353468311648,0.));
#128560=CARTESIAN_POINT('Ctrl Pts',(17.2787752592475,-68.353468311648,12.));
#128561=CARTESIAN_POINT('Ctrl Pts',(17.2795424631789,-68.3327214657533,
0.));
#128562=CARTESIAN_POINT('Ctrl Pts',(17.2795424631789,-68.3327214657533,
12.));
#128563=CARTESIAN_POINT('Ctrl Pts',(17.2802860705807,-68.3120245763884,
0.));
#128564=CARTESIAN_POINT('Ctrl Pts',(17.2802860705807,-68.3120245763884,
12.));
#128565=CARTESIAN_POINT('Ctrl Pts',(17.2810061574352,-68.2913778177258,
0.));
#128566=CARTESIAN_POINT('Ctrl Pts',(17.2810061574352,-68.2913778177258,
12.));
#128567=CARTESIAN_POINT('Ctrl Pts',(17.2817027995838,-68.2707813631761,
0.));
#128568=CARTESIAN_POINT('Ctrl Pts',(17.2817027995838,-68.2707813631761,
12.));
#128569=CARTESIAN_POINT('Ctrl Pts',(17.2823760723886,-68.250235384512,0.));
#128570=CARTESIAN_POINT('Ctrl Pts',(17.2823760723886,-68.250235384512,12.));
#128571=CARTESIAN_POINT('Ctrl Pts',(17.2830260513878,-68.2297400535339,
0.));
#128572=CARTESIAN_POINT('Ctrl Pts',(17.2830260513878,-68.2297400535339,
12.));
#128573=CARTESIAN_POINT('Ctrl Pts',(17.2836528130825,-68.2092955440591,
0.));
#128574=CARTESIAN_POINT('Ctrl Pts',(17.2836528130825,-68.2092955440591,
12.));
#128575=CARTESIAN_POINT('Ctrl Pts',(17.2842564355796,-68.1889020335418,
0.));
#128576=CARTESIAN_POINT('Ctrl Pts',(17.2842564355796,-68.1889020335418,
12.));
#128577=CARTESIAN_POINT('Ctrl Pts',(17.2848369995283,-68.1685597054193,
0.));
#128578=CARTESIAN_POINT('Ctrl Pts',(17.2848369995283,-68.1685597054193,
12.));
#128579=CARTESIAN_POINT('Ctrl Pts',(17.2853945882059,-68.1482687493176,
0.));
#128580=CARTESIAN_POINT('Ctrl Pts',(17.2853945882059,-68.1482687493176,
12.));
#128581=CARTESIAN_POINT('Ctrl Pts',(17.2859292855694,-68.1280293561473,
0.));
#128582=CARTESIAN_POINT('Ctrl Pts',(17.2859292855694,-68.1280293561473,
12.));
#128583=CARTESIAN_POINT('Ctrl Pts',(17.2864411745455,-68.1078417137865,
0.));
#128584=CARTESIAN_POINT('Ctrl Pts',(17.2864411745455,-68.1078417137865,
12.));
#128585=CARTESIAN_POINT('Ctrl Pts',(17.2869303355438,-68.0877060033229,
0.));
#128586=CARTESIAN_POINT('Ctrl Pts',(17.2869303355438,-68.0877060033229,
12.));
#128587=CARTESIAN_POINT('Ctrl Pts',(17.2873968440855,-68.0676223930469,
0.));
#128588=CARTESIAN_POINT('Ctrl Pts',(17.2873968440855,-68.0676223930469,
12.));
#128589=CARTESIAN_POINT('Ctrl Pts',(17.2878407730981,-68.0475910442494,
0.));
#128590=CARTESIAN_POINT('Ctrl Pts',(17.2878407730981,-68.0475910442494,
12.));
#128591=CARTESIAN_POINT('Ctrl Pts',(17.2882621974737,-68.027612122741,0.));
#128592=CARTESIAN_POINT('Ctrl Pts',(17.2882621974737,-68.027612122741,12.));
#128593=CARTESIAN_POINT('Ctrl Pts',(17.28866119774,-68.007685808115,0.));
#128594=CARTESIAN_POINT('Ctrl Pts',(17.28866119774,-68.007685808115,12.));
#128595=CARTESIAN_POINT('Ctrl Pts',(17.2890378644843,-67.9878123049132,
0.));
#128596=CARTESIAN_POINT('Ctrl Pts',(17.2890378644843,-67.9878123049132,
12.));
#128597=CARTESIAN_POINT('Ctrl Pts',(17.2893923013852,-67.9679918502441,
0.));
#128598=CARTESIAN_POINT('Ctrl Pts',(17.2893923013852,-67.9679918502441,
12.));
#128599=CARTESIAN_POINT('Ctrl Pts',(17.2897246158895,-67.9482246901517,
0.));
#128600=CARTESIAN_POINT('Ctrl Pts',(17.2897246158895,-67.9482246901517,
12.));
#128601=CARTESIAN_POINT('Ctrl Pts',(17.2900349103956,-67.9285110571662,
0.));
#128602=CARTESIAN_POINT('Ctrl Pts',(17.2900349103956,-67.9285110571662,
12.));
#128603=CARTESIAN_POINT('Ctrl Pts',(17.2903232740717,-67.908851149676,0.));
#128604=CARTESIAN_POINT('Ctrl Pts',(17.2903232740717,-67.908851149676,12.));
#128605=CARTESIAN_POINT('Ctrl Pts',(17.2905897724029,-67.8892451049871,
0.));
#128606=CARTESIAN_POINT('Ctrl Pts',(17.2905897724029,-67.8892451049871,
12.));
#128607=CARTESIAN_POINT('Ctrl Pts',(17.2908344459816,-67.8696929979178,
0.));
#128608=CARTESIAN_POINT('Ctrl Pts',(17.2908344459816,-67.8696929979178,
12.));
#128609=CARTESIAN_POINT('Ctrl Pts',(17.2910127431203,-67.8540944890057,
0.));
#128610=CARTESIAN_POINT('Ctrl Pts',(17.2910127431203,-67.8540944890057,
12.));
#128611=CARTESIAN_POINT('Ctrl Pts',(17.2911366591419,-67.8424198971214,
0.));
#128612=CARTESIAN_POINT('Ctrl Pts',(17.2911366591419,-67.8424198971214,
12.));
#128613=CARTESIAN_POINT('Ctrl Pts',(17.2912149114145,-67.8346476309106,
0.));
#128614=CARTESIAN_POINT('Ctrl Pts',(17.2912149114145,-67.8346476309106,
12.));
#128615=CARTESIAN_POINT('Ctrl Pts',(17.2912529479484,-67.8307641965655,
0.));
#128616=CARTESIAN_POINT('Ctrl Pts',(17.2912529479484,-67.8307641965655,
12.));
#128617=CARTESIAN_POINT('',(17.2912529479484,-67.8307641965655,12.));
#128618=CARTESIAN_POINT('Ctrl Pts',(17.2912529479484,-67.8307641965655,
12.));
#128619=CARTESIAN_POINT('Ctrl Pts',(17.2912149114145,-67.8346476309106,
12.));
#128620=CARTESIAN_POINT('Ctrl Pts',(17.2911366591419,-67.8424198971214,
12.));
#128621=CARTESIAN_POINT('Ctrl Pts',(17.2910127431203,-67.8540944890057,
12.));
#128622=CARTESIAN_POINT('Ctrl Pts',(17.2908344459816,-67.8696929979178,
12.));
#128623=CARTESIAN_POINT('Ctrl Pts',(17.2905897724029,-67.8892451049871,
12.));
#128624=CARTESIAN_POINT('Ctrl Pts',(17.2903232740717,-67.908851149676,12.));
#128625=CARTESIAN_POINT('Ctrl Pts',(17.2900349103956,-67.9285110571662,
12.));
#128626=CARTESIAN_POINT('Ctrl Pts',(17.2897246158895,-67.9482246901517,
12.));
#128627=CARTESIAN_POINT('Ctrl Pts',(17.2893923013852,-67.9679918502441,
12.));
#128628=CARTESIAN_POINT('Ctrl Pts',(17.2890378644843,-67.9878123049132,
12.));
#128629=CARTESIAN_POINT('Ctrl Pts',(17.28866119774,-68.007685808115,12.));
#128630=CARTESIAN_POINT('Ctrl Pts',(17.2882621974737,-68.027612122741,12.));
#128631=CARTESIAN_POINT('Ctrl Pts',(17.2878407730981,-68.0475910442494,
12.));
#128632=CARTESIAN_POINT('Ctrl Pts',(17.2873968440855,-68.0676223930469,
12.));
#128633=CARTESIAN_POINT('Ctrl Pts',(17.2869303355438,-68.0877060033229,
12.));
#128634=CARTESIAN_POINT('Ctrl Pts',(17.2864411745455,-68.1078417137865,
12.));
#128635=CARTESIAN_POINT('Ctrl Pts',(17.2859292855694,-68.1280293561473,
12.));
#128636=CARTESIAN_POINT('Ctrl Pts',(17.2853945882059,-68.1482687493176,
12.));
#128637=CARTESIAN_POINT('Ctrl Pts',(17.2848369995283,-68.1685597054193,
12.));
#128638=CARTESIAN_POINT('Ctrl Pts',(17.2842564355796,-68.1889020335418,
12.));
#128639=CARTESIAN_POINT('Ctrl Pts',(17.2836528130825,-68.2092955440591,
12.));
#128640=CARTESIAN_POINT('Ctrl Pts',(17.2830260513878,-68.2297400535339,
12.));
#128641=CARTESIAN_POINT('Ctrl Pts',(17.2823760723886,-68.250235384512,12.));
#128642=CARTESIAN_POINT('Ctrl Pts',(17.2817027995838,-68.2707813631761,
12.));
#128643=CARTESIAN_POINT('Ctrl Pts',(17.2810061574352,-68.2913778177258,
12.));
#128644=CARTESIAN_POINT('Ctrl Pts',(17.2802860705807,-68.3120245763884,
12.));
#128645=CARTESIAN_POINT('Ctrl Pts',(17.2795424631789,-68.3327214657533,
12.));
#128646=CARTESIAN_POINT('Ctrl Pts',(17.2787752592475,-68.353468311648,12.));
#128647=CARTESIAN_POINT('Ctrl Pts',(17.2779843829605,-68.374264939895,12.));
#128648=CARTESIAN_POINT('Ctrl Pts',(17.2771697589387,-68.3951111770498,
12.));
#128649=CARTESIAN_POINT('Ctrl Pts',(17.2763313126025,-68.4160068512781,
12.));
#128650=CARTESIAN_POINT('Ctrl Pts',(17.2754689703001,-68.4369517926803,
12.));
#128651=CARTESIAN_POINT('Ctrl Pts',(17.2745826591125,-68.4579458328208,
12.));
#128652=CARTESIAN_POINT('Ctrl Pts',(17.2736723067366,-68.4789888044357,
12.));
#128653=CARTESIAN_POINT('Ctrl Pts',(17.2727378413485,-68.5000805410896,
12.));
#128654=CARTESIAN_POINT('Ctrl Pts',(17.2717791914537,-68.5212208767835,
12.));
#128655=CARTESIAN_POINT('Ctrl Pts',(17.2707962858912,-68.5424096459746,
12.));
#128656=CARTESIAN_POINT('Ctrl Pts',(17.2697890538956,-68.5636466837502,
12.));
#128657=CARTESIAN_POINT('Ctrl Pts',(17.2687574251428,-68.5849318259449,
12.));
#128658=CARTESIAN_POINT('Ctrl Pts',(17.2677013298061,-68.606264909278,12.));
#128659=CARTESIAN_POINT('Ctrl Pts',(17.266620698609,-68.6276457714757,12.));
#128660=CARTESIAN_POINT('Ctrl Pts',(17.2655154627935,-68.6490742512085,
12.));
#128661=CARTESIAN_POINT('Ctrl Pts',(17.2643855540895,-68.6705501880263,
12.));
#128662=CARTESIAN_POINT('Ctrl Pts',(17.263230904689,-68.6920734222932,12.));
#128663=CARTESIAN_POINT('Ctrl Pts',(17.2620514472176,-68.7136437951074,
12.));
#128664=CARTESIAN_POINT('Ctrl Pts',(17.2608471147178,-68.7352611482519,
12.));
#128665=CARTESIAN_POINT('Ctrl Pts',(17.2596178406545,-68.7569253242312,
12.));
#128666=CARTESIAN_POINT('Ctrl Pts',(17.2583635589196,-68.7786361662876,
12.));
#128667=CARTESIAN_POINT('Ctrl Pts',(17.2570842038385,-68.8003935184193,
12.));
#128668=CARTESIAN_POINT('Ctrl Pts',(17.2557797101815,-68.8221972253954,
12.));
#128669=CARTESIAN_POINT('Ctrl Pts',(17.2544500131627,-68.8440471327563,
12.));
#128670=CARTESIAN_POINT('Ctrl Pts',(17.2530950484259,-68.8659430867977,
12.));
#128671=CARTESIAN_POINT('Ctrl Pts',(17.2517147520376,-68.8878849345557,
12.));
#128672=CARTESIAN_POINT('Ctrl Pts',(17.2503090604792,-68.9098725237868,
12.));
#128673=CARTESIAN_POINT('Ctrl Pts',(17.248877910643,-68.9319057029407,12.));
#128674=CARTESIAN_POINT('Ctrl Pts',(17.2474212398275,-68.9539843211618,
12.));
#128675=CARTESIAN_POINT('Ctrl Pts',(17.2459389857327,-68.9761082282922,
12.));
#128676=CARTESIAN_POINT('Ctrl Pts',(17.2444310864585,-68.9982772748694,
12.));
#128677=CARTESIAN_POINT('Ctrl Pts',(17.2428974805043,-69.0204913121226,
12.));
#128678=CARTESIAN_POINT('Ctrl Pts',(17.2413381067722,-69.0427501919636,
12.));
#128679=CARTESIAN_POINT('Ctrl Pts',(17.2397529045587,-69.0650537669859,
12.));
#128680=CARTESIAN_POINT('Ctrl Pts',(17.2381418135489,-69.0874018904598,
12.));
#128681=CARTESIAN_POINT('Ctrl Pts',(17.2365047738125,-69.1097944163244,
12.));
#128682=CARTESIAN_POINT('Ctrl Pts',(17.2348417258017,-69.1322311991759,
12.));
#128683=CARTESIAN_POINT('Ctrl Pts',(17.2331526103511,-69.1547120942542,
12.));
#128684=CARTESIAN_POINT('Ctrl Pts',(17.2314373686705,-69.1772369574462,
12.));
#128685=CARTESIAN_POINT('Ctrl Pts',(17.229695942341,-69.1998056452837,12.));
#128686=CARTESIAN_POINT('Ctrl Pts',(17.2279282733119,-69.2224180149377,
12.));
#128687=CARTESIAN_POINT('Ctrl Pts',(17.2261343039015,-69.2450739242092,
12.));
#128688=CARTESIAN_POINT('Ctrl Pts',(17.2243139767963,-69.2677732315199,
12.));
#128689=CARTESIAN_POINT('Ctrl Pts',(17.2224672350432,-69.2905157959141,
12.));
#128690=CARTESIAN_POINT('Ctrl Pts',(17.2205940220455,-69.3133014770542,
12.));
#128691=CARTESIAN_POINT('Ctrl Pts',(17.2186942815603,-69.3361301352149,
12.));
#128692=CARTESIAN_POINT('Ctrl Pts',(17.2167679576991,-69.359001631272,12.));
#128693=CARTESIAN_POINT('Ctrl Pts',(17.2148149949261,-69.3819158266955,
12.));
#128694=CARTESIAN_POINT('Ctrl Pts',(17.2128353380511,-69.4048725835516,
12.));
#128695=CARTESIAN_POINT('Ctrl Pts',(17.2108289322258,-69.4278717644989,
12.));
#128696=CARTESIAN_POINT('Ctrl Pts',(17.208795722942,-69.4509132327836,12.));
#128697=CARTESIAN_POINT('Ctrl Pts',(17.2067356560326,-69.4739968522271,
12.));
#128698=CARTESIAN_POINT('Ctrl Pts',(17.2046486776697,-69.497122487222,12.));
#128699=CARTESIAN_POINT('Ctrl Pts',(17.2025347343568,-69.5202900027329,
12.));
#128700=CARTESIAN_POINT('Ctrl Pts',(17.2003937729266,-69.5434992642932,
12.));
#128701=CARTESIAN_POINT('Ctrl Pts',(17.198225740538,-69.5667501379984,12.));
#128702=CARTESIAN_POINT('Ctrl Pts',(17.1960305846787,-69.5900424904954,
12.));
#128703=CARTESIAN_POINT('Ctrl Pts',(17.1938082531619,-69.6133761889787,
12.));
#128704=CARTESIAN_POINT('Ctrl Pts',(17.1915586941198,-69.6367511011927,
12.));
#128705=CARTESIAN_POINT('Ctrl Pts',(17.1892818560004,-69.6601670954277,
12.));
#128706=CARTESIAN_POINT('Ctrl Pts',(17.1869776875663,-69.6836240405151,
12.));
#128707=CARTESIAN_POINT('Ctrl Pts',(17.1846461378966,-69.7071218058149,
12.));
#128708=CARTESIAN_POINT('Ctrl Pts',(17.1822871563834,-69.7306602612125,
12.));
#128709=CARTESIAN_POINT('Ctrl Pts',(17.1799006927255,-69.7542392771216,
12.));
#128710=CARTESIAN_POINT('Ctrl Pts',(17.1774866969255,-69.7778587244788,
12.));
#128711=CARTESIAN_POINT('Ctrl Pts',(17.1750451192887,-69.8015184747404,
12.));
#128712=CARTESIAN_POINT('Ctrl Pts',(17.1725759104254,-69.8252183998713,
12.));
#128713=CARTESIAN_POINT('Ctrl Pts',(17.1700790212476,-69.8489583723417,
12.));
#128714=CARTESIAN_POINT('Ctrl Pts',(17.1675544029621,-69.8727382651292,
12.));
#128715=CARTESIAN_POINT('Ctrl Pts',(17.1650020070686,-69.8965579517147,
12.));
#128716=CARTESIAN_POINT('Ctrl Pts',(17.1624217853577,-69.9204173060779,
12.));
#128717=CARTESIAN_POINT('Ctrl Pts',(17.1598136899144,-69.9443162026865,
12.));
#128718=CARTESIAN_POINT('Ctrl Pts',(17.157177673114,-69.9682545164942,12.));
#128719=CARTESIAN_POINT('Ctrl Pts',(17.1545136876161,-69.9922321229428,
12.));
#128720=CARTESIAN_POINT('Ctrl Pts',(17.1518216863624,-70.0162488979586,
12.));
#128721=CARTESIAN_POINT('Ctrl Pts',(17.1491016225748,-70.040304717948,12.));
#128722=CARTESIAN_POINT('Ctrl Pts',(17.1463534497592,-70.0643994597865,
12.));
#128723=CARTESIAN_POINT('Ctrl Pts',(17.1435771217015,-70.0885330008169,
12.));
#128724=CARTESIAN_POINT('Ctrl Pts',(17.1407725924615,-70.1127052188515,
12.));
#128725=CARTESIAN_POINT('Ctrl Pts',(17.1379398163708,-70.1369159921686,
12.));
#128726=CARTESIAN_POINT('Ctrl Pts',(17.1350787480313,-70.1611651995085,
12.));
#128727=CARTESIAN_POINT('Ctrl Pts',(17.1321893423183,-70.1854527200636,
12.));
#128728=CARTESIAN_POINT('Ctrl Pts',(17.1292715543779,-70.2097784334749,
12.));
#128729=CARTESIAN_POINT('Ctrl Pts',(17.1263253396202,-70.2341422198362,
12.));
#128730=CARTESIAN_POINT('Ctrl Pts',(17.1233506537176,-70.2585439596899,
12.));
#128731=CARTESIAN_POINT('Ctrl Pts',(17.1203474526031,-70.2829835340239,
12.));
#128732=CARTESIAN_POINT('Ctrl Pts',(17.1173156924733,-70.3074608242613,
12.));
#128733=CARTESIAN_POINT('Ctrl Pts',(17.1142553297869,-70.3319757122576,
12.));
#128734=CARTESIAN_POINT('Ctrl Pts',(17.111166321257,-70.356528080303,12.));
#128735=CARTESIAN_POINT('Ctrl Pts',(17.1080486238499,-70.3811178111206,
12.));
#128736=CARTESIAN_POINT('Ctrl Pts',(17.1049021947833,-70.4057447878621,
12.));
#128737=CARTESIAN_POINT('Ctrl Pts',(17.1017269915289,-70.4304088940998,
12.));
#128738=CARTESIAN_POINT('Ctrl Pts',(17.098522971812,-70.4551100138221,12.));
#128739=CARTESIAN_POINT('Ctrl Pts',(17.0952900936044,-70.4798480314364,
12.));
#128740=CARTESIAN_POINT('Ctrl Pts',(17.0920283151217,-70.5046228317669,
12.));
#128741=CARTESIAN_POINT('Ctrl Pts',(17.0887375948221,-70.5294343000516,
12.));
#128742=CARTESIAN_POINT('Ctrl Pts',(17.085417891409,-70.5542823219346,12.));
#128743=CARTESIAN_POINT('Ctrl Pts',(17.0820691638314,-70.5791667834599,
12.));
#128744=CARTESIAN_POINT('Ctrl Pts',(17.0786913712766,-70.6040875710762,
12.));
#128745=CARTESIAN_POINT('Ctrl Pts',(17.0752844731679,-70.6290445716341,
12.));
#128746=CARTESIAN_POINT('Ctrl Pts',(17.0718484291623,-70.6540376723839,
12.));
#128747=CARTESIAN_POINT('Ctrl Pts',(17.0683831991532,-70.6790667609678,
12.));
#128748=CARTESIAN_POINT('Ctrl Pts',(17.0648887432714,-70.7041317254127,
12.));
#128749=CARTESIAN_POINT('Ctrl Pts',(17.0613650218788,-70.7292324541348,
12.));
#128750=CARTESIAN_POINT('Ctrl Pts',(17.0578119955651,-70.754368835938,12.));
#128751=CARTESIAN_POINT('Ctrl Pts',(17.0542296251462,-70.7795407600127,
12.));
#128752=CARTESIAN_POINT('Ctrl Pts',(17.0506178716661,-70.8047481159298,
12.));
#128753=CARTESIAN_POINT('Ctrl Pts',(17.0469766964001,-70.8299907936334,
12.));
#128754=CARTESIAN_POINT('Ctrl Pts',(17.0433060608474,-70.8552686834423,
12.));
#128755=CARTESIAN_POINT('Ctrl Pts',(17.0396059267277,-70.8805816760501,
12.));
#128756=CARTESIAN_POINT('Ctrl Pts',(17.0358762559786,-70.9059296625214,
12.));
#128757=CARTESIAN_POINT('Ctrl Pts',(17.0321170107564,-70.9313125342876,
12.));
#128758=CARTESIAN_POINT('Ctrl Pts',(17.0283281534392,-70.956730183136,12.));
#128759=CARTESIAN_POINT('Ctrl Pts',(17.0245096466229,-70.9821825012136,
12.));
#128760=CARTESIAN_POINT('Ctrl Pts',(17.0206614531166,-71.0076693810301,
12.));
#128761=CARTESIAN_POINT('Ctrl Pts',(17.0167835359419,-71.0331907154574,
12.));
#128762=CARTESIAN_POINT('Ctrl Pts',(17.0128758583334,-71.0587463977268,
12.));
#128763=CARTESIAN_POINT('Ctrl Pts',(17.0089383837437,-71.0843363214221,
12.));
#128764=CARTESIAN_POINT('Ctrl Pts',(17.0049710758393,-71.1099603804786,
12.));
#128765=CARTESIAN_POINT('Ctrl Pts',(17.0009738984935,-71.1356184691806,
12.));
#128766=CARTESIAN_POINT('Ctrl Pts',(16.9969468157824,-71.1613104821568,
12.));
#128767=CARTESIAN_POINT('Ctrl Pts',(16.9928897919828,-71.187036314374,12.));
#128768=CARTESIAN_POINT('Ctrl Pts',(16.9888027915742,-71.212795861124,12.));
#128769=CARTESIAN_POINT('Ctrl Pts',(16.9846857792383,-71.2385890180221,
12.));
#128770=CARTESIAN_POINT('Ctrl Pts',(16.9805387198571,-71.2644156810198,
12.));
#128771=CARTESIAN_POINT('Ctrl Pts',(16.9763615785136,-71.290275746412,12.));
#128772=CARTESIAN_POINT('Ctrl Pts',(16.9721543204951,-71.3161691108427,
12.));
#128773=CARTESIAN_POINT('Ctrl Pts',(16.9679169112994,-71.3420956713082,
12.));
#128774=CARTESIAN_POINT('Ctrl Pts',(16.9636493166397,-71.3680553251562,
12.));
#128775=CARTESIAN_POINT('Ctrl Pts',(16.9593515024276,-71.3940479700677,
12.));
#128776=CARTESIAN_POINT('Ctrl Pts',(16.955023434762,-71.4200735040384,12.));
#128777=CARTESIAN_POINT('Ctrl Pts',(16.9506650799188,-71.4461318253563,
12.));
#128778=CARTESIAN_POINT('Ctrl Pts',(16.9462764043443,-71.4722228325794,
12.));
#128779=CARTESIAN_POINT('Ctrl Pts',(16.9418573746488,-71.4983464245055,
12.));
#128780=CARTESIAN_POINT('Ctrl Pts',(16.9374079576201,-71.5245025002139,
12.));
#128781=CARTESIAN_POINT('Ctrl Pts',(16.9329281202377,-71.5506909591128,
12.));
#128782=CARTESIAN_POINT('Ctrl Pts',(16.9284178296933,-71.5769117009842,
12.));
#128783=CARTESIAN_POINT('Ctrl Pts',(16.9238770534071,-71.6031646260174,
12.));
#128784=CARTESIAN_POINT('Ctrl Pts',(16.9193057590607,-71.6294496348652,
12.));
#128785=CARTESIAN_POINT('Ctrl Pts',(16.9147039145717,-71.6557666285917,
12.));
#128786=CARTESIAN_POINT('Ctrl Pts',(16.9100714880368,-71.6821155085612,
12.));
#128787=CARTESIAN_POINT('Ctrl Pts',(16.9054084476847,-71.7084961763357,
12.));
#128788=CARTESIAN_POINT('Ctrl Pts',(16.9007147618344,-71.7349085335796,
12.));
#128789=CARTESIAN_POINT('Ctrl Pts',(16.8959903988409,-71.7613524819235,
12.));
#128790=CARTESIAN_POINT('Ctrl Pts',(16.8912353270942,-71.7878279229546,
12.));
#128791=CARTESIAN_POINT('Ctrl Pts',(16.8864495151344,-71.8143347584962,
12.));
#128792=CARTESIAN_POINT('Ctrl Pts',(16.881632931747,-71.8408728908258,12.));
#128793=CARTESIAN_POINT('Ctrl Pts',(16.87678554607,-71.8674422229149,12.));
#128794=CARTESIAN_POINT('Ctrl Pts',(16.871907327697,-71.8940426586534,12.));
#128795=CARTESIAN_POINT('Ctrl Pts',(16.866998246792,-71.9206741030887,12.));
#128796=CARTESIAN_POINT('Ctrl Pts',(16.8620582738437,-71.9473364618922,
12.));
#128797=CARTESIAN_POINT('Ctrl Pts',(16.8570873794269,-71.9740296408347,
12.));
#128798=CARTESIAN_POINT('Ctrl Pts',(16.8520855339445,-72.0007535452081,
12.));
#128799=CARTESIAN_POINT('Ctrl Pts',(16.8470527074275,-72.0275080793727,
12.));
#128800=CARTESIAN_POINT('Ctrl Pts',(16.8419888691976,-72.0542931459825,
12.));
#128801=CARTESIAN_POINT('Ctrl Pts',(16.8368939881446,-72.0811086466121,
12.));
#128802=CARTESIAN_POINT('Ctrl Pts',(16.8317680333404,-72.1079544831513,
12.));
#128803=CARTESIAN_POINT('Ctrl Pts',(16.8266109745795,-72.13483055902,12.));
#128804=CARTESIAN_POINT('Ctrl Pts',(16.8214227828942,-72.1617367803235,
12.));
#128805=CARTESIAN_POINT('Ctrl Pts',(16.8162034312269,-72.1886730573452,
12.));
#128806=CARTESIAN_POINT('Ctrl Pts',(16.8109528945896,-72.2156393048975,
12.));
#128807=CARTESIAN_POINT('Ctrl Pts',(16.8064254147775,-72.2387802230856,
12.));
#128808=CARTESIAN_POINT('Ctrl Pts',(16.8029374213794,-72.256538003526,12.));
#128809=CARTESIAN_POINT('Ctrl Pts',(16.8005027425862,-72.2688994295264,
12.));
#128810=CARTESIAN_POINT('Ctrl Pts',(16.7991305317749,-72.2758557891329,
12.));
#128811=CARTESIAN_POINT('Ctrl Pts',(16.7988252568748,-72.2774028393915,
12.));
#128812=CARTESIAN_POINT('',(17.2912529479484,-67.8307641965655,0.));
#128813=CARTESIAN_POINT('',(17.2912529479484,-67.8307641965655,0.));
#128814=CARTESIAN_POINT('Ctrl Pts',(16.7988252568748,-72.2774028393915,
0.));
#128815=CARTESIAN_POINT('Ctrl Pts',(16.7991305317749,-72.275855789133,0.));
#128816=CARTESIAN_POINT('Ctrl Pts',(16.8005027425862,-72.2688994295265,
0.));
#128817=CARTESIAN_POINT('Ctrl Pts',(16.8029374213794,-72.2565380035261,
0.));
#128818=CARTESIAN_POINT('Ctrl Pts',(16.8064254147775,-72.2387802230856,
0.));
#128819=CARTESIAN_POINT('Ctrl Pts',(16.8109528945896,-72.2156393048975,
0.));
#128820=CARTESIAN_POINT('Ctrl Pts',(16.8162034312269,-72.1886730573452,
0.));
#128821=CARTESIAN_POINT('Ctrl Pts',(16.8214227828942,-72.1617367803235,
0.));
#128822=CARTESIAN_POINT('Ctrl Pts',(16.8266109745795,-72.13483055902,0.));
#128823=CARTESIAN_POINT('Ctrl Pts',(16.8317680333404,-72.1079544831513,
0.));
#128824=CARTESIAN_POINT('Ctrl Pts',(16.8368939881446,-72.0811086466121,
0.));
#128825=CARTESIAN_POINT('Ctrl Pts',(16.8419888691976,-72.0542931459825,
0.));
#128826=CARTESIAN_POINT('Ctrl Pts',(16.8470527074275,-72.0275080793727,
0.));
#128827=CARTESIAN_POINT('Ctrl Pts',(16.8520855339445,-72.0007535452081,
0.));
#128828=CARTESIAN_POINT('Ctrl Pts',(16.8570873794269,-71.9740296408347,
0.));
#128829=CARTESIAN_POINT('Ctrl Pts',(16.8620582738437,-71.9473364618922,
0.));
#128830=CARTESIAN_POINT('Ctrl Pts',(16.866998246792,-71.9206741030887,0.));
#128831=CARTESIAN_POINT('Ctrl Pts',(16.871907327697,-71.8940426586534,0.));
#128832=CARTESIAN_POINT('Ctrl Pts',(16.87678554607,-71.8674422229149,0.));
#128833=CARTESIAN_POINT('Ctrl Pts',(16.881632931747,-71.8408728908258,0.));
#128834=CARTESIAN_POINT('Ctrl Pts',(16.8864495151344,-71.8143347584962,
0.));
#128835=CARTESIAN_POINT('Ctrl Pts',(16.8912353270942,-71.7878279229546,
0.));
#128836=CARTESIAN_POINT('Ctrl Pts',(16.8959903988409,-71.7613524819235,
0.));
#128837=CARTESIAN_POINT('Ctrl Pts',(16.9007147618344,-71.7349085335796,
0.));
#128838=CARTESIAN_POINT('Ctrl Pts',(16.9054084476847,-71.7084961763357,
0.));
#128839=CARTESIAN_POINT('Ctrl Pts',(16.9100714880368,-71.6821155085612,
0.));
#128840=CARTESIAN_POINT('Ctrl Pts',(16.9147039145717,-71.6557666285917,
0.));
#128841=CARTESIAN_POINT('Ctrl Pts',(16.9193057590607,-71.6294496348652,
0.));
#128842=CARTESIAN_POINT('Ctrl Pts',(16.9238770534071,-71.6031646260174,
0.));
#128843=CARTESIAN_POINT('Ctrl Pts',(16.9284178296933,-71.5769117009842,
0.));
#128844=CARTESIAN_POINT('Ctrl Pts',(16.9329281202377,-71.5506909591128,
0.));
#128845=CARTESIAN_POINT('Ctrl Pts',(16.9374079576201,-71.5245025002139,
0.));
#128846=CARTESIAN_POINT('Ctrl Pts',(16.9418573746488,-71.4983464245055,
0.));
#128847=CARTESIAN_POINT('Ctrl Pts',(16.9462764043443,-71.4722228325794,
0.));
#128848=CARTESIAN_POINT('Ctrl Pts',(16.9506650799188,-71.4461318253563,
0.));
#128849=CARTESIAN_POINT('Ctrl Pts',(16.955023434762,-71.4200735040384,0.));
#128850=CARTESIAN_POINT('Ctrl Pts',(16.9593515024276,-71.3940479700677,
0.));
#128851=CARTESIAN_POINT('Ctrl Pts',(16.9636493166397,-71.3680553251562,
0.));
#128852=CARTESIAN_POINT('Ctrl Pts',(16.9679169112994,-71.3420956713082,
0.));
#128853=CARTESIAN_POINT('Ctrl Pts',(16.9721543204951,-71.3161691108427,
0.));
#128854=CARTESIAN_POINT('Ctrl Pts',(16.9763615785136,-71.290275746412,0.));
#128855=CARTESIAN_POINT('Ctrl Pts',(16.9805387198571,-71.2644156810198,
0.));
#128856=CARTESIAN_POINT('Ctrl Pts',(16.9846857792383,-71.2385890180221,
0.));
#128857=CARTESIAN_POINT('Ctrl Pts',(16.9888027915742,-71.212795861124,0.));
#128858=CARTESIAN_POINT('Ctrl Pts',(16.9928897919828,-71.187036314374,0.));
#128859=CARTESIAN_POINT('Ctrl Pts',(16.9969468157824,-71.1613104821568,
0.));
#128860=CARTESIAN_POINT('Ctrl Pts',(17.0009738984935,-71.1356184691806,
0.));
#128861=CARTESIAN_POINT('Ctrl Pts',(17.0049710758393,-71.1099603804786,
0.));
#128862=CARTESIAN_POINT('Ctrl Pts',(17.0089383837437,-71.0843363214221,
0.));
#128863=CARTESIAN_POINT('Ctrl Pts',(17.0128758583334,-71.0587463977268,
0.));
#128864=CARTESIAN_POINT('Ctrl Pts',(17.0167835359419,-71.0331907154574,
0.));
#128865=CARTESIAN_POINT('Ctrl Pts',(17.0206614531166,-71.0076693810301,
0.));
#128866=CARTESIAN_POINT('Ctrl Pts',(17.0245096466229,-70.9821825012136,
0.));
#128867=CARTESIAN_POINT('Ctrl Pts',(17.0283281534392,-70.956730183136,0.));
#128868=CARTESIAN_POINT('Ctrl Pts',(17.0321170107564,-70.9313125342876,
0.));
#128869=CARTESIAN_POINT('Ctrl Pts',(17.0358762559786,-70.9059296625214,
0.));
#128870=CARTESIAN_POINT('Ctrl Pts',(17.0396059267277,-70.8805816760501,
0.));
#128871=CARTESIAN_POINT('Ctrl Pts',(17.0433060608474,-70.8552686834423,
0.));
#128872=CARTESIAN_POINT('Ctrl Pts',(17.0469766964001,-70.8299907936334,
0.));
#128873=CARTESIAN_POINT('Ctrl Pts',(17.0506178716661,-70.8047481159298,
0.));
#128874=CARTESIAN_POINT('Ctrl Pts',(17.0542296251462,-70.7795407600127,
0.));
#128875=CARTESIAN_POINT('Ctrl Pts',(17.0578119955651,-70.754368835938,0.));
#128876=CARTESIAN_POINT('Ctrl Pts',(17.0613650218788,-70.7292324541348,
0.));
#128877=CARTESIAN_POINT('Ctrl Pts',(17.0648887432714,-70.7041317254127,
0.));
#128878=CARTESIAN_POINT('Ctrl Pts',(17.0683831991532,-70.6790667609678,
0.));
#128879=CARTESIAN_POINT('Ctrl Pts',(17.0718484291623,-70.6540376723839,
0.));
#128880=CARTESIAN_POINT('Ctrl Pts',(17.0752844731679,-70.6290445716341,
0.));
#128881=CARTESIAN_POINT('Ctrl Pts',(17.0786913712766,-70.6040875710762,
0.));
#128882=CARTESIAN_POINT('Ctrl Pts',(17.0820691638314,-70.5791667834599,
0.));
#128883=CARTESIAN_POINT('Ctrl Pts',(17.085417891409,-70.5542823219346,0.));
#128884=CARTESIAN_POINT('Ctrl Pts',(17.0887375948221,-70.5294343000516,
0.));
#128885=CARTESIAN_POINT('Ctrl Pts',(17.0920283151217,-70.5046228317669,
0.));
#128886=CARTESIAN_POINT('Ctrl Pts',(17.0952900936044,-70.4798480314364,
0.));
#128887=CARTESIAN_POINT('Ctrl Pts',(17.098522971812,-70.4551100138221,0.));
#128888=CARTESIAN_POINT('Ctrl Pts',(17.1017269915289,-70.4304088940998,
0.));
#128889=CARTESIAN_POINT('Ctrl Pts',(17.1049021947833,-70.4057447878621,
0.));
#128890=CARTESIAN_POINT('Ctrl Pts',(17.1080486238499,-70.3811178111206,
0.));
#128891=CARTESIAN_POINT('Ctrl Pts',(17.111166321257,-70.356528080303,0.));
#128892=CARTESIAN_POINT('Ctrl Pts',(17.1142553297869,-70.3319757122576,
0.));
#128893=CARTESIAN_POINT('Ctrl Pts',(17.1173156924733,-70.3074608242613,
0.));
#128894=CARTESIAN_POINT('Ctrl Pts',(17.1203474526031,-70.2829835340239,
0.));
#128895=CARTESIAN_POINT('Ctrl Pts',(17.1233506537176,-70.2585439596899,
0.));
#128896=CARTESIAN_POINT('Ctrl Pts',(17.1263253396202,-70.2341422198362,
0.));
#128897=CARTESIAN_POINT('Ctrl Pts',(17.1292715543779,-70.2097784334749,
0.));
#128898=CARTESIAN_POINT('Ctrl Pts',(17.1321893423183,-70.1854527200636,
0.));
#128899=CARTESIAN_POINT('Ctrl Pts',(17.1350787480313,-70.1611651995085,
0.));
#128900=CARTESIAN_POINT('Ctrl Pts',(17.1379398163708,-70.1369159921686,
0.));
#128901=CARTESIAN_POINT('Ctrl Pts',(17.1407725924615,-70.1127052188515,
0.));
#128902=CARTESIAN_POINT('Ctrl Pts',(17.1435771217015,-70.0885330008169,
0.));
#128903=CARTESIAN_POINT('Ctrl Pts',(17.1463534497592,-70.0643994597865,
0.));
#128904=CARTESIAN_POINT('Ctrl Pts',(17.1491016225748,-70.040304717948,0.));
#128905=CARTESIAN_POINT('Ctrl Pts',(17.1518216863624,-70.0162488979586,
0.));
#128906=CARTESIAN_POINT('Ctrl Pts',(17.1545136876161,-69.9922321229428,
0.));
#128907=CARTESIAN_POINT('Ctrl Pts',(17.157177673114,-69.9682545164942,0.));
#128908=CARTESIAN_POINT('Ctrl Pts',(17.1598136899144,-69.9443162026865,
0.));
#128909=CARTESIAN_POINT('Ctrl Pts',(17.1624217853577,-69.9204173060779,
0.));
#128910=CARTESIAN_POINT('Ctrl Pts',(17.1650020070686,-69.8965579517147,
0.));
#128911=CARTESIAN_POINT('Ctrl Pts',(17.1675544029621,-69.8727382651292,
0.));
#128912=CARTESIAN_POINT('Ctrl Pts',(17.1700790212476,-69.8489583723417,
0.));
#128913=CARTESIAN_POINT('Ctrl Pts',(17.1725759104254,-69.8252183998713,
0.));
#128914=CARTESIAN_POINT('Ctrl Pts',(17.1750451192887,-69.8015184747404,
0.));
#128915=CARTESIAN_POINT('Ctrl Pts',(17.1774866969255,-69.7778587244788,
0.));
#128916=CARTESIAN_POINT('Ctrl Pts',(17.1799006927255,-69.7542392771216,
0.));
#128917=CARTESIAN_POINT('Ctrl Pts',(17.1822871563834,-69.7306602612125,
0.));
#128918=CARTESIAN_POINT('Ctrl Pts',(17.1846461378966,-69.7071218058149,
0.));
#128919=CARTESIAN_POINT('Ctrl Pts',(17.1869776875663,-69.6836240405151,
0.));
#128920=CARTESIAN_POINT('Ctrl Pts',(17.1892818560004,-69.6601670954277,
0.));
#128921=CARTESIAN_POINT('Ctrl Pts',(17.1915586941198,-69.6367511011927,
0.));
#128922=CARTESIAN_POINT('Ctrl Pts',(17.1938082531619,-69.6133761889787,
0.));
#128923=CARTESIAN_POINT('Ctrl Pts',(17.1960305846787,-69.5900424904954,
0.));
#128924=CARTESIAN_POINT('Ctrl Pts',(17.198225740538,-69.5667501379984,0.));
#128925=CARTESIAN_POINT('Ctrl Pts',(17.2003937729266,-69.5434992642932,
0.));
#128926=CARTESIAN_POINT('Ctrl Pts',(17.2025347343568,-69.5202900027329,
0.));
#128927=CARTESIAN_POINT('Ctrl Pts',(17.2046486776697,-69.497122487222,0.));
#128928=CARTESIAN_POINT('Ctrl Pts',(17.2067356560326,-69.4739968522271,
0.));
#128929=CARTESIAN_POINT('Ctrl Pts',(17.208795722942,-69.4509132327836,0.));
#128930=CARTESIAN_POINT('Ctrl Pts',(17.2108289322258,-69.4278717644989,
0.));
#128931=CARTESIAN_POINT('Ctrl Pts',(17.2128353380511,-69.4048725835516,
0.));
#128932=CARTESIAN_POINT('Ctrl Pts',(17.2148149949261,-69.3819158266955,
0.));
#128933=CARTESIAN_POINT('Ctrl Pts',(17.2167679576991,-69.359001631272,0.));
#128934=CARTESIAN_POINT('Ctrl Pts',(17.2186942815603,-69.3361301352149,
0.));
#128935=CARTESIAN_POINT('Ctrl Pts',(17.2205940220455,-69.3133014770542,
0.));
#128936=CARTESIAN_POINT('Ctrl Pts',(17.2224672350432,-69.2905157959141,
0.));
#128937=CARTESIAN_POINT('Ctrl Pts',(17.2243139767963,-69.2677732315199,
0.));
#128938=CARTESIAN_POINT('Ctrl Pts',(17.2261343039015,-69.2450739242092,
0.));
#128939=CARTESIAN_POINT('Ctrl Pts',(17.2279282733119,-69.2224180149377,
0.));
#128940=CARTESIAN_POINT('Ctrl Pts',(17.229695942341,-69.1998056452837,0.));
#128941=CARTESIAN_POINT('Ctrl Pts',(17.2314373686705,-69.1772369574462,
0.));
#128942=CARTESIAN_POINT('Ctrl Pts',(17.2331526103511,-69.1547120942542,
0.));
#128943=CARTESIAN_POINT('Ctrl Pts',(17.2348417258017,-69.1322311991759,
0.));
#128944=CARTESIAN_POINT('Ctrl Pts',(17.2365047738125,-69.1097944163244,
0.));
#128945=CARTESIAN_POINT('Ctrl Pts',(17.2381418135489,-69.0874018904598,
0.));
#128946=CARTESIAN_POINT('Ctrl Pts',(17.2397529045587,-69.0650537669859,
0.));
#128947=CARTESIAN_POINT('Ctrl Pts',(17.2413381067722,-69.0427501919636,
0.));
#128948=CARTESIAN_POINT('Ctrl Pts',(17.2428974805043,-69.0204913121226,
0.));
#128949=CARTESIAN_POINT('Ctrl Pts',(17.2444310864585,-68.9982772748694,
0.));
#128950=CARTESIAN_POINT('Ctrl Pts',(17.2459389857327,-68.9761082282922,
0.));
#128951=CARTESIAN_POINT('Ctrl Pts',(17.2474212398275,-68.9539843211618,
0.));
#128952=CARTESIAN_POINT('Ctrl Pts',(17.248877910643,-68.9319057029407,0.));
#128953=CARTESIAN_POINT('Ctrl Pts',(17.2503090604792,-68.9098725237868,
0.));
#128954=CARTESIAN_POINT('Ctrl Pts',(17.2517147520376,-68.8878849345557,
0.));
#128955=CARTESIAN_POINT('Ctrl Pts',(17.2530950484259,-68.8659430867977,
0.));
#128956=CARTESIAN_POINT('Ctrl Pts',(17.2544500131627,-68.8440471327563,
0.));
#128957=CARTESIAN_POINT('Ctrl Pts',(17.2557797101815,-68.8221972253954,
0.));
#128958=CARTESIAN_POINT('Ctrl Pts',(17.2570842038385,-68.8003935184193,
0.));
#128959=CARTESIAN_POINT('Ctrl Pts',(17.2583635589196,-68.7786361662876,
0.));
#128960=CARTESIAN_POINT('Ctrl Pts',(17.2596178406545,-68.7569253242312,
0.));
#128961=CARTESIAN_POINT('Ctrl Pts',(17.2608471147178,-68.7352611482519,
0.));
#128962=CARTESIAN_POINT('Ctrl Pts',(17.2620514472176,-68.7136437951074,
0.));
#128963=CARTESIAN_POINT('Ctrl Pts',(17.263230904689,-68.6920734222932,0.));
#128964=CARTESIAN_POINT('Ctrl Pts',(17.2643855540895,-68.6705501880263,
0.));
#128965=CARTESIAN_POINT('Ctrl Pts',(17.2655154627935,-68.6490742512085,
0.));
#128966=CARTESIAN_POINT('Ctrl Pts',(17.266620698609,-68.6276457714757,0.));
#128967=CARTESIAN_POINT('Ctrl Pts',(17.2677013298061,-68.606264909278,0.));
#128968=CARTESIAN_POINT('Ctrl Pts',(17.2687574251428,-68.5849318259449,
0.));
#128969=CARTESIAN_POINT('Ctrl Pts',(17.2697890538956,-68.5636466837502,
0.));
#128970=CARTESIAN_POINT('Ctrl Pts',(17.2707962858912,-68.5424096459746,
0.));
#128971=CARTESIAN_POINT('Ctrl Pts',(17.2717791914537,-68.5212208767835,
0.));
#128972=CARTESIAN_POINT('Ctrl Pts',(17.2727378413485,-68.5000805410896,
0.));
#128973=CARTESIAN_POINT('Ctrl Pts',(17.2736723067366,-68.4789888044357,
0.));
#128974=CARTESIAN_POINT('Ctrl Pts',(17.2745826591125,-68.4579458328208,
0.));
#128975=CARTESIAN_POINT('Ctrl Pts',(17.2754689703001,-68.4369517926803,
0.));
#128976=CARTESIAN_POINT('Ctrl Pts',(17.2763313126025,-68.4160068512781,
0.));
#128977=CARTESIAN_POINT('Ctrl Pts',(17.2771697589387,-68.3951111770498,
0.));
#128978=CARTESIAN_POINT('Ctrl Pts',(17.2779843829605,-68.374264939895,0.));
#128979=CARTESIAN_POINT('Ctrl Pts',(17.2787752592475,-68.353468311648,0.));
#128980=CARTESIAN_POINT('Ctrl Pts',(17.2795424631789,-68.3327214657533,
0.));
#128981=CARTESIAN_POINT('Ctrl Pts',(17.2802860705807,-68.3120245763884,
0.));
#128982=CARTESIAN_POINT('Ctrl Pts',(17.2810061574352,-68.2913778177258,
0.));
#128983=CARTESIAN_POINT('Ctrl Pts',(17.2817027995838,-68.2707813631761,
0.));
#128984=CARTESIAN_POINT('Ctrl Pts',(17.2823760723886,-68.250235384512,0.));
#128985=CARTESIAN_POINT('Ctrl Pts',(17.2830260513878,-68.2297400535339,
0.));
#128986=CARTESIAN_POINT('Ctrl Pts',(17.2836528130825,-68.2092955440591,
0.));
#128987=CARTESIAN_POINT('Ctrl Pts',(17.2842564355796,-68.1889020335418,
0.));
#128988=CARTESIAN_POINT('Ctrl Pts',(17.2848369995283,-68.1685597054193,
0.));
#128989=CARTESIAN_POINT('Ctrl Pts',(17.2853945882059,-68.1482687493176,
0.));
#128990=CARTESIAN_POINT('Ctrl Pts',(17.2859292855694,-68.1280293561473,
0.));
#128991=CARTESIAN_POINT('Ctrl Pts',(17.2864411745455,-68.1078417137865,
0.));
#128992=CARTESIAN_POINT('Ctrl Pts',(17.2869303355438,-68.0877060033229,
0.));
#128993=CARTESIAN_POINT('Ctrl Pts',(17.2873968440855,-68.0676223930469,
0.));
#128994=CARTESIAN_POINT('Ctrl Pts',(17.2878407730981,-68.0475910442494,
0.));
#128995=CARTESIAN_POINT('Ctrl Pts',(17.2882621974737,-68.027612122741,0.));
#128996=CARTESIAN_POINT('Ctrl Pts',(17.28866119774,-68.007685808115,0.));
#128997=CARTESIAN_POINT('Ctrl Pts',(17.2890378644843,-67.9878123049132,
0.));
#128998=CARTESIAN_POINT('Ctrl Pts',(17.2893923013852,-67.9679918502441,
0.));
#128999=CARTESIAN_POINT('Ctrl Pts',(17.2897246158895,-67.9482246901517,
0.));
#129000=CARTESIAN_POINT('Ctrl Pts',(17.2900349103956,-67.9285110571662,
0.));
#129001=CARTESIAN_POINT('Ctrl Pts',(17.2903232740717,-67.908851149676,0.));
#129002=CARTESIAN_POINT('Ctrl Pts',(17.2905897724029,-67.8892451049871,
0.));
#129003=CARTESIAN_POINT('Ctrl Pts',(17.2908344459816,-67.8696929979178,
0.));
#129004=CARTESIAN_POINT('Ctrl Pts',(17.2910127431203,-67.8540944890057,
0.));
#129005=CARTESIAN_POINT('Ctrl Pts',(17.2911366591419,-67.8424198971214,
0.));
#129006=CARTESIAN_POINT('Ctrl Pts',(17.2912149114145,-67.8346476309106,
0.));
#129007=CARTESIAN_POINT('Ctrl Pts',(17.2912529479484,-67.8307641965655,
0.));
#129008=CARTESIAN_POINT('Ctrl Pts',(10.343287191141,-73.778495580227,0.));
#129009=CARTESIAN_POINT('Ctrl Pts',(10.343287191141,-73.778495580227,12.));
#129010=CARTESIAN_POINT('Ctrl Pts',(10.3449014384453,-73.7731377048058,
0.));
#129011=CARTESIAN_POINT('Ctrl Pts',(10.3449014384453,-73.7731377048058,
12.));
#129012=CARTESIAN_POINT('Ctrl Pts',(10.3481265449342,-73.7624245587789,
0.));
#129013=CARTESIAN_POINT('Ctrl Pts',(10.3481265449342,-73.7624245587789,
12.));
#129014=CARTESIAN_POINT('Ctrl Pts',(10.3529540403092,-73.7463626541854,
0.));
#129015=CARTESIAN_POINT('Ctrl Pts',(10.3529540403092,-73.7463626541854,
12.));
#129016=CARTESIAN_POINT('Ctrl Pts',(10.359370371262,-73.7249624109173,0.));
#129017=CARTESIAN_POINT('Ctrl Pts',(10.359370371262,-73.7249624109173,12.));
#129018=CARTESIAN_POINT('Ctrl Pts',(10.3673568984582,-73.6982381645206,
0.));
#129019=CARTESIAN_POINT('Ctrl Pts',(10.3673568984582,-73.6982381645206,
12.));
#129020=CARTESIAN_POINT('Ctrl Pts',(10.3753095356342,-73.6715399947839,
0.));
#129021=CARTESIAN_POINT('Ctrl Pts',(10.3753095356342,-73.6715399947839,
12.));
#129022=CARTESIAN_POINT('Ctrl Pts',(10.3832282820371,-73.6448679350696,
0.));
#129023=CARTESIAN_POINT('Ctrl Pts',(10.3832282820371,-73.6448679350696,
12.));
#129024=CARTESIAN_POINT('Ctrl Pts',(10.3911131417463,-73.6182220363156,
0.));
#129025=CARTESIAN_POINT('Ctrl Pts',(10.3911131417463,-73.6182220363156,
12.));
#129026=CARTESIAN_POINT('Ctrl Pts',(10.3989641265285,-73.5916023719713,
0.));
#129027=CARTESIAN_POINT('Ctrl Pts',(10.3989641265285,-73.5916023719713,
12.));
#129028=CARTESIAN_POINT('Ctrl Pts',(10.406781255551,-73.5650090359839,0.));
#129029=CARTESIAN_POINT('Ctrl Pts',(10.406781255551,-73.5650090359839,12.));
#129030=CARTESIAN_POINT('Ctrl Pts',(10.414564552681,-73.5384421354543,0.));
#129031=CARTESIAN_POINT('Ctrl Pts',(10.414564552681,-73.5384421354543,12.));
#129032=CARTESIAN_POINT('Ctrl Pts',(10.4223140444605,-73.5119017847575,
0.));
#129033=CARTESIAN_POINT('Ctrl Pts',(10.4223140444605,-73.5119017847575,
12.));
#129034=CARTESIAN_POINT('Ctrl Pts',(10.430029757865,-73.485388099225,0.));
#129035=CARTESIAN_POINT('Ctrl Pts',(10.430029757865,-73.485388099225,12.));
#129036=CARTESIAN_POINT('Ctrl Pts',(10.4377117180222,-73.4589011886197,
0.));
#129037=CARTESIAN_POINT('Ctrl Pts',(10.4377117180222,-73.4589011886197,
12.));
#129038=CARTESIAN_POINT('Ctrl Pts',(10.4453599463547,-73.4324411518554,
0.));
#129039=CARTESIAN_POINT('Ctrl Pts',(10.4453599463547,-73.4324411518554,
12.));
#129040=CARTESIAN_POINT('Ctrl Pts',(10.452974461845,-73.4060080806686,0.));
#129041=CARTESIAN_POINT('Ctrl Pts',(10.452974461845,-73.4060080806686,12.));
#129042=CARTESIAN_POINT('Ctrl Pts',(10.4605552819397,-73.37960206225,0.));
#129043=CARTESIAN_POINT('Ctrl Pts',(10.4605552819397,-73.37960206225,12.));
#129044=CARTESIAN_POINT('Ctrl Pts',(10.4681024236289,-73.3532231823659,
0.));
#129045=CARTESIAN_POINT('Ctrl Pts',(10.4681024236289,-73.3532231823659,
12.));
#129046=CARTESIAN_POINT('Ctrl Pts',(10.4756159043806,-73.3268715280575,
0.));
#129047=CARTESIAN_POINT('Ctrl Pts',(10.4756159043806,-73.3268715280575,
12.));
#129048=CARTESIAN_POINT('Ctrl Pts',(10.4830957433305,-73.3005471910583,
0.));
#129049=CARTESIAN_POINT('Ctrl Pts',(10.4830957433305,-73.3005471910583,
12.));
#129050=CARTESIAN_POINT('Ctrl Pts',(10.4905419611523,-73.2742502674304,
0.));
#129051=CARTESIAN_POINT('Ctrl Pts',(10.4905419611523,-73.2742502674304,
12.));
#129052=CARTESIAN_POINT('Ctrl Pts',(10.4979545795192,-73.2479808560189,
0.));
#129053=CARTESIAN_POINT('Ctrl Pts',(10.4979545795192,-73.2479808560189,
12.));
#129054=CARTESIAN_POINT('Ctrl Pts',(10.5053336206908,-73.2217390572562,
0.));
#129055=CARTESIAN_POINT('Ctrl Pts',(10.5053336206908,-73.2217390572562,
12.));
#129056=CARTESIAN_POINT('Ctrl Pts',(10.5126791070805,-73.1955249719048,
0.));
#129057=CARTESIAN_POINT('Ctrl Pts',(10.5126791070805,-73.1955249719048,
12.));
#129058=CARTESIAN_POINT('Ctrl Pts',(10.5199910607654,-73.1693386996138,
0.));
#129059=CARTESIAN_POINT('Ctrl Pts',(10.5199910607654,-73.1693386996138,
12.));
#129060=CARTESIAN_POINT('Ctrl Pts',(10.5272695032653,-73.1431803382711,
0.));
#129061=CARTESIAN_POINT('Ctrl Pts',(10.5272695032653,-73.1431803382711,
12.));
#129062=CARTESIAN_POINT('Ctrl Pts',(10.53451445581,-73.1170499848039,0.));
#129063=CARTESIAN_POINT('Ctrl Pts',(10.53451445581,-73.1170499848039,12.));
#129064=CARTESIAN_POINT('Ctrl Pts',(10.5417259395002,-73.0909477356474,
0.));
#129065=CARTESIAN_POINT('Ctrl Pts',(10.5417259395002,-73.0909477356474,
12.));
#129066=CARTESIAN_POINT('Ctrl Pts',(10.5489039755138,-73.0648736873434,
0.));
#129067=CARTESIAN_POINT('Ctrl Pts',(10.5489039755138,-73.0648736873434,
12.));
#129068=CARTESIAN_POINT('Ctrl Pts',(10.5560485852974,-73.0388279370834,
0.));
#129069=CARTESIAN_POINT('Ctrl Pts',(10.5560485852974,-73.0388279370834,
12.));
#129070=CARTESIAN_POINT('Ctrl Pts',(10.5631597907651,-73.0128105832621,
0.));
#129071=CARTESIAN_POINT('Ctrl Pts',(10.5631597907651,-73.0128105832621,
12.));
#129072=CARTESIAN_POINT('Ctrl Pts',(10.570237614205,-72.9868217252283,0.));
#129073=CARTESIAN_POINT('Ctrl Pts',(10.570237614205,-72.9868217252283,12.));
#129074=CARTESIAN_POINT('Ctrl Pts',(10.5772820781958,-72.9608614630534,
0.));
#129075=CARTESIAN_POINT('Ctrl Pts',(10.5772820781958,-72.9608614630534,
12.));
#129076=CARTESIAN_POINT('Ctrl Pts',(10.5842932055209,-72.9349298972822,
0.));
#129077=CARTESIAN_POINT('Ctrl Pts',(10.5842932055209,-72.9349298972822,
12.));
#129078=CARTESIAN_POINT('Ctrl Pts',(10.5912710190928,-72.9090271287083,
0.));
#129079=CARTESIAN_POINT('Ctrl Pts',(10.5912710190928,-72.9090271287083,
12.));
#129080=CARTESIAN_POINT('Ctrl Pts',(10.5982155418626,-72.8831532580845,
0.));
#129081=CARTESIAN_POINT('Ctrl Pts',(10.5982155418626,-72.8831532580845,
12.));
#129082=CARTESIAN_POINT('Ctrl Pts',(10.6051267968203,-72.8573083861337,
0.));
#129083=CARTESIAN_POINT('Ctrl Pts',(10.6051267968203,-72.8573083861337,
12.));
#129084=CARTESIAN_POINT('Ctrl Pts',(10.6120048070367,-72.8314926136881,
0.));
#129085=CARTESIAN_POINT('Ctrl Pts',(10.6120048070367,-72.8314926136881,
12.));
#129086=CARTESIAN_POINT('Ctrl Pts',(10.6188495956973,-72.8057060417887,
0.));
#129087=CARTESIAN_POINT('Ctrl Pts',(10.6188495956973,-72.8057060417887,
12.));
#129088=CARTESIAN_POINT('Ctrl Pts',(10.6256611861394,-72.7799487717911,
0.));
#129089=CARTESIAN_POINT('Ctrl Pts',(10.6256611861394,-72.7799487717911,
12.));
#129090=CARTESIAN_POINT('Ctrl Pts',(10.6324396018998,-72.7542209054812,
0.));
#129091=CARTESIAN_POINT('Ctrl Pts',(10.6324396018998,-72.7542209054812,
12.));
#129092=CARTESIAN_POINT('Ctrl Pts',(10.6391848667352,-72.7285225451293,
0.));
#129093=CARTESIAN_POINT('Ctrl Pts',(10.6391848667352,-72.7285225451293,
12.));
#129094=CARTESIAN_POINT('Ctrl Pts',(10.6458970045946,-72.7028537934317,
0.));
#129095=CARTESIAN_POINT('Ctrl Pts',(10.6458970045946,-72.7028537934317,
12.));
#129096=CARTESIAN_POINT('Ctrl Pts',(10.6525760396054,-72.6772147534752,
0.));
#129097=CARTESIAN_POINT('Ctrl Pts',(10.6525760396054,-72.6772147534752,
12.));
#129098=CARTESIAN_POINT('Ctrl Pts',(10.659221996058,-72.651605528691,0.));
#129099=CARTESIAN_POINT('Ctrl Pts',(10.659221996058,-72.651605528691,12.));
#129100=CARTESIAN_POINT('Ctrl Pts',(10.6658348983944,-72.6260262228065,
0.));
#129101=CARTESIAN_POINT('Ctrl Pts',(10.6658348983944,-72.6260262228065,
12.));
#129102=CARTESIAN_POINT('Ctrl Pts',(10.6724147711995,-72.6004769398019,
0.));
#129103=CARTESIAN_POINT('Ctrl Pts',(10.6724147711995,-72.6004769398019,
12.));
#129104=CARTESIAN_POINT('Ctrl Pts',(10.6789616392042,-72.5749577839415,
0.));
#129105=CARTESIAN_POINT('Ctrl Pts',(10.6789616392042,-72.5749577839415,
12.));
#129106=CARTESIAN_POINT('Ctrl Pts',(10.6854755272904,-72.5494688597961,
0.));
#129107=CARTESIAN_POINT('Ctrl Pts',(10.6854755272904,-72.5494688597961,
12.));
#129108=CARTESIAN_POINT('Ctrl Pts',(10.691956460499,-72.5240102722664,0.));
#129109=CARTESIAN_POINT('Ctrl Pts',(10.691956460499,-72.5240102722664,12.));
#129110=CARTESIAN_POINT('Ctrl Pts',(10.6984044640398,-72.4985821266023,
0.));
#129111=CARTESIAN_POINT('Ctrl Pts',(10.6984044640398,-72.4985821266023,
12.));
#129112=CARTESIAN_POINT('Ctrl Pts',(10.7048195633061,-72.4731845284227,
0.));
#129113=CARTESIAN_POINT('Ctrl Pts',(10.7048195633061,-72.4731845284227,
12.));
#129114=CARTESIAN_POINT('Ctrl Pts',(10.7112017838706,-72.4478175837156,
0.));
#129115=CARTESIAN_POINT('Ctrl Pts',(10.7112017838706,-72.4478175837156,
12.));
#129116=CARTESIAN_POINT('Ctrl Pts',(10.7175511514788,-72.4224813988347,
0.));
#129117=CARTESIAN_POINT('Ctrl Pts',(10.7175511514788,-72.4224813988347,
12.));
#129118=CARTESIAN_POINT('Ctrl Pts',(10.7238676920469,-72.3971760804933,
0.));
#129119=CARTESIAN_POINT('Ctrl Pts',(10.7238676920469,-72.3971760804933,
12.));
#129120=CARTESIAN_POINT('Ctrl Pts',(10.7301514316607,-72.3719017357571,
0.));
#129121=CARTESIAN_POINT('Ctrl Pts',(10.7301514316607,-72.3719017357571,
12.));
#129122=CARTESIAN_POINT('Ctrl Pts',(10.73640239658,-72.3466584720318,0.));
#129123=CARTESIAN_POINT('Ctrl Pts',(10.73640239658,-72.3466584720318,12.));
#129124=CARTESIAN_POINT('Ctrl Pts',(10.7426206132375,-72.3214463970641,
0.));
#129125=CARTESIAN_POINT('Ctrl Pts',(10.7426206132375,-72.3214463970641,
12.));
#129126=CARTESIAN_POINT('Ctrl Pts',(10.7488061082367,-72.2962656189556,
0.));
#129127=CARTESIAN_POINT('Ctrl Pts',(10.7488061082367,-72.2962656189556,
12.));
#129128=CARTESIAN_POINT('Ctrl Pts',(10.7549589083535,-72.2711162461681,
0.));
#129129=CARTESIAN_POINT('Ctrl Pts',(10.7549589083535,-72.2711162461681,
12.));
#129130=CARTESIAN_POINT('Ctrl Pts',(10.7610790405385,-72.2459983875296,
0.));
#129131=CARTESIAN_POINT('Ctrl Pts',(10.7610790405385,-72.2459983875296,
12.));
#129132=CARTESIAN_POINT('Ctrl Pts',(10.7671665319255,-72.2209121522366,
0.));
#129133=CARTESIAN_POINT('Ctrl Pts',(10.7671665319255,-72.2209121522366,
12.));
#129134=CARTESIAN_POINT('Ctrl Pts',(10.7732214098344,-72.1958576498558,
0.));
#129135=CARTESIAN_POINT('Ctrl Pts',(10.7732214098344,-72.1958576498558,
12.));
#129136=CARTESIAN_POINT('Ctrl Pts',(10.7792437017662,-72.1708349903305,
0.));
#129137=CARTESIAN_POINT('Ctrl Pts',(10.7792437017662,-72.1708349903305,
12.));
#129138=CARTESIAN_POINT('Ctrl Pts',(10.7852334354016,-72.1458442839834,
0.));
#129139=CARTESIAN_POINT('Ctrl Pts',(10.7852334354016,-72.1458442839834,
12.));
#129140=CARTESIAN_POINT('Ctrl Pts',(10.7911906386027,-72.1208856415171,
0.));
#129141=CARTESIAN_POINT('Ctrl Pts',(10.7911906386027,-72.1208856415171,
12.));
#129142=CARTESIAN_POINT('Ctrl Pts',(10.7971153394166,-72.0959591740114,
0.));
#129143=CARTESIAN_POINT('Ctrl Pts',(10.7971153394166,-72.0959591740114,
12.));
#129144=CARTESIAN_POINT('Ctrl Pts',(10.8030075660808,-72.0710649929202,
0.));
#129145=CARTESIAN_POINT('Ctrl Pts',(10.8030075660808,-72.0710649929202,
12.));
#129146=CARTESIAN_POINT('Ctrl Pts',(10.8088673470184,-72.0462032100815,
0.));
#129147=CARTESIAN_POINT('Ctrl Pts',(10.8088673470184,-72.0462032100815,
12.));
#129148=CARTESIAN_POINT('Ctrl Pts',(10.8146947108375,-72.0213739377223,
0.));
#129149=CARTESIAN_POINT('Ctrl Pts',(10.8146947108375,-72.0213739377223,
12.));
#129150=CARTESIAN_POINT('Ctrl Pts',(10.8204896863328,-71.9965772884619,
0.));
#129151=CARTESIAN_POINT('Ctrl Pts',(10.8204896863328,-71.9965772884619,
12.));
#129152=CARTESIAN_POINT('Ctrl Pts',(10.8262523024897,-71.9718133753127,
0.));
#129153=CARTESIAN_POINT('Ctrl Pts',(10.8262523024897,-71.9718133753127,
12.));
#129154=CARTESIAN_POINT('Ctrl Pts',(10.8319825884918,-71.9470823116785,
0.));
#129155=CARTESIAN_POINT('Ctrl Pts',(10.8319825884918,-71.9470823116785,
12.));
#129156=CARTESIAN_POINT('Ctrl Pts',(10.8376805737159,-71.9223842113625,
0.));
#129157=CARTESIAN_POINT('Ctrl Pts',(10.8376805737159,-71.9223842113625,
12.));
#129158=CARTESIAN_POINT('Ctrl Pts',(10.8433462877311,-71.8977191885725,
0.));
#129159=CARTESIAN_POINT('Ctrl Pts',(10.8433462877311,-71.8977191885725,
12.));
#129160=CARTESIAN_POINT('Ctrl Pts',(10.8489797602997,-71.8730873579224,
0.));
#129161=CARTESIAN_POINT('Ctrl Pts',(10.8489797602997,-71.8730873579224,
12.));
#129162=CARTESIAN_POINT('Ctrl Pts',(10.8545810213799,-71.8484888344339,
0.));
#129163=CARTESIAN_POINT('Ctrl Pts',(10.8545810213799,-71.8484888344339,
12.));
#129164=CARTESIAN_POINT('Ctrl Pts',(10.8601501011332,-71.8239237335331,
0.));
#129165=CARTESIAN_POINT('Ctrl Pts',(10.8601501011332,-71.8239237335331,
12.));
#129166=CARTESIAN_POINT('Ctrl Pts',(10.865687029922,-71.7993921710564,0.));
#129167=CARTESIAN_POINT('Ctrl Pts',(10.865687029922,-71.7993921710564,12.));
#129168=CARTESIAN_POINT('Ctrl Pts',(10.8711918383073,-71.7748942632593,
0.));
#129169=CARTESIAN_POINT('Ctrl Pts',(10.8711918383073,-71.7748942632593,
12.));
#129170=CARTESIAN_POINT('Ctrl Pts',(10.8766645570497,-71.7504301268181,
0.));
#129171=CARTESIAN_POINT('Ctrl Pts',(10.8766645570497,-71.7504301268181,
12.));
#129172=CARTESIAN_POINT('Ctrl Pts',(10.882105217112,-71.7259998788328,0.));
#129173=CARTESIAN_POINT('Ctrl Pts',(10.882105217112,-71.7259998788328,12.));
#129174=CARTESIAN_POINT('Ctrl Pts',(10.8875138496671,-71.7016036368236,
0.));
#129175=CARTESIAN_POINT('Ctrl Pts',(10.8875138496671,-71.7016036368236,
12.));
#129176=CARTESIAN_POINT('Ctrl Pts',(10.8928904860964,-71.6772415187364,
0.));
#129177=CARTESIAN_POINT('Ctrl Pts',(10.8928904860964,-71.6772415187364,
12.));
#129178=CARTESIAN_POINT('Ctrl Pts',(10.898235157987,-71.6529136429504,0.));
#129179=CARTESIAN_POINT('Ctrl Pts',(10.898235157987,-71.6529136429504,12.));
#129180=CARTESIAN_POINT('Ctrl Pts',(10.9035478971328,-71.6286201282812,
0.));
#129181=CARTESIAN_POINT('Ctrl Pts',(10.9035478971328,-71.6286201282812,
12.));
#129182=CARTESIAN_POINT('Ctrl Pts',(10.9088287355365,-71.6043610939835,
0.));
#129183=CARTESIAN_POINT('Ctrl Pts',(10.9088287355365,-71.6043610939835,
12.));
#129184=CARTESIAN_POINT('Ctrl Pts',(10.914077705417,-71.5801366597488,0.));
#129185=CARTESIAN_POINT('Ctrl Pts',(10.914077705417,-71.5801366597488,12.));
#129186=CARTESIAN_POINT('Ctrl Pts',(10.91929483921,-71.5559469457091,0.));
#129187=CARTESIAN_POINT('Ctrl Pts',(10.91929483921,-71.5559469457091,12.));
#129188=CARTESIAN_POINT('Ctrl Pts',(10.9244801695642,-71.5317920724459,
0.));
#129189=CARTESIAN_POINT('Ctrl Pts',(10.9244801695642,-71.5317920724459,
12.));
#129190=CARTESIAN_POINT('Ctrl Pts',(10.9296337293424,-71.5076721609937,
0.));
#129191=CARTESIAN_POINT('Ctrl Pts',(10.9296337293424,-71.5076721609937,
12.));
#129192=CARTESIAN_POINT('Ctrl Pts',(10.9347555516235,-71.4835873328423,
0.));
#129193=CARTESIAN_POINT('Ctrl Pts',(10.9347555516235,-71.4835873328423,
12.));
#129194=CARTESIAN_POINT('Ctrl Pts',(10.9398456697095,-71.4595377099351,
0.));
#129195=CARTESIAN_POINT('Ctrl Pts',(10.9398456697095,-71.4595377099351,
12.));
#129196=CARTESIAN_POINT('Ctrl Pts',(10.944904117127,-71.435523414672,0.));
#129197=CARTESIAN_POINT('Ctrl Pts',(10.944904117127,-71.435523414672,12.));
#129198=CARTESIAN_POINT('Ctrl Pts',(10.9499309276236,-71.4115445699194,
0.));
#129199=CARTESIAN_POINT('Ctrl Pts',(10.9499309276236,-71.4115445699194,
12.));
#129200=CARTESIAN_POINT('Ctrl Pts',(10.954926135169,-71.3876012990138,0.));
#129201=CARTESIAN_POINT('Ctrl Pts',(10.954926135169,-71.3876012990138,12.));
#129202=CARTESIAN_POINT('Ctrl Pts',(10.9598897739564,-71.3636937257649,
0.));
#129203=CARTESIAN_POINT('Ctrl Pts',(10.9598897739564,-71.3636937257649,
12.));
#129204=CARTESIAN_POINT('Ctrl Pts',(10.9648218784098,-71.339821974454,0.));
#129205=CARTESIAN_POINT('Ctrl Pts',(10.9648218784098,-71.339821974454,12.));
#129206=CARTESIAN_POINT('Ctrl Pts',(10.969722483186,-71.3159861698358,0.));
#129207=CARTESIAN_POINT('Ctrl Pts',(10.969722483186,-71.3159861698358,12.));
#129208=CARTESIAN_POINT('Ctrl Pts',(10.9745916231709,-71.2921864371491,
0.));
#129209=CARTESIAN_POINT('Ctrl Pts',(10.9745916231709,-71.2921864371491,
12.));
#129210=CARTESIAN_POINT('Ctrl Pts',(10.9794293334805,-71.2684229021207,
0.));
#129211=CARTESIAN_POINT('Ctrl Pts',(10.9794293334805,-71.2684229021207,
12.));
#129212=CARTESIAN_POINT('Ctrl Pts',(10.9842356494627,-71.2446956909687,
0.));
#129213=CARTESIAN_POINT('Ctrl Pts',(10.9842356494627,-71.2446956909687,
12.));
#129214=CARTESIAN_POINT('Ctrl Pts',(10.9890106067039,-71.2210049304014,
0.));
#129215=CARTESIAN_POINT('Ctrl Pts',(10.9890106067039,-71.2210049304014,
12.));
#129216=CARTESIAN_POINT('Ctrl Pts',(10.993754241032,-71.1973507476191,0.));
#129217=CARTESIAN_POINT('Ctrl Pts',(10.993754241032,-71.1973507476191,12.));
#129218=CARTESIAN_POINT('Ctrl Pts',(10.9984665885127,-71.1737332703248,
0.));
#129219=CARTESIAN_POINT('Ctrl Pts',(10.9984665885127,-71.1737332703248,
12.));
#129220=CARTESIAN_POINT('Ctrl Pts',(11.0031476854502,-71.1501526267286,
0.));
#129221=CARTESIAN_POINT('Ctrl Pts',(11.0031476854502,-71.1501526267286,
12.));
#129222=CARTESIAN_POINT('Ctrl Pts',(11.0077975683895,-71.1266089455517,
0.));
#129223=CARTESIAN_POINT('Ctrl Pts',(11.0077975683895,-71.1266089455517,
12.));
#129224=CARTESIAN_POINT('Ctrl Pts',(11.0124162741224,-71.1031023560249,
0.));
#129225=CARTESIAN_POINT('Ctrl Pts',(11.0124162741224,-71.1031023560249,
12.));
#129226=CARTESIAN_POINT('Ctrl Pts',(11.0170038396915,-71.0796329878907,
0.));
#129227=CARTESIAN_POINT('Ctrl Pts',(11.0170038396915,-71.0796329878907,
12.));
#129228=CARTESIAN_POINT('Ctrl Pts',(11.0215603023856,-71.0562009714136,
0.));
#129229=CARTESIAN_POINT('Ctrl Pts',(11.0215603023856,-71.0562009714136,
12.));
#129230=CARTESIAN_POINT('Ctrl Pts',(11.0260856997415,-71.0328064373856,
0.));
#129231=CARTESIAN_POINT('Ctrl Pts',(11.0260856997415,-71.0328064373856,
12.));
#129232=CARTESIAN_POINT('Ctrl Pts',(11.0305800695456,-71.0094495171292,
0.));
#129233=CARTESIAN_POINT('Ctrl Pts',(11.0305800695456,-71.0094495171292,
12.));
#129234=CARTESIAN_POINT('Ctrl Pts',(11.0350434498405,-70.986130342497,0.));
#129235=CARTESIAN_POINT('Ctrl Pts',(11.0350434498405,-70.986130342497,12.));
#129236=CARTESIAN_POINT('Ctrl Pts',(11.0394758789285,-70.9628490458748,
0.));
#129237=CARTESIAN_POINT('Ctrl Pts',(11.0394758789285,-70.9628490458748,
12.));
#129238=CARTESIAN_POINT('Ctrl Pts',(11.0438773953681,-70.9396057601924,
0.));
#129239=CARTESIAN_POINT('Ctrl Pts',(11.0438773953681,-70.9396057601924,
12.));
#129240=CARTESIAN_POINT('Ctrl Pts',(11.048248037975,-70.916400618927,0.));
#129241=CARTESIAN_POINT('Ctrl Pts',(11.048248037975,-70.916400618927,12.));
#129242=CARTESIAN_POINT('Ctrl Pts',(11.0525878458243,-70.8932337561087,
0.));
#129243=CARTESIAN_POINT('Ctrl Pts',(11.0525878458243,-70.8932337561087,
12.));
#129244=CARTESIAN_POINT('Ctrl Pts',(11.0568968582569,-70.8701053063186,
0.));
#129245=CARTESIAN_POINT('Ctrl Pts',(11.0568968582569,-70.8701053063186,
12.));
#129246=CARTESIAN_POINT('Ctrl Pts',(11.0611751148834,-70.8470154046919,
0.));
#129247=CARTESIAN_POINT('Ctrl Pts',(11.0611751148834,-70.8470154046919,
12.));
#129248=CARTESIAN_POINT('Ctrl Pts',(11.0654226555802,-70.8239641869299,
0.));
#129249=CARTESIAN_POINT('Ctrl Pts',(11.0654226555802,-70.8239641869299,
12.));
#129250=CARTESIAN_POINT('Ctrl Pts',(11.0696395204909,-70.8009517893057,
0.));
#129251=CARTESIAN_POINT('Ctrl Pts',(11.0696395204909,-70.8009517893057,
12.));
#129252=CARTESIAN_POINT('Ctrl Pts',(11.073825750029,-70.7779783486677,0.));
#129253=CARTESIAN_POINT('Ctrl Pts',(11.073825750029,-70.7779783486677,12.));
#129254=CARTESIAN_POINT('Ctrl Pts',(11.0779813848846,-70.7550440024384,
0.));
#129255=CARTESIAN_POINT('Ctrl Pts',(11.0779813848846,-70.7550440024384,
12.));
#129256=CARTESIAN_POINT('Ctrl Pts',(11.0821064660269,-70.732148888618,0.));
#129257=CARTESIAN_POINT('Ctrl Pts',(11.0821064660269,-70.732148888618,12.));
#129258=CARTESIAN_POINT('Ctrl Pts',(11.0862010347016,-70.7092931457954,
0.));
#129259=CARTESIAN_POINT('Ctrl Pts',(11.0862010347016,-70.7092931457954,
12.));
#129260=CARTESIAN_POINT('Ctrl Pts',(11.0902651324323,-70.6864769131546,
0.));
#129261=CARTESIAN_POINT('Ctrl Pts',(11.0902651324323,-70.6864769131546,
12.));
#129262=CARTESIAN_POINT('Ctrl Pts',(11.0942988010233,-70.6637003304785,
0.));
#129263=CARTESIAN_POINT('Ctrl Pts',(11.0942988010233,-70.6637003304785,
12.));
#129264=CARTESIAN_POINT('Ctrl Pts',(11.0983020825667,-70.6409635381482,
0.));
#129265=CARTESIAN_POINT('Ctrl Pts',(11.0983020825667,-70.6409635381482,
12.));
#129266=CARTESIAN_POINT('Ctrl Pts',(11.1022750194445,-70.6182666771481,
0.));
#129267=CARTESIAN_POINT('Ctrl Pts',(11.1022750194445,-70.6182666771481,
12.));
#129268=CARTESIAN_POINT('Ctrl Pts',(11.1062176543262,-70.5956098890773,
0.));
#129269=CARTESIAN_POINT('Ctrl Pts',(11.1062176543262,-70.5956098890773,
12.));
#129270=CARTESIAN_POINT('Ctrl Pts',(11.1101300301701,-70.5729933161546,
0.));
#129271=CARTESIAN_POINT('Ctrl Pts',(11.1101300301701,-70.5729933161546,
12.));
#129272=CARTESIAN_POINT('Ctrl Pts',(11.1140121902271,-70.5504171012234,
0.));
#129273=CARTESIAN_POINT('Ctrl Pts',(11.1140121902271,-70.5504171012234,
12.));
#129274=CARTESIAN_POINT('Ctrl Pts',(11.1178641780476,-70.5278813877494,
0.));
#129275=CARTESIAN_POINT('Ctrl Pts',(11.1178641780476,-70.5278813877494,
12.));
#129276=CARTESIAN_POINT('Ctrl Pts',(11.1216860374826,-70.505386319828,0.));
#129277=CARTESIAN_POINT('Ctrl Pts',(11.1216860374826,-70.505386319828,12.));
#129278=CARTESIAN_POINT('Ctrl Pts',(11.1254778126821,-70.4829320421957,
0.));
#129279=CARTESIAN_POINT('Ctrl Pts',(11.1254778126821,-70.4829320421957,
12.));
#129280=CARTESIAN_POINT('Ctrl Pts',(11.1292395480974,-70.4605187002354,
0.));
#129281=CARTESIAN_POINT('Ctrl Pts',(11.1292395480974,-70.4605187002354,
12.));
#129282=CARTESIAN_POINT('Ctrl Pts',(11.1329712884846,-70.4381464399819,
0.));
#129283=CARTESIAN_POINT('Ctrl Pts',(11.1329712884846,-70.4381464399819,
12.));
#129284=CARTESIAN_POINT('Ctrl Pts',(11.1366730789125,-70.4158154081205,
0.));
#129285=CARTESIAN_POINT('Ctrl Pts',(11.1366730789125,-70.4158154081205,
12.));
#129286=CARTESIAN_POINT('Ctrl Pts',(11.1403449647625,-70.393525751996,0.));
#129287=CARTESIAN_POINT('Ctrl Pts',(11.1403449647625,-70.393525751996,12.));
#129288=CARTESIAN_POINT('Ctrl Pts',(11.143986991727,-70.3712776196223,0.));
#129289=CARTESIAN_POINT('Ctrl Pts',(11.143986991727,-70.3712776196223,12.));
#129290=CARTESIAN_POINT('Ctrl Pts',(11.1475992058124,-70.349071159688,0.));
#129291=CARTESIAN_POINT('Ctrl Pts',(11.1475992058124,-70.349071159688,12.));
#129292=CARTESIAN_POINT('Ctrl Pts',(11.1511816533421,-70.326906521559,0.));
#129293=CARTESIAN_POINT('Ctrl Pts',(11.1511816533421,-70.326906521559,12.));
#129294=CARTESIAN_POINT('Ctrl Pts',(11.1547343809646,-70.3047838552756,
0.));
#129295=CARTESIAN_POINT('Ctrl Pts',(11.1547343809646,-70.3047838552756,
12.));
#129296=CARTESIAN_POINT('Ctrl Pts',(11.158257435652,-70.2827033115662,0.));
#129297=CARTESIAN_POINT('Ctrl Pts',(11.158257435652,-70.2827033115662,12.));
#129298=CARTESIAN_POINT('Ctrl Pts',(11.1617508647016,-70.260665041859,0.));
#129299=CARTESIAN_POINT('Ctrl Pts',(11.1617508647016,-70.260665041859,12.));
#129300=CARTESIAN_POINT('Ctrl Pts',(11.1652147157383,-70.2386691982902,
0.));
#129301=CARTESIAN_POINT('Ctrl Pts',(11.1652147157383,-70.2386691982902,
12.));
#129302=CARTESIAN_POINT('Ctrl Pts',(11.168649036721,-70.2167159337094,0.));
#129303=CARTESIAN_POINT('Ctrl Pts',(11.168649036721,-70.2167159337094,12.));
#129304=CARTESIAN_POINT('Ctrl Pts',(11.1720538759499,-70.1948054016816,
0.));
#129305=CARTESIAN_POINT('Ctrl Pts',(11.1720538759499,-70.1948054016816,
12.));
#129306=CARTESIAN_POINT('Ctrl Pts',(11.1754292820631,-70.1729377564954,
0.));
#129307=CARTESIAN_POINT('Ctrl Pts',(11.1754292820631,-70.1729377564954,
12.));
#129308=CARTESIAN_POINT('Ctrl Pts',(11.1787753040363,-70.1511131531672,
0.));
#129309=CARTESIAN_POINT('Ctrl Pts',(11.1787753040363,-70.1511131531672,
12.));
#129310=CARTESIAN_POINT('Ctrl Pts',(11.1820919911846,-70.1293317474432,
0.));
#129311=CARTESIAN_POINT('Ctrl Pts',(11.1820919911846,-70.1293317474432,
12.));
#129312=CARTESIAN_POINT('Ctrl Pts',(11.185379393167,-70.1075936957973,0.));
#129313=CARTESIAN_POINT('Ctrl Pts',(11.185379393167,-70.1075936957973,12.));
#129314=CARTESIAN_POINT('Ctrl Pts',(11.1886375599916,-70.0858991554295,
0.));
#129315=CARTESIAN_POINT('Ctrl Pts',(11.1886375599916,-70.0858991554295,
12.));
#129316=CARTESIAN_POINT('Ctrl Pts',(11.1918665420168,-70.0642482842942,
0.));
#129317=CARTESIAN_POINT('Ctrl Pts',(11.1918665420168,-70.0642482842942,
12.));
#129318=CARTESIAN_POINT('Ctrl Pts',(11.1950663899578,-70.0426412411194,
0.));
#129319=CARTESIAN_POINT('Ctrl Pts',(11.1950663899578,-70.0426412411194,
12.));
#129320=CARTESIAN_POINT('Ctrl Pts',(11.1982371548918,-70.0210781854236,
0.));
#129321=CARTESIAN_POINT('Ctrl Pts',(11.1982371548918,-70.0210781854236,
12.));
#129322=CARTESIAN_POINT('Ctrl Pts',(11.2013788882711,-69.9995592775322,
0.));
#129323=CARTESIAN_POINT('Ctrl Pts',(11.2013788882711,-69.9995592775322,
12.));
#129324=CARTESIAN_POINT('Ctrl Pts',(11.2044916419239,-69.9780846785771,
0.));
#129325=CARTESIAN_POINT('Ctrl Pts',(11.2044916419239,-69.9780846785771,
12.));
#129326=CARTESIAN_POINT('Ctrl Pts',(11.2075754680445,-69.9566545504813,
0.));
#129327=CARTESIAN_POINT('Ctrl Pts',(11.2075754680445,-69.9566545504813,
12.));
#129328=CARTESIAN_POINT('Ctrl Pts',(11.2106304191881,-69.9352690559399,
0.));
#129329=CARTESIAN_POINT('Ctrl Pts',(11.2106304191881,-69.9352690559399,
12.));
#129330=CARTESIAN_POINT('Ctrl Pts',(11.2136565482679,-69.9139283584036,
0.));
#129331=CARTESIAN_POINT('Ctrl Pts',(11.2136565482679,-69.9139283584036,
12.));
#129332=CARTESIAN_POINT('Ctrl Pts',(11.2166539085527,-69.8926326220414,
0.));
#129333=CARTESIAN_POINT('Ctrl Pts',(11.2166539085527,-69.8926326220414,
12.));
#129334=CARTESIAN_POINT('Ctrl Pts',(11.2196225536794,-69.8713820117918,
0.));
#129335=CARTESIAN_POINT('Ctrl Pts',(11.2196225536794,-69.8713820117918,
12.));
#129336=CARTESIAN_POINT('Ctrl Pts',(11.2225625376739,-69.8501766934445,
0.));
#129337=CARTESIAN_POINT('Ctrl Pts',(11.2225625376739,-69.8501766934445,
12.));
#129338=CARTESIAN_POINT('Ctrl Pts',(11.225473914972,-69.8290168337076,0.));
#129339=CARTESIAN_POINT('Ctrl Pts',(11.225473914972,-69.8290168337076,12.));
#129340=CARTESIAN_POINT('Ctrl Pts',(11.2283567404434,-69.8079026002753,
0.));
#129341=CARTESIAN_POINT('Ctrl Pts',(11.2283567404434,-69.8079026002753,
12.));
#129342=CARTESIAN_POINT('Ctrl Pts',(11.2312110694183,-69.7868341618927,
0.));
#129343=CARTESIAN_POINT('Ctrl Pts',(11.2312110694183,-69.7868341618927,
12.));
#129344=CARTESIAN_POINT('Ctrl Pts',(11.2340369576452,-69.7658116882298,
0.));
#129345=CARTESIAN_POINT('Ctrl Pts',(11.2340369576452,-69.7658116882298,
12.));
#129346=CARTESIAN_POINT('Ctrl Pts',(11.236834461247,-69.7448353497394,0.));
#129347=CARTESIAN_POINT('Ctrl Pts',(11.236834461247,-69.7448353497394,12.));
#129348=CARTESIAN_POINT('Ctrl Pts',(11.2396036366861,-69.7239053175362,
0.));
#129349=CARTESIAN_POINT('Ctrl Pts',(11.2396036366861,-69.7239053175362,
12.));
#129350=CARTESIAN_POINT('Ctrl Pts',(11.242344540717,-69.7030217632187,0.));
#129351=CARTESIAN_POINT('Ctrl Pts',(11.242344540717,-69.7030217632187,12.));
#129352=CARTESIAN_POINT('Ctrl Pts',(11.2450572303847,-69.6821848588492,
0.));
#129353=CARTESIAN_POINT('Ctrl Pts',(11.2450572303847,-69.6821848588492,
12.));
#129354=CARTESIAN_POINT('Ctrl Pts',(11.247741763139,-69.6613947773563,0.));
#129355=CARTESIAN_POINT('Ctrl Pts',(11.247741763139,-69.6613947773563,12.));
#129356=CARTESIAN_POINT('Ctrl Pts',(11.2503981969413,-69.6406516928902,
0.));
#129357=CARTESIAN_POINT('Ctrl Pts',(11.2503981969413,-69.6406516928902,
12.));
#129358=CARTESIAN_POINT('Ctrl Pts',(11.2530265903555,-69.6199557811231,
0.));
#129359=CARTESIAN_POINT('Ctrl Pts',(11.2530265903555,-69.6199557811231,
12.));
#129360=CARTESIAN_POINT('Ctrl Pts',(11.255627002701,-69.5993072197355,0.));
#129361=CARTESIAN_POINT('Ctrl Pts',(11.255627002701,-69.5993072197355,12.));
#129362=CARTESIAN_POINT('Ctrl Pts',(11.2581994939534,-69.5787061880815,
0.));
#129363=CARTESIAN_POINT('Ctrl Pts',(11.2581994939534,-69.5787061880815,
12.));
#129364=CARTESIAN_POINT('Ctrl Pts',(11.2607441244697,-69.5581528662846,
0.));
#129365=CARTESIAN_POINT('Ctrl Pts',(11.2607441244697,-69.5581528662846,
12.));
#129366=CARTESIAN_POINT('Ctrl Pts',(11.2632609547629,-69.5376474344768,
0.));
#129367=CARTESIAN_POINT('Ctrl Pts',(11.2632609547629,-69.5376474344768,
12.));
#129368=CARTESIAN_POINT('Ctrl Pts',(11.265750045272,-69.5171900720188,0.));
#129369=CARTESIAN_POINT('Ctrl Pts',(11.265750045272,-69.5171900720188,12.));
#129370=CARTESIAN_POINT('Ctrl Pts',(11.2682114561015,-69.4967809565978,
0.));
#129371=CARTESIAN_POINT('Ctrl Pts',(11.2682114561015,-69.4967809565978,
12.));
#129372=CARTESIAN_POINT('Ctrl Pts',(11.2706452475287,-69.4764202659443,
0.));
#129373=CARTESIAN_POINT('Ctrl Pts',(11.2706452475287,-69.4764202659443,
12.));
#129374=CARTESIAN_POINT('Ctrl Pts',(11.2730514806143,-69.4561081798815,
0.));
#129375=CARTESIAN_POINT('Ctrl Pts',(11.2730514806143,-69.4561081798815,
12.));
#129376=CARTESIAN_POINT('Ctrl Pts',(11.2754302177019,-69.4358448819957,
0.));
#129377=CARTESIAN_POINT('Ctrl Pts',(11.2754302177019,-69.4358448819957,
12.));
#129378=CARTESIAN_POINT('Ctrl Pts',(11.2777815231462,-69.4156305620554,
0.));
#129379=CARTESIAN_POINT('Ctrl Pts',(11.2777815231462,-69.4156305620554,
12.));
#129380=CARTESIAN_POINT('Ctrl Pts',(11.2801054633807,-69.395465416223,0.));
#129381=CARTESIAN_POINT('Ctrl Pts',(11.2801054633807,-69.395465416223,12.));
#129382=CARTESIAN_POINT('Ctrl Pts',(11.2824021054038,-69.375349642,0.));
#129383=CARTESIAN_POINT('Ctrl Pts',(11.2824021054038,-69.375349642,12.));
#129384=CARTESIAN_POINT('Ctrl Pts',(11.2846715154521,-69.3552834337771,
0.));
#129385=CARTESIAN_POINT('Ctrl Pts',(11.2846715154521,-69.3552834337771,
12.));
#129386=CARTESIAN_POINT('Ctrl Pts',(11.2869137578463,-69.3352669789611,
0.));
#129387=CARTESIAN_POINT('Ctrl Pts',(11.2869137578463,-69.3352669789611,
12.));
#129388=CARTESIAN_POINT('Ctrl Pts',(11.2891288931528,-69.315300451784,0.));
#129389=CARTESIAN_POINT('Ctrl Pts',(11.2891288931528,-69.315300451784,12.));
#129390=CARTESIAN_POINT('Ctrl Pts',(11.2913169799642,-69.2953840192792,
0.));
#129391=CARTESIAN_POINT('Ctrl Pts',(11.2913169799642,-69.2953840192792,
12.));
#129392=CARTESIAN_POINT('Ctrl Pts',(11.2934780784361,-69.2755178531534,
0.));
#129393=CARTESIAN_POINT('Ctrl Pts',(11.2934780784361,-69.2755178531534,
12.));
#129394=CARTESIAN_POINT('Ctrl Pts',(11.2956122531375,-69.255702139335,0.));
#129395=CARTESIAN_POINT('Ctrl Pts',(11.2956122531375,-69.255702139335,12.));
#129396=CARTESIAN_POINT('Ctrl Pts',(11.2977195764836,-69.2359370894828,
0.));
#129397=CARTESIAN_POINT('Ctrl Pts',(11.2977195764836,-69.2359370894828,
12.));
#129398=CARTESIAN_POINT('Ctrl Pts',(11.2998001310934,-69.216222948839,0.));
#129399=CARTESIAN_POINT('Ctrl Pts',(11.2998001310934,-69.216222948839,12.));
#129400=CARTESIAN_POINT('Ctrl Pts',(11.3018540025605,-69.1965599718761,
0.));
#129401=CARTESIAN_POINT('Ctrl Pts',(11.3018540025605,-69.1965599718761,
12.));
#129402=CARTESIAN_POINT('Ctrl Pts',(11.3038812726275,-69.1769483991639,
0.));
#129403=CARTESIAN_POINT('Ctrl Pts',(11.3038812726275,-69.1769483991639,
12.));
#129404=CARTESIAN_POINT('Ctrl Pts',(11.3058820128323,-69.1573884361076,
0.));
#129405=CARTESIAN_POINT('Ctrl Pts',(11.3058820128323,-69.1573884361076,
12.));
#129406=CARTESIAN_POINT('Ctrl Pts',(11.3078562764442,-69.137880225198,0.));
#129407=CARTESIAN_POINT('Ctrl Pts',(11.3078562764442,-69.137880225198,12.));
#129408=CARTESIAN_POINT('Ctrl Pts',(11.3098040973799,-69.1184238445065,
0.));
#129409=CARTESIAN_POINT('Ctrl Pts',(11.3098040973799,-69.1184238445065,
12.));
#129410=CARTESIAN_POINT('Ctrl Pts',(11.3113412156741,-69.1029002322497,
0.));
#129411=CARTESIAN_POINT('Ctrl Pts',(11.3113412156741,-69.1029002322497,
12.));
#129412=CARTESIAN_POINT('Ctrl Pts',(11.3124821678849,-69.0912808657051,
0.));
#129413=CARTESIAN_POINT('Ctrl Pts',(11.3124821678849,-69.0912808657051,
12.));
#129414=CARTESIAN_POINT('Ctrl Pts',(11.3132375200184,-69.0835449954486,
0.));
#129415=CARTESIAN_POINT('Ctrl Pts',(11.3132375200184,-69.0835449954486,
12.));
#129416=CARTESIAN_POINT('Ctrl Pts',(11.3136138754165,-69.079679653846,0.));
#129417=CARTESIAN_POINT('Ctrl Pts',(11.3136138754165,-69.079679653846,12.));
#129418=CARTESIAN_POINT('',(11.3136138754165,-69.079679653846,12.));
#129419=CARTESIAN_POINT('Ctrl Pts',(11.3136138754165,-69.079679653846,12.));
#129420=CARTESIAN_POINT('Ctrl Pts',(11.3132375200184,-69.0835449954486,
12.));
#129421=CARTESIAN_POINT('Ctrl Pts',(11.3124821678849,-69.0912808657051,
12.));
#129422=CARTESIAN_POINT('Ctrl Pts',(11.3113412156741,-69.1029002322497,
12.));
#129423=CARTESIAN_POINT('Ctrl Pts',(11.3098040973799,-69.1184238445065,
12.));
#129424=CARTESIAN_POINT('Ctrl Pts',(11.3078562764442,-69.137880225198,12.));
#129425=CARTESIAN_POINT('Ctrl Pts',(11.3058820128323,-69.1573884361076,
12.));
#129426=CARTESIAN_POINT('Ctrl Pts',(11.3038812726275,-69.1769483991639,
12.));
#129427=CARTESIAN_POINT('Ctrl Pts',(11.3018540025605,-69.1965599718761,
12.));
#129428=CARTESIAN_POINT('Ctrl Pts',(11.2998001310934,-69.216222948839,12.));
#129429=CARTESIAN_POINT('Ctrl Pts',(11.2977195764836,-69.2359370894828,
12.));
#129430=CARTESIAN_POINT('Ctrl Pts',(11.2956122531375,-69.255702139335,12.));
#129431=CARTESIAN_POINT('Ctrl Pts',(11.2934780784361,-69.2755178531534,
12.));
#129432=CARTESIAN_POINT('Ctrl Pts',(11.2913169799642,-69.2953840192792,
12.));
#129433=CARTESIAN_POINT('Ctrl Pts',(11.2891288931528,-69.315300451784,12.));
#129434=CARTESIAN_POINT('Ctrl Pts',(11.2869137578463,-69.3352669789611,
12.));
#129435=CARTESIAN_POINT('Ctrl Pts',(11.2846715154521,-69.3552834337771,
12.));
#129436=CARTESIAN_POINT('Ctrl Pts',(11.2824021054038,-69.375349642,12.));
#129437=CARTESIAN_POINT('Ctrl Pts',(11.2801054633807,-69.395465416223,12.));
#129438=CARTESIAN_POINT('Ctrl Pts',(11.2777815231462,-69.4156305620554,
12.));
#129439=CARTESIAN_POINT('Ctrl Pts',(11.2754302177019,-69.4358448819957,
12.));
#129440=CARTESIAN_POINT('Ctrl Pts',(11.2730514806143,-69.4561081798815,
12.));
#129441=CARTESIAN_POINT('Ctrl Pts',(11.2706452475287,-69.4764202659443,
12.));
#129442=CARTESIAN_POINT('Ctrl Pts',(11.2682114561015,-69.4967809565978,
12.));
#129443=CARTESIAN_POINT('Ctrl Pts',(11.265750045272,-69.5171900720188,12.));
#129444=CARTESIAN_POINT('Ctrl Pts',(11.2632609547629,-69.5376474344768,
12.));
#129445=CARTESIAN_POINT('Ctrl Pts',(11.2607441244697,-69.5581528662846,
12.));
#129446=CARTESIAN_POINT('Ctrl Pts',(11.2581994939534,-69.5787061880815,
12.));
#129447=CARTESIAN_POINT('Ctrl Pts',(11.255627002701,-69.5993072197355,12.));
#129448=CARTESIAN_POINT('Ctrl Pts',(11.2530265903555,-69.6199557811231,
12.));
#129449=CARTESIAN_POINT('Ctrl Pts',(11.2503981969413,-69.6406516928902,
12.));
#129450=CARTESIAN_POINT('Ctrl Pts',(11.247741763139,-69.6613947773563,12.));
#129451=CARTESIAN_POINT('Ctrl Pts',(11.2450572303847,-69.6821848588492,
12.));
#129452=CARTESIAN_POINT('Ctrl Pts',(11.242344540717,-69.7030217632187,12.));
#129453=CARTESIAN_POINT('Ctrl Pts',(11.2396036366861,-69.7239053175362,
12.));
#129454=CARTESIAN_POINT('Ctrl Pts',(11.236834461247,-69.7448353497394,12.));
#129455=CARTESIAN_POINT('Ctrl Pts',(11.2340369576452,-69.7658116882298,
12.));
#129456=CARTESIAN_POINT('Ctrl Pts',(11.2312110694183,-69.7868341618927,
12.));
#129457=CARTESIAN_POINT('Ctrl Pts',(11.2283567404434,-69.8079026002753,
12.));
#129458=CARTESIAN_POINT('Ctrl Pts',(11.225473914972,-69.8290168337076,12.));
#129459=CARTESIAN_POINT('Ctrl Pts',(11.2225625376739,-69.8501766934445,
12.));
#129460=CARTESIAN_POINT('Ctrl Pts',(11.2196225536794,-69.8713820117918,
12.));
#129461=CARTESIAN_POINT('Ctrl Pts',(11.2166539085527,-69.8926326220414,
12.));
#129462=CARTESIAN_POINT('Ctrl Pts',(11.2136565482679,-69.9139283584036,
12.));
#129463=CARTESIAN_POINT('Ctrl Pts',(11.2106304191881,-69.9352690559399,
12.));
#129464=CARTESIAN_POINT('Ctrl Pts',(11.2075754680445,-69.9566545504813,
12.));
#129465=CARTESIAN_POINT('Ctrl Pts',(11.2044916419239,-69.9780846785771,
12.));
#129466=CARTESIAN_POINT('Ctrl Pts',(11.2013788882711,-69.9995592775322,
12.));
#129467=CARTESIAN_POINT('Ctrl Pts',(11.1982371548918,-70.0210781854236,
12.));
#129468=CARTESIAN_POINT('Ctrl Pts',(11.1950663899578,-70.0426412411194,
12.));
#129469=CARTESIAN_POINT('Ctrl Pts',(11.1918665420168,-70.0642482842942,
12.));
#129470=CARTESIAN_POINT('Ctrl Pts',(11.1886375599916,-70.0858991554295,
12.));
#129471=CARTESIAN_POINT('Ctrl Pts',(11.185379393167,-70.1075936957973,12.));
#129472=CARTESIAN_POINT('Ctrl Pts',(11.1820919911846,-70.1293317474432,
12.));
#129473=CARTESIAN_POINT('Ctrl Pts',(11.1787753040363,-70.1511131531672,
12.));
#129474=CARTESIAN_POINT('Ctrl Pts',(11.1754292820631,-70.1729377564954,
12.));
#129475=CARTESIAN_POINT('Ctrl Pts',(11.1720538759499,-70.1948054016816,
12.));
#129476=CARTESIAN_POINT('Ctrl Pts',(11.168649036721,-70.2167159337094,12.));
#129477=CARTESIAN_POINT('Ctrl Pts',(11.1652147157383,-70.2386691982902,
12.));
#129478=CARTESIAN_POINT('Ctrl Pts',(11.1617508647016,-70.260665041859,12.));
#129479=CARTESIAN_POINT('Ctrl Pts',(11.158257435652,-70.2827033115662,12.));
#129480=CARTESIAN_POINT('Ctrl Pts',(11.1547343809646,-70.3047838552756,
12.));
#129481=CARTESIAN_POINT('Ctrl Pts',(11.1511816533421,-70.326906521559,12.));
#129482=CARTESIAN_POINT('Ctrl Pts',(11.1475992058124,-70.349071159688,12.));
#129483=CARTESIAN_POINT('Ctrl Pts',(11.143986991727,-70.3712776196223,12.));
#129484=CARTESIAN_POINT('Ctrl Pts',(11.1403449647625,-70.393525751996,12.));
#129485=CARTESIAN_POINT('Ctrl Pts',(11.1366730789125,-70.4158154081205,
12.));
#129486=CARTESIAN_POINT('Ctrl Pts',(11.1329712884846,-70.4381464399819,
12.));
#129487=CARTESIAN_POINT('Ctrl Pts',(11.1292395480974,-70.4605187002354,
12.));
#129488=CARTESIAN_POINT('Ctrl Pts',(11.1254778126821,-70.4829320421957,
12.));
#129489=CARTESIAN_POINT('Ctrl Pts',(11.1216860374826,-70.505386319828,12.));
#129490=CARTESIAN_POINT('Ctrl Pts',(11.1178641780476,-70.5278813877494,
12.));
#129491=CARTESIAN_POINT('Ctrl Pts',(11.1140121902271,-70.5504171012234,
12.));
#129492=CARTESIAN_POINT('Ctrl Pts',(11.1101300301701,-70.5729933161546,
12.));
#129493=CARTESIAN_POINT('Ctrl Pts',(11.1062176543262,-70.5956098890773,
12.));
#129494=CARTESIAN_POINT('Ctrl Pts',(11.1022750194445,-70.6182666771481,
12.));
#129495=CARTESIAN_POINT('Ctrl Pts',(11.0983020825667,-70.6409635381482,
12.));
#129496=CARTESIAN_POINT('Ctrl Pts',(11.0942988010233,-70.6637003304785,
12.));
#129497=CARTESIAN_POINT('Ctrl Pts',(11.0902651324323,-70.6864769131546,
12.));
#129498=CARTESIAN_POINT('Ctrl Pts',(11.0862010347016,-70.7092931457954,
12.));
#129499=CARTESIAN_POINT('Ctrl Pts',(11.0821064660269,-70.732148888618,12.));
#129500=CARTESIAN_POINT('Ctrl Pts',(11.0779813848846,-70.7550440024384,
12.));
#129501=CARTESIAN_POINT('Ctrl Pts',(11.073825750029,-70.7779783486677,12.));
#129502=CARTESIAN_POINT('Ctrl Pts',(11.0696395204909,-70.8009517893057,
12.));
#129503=CARTESIAN_POINT('Ctrl Pts',(11.0654226555802,-70.8239641869299,
12.));
#129504=CARTESIAN_POINT('Ctrl Pts',(11.0611751148834,-70.8470154046919,
12.));
#129505=CARTESIAN_POINT('Ctrl Pts',(11.0568968582569,-70.8701053063186,
12.));
#129506=CARTESIAN_POINT('Ctrl Pts',(11.0525878458243,-70.8932337561087,
12.));
#129507=CARTESIAN_POINT('Ctrl Pts',(11.048248037975,-70.916400618927,12.));
#129508=CARTESIAN_POINT('Ctrl Pts',(11.0438773953681,-70.9396057601924,
12.));
#129509=CARTESIAN_POINT('Ctrl Pts',(11.0394758789285,-70.9628490458748,
12.));
#129510=CARTESIAN_POINT('Ctrl Pts',(11.0350434498405,-70.986130342497,12.));
#129511=CARTESIAN_POINT('Ctrl Pts',(11.0305800695456,-71.0094495171292,
12.));
#129512=CARTESIAN_POINT('Ctrl Pts',(11.0260856997415,-71.0328064373856,
12.));
#129513=CARTESIAN_POINT('Ctrl Pts',(11.0215603023856,-71.0562009714136,
12.));
#129514=CARTESIAN_POINT('Ctrl Pts',(11.0170038396915,-71.0796329878907,
12.));
#129515=CARTESIAN_POINT('Ctrl Pts',(11.0124162741224,-71.1031023560249,
12.));
#129516=CARTESIAN_POINT('Ctrl Pts',(11.0077975683895,-71.1266089455517,
12.));
#129517=CARTESIAN_POINT('Ctrl Pts',(11.0031476854502,-71.1501526267286,
12.));
#129518=CARTESIAN_POINT('Ctrl Pts',(10.9984665885127,-71.1737332703248,
12.));
#129519=CARTESIAN_POINT('Ctrl Pts',(10.993754241032,-71.1973507476191,12.));
#129520=CARTESIAN_POINT('Ctrl Pts',(10.9890106067039,-71.2210049304014,
12.));
#129521=CARTESIAN_POINT('Ctrl Pts',(10.9842356494627,-71.2446956909687,
12.));
#129522=CARTESIAN_POINT('Ctrl Pts',(10.9794293334805,-71.2684229021207,
12.));
#129523=CARTESIAN_POINT('Ctrl Pts',(10.9745916231709,-71.2921864371491,
12.));
#129524=CARTESIAN_POINT('Ctrl Pts',(10.969722483186,-71.3159861698358,12.));
#129525=CARTESIAN_POINT('Ctrl Pts',(10.9648218784098,-71.339821974454,12.));
#129526=CARTESIAN_POINT('Ctrl Pts',(10.9598897739564,-71.3636937257649,
12.));
#129527=CARTESIAN_POINT('Ctrl Pts',(10.954926135169,-71.3876012990138,12.));
#129528=CARTESIAN_POINT('Ctrl Pts',(10.9499309276236,-71.4115445699194,
12.));
#129529=CARTESIAN_POINT('Ctrl Pts',(10.944904117127,-71.435523414672,12.));
#129530=CARTESIAN_POINT('Ctrl Pts',(10.9398456697095,-71.4595377099351,
12.));
#129531=CARTESIAN_POINT('Ctrl Pts',(10.9347555516235,-71.4835873328423,
12.));
#129532=CARTESIAN_POINT('Ctrl Pts',(10.9296337293424,-71.5076721609937,
12.));
#129533=CARTESIAN_POINT('Ctrl Pts',(10.9244801695642,-71.5317920724459,
12.));
#129534=CARTESIAN_POINT('Ctrl Pts',(10.91929483921,-71.5559469457091,12.));
#129535=CARTESIAN_POINT('Ctrl Pts',(10.914077705417,-71.5801366597488,12.));
#129536=CARTESIAN_POINT('Ctrl Pts',(10.9088287355365,-71.6043610939835,
12.));
#129537=CARTESIAN_POINT('Ctrl Pts',(10.9035478971328,-71.6286201282812,
12.));
#129538=CARTESIAN_POINT('Ctrl Pts',(10.898235157987,-71.6529136429504,12.));
#129539=CARTESIAN_POINT('Ctrl Pts',(10.8928904860964,-71.6772415187364,
12.));
#129540=CARTESIAN_POINT('Ctrl Pts',(10.8875138496671,-71.7016036368236,
12.));
#129541=CARTESIAN_POINT('Ctrl Pts',(10.882105217112,-71.7259998788328,12.));
#129542=CARTESIAN_POINT('Ctrl Pts',(10.8766645570497,-71.7504301268181,
12.));
#129543=CARTESIAN_POINT('Ctrl Pts',(10.8711918383073,-71.7748942632593,
12.));
#129544=CARTESIAN_POINT('Ctrl Pts',(10.865687029922,-71.7993921710564,12.));
#129545=CARTESIAN_POINT('Ctrl Pts',(10.8601501011332,-71.8239237335331,
12.));
#129546=CARTESIAN_POINT('Ctrl Pts',(10.8545810213799,-71.8484888344339,
12.));
#129547=CARTESIAN_POINT('Ctrl Pts',(10.8489797602997,-71.8730873579224,
12.));
#129548=CARTESIAN_POINT('Ctrl Pts',(10.8433462877311,-71.8977191885725,
12.));
#129549=CARTESIAN_POINT('Ctrl Pts',(10.8376805737159,-71.9223842113625,
12.));
#129550=CARTESIAN_POINT('Ctrl Pts',(10.8319825884918,-71.9470823116785,
12.));
#129551=CARTESIAN_POINT('Ctrl Pts',(10.8262523024897,-71.9718133753127,
12.));
#129552=CARTESIAN_POINT('Ctrl Pts',(10.8204896863328,-71.9965772884619,
12.));
#129553=CARTESIAN_POINT('Ctrl Pts',(10.8146947108375,-72.0213739377223,
12.));
#129554=CARTESIAN_POINT('Ctrl Pts',(10.8088673470184,-72.0462032100815,
12.));
#129555=CARTESIAN_POINT('Ctrl Pts',(10.8030075660808,-72.0710649929202,
12.));
#129556=CARTESIAN_POINT('Ctrl Pts',(10.7971153394166,-72.0959591740114,
12.));
#129557=CARTESIAN_POINT('Ctrl Pts',(10.7911906386027,-72.1208856415171,
12.));
#129558=CARTESIAN_POINT('Ctrl Pts',(10.7852334354016,-72.1458442839834,
12.));
#129559=CARTESIAN_POINT('Ctrl Pts',(10.7792437017662,-72.1708349903305,
12.));
#129560=CARTESIAN_POINT('Ctrl Pts',(10.7732214098344,-72.1958576498558,
12.));
#129561=CARTESIAN_POINT('Ctrl Pts',(10.7671665319255,-72.2209121522366,
12.));
#129562=CARTESIAN_POINT('Ctrl Pts',(10.7610790405385,-72.2459983875296,
12.));
#129563=CARTESIAN_POINT('Ctrl Pts',(10.7549589083535,-72.2711162461681,
12.));
#129564=CARTESIAN_POINT('Ctrl Pts',(10.7488061082367,-72.2962656189556,
12.));
#129565=CARTESIAN_POINT('Ctrl Pts',(10.7426206132375,-72.3214463970641,
12.));
#129566=CARTESIAN_POINT('Ctrl Pts',(10.73640239658,-72.3466584720318,12.));
#129567=CARTESIAN_POINT('Ctrl Pts',(10.7301514316607,-72.3719017357571,
12.));
#129568=CARTESIAN_POINT('Ctrl Pts',(10.7238676920469,-72.3971760804933,
12.));
#129569=CARTESIAN_POINT('Ctrl Pts',(10.7175511514788,-72.4224813988347,
12.));
#129570=CARTESIAN_POINT('Ctrl Pts',(10.7112017838706,-72.4478175837156,
12.));
#129571=CARTESIAN_POINT('Ctrl Pts',(10.7048195633061,-72.4731845284227,
12.));
#129572=CARTESIAN_POINT('Ctrl Pts',(10.6984044640398,-72.4985821266023,
12.));
#129573=CARTESIAN_POINT('Ctrl Pts',(10.691956460499,-72.5240102722664,12.));
#129574=CARTESIAN_POINT('Ctrl Pts',(10.6854755272904,-72.5494688597961,
12.));
#129575=CARTESIAN_POINT('Ctrl Pts',(10.6789616392042,-72.5749577839415,
12.));
#129576=CARTESIAN_POINT('Ctrl Pts',(10.6724147711995,-72.6004769398019,
12.));
#129577=CARTESIAN_POINT('Ctrl Pts',(10.6658348983944,-72.6260262228065,
12.));
#129578=CARTESIAN_POINT('Ctrl Pts',(10.659221996058,-72.651605528691,12.));
#129579=CARTESIAN_POINT('Ctrl Pts',(10.6525760396054,-72.6772147534752,
12.));
#129580=CARTESIAN_POINT('Ctrl Pts',(10.6458970045946,-72.7028537934317,
12.));
#129581=CARTESIAN_POINT('Ctrl Pts',(10.6391848667352,-72.7285225451293,
12.));
#129582=CARTESIAN_POINT('Ctrl Pts',(10.6324396018998,-72.7542209054812,
12.));
#129583=CARTESIAN_POINT('Ctrl Pts',(10.6256611861394,-72.7799487717911,
12.));
#129584=CARTESIAN_POINT('Ctrl Pts',(10.6188495956973,-72.8057060417887,
12.));
#129585=CARTESIAN_POINT('Ctrl Pts',(10.6120048070367,-72.8314926136881,
12.));
#129586=CARTESIAN_POINT('Ctrl Pts',(10.6051267968203,-72.8573083861337,
12.));
#129587=CARTESIAN_POINT('Ctrl Pts',(10.5982155418626,-72.8831532580845,
12.));
#129588=CARTESIAN_POINT('Ctrl Pts',(10.5912710190928,-72.9090271287083,
12.));
#129589=CARTESIAN_POINT('Ctrl Pts',(10.5842932055209,-72.9349298972822,
12.));
#129590=CARTESIAN_POINT('Ctrl Pts',(10.5772820781958,-72.9608614630534,
12.));
#129591=CARTESIAN_POINT('Ctrl Pts',(10.570237614205,-72.9868217252283,12.));
#129592=CARTESIAN_POINT('Ctrl Pts',(10.5631597907651,-73.0128105832621,
12.));
#129593=CARTESIAN_POINT('Ctrl Pts',(10.5560485852974,-73.0388279370834,
12.));
#129594=CARTESIAN_POINT('Ctrl Pts',(10.5489039755138,-73.0648736873434,
12.));
#129595=CARTESIAN_POINT('Ctrl Pts',(10.5417259395002,-73.0909477356474,
12.));
#129596=CARTESIAN_POINT('Ctrl Pts',(10.53451445581,-73.1170499848039,12.));
#129597=CARTESIAN_POINT('Ctrl Pts',(10.5272695032653,-73.1431803382711,
12.));
#129598=CARTESIAN_POINT('Ctrl Pts',(10.5199910607654,-73.1693386996138,
12.));
#129599=CARTESIAN_POINT('Ctrl Pts',(10.5126791070805,-73.1955249719048,
12.));
#129600=CARTESIAN_POINT('Ctrl Pts',(10.5053336206908,-73.2217390572562,
12.));
#129601=CARTESIAN_POINT('Ctrl Pts',(10.4979545795192,-73.2479808560189,
12.));
#129602=CARTESIAN_POINT('Ctrl Pts',(10.4905419611523,-73.2742502674304,
12.));
#129603=CARTESIAN_POINT('Ctrl Pts',(10.4830957433305,-73.3005471910583,
12.));
#129604=CARTESIAN_POINT('Ctrl Pts',(10.4756159043806,-73.3268715280575,
12.));
#129605=CARTESIAN_POINT('Ctrl Pts',(10.4681024236289,-73.3532231823659,
12.));
#129606=CARTESIAN_POINT('Ctrl Pts',(10.4605552819397,-73.37960206225,12.));
#129607=CARTESIAN_POINT('Ctrl Pts',(10.452974461845,-73.4060080806686,12.));
#129608=CARTESIAN_POINT('Ctrl Pts',(10.4464473465479,-73.4286663448107,
12.));
#129609=CARTESIAN_POINT('Ctrl Pts',(10.4414249334739,-73.44605255288,12.));
#129610=CARTESIAN_POINT('Ctrl Pts',(10.4379221501041,-73.4581547436838,
12.));
#129611=CARTESIAN_POINT('Ctrl Pts',(10.4359488742809,-73.4649650361893,
12.));
#129612=CARTESIAN_POINT('Ctrl Pts',(10.4355099267296,-73.4664795929938,
12.));
#129613=CARTESIAN_POINT('',(11.3136138754165,-69.079679653846,0.));
#129614=CARTESIAN_POINT('',(11.3136138754165,-69.079679653846,0.));
#129615=CARTESIAN_POINT('Ctrl Pts',(10.4355099267296,-73.4664795929938,
0.));
#129616=CARTESIAN_POINT('Ctrl Pts',(10.4359488742809,-73.4649650361893,
0.));
#129617=CARTESIAN_POINT('Ctrl Pts',(10.4379221501041,-73.4581547436838,
0.));
#129618=CARTESIAN_POINT('Ctrl Pts',(10.4414249334739,-73.44605255288,0.));
#129619=CARTESIAN_POINT('Ctrl Pts',(10.4464473465479,-73.4286663448107,
0.));
#129620=CARTESIAN_POINT('Ctrl Pts',(10.452974461845,-73.4060080806686,0.));
#129621=CARTESIAN_POINT('Ctrl Pts',(10.4605552819397,-73.37960206225,0.));
#129622=CARTESIAN_POINT('Ctrl Pts',(10.4681024236289,-73.3532231823659,
0.));
#129623=CARTESIAN_POINT('Ctrl Pts',(10.4756159043806,-73.3268715280575,
0.));
#129624=CARTESIAN_POINT('Ctrl Pts',(10.4830957433305,-73.3005471910583,
0.));
#129625=CARTESIAN_POINT('Ctrl Pts',(10.4905419611523,-73.2742502674304,
0.));
#129626=CARTESIAN_POINT('Ctrl Pts',(10.4979545795192,-73.2479808560189,
0.));
#129627=CARTESIAN_POINT('Ctrl Pts',(10.5053336206908,-73.2217390572562,
0.));
#129628=CARTESIAN_POINT('Ctrl Pts',(10.5126791070805,-73.1955249719048,
0.));
#129629=CARTESIAN_POINT('Ctrl Pts',(10.5199910607654,-73.1693386996138,
0.));
#129630=CARTESIAN_POINT('Ctrl Pts',(10.5272695032653,-73.1431803382711,
0.));
#129631=CARTESIAN_POINT('Ctrl Pts',(10.53451445581,-73.1170499848039,0.));
#129632=CARTESIAN_POINT('Ctrl Pts',(10.5417259395002,-73.0909477356474,
0.));
#129633=CARTESIAN_POINT('Ctrl Pts',(10.5489039755138,-73.0648736873434,
0.));
#129634=CARTESIAN_POINT('Ctrl Pts',(10.5560485852974,-73.0388279370834,
0.));
#129635=CARTESIAN_POINT('Ctrl Pts',(10.5631597907651,-73.0128105832621,
0.));
#129636=CARTESIAN_POINT('Ctrl Pts',(10.570237614205,-72.9868217252283,0.));
#129637=CARTESIAN_POINT('Ctrl Pts',(10.5772820781958,-72.9608614630534,
0.));
#129638=CARTESIAN_POINT('Ctrl Pts',(10.5842932055209,-72.9349298972822,
0.));
#129639=CARTESIAN_POINT('Ctrl Pts',(10.5912710190928,-72.9090271287083,
0.));
#129640=CARTESIAN_POINT('Ctrl Pts',(10.5982155418626,-72.8831532580845,
0.));
#129641=CARTESIAN_POINT('Ctrl Pts',(10.6051267968203,-72.8573083861337,
0.));
#129642=CARTESIAN_POINT('Ctrl Pts',(10.6120048070367,-72.8314926136881,
0.));
#129643=CARTESIAN_POINT('Ctrl Pts',(10.6188495956973,-72.8057060417887,
0.));
#129644=CARTESIAN_POINT('Ctrl Pts',(10.6256611861394,-72.7799487717911,
0.));
#129645=CARTESIAN_POINT('Ctrl Pts',(10.6324396018998,-72.7542209054812,
0.));
#129646=CARTESIAN_POINT('Ctrl Pts',(10.6391848667352,-72.7285225451293,
0.));
#129647=CARTESIAN_POINT('Ctrl Pts',(10.6458970045946,-72.7028537934317,
0.));
#129648=CARTESIAN_POINT('Ctrl Pts',(10.6525760396054,-72.6772147534752,
0.));
#129649=CARTESIAN_POINT('Ctrl Pts',(10.659221996058,-72.651605528691,0.));
#129650=CARTESIAN_POINT('Ctrl Pts',(10.6658348983944,-72.6260262228065,
0.));
#129651=CARTESIAN_POINT('Ctrl Pts',(10.6724147711995,-72.6004769398019,
0.));
#129652=CARTESIAN_POINT('Ctrl Pts',(10.6789616392042,-72.5749577839415,
0.));
#129653=CARTESIAN_POINT('Ctrl Pts',(10.6854755272904,-72.5494688597961,
0.));
#129654=CARTESIAN_POINT('Ctrl Pts',(10.691956460499,-72.5240102722664,0.));
#129655=CARTESIAN_POINT('Ctrl Pts',(10.6984044640398,-72.4985821266023,
0.));
#129656=CARTESIAN_POINT('Ctrl Pts',(10.7048195633061,-72.4731845284227,
0.));
#129657=CARTESIAN_POINT('Ctrl Pts',(10.7112017838706,-72.4478175837156,
0.));
#129658=CARTESIAN_POINT('Ctrl Pts',(10.7175511514788,-72.4224813988347,
0.));
#129659=CARTESIAN_POINT('Ctrl Pts',(10.7238676920469,-72.3971760804933,
0.));
#129660=CARTESIAN_POINT('Ctrl Pts',(10.7301514316607,-72.3719017357571,
0.));
#129661=CARTESIAN_POINT('Ctrl Pts',(10.73640239658,-72.3466584720318,0.));
#129662=CARTESIAN_POINT('Ctrl Pts',(10.7426206132375,-72.3214463970641,
0.));
#129663=CARTESIAN_POINT('Ctrl Pts',(10.7488061082367,-72.2962656189556,
0.));
#129664=CARTESIAN_POINT('Ctrl Pts',(10.7549589083535,-72.2711162461681,
0.));
#129665=CARTESIAN_POINT('Ctrl Pts',(10.7610790405385,-72.2459983875296,
0.));
#129666=CARTESIAN_POINT('Ctrl Pts',(10.7671665319255,-72.2209121522366,
0.));
#129667=CARTESIAN_POINT('Ctrl Pts',(10.7732214098344,-72.1958576498558,
0.));
#129668=CARTESIAN_POINT('Ctrl Pts',(10.7792437017662,-72.1708349903305,
0.));
#129669=CARTESIAN_POINT('Ctrl Pts',(10.7852334354016,-72.1458442839834,
0.));
#129670=CARTESIAN_POINT('Ctrl Pts',(10.7911906386027,-72.1208856415171,
0.));
#129671=CARTESIAN_POINT('Ctrl Pts',(10.7971153394166,-72.0959591740114,
0.));
#129672=CARTESIAN_POINT('Ctrl Pts',(10.8030075660808,-72.0710649929202,
0.));
#129673=CARTESIAN_POINT('Ctrl Pts',(10.8088673470184,-72.0462032100815,
0.));
#129674=CARTESIAN_POINT('Ctrl Pts',(10.8146947108375,-72.0213739377223,
0.));
#129675=CARTESIAN_POINT('Ctrl Pts',(10.8204896863328,-71.9965772884619,
0.));
#129676=CARTESIAN_POINT('Ctrl Pts',(10.8262523024897,-71.9718133753127,
0.));
#129677=CARTESIAN_POINT('Ctrl Pts',(10.8319825884918,-71.9470823116785,
0.));
#129678=CARTESIAN_POINT('Ctrl Pts',(10.8376805737159,-71.9223842113625,
0.));
#129679=CARTESIAN_POINT('Ctrl Pts',(10.8433462877311,-71.8977191885725,
0.));
#129680=CARTESIAN_POINT('Ctrl Pts',(10.8489797602997,-71.8730873579224,
0.));
#129681=CARTESIAN_POINT('Ctrl Pts',(10.8545810213799,-71.8484888344339,
0.));
#129682=CARTESIAN_POINT('Ctrl Pts',(10.8601501011332,-71.8239237335331,
0.));
#129683=CARTESIAN_POINT('Ctrl Pts',(10.865687029922,-71.7993921710564,0.));
#129684=CARTESIAN_POINT('Ctrl Pts',(10.8711918383073,-71.7748942632593,
0.));
#129685=CARTESIAN_POINT('Ctrl Pts',(10.8766645570497,-71.7504301268181,
0.));
#129686=CARTESIAN_POINT('Ctrl Pts',(10.882105217112,-71.7259998788328,0.));
#129687=CARTESIAN_POINT('Ctrl Pts',(10.8875138496671,-71.7016036368236,
0.));
#129688=CARTESIAN_POINT('Ctrl Pts',(10.8928904860964,-71.6772415187364,
0.));
#129689=CARTESIAN_POINT('Ctrl Pts',(10.898235157987,-71.6529136429504,0.));
#129690=CARTESIAN_POINT('Ctrl Pts',(10.9035478971328,-71.6286201282812,
0.));
#129691=CARTESIAN_POINT('Ctrl Pts',(10.9088287355365,-71.6043610939835,
0.));
#129692=CARTESIAN_POINT('Ctrl Pts',(10.914077705417,-71.5801366597488,0.));
#129693=CARTESIAN_POINT('Ctrl Pts',(10.91929483921,-71.5559469457091,0.));
#129694=CARTESIAN_POINT('Ctrl Pts',(10.9244801695642,-71.5317920724459,
0.));
#129695=CARTESIAN_POINT('Ctrl Pts',(10.9296337293424,-71.5076721609937,
0.));
#129696=CARTESIAN_POINT('Ctrl Pts',(10.9347555516235,-71.4835873328423,
0.));
#129697=CARTESIAN_POINT('Ctrl Pts',(10.9398456697095,-71.4595377099351,
0.));
#129698=CARTESIAN_POINT('Ctrl Pts',(10.944904117127,-71.435523414672,0.));
#129699=CARTESIAN_POINT('Ctrl Pts',(10.9499309276236,-71.4115445699194,
0.));
#129700=CARTESIAN_POINT('Ctrl Pts',(10.954926135169,-71.3876012990138,0.));
#129701=CARTESIAN_POINT('Ctrl Pts',(10.9598897739564,-71.3636937257649,
0.));
#129702=CARTESIAN_POINT('Ctrl Pts',(10.9648218784098,-71.339821974454,0.));
#129703=CARTESIAN_POINT('Ctrl Pts',(10.969722483186,-71.3159861698358,0.));
#129704=CARTESIAN_POINT('Ctrl Pts',(10.9745916231709,-71.2921864371491,
0.));
#129705=CARTESIAN_POINT('Ctrl Pts',(10.9794293334805,-71.2684229021207,
0.));
#129706=CARTESIAN_POINT('Ctrl Pts',(10.9842356494627,-71.2446956909687,
0.));
#129707=CARTESIAN_POINT('Ctrl Pts',(10.9890106067039,-71.2210049304014,
0.));
#129708=CARTESIAN_POINT('Ctrl Pts',(10.993754241032,-71.1973507476191,0.));
#129709=CARTESIAN_POINT('Ctrl Pts',(10.9984665885127,-71.1737332703248,
0.));
#129710=CARTESIAN_POINT('Ctrl Pts',(11.0031476854502,-71.1501526267286,
0.));
#129711=CARTESIAN_POINT('Ctrl Pts',(11.0077975683895,-71.1266089455517,
0.));
#129712=CARTESIAN_POINT('Ctrl Pts',(11.0124162741224,-71.1031023560249,
0.));
#129713=CARTESIAN_POINT('Ctrl Pts',(11.0170038396915,-71.0796329878907,
0.));
#129714=CARTESIAN_POINT('Ctrl Pts',(11.0215603023856,-71.0562009714136,
0.));
#129715=CARTESIAN_POINT('Ctrl Pts',(11.0260856997415,-71.0328064373856,
0.));
#129716=CARTESIAN_POINT('Ctrl Pts',(11.0305800695456,-71.0094495171292,
0.));
#129717=CARTESIAN_POINT('Ctrl Pts',(11.0350434498405,-70.986130342497,0.));
#129718=CARTESIAN_POINT('Ctrl Pts',(11.0394758789285,-70.9628490458748,
0.));
#129719=CARTESIAN_POINT('Ctrl Pts',(11.0438773953681,-70.9396057601924,
0.));
#129720=CARTESIAN_POINT('Ctrl Pts',(11.048248037975,-70.916400618927,0.));
#129721=CARTESIAN_POINT('Ctrl Pts',(11.0525878458243,-70.8932337561087,
0.));
#129722=CARTESIAN_POINT('Ctrl Pts',(11.0568968582569,-70.8701053063186,
0.));
#129723=CARTESIAN_POINT('Ctrl Pts',(11.0611751148834,-70.8470154046919,
0.));
#129724=CARTESIAN_POINT('Ctrl Pts',(11.0654226555802,-70.8239641869299,
0.));
#129725=CARTESIAN_POINT('Ctrl Pts',(11.0696395204909,-70.8009517893057,
0.));
#129726=CARTESIAN_POINT('Ctrl Pts',(11.073825750029,-70.7779783486677,0.));
#129727=CARTESIAN_POINT('Ctrl Pts',(11.0779813848846,-70.7550440024384,
0.));
#129728=CARTESIAN_POINT('Ctrl Pts',(11.0821064660269,-70.732148888618,0.));
#129729=CARTESIAN_POINT('Ctrl Pts',(11.0862010347016,-70.7092931457954,
0.));
#129730=CARTESIAN_POINT('Ctrl Pts',(11.0902651324323,-70.6864769131546,
0.));
#129731=CARTESIAN_POINT('Ctrl Pts',(11.0942988010233,-70.6637003304785,
0.));
#129732=CARTESIAN_POINT('Ctrl Pts',(11.0983020825667,-70.6409635381482,
0.));
#129733=CARTESIAN_POINT('Ctrl Pts',(11.1022750194445,-70.6182666771481,
0.));
#129734=CARTESIAN_POINT('Ctrl Pts',(11.1062176543262,-70.5956098890773,
0.));
#129735=CARTESIAN_POINT('Ctrl Pts',(11.1101300301701,-70.5729933161546,
0.));
#129736=CARTESIAN_POINT('Ctrl Pts',(11.1140121902271,-70.5504171012234,
0.));
#129737=CARTESIAN_POINT('Ctrl Pts',(11.1178641780476,-70.5278813877494,
0.));
#129738=CARTESIAN_POINT('Ctrl Pts',(11.1216860374826,-70.505386319828,0.));
#129739=CARTESIAN_POINT('Ctrl Pts',(11.1254778126821,-70.4829320421957,
0.));
#129740=CARTESIAN_POINT('Ctrl Pts',(11.1292395480974,-70.4605187002354,
0.));
#129741=CARTESIAN_POINT('Ctrl Pts',(11.1329712884846,-70.4381464399819,
0.));
#129742=CARTESIAN_POINT('Ctrl Pts',(11.1366730789125,-70.4158154081205,
0.));
#129743=CARTESIAN_POINT('Ctrl Pts',(11.1403449647625,-70.393525751996,0.));
#129744=CARTESIAN_POINT('Ctrl Pts',(11.143986991727,-70.3712776196223,0.));
#129745=CARTESIAN_POINT('Ctrl Pts',(11.1475992058124,-70.349071159688,0.));
#129746=CARTESIAN_POINT('Ctrl Pts',(11.1511816533421,-70.326906521559,0.));
#129747=CARTESIAN_POINT('Ctrl Pts',(11.1547343809646,-70.3047838552756,
0.));
#129748=CARTESIAN_POINT('Ctrl Pts',(11.158257435652,-70.2827033115662,0.));
#129749=CARTESIAN_POINT('Ctrl Pts',(11.1617508647016,-70.260665041859,0.));
#129750=CARTESIAN_POINT('Ctrl Pts',(11.1652147157383,-70.2386691982902,
0.));
#129751=CARTESIAN_POINT('Ctrl Pts',(11.168649036721,-70.2167159337094,0.));
#129752=CARTESIAN_POINT('Ctrl Pts',(11.1720538759499,-70.1948054016816,
0.));
#129753=CARTESIAN_POINT('Ctrl Pts',(11.1754292820631,-70.1729377564954,
0.));
#129754=CARTESIAN_POINT('Ctrl Pts',(11.1787753040363,-70.1511131531672,
0.));
#129755=CARTESIAN_POINT('Ctrl Pts',(11.1820919911846,-70.1293317474432,
0.));
#129756=CARTESIAN_POINT('Ctrl Pts',(11.185379393167,-70.1075936957973,0.));
#129757=CARTESIAN_POINT('Ctrl Pts',(11.1886375599916,-70.0858991554295,
0.));
#129758=CARTESIAN_POINT('Ctrl Pts',(11.1918665420168,-70.0642482842942,
0.));
#129759=CARTESIAN_POINT('Ctrl Pts',(11.1950663899578,-70.0426412411194,
0.));
#129760=CARTESIAN_POINT('Ctrl Pts',(11.1982371548918,-70.0210781854236,
0.));
#129761=CARTESIAN_POINT('Ctrl Pts',(11.2013788882711,-69.9995592775322,
0.));
#129762=CARTESIAN_POINT('Ctrl Pts',(11.2044916419239,-69.9780846785771,
0.));
#129763=CARTESIAN_POINT('Ctrl Pts',(11.2075754680445,-69.9566545504813,
0.));
#129764=CARTESIAN_POINT('Ctrl Pts',(11.2106304191881,-69.9352690559399,
0.));
#129765=CARTESIAN_POINT('Ctrl Pts',(11.2136565482679,-69.9139283584036,
0.));
#129766=CARTESIAN_POINT('Ctrl Pts',(11.2166539085527,-69.8926326220414,
0.));
#129767=CARTESIAN_POINT('Ctrl Pts',(11.2196225536794,-69.8713820117918,
0.));
#129768=CARTESIAN_POINT('Ctrl Pts',(11.2225625376739,-69.8501766934445,
0.));
#129769=CARTESIAN_POINT('Ctrl Pts',(11.225473914972,-69.8290168337076,0.));
#129770=CARTESIAN_POINT('Ctrl Pts',(11.2283567404434,-69.8079026002753,
0.));
#129771=CARTESIAN_POINT('Ctrl Pts',(11.2312110694183,-69.7868341618927,
0.));
#129772=CARTESIAN_POINT('Ctrl Pts',(11.2340369576452,-69.7658116882298,
0.));
#129773=CARTESIAN_POINT('Ctrl Pts',(11.236834461247,-69.7448353497394,0.));
#129774=CARTESIAN_POINT('Ctrl Pts',(11.2396036366861,-69.7239053175362,
0.));
#129775=CARTESIAN_POINT('Ctrl Pts',(11.242344540717,-69.7030217632187,0.));
#129776=CARTESIAN_POINT('Ctrl Pts',(11.2450572303847,-69.6821848588492,
0.));
#129777=CARTESIAN_POINT('Ctrl Pts',(11.247741763139,-69.6613947773563,0.));
#129778=CARTESIAN_POINT('Ctrl Pts',(11.2503981969413,-69.6406516928902,
0.));
#129779=CARTESIAN_POINT('Ctrl Pts',(11.2530265903555,-69.6199557811231,
0.));
#129780=CARTESIAN_POINT('Ctrl Pts',(11.255627002701,-69.5993072197355,0.));
#129781=CARTESIAN_POINT('Ctrl Pts',(11.2581994939534,-69.5787061880815,
0.));
#129782=CARTESIAN_POINT('Ctrl Pts',(11.2607441244697,-69.5581528662846,
0.));
#129783=CARTESIAN_POINT('Ctrl Pts',(11.2632609547629,-69.5376474344768,
0.));
#129784=CARTESIAN_POINT('Ctrl Pts',(11.265750045272,-69.5171900720188,0.));
#129785=CARTESIAN_POINT('Ctrl Pts',(11.2682114561015,-69.4967809565978,
0.));
#129786=CARTESIAN_POINT('Ctrl Pts',(11.2706452475287,-69.4764202659443,
0.));
#129787=CARTESIAN_POINT('Ctrl Pts',(11.2730514806143,-69.4561081798815,
0.));
#129788=CARTESIAN_POINT('Ctrl Pts',(11.2754302177019,-69.4358448819957,
0.));
#129789=CARTESIAN_POINT('Ctrl Pts',(11.2777815231462,-69.4156305620554,
0.));
#129790=CARTESIAN_POINT('Ctrl Pts',(11.2801054633807,-69.395465416223,0.));
#129791=CARTESIAN_POINT('Ctrl Pts',(11.2824021054038,-69.375349642,0.));
#129792=CARTESIAN_POINT('Ctrl Pts',(11.2846715154521,-69.3552834337771,
0.));
#129793=CARTESIAN_POINT('Ctrl Pts',(11.2869137578463,-69.3352669789611,
0.));
#129794=CARTESIAN_POINT('Ctrl Pts',(11.2891288931528,-69.315300451784,0.));
#129795=CARTESIAN_POINT('Ctrl Pts',(11.2913169799642,-69.2953840192792,
0.));
#129796=CARTESIAN_POINT('Ctrl Pts',(11.2934780784361,-69.2755178531534,
0.));
#129797=CARTESIAN_POINT('Ctrl Pts',(11.2956122531375,-69.255702139335,0.));
#129798=CARTESIAN_POINT('Ctrl Pts',(11.2977195764836,-69.2359370894828,
0.));
#129799=CARTESIAN_POINT('Ctrl Pts',(11.2998001310934,-69.216222948839,0.));
#129800=CARTESIAN_POINT('Ctrl Pts',(11.3018540025605,-69.1965599718761,
0.));
#129801=CARTESIAN_POINT('Ctrl Pts',(11.3038812726275,-69.1769483991639,
0.));
#129802=CARTESIAN_POINT('Ctrl Pts',(11.3058820128323,-69.1573884361076,
0.));
#129803=CARTESIAN_POINT('Ctrl Pts',(11.3078562764442,-69.137880225198,0.));
#129804=CARTESIAN_POINT('Ctrl Pts',(11.3098040973799,-69.1184238445065,
0.));
#129805=CARTESIAN_POINT('Ctrl Pts',(11.3113412156741,-69.1029002322497,
0.));
#129806=CARTESIAN_POINT('Ctrl Pts',(11.3124821678849,-69.0912808657051,
0.));
#129807=CARTESIAN_POINT('Ctrl Pts',(11.3132375200184,-69.0835449954486,
0.));
#129808=CARTESIAN_POINT('Ctrl Pts',(11.3136138754165,-69.079679653846,0.));
#129809=CARTESIAN_POINT('Ctrl Pts',(3.87370827955543,-74.3992230078037,
0.));
#129810=CARTESIAN_POINT('Ctrl Pts',(3.87370827955543,-74.3992230078037,
12.));
#129811=CARTESIAN_POINT('Ctrl Pts',(3.87578335377324,-74.3940262116388,
0.));
#129812=CARTESIAN_POINT('Ctrl Pts',(3.87578335377324,-74.3940262116388,
12.));
#129813=CARTESIAN_POINT('Ctrl Pts',(3.87992989995746,-74.3836349189184,
0.));
#129814=CARTESIAN_POINT('Ctrl Pts',(3.87992989995746,-74.3836349189184,
12.));
#129815=CARTESIAN_POINT('Ctrl Pts',(3.88613891247983,-74.3680548786661,
0.));
#129816=CARTESIAN_POINT('Ctrl Pts',(3.88613891247983,-74.3680548786661,
12.));
#129817=CARTESIAN_POINT('Ctrl Pts',(3.89439598145328,-74.3472952898745,
0.));
#129818=CARTESIAN_POINT('Ctrl Pts',(3.89439598145328,-74.3472952898745,
12.));
#129819=CARTESIAN_POINT('Ctrl Pts',(3.90468128904633,-74.3213688090134,
0.));
#129820=CARTESIAN_POINT('Ctrl Pts',(3.90468128904633,-74.3213688090134,
12.));
#129821=CARTESIAN_POINT('Ctrl Pts',(3.9149305628503,-74.2954653518728,0.));
#129822=CARTESIAN_POINT('Ctrl Pts',(3.9149305628503,-74.2954653518728,12.));
#129823=CARTESIAN_POINT('Ctrl Pts',(3.92514379920743,-74.2695849516226,
0.));
#129824=CARTESIAN_POINT('Ctrl Pts',(3.92514379920743,-74.2695849516226,
12.));
#129825=CARTESIAN_POINT('Ctrl Pts',(3.93532099774203,-74.2437276593623,
0.));
#129826=CARTESIAN_POINT('Ctrl Pts',(3.93532099774203,-74.2437276593623,
12.));
#129827=CARTESIAN_POINT('Ctrl Pts',(3.9454621637745,-74.2178935492876,0.));
#129828=CARTESIAN_POINT('Ctrl Pts',(3.9454621637745,-74.2178935492876,12.));
#129829=CARTESIAN_POINT('Ctrl Pts',(3.9555673082111,-74.1920827166585,0.));
#129830=CARTESIAN_POINT('Ctrl Pts',(3.9555673082111,-74.1920827166585,12.));
#129831=CARTESIAN_POINT('Ctrl Pts',(3.96563644549385,-74.1662952702485,
0.));
#129832=CARTESIAN_POINT('Ctrl Pts',(3.96563644549385,-74.1662952702485,
12.));
#129833=CARTESIAN_POINT('Ctrl Pts',(3.97566959209528,-74.1405313263109,
0.));
#129834=CARTESIAN_POINT('Ctrl Pts',(3.97566959209528,-74.1405313263109,
12.));
#129835=CARTESIAN_POINT('Ctrl Pts',(3.98566676483641,-74.1147910020891,
0.));
#129836=CARTESIAN_POINT('Ctrl Pts',(3.98566676483641,-74.1147910020891,
12.));
#129837=CARTESIAN_POINT('Ctrl Pts',(3.99562797918286,-74.0890744091186,
0.));
#129838=CARTESIAN_POINT('Ctrl Pts',(3.99562797918286,-74.0890744091186,
12.));
#129839=CARTESIAN_POINT('Ctrl Pts',(4.00555324785479,-74.0633816478037,
0.));
#129840=CARTESIAN_POINT('Ctrl Pts',(4.00555324785479,-74.0633816478037,
12.));
#129841=CARTESIAN_POINT('Ctrl Pts',(4.0154425817671,-74.0377128111863,0.));
#129842=CARTESIAN_POINT('Ctrl Pts',(4.0154425817671,-74.0377128111863,12.));
#129843=CARTESIAN_POINT('Ctrl Pts',(4.02529599070094,-74.012067987646,0.));
#129844=CARTESIAN_POINT('Ctrl Pts',(4.02529599070094,-74.012067987646,12.));
#129845=CARTESIAN_POINT('Ctrl Pts',(4.03511348410659,-73.9864472641033,
0.));
#129846=CARTESIAN_POINT('Ctrl Pts',(4.03511348410659,-73.9864472641033,
12.));
#129847=CARTESIAN_POINT('Ctrl Pts',(4.04489507179957,-73.9608507287909,
0.));
#129848=CARTESIAN_POINT('Ctrl Pts',(4.04489507179957,-73.9608507287909,
12.));
#129849=CARTESIAN_POINT('Ctrl Pts',(4.05464076484751,-73.9352784747608,
0.));
#129850=CARTESIAN_POINT('Ctrl Pts',(4.05464076484751,-73.9352784747608,
12.));
#129851=CARTESIAN_POINT('Ctrl Pts',(4.06435057547324,-73.9097305995115,
0.));
#129852=CARTESIAN_POINT('Ctrl Pts',(4.06435057547324,-73.9097305995115,
12.));
#129853=CARTESIAN_POINT('Ctrl Pts',(4.07402451665244,-73.8842072034008,
0.));
#129854=CARTESIAN_POINT('Ctrl Pts',(4.07402451665244,-73.8842072034008,
12.));
#129855=CARTESIAN_POINT('Ctrl Pts',(4.08366260180674,-73.8587083884191,
0.));
#129856=CARTESIAN_POINT('Ctrl Pts',(4.08366260180674,-73.8587083884191,
12.));
#129857=CARTESIAN_POINT('Ctrl Pts',(4.09326484448232,-73.8332342568989,
0.));
#129858=CARTESIAN_POINT('Ctrl Pts',(4.09326484448232,-73.8332342568989,
12.));
#129859=CARTESIAN_POINT('Ctrl Pts',(4.10283125798728,-73.8077849100342,
0.));
#129860=CARTESIAN_POINT('Ctrl Pts',(4.10283125798728,-73.8077849100342,
12.));
#129861=CARTESIAN_POINT('Ctrl Pts',(4.11236185522786,-73.7823604472159,
0.));
#129862=CARTESIAN_POINT('Ctrl Pts',(4.11236185522786,-73.7823604472159,
12.));
#129863=CARTESIAN_POINT('Ctrl Pts',(4.12185664890556,-73.7569609668528,
0.));
#129864=CARTESIAN_POINT('Ctrl Pts',(4.12185664890556,-73.7569609668528,
12.));
#129865=CARTESIAN_POINT('Ctrl Pts',(4.13131565163577,-73.7315865668522,
0.));
#129866=CARTESIAN_POINT('Ctrl Pts',(4.13131565163577,-73.7315865668522,
12.));
#129867=CARTESIAN_POINT('Ctrl Pts',(4.14073887610152,-73.7062373452342,
0.));
#129868=CARTESIAN_POINT('Ctrl Pts',(4.14073887610152,-73.7062373452342,
12.));
#129869=CARTESIAN_POINT('Ctrl Pts',(4.15012633519722,-73.6809134006897,
0.));
#129870=CARTESIAN_POINT('Ctrl Pts',(4.15012633519722,-73.6809134006897,
12.));
#129871=CARTESIAN_POINT('Ctrl Pts',(4.15947804217783,-73.6556148331489,
0.));
#129872=CARTESIAN_POINT('Ctrl Pts',(4.15947804217783,-73.6556148331489,
12.));
#129873=CARTESIAN_POINT('Ctrl Pts',(4.1687940105878,-73.6303417435251,0.));
#129874=CARTESIAN_POINT('Ctrl Pts',(4.1687940105878,-73.6303417435251,12.));
#129875=CARTESIAN_POINT('Ctrl Pts',(4.17807425419812,-73.6050942334768,
0.));
#129876=CARTESIAN_POINT('Ctrl Pts',(4.17807425419812,-73.6050942334768,
12.));
#129877=CARTESIAN_POINT('Ctrl Pts',(4.18731878694235,-73.5798724051519,
0.));
#129878=CARTESIAN_POINT('Ctrl Pts',(4.18731878694235,-73.5798724051519,
12.));
#129879=CARTESIAN_POINT('Ctrl Pts',(4.19652762286126,-73.5546763609572,
0.));
#129880=CARTESIAN_POINT('Ctrl Pts',(4.19652762286126,-73.5546763609572,
12.));
#129881=CARTESIAN_POINT('Ctrl Pts',(4.20570077603729,-73.5295062032628,
0.));
#129882=CARTESIAN_POINT('Ctrl Pts',(4.20570077603729,-73.5295062032628,
12.));
#129883=CARTESIAN_POINT('Ctrl Pts',(4.2148382605944,-73.5043620344116,0.));
#129884=CARTESIAN_POINT('Ctrl Pts',(4.2148382605944,-73.5043620344116,12.));
#129885=CARTESIAN_POINT('Ctrl Pts',(4.22394009072755,-73.4792439568633,
0.));
#129886=CARTESIAN_POINT('Ctrl Pts',(4.22394009072755,-73.4792439568633,
12.));
#129887=CARTESIAN_POINT('Ctrl Pts',(4.23300628072757,-73.4541520732948,
0.));
#129888=CARTESIAN_POINT('Ctrl Pts',(4.23300628072757,-73.4541520732948,
12.));
#129889=CARTESIAN_POINT('Ctrl Pts',(4.24203684500938,-73.4290864867101,
0.));
#129890=CARTESIAN_POINT('Ctrl Pts',(4.24203684500938,-73.4290864867101,
12.));
#129891=CARTESIAN_POINT('Ctrl Pts',(4.25103179814886,-73.4040473005592,
0.));
#129892=CARTESIAN_POINT('Ctrl Pts',(4.25103179814886,-73.4040473005592,
12.));
#129893=CARTESIAN_POINT('Ctrl Pts',(4.25999115489898,-73.3790346187938,
0.));
#129894=CARTESIAN_POINT('Ctrl Pts',(4.25999115489898,-73.3790346187938,
12.));
#129895=CARTESIAN_POINT('Ctrl Pts',(4.26891493016699,-73.3540485458065,
0.));
#129896=CARTESIAN_POINT('Ctrl Pts',(4.26891493016699,-73.3540485458065,
12.));
#129897=CARTESIAN_POINT('Ctrl Pts',(4.27780313900389,-73.3290891863949,
0.));
#129898=CARTESIAN_POINT('Ctrl Pts',(4.27780313900389,-73.3290891863949,
12.));
#129899=CARTESIAN_POINT('Ctrl Pts',(4.286655796593,-73.3041566457135,0.));
#129900=CARTESIAN_POINT('Ctrl Pts',(4.286655796593,-73.3041566457135,12.));
#129901=CARTESIAN_POINT('Ctrl Pts',(4.29547291824286,-73.2792510292254,
0.));
#129902=CARTESIAN_POINT('Ctrl Pts',(4.29547291824286,-73.2792510292254,
12.));
#129903=CARTESIAN_POINT('Ctrl Pts',(4.30425451938229,-73.2543724426577,
0.));
#129904=CARTESIAN_POINT('Ctrl Pts',(4.30425451938229,-73.2543724426577,
12.));
#129905=CARTESIAN_POINT('Ctrl Pts',(4.31300061556097,-73.2295209920334,
0.));
#129906=CARTESIAN_POINT('Ctrl Pts',(4.31300061556097,-73.2295209920334,
12.));
#129907=CARTESIAN_POINT('Ctrl Pts',(4.32171122245213,-73.204696783694,0.));
#129908=CARTESIAN_POINT('Ctrl Pts',(4.32171122245213,-73.204696783694,12.));
#129909=CARTESIAN_POINT('Ctrl Pts',(4.33038635585876,-73.1798999243235,
0.));
#129910=CARTESIAN_POINT('Ctrl Pts',(4.33038635585876,-73.1798999243235,
12.));
#129911=CARTESIAN_POINT('Ctrl Pts',(4.3390260317214,-73.1551305209685,0.));
#129912=CARTESIAN_POINT('Ctrl Pts',(4.3390260317214,-73.1551305209685,12.));
#129913=CARTESIAN_POINT('Ctrl Pts',(4.34763026613157,-73.130388681059,0.));
#129914=CARTESIAN_POINT('Ctrl Pts',(4.34763026613157,-73.130388681059,12.));
#129915=CARTESIAN_POINT('Ctrl Pts',(4.35619907532719,-73.1056745124087,
0.));
#129916=CARTESIAN_POINT('Ctrl Pts',(4.35619907532719,-73.1056745124087,
12.));
#129917=CARTESIAN_POINT('Ctrl Pts',(4.3647324756864,-73.0809881232103,0.));
#129918=CARTESIAN_POINT('Ctrl Pts',(4.3647324756864,-73.0809881232103,12.));
#129919=CARTESIAN_POINT('Ctrl Pts',(4.37323048372606,-73.0563296220299,
0.));
#129920=CARTESIAN_POINT('Ctrl Pts',(4.37323048372606,-73.0563296220299,
12.));
#129921=CARTESIAN_POINT('Ctrl Pts',(4.3816931161015,-73.0316991177993,0.));
#129922=CARTESIAN_POINT('Ctrl Pts',(4.3816931161015,-73.0316991177993,12.));
#129923=CARTESIAN_POINT('Ctrl Pts',(4.39012038961138,-73.007096719804,0.));
#129924=CARTESIAN_POINT('Ctrl Pts',(4.39012038961138,-73.007096719804,12.));
#129925=CARTESIAN_POINT('Ctrl Pts',(4.39851232119721,-72.9825225376847,
0.));
#129926=CARTESIAN_POINT('Ctrl Pts',(4.39851232119721,-72.9825225376847,
12.));
#129927=CARTESIAN_POINT('Ctrl Pts',(4.40686892793957,-72.95797668145,0.));
#129928=CARTESIAN_POINT('Ctrl Pts',(4.40686892793957,-72.95797668145,12.));
#129929=CARTESIAN_POINT('Ctrl Pts',(4.41519022705921,-72.9334592614829,
0.));
#129930=CARTESIAN_POINT('Ctrl Pts',(4.41519022705921,-72.9334592614829,
12.));
#129931=CARTESIAN_POINT('Ctrl Pts',(4.42347623591941,-72.9089703885462,
0.));
#129932=CARTESIAN_POINT('Ctrl Pts',(4.42347623591941,-72.9089703885462,
12.));
#129933=CARTESIAN_POINT('Ctrl Pts',(4.43172697203349,-72.8845101737855,
0.));
#129934=CARTESIAN_POINT('Ctrl Pts',(4.43172697203349,-72.8845101737855,
12.));
#129935=CARTESIAN_POINT('Ctrl Pts',(4.43994245306817,-72.8600787287318,
0.));
#129936=CARTESIAN_POINT('Ctrl Pts',(4.43994245306817,-72.8600787287318,
12.));
#129937=CARTESIAN_POINT('Ctrl Pts',(4.44812269683737,-72.8356761653069,
0.));
#129938=CARTESIAN_POINT('Ctrl Pts',(4.44812269683737,-72.8356761653069,
12.));
#129939=CARTESIAN_POINT('Ctrl Pts',(4.45626772130145,-72.8113025958262,
0.));
#129940=CARTESIAN_POINT('Ctrl Pts',(4.45626772130145,-72.8113025958262,
12.));
#129941=CARTESIAN_POINT('Ctrl Pts',(4.46437754456792,-72.7869581329994,
0.));
#129942=CARTESIAN_POINT('Ctrl Pts',(4.46437754456792,-72.7869581329994,
12.));
#129943=CARTESIAN_POINT('Ctrl Pts',(4.47245218489609,-72.7626428899281,
0.));
#129944=CARTESIAN_POINT('Ctrl Pts',(4.47245218489609,-72.7626428899281,
12.));
#129945=CARTESIAN_POINT('Ctrl Pts',(4.48049166070205,-72.738356980103,0.));
#129946=CARTESIAN_POINT('Ctrl Pts',(4.48049166070205,-72.738356980103,12.));
#129947=CARTESIAN_POINT('Ctrl Pts',(4.48849599055337,-72.714100517414,0.));
#129948=CARTESIAN_POINT('Ctrl Pts',(4.48849599055337,-72.714100517414,12.));
#129949=CARTESIAN_POINT('Ctrl Pts',(4.49646519316812,-72.6898736161542,
0.));
#129950=CARTESIAN_POINT('Ctrl Pts',(4.49646519316812,-72.6898736161542,
12.));
#129951=CARTESIAN_POINT('Ctrl Pts',(4.50439928741603,-72.6656763910241,
0.));
#129952=CARTESIAN_POINT('Ctrl Pts',(4.50439928741603,-72.6656763910241,
12.));
#129953=CARTESIAN_POINT('Ctrl Pts',(4.51229829232263,-72.6415089571321,
0.));
#129954=CARTESIAN_POINT('Ctrl Pts',(4.51229829232263,-72.6415089571321,
12.));
#129955=CARTESIAN_POINT('Ctrl Pts',(4.52016222707637,-72.6173714299942,
0.));
#129956=CARTESIAN_POINT('Ctrl Pts',(4.52016222707637,-72.6173714299942,
12.));
#129957=CARTESIAN_POINT('Ctrl Pts',(4.52799111102391,-72.5932639255409,
0.));
#129958=CARTESIAN_POINT('Ctrl Pts',(4.52799111102391,-72.5932639255409,
12.));
#129959=CARTESIAN_POINT('Ctrl Pts',(4.53578496366799,-72.5691865601223,
0.));
#129960=CARTESIAN_POINT('Ctrl Pts',(4.53578496366799,-72.5691865601223,
12.));
#129961=CARTESIAN_POINT('Ctrl Pts',(4.54354380466821,-72.5451394505104,
0.));
#129962=CARTESIAN_POINT('Ctrl Pts',(4.54354380466821,-72.5451394505104,
12.));
#129963=CARTESIAN_POINT('Ctrl Pts',(4.55126765384403,-72.5211227139001,
0.));
#129964=CARTESIAN_POINT('Ctrl Pts',(4.55126765384403,-72.5211227139001,
12.));
#129965=CARTESIAN_POINT('Ctrl Pts',(4.5589565311822,-72.4971364679068,0.));
#129966=CARTESIAN_POINT('Ctrl Pts',(4.5589565311822,-72.4971364679068,12.));
#129967=CARTESIAN_POINT('Ctrl Pts',(4.56661045683375,-72.4731808305728,
0.));
#129968=CARTESIAN_POINT('Ctrl Pts',(4.56661045683375,-72.4731808305728,
12.));
#129969=CARTESIAN_POINT('Ctrl Pts',(4.57422945111101,-72.4492559203745,
0.));
#129970=CARTESIAN_POINT('Ctrl Pts',(4.57422945111101,-72.4492559203745,
12.));
#129971=CARTESIAN_POINT('Ctrl Pts',(4.58181353448851,-72.4253618562252,
0.));
#129972=CARTESIAN_POINT('Ctrl Pts',(4.58181353448851,-72.4253618562252,
12.));
#129973=CARTESIAN_POINT('Ctrl Pts',(4.58936272760543,-72.401498757478,0.));
#129974=CARTESIAN_POINT('Ctrl Pts',(4.58936272760543,-72.401498757478,12.));
#129975=CARTESIAN_POINT('Ctrl Pts',(4.59687705127329,-72.3776667439227,
0.));
#129976=CARTESIAN_POINT('Ctrl Pts',(4.59687705127329,-72.3776667439227,
12.));
#129977=CARTESIAN_POINT('Ctrl Pts',(4.60435652647452,-72.3538659357913,
0.));
#129978=CARTESIAN_POINT('Ctrl Pts',(4.60435652647452,-72.3538659357913,
12.));
#129979=CARTESIAN_POINT('Ctrl Pts',(4.61180117435862,-72.3300964537658,
0.));
#129980=CARTESIAN_POINT('Ctrl Pts',(4.61180117435862,-72.3300964537658,
12.));
#129981=CARTESIAN_POINT('Ctrl Pts',(4.61921101624291,-72.3063584189807,
0.));
#129982=CARTESIAN_POINT('Ctrl Pts',(4.61921101624291,-72.3063584189807,
12.));
#129983=CARTESIAN_POINT('Ctrl Pts',(4.62658607361465,-72.2826519530259,
0.));
#129984=CARTESIAN_POINT('Ctrl Pts',(4.62658607361465,-72.2826519530259,
12.));
#129985=CARTESIAN_POINT('Ctrl Pts',(4.63392636813843,-72.2589771779456,
0.));
#129986=CARTESIAN_POINT('Ctrl Pts',(4.63392636813843,-72.2589771779456,
12.));
#129987=CARTESIAN_POINT('Ctrl Pts',(4.64123192165627,-72.2353342162417,
0.));
#129988=CARTESIAN_POINT('Ctrl Pts',(4.64123192165627,-72.2353342162417,
12.));
#129989=CARTESIAN_POINT('Ctrl Pts',(4.64850275618323,-72.2117231908822,
0.));
#129990=CARTESIAN_POINT('Ctrl Pts',(4.64850275618323,-72.2117231908822,
12.));
#129991=CARTESIAN_POINT('Ctrl Pts',(4.65573889390821,-72.1881442253053,
0.));
#129992=CARTESIAN_POINT('Ctrl Pts',(4.65573889390821,-72.1881442253053,
12.));
#129993=CARTESIAN_POINT('Ctrl Pts',(4.66294035719569,-72.1645974434216,
0.));
#129994=CARTESIAN_POINT('Ctrl Pts',(4.66294035719569,-72.1645974434216,
12.));
#129995=CARTESIAN_POINT('Ctrl Pts',(4.67010716859284,-72.1410829696128,
0.));
#129996=CARTESIAN_POINT('Ctrl Pts',(4.67010716859284,-72.1410829696128,
12.));
#129997=CARTESIAN_POINT('Ctrl Pts',(4.67723935083094,-72.1176009287351,
0.));
#129998=CARTESIAN_POINT('Ctrl Pts',(4.67723935083094,-72.1176009287351,
12.));
#129999=CARTESIAN_POINT('Ctrl Pts',(4.68433692682068,-72.0941514461287,
0.));
#130000=CARTESIAN_POINT('Ctrl Pts',(4.68433692682068,-72.0941514461287,
12.));
#130001=CARTESIAN_POINT('Ctrl Pts',(4.69139991965283,-72.0707346476213,
0.));
#130002=CARTESIAN_POINT('Ctrl Pts',(4.69139991965283,-72.0707346476213,
12.));
#130003=CARTESIAN_POINT('Ctrl Pts',(4.69842835259991,-72.0473506595318,
0.));
#130004=CARTESIAN_POINT('Ctrl Pts',(4.69842835259991,-72.0473506595318,
12.));
#130005=CARTESIAN_POINT('Ctrl Pts',(4.705422249123,-72.0239996086686,0.));
#130006=CARTESIAN_POINT('Ctrl Pts',(4.705422249123,-72.0239996086686,12.));
#130007=CARTESIAN_POINT('Ctrl Pts',(4.71238163287396,-72.0006816223325,
0.));
#130008=CARTESIAN_POINT('Ctrl Pts',(4.71238163287396,-72.0006816223325,
12.));
#130009=CARTESIAN_POINT('Ctrl Pts',(4.7193065276907,-71.9773968283259,0.));
#130010=CARTESIAN_POINT('Ctrl Pts',(4.7193065276907,-71.9773968283259,12.));
#130011=CARTESIAN_POINT('Ctrl Pts',(4.72619695759773,-71.9541453549579,
0.));
#130012=CARTESIAN_POINT('Ctrl Pts',(4.72619695759773,-71.9541453549579,
12.));
#130013=CARTESIAN_POINT('Ctrl Pts',(4.73305294680785,-71.9309273310471,
0.));
#130014=CARTESIAN_POINT('Ctrl Pts',(4.73305294680785,-71.9309273310471,
12.));
#130015=CARTESIAN_POINT('Ctrl Pts',(4.73987451972863,-71.9077428859212,
0.));
#130016=CARTESIAN_POINT('Ctrl Pts',(4.73987451972863,-71.9077428859212,
12.));
#130017=CARTESIAN_POINT('Ctrl Pts',(4.74666170096546,-71.8845921494189,
0.));
#130018=CARTESIAN_POINT('Ctrl Pts',(4.74666170096546,-71.8845921494189,
12.));
#130019=CARTESIAN_POINT('Ctrl Pts',(4.75341451531669,-71.8614752519008,
0.));
#130020=CARTESIAN_POINT('Ctrl Pts',(4.75341451531669,-71.8614752519008,
12.));
#130021=CARTESIAN_POINT('Ctrl Pts',(4.76013298777419,-71.8383923242531,
0.));
#130022=CARTESIAN_POINT('Ctrl Pts',(4.76013298777419,-71.8383923242531,
12.));
#130023=CARTESIAN_POINT('Ctrl Pts',(4.76681714352501,-71.8153434978923,
0.));
#130024=CARTESIAN_POINT('Ctrl Pts',(4.76681714352501,-71.8153434978923,
12.));
#130025=CARTESIAN_POINT('Ctrl Pts',(4.77346700795791,-71.7923289047643,
0.));
#130026=CARTESIAN_POINT('Ctrl Pts',(4.77346700795791,-71.7923289047643,
12.));
#130027=CARTESIAN_POINT('Ctrl Pts',(4.78008260666649,-71.769348677346,0.));
#130028=CARTESIAN_POINT('Ctrl Pts',(4.78008260666649,-71.769348677346,12.));
#130029=CARTESIAN_POINT('Ctrl Pts',(4.78666396544457,-71.7464029486563,
0.));
#130030=CARTESIAN_POINT('Ctrl Pts',(4.78666396544457,-71.7464029486563,
12.));
#130031=CARTESIAN_POINT('Ctrl Pts',(4.79321111028675,-71.723491852261,0.));
#130032=CARTESIAN_POINT('Ctrl Pts',(4.79321111028675,-71.723491852261,12.));
#130033=CARTESIAN_POINT('Ctrl Pts',(4.7997240673901,-71.7006155222764,0.));
#130034=CARTESIAN_POINT('Ctrl Pts',(4.7997240673901,-71.7006155222764,12.));
#130035=CARTESIAN_POINT('Ctrl Pts',(4.80620286316074,-71.6777740933687,
0.));
#130036=CARTESIAN_POINT('Ctrl Pts',(4.80620286316074,-71.6777740933687,
12.));
#130037=CARTESIAN_POINT('Ctrl Pts',(4.81264752421712,-71.6549677007582,
0.));
#130038=CARTESIAN_POINT('Ctrl Pts',(4.81264752421712,-71.6549677007582,
12.));
#130039=CARTESIAN_POINT('Ctrl Pts',(4.81905807738541,-71.6321964802297,
0.));
#130040=CARTESIAN_POINT('Ctrl Pts',(4.81905807738541,-71.6321964802297,
12.));
#130041=CARTESIAN_POINT('Ctrl Pts',(4.8254345497002,-71.6094605681353,0.));
#130042=CARTESIAN_POINT('Ctrl Pts',(4.8254345497002,-71.6094605681353,12.));
#130043=CARTESIAN_POINT('Ctrl Pts',(4.83177696840639,-71.5867601014008,
0.));
#130044=CARTESIAN_POINT('Ctrl Pts',(4.83177696840639,-71.5867601014008,
12.));
#130045=CARTESIAN_POINT('Ctrl Pts',(4.83808536096589,-71.5640952175239,
0.));
#130046=CARTESIAN_POINT('Ctrl Pts',(4.83808536096589,-71.5640952175239,
12.));
#130047=CARTESIAN_POINT('Ctrl Pts',(4.84435975506055,-71.5414660545778,
0.));
#130048=CARTESIAN_POINT('Ctrl Pts',(4.84435975506055,-71.5414660545778,
12.));
#130049=CARTESIAN_POINT('Ctrl Pts',(4.85060017858786,-71.5188727512231,
0.));
#130050=CARTESIAN_POINT('Ctrl Pts',(4.85060017858786,-71.5188727512231,
12.));
#130051=CARTESIAN_POINT('Ctrl Pts',(4.85680665966184,-71.4963154467128,
0.));
#130052=CARTESIAN_POINT('Ctrl Pts',(4.85680665966184,-71.4963154467128,
12.));
#130053=CARTESIAN_POINT('Ctrl Pts',(4.86297922661498,-71.4737942808971,
0.));
#130054=CARTESIAN_POINT('Ctrl Pts',(4.86297922661498,-71.4737942808971,
12.));
#130055=CARTESIAN_POINT('Ctrl Pts',(4.86911790800533,-71.4513093942216,
0.));
#130056=CARTESIAN_POINT('Ctrl Pts',(4.86911790800533,-71.4513093942216,
12.));
#130057=CARTESIAN_POINT('Ctrl Pts',(4.8752227326188,-71.4288609277324,0.));
#130058=CARTESIAN_POINT('Ctrl Pts',(4.8752227326188,-71.4288609277324,12.));
#130059=CARTESIAN_POINT('Ctrl Pts',(4.88129372946524,-71.4064490230857,
0.));
#130060=CARTESIAN_POINT('Ctrl Pts',(4.88129372946524,-71.4064490230857,
12.));
#130061=CARTESIAN_POINT('Ctrl Pts',(4.88733092777963,-71.3840738225548,
0.));
#130062=CARTESIAN_POINT('Ctrl Pts',(4.88733092777963,-71.3840738225548,
12.));
#130063=CARTESIAN_POINT('Ctrl Pts',(4.89333435702423,-71.3617354690342,
0.));
#130064=CARTESIAN_POINT('Ctrl Pts',(4.89333435702423,-71.3617354690342,
12.));
#130065=CARTESIAN_POINT('Ctrl Pts',(4.89930404689598,-71.3394341060396,
0.));
#130066=CARTESIAN_POINT('Ctrl Pts',(4.89930404689598,-71.3394341060396,
12.));
#130067=CARTESIAN_POINT('Ctrl Pts',(4.90524002732805,-71.3171698777124,
0.));
#130068=CARTESIAN_POINT('Ctrl Pts',(4.90524002732805,-71.3171698777124,
12.));
#130069=CARTESIAN_POINT('Ctrl Pts',(4.91114232848622,-71.2949429288319,
0.));
#130070=CARTESIAN_POINT('Ctrl Pts',(4.91114232848622,-71.2949429288319,
12.));
#130071=CARTESIAN_POINT('Ctrl Pts',(4.91701098077041,-71.27275340482,0.));
#130072=CARTESIAN_POINT('Ctrl Pts',(4.91701098077041,-71.27275340482,12.));
#130073=CARTESIAN_POINT('Ctrl Pts',(4.92284601481709,-71.2506014517457,
0.));
#130074=CARTESIAN_POINT('Ctrl Pts',(4.92284601481709,-71.2506014517457,
12.));
#130075=CARTESIAN_POINT('Ctrl Pts',(4.9286474615071,-71.2284872163248,0.));
#130076=CARTESIAN_POINT('Ctrl Pts',(4.9286474615071,-71.2284872163248,12.));
#130077=CARTESIAN_POINT('Ctrl Pts',(4.93441535196593,-71.206410845926,0.));
#130078=CARTESIAN_POINT('Ctrl Pts',(4.93441535196593,-71.206410845926,12.));
#130079=CARTESIAN_POINT('Ctrl Pts',(4.94014971756096,-71.184372488583,0.));
#130080=CARTESIAN_POINT('Ctrl Pts',(4.94014971756096,-71.184372488583,12.));
#130081=CARTESIAN_POINT('Ctrl Pts',(4.94585058990336,-71.1623722929998,
0.));
#130082=CARTESIAN_POINT('Ctrl Pts',(4.94585058990336,-71.1623722929998,
12.));
#130083=CARTESIAN_POINT('Ctrl Pts',(4.9515180008511,-71.1404104085561,0.));
#130084=CARTESIAN_POINT('Ctrl Pts',(4.9515180008511,-71.1404104085561,12.));
#130085=CARTESIAN_POINT('Ctrl Pts',(4.95715198251703,-71.1184869853071,
0.));
#130086=CARTESIAN_POINT('Ctrl Pts',(4.95715198251703,-71.1184869853071,
12.));
#130087=CARTESIAN_POINT('Ctrl Pts',(4.96275256726786,-71.0966021739922,
0.));
#130088=CARTESIAN_POINT('Ctrl Pts',(4.96275256726786,-71.0966021739922,
12.));
#130089=CARTESIAN_POINT('Ctrl Pts',(4.96831978772201,-71.0747561260443,
0.));
#130090=CARTESIAN_POINT('Ctrl Pts',(4.96831978772201,-71.0747561260443,
12.));
#130091=CARTESIAN_POINT('Ctrl Pts',(4.97385367675156,-71.0529489935959,
0.));
#130092=CARTESIAN_POINT('Ctrl Pts',(4.97385367675156,-71.0529489935959,
12.));
#130093=CARTESIAN_POINT('Ctrl Pts',(4.97935426748576,-71.031180929482,0.));
#130094=CARTESIAN_POINT('Ctrl Pts',(4.97935426748576,-71.031180929482,12.));
#130095=CARTESIAN_POINT('Ctrl Pts',(4.9848215933185,-71.0094520872375,0.));
#130096=CARTESIAN_POINT('Ctrl Pts',(4.9848215933185,-71.0094520872375,12.));
#130097=CARTESIAN_POINT('Ctrl Pts',(4.99025568790652,-70.9877626211112,
0.));
#130098=CARTESIAN_POINT('Ctrl Pts',(4.99025568790652,-70.9877626211112,
12.));
#130099=CARTESIAN_POINT('Ctrl Pts',(4.99565658516905,-70.9661126860773,
0.));
#130100=CARTESIAN_POINT('Ctrl Pts',(4.99565658516905,-70.9661126860773,
12.));
#130101=CARTESIAN_POINT('Ctrl Pts',(5.00102431929038,-70.9445024378439,
0.));
#130102=CARTESIAN_POINT('Ctrl Pts',(5.00102431929038,-70.9445024378439,
12.));
#130103=CARTESIAN_POINT('Ctrl Pts',(5.00635892472517,-70.9229320328588,
0.));
#130104=CARTESIAN_POINT('Ctrl Pts',(5.00635892472517,-70.9229320328588,
12.));
#130105=CARTESIAN_POINT('Ctrl Pts',(5.01166043620572,-70.9014016283123,
0.));
#130106=CARTESIAN_POINT('Ctrl Pts',(5.01166043620572,-70.9014016283123,
12.));
#130107=CARTESIAN_POINT('Ctrl Pts',(5.01692888873792,-70.8799113821449,
0.));
#130108=CARTESIAN_POINT('Ctrl Pts',(5.01692888873792,-70.8799113821449,
12.));
#130109=CARTESIAN_POINT('Ctrl Pts',(5.02216431760059,-70.8584614530517,
0.));
#130110=CARTESIAN_POINT('Ctrl Pts',(5.02216431760059,-70.8584614530517,
12.));
#130111=CARTESIAN_POINT('Ctrl Pts',(5.0273667583469,-70.8370520004844,0.));
#130112=CARTESIAN_POINT('Ctrl Pts',(5.0273667583469,-70.8370520004844,12.));
#130113=CARTESIAN_POINT('Ctrl Pts',(5.0325362468094,-70.8156831846494,0.));
#130114=CARTESIAN_POINT('Ctrl Pts',(5.0325362468094,-70.8156831846494,12.));
#130115=CARTESIAN_POINT('Ctrl Pts',(5.03767281910483,-70.7943551665071,
0.));
#130116=CARTESIAN_POINT('Ctrl Pts',(5.03767281910483,-70.7943551665071,
12.));
#130117=CARTESIAN_POINT('Ctrl Pts',(5.04277651163356,-70.7730681077997,
0.));
#130118=CARTESIAN_POINT('Ctrl Pts',(5.04277651163356,-70.7730681077997,
12.));
#130119=CARTESIAN_POINT('Ctrl Pts',(5.0478473610835,-70.7518221710715,0.));
#130120=CARTESIAN_POINT('Ctrl Pts',(5.0478473610835,-70.7518221710715,12.));
#130121=CARTESIAN_POINT('Ctrl Pts',(5.05288540443477,-70.7306175196856,
0.));
#130122=CARTESIAN_POINT('Ctrl Pts',(5.05288540443477,-70.7306175196856,
12.));
#130123=CARTESIAN_POINT('Ctrl Pts',(5.0578906789704,-70.7094543178416,0.));
#130124=CARTESIAN_POINT('Ctrl Pts',(5.0578906789704,-70.7094543178416,12.));
#130125=CARTESIAN_POINT('Ctrl Pts',(5.06286322227796,-70.6883327305755,
0.));
#130126=CARTESIAN_POINT('Ctrl Pts',(5.06286322227796,-70.6883327305755,
12.));
#130127=CARTESIAN_POINT('Ctrl Pts',(5.06780307224052,-70.6672529237431,
0.));
#130128=CARTESIAN_POINT('Ctrl Pts',(5.06780307224052,-70.6672529237431,
12.));
#130129=CARTESIAN_POINT('Ctrl Pts',(5.07271026703349,-70.6462150640009,
0.));
#130130=CARTESIAN_POINT('Ctrl Pts',(5.07271026703349,-70.6462150640009,
12.));
#130131=CARTESIAN_POINT('Ctrl Pts',(5.07758484512309,-70.6252193187892,
0.));
#130132=CARTESIAN_POINT('Ctrl Pts',(5.07758484512309,-70.6252193187892,
12.));
#130133=CARTESIAN_POINT('Ctrl Pts',(5.08242684526703,-70.6042658562951,
0.));
#130134=CARTESIAN_POINT('Ctrl Pts',(5.08242684526703,-70.6042658562951,
12.));
#130135=CARTESIAN_POINT('Ctrl Pts',(5.0872363065229,-70.5833548455043,0.));
#130136=CARTESIAN_POINT('Ctrl Pts',(5.0872363065229,-70.5833548455043,12.));
#130137=CARTESIAN_POINT('Ctrl Pts',(5.09201326826145,-70.5624864562841,
0.));
#130138=CARTESIAN_POINT('Ctrl Pts',(5.09201326826145,-70.5624864562841,
12.));
#130139=CARTESIAN_POINT('Ctrl Pts',(5.09675777018181,-70.5416608594526,
0.));
#130140=CARTESIAN_POINT('Ctrl Pts',(5.09675777018181,-70.5416608594526,
12.));
#130141=CARTESIAN_POINT('Ctrl Pts',(5.10146985232927,-70.5208782268482,
0.));
#130142=CARTESIAN_POINT('Ctrl Pts',(5.10146985232927,-70.5208782268482,
12.));
#130143=CARTESIAN_POINT('Ctrl Pts',(5.10614955511642,-70.5001387313963,
0.));
#130144=CARTESIAN_POINT('Ctrl Pts',(5.10614955511642,-70.5001387313963,
12.));
#130145=CARTESIAN_POINT('Ctrl Pts',(5.11079691929192,-70.4794425469799,
0.));
#130146=CARTESIAN_POINT('Ctrl Pts',(5.11079691929192,-70.4794425469799,
12.));
#130147=CARTESIAN_POINT('Ctrl Pts',(5.11541198590919,-70.4587898482946,
0.));
#130148=CARTESIAN_POINT('Ctrl Pts',(5.11541198590919,-70.4587898482946,
12.));
#130149=CARTESIAN_POINT('Ctrl Pts',(5.11999479630214,-70.438180810725,0.));
#130150=CARTESIAN_POINT('Ctrl Pts',(5.11999479630214,-70.438180810725,12.));
#130151=CARTESIAN_POINT('Ctrl Pts',(5.12454539205346,-70.4176156101633,
0.));
#130152=CARTESIAN_POINT('Ctrl Pts',(5.12454539205346,-70.4176156101633,
12.));
#130153=CARTESIAN_POINT('Ctrl Pts',(5.12906381499485,-70.3970944229885,
0.));
#130154=CARTESIAN_POINT('Ctrl Pts',(5.12906381499485,-70.3970944229885,
12.));
#130155=CARTESIAN_POINT('Ctrl Pts',(5.1335501072859,-70.3766174264786,0.));
#130156=CARTESIAN_POINT('Ctrl Pts',(5.1335501072859,-70.3766174264786,12.));
#130157=CARTESIAN_POINT('Ctrl Pts',(5.1380043114891,-70.3561847991725,0.));
#130158=CARTESIAN_POINT('Ctrl Pts',(5.1380043114891,-70.3561847991725,12.));
#130159=CARTESIAN_POINT('Ctrl Pts',(5.14242647063466,-70.3357967211782,
0.));
#130160=CARTESIAN_POINT('Ctrl Pts',(5.14242647063466,-70.3357967211782,
12.));
#130161=CARTESIAN_POINT('Ctrl Pts',(5.14681662833053,-70.31545337467,0.));
#130162=CARTESIAN_POINT('Ctrl Pts',(5.14681662833053,-70.31545337467,12.));
#130163=CARTESIAN_POINT('Ctrl Pts',(5.15117482869224,-70.2951549435469,
0.));
#130164=CARTESIAN_POINT('Ctrl Pts',(5.15117482869224,-70.2951549435469,
12.));
#130165=CARTESIAN_POINT('Ctrl Pts',(5.15550111614837,-70.2749016125073,
0.));
#130166=CARTESIAN_POINT('Ctrl Pts',(5.15550111614837,-70.2749016125073,
12.));
#130167=CARTESIAN_POINT('Ctrl Pts',(5.159795535282,-70.2546935662719,0.));
#130168=CARTESIAN_POINT('Ctrl Pts',(5.159795535282,-70.2546935662719,12.));
#130169=CARTESIAN_POINT('Ctrl Pts',(5.16405813066993,-70.2345309887864,
0.));
#130170=CARTESIAN_POINT('Ctrl Pts',(5.16405813066993,-70.2345309887864,
12.));
#130171=CARTESIAN_POINT('Ctrl Pts',(5.16828894670139,-70.2144140623004,
0.));
#130172=CARTESIAN_POINT('Ctrl Pts',(5.16828894670139,-70.2144140623004,
12.));
#130173=CARTESIAN_POINT('Ctrl Pts',(5.17248802793419,-70.1943429691214,
0.));
#130174=CARTESIAN_POINT('Ctrl Pts',(5.17248802793419,-70.1943429691214,
12.));
#130175=CARTESIAN_POINT('Ctrl Pts',(5.17665541952399,-70.1743178937102,
0.));
#130176=CARTESIAN_POINT('Ctrl Pts',(5.17665541952399,-70.1743178937102,
12.));
#130177=CARTESIAN_POINT('Ctrl Pts',(5.18079116757658,-70.1543390243882,
0.));
#130178=CARTESIAN_POINT('Ctrl Pts',(5.18079116757658,-70.1543390243882,
12.));
#130179=CARTESIAN_POINT('Ctrl Pts',(5.18489531966234,-70.1344065558106,
0.));
#130180=CARTESIAN_POINT('Ctrl Pts',(5.18489531966234,-70.1344065558106,
12.));
#130181=CARTESIAN_POINT('Ctrl Pts',(5.18896792486522,-70.1145206891833,
0.));
#130182=CARTESIAN_POINT('Ctrl Pts',(5.18896792486522,-70.1145206891833,
12.));
#130183=CARTESIAN_POINT('Ctrl Pts',(5.19300903271543,-70.0946816270957,
0.));
#130184=CARTESIAN_POINT('Ctrl Pts',(5.19300903271543,-70.0946816270957,
12.));
#130185=CARTESIAN_POINT('Ctrl Pts',(5.19701869225514,-70.0748895689716,
0.));
#130186=CARTESIAN_POINT('Ctrl Pts',(5.19701869225514,-70.0748895689716,
12.));
#130187=CARTESIAN_POINT('Ctrl Pts',(5.20099695122676,-70.0551447071106,
0.));
#130188=CARTESIAN_POINT('Ctrl Pts',(5.20099695122676,-70.0551447071106,
12.));
#130189=CARTESIAN_POINT('Ctrl Pts',(5.20494385478083,-70.0354472203604,
0.));
#130190=CARTESIAN_POINT('Ctrl Pts',(5.20494385478083,-70.0354472203604,
12.));
#130191=CARTESIAN_POINT('Ctrl Pts',(5.20885944672914,-70.0157972802255,
0.));
#130192=CARTESIAN_POINT('Ctrl Pts',(5.20885944672914,-70.0157972802255,
12.));
#130193=CARTESIAN_POINT('Ctrl Pts',(5.2127437720332,-69.996195063002,0.));
#130194=CARTESIAN_POINT('Ctrl Pts',(5.2127437720332,-69.996195063002,12.));
#130195=CARTESIAN_POINT('Ctrl Pts',(5.21659687881138,-69.9766407595385,
0.));
#130196=CARTESIAN_POINT('Ctrl Pts',(5.21659687881138,-69.9766407595385,
12.));
#130197=CARTESIAN_POINT('Ctrl Pts',(5.22041882075626,-69.9571345869996,
0.));
#130198=CARTESIAN_POINT('Ctrl Pts',(5.22041882075626,-69.9571345869996,
12.));
#130199=CARTESIAN_POINT('Ctrl Pts',(5.22420965879807,-69.9376767968951,
0.));
#130200=CARTESIAN_POINT('Ctrl Pts',(5.22420965879807,-69.9376767968951,
12.));
#130201=CARTESIAN_POINT('Ctrl Pts',(5.22796945602602,-69.9182676501892,
0.));
#130202=CARTESIAN_POINT('Ctrl Pts',(5.22796945602602,-69.9182676501892,
12.));
#130203=CARTESIAN_POINT('Ctrl Pts',(5.23169827290451,-69.8989073936606,
0.));
#130204=CARTESIAN_POINT('Ctrl Pts',(5.23169827290451,-69.8989073936606,
12.));
#130205=CARTESIAN_POINT('Ctrl Pts',(5.23539616279714,-69.8795962381676,
0.));
#130206=CARTESIAN_POINT('Ctrl Pts',(5.23539616279714,-69.8795962381676,
12.));
#130207=CARTESIAN_POINT('Ctrl Pts',(5.2390631663514,-69.8603343303016,0.));
#130208=CARTESIAN_POINT('Ctrl Pts',(5.2390631663514,-69.8603343303016,12.));
#130209=CARTESIAN_POINT('Ctrl Pts',(5.24269931055074,-69.8411217507931,
0.));
#130210=CARTESIAN_POINT('Ctrl Pts',(5.24269931055074,-69.8411217507931,
12.));
#130211=CARTESIAN_POINT('Ctrl Pts',(5.24558355160219,-69.8257911792542,
0.));
#130212=CARTESIAN_POINT('Ctrl Pts',(5.24558355160219,-69.8257911792542,
12.));
#130213=CARTESIAN_POINT('Ctrl Pts',(5.24773285666673,-69.8143154684447,
0.));
#130214=CARTESIAN_POINT('Ctrl Pts',(5.24773285666673,-69.8143154684447,
12.));
#130215=CARTESIAN_POINT('Ctrl Pts',(5.24915955997536,-69.8066748687863,
0.));
#130216=CARTESIAN_POINT('Ctrl Pts',(5.24915955997536,-69.8066748687863,
12.));
#130217=CARTESIAN_POINT('Ctrl Pts',(5.2498713699459,-69.8028570375098,0.));
#130218=CARTESIAN_POINT('Ctrl Pts',(5.2498713699459,-69.8028570375098,12.));
#130219=CARTESIAN_POINT('',(5.2498713699459,-69.8028570375098,12.));
#130220=CARTESIAN_POINT('Ctrl Pts',(5.2498713699459,-69.8028570375098,12.));
#130221=CARTESIAN_POINT('Ctrl Pts',(5.24915955997536,-69.8066748687863,
12.));
#130222=CARTESIAN_POINT('Ctrl Pts',(5.24773285666673,-69.8143154684447,
12.));
#130223=CARTESIAN_POINT('Ctrl Pts',(5.24558355160219,-69.8257911792542,
12.));
#130224=CARTESIAN_POINT('Ctrl Pts',(5.24269931055074,-69.8411217507931,
12.));
#130225=CARTESIAN_POINT('Ctrl Pts',(5.2390631663514,-69.8603343303016,12.));
#130226=CARTESIAN_POINT('Ctrl Pts',(5.23539616279714,-69.8795962381676,
12.));
#130227=CARTESIAN_POINT('Ctrl Pts',(5.23169827290451,-69.8989073936606,
12.));
#130228=CARTESIAN_POINT('Ctrl Pts',(5.22796945602602,-69.9182676501892,
12.));
#130229=CARTESIAN_POINT('Ctrl Pts',(5.22420965879807,-69.9376767968951,
12.));
#130230=CARTESIAN_POINT('Ctrl Pts',(5.22041882075626,-69.9571345869996,
12.));
#130231=CARTESIAN_POINT('Ctrl Pts',(5.21659687881138,-69.9766407595385,
12.));
#130232=CARTESIAN_POINT('Ctrl Pts',(5.2127437720332,-69.996195063002,12.));
#130233=CARTESIAN_POINT('Ctrl Pts',(5.20885944672914,-70.0157972802255,
12.));
#130234=CARTESIAN_POINT('Ctrl Pts',(5.20494385478083,-70.0354472203604,
12.));
#130235=CARTESIAN_POINT('Ctrl Pts',(5.20099695122676,-70.0551447071106,
12.));
#130236=CARTESIAN_POINT('Ctrl Pts',(5.19701869225514,-70.0748895689716,
12.));
#130237=CARTESIAN_POINT('Ctrl Pts',(5.19300903271543,-70.0946816270957,
12.));
#130238=CARTESIAN_POINT('Ctrl Pts',(5.18896792486522,-70.1145206891833,
12.));
#130239=CARTESIAN_POINT('Ctrl Pts',(5.18489531966234,-70.1344065558106,
12.));
#130240=CARTESIAN_POINT('Ctrl Pts',(5.18079116757658,-70.1543390243882,
12.));
#130241=CARTESIAN_POINT('Ctrl Pts',(5.17665541952399,-70.1743178937102,
12.));
#130242=CARTESIAN_POINT('Ctrl Pts',(5.17248802793419,-70.1943429691214,
12.));
#130243=CARTESIAN_POINT('Ctrl Pts',(5.16828894670139,-70.2144140623004,
12.));
#130244=CARTESIAN_POINT('Ctrl Pts',(5.16405813066993,-70.2345309887864,
12.));
#130245=CARTESIAN_POINT('Ctrl Pts',(5.159795535282,-70.2546935662719,12.));
#130246=CARTESIAN_POINT('Ctrl Pts',(5.15550111614837,-70.2749016125073,
12.));
#130247=CARTESIAN_POINT('Ctrl Pts',(5.15117482869224,-70.2951549435469,
12.));
#130248=CARTESIAN_POINT('Ctrl Pts',(5.14681662833053,-70.31545337467,12.));
#130249=CARTESIAN_POINT('Ctrl Pts',(5.14242647063466,-70.3357967211782,
12.));
#130250=CARTESIAN_POINT('Ctrl Pts',(5.1380043114891,-70.3561847991725,12.));
#130251=CARTESIAN_POINT('Ctrl Pts',(5.1335501072859,-70.3766174264786,12.));
#130252=CARTESIAN_POINT('Ctrl Pts',(5.12906381499485,-70.3970944229885,
12.));
#130253=CARTESIAN_POINT('Ctrl Pts',(5.12454539205346,-70.4176156101633,
12.));
#130254=CARTESIAN_POINT('Ctrl Pts',(5.11999479630214,-70.438180810725,12.));
#130255=CARTESIAN_POINT('Ctrl Pts',(5.11541198590919,-70.4587898482946,
12.));
#130256=CARTESIAN_POINT('Ctrl Pts',(5.11079691929192,-70.4794425469799,
12.));
#130257=CARTESIAN_POINT('Ctrl Pts',(5.10614955511642,-70.5001387313963,
12.));
#130258=CARTESIAN_POINT('Ctrl Pts',(5.10146985232927,-70.5208782268482,
12.));
#130259=CARTESIAN_POINT('Ctrl Pts',(5.09675777018181,-70.5416608594526,
12.));
#130260=CARTESIAN_POINT('Ctrl Pts',(5.09201326826145,-70.5624864562841,
12.));
#130261=CARTESIAN_POINT('Ctrl Pts',(5.0872363065229,-70.5833548455043,12.));
#130262=CARTESIAN_POINT('Ctrl Pts',(5.08242684526703,-70.6042658562951,
12.));
#130263=CARTESIAN_POINT('Ctrl Pts',(5.07758484512309,-70.6252193187892,
12.));
#130264=CARTESIAN_POINT('Ctrl Pts',(5.07271026703349,-70.6462150640009,
12.));
#130265=CARTESIAN_POINT('Ctrl Pts',(5.06780307224052,-70.6672529237431,
12.));
#130266=CARTESIAN_POINT('Ctrl Pts',(5.06286322227796,-70.6883327305755,
12.));
#130267=CARTESIAN_POINT('Ctrl Pts',(5.0578906789704,-70.7094543178416,12.));
#130268=CARTESIAN_POINT('Ctrl Pts',(5.05288540443477,-70.7306175196856,
12.));
#130269=CARTESIAN_POINT('Ctrl Pts',(5.0478473610835,-70.7518221710715,12.));
#130270=CARTESIAN_POINT('Ctrl Pts',(5.04277651163356,-70.7730681077997,
12.));
#130271=CARTESIAN_POINT('Ctrl Pts',(5.03767281910483,-70.7943551665071,
12.));
#130272=CARTESIAN_POINT('Ctrl Pts',(5.0325362468094,-70.8156831846494,12.));
#130273=CARTESIAN_POINT('Ctrl Pts',(5.0273667583469,-70.8370520004844,12.));
#130274=CARTESIAN_POINT('Ctrl Pts',(5.02216431760059,-70.8584614530517,
12.));
#130275=CARTESIAN_POINT('Ctrl Pts',(5.01692888873792,-70.8799113821449,
12.));
#130276=CARTESIAN_POINT('Ctrl Pts',(5.01166043620572,-70.9014016283123,
12.));
#130277=CARTESIAN_POINT('Ctrl Pts',(5.00635892472517,-70.9229320328588,
12.));
#130278=CARTESIAN_POINT('Ctrl Pts',(5.00102431929038,-70.9445024378439,
12.));
#130279=CARTESIAN_POINT('Ctrl Pts',(4.99565658516905,-70.9661126860773,
12.));
#130280=CARTESIAN_POINT('Ctrl Pts',(4.99025568790652,-70.9877626211112,
12.));
#130281=CARTESIAN_POINT('Ctrl Pts',(4.9848215933185,-71.0094520872375,12.));
#130282=CARTESIAN_POINT('Ctrl Pts',(4.97935426748576,-71.031180929482,12.));
#130283=CARTESIAN_POINT('Ctrl Pts',(4.97385367675156,-71.0529489935959,
12.));
#130284=CARTESIAN_POINT('Ctrl Pts',(4.96831978772201,-71.0747561260443,
12.));
#130285=CARTESIAN_POINT('Ctrl Pts',(4.96275256726786,-71.0966021739922,
12.));
#130286=CARTESIAN_POINT('Ctrl Pts',(4.95715198251703,-71.1184869853071,
12.));
#130287=CARTESIAN_POINT('Ctrl Pts',(4.9515180008511,-71.1404104085561,12.));
#130288=CARTESIAN_POINT('Ctrl Pts',(4.94585058990336,-71.1623722929998,
12.));
#130289=CARTESIAN_POINT('Ctrl Pts',(4.94014971756096,-71.184372488583,12.));
#130290=CARTESIAN_POINT('Ctrl Pts',(4.93441535196593,-71.206410845926,12.));
#130291=CARTESIAN_POINT('Ctrl Pts',(4.9286474615071,-71.2284872163248,12.));
#130292=CARTESIAN_POINT('Ctrl Pts',(4.92284601481709,-71.2506014517457,
12.));
#130293=CARTESIAN_POINT('Ctrl Pts',(4.91701098077041,-71.27275340482,12.));
#130294=CARTESIAN_POINT('Ctrl Pts',(4.91114232848622,-71.2949429288319,
12.));
#130295=CARTESIAN_POINT('Ctrl Pts',(4.90524002732805,-71.3171698777124,
12.));
#130296=CARTESIAN_POINT('Ctrl Pts',(4.89930404689598,-71.3394341060396,
12.));
#130297=CARTESIAN_POINT('Ctrl Pts',(4.89333435702423,-71.3617354690342,
12.));
#130298=CARTESIAN_POINT('Ctrl Pts',(4.88733092777963,-71.3840738225548,
12.));
#130299=CARTESIAN_POINT('Ctrl Pts',(4.88129372946524,-71.4064490230857,
12.));
#130300=CARTESIAN_POINT('Ctrl Pts',(4.8752227326188,-71.4288609277324,12.));
#130301=CARTESIAN_POINT('Ctrl Pts',(4.86911790800533,-71.4513093942216,
12.));
#130302=CARTESIAN_POINT('Ctrl Pts',(4.86297922661498,-71.4737942808971,
12.));
#130303=CARTESIAN_POINT('Ctrl Pts',(4.85680665966184,-71.4963154467128,
12.));
#130304=CARTESIAN_POINT('Ctrl Pts',(4.85060017858786,-71.5188727512231,
12.));
#130305=CARTESIAN_POINT('Ctrl Pts',(4.84435975506055,-71.5414660545778,
12.));
#130306=CARTESIAN_POINT('Ctrl Pts',(4.83808536096589,-71.5640952175239,
12.));
#130307=CARTESIAN_POINT('Ctrl Pts',(4.83177696840639,-71.5867601014008,
12.));
#130308=CARTESIAN_POINT('Ctrl Pts',(4.8254345497002,-71.6094605681353,12.));
#130309=CARTESIAN_POINT('Ctrl Pts',(4.81905807738541,-71.6321964802297,
12.));
#130310=CARTESIAN_POINT('Ctrl Pts',(4.81264752421712,-71.6549677007582,
12.));
#130311=CARTESIAN_POINT('Ctrl Pts',(4.80620286316074,-71.6777740933687,
12.));
#130312=CARTESIAN_POINT('Ctrl Pts',(4.7997240673901,-71.7006155222764,12.));
#130313=CARTESIAN_POINT('Ctrl Pts',(4.79321111028675,-71.723491852261,12.));
#130314=CARTESIAN_POINT('Ctrl Pts',(4.78666396544457,-71.7464029486563,
12.));
#130315=CARTESIAN_POINT('Ctrl Pts',(4.78008260666649,-71.769348677346,12.));
#130316=CARTESIAN_POINT('Ctrl Pts',(4.77346700795791,-71.7923289047643,
12.));
#130317=CARTESIAN_POINT('Ctrl Pts',(4.76681714352501,-71.8153434978923,
12.));
#130318=CARTESIAN_POINT('Ctrl Pts',(4.76013298777419,-71.8383923242531,
12.));
#130319=CARTESIAN_POINT('Ctrl Pts',(4.75341451531669,-71.8614752519008,
12.));
#130320=CARTESIAN_POINT('Ctrl Pts',(4.74666170096546,-71.8845921494189,
12.));
#130321=CARTESIAN_POINT('Ctrl Pts',(4.73987451972863,-71.9077428859212,
12.));
#130322=CARTESIAN_POINT('Ctrl Pts',(4.73305294680785,-71.9309273310471,
12.));
#130323=CARTESIAN_POINT('Ctrl Pts',(4.72619695759773,-71.9541453549579,
12.));
#130324=CARTESIAN_POINT('Ctrl Pts',(4.7193065276907,-71.9773968283259,12.));
#130325=CARTESIAN_POINT('Ctrl Pts',(4.71238163287396,-72.0006816223325,
12.));
#130326=CARTESIAN_POINT('Ctrl Pts',(4.705422249123,-72.0239996086686,12.));
#130327=CARTESIAN_POINT('Ctrl Pts',(4.69842835259991,-72.0473506595318,
12.));
#130328=CARTESIAN_POINT('Ctrl Pts',(4.69139991965283,-72.0707346476213,
12.));
#130329=CARTESIAN_POINT('Ctrl Pts',(4.68433692682068,-72.0941514461287,
12.));
#130330=CARTESIAN_POINT('Ctrl Pts',(4.67723935083094,-72.1176009287351,
12.));
#130331=CARTESIAN_POINT('Ctrl Pts',(4.67010716859284,-72.1410829696128,
12.));
#130332=CARTESIAN_POINT('Ctrl Pts',(4.66294035719569,-72.1645974434216,
12.));
#130333=CARTESIAN_POINT('Ctrl Pts',(4.65573889390821,-72.1881442253053,
12.));
#130334=CARTESIAN_POINT('Ctrl Pts',(4.64850275618323,-72.2117231908822,
12.));
#130335=CARTESIAN_POINT('Ctrl Pts',(4.64123192165627,-72.2353342162417,
12.));
#130336=CARTESIAN_POINT('Ctrl Pts',(4.63392636813843,-72.2589771779456,
12.));
#130337=CARTESIAN_POINT('Ctrl Pts',(4.62658607361465,-72.2826519530259,
12.));
#130338=CARTESIAN_POINT('Ctrl Pts',(4.61921101624291,-72.3063584189807,
12.));
#130339=CARTESIAN_POINT('Ctrl Pts',(4.61180117435862,-72.3300964537658,
12.));
#130340=CARTESIAN_POINT('Ctrl Pts',(4.60435652647452,-72.3538659357913,
12.));
#130341=CARTESIAN_POINT('Ctrl Pts',(4.59687705127329,-72.3776667439227,
12.));
#130342=CARTESIAN_POINT('Ctrl Pts',(4.58936272760543,-72.401498757478,12.));
#130343=CARTESIAN_POINT('Ctrl Pts',(4.58181353448851,-72.4253618562252,
12.));
#130344=CARTESIAN_POINT('Ctrl Pts',(4.57422945111101,-72.4492559203745,
12.));
#130345=CARTESIAN_POINT('Ctrl Pts',(4.56661045683375,-72.4731808305728,
12.));
#130346=CARTESIAN_POINT('Ctrl Pts',(4.5589565311822,-72.4971364679068,12.));
#130347=CARTESIAN_POINT('Ctrl Pts',(4.55126765384403,-72.5211227139001,
12.));
#130348=CARTESIAN_POINT('Ctrl Pts',(4.54354380466821,-72.5451394505104,
12.));
#130349=CARTESIAN_POINT('Ctrl Pts',(4.53578496366799,-72.5691865601223,
12.));
#130350=CARTESIAN_POINT('Ctrl Pts',(4.52799111102391,-72.5932639255409,
12.));
#130351=CARTESIAN_POINT('Ctrl Pts',(4.52016222707637,-72.6173714299942,
12.));
#130352=CARTESIAN_POINT('Ctrl Pts',(4.51229829232263,-72.6415089571321,
12.));
#130353=CARTESIAN_POINT('Ctrl Pts',(4.50439928741603,-72.6656763910241,
12.));
#130354=CARTESIAN_POINT('Ctrl Pts',(4.49646519316812,-72.6898736161542,
12.));
#130355=CARTESIAN_POINT('Ctrl Pts',(4.48849599055337,-72.714100517414,12.));
#130356=CARTESIAN_POINT('Ctrl Pts',(4.48049166070205,-72.738356980103,12.));
#130357=CARTESIAN_POINT('Ctrl Pts',(4.47245218489609,-72.7626428899281,
12.));
#130358=CARTESIAN_POINT('Ctrl Pts',(4.46437754456792,-72.7869581329994,
12.));
#130359=CARTESIAN_POINT('Ctrl Pts',(4.45626772130145,-72.8113025958262,
12.));
#130360=CARTESIAN_POINT('Ctrl Pts',(4.44812269683737,-72.8356761653069,
12.));
#130361=CARTESIAN_POINT('Ctrl Pts',(4.43994245306817,-72.8600787287318,
12.));
#130362=CARTESIAN_POINT('Ctrl Pts',(4.43172697203349,-72.8845101737855,
12.));
#130363=CARTESIAN_POINT('Ctrl Pts',(4.42347623591941,-72.9089703885462,
12.));
#130364=CARTESIAN_POINT('Ctrl Pts',(4.41519022705921,-72.9334592614829,
12.));
#130365=CARTESIAN_POINT('Ctrl Pts',(4.40686892793957,-72.95797668145,12.));
#130366=CARTESIAN_POINT('Ctrl Pts',(4.39851232119721,-72.9825225376847,
12.));
#130367=CARTESIAN_POINT('Ctrl Pts',(4.39012038961138,-73.007096719804,12.));
#130368=CARTESIAN_POINT('Ctrl Pts',(4.3816931161015,-73.0316991177993,12.));
#130369=CARTESIAN_POINT('Ctrl Pts',(4.37323048372606,-73.0563296220299,
12.));
#130370=CARTESIAN_POINT('Ctrl Pts',(4.3647324756864,-73.0809881232103,12.));
#130371=CARTESIAN_POINT('Ctrl Pts',(4.35619907532719,-73.1056745124087,
12.));
#130372=CARTESIAN_POINT('Ctrl Pts',(4.34763026613157,-73.130388681059,12.));
#130373=CARTESIAN_POINT('Ctrl Pts',(4.3390260317214,-73.1551305209685,12.));
#130374=CARTESIAN_POINT('Ctrl Pts',(4.33038635585876,-73.1798999243235,
12.));
#130375=CARTESIAN_POINT('Ctrl Pts',(4.32171122245213,-73.204696783694,12.));
#130376=CARTESIAN_POINT('Ctrl Pts',(4.31300061556097,-73.2295209920334,
12.));
#130377=CARTESIAN_POINT('Ctrl Pts',(4.30425451938229,-73.2543724426577,
12.));
#130378=CARTESIAN_POINT('Ctrl Pts',(4.29547291824286,-73.2792510292254,
12.));
#130379=CARTESIAN_POINT('Ctrl Pts',(4.286655796593,-73.3041566457135,12.));
#130380=CARTESIAN_POINT('Ctrl Pts',(4.27780313900389,-73.3290891863949,
12.));
#130381=CARTESIAN_POINT('Ctrl Pts',(4.26891493016699,-73.3540485458065,
12.));
#130382=CARTESIAN_POINT('Ctrl Pts',(4.25999115489898,-73.3790346187938,
12.));
#130383=CARTESIAN_POINT('Ctrl Pts',(4.25103179814886,-73.4040473005592,
12.));
#130384=CARTESIAN_POINT('Ctrl Pts',(4.24203684500938,-73.4290864867101,
12.));
#130385=CARTESIAN_POINT('Ctrl Pts',(4.23300628072757,-73.4541520732948,
12.));
#130386=CARTESIAN_POINT('Ctrl Pts',(4.22394009072755,-73.4792439568633,
12.));
#130387=CARTESIAN_POINT('Ctrl Pts',(4.2148382605944,-73.5043620344116,12.));
#130388=CARTESIAN_POINT('Ctrl Pts',(4.20570077603729,-73.5295062032628,
12.));
#130389=CARTESIAN_POINT('Ctrl Pts',(4.19652762286126,-73.5546763609572,
12.));
#130390=CARTESIAN_POINT('Ctrl Pts',(4.18731878694235,-73.5798724051519,
12.));
#130391=CARTESIAN_POINT('Ctrl Pts',(4.17807425419812,-73.6050942334768,
12.));
#130392=CARTESIAN_POINT('Ctrl Pts',(4.1687940105878,-73.6303417435251,12.));
#130393=CARTESIAN_POINT('Ctrl Pts',(4.15947804217783,-73.6556148331489,
12.));
#130394=CARTESIAN_POINT('Ctrl Pts',(4.15012633519722,-73.6809134006897,
12.));
#130395=CARTESIAN_POINT('Ctrl Pts',(4.14073887610152,-73.7062373452342,
12.));
#130396=CARTESIAN_POINT('Ctrl Pts',(4.13131565163577,-73.7315865668522,
12.));
#130397=CARTESIAN_POINT('Ctrl Pts',(4.12185664890556,-73.7569609668528,
12.));
#130398=CARTESIAN_POINT('Ctrl Pts',(4.11236185522786,-73.7823604472159,
12.));
#130399=CARTESIAN_POINT('Ctrl Pts',(4.10283125798728,-73.8077849100342,
12.));
#130400=CARTESIAN_POINT('Ctrl Pts',(4.09326484448232,-73.8332342568989,
12.));
#130401=CARTESIAN_POINT('Ctrl Pts',(4.08366260180674,-73.8587083884191,
12.));
#130402=CARTESIAN_POINT('Ctrl Pts',(4.07402451665244,-73.8842072034008,
12.));
#130403=CARTESIAN_POINT('Ctrl Pts',(4.06435057547324,-73.9097305995115,
12.));
#130404=CARTESIAN_POINT('Ctrl Pts',(4.05464076484751,-73.9352784747608,
12.));
#130405=CARTESIAN_POINT('Ctrl Pts',(4.04489507179957,-73.9608507287909,
12.));
#130406=CARTESIAN_POINT('Ctrl Pts',(4.03511348410659,-73.9864472641033,
12.));
#130407=CARTESIAN_POINT('Ctrl Pts',(4.02529599070094,-74.012067987646,12.));
#130408=CARTESIAN_POINT('Ctrl Pts',(4.0154425817671,-74.0377128111863,12.));
#130409=CARTESIAN_POINT('Ctrl Pts',(4.00696550627364,-74.0597159782109,
12.));
#130410=CARTESIAN_POINT('Ctrl Pts',(4.00044689711983,-74.0765982943677,
12.));
#130411=CARTESIAN_POINT('Ctrl Pts',(3.99590266746991,-74.0883491449954,
12.));
#130412=CARTESIAN_POINT('Ctrl Pts',(3.99334334445528,-74.0949615399619,
12.));
#130413=CARTESIAN_POINT('Ctrl Pts',(3.99277406490872,-74.0964320766207,
12.));
#130414=CARTESIAN_POINT('',(5.2498713699459,-69.8028570375098,0.));
#130415=CARTESIAN_POINT('',(5.2498713699459,-69.8028570375097,0.));
#130416=CARTESIAN_POINT('Ctrl Pts',(3.99277406490873,-74.0964320766207,
0.));
#130417=CARTESIAN_POINT('Ctrl Pts',(3.9933433444553,-74.0949615399619,0.));
#130418=CARTESIAN_POINT('Ctrl Pts',(3.99590266746992,-74.0883491449954,
0.));
#130419=CARTESIAN_POINT('Ctrl Pts',(4.00044689711983,-74.0765982943676,
0.));
#130420=CARTESIAN_POINT('Ctrl Pts',(4.00696550627364,-74.0597159782109,
0.));
#130421=CARTESIAN_POINT('Ctrl Pts',(4.0154425817671,-74.0377128111863,0.));
#130422=CARTESIAN_POINT('Ctrl Pts',(4.02529599070094,-74.012067987646,0.));
#130423=CARTESIAN_POINT('Ctrl Pts',(4.03511348410659,-73.9864472641033,
0.));
#130424=CARTESIAN_POINT('Ctrl Pts',(4.04489507179957,-73.9608507287909,
0.));
#130425=CARTESIAN_POINT('Ctrl Pts',(4.05464076484751,-73.9352784747608,
0.));
#130426=CARTESIAN_POINT('Ctrl Pts',(4.06435057547324,-73.9097305995115,
0.));
#130427=CARTESIAN_POINT('Ctrl Pts',(4.07402451665244,-73.8842072034008,
0.));
#130428=CARTESIAN_POINT('Ctrl Pts',(4.08366260180674,-73.8587083884191,
0.));
#130429=CARTESIAN_POINT('Ctrl Pts',(4.09326484448232,-73.8332342568989,
0.));
#130430=CARTESIAN_POINT('Ctrl Pts',(4.10283125798728,-73.8077849100342,
0.));
#130431=CARTESIAN_POINT('Ctrl Pts',(4.11236185522786,-73.7823604472159,
0.));
#130432=CARTESIAN_POINT('Ctrl Pts',(4.12185664890556,-73.7569609668528,
0.));
#130433=CARTESIAN_POINT('Ctrl Pts',(4.13131565163577,-73.7315865668522,
0.));
#130434=CARTESIAN_POINT('Ctrl Pts',(4.14073887610152,-73.7062373452342,
0.));
#130435=CARTESIAN_POINT('Ctrl Pts',(4.15012633519722,-73.6809134006897,
0.));
#130436=CARTESIAN_POINT('Ctrl Pts',(4.15947804217783,-73.6556148331489,
0.));
#130437=CARTESIAN_POINT('Ctrl Pts',(4.1687940105878,-73.6303417435251,0.));
#130438=CARTESIAN_POINT('Ctrl Pts',(4.17807425419812,-73.6050942334768,
0.));
#130439=CARTESIAN_POINT('Ctrl Pts',(4.18731878694235,-73.5798724051519,
0.));
#130440=CARTESIAN_POINT('Ctrl Pts',(4.19652762286126,-73.5546763609572,
0.));
#130441=CARTESIAN_POINT('Ctrl Pts',(4.20570077603729,-73.5295062032628,
0.));
#130442=CARTESIAN_POINT('Ctrl Pts',(4.2148382605944,-73.5043620344116,0.));
#130443=CARTESIAN_POINT('Ctrl Pts',(4.22394009072755,-73.4792439568633,
0.));
#130444=CARTESIAN_POINT('Ctrl Pts',(4.23300628072757,-73.4541520732948,
0.));
#130445=CARTESIAN_POINT('Ctrl Pts',(4.24203684500938,-73.4290864867101,
0.));
#130446=CARTESIAN_POINT('Ctrl Pts',(4.25103179814886,-73.4040473005592,
0.));
#130447=CARTESIAN_POINT('Ctrl Pts',(4.25999115489898,-73.3790346187938,
0.));
#130448=CARTESIAN_POINT('Ctrl Pts',(4.26891493016699,-73.3540485458065,
0.));
#130449=CARTESIAN_POINT('Ctrl Pts',(4.27780313900389,-73.3290891863949,
0.));
#130450=CARTESIAN_POINT('Ctrl Pts',(4.286655796593,-73.3041566457135,0.));
#130451=CARTESIAN_POINT('Ctrl Pts',(4.29547291824286,-73.2792510292254,
0.));
#130452=CARTESIAN_POINT('Ctrl Pts',(4.30425451938229,-73.2543724426577,
0.));
#130453=CARTESIAN_POINT('Ctrl Pts',(4.31300061556097,-73.2295209920334,
0.));
#130454=CARTESIAN_POINT('Ctrl Pts',(4.32171122245213,-73.204696783694,0.));
#130455=CARTESIAN_POINT('Ctrl Pts',(4.33038635585876,-73.1798999243235,
0.));
#130456=CARTESIAN_POINT('Ctrl Pts',(4.3390260317214,-73.1551305209685,0.));
#130457=CARTESIAN_POINT('Ctrl Pts',(4.34763026613157,-73.130388681059,0.));
#130458=CARTESIAN_POINT('Ctrl Pts',(4.35619907532719,-73.1056745124087,
0.));
#130459=CARTESIAN_POINT('Ctrl Pts',(4.3647324756864,-73.0809881232103,0.));
#130460=CARTESIAN_POINT('Ctrl Pts',(4.37323048372606,-73.0563296220299,
0.));
#130461=CARTESIAN_POINT('Ctrl Pts',(4.3816931161015,-73.0316991177993,0.));
#130462=CARTESIAN_POINT('Ctrl Pts',(4.39012038961138,-73.007096719804,0.));
#130463=CARTESIAN_POINT('Ctrl Pts',(4.39851232119721,-72.9825225376847,
0.));
#130464=CARTESIAN_POINT('Ctrl Pts',(4.40686892793957,-72.95797668145,0.));
#130465=CARTESIAN_POINT('Ctrl Pts',(4.41519022705921,-72.9334592614829,
0.));
#130466=CARTESIAN_POINT('Ctrl Pts',(4.42347623591941,-72.9089703885462,
0.));
#130467=CARTESIAN_POINT('Ctrl Pts',(4.43172697203349,-72.8845101737855,
0.));
#130468=CARTESIAN_POINT('Ctrl Pts',(4.43994245306817,-72.8600787287318,
0.));
#130469=CARTESIAN_POINT('Ctrl Pts',(4.44812269683737,-72.8356761653069,
0.));
#130470=CARTESIAN_POINT('Ctrl Pts',(4.45626772130145,-72.8113025958262,
0.));
#130471=CARTESIAN_POINT('Ctrl Pts',(4.46437754456792,-72.7869581329994,
0.));
#130472=CARTESIAN_POINT('Ctrl Pts',(4.47245218489609,-72.7626428899281,
0.));
#130473=CARTESIAN_POINT('Ctrl Pts',(4.48049166070205,-72.738356980103,0.));
#130474=CARTESIAN_POINT('Ctrl Pts',(4.48849599055337,-72.714100517414,0.));
#130475=CARTESIAN_POINT('Ctrl Pts',(4.49646519316812,-72.6898736161542,
0.));
#130476=CARTESIAN_POINT('Ctrl Pts',(4.50439928741603,-72.6656763910241,
0.));
#130477=CARTESIAN_POINT('Ctrl Pts',(4.51229829232263,-72.6415089571321,
0.));
#130478=CARTESIAN_POINT('Ctrl Pts',(4.52016222707637,-72.6173714299942,
0.));
#130479=CARTESIAN_POINT('Ctrl Pts',(4.52799111102391,-72.5932639255409,
0.));
#130480=CARTESIAN_POINT('Ctrl Pts',(4.53578496366799,-72.5691865601223,
0.));
#130481=CARTESIAN_POINT('Ctrl Pts',(4.54354380466821,-72.5451394505104,
0.));
#130482=CARTESIAN_POINT('Ctrl Pts',(4.55126765384403,-72.5211227139001,
0.));
#130483=CARTESIAN_POINT('Ctrl Pts',(4.5589565311822,-72.4971364679068,0.));
#130484=CARTESIAN_POINT('Ctrl Pts',(4.56661045683375,-72.4731808305728,
0.));
#130485=CARTESIAN_POINT('Ctrl Pts',(4.57422945111101,-72.4492559203745,
0.));
#130486=CARTESIAN_POINT('Ctrl Pts',(4.58181353448851,-72.4253618562252,
0.));
#130487=CARTESIAN_POINT('Ctrl Pts',(4.58936272760543,-72.401498757478,0.));
#130488=CARTESIAN_POINT('Ctrl Pts',(4.59687705127329,-72.3776667439227,
0.));
#130489=CARTESIAN_POINT('Ctrl Pts',(4.60435652647452,-72.3538659357913,
0.));
#130490=CARTESIAN_POINT('Ctrl Pts',(4.61180117435862,-72.3300964537658,
0.));
#130491=CARTESIAN_POINT('Ctrl Pts',(4.61921101624291,-72.3063584189807,
0.));
#130492=CARTESIAN_POINT('Ctrl Pts',(4.62658607361465,-72.2826519530259,
0.));
#130493=CARTESIAN_POINT('Ctrl Pts',(4.63392636813843,-72.2589771779456,
0.));
#130494=CARTESIAN_POINT('Ctrl Pts',(4.64123192165627,-72.2353342162417,
0.));
#130495=CARTESIAN_POINT('Ctrl Pts',(4.64850275618323,-72.2117231908822,
0.));
#130496=CARTESIAN_POINT('Ctrl Pts',(4.65573889390821,-72.1881442253053,
0.));
#130497=CARTESIAN_POINT('Ctrl Pts',(4.66294035719569,-72.1645974434216,
0.));
#130498=CARTESIAN_POINT('Ctrl Pts',(4.67010716859284,-72.1410829696128,
0.));
#130499=CARTESIAN_POINT('Ctrl Pts',(4.67723935083094,-72.1176009287351,
0.));
#130500=CARTESIAN_POINT('Ctrl Pts',(4.68433692682068,-72.0941514461287,
0.));
#130501=CARTESIAN_POINT('Ctrl Pts',(4.69139991965283,-72.0707346476213,
0.));
#130502=CARTESIAN_POINT('Ctrl Pts',(4.69842835259991,-72.0473506595318,
0.));
#130503=CARTESIAN_POINT('Ctrl Pts',(4.705422249123,-72.0239996086686,0.));
#130504=CARTESIAN_POINT('Ctrl Pts',(4.71238163287396,-72.0006816223325,
0.));
#130505=CARTESIAN_POINT('Ctrl Pts',(4.7193065276907,-71.9773968283259,0.));
#130506=CARTESIAN_POINT('Ctrl Pts',(4.72619695759773,-71.9541453549579,
0.));
#130507=CARTESIAN_POINT('Ctrl Pts',(4.73305294680785,-71.9309273310471,
0.));
#130508=CARTESIAN_POINT('Ctrl Pts',(4.73987451972863,-71.9077428859212,
0.));
#130509=CARTESIAN_POINT('Ctrl Pts',(4.74666170096546,-71.8845921494189,
0.));
#130510=CARTESIAN_POINT('Ctrl Pts',(4.75341451531669,-71.8614752519008,
0.));
#130511=CARTESIAN_POINT('Ctrl Pts',(4.76013298777419,-71.8383923242531,
0.));
#130512=CARTESIAN_POINT('Ctrl Pts',(4.76681714352501,-71.8153434978923,
0.));
#130513=CARTESIAN_POINT('Ctrl Pts',(4.77346700795791,-71.7923289047643,
0.));
#130514=CARTESIAN_POINT('Ctrl Pts',(4.78008260666649,-71.769348677346,0.));
#130515=CARTESIAN_POINT('Ctrl Pts',(4.78666396544457,-71.7464029486563,
0.));
#130516=CARTESIAN_POINT('Ctrl Pts',(4.79321111028675,-71.723491852261,0.));
#130517=CARTESIAN_POINT('Ctrl Pts',(4.7997240673901,-71.7006155222764,0.));
#130518=CARTESIAN_POINT('Ctrl Pts',(4.80620286316074,-71.6777740933687,
0.));
#130519=CARTESIAN_POINT('Ctrl Pts',(4.81264752421712,-71.6549677007582,
0.));
#130520=CARTESIAN_POINT('Ctrl Pts',(4.81905807738541,-71.6321964802297,
0.));
#130521=CARTESIAN_POINT('Ctrl Pts',(4.8254345497002,-71.6094605681353,0.));
#130522=CARTESIAN_POINT('Ctrl Pts',(4.83177696840639,-71.5867601014008,
0.));
#130523=CARTESIAN_POINT('Ctrl Pts',(4.83808536096589,-71.5640952175239,
0.));
#130524=CARTESIAN_POINT('Ctrl Pts',(4.84435975506055,-71.5414660545778,
0.));
#130525=CARTESIAN_POINT('Ctrl Pts',(4.85060017858786,-71.5188727512231,
0.));
#130526=CARTESIAN_POINT('Ctrl Pts',(4.85680665966184,-71.4963154467128,
0.));
#130527=CARTESIAN_POINT('Ctrl Pts',(4.86297922661498,-71.4737942808971,
0.));
#130528=CARTESIAN_POINT('Ctrl Pts',(4.86911790800533,-71.4513093942216,
0.));
#130529=CARTESIAN_POINT('Ctrl Pts',(4.8752227326188,-71.4288609277324,0.));
#130530=CARTESIAN_POINT('Ctrl Pts',(4.88129372946524,-71.4064490230857,
0.));
#130531=CARTESIAN_POINT('Ctrl Pts',(4.88733092777963,-71.3840738225548,
0.));
#130532=CARTESIAN_POINT('Ctrl Pts',(4.89333435702423,-71.3617354690342,
0.));
#130533=CARTESIAN_POINT('Ctrl Pts',(4.89930404689598,-71.3394341060396,
0.));
#130534=CARTESIAN_POINT('Ctrl Pts',(4.90524002732805,-71.3171698777124,
0.));
#130535=CARTESIAN_POINT('Ctrl Pts',(4.91114232848622,-71.2949429288319,
0.));
#130536=CARTESIAN_POINT('Ctrl Pts',(4.91701098077041,-71.27275340482,0.));
#130537=CARTESIAN_POINT('Ctrl Pts',(4.92284601481709,-71.2506014517457,
0.));
#130538=CARTESIAN_POINT('Ctrl Pts',(4.9286474615071,-71.2284872163248,0.));
#130539=CARTESIAN_POINT('Ctrl Pts',(4.93441535196593,-71.206410845926,0.));
#130540=CARTESIAN_POINT('Ctrl Pts',(4.94014971756096,-71.184372488583,0.));
#130541=CARTESIAN_POINT('Ctrl Pts',(4.94585058990336,-71.1623722929998,
0.));
#130542=CARTESIAN_POINT('Ctrl Pts',(4.9515180008511,-71.1404104085561,0.));
#130543=CARTESIAN_POINT('Ctrl Pts',(4.95715198251703,-71.1184869853071,
0.));
#130544=CARTESIAN_POINT('Ctrl Pts',(4.96275256726786,-71.0966021739922,
0.));
#130545=CARTESIAN_POINT('Ctrl Pts',(4.96831978772201,-71.0747561260443,
0.));
#130546=CARTESIAN_POINT('Ctrl Pts',(4.97385367675156,-71.0529489935959,
0.));
#130547=CARTESIAN_POINT('Ctrl Pts',(4.97935426748576,-71.031180929482,0.));
#130548=CARTESIAN_POINT('Ctrl Pts',(4.9848215933185,-71.0094520872375,0.));
#130549=CARTESIAN_POINT('Ctrl Pts',(4.99025568790652,-70.9877626211112,
0.));
#130550=CARTESIAN_POINT('Ctrl Pts',(4.99565658516905,-70.9661126860773,
0.));
#130551=CARTESIAN_POINT('Ctrl Pts',(5.00102431929038,-70.9445024378439,
0.));
#130552=CARTESIAN_POINT('Ctrl Pts',(5.00635892472517,-70.9229320328588,
0.));
#130553=CARTESIAN_POINT('Ctrl Pts',(5.01166043620572,-70.9014016283123,
0.));
#130554=CARTESIAN_POINT('Ctrl Pts',(5.01692888873792,-70.8799113821449,
0.));
#130555=CARTESIAN_POINT('Ctrl Pts',(5.02216431760059,-70.8584614530517,
0.));
#130556=CARTESIAN_POINT('Ctrl Pts',(5.0273667583469,-70.8370520004844,0.));
#130557=CARTESIAN_POINT('Ctrl Pts',(5.0325362468094,-70.8156831846494,0.));
#130558=CARTESIAN_POINT('Ctrl Pts',(5.03767281910483,-70.7943551665071,
0.));
#130559=CARTESIAN_POINT('Ctrl Pts',(5.04277651163356,-70.7730681077997,
0.));
#130560=CARTESIAN_POINT('Ctrl Pts',(5.0478473610835,-70.7518221710715,0.));
#130561=CARTESIAN_POINT('Ctrl Pts',(5.05288540443477,-70.7306175196856,
0.));
#130562=CARTESIAN_POINT('Ctrl Pts',(5.0578906789704,-70.7094543178416,0.));
#130563=CARTESIAN_POINT('Ctrl Pts',(5.06286322227796,-70.6883327305755,
0.));
#130564=CARTESIAN_POINT('Ctrl Pts',(5.06780307224052,-70.6672529237431,
0.));
#130565=CARTESIAN_POINT('Ctrl Pts',(5.07271026703349,-70.6462150640009,
0.));
#130566=CARTESIAN_POINT('Ctrl Pts',(5.07758484512309,-70.6252193187892,
0.));
#130567=CARTESIAN_POINT('Ctrl Pts',(5.08242684526703,-70.6042658562951,
0.));
#130568=CARTESIAN_POINT('Ctrl Pts',(5.0872363065229,-70.5833548455043,0.));
#130569=CARTESIAN_POINT('Ctrl Pts',(5.09201326826145,-70.5624864562841,
0.));
#130570=CARTESIAN_POINT('Ctrl Pts',(5.09675777018181,-70.5416608594526,
0.));
#130571=CARTESIAN_POINT('Ctrl Pts',(5.10146985232927,-70.5208782268482,
0.));
#130572=CARTESIAN_POINT('Ctrl Pts',(5.10614955511642,-70.5001387313963,
0.));
#130573=CARTESIAN_POINT('Ctrl Pts',(5.11079691929192,-70.4794425469799,
0.));
#130574=CARTESIAN_POINT('Ctrl Pts',(5.11541198590919,-70.4587898482946,
0.));
#130575=CARTESIAN_POINT('Ctrl Pts',(5.11999479630214,-70.438180810725,0.));
#130576=CARTESIAN_POINT('Ctrl Pts',(5.12454539205346,-70.4176156101633,
0.));
#130577=CARTESIAN_POINT('Ctrl Pts',(5.12906381499485,-70.3970944229885,
0.));
#130578=CARTESIAN_POINT('Ctrl Pts',(5.1335501072859,-70.3766174264786,0.));
#130579=CARTESIAN_POINT('Ctrl Pts',(5.1380043114891,-70.3561847991725,0.));
#130580=CARTESIAN_POINT('Ctrl Pts',(5.14242647063466,-70.3357967211782,
0.));
#130581=CARTESIAN_POINT('Ctrl Pts',(5.14681662833053,-70.31545337467,0.));
#130582=CARTESIAN_POINT('Ctrl Pts',(5.15117482869224,-70.2951549435469,
0.));
#130583=CARTESIAN_POINT('Ctrl Pts',(5.15550111614837,-70.2749016125073,
0.));
#130584=CARTESIAN_POINT('Ctrl Pts',(5.159795535282,-70.2546935662719,0.));
#130585=CARTESIAN_POINT('Ctrl Pts',(5.16405813066993,-70.2345309887864,
0.));
#130586=CARTESIAN_POINT('Ctrl Pts',(5.16828894670139,-70.2144140623004,
0.));
#130587=CARTESIAN_POINT('Ctrl Pts',(5.17248802793419,-70.1943429691214,
0.));
#130588=CARTESIAN_POINT('Ctrl Pts',(5.17665541952399,-70.1743178937102,
0.));
#130589=CARTESIAN_POINT('Ctrl Pts',(5.18079116757658,-70.1543390243882,
0.));
#130590=CARTESIAN_POINT('Ctrl Pts',(5.18489531966234,-70.1344065558106,
0.));
#130591=CARTESIAN_POINT('Ctrl Pts',(5.18896792486522,-70.1145206891833,
0.));
#130592=CARTESIAN_POINT('Ctrl Pts',(5.19300903271543,-70.0946816270957,
0.));
#130593=CARTESIAN_POINT('Ctrl Pts',(5.19701869225514,-70.0748895689716,
0.));
#130594=CARTESIAN_POINT('Ctrl Pts',(5.20099695122676,-70.0551447071106,
0.));
#130595=CARTESIAN_POINT('Ctrl Pts',(5.20494385478083,-70.0354472203604,
0.));
#130596=CARTESIAN_POINT('Ctrl Pts',(5.20885944672914,-70.0157972802255,
0.));
#130597=CARTESIAN_POINT('Ctrl Pts',(5.2127437720332,-69.996195063002,0.));
#130598=CARTESIAN_POINT('Ctrl Pts',(5.21659687881138,-69.9766407595385,
0.));
#130599=CARTESIAN_POINT('Ctrl Pts',(5.22041882075626,-69.9571345869996,
0.));
#130600=CARTESIAN_POINT('Ctrl Pts',(5.22420965879807,-69.9376767968951,
0.));
#130601=CARTESIAN_POINT('Ctrl Pts',(5.22796945602602,-69.9182676501892,
0.));
#130602=CARTESIAN_POINT('Ctrl Pts',(5.23169827290451,-69.8989073936606,
0.));
#130603=CARTESIAN_POINT('Ctrl Pts',(5.23539616279714,-69.8795962381676,
0.));
#130604=CARTESIAN_POINT('Ctrl Pts',(5.2390631663514,-69.8603343303016,0.));
#130605=CARTESIAN_POINT('Ctrl Pts',(5.24269931055074,-69.8411217507931,
0.));
#130606=CARTESIAN_POINT('Ctrl Pts',(5.24558355160219,-69.8257911792542,
0.));
#130607=CARTESIAN_POINT('Ctrl Pts',(5.24773285666673,-69.8143154684447,
0.));
#130608=CARTESIAN_POINT('Ctrl Pts',(5.24915955997536,-69.8066748687863,
0.));
#130609=CARTESIAN_POINT('Ctrl Pts',(5.2498713699459,-69.8028570375098,0.));
#130610=CARTESIAN_POINT('Ctrl Pts',(-2.62535189104656,-74.4537274248118,
0.));
#130611=CARTESIAN_POINT('Ctrl Pts',(-2.62535189104656,-74.4537274248118,
12.));
#130612=CARTESIAN_POINT('Ctrl Pts',(-2.62283178248297,-74.4487312586601,
0.));
#130613=CARTESIAN_POINT('Ctrl Pts',(-2.62283178248297,-74.4487312586601,
12.));
#130614=CARTESIAN_POINT('Ctrl Pts',(-2.6177953543237,-74.4387409032582,
0.));
#130615=CARTESIAN_POINT('Ctrl Pts',(-2.6177953543237,-74.4387409032582,
12.));
#130616=CARTESIAN_POINT('Ctrl Pts',(-2.61025207898831,-74.4237613008609,
0.));
#130617=CARTESIAN_POINT('Ctrl Pts',(-2.61025207898831,-74.4237613008609,
12.));
#130618=CARTESIAN_POINT('Ctrl Pts',(-2.60021711327491,-74.4038003595514,
0.));
#130619=CARTESIAN_POINT('Ctrl Pts',(-2.60021711327491,-74.4038003595514,
12.));
#130620=CARTESIAN_POINT('Ctrl Pts',(-2.58771130268619,-74.3788689604,0.));
#130621=CARTESIAN_POINT('Ctrl Pts',(-2.58771130268619,-74.3788689604,12.));
#130622=CARTESIAN_POINT('Ctrl Pts',(-2.57524339541657,-74.3539573568054,
0.));
#130623=CARTESIAN_POINT('Ctrl Pts',(-2.57524339541657,-74.3539573568054,
12.));
#130624=CARTESIAN_POINT('Ctrl Pts',(-2.56281339800082,-74.3290655814922,
0.));
#130625=CARTESIAN_POINT('Ctrl Pts',(-2.56281339800082,-74.3290655814922,
12.));
#130626=CARTESIAN_POINT('Ctrl Pts',(-2.55042131526684,-74.3041936853329,
0.));
#130627=CARTESIAN_POINT('Ctrl Pts',(-2.55042131526684,-74.3041936853329,
12.));
#130628=CARTESIAN_POINT('Ctrl Pts',(-2.53806714838103,-74.2793417427044,
0.));
#130629=CARTESIAN_POINT('Ctrl Pts',(-2.53806714838103,-74.2793417427044,
12.));
#130630=CARTESIAN_POINT('Ctrl Pts',(-2.52575089478112,-74.2545098494549,
0.));
#130631=CARTESIAN_POINT('Ctrl Pts',(-2.52575089478112,-74.2545098494549,
12.));
#130632=CARTESIAN_POINT('Ctrl Pts',(-2.51347254956027,-74.2296981152027,
0.));
#130633=CARTESIAN_POINT('Ctrl Pts',(-2.51347254956027,-74.2296981152027,
12.));
#130634=CARTESIAN_POINT('Ctrl Pts',(-2.50123210644075,-74.2049066571942,
0.));
#130635=CARTESIAN_POINT('Ctrl Pts',(-2.50123210644075,-74.2049066571942,
12.));
#130636=CARTESIAN_POINT('Ctrl Pts',(-2.48902955888401,-74.180135593693,
0.));
#130637=CARTESIAN_POINT('Ctrl Pts',(-2.48902955888401,-74.180135593693,
12.));
#130638=CARTESIAN_POINT('Ctrl Pts',(-2.47686490120423,-74.1553850371577,
0.));
#130639=CARTESIAN_POINT('Ctrl Pts',(-2.47686490120423,-74.1553850371577,
12.));
#130640=CARTESIAN_POINT('Ctrl Pts',(-2.46473812948048,-74.1306550887196,
0.));
#130641=CARTESIAN_POINT('Ctrl Pts',(-2.46473812948048,-74.1306550887196,
12.));
#130642=CARTESIAN_POINT('Ctrl Pts',(-2.45264924094852,-74.1059458420175,
0.));
#130643=CARTESIAN_POINT('Ctrl Pts',(-2.45264924094852,-74.1059458420175,
12.));
#130644=CARTESIAN_POINT('Ctrl Pts',(-2.44059823356722,-74.0812573859474,
0.));
#130645=CARTESIAN_POINT('Ctrl Pts',(-2.44059823356722,-74.0812573859474,
12.));
#130646=CARTESIAN_POINT('Ctrl Pts',(-2.42858510549786,-74.0565898079227,
0.));
#130647=CARTESIAN_POINT('Ctrl Pts',(-2.42858510549786,-74.0565898079227,
12.));
#130648=CARTESIAN_POINT('Ctrl Pts',(-2.41660985465228,-74.0319431966956,
0.));
#130649=CARTESIAN_POINT('Ctrl Pts',(-2.41660985465228,-74.0319431966956,
12.));
#130650=CARTESIAN_POINT('Ctrl Pts',(-2.40467247811497,-74.0073176459287,
0.));
#130651=CARTESIAN_POINT('Ctrl Pts',(-2.40467247811497,-74.0073176459287,
12.));
#130652=CARTESIAN_POINT('Ctrl Pts',(-2.39277297220716,-73.9827132538149,
0.));
#130653=CARTESIAN_POINT('Ctrl Pts',(-2.39277297220716,-73.9827132538149,
12.));
#130654=CARTESIAN_POINT('Ctrl Pts',(-2.38091133274933,-73.9581301214609,
0.));
#130655=CARTESIAN_POINT('Ctrl Pts',(-2.38091133274933,-73.9581301214609,
12.));
#130656=CARTESIAN_POINT('Ctrl Pts',(-2.36908755525994,-73.9335683516388,
0.));
#130657=CARTESIAN_POINT('Ctrl Pts',(-2.36908755525994,-73.9335683516388,
12.));
#130658=CARTESIAN_POINT('Ctrl Pts',(-2.35730163516324,-73.9090280474723,
0.));
#130659=CARTESIAN_POINT('Ctrl Pts',(-2.35730163516324,-73.9090280474723,
12.));
#130660=CARTESIAN_POINT('Ctrl Pts',(-2.3455535680214,-73.8845093109302,
0.));
#130661=CARTESIAN_POINT('Ctrl Pts',(-2.3455535680214,-73.8845093109302,
12.));
#130662=CARTESIAN_POINT('Ctrl Pts',(-2.3338433496398,-73.8600122421502,
0.));
#130663=CARTESIAN_POINT('Ctrl Pts',(-2.3338433496398,-73.8600122421502,
12.));
#130664=CARTESIAN_POINT('Ctrl Pts',(-2.32217097594215,-73.8355369402733,
0.));
#130665=CARTESIAN_POINT('Ctrl Pts',(-2.32217097594215,-73.8355369402733,
12.));
#130666=CARTESIAN_POINT('Ctrl Pts',(-2.31053644289425,-73.8110835039341,
0.));
#130667=CARTESIAN_POINT('Ctrl Pts',(-2.31053644289425,-73.8110835039341,
12.));
#130668=CARTESIAN_POINT('Ctrl Pts',(-2.29893974640435,-73.7866520318849,
0.));
#130669=CARTESIAN_POINT('Ctrl Pts',(-2.29893974640435,-73.7866520318849,
12.));
#130670=CARTESIAN_POINT('Ctrl Pts',(-2.28738088222858,-73.7622426235648,
0.));
#130671=CARTESIAN_POINT('Ctrl Pts',(-2.28738088222858,-73.7622426235648,
12.));
#130672=CARTESIAN_POINT('Ctrl Pts',(-2.27585984587193,-73.7378553796792,
0.));
#130673=CARTESIAN_POINT('Ctrl Pts',(-2.27585984587193,-73.7378553796792,
12.));
#130674=CARTESIAN_POINT('Ctrl Pts',(-2.26437663263663,-73.7134904019378,
0.));
#130675=CARTESIAN_POINT('Ctrl Pts',(-2.26437663263663,-73.7134904019378,
12.));
#130676=CARTESIAN_POINT('Ctrl Pts',(-2.25293123766425,-73.6891477928124,
0.));
#130677=CARTESIAN_POINT('Ctrl Pts',(-2.25293123766425,-73.6891477928124,
12.));
#130678=CARTESIAN_POINT('Ctrl Pts',(-2.24152365597699,-73.6648276552766,
0.));
#130679=CARTESIAN_POINT('Ctrl Pts',(-2.24152365597699,-73.6648276552766,
12.));
#130680=CARTESIAN_POINT('Ctrl Pts',(-2.23015388251289,-73.6405300925714,
0.));
#130681=CARTESIAN_POINT('Ctrl Pts',(-2.23015388251289,-73.6405300925714,
12.));
#130682=CARTESIAN_POINT('Ctrl Pts',(-2.21882191216521,-73.6162552079044,
0.));
#130683=CARTESIAN_POINT('Ctrl Pts',(-2.21882191216521,-73.6162552079044,
12.));
#130684=CARTESIAN_POINT('Ctrl Pts',(-2.20752773978353,-73.5920031044604,
0.));
#130685=CARTESIAN_POINT('Ctrl Pts',(-2.20752773978353,-73.5920031044604,
12.));
#130686=CARTESIAN_POINT('Ctrl Pts',(-2.19627136015683,-73.5677738855461,
0.));
#130687=CARTESIAN_POINT('Ctrl Pts',(-2.19627136015683,-73.5677738855461,
12.));
#130688=CARTESIAN_POINT('Ctrl Pts',(-2.18505276799756,-73.5435676546934,
0.));
#130689=CARTESIAN_POINT('Ctrl Pts',(-2.18505276799756,-73.5435676546934,
12.));
#130690=CARTESIAN_POINT('Ctrl Pts',(-2.17387195792306,-73.5193845157705,
0.));
#130691=CARTESIAN_POINT('Ctrl Pts',(-2.17387195792306,-73.5193845157705,
12.));
#130692=CARTESIAN_POINT('Ctrl Pts',(-2.16272892442915,-73.4952245731044,
0.));
#130693=CARTESIAN_POINT('Ctrl Pts',(-2.16272892442915,-73.4952245731044,
12.));
#130694=CARTESIAN_POINT('Ctrl Pts',(-2.15162366187899,-73.4710879315367,
0.));
#130695=CARTESIAN_POINT('Ctrl Pts',(-2.15162366187899,-73.4710879315367,
12.));
#130696=CARTESIAN_POINT('Ctrl Pts',(-2.14055616452049,-73.4469746963622,
0.));
#130697=CARTESIAN_POINT('Ctrl Pts',(-2.14055616452049,-73.4469746963622,
12.));
#130698=CARTESIAN_POINT('Ctrl Pts',(-2.1295264264936,-73.4228849732914,
0.));
#130699=CARTESIAN_POINT('Ctrl Pts',(-2.1295264264936,-73.4228849732914,
12.));
#130700=CARTESIAN_POINT('Ctrl Pts',(-2.11853444183764,-73.3988188684022,
0.));
#130701=CARTESIAN_POINT('Ctrl Pts',(-2.11853444183764,-73.3988188684022,
12.));
#130702=CARTESIAN_POINT('Ctrl Pts',(-2.10758020449401,-73.3747764880903,
0.));
#130703=CARTESIAN_POINT('Ctrl Pts',(-2.10758020449401,-73.3747764880903,
12.));
#130704=CARTESIAN_POINT('Ctrl Pts',(-2.09666370830733,-73.3507579390254,
0.));
#130705=CARTESIAN_POINT('Ctrl Pts',(-2.09666370830733,-73.3507579390254,
12.));
#130706=CARTESIAN_POINT('Ctrl Pts',(-2.08578494702762,-73.3267633281822,
0.));
#130707=CARTESIAN_POINT('Ctrl Pts',(-2.08578494702762,-73.3267633281822,
12.));
#130708=CARTESIAN_POINT('Ctrl Pts',(-2.07494391430954,-73.3027927628636,
0.));
#130709=CARTESIAN_POINT('Ctrl Pts',(-2.07494391430954,-73.3027927628636,
12.));
#130710=CARTESIAN_POINT('Ctrl Pts',(-2.06414060370837,-73.2788463507248,
0.));
#130711=CARTESIAN_POINT('Ctrl Pts',(-2.06414060370837,-73.2788463507248,
12.));
#130712=CARTESIAN_POINT('Ctrl Pts',(-2.05337500867395,-73.2549241997946,
0.));
#130713=CARTESIAN_POINT('Ctrl Pts',(-2.05337500867395,-73.2549241997946,
12.));
#130714=CARTESIAN_POINT('Ctrl Pts',(-2.04264712253915,-73.2310264184965,
0.));
#130715=CARTESIAN_POINT('Ctrl Pts',(-2.04264712253915,-73.2310264184965,
12.));
#130716=CARTESIAN_POINT('Ctrl Pts',(-2.0319569385244,-73.2071531156492,
0.));
#130717=CARTESIAN_POINT('Ctrl Pts',(-2.0319569385244,-73.2071531156492,
12.));
#130718=CARTESIAN_POINT('Ctrl Pts',(-2.02130444974352,-73.1833044004612,
0.));
#130719=CARTESIAN_POINT('Ctrl Pts',(-2.02130444974352,-73.1833044004612,
12.));
#130720=CARTESIAN_POINT('Ctrl Pts',(-2.01068964920465,-73.159480382525,
0.));
#130721=CARTESIAN_POINT('Ctrl Pts',(-2.01068964920465,-73.159480382525,
12.));
#130722=CARTESIAN_POINT('Ctrl Pts',(-2.00011252980987,-73.1356811718094,
0.));
#130723=CARTESIAN_POINT('Ctrl Pts',(-2.00011252980987,-73.1356811718094,
12.));
#130724=CARTESIAN_POINT('Ctrl Pts',(-1.9895730843493,-73.1119068786482,
0.));
#130725=CARTESIAN_POINT('Ctrl Pts',(-1.9895730843493,-73.1119068786482,
12.));
#130726=CARTESIAN_POINT('Ctrl Pts',(-1.97907130550172,-73.0881576137415,
0.));
#130727=CARTESIAN_POINT('Ctrl Pts',(-1.97907130550172,-73.0881576137415,
12.));
#130728=CARTESIAN_POINT('Ctrl Pts',(-1.96860718583944,-73.0644334881679,
0.));
#130729=CARTESIAN_POINT('Ctrl Pts',(-1.96860718583944,-73.0644334881679,
12.));
#130730=CARTESIAN_POINT('Ctrl Pts',(-1.95818071782773,-73.0407346133912,
0.));
#130731=CARTESIAN_POINT('Ctrl Pts',(-1.95818071782773,-73.0407346133912,
12.));
#130732=CARTESIAN_POINT('Ctrl Pts',(-1.947791893823,-73.0170611012659,0.));
#130733=CARTESIAN_POINT('Ctrl Pts',(-1.947791893823,-73.0170611012659,12.));
#130734=CARTESIAN_POINT('Ctrl Pts',(-1.93744070606557,-72.9934130640414,
0.));
#130735=CARTESIAN_POINT('Ctrl Pts',(-1.93744070606557,-72.9934130640414,
12.));
#130736=CARTESIAN_POINT('Ctrl Pts',(-1.92712714667648,-72.9697906143638,
0.));
#130737=CARTESIAN_POINT('Ctrl Pts',(-1.92712714667648,-72.9697906143638,
12.));
#130738=CARTESIAN_POINT('Ctrl Pts',(-1.91685120766428,-72.9461938652816,
0.));
#130739=CARTESIAN_POINT('Ctrl Pts',(-1.91685120766428,-72.9461938652816,
12.));
#130740=CARTESIAN_POINT('Ctrl Pts',(-1.90661288092583,-72.9226229302483,
0.));
#130741=CARTESIAN_POINT('Ctrl Pts',(-1.90661288092583,-72.9226229302483,
12.));
#130742=CARTESIAN_POINT('Ctrl Pts',(-1.89641215824584,-72.8990779231226,
0.));
#130743=CARTESIAN_POINT('Ctrl Pts',(-1.89641215824584,-72.8990779231226,
12.));
#130744=CARTESIAN_POINT('Ctrl Pts',(-1.88624903129195,-72.8755589581674,
0.));
#130745=CARTESIAN_POINT('Ctrl Pts',(-1.88624903129195,-72.8755589581674,
12.));
#130746=CARTESIAN_POINT('Ctrl Pts',(-1.87612349160952,-72.8520661500465,
0.));
#130747=CARTESIAN_POINT('Ctrl Pts',(-1.87612349160952,-72.8520661500465,
12.));
#130748=CARTESIAN_POINT('Ctrl Pts',(-1.86603553062776,-72.8285996138346,
0.));
#130749=CARTESIAN_POINT('Ctrl Pts',(-1.86603553062776,-72.8285996138346,
12.));
#130750=CARTESIAN_POINT('Ctrl Pts',(-1.85598513966115,-72.8051594650214,
0.));
#130751=CARTESIAN_POINT('Ctrl Pts',(-1.85598513966115,-72.8051594650214,
12.));
#130752=CARTESIAN_POINT('Ctrl Pts',(-1.84597230990858,-72.7817458195155,
0.));
#130753=CARTESIAN_POINT('Ctrl Pts',(-1.84597230990858,-72.7817458195155,
12.));
#130754=CARTESIAN_POINT('Ctrl Pts',(-1.83599703244926,-72.7583587936454,
0.));
#130755=CARTESIAN_POINT('Ctrl Pts',(-1.83599703244926,-72.7583587936454,
12.));
#130756=CARTESIAN_POINT('Ctrl Pts',(-1.82605929823565,-72.73499850416,0.));
#130757=CARTESIAN_POINT('Ctrl Pts',(-1.82605929823565,-72.73499850416,12.));
#130758=CARTESIAN_POINT('Ctrl Pts',(-1.81615909809872,-72.7116650682347,
0.));
#130759=CARTESIAN_POINT('Ctrl Pts',(-1.81615909809872,-72.7116650682347,
12.));
#130760=CARTESIAN_POINT('Ctrl Pts',(-1.80629642275051,-72.6883586034768,
0.));
#130761=CARTESIAN_POINT('Ctrl Pts',(-1.80629642275051,-72.6883586034768,
12.));
#130762=CARTESIAN_POINT('Ctrl Pts',(-1.79647126278359,-72.6650792279271,
0.));
#130763=CARTESIAN_POINT('Ctrl Pts',(-1.79647126278359,-72.6650792279271,
12.));
#130764=CARTESIAN_POINT('Ctrl Pts',(-1.78668360866813,-72.6418270600623,
0.));
#130765=CARTESIAN_POINT('Ctrl Pts',(-1.78668360866813,-72.6418270600623,
12.));
#130766=CARTESIAN_POINT('Ctrl Pts',(-1.7769334507443,-72.618602218792,0.));
#130767=CARTESIAN_POINT('Ctrl Pts',(-1.7769334507443,-72.618602218792,12.));
#130768=CARTESIAN_POINT('Ctrl Pts',(-1.7672207792258,-72.5954048234655,
0.));
#130769=CARTESIAN_POINT('Ctrl Pts',(-1.7672207792258,-72.5954048234655,
12.));
#130770=CARTESIAN_POINT('Ctrl Pts',(-1.7575455842035,-72.5722349938789,
0.));
#130771=CARTESIAN_POINT('Ctrl Pts',(-1.7575455842035,-72.5722349938789,
12.));
#130772=CARTESIAN_POINT('Ctrl Pts',(-1.74790785564476,-72.5490928502773,
0.));
#130773=CARTESIAN_POINT('Ctrl Pts',(-1.74790785564476,-72.5490928502773,
12.));
#130774=CARTESIAN_POINT('Ctrl Pts',(-1.73830758339123,-72.5259785133586,
0.));
#130775=CARTESIAN_POINT('Ctrl Pts',(-1.73830758339123,-72.5259785133586,
12.));
#130776=CARTESIAN_POINT('Ctrl Pts',(-1.72874475715098,-72.5028921042704,
0.));
#130777=CARTESIAN_POINT('Ctrl Pts',(-1.72874475715098,-72.5028921042704,
12.));
#130778=CARTESIAN_POINT('Ctrl Pts',(-1.71921936650032,-72.4798337446162,
0.));
#130779=CARTESIAN_POINT('Ctrl Pts',(-1.71921936650032,-72.4798337446162,
12.));
#130780=CARTESIAN_POINT('Ctrl Pts',(-1.70973140088837,-72.4568035564618,
0.));
#130781=CARTESIAN_POINT('Ctrl Pts',(-1.70973140088837,-72.4568035564618,
12.));
#130782=CARTESIAN_POINT('Ctrl Pts',(-1.70028084963647,-72.4338016623388,
0.));
#130783=CARTESIAN_POINT('Ctrl Pts',(-1.70028084963647,-72.4338016623388,
12.));
#130784=CARTESIAN_POINT('Ctrl Pts',(-1.69086770193641,-72.4108281852473,
0.));
#130785=CARTESIAN_POINT('Ctrl Pts',(-1.69086770193641,-72.4108281852473,
12.));
#130786=CARTESIAN_POINT('Ctrl Pts',(-1.68149194684288,-72.3878832486549,
0.));
#130787=CARTESIAN_POINT('Ctrl Pts',(-1.68149194684288,-72.3878832486549,
12.));
#130788=CARTESIAN_POINT('Ctrl Pts',(-1.67215357327372,-72.3649669765013,
0.));
#130789=CARTESIAN_POINT('Ctrl Pts',(-1.67215357327372,-72.3649669765013,
12.));
#130790=CARTESIAN_POINT('Ctrl Pts',(-1.66285257001502,-72.3420794932052,
0.));
#130791=CARTESIAN_POINT('Ctrl Pts',(-1.66285257001502,-72.3420794932052,
12.));
#130792=CARTESIAN_POINT('Ctrl Pts',(-1.65358892572066,-72.3192209236691,
0.));
#130793=CARTESIAN_POINT('Ctrl Pts',(-1.65358892572066,-72.3192209236691,
12.));
#130794=CARTESIAN_POINT('Ctrl Pts',(-1.64436262891078,-72.2963913932811,
0.));
#130795=CARTESIAN_POINT('Ctrl Pts',(-1.64436262891078,-72.2963913932811,
12.));
#130796=CARTESIAN_POINT('Ctrl Pts',(-1.63517366796459,-72.2735910279149,
0.));
#130797=CARTESIAN_POINT('Ctrl Pts',(-1.63517366796459,-72.2735910279149,
12.));
#130798=CARTESIAN_POINT('Ctrl Pts',(-1.62602203111924,-72.2508199539325,
0.));
#130799=CARTESIAN_POINT('Ctrl Pts',(-1.62602203111924,-72.2508199539325,
12.));
#130800=CARTESIAN_POINT('Ctrl Pts',(-1.61690770647536,-72.2280782981941,
0.));
#130801=CARTESIAN_POINT('Ctrl Pts',(-1.61690770647536,-72.2280782981941,
12.));
#130802=CARTESIAN_POINT('Ctrl Pts',(-1.60783068199662,-72.2053661880611,
0.));
#130803=CARTESIAN_POINT('Ctrl Pts',(-1.60783068199662,-72.2053661880611,
12.));
#130804=CARTESIAN_POINT('Ctrl Pts',(-1.5987909455085,-72.1826837514,0.));
#130805=CARTESIAN_POINT('Ctrl Pts',(-1.5987909455085,-72.1826837514,12.));
#130806=CARTESIAN_POINT('Ctrl Pts',(-1.58978848469128,-72.1600311165813,
0.));
#130807=CARTESIAN_POINT('Ctrl Pts',(-1.58978848469128,-72.1600311165813,
12.));
#130808=CARTESIAN_POINT('Ctrl Pts',(-1.58082328707808,-72.1374084124829,
0.));
#130809=CARTESIAN_POINT('Ctrl Pts',(-1.58082328707808,-72.1374084124829,
12.));
#130810=CARTESIAN_POINT('Ctrl Pts',(-1.57189534006043,-72.1148157684987,
0.));
#130811=CARTESIAN_POINT('Ctrl Pts',(-1.57189534006043,-72.1148157684987,
12.));
#130812=CARTESIAN_POINT('Ctrl Pts',(-1.56300463088811,-72.092253314543,
0.));
#130813=CARTESIAN_POINT('Ctrl Pts',(-1.56300463088811,-72.092253314543,
12.));
#130814=CARTESIAN_POINT('Ctrl Pts',(-1.55415114666774,-72.0697211810548,
0.));
#130815=CARTESIAN_POINT('Ctrl Pts',(-1.55415114666774,-72.0697211810548,
12.));
#130816=CARTESIAN_POINT('Ctrl Pts',(-1.54533487435626,-72.0472194989968,
0.));
#130817=CARTESIAN_POINT('Ctrl Pts',(-1.54533487435626,-72.0472194989968,
12.));
#130818=CARTESIAN_POINT('Ctrl Pts',(-1.53655580075814,-72.0247483998582,
0.));
#130819=CARTESIAN_POINT('Ctrl Pts',(-1.53655580075814,-72.0247483998582,
12.));
#130820=CARTESIAN_POINT('Ctrl Pts',(-1.52781391253103,-72.0023080156647,
0.));
#130821=CARTESIAN_POINT('Ctrl Pts',(-1.52781391253103,-72.0023080156647,
12.));
#130822=CARTESIAN_POINT('Ctrl Pts',(-1.51910919618567,-71.9798984789828,
0.));
#130823=CARTESIAN_POINT('Ctrl Pts',(-1.51910919618567,-71.9798984789828,
12.));
#130824=CARTESIAN_POINT('Ctrl Pts',(-1.51044163808455,-71.9575199229241,
0.));
#130825=CARTESIAN_POINT('Ctrl Pts',(-1.51044163808455,-71.9575199229241,
12.));
#130826=CARTESIAN_POINT('Ctrl Pts',(-1.50181122443535,-71.935172481145,
0.));
#130827=CARTESIAN_POINT('Ctrl Pts',(-1.50181122443535,-71.935172481145,
12.));
#130828=CARTESIAN_POINT('Ctrl Pts',(-1.493217941288,-71.9128562878491,0.));
#130829=CARTESIAN_POINT('Ctrl Pts',(-1.493217941288,-71.9128562878491,12.));
#130830=CARTESIAN_POINT('Ctrl Pts',(-1.48466177454021,-71.8905714777972,
0.));
#130831=CARTESIAN_POINT('Ctrl Pts',(-1.48466177454021,-71.8905714777972,
12.));
#130832=CARTESIAN_POINT('Ctrl Pts',(-1.4761427099373,-71.8683181863123,
0.));
#130833=CARTESIAN_POINT('Ctrl Pts',(-1.4761427099373,-71.8683181863123,
12.));
#130834=CARTESIAN_POINT('Ctrl Pts',(-1.46766073307089,-71.8460965492836,
0.));
#130835=CARTESIAN_POINT('Ctrl Pts',(-1.46766073307089,-71.8460965492836,
12.));
#130836=CARTESIAN_POINT('Ctrl Pts',(-1.45921582937229,-71.8239067031664,
0.));
#130837=CARTESIAN_POINT('Ctrl Pts',(-1.45921582937229,-71.8239067031664,
12.));
#130838=CARTESIAN_POINT('Ctrl Pts',(-1.45080798410957,-71.8017487849865,
0.));
#130839=CARTESIAN_POINT('Ctrl Pts',(-1.45080798410957,-71.8017487849865,
12.));
#130840=CARTESIAN_POINT('Ctrl Pts',(-1.44243718239305,-71.7796229323496,
0.));
#130841=CARTESIAN_POINT('Ctrl Pts',(-1.44243718239305,-71.7796229323496,
12.));
#130842=CARTESIAN_POINT('Ctrl Pts',(-1.43410340917489,-71.7575292834456,
0.));
#130843=CARTESIAN_POINT('Ctrl Pts',(-1.43410340917489,-71.7575292834456,
12.));
#130844=CARTESIAN_POINT('Ctrl Pts',(-1.42580664924774,-71.7354679770537,
0.));
#130845=CARTESIAN_POINT('Ctrl Pts',(-1.42580664924774,-71.7354679770537,
12.));
#130846=CARTESIAN_POINT('Ctrl Pts',(-1.41754688723791,-71.7134391525417,
0.));
#130847=CARTESIAN_POINT('Ctrl Pts',(-1.41754688723791,-71.7134391525417,
12.));
#130848=CARTESIAN_POINT('Ctrl Pts',(-1.40932410760275,-71.6914429498702,
0.));
#130849=CARTESIAN_POINT('Ctrl Pts',(-1.40932410760275,-71.6914429498702,
12.));
#130850=CARTESIAN_POINT('Ctrl Pts',(-1.401138294636,-71.6694795096034,0.));
#130851=CARTESIAN_POINT('Ctrl Pts',(-1.401138294636,-71.6694795096034,12.));
#130852=CARTESIAN_POINT('Ctrl Pts',(-1.39298943246731,-71.6475489729149,
0.));
#130853=CARTESIAN_POINT('Ctrl Pts',(-1.39298943246731,-71.6475489729149,
12.));
#130854=CARTESIAN_POINT('Ctrl Pts',(-1.38487750506076,-71.6256514815918,
0.));
#130855=CARTESIAN_POINT('Ctrl Pts',(-1.38487750506076,-71.6256514815918,
12.));
#130856=CARTESIAN_POINT('Ctrl Pts',(-1.37680249620763,-71.6037871780347,
0.));
#130857=CARTESIAN_POINT('Ctrl Pts',(-1.37680249620763,-71.6037871780347,
12.));
#130858=CARTESIAN_POINT('Ctrl Pts',(-1.36876438952449,-71.5819562052613,
0.));
#130859=CARTESIAN_POINT('Ctrl Pts',(-1.36876438952449,-71.5819562052613,
12.));
#130860=CARTESIAN_POINT('Ctrl Pts',(-1.36076316845806,-71.5601587069175,
0.));
#130861=CARTESIAN_POINT('Ctrl Pts',(-1.36076316845806,-71.5601587069175,
12.));
#130862=CARTESIAN_POINT('Ctrl Pts',(-1.35279881628453,-71.538394827283,
0.));
#130863=CARTESIAN_POINT('Ctrl Pts',(-1.35279881628453,-71.538394827283,
12.));
#130864=CARTESIAN_POINT('Ctrl Pts',(-1.34487131610785,-71.5166647112766,
0.));
#130865=CARTESIAN_POINT('Ctrl Pts',(-1.34487131610785,-71.5166647112766,
12.));
#130866=CARTESIAN_POINT('Ctrl Pts',(-1.33698065085228,-71.4949685044559,
0.));
#130867=CARTESIAN_POINT('Ctrl Pts',(-1.33698065085228,-71.4949685044559,
12.));
#130868=CARTESIAN_POINT('Ctrl Pts',(-1.32912680326131,-71.4733063530227,
0.));
#130869=CARTESIAN_POINT('Ctrl Pts',(-1.32912680326131,-71.4733063530227,
12.));
#130870=CARTESIAN_POINT('Ctrl Pts',(-1.32130975590231,-71.4516784038346,
0.));
#130871=CARTESIAN_POINT('Ctrl Pts',(-1.32130975590231,-71.4516784038346,
12.));
#130872=CARTESIAN_POINT('Ctrl Pts',(-1.31352949116539,-71.4300848044095,
0.));
#130873=CARTESIAN_POINT('Ctrl Pts',(-1.31352949116539,-71.4300848044095,
12.));
#130874=CARTESIAN_POINT('Ctrl Pts',(-1.30578599126139,-71.4085257029308,
0.));
#130875=CARTESIAN_POINT('Ctrl Pts',(-1.30578599126139,-71.4085257029308,
12.));
#130876=CARTESIAN_POINT('Ctrl Pts',(-1.29807923821414,-71.3870012482474,
0.));
#130877=CARTESIAN_POINT('Ctrl Pts',(-1.29807923821414,-71.3870012482474,
12.));
#130878=CARTESIAN_POINT('Ctrl Pts',(-1.29040921386061,-71.3655115898801,
0.));
#130879=CARTESIAN_POINT('Ctrl Pts',(-1.29040921386061,-71.3655115898801,
12.));
#130880=CARTESIAN_POINT('Ctrl Pts',(-1.28277589985475,-71.344056878033,
0.));
#130881=CARTESIAN_POINT('Ctrl Pts',(-1.28277589985475,-71.344056878033,
12.));
#130882=CARTESIAN_POINT('Ctrl Pts',(-1.27517927766611,-71.3226372635993,
0.));
#130883=CARTESIAN_POINT('Ctrl Pts',(-1.27517927766611,-71.3226372635993,
12.));
#130884=CARTESIAN_POINT('Ctrl Pts',(-1.26761932857723,-71.301252898167,
0.));
#130885=CARTESIAN_POINT('Ctrl Pts',(-1.26761932857723,-71.301252898167,
12.));
#130886=CARTESIAN_POINT('Ctrl Pts',(-1.26009603367565,-71.2799039340191,
0.));
#130887=CARTESIAN_POINT('Ctrl Pts',(-1.26009603367565,-71.2799039340191,
12.));
#130888=CARTESIAN_POINT('Ctrl Pts',(-1.25260937385561,-71.2585905241422,
0.));
#130889=CARTESIAN_POINT('Ctrl Pts',(-1.25260937385561,-71.2585905241422,
12.));
#130890=CARTESIAN_POINT('Ctrl Pts',(-1.24515932982108,-71.2373128222359,
0.));
#130891=CARTESIAN_POINT('Ctrl Pts',(-1.24515932982108,-71.2373128222359,
12.));
#130892=CARTESIAN_POINT('Ctrl Pts',(-1.23774588208427,-71.2160709827189,
0.));
#130893=CARTESIAN_POINT('Ctrl Pts',(-1.23774588208427,-71.2160709827189,
12.));
#130894=CARTESIAN_POINT('Ctrl Pts',(-1.23036901096246,-71.1948651607319,
0.));
#130895=CARTESIAN_POINT('Ctrl Pts',(-1.23036901096246,-71.1948651607319,
12.));
#130896=CARTESIAN_POINT('Ctrl Pts',(-1.22302869657028,-71.1736955121361,
0.));
#130897=CARTESIAN_POINT('Ctrl Pts',(-1.22302869657028,-71.1736955121361,
12.));
#130898=CARTESIAN_POINT('Ctrl Pts',(-1.21572491882273,-71.1525621935266,
0.));
#130899=CARTESIAN_POINT('Ctrl Pts',(-1.21572491882273,-71.1525621935266,
12.));
#130900=CARTESIAN_POINT('Ctrl Pts',(-1.20845765743654,-71.1314653622442,
0.));
#130901=CARTESIAN_POINT('Ctrl Pts',(-1.20845765743654,-71.1314653622442,
12.));
#130902=CARTESIAN_POINT('Ctrl Pts',(-1.20122689192836,-71.1104051763839,
0.));
#130903=CARTESIAN_POINT('Ctrl Pts',(-1.20122689192836,-71.1104051763839,
12.));
#130904=CARTESIAN_POINT('Ctrl Pts',(-1.19403260160998,-71.089381794801,
0.));
#130905=CARTESIAN_POINT('Ctrl Pts',(-1.19403260160998,-71.089381794801,
12.));
#130906=CARTESIAN_POINT('Ctrl Pts',(-1.18687476558127,-71.0683953771147,
0.));
#130907=CARTESIAN_POINT('Ctrl Pts',(-1.18687476558127,-71.0683953771147,
12.));
#130908=CARTESIAN_POINT('Ctrl Pts',(-1.179753362735,-71.0474460837157,0.));
#130909=CARTESIAN_POINT('Ctrl Pts',(-1.179753362735,-71.0474460837157,12.));
#130910=CARTESIAN_POINT('Ctrl Pts',(-1.17266837175776,-71.0265340757697,
0.));
#130911=CARTESIAN_POINT('Ctrl Pts',(-1.17266837175776,-71.0265340757697,
12.));
#130912=CARTESIAN_POINT('Ctrl Pts',(-1.16561977112882,-71.0056595152204,
0.));
#130913=CARTESIAN_POINT('Ctrl Pts',(-1.16561977112882,-71.0056595152204,
12.));
#130914=CARTESIAN_POINT('Ctrl Pts',(-1.1586075391149,-70.9848225647876,
0.));
#130915=CARTESIAN_POINT('Ctrl Pts',(-1.1586075391149,-70.9848225647876,
12.));
#130916=CARTESIAN_POINT('Ctrl Pts',(-1.1516316537653,-70.9640233879671,
0.));
#130917=CARTESIAN_POINT('Ctrl Pts',(-1.1516316537653,-70.9640233879671,
12.));
#130918=CARTESIAN_POINT('Ctrl Pts',(-1.14469209291494,-70.943262149058,
0.));
#130919=CARTESIAN_POINT('Ctrl Pts',(-1.14469209291494,-70.943262149058,
12.));
#130920=CARTESIAN_POINT('Ctrl Pts',(-1.13778883418216,-70.9225390131835,
0.));
#130921=CARTESIAN_POINT('Ctrl Pts',(-1.13778883418216,-70.9225390131835,
12.));
#130922=CARTESIAN_POINT('Ctrl Pts',(-1.13092185496563,-70.9018541463083,
0.));
#130923=CARTESIAN_POINT('Ctrl Pts',(-1.13092185496563,-70.9018541463083,
12.));
#130924=CARTESIAN_POINT('Ctrl Pts',(-1.12409113243511,-70.8812077152564,
0.));
#130925=CARTESIAN_POINT('Ctrl Pts',(-1.12409113243511,-70.8812077152564,
12.));
#130926=CARTESIAN_POINT('Ctrl Pts',(-1.1172966435299,-70.860599887712,0.));
#130927=CARTESIAN_POINT('Ctrl Pts',(-1.1172966435299,-70.860599887712,12.));
#130928=CARTESIAN_POINT('Ctrl Pts',(-1.11053836496638,-70.8400308322013,
0.));
#130929=CARTESIAN_POINT('Ctrl Pts',(-1.11053836496638,-70.8400308322013,
12.));
#130930=CARTESIAN_POINT('Ctrl Pts',(-1.10381627323946,-70.8195007180739,
0.));
#130931=CARTESIAN_POINT('Ctrl Pts',(-1.10381627323946,-70.8195007180739,
12.));
#130932=CARTESIAN_POINT('Ctrl Pts',(-1.0971303446227,-70.7990097154855,
0.));
#130933=CARTESIAN_POINT('Ctrl Pts',(-1.0971303446227,-70.7990097154855,
12.));
#130934=CARTESIAN_POINT('Ctrl Pts',(-1.09048055516434,-70.7785579953611,
0.));
#130935=CARTESIAN_POINT('Ctrl Pts',(-1.09048055516434,-70.7785579953611,
12.));
#130936=CARTESIAN_POINT('Ctrl Pts',(-1.08386688068349,-70.7581457294475,
0.));
#130937=CARTESIAN_POINT('Ctrl Pts',(-1.08386688068349,-70.7581457294475,
12.));
#130938=CARTESIAN_POINT('Ctrl Pts',(-1.07728929676412,-70.737773090397,
0.));
#130939=CARTESIAN_POINT('Ctrl Pts',(-1.07728929676412,-70.737773090397,
12.));
#130940=CARTESIAN_POINT('Ctrl Pts',(-1.07074777874596,-70.7174402518378,
0.));
#130941=CARTESIAN_POINT('Ctrl Pts',(-1.07074777874596,-70.7174402518378,
12.));
#130942=CARTESIAN_POINT('Ctrl Pts',(-1.0642423017128,-70.6971473884443,
0.));
#130943=CARTESIAN_POINT('Ctrl Pts',(-1.0642423017128,-70.6971473884443,
12.));
#130944=CARTESIAN_POINT('Ctrl Pts',(-1.05777284047728,-70.6768946760063,
0.));
#130945=CARTESIAN_POINT('Ctrl Pts',(-1.05777284047728,-70.6768946760063,
12.));
#130946=CARTESIAN_POINT('Ctrl Pts',(-1.05133936960069,-70.6566822912965,
0.));
#130947=CARTESIAN_POINT('Ctrl Pts',(-1.05133936960069,-70.6566822912965,
12.));
#130948=CARTESIAN_POINT('Ctrl Pts',(-1.04494186341156,-70.6365104119238,
0.));
#130949=CARTESIAN_POINT('Ctrl Pts',(-1.04494186341156,-70.6365104119238,
12.));
#130950=CARTESIAN_POINT('Ctrl Pts',(-1.03858029601906,-70.6163792162079,
0.));
#130951=CARTESIAN_POINT('Ctrl Pts',(-1.03858029601906,-70.6163792162079,
12.));
#130952=CARTESIAN_POINT('Ctrl Pts',(-1.03225464132872,-70.5962888829958,
0.));
#130953=CARTESIAN_POINT('Ctrl Pts',(-1.03225464132872,-70.5962888829958,
12.));
#130954=CARTESIAN_POINT('Ctrl Pts',(-1.02596487304049,-70.5762395916412,
0.));
#130955=CARTESIAN_POINT('Ctrl Pts',(-1.02596487304049,-70.5762395916412,
12.));
#130956=CARTESIAN_POINT('Ctrl Pts',(-1.01971096460599,-70.5562315224219,
0.));
#130957=CARTESIAN_POINT('Ctrl Pts',(-1.01971096460599,-70.5562315224219,
12.));
#130958=CARTESIAN_POINT('Ctrl Pts',(-1.0134928891854,-70.5362648569072,
0.));
#130959=CARTESIAN_POINT('Ctrl Pts',(-1.0134928891854,-70.5362648569072,
12.));
#130960=CARTESIAN_POINT('Ctrl Pts',(-1.00731061960968,-70.5163397782699,
0.));
#130961=CARTESIAN_POINT('Ctrl Pts',(-1.00731061960968,-70.5163397782699,
12.));
#130962=CARTESIAN_POINT('Ctrl Pts',(-1.00116412831438,-70.4964564717917,
0.));
#130963=CARTESIAN_POINT('Ctrl Pts',(-1.00116412831438,-70.4964564717917,
12.));
#130964=CARTESIAN_POINT('Ctrl Pts',(-0.995053387379681,-70.476615124517,
0.));
#130965=CARTESIAN_POINT('Ctrl Pts',(-0.995053387379681,-70.476615124517,
12.));
#130966=CARTESIAN_POINT('Ctrl Pts',(-0.98897836864359,-70.4568159243131,
0.));
#130967=CARTESIAN_POINT('Ctrl Pts',(-0.98897836864359,-70.4568159243131,
12.));
#130968=CARTESIAN_POINT('Ctrl Pts',(-0.982939043792158,-70.4370590590839,
0.));
#130969=CARTESIAN_POINT('Ctrl Pts',(-0.982939043792158,-70.4370590590839,
12.));
#130970=CARTESIAN_POINT('Ctrl Pts',(-0.976935384450128,-70.41734471596,
0.));
#130971=CARTESIAN_POINT('Ctrl Pts',(-0.976935384450128,-70.41734471596,
12.));
#130972=CARTESIAN_POINT('Ctrl Pts',(-0.970967362281301,-70.3976730803664,
0.));
#130973=CARTESIAN_POINT('Ctrl Pts',(-0.970967362281301,-70.3976730803664,
12.));
#130974=CARTESIAN_POINT('Ctrl Pts',(-0.965034948786559,-70.3780443378003,
0.));
#130975=CARTESIAN_POINT('Ctrl Pts',(-0.965034948786559,-70.3780443378003,
12.));
#130976=CARTESIAN_POINT('Ctrl Pts',(-0.959138115058886,-70.3584586759561,
0.));
#130977=CARTESIAN_POINT('Ctrl Pts',(-0.959138115058886,-70.3584586759561,
12.));
#130978=CARTESIAN_POINT('Ctrl Pts',(-0.953276831581232,-70.338916286457,
0.));
#130979=CARTESIAN_POINT('Ctrl Pts',(-0.953276831581232,-70.338916286457,
12.));
#130980=CARTESIAN_POINT('Ctrl Pts',(-0.947451067929564,-70.3194173673635,
0.));
#130981=CARTESIAN_POINT('Ctrl Pts',(-0.947451067929564,-70.3194173673635,
12.));
#130982=CARTESIAN_POINT('Ctrl Pts',(-0.941660792742953,-70.2999621233938,
0.));
#130983=CARTESIAN_POINT('Ctrl Pts',(-0.941660792742953,-70.2999621233938,
12.));
#130984=CARTESIAN_POINT('Ctrl Pts',(-0.935905974336492,-70.2805507606832,
0.));
#130985=CARTESIAN_POINT('Ctrl Pts',(-0.935905974336492,-70.2805507606832,
12.));
#130986=CARTESIAN_POINT('Ctrl Pts',(-0.930186581235576,-70.2611834821711,
0.));
#130987=CARTESIAN_POINT('Ctrl Pts',(-0.930186581235576,-70.2611834821711,
12.));
#130988=CARTESIAN_POINT('Ctrl Pts',(-0.924502582639453,-70.241860483586,
0.));
#130989=CARTESIAN_POINT('Ctrl Pts',(-0.924502582639453,-70.241860483586,
12.));
#130990=CARTESIAN_POINT('Ctrl Pts',(-0.918853949157045,-70.2225819470306,
0.));
#130991=CARTESIAN_POINT('Ctrl Pts',(-0.918853949157045,-70.2225819470306,
12.));
#130992=CARTESIAN_POINT('Ctrl Pts',(-0.913240652090839,-70.2033480471749,
0.));
#130993=CARTESIAN_POINT('Ctrl Pts',(-0.913240652090839,-70.2033480471749,
12.));
#130994=CARTESIAN_POINT('Ctrl Pts',(-0.90766266201565,-70.184158963563,
0.));
#130995=CARTESIAN_POINT('Ctrl Pts',(-0.90766266201565,-70.184158963563,
12.));
#130996=CARTESIAN_POINT('Ctrl Pts',(-0.902119947629773,-70.1650148905109,
0.));
#130997=CARTESIAN_POINT('Ctrl Pts',(-0.902119947629773,-70.1650148905109,
12.));
#130998=CARTESIAN_POINT('Ctrl Pts',(-0.896612474372085,-70.1459160490366,
0.));
#130999=CARTESIAN_POINT('Ctrl Pts',(-0.896612474372085,-70.1459160490366,
12.));
#131000=CARTESIAN_POINT('Ctrl Pts',(-0.891140203464724,-70.1268626950031,
0.));
#131001=CARTESIAN_POINT('Ctrl Pts',(-0.891140203464724,-70.1268626950031,
12.));
#131002=CARTESIAN_POINT('Ctrl Pts',(-0.885703094803086,-70.1078550938801,
0.));
#131003=CARTESIAN_POINT('Ctrl Pts',(-0.885703094803086,-70.1078550938801,
12.));
#131004=CARTESIAN_POINT('Ctrl Pts',(-0.880301109661037,-70.0888934967772,
0.));
#131005=CARTESIAN_POINT('Ctrl Pts',(-0.880301109661037,-70.0888934967772,
12.));
#131006=CARTESIAN_POINT('Ctrl Pts',(-0.87493421325557,-70.0699781184013,
0.));
#131007=CARTESIAN_POINT('Ctrl Pts',(-0.87493421325557,-70.0699781184013,
12.));
#131008=CARTESIAN_POINT('Ctrl Pts',(-0.869602377870139,-70.0511091083285,
0.));
#131009=CARTESIAN_POINT('Ctrl Pts',(-0.869602377870139,-70.0511091083285,
12.));
#131010=CARTESIAN_POINT('Ctrl Pts',(-0.86430558366009,-70.0322865493339,
0.));
#131011=CARTESIAN_POINT('Ctrl Pts',(-0.86430558366009,-70.0322865493339,
12.));
#131012=CARTESIAN_POINT('Ctrl Pts',(-0.860096170667398,-70.0172656934192,
0.));
#131013=CARTESIAN_POINT('Ctrl Pts',(-0.860096170667398,-70.0172656934192,
12.));
#131014=CARTESIAN_POINT('Ctrl Pts',(-0.856954870258371,-70.0060209754332,
0.));
#131015=CARTESIAN_POINT('Ctrl Pts',(-0.856954870258371,-70.0060209754332,
12.));
#131016=CARTESIAN_POINT('Ctrl Pts',(-0.854867673848293,-69.9985337959499,
0.));
#131017=CARTESIAN_POINT('Ctrl Pts',(-0.854867673848293,-69.9985337959499,
12.));
#131018=CARTESIAN_POINT('Ctrl Pts',(-0.853825826608993,-69.9947925310006,
0.));
#131019=CARTESIAN_POINT('Ctrl Pts',(-0.853825826608993,-69.9947925310006,
12.));
#131020=CARTESIAN_POINT('',(-0.853825826608993,-69.9947925310006,12.));
#131021=CARTESIAN_POINT('Ctrl Pts',(-0.853825826608993,-69.9947925310006,
12.));
#131022=CARTESIAN_POINT('Ctrl Pts',(-0.854867673848293,-69.9985337959499,
12.));
#131023=CARTESIAN_POINT('Ctrl Pts',(-0.856954870258371,-70.0060209754332,
12.));
#131024=CARTESIAN_POINT('Ctrl Pts',(-0.860096170667398,-70.0172656934192,
12.));
#131025=CARTESIAN_POINT('Ctrl Pts',(-0.86430558366009,-70.0322865493339,
12.));
#131026=CARTESIAN_POINT('Ctrl Pts',(-0.869602377870139,-70.0511091083285,
12.));
#131027=CARTESIAN_POINT('Ctrl Pts',(-0.87493421325557,-70.0699781184013,
12.));
#131028=CARTESIAN_POINT('Ctrl Pts',(-0.880301109661037,-70.0888934967772,
12.));
#131029=CARTESIAN_POINT('Ctrl Pts',(-0.885703094803086,-70.1078550938801,
12.));
#131030=CARTESIAN_POINT('Ctrl Pts',(-0.891140203464724,-70.1268626950031,
12.));
#131031=CARTESIAN_POINT('Ctrl Pts',(-0.896612474372085,-70.1459160490366,
12.));
#131032=CARTESIAN_POINT('Ctrl Pts',(-0.902119947629773,-70.1650148905109,
12.));
#131033=CARTESIAN_POINT('Ctrl Pts',(-0.90766266201565,-70.184158963563,
12.));
#131034=CARTESIAN_POINT('Ctrl Pts',(-0.913240652090839,-70.2033480471749,
12.));
#131035=CARTESIAN_POINT('Ctrl Pts',(-0.918853949157045,-70.2225819470306,
12.));
#131036=CARTESIAN_POINT('Ctrl Pts',(-0.924502582639453,-70.241860483586,
12.));
#131037=CARTESIAN_POINT('Ctrl Pts',(-0.930186581235576,-70.2611834821711,
12.));
#131038=CARTESIAN_POINT('Ctrl Pts',(-0.935905974336492,-70.2805507606832,
12.));
#131039=CARTESIAN_POINT('Ctrl Pts',(-0.941660792742953,-70.2999621233938,
12.));
#131040=CARTESIAN_POINT('Ctrl Pts',(-0.947451067929564,-70.3194173673635,
12.));
#131041=CARTESIAN_POINT('Ctrl Pts',(-0.953276831581232,-70.338916286457,
12.));
#131042=CARTESIAN_POINT('Ctrl Pts',(-0.959138115058886,-70.3584586759561,
12.));
#131043=CARTESIAN_POINT('Ctrl Pts',(-0.965034948786559,-70.3780443378003,
12.));
#131044=CARTESIAN_POINT('Ctrl Pts',(-0.970967362281301,-70.3976730803664,
12.));
#131045=CARTESIAN_POINT('Ctrl Pts',(-0.976935384450128,-70.41734471596,
12.));
#131046=CARTESIAN_POINT('Ctrl Pts',(-0.982939043792158,-70.4370590590839,
12.));
#131047=CARTESIAN_POINT('Ctrl Pts',(-0.98897836864359,-70.4568159243131,
12.));
#131048=CARTESIAN_POINT('Ctrl Pts',(-0.995053387379681,-70.476615124517,
12.));
#131049=CARTESIAN_POINT('Ctrl Pts',(-1.00116412831438,-70.4964564717917,
12.));
#131050=CARTESIAN_POINT('Ctrl Pts',(-1.00731061960968,-70.5163397782699,
12.));
#131051=CARTESIAN_POINT('Ctrl Pts',(-1.0134928891854,-70.5362648569072,
12.));
#131052=CARTESIAN_POINT('Ctrl Pts',(-1.01971096460599,-70.5562315224219,
12.));
#131053=CARTESIAN_POINT('Ctrl Pts',(-1.02596487304049,-70.5762395916412,
12.));
#131054=CARTESIAN_POINT('Ctrl Pts',(-1.03225464132872,-70.5962888829958,
12.));
#131055=CARTESIAN_POINT('Ctrl Pts',(-1.03858029601906,-70.6163792162079,
12.));
#131056=CARTESIAN_POINT('Ctrl Pts',(-1.04494186341156,-70.6365104119238,
12.));
#131057=CARTESIAN_POINT('Ctrl Pts',(-1.05133936960069,-70.6566822912965,
12.));
#131058=CARTESIAN_POINT('Ctrl Pts',(-1.05777284047728,-70.6768946760063,
12.));
#131059=CARTESIAN_POINT('Ctrl Pts',(-1.0642423017128,-70.6971473884443,
12.));
#131060=CARTESIAN_POINT('Ctrl Pts',(-1.07074777874596,-70.7174402518378,
12.));
#131061=CARTESIAN_POINT('Ctrl Pts',(-1.07728929676412,-70.737773090397,
12.));
#131062=CARTESIAN_POINT('Ctrl Pts',(-1.08386688068349,-70.7581457294475,
12.));
#131063=CARTESIAN_POINT('Ctrl Pts',(-1.09048055516434,-70.7785579953611,
12.));
#131064=CARTESIAN_POINT('Ctrl Pts',(-1.0971303446227,-70.7990097154855,
12.));
#131065=CARTESIAN_POINT('Ctrl Pts',(-1.10381627323946,-70.8195007180739,
12.));
#131066=CARTESIAN_POINT('Ctrl Pts',(-1.11053836496638,-70.8400308322013,
12.));
#131067=CARTESIAN_POINT('Ctrl Pts',(-1.1172966435299,-70.860599887712,12.));
#131068=CARTESIAN_POINT('Ctrl Pts',(-1.12409113243511,-70.8812077152564,
12.));
#131069=CARTESIAN_POINT('Ctrl Pts',(-1.13092185496563,-70.9018541463083,
12.));
#131070=CARTESIAN_POINT('Ctrl Pts',(-1.13778883418216,-70.9225390131835,
12.));
#131071=CARTESIAN_POINT('Ctrl Pts',(-1.14469209291494,-70.943262149058,
12.));
#131072=CARTESIAN_POINT('Ctrl Pts',(-1.1516316537653,-70.9640233879671,
12.));
#131073=CARTESIAN_POINT('Ctrl Pts',(-1.1586075391149,-70.9848225647876,
12.));
#131074=CARTESIAN_POINT('Ctrl Pts',(-1.16561977112882,-71.0056595152204,
12.));
#131075=CARTESIAN_POINT('Ctrl Pts',(-1.17266837175776,-71.0265340757697,
12.));
#131076=CARTESIAN_POINT('Ctrl Pts',(-1.179753362735,-71.0474460837157,12.));
#131077=CARTESIAN_POINT('Ctrl Pts',(-1.18687476558127,-71.0683953771147,
12.));
#131078=CARTESIAN_POINT('Ctrl Pts',(-1.19403260160998,-71.089381794801,
12.));
#131079=CARTESIAN_POINT('Ctrl Pts',(-1.20122689192836,-71.1104051763839,
12.));
#131080=CARTESIAN_POINT('Ctrl Pts',(-1.20845765743654,-71.1314653622442,
12.));
#131081=CARTESIAN_POINT('Ctrl Pts',(-1.21572491882273,-71.1525621935266,
12.));
#131082=CARTESIAN_POINT('Ctrl Pts',(-1.22302869657028,-71.1736955121361,
12.));
#131083=CARTESIAN_POINT('Ctrl Pts',(-1.23036901096246,-71.1948651607319,
12.));
#131084=CARTESIAN_POINT('Ctrl Pts',(-1.23774588208427,-71.2160709827189,
12.));
#131085=CARTESIAN_POINT('Ctrl Pts',(-1.24515932982108,-71.2373128222359,
12.));
#131086=CARTESIAN_POINT('Ctrl Pts',(-1.25260937385561,-71.2585905241422,
12.));
#131087=CARTESIAN_POINT('Ctrl Pts',(-1.26009603367565,-71.2799039340191,
12.));
#131088=CARTESIAN_POINT('Ctrl Pts',(-1.26761932857723,-71.301252898167,
12.));
#131089=CARTESIAN_POINT('Ctrl Pts',(-1.27517927766611,-71.3226372635993,
12.));
#131090=CARTESIAN_POINT('Ctrl Pts',(-1.28277589985475,-71.344056878033,
12.));
#131091=CARTESIAN_POINT('Ctrl Pts',(-1.29040921386061,-71.3655115898801,
12.));
#131092=CARTESIAN_POINT('Ctrl Pts',(-1.29807923821414,-71.3870012482474,
12.));
#131093=CARTESIAN_POINT('Ctrl Pts',(-1.30578599126139,-71.4085257029308,
12.));
#131094=CARTESIAN_POINT('Ctrl Pts',(-1.31352949116539,-71.4300848044095,
12.));
#131095=CARTESIAN_POINT('Ctrl Pts',(-1.32130975590231,-71.4516784038346,
12.));
#131096=CARTESIAN_POINT('Ctrl Pts',(-1.32912680326131,-71.4733063530227,
12.));
#131097=CARTESIAN_POINT('Ctrl Pts',(-1.33698065085228,-71.4949685044559,
12.));
#131098=CARTESIAN_POINT('Ctrl Pts',(-1.34487131610785,-71.5166647112766,
12.));
#131099=CARTESIAN_POINT('Ctrl Pts',(-1.35279881628453,-71.538394827283,
12.));
#131100=CARTESIAN_POINT('Ctrl Pts',(-1.36076316845806,-71.5601587069175,
12.));
#131101=CARTESIAN_POINT('Ctrl Pts',(-1.36876438952449,-71.5819562052613,
12.));
#131102=CARTESIAN_POINT('Ctrl Pts',(-1.37680249620763,-71.6037871780347,
12.));
#131103=CARTESIAN_POINT('Ctrl Pts',(-1.38487750506076,-71.6256514815918,
12.));
#131104=CARTESIAN_POINT('Ctrl Pts',(-1.39298943246731,-71.6475489729149,
12.));
#131105=CARTESIAN_POINT('Ctrl Pts',(-1.401138294636,-71.6694795096034,12.));
#131106=CARTESIAN_POINT('Ctrl Pts',(-1.40932410760275,-71.6914429498702,
12.));
#131107=CARTESIAN_POINT('Ctrl Pts',(-1.41754688723791,-71.7134391525417,
12.));
#131108=CARTESIAN_POINT('Ctrl Pts',(-1.42580664924774,-71.7354679770537,
12.));
#131109=CARTESIAN_POINT('Ctrl Pts',(-1.43410340917489,-71.7575292834456,
12.));
#131110=CARTESIAN_POINT('Ctrl Pts',(-1.44243718239305,-71.7796229323496,
12.));
#131111=CARTESIAN_POINT('Ctrl Pts',(-1.45080798410957,-71.8017487849865,
12.));
#131112=CARTESIAN_POINT('Ctrl Pts',(-1.45921582937229,-71.8239067031664,
12.));
#131113=CARTESIAN_POINT('Ctrl Pts',(-1.46766073307089,-71.8460965492836,
12.));
#131114=CARTESIAN_POINT('Ctrl Pts',(-1.4761427099373,-71.8683181863123,
12.));
#131115=CARTESIAN_POINT('Ctrl Pts',(-1.48466177454021,-71.8905714777972,
12.));
#131116=CARTESIAN_POINT('Ctrl Pts',(-1.493217941288,-71.9128562878491,12.));
#131117=CARTESIAN_POINT('Ctrl Pts',(-1.50181122443535,-71.935172481145,
12.));
#131118=CARTESIAN_POINT('Ctrl Pts',(-1.51044163808455,-71.9575199229241,
12.));
#131119=CARTESIAN_POINT('Ctrl Pts',(-1.51910919618567,-71.9798984789828,
12.));
#131120=CARTESIAN_POINT('Ctrl Pts',(-1.52781391253103,-72.0023080156647,
12.));
#131121=CARTESIAN_POINT('Ctrl Pts',(-1.53655580075814,-72.0247483998582,
12.));
#131122=CARTESIAN_POINT('Ctrl Pts',(-1.54533487435626,-72.0472194989968,
12.));
#131123=CARTESIAN_POINT('Ctrl Pts',(-1.55415114666774,-72.0697211810548,
12.));
#131124=CARTESIAN_POINT('Ctrl Pts',(-1.56300463088811,-72.092253314543,
12.));
#131125=CARTESIAN_POINT('Ctrl Pts',(-1.57189534006043,-72.1148157684987,
12.));
#131126=CARTESIAN_POINT('Ctrl Pts',(-1.58082328707808,-72.1374084124829,
12.));
#131127=CARTESIAN_POINT('Ctrl Pts',(-1.58978848469128,-72.1600311165813,
12.));
#131128=CARTESIAN_POINT('Ctrl Pts',(-1.5987909455085,-72.1826837514,12.));
#131129=CARTESIAN_POINT('Ctrl Pts',(-1.60783068199662,-72.2053661880611,
12.));
#131130=CARTESIAN_POINT('Ctrl Pts',(-1.61690770647536,-72.2280782981941,
12.));
#131131=CARTESIAN_POINT('Ctrl Pts',(-1.62602203111924,-72.2508199539325,
12.));
#131132=CARTESIAN_POINT('Ctrl Pts',(-1.63517366796459,-72.2735910279149,
12.));
#131133=CARTESIAN_POINT('Ctrl Pts',(-1.64436262891078,-72.2963913932811,
12.));
#131134=CARTESIAN_POINT('Ctrl Pts',(-1.65358892572066,-72.3192209236691,
12.));
#131135=CARTESIAN_POINT('Ctrl Pts',(-1.66285257001502,-72.3420794932052,
12.));
#131136=CARTESIAN_POINT('Ctrl Pts',(-1.67215357327372,-72.3649669765013,
12.));
#131137=CARTESIAN_POINT('Ctrl Pts',(-1.68149194684288,-72.3878832486549,
12.));
#131138=CARTESIAN_POINT('Ctrl Pts',(-1.69086770193641,-72.4108281852473,
12.));
#131139=CARTESIAN_POINT('Ctrl Pts',(-1.70028084963647,-72.4338016623388,
12.));
#131140=CARTESIAN_POINT('Ctrl Pts',(-1.70973140088837,-72.4568035564618,
12.));
#131141=CARTESIAN_POINT('Ctrl Pts',(-1.71921936650032,-72.4798337446162,
12.));
#131142=CARTESIAN_POINT('Ctrl Pts',(-1.72874475715098,-72.5028921042704,
12.));
#131143=CARTESIAN_POINT('Ctrl Pts',(-1.73830758339123,-72.5259785133586,
12.));
#131144=CARTESIAN_POINT('Ctrl Pts',(-1.74790785564476,-72.5490928502773,
12.));
#131145=CARTESIAN_POINT('Ctrl Pts',(-1.7575455842035,-72.5722349938789,
12.));
#131146=CARTESIAN_POINT('Ctrl Pts',(-1.7672207792258,-72.5954048234655,
12.));
#131147=CARTESIAN_POINT('Ctrl Pts',(-1.7769334507443,-72.618602218792,12.));
#131148=CARTESIAN_POINT('Ctrl Pts',(-1.78668360866813,-72.6418270600623,
12.));
#131149=CARTESIAN_POINT('Ctrl Pts',(-1.79647126278359,-72.6650792279271,
12.));
#131150=CARTESIAN_POINT('Ctrl Pts',(-1.80629642275051,-72.6883586034768,
12.));
#131151=CARTESIAN_POINT('Ctrl Pts',(-1.81615909809872,-72.7116650682347,
12.));
#131152=CARTESIAN_POINT('Ctrl Pts',(-1.82605929823565,-72.73499850416,12.));
#131153=CARTESIAN_POINT('Ctrl Pts',(-1.83599703244926,-72.7583587936454,
12.));
#131154=CARTESIAN_POINT('Ctrl Pts',(-1.84597230990858,-72.7817458195155,
12.));
#131155=CARTESIAN_POINT('Ctrl Pts',(-1.85598513966115,-72.8051594650214,
12.));
#131156=CARTESIAN_POINT('Ctrl Pts',(-1.86603553062776,-72.8285996138346,
12.));
#131157=CARTESIAN_POINT('Ctrl Pts',(-1.87612349160952,-72.8520661500465,
12.));
#131158=CARTESIAN_POINT('Ctrl Pts',(-1.88624903129195,-72.8755589581674,
12.));
#131159=CARTESIAN_POINT('Ctrl Pts',(-1.89641215824584,-72.8990779231226,
12.));
#131160=CARTESIAN_POINT('Ctrl Pts',(-1.90661288092583,-72.9226229302483,
12.));
#131161=CARTESIAN_POINT('Ctrl Pts',(-1.91685120766428,-72.9461938652816,
12.));
#131162=CARTESIAN_POINT('Ctrl Pts',(-1.92712714667648,-72.9697906143638,
12.));
#131163=CARTESIAN_POINT('Ctrl Pts',(-1.93744070606557,-72.9934130640414,
12.));
#131164=CARTESIAN_POINT('Ctrl Pts',(-1.947791893823,-73.0170611012659,12.));
#131165=CARTESIAN_POINT('Ctrl Pts',(-1.95818071782773,-73.0407346133912,
12.));
#131166=CARTESIAN_POINT('Ctrl Pts',(-1.96860718583944,-73.0644334881679,
12.));
#131167=CARTESIAN_POINT('Ctrl Pts',(-1.97907130550172,-73.0881576137415,
12.));
#131168=CARTESIAN_POINT('Ctrl Pts',(-1.9895730843493,-73.1119068786482,
12.));
#131169=CARTESIAN_POINT('Ctrl Pts',(-2.00011252980987,-73.1356811718094,
12.));
#131170=CARTESIAN_POINT('Ctrl Pts',(-2.01068964920465,-73.159480382525,
12.));
#131171=CARTESIAN_POINT('Ctrl Pts',(-2.02130444974352,-73.1833044004612,
12.));
#131172=CARTESIAN_POINT('Ctrl Pts',(-2.0319569385244,-73.2071531156492,
12.));
#131173=CARTESIAN_POINT('Ctrl Pts',(-2.04264712253915,-73.2310264184965,
12.));
#131174=CARTESIAN_POINT('Ctrl Pts',(-2.05337500867395,-73.2549241997946,
12.));
#131175=CARTESIAN_POINT('Ctrl Pts',(-2.06414060370837,-73.2788463507248,
12.));
#131176=CARTESIAN_POINT('Ctrl Pts',(-2.07494391430954,-73.3027927628636,
12.));
#131177=CARTESIAN_POINT('Ctrl Pts',(-2.08578494702762,-73.3267633281822,
12.));
#131178=CARTESIAN_POINT('Ctrl Pts',(-2.09666370830733,-73.3507579390254,
12.));
#131179=CARTESIAN_POINT('Ctrl Pts',(-2.10758020449401,-73.3747764880903,
12.));
#131180=CARTESIAN_POINT('Ctrl Pts',(-2.11853444183764,-73.3988188684022,
12.));
#131181=CARTESIAN_POINT('Ctrl Pts',(-2.1295264264936,-73.4228849732914,
12.));
#131182=CARTESIAN_POINT('Ctrl Pts',(-2.14055616452049,-73.4469746963622,
12.));
#131183=CARTESIAN_POINT('Ctrl Pts',(-2.15162366187899,-73.4710879315367,
12.));
#131184=CARTESIAN_POINT('Ctrl Pts',(-2.16272892442915,-73.4952245731044,
12.));
#131185=CARTESIAN_POINT('Ctrl Pts',(-2.17387195792306,-73.5193845157705,
12.));
#131186=CARTESIAN_POINT('Ctrl Pts',(-2.18505276799756,-73.5435676546934,
12.));
#131187=CARTESIAN_POINT('Ctrl Pts',(-2.19627136015683,-73.5677738855461,
12.));
#131188=CARTESIAN_POINT('Ctrl Pts',(-2.20752773978353,-73.5920031044604,
12.));
#131189=CARTESIAN_POINT('Ctrl Pts',(-2.21882191216521,-73.6162552079044,
12.));
#131190=CARTESIAN_POINT('Ctrl Pts',(-2.23015388251289,-73.6405300925714,
12.));
#131191=CARTESIAN_POINT('Ctrl Pts',(-2.24152365597699,-73.6648276552766,
12.));
#131192=CARTESIAN_POINT('Ctrl Pts',(-2.25293123766425,-73.6891477928124,
12.));
#131193=CARTESIAN_POINT('Ctrl Pts',(-2.26437663263663,-73.7134904019378,
12.));
#131194=CARTESIAN_POINT('Ctrl Pts',(-2.27585984587193,-73.7378553796792,
12.));
#131195=CARTESIAN_POINT('Ctrl Pts',(-2.28738088222858,-73.7622426235648,
12.));
#131196=CARTESIAN_POINT('Ctrl Pts',(-2.29893974640435,-73.7866520318849,
12.));
#131197=CARTESIAN_POINT('Ctrl Pts',(-2.31053644289425,-73.8110835039341,
12.));
#131198=CARTESIAN_POINT('Ctrl Pts',(-2.32217097594215,-73.8355369402733,
12.));
#131199=CARTESIAN_POINT('Ctrl Pts',(-2.3338433496398,-73.8600122421502,
12.));
#131200=CARTESIAN_POINT('Ctrl Pts',(-2.3455535680214,-73.8845093109302,
12.));
#131201=CARTESIAN_POINT('Ctrl Pts',(-2.35730163516324,-73.9090280474723,
12.));
#131202=CARTESIAN_POINT('Ctrl Pts',(-2.36908755525994,-73.9335683516388,
12.));
#131203=CARTESIAN_POINT('Ctrl Pts',(-2.38091133274933,-73.9581301214609,
12.));
#131204=CARTESIAN_POINT('Ctrl Pts',(-2.39277297220716,-73.9827132538149,
12.));
#131205=CARTESIAN_POINT('Ctrl Pts',(-2.40467247811497,-74.0073176459287,
12.));
#131206=CARTESIAN_POINT('Ctrl Pts',(-2.41660985465228,-74.0319431966956,
12.));
#131207=CARTESIAN_POINT('Ctrl Pts',(-2.42858510549786,-74.0565898079227,
12.));
#131208=CARTESIAN_POINT('Ctrl Pts',(-2.44059823356722,-74.0812573859474,
12.));
#131209=CARTESIAN_POINT('Ctrl Pts',(-2.45264924094852,-74.1059458420175,
12.));
#131210=CARTESIAN_POINT('Ctrl Pts',(-2.46301176097527,-74.1271264545378,
12.));
#131211=CARTESIAN_POINT('Ctrl Pts',(-2.47097695565717,-74.1433763941622,
12.));
#131212=CARTESIAN_POINT('Ctrl Pts',(-2.47652804725572,-74.1546864735453,
12.));
#131213=CARTESIAN_POINT('Ctrl Pts',(-2.47965393946824,-74.1610506466543,
12.));
#131214=CARTESIAN_POINT('Ctrl Pts',(-2.480349218449,-74.1624659714954,12.));
#131215=CARTESIAN_POINT('',(-0.853825826608993,-69.9947925310006,0.));
#131216=CARTESIAN_POINT('',(-0.853825826608992,-69.9947925310006,0.));
#131217=CARTESIAN_POINT('Ctrl Pts',(-2.480349218449,-74.1624659714955,0.));
#131218=CARTESIAN_POINT('Ctrl Pts',(-2.47965393946824,-74.1610506466543,
0.));
#131219=CARTESIAN_POINT('Ctrl Pts',(-2.47652804725572,-74.1546864735453,
0.));
#131220=CARTESIAN_POINT('Ctrl Pts',(-2.47097695565718,-74.1433763941622,
0.));
#131221=CARTESIAN_POINT('Ctrl Pts',(-2.46301176097527,-74.1271264545378,
0.));
#131222=CARTESIAN_POINT('Ctrl Pts',(-2.45264924094852,-74.1059458420175,
0.));
#131223=CARTESIAN_POINT('Ctrl Pts',(-2.44059823356722,-74.0812573859474,
0.));
#131224=CARTESIAN_POINT('Ctrl Pts',(-2.42858510549786,-74.0565898079227,
0.));
#131225=CARTESIAN_POINT('Ctrl Pts',(-2.41660985465228,-74.0319431966956,
0.));
#131226=CARTESIAN_POINT('Ctrl Pts',(-2.40467247811497,-74.0073176459287,
0.));
#131227=CARTESIAN_POINT('Ctrl Pts',(-2.39277297220716,-73.9827132538149,
0.));
#131228=CARTESIAN_POINT('Ctrl Pts',(-2.38091133274933,-73.9581301214609,
0.));
#131229=CARTESIAN_POINT('Ctrl Pts',(-2.36908755525994,-73.9335683516388,
0.));
#131230=CARTESIAN_POINT('Ctrl Pts',(-2.35730163516324,-73.9090280474723,
0.));
#131231=CARTESIAN_POINT('Ctrl Pts',(-2.3455535680214,-73.8845093109302,
0.));
#131232=CARTESIAN_POINT('Ctrl Pts',(-2.3338433496398,-73.8600122421502,
0.));
#131233=CARTESIAN_POINT('Ctrl Pts',(-2.32217097594215,-73.8355369402733,
0.));
#131234=CARTESIAN_POINT('Ctrl Pts',(-2.31053644289425,-73.8110835039341,
0.));
#131235=CARTESIAN_POINT('Ctrl Pts',(-2.29893974640435,-73.7866520318849,
0.));
#131236=CARTESIAN_POINT('Ctrl Pts',(-2.28738088222858,-73.7622426235648,
0.));
#131237=CARTESIAN_POINT('Ctrl Pts',(-2.27585984587193,-73.7378553796792,
0.));
#131238=CARTESIAN_POINT('Ctrl Pts',(-2.26437663263663,-73.7134904019378,
0.));
#131239=CARTESIAN_POINT('Ctrl Pts',(-2.25293123766425,-73.6891477928124,
0.));
#131240=CARTESIAN_POINT('Ctrl Pts',(-2.24152365597699,-73.6648276552766,
0.));
#131241=CARTESIAN_POINT('Ctrl Pts',(-2.23015388251289,-73.6405300925714,
0.));
#131242=CARTESIAN_POINT('Ctrl Pts',(-2.21882191216521,-73.6162552079044,
0.));
#131243=CARTESIAN_POINT('Ctrl Pts',(-2.20752773978353,-73.5920031044604,
0.));
#131244=CARTESIAN_POINT('Ctrl Pts',(-2.19627136015683,-73.5677738855461,
0.));
#131245=CARTESIAN_POINT('Ctrl Pts',(-2.18505276799756,-73.5435676546934,
0.));
#131246=CARTESIAN_POINT('Ctrl Pts',(-2.17387195792306,-73.5193845157705,
0.));
#131247=CARTESIAN_POINT('Ctrl Pts',(-2.16272892442915,-73.4952245731044,
0.));
#131248=CARTESIAN_POINT('Ctrl Pts',(-2.15162366187899,-73.4710879315367,
0.));
#131249=CARTESIAN_POINT('Ctrl Pts',(-2.14055616452049,-73.4469746963622,
0.));
#131250=CARTESIAN_POINT('Ctrl Pts',(-2.1295264264936,-73.4228849732914,
0.));
#131251=CARTESIAN_POINT('Ctrl Pts',(-2.11853444183764,-73.3988188684022,
0.));
#131252=CARTESIAN_POINT('Ctrl Pts',(-2.10758020449401,-73.3747764880903,
0.));
#131253=CARTESIAN_POINT('Ctrl Pts',(-2.09666370830733,-73.3507579390254,
0.));
#131254=CARTESIAN_POINT('Ctrl Pts',(-2.08578494702762,-73.3267633281822,
0.));
#131255=CARTESIAN_POINT('Ctrl Pts',(-2.07494391430954,-73.3027927628636,
0.));
#131256=CARTESIAN_POINT('Ctrl Pts',(-2.06414060370837,-73.2788463507248,
0.));
#131257=CARTESIAN_POINT('Ctrl Pts',(-2.05337500867395,-73.2549241997946,
0.));
#131258=CARTESIAN_POINT('Ctrl Pts',(-2.04264712253915,-73.2310264184965,
0.));
#131259=CARTESIAN_POINT('Ctrl Pts',(-2.0319569385244,-73.2071531156492,
0.));
#131260=CARTESIAN_POINT('Ctrl Pts',(-2.02130444974352,-73.1833044004612,
0.));
#131261=CARTESIAN_POINT('Ctrl Pts',(-2.01068964920465,-73.159480382525,
0.));
#131262=CARTESIAN_POINT('Ctrl Pts',(-2.00011252980987,-73.1356811718094,
0.));
#131263=CARTESIAN_POINT('Ctrl Pts',(-1.9895730843493,-73.1119068786482,
0.));
#131264=CARTESIAN_POINT('Ctrl Pts',(-1.97907130550172,-73.0881576137415,
0.));
#131265=CARTESIAN_POINT('Ctrl Pts',(-1.96860718583944,-73.0644334881679,
0.));
#131266=CARTESIAN_POINT('Ctrl Pts',(-1.95818071782773,-73.0407346133912,
0.));
#131267=CARTESIAN_POINT('Ctrl Pts',(-1.947791893823,-73.0170611012659,0.));
#131268=CARTESIAN_POINT('Ctrl Pts',(-1.93744070606557,-72.9934130640414,
0.));
#131269=CARTESIAN_POINT('Ctrl Pts',(-1.92712714667648,-72.9697906143638,
0.));
#131270=CARTESIAN_POINT('Ctrl Pts',(-1.91685120766428,-72.9461938652816,
0.));
#131271=CARTESIAN_POINT('Ctrl Pts',(-1.90661288092583,-72.9226229302483,
0.));
#131272=CARTESIAN_POINT('Ctrl Pts',(-1.89641215824584,-72.8990779231226,
0.));
#131273=CARTESIAN_POINT('Ctrl Pts',(-1.88624903129195,-72.8755589581674,
0.));
#131274=CARTESIAN_POINT('Ctrl Pts',(-1.87612349160952,-72.8520661500465,
0.));
#131275=CARTESIAN_POINT('Ctrl Pts',(-1.86603553062776,-72.8285996138346,
0.));
#131276=CARTESIAN_POINT('Ctrl Pts',(-1.85598513966115,-72.8051594650214,
0.));
#131277=CARTESIAN_POINT('Ctrl Pts',(-1.84597230990858,-72.7817458195155,
0.));
#131278=CARTESIAN_POINT('Ctrl Pts',(-1.83599703244926,-72.7583587936454,
0.));
#131279=CARTESIAN_POINT('Ctrl Pts',(-1.82605929823565,-72.73499850416,0.));
#131280=CARTESIAN_POINT('Ctrl Pts',(-1.81615909809872,-72.7116650682347,
0.));
#131281=CARTESIAN_POINT('Ctrl Pts',(-1.80629642275051,-72.6883586034768,
0.));
#131282=CARTESIAN_POINT('Ctrl Pts',(-1.79647126278359,-72.6650792279271,
0.));
#131283=CARTESIAN_POINT('Ctrl Pts',(-1.78668360866813,-72.6418270600623,
0.));
#131284=CARTESIAN_POINT('Ctrl Pts',(-1.7769334507443,-72.618602218792,0.));
#131285=CARTESIAN_POINT('Ctrl Pts',(-1.7672207792258,-72.5954048234655,
0.));
#131286=CARTESIAN_POINT('Ctrl Pts',(-1.7575455842035,-72.5722349938789,
0.));
#131287=CARTESIAN_POINT('Ctrl Pts',(-1.74790785564476,-72.5490928502773,
0.));
#131288=CARTESIAN_POINT('Ctrl Pts',(-1.73830758339123,-72.5259785133586,
0.));
#131289=CARTESIAN_POINT('Ctrl Pts',(-1.72874475715098,-72.5028921042704,
0.));
#131290=CARTESIAN_POINT('Ctrl Pts',(-1.71921936650032,-72.4798337446162,
0.));
#131291=CARTESIAN_POINT('Ctrl Pts',(-1.70973140088837,-72.4568035564618,
0.));
#131292=CARTESIAN_POINT('Ctrl Pts',(-1.70028084963647,-72.4338016623388,
0.));
#131293=CARTESIAN_POINT('Ctrl Pts',(-1.69086770193641,-72.4108281852473,
0.));
#131294=CARTESIAN_POINT('Ctrl Pts',(-1.68149194684288,-72.3878832486549,
0.));
#131295=CARTESIAN_POINT('Ctrl Pts',(-1.67215357327372,-72.3649669765013,
0.));
#131296=CARTESIAN_POINT('Ctrl Pts',(-1.66285257001502,-72.3420794932052,
0.));
#131297=CARTESIAN_POINT('Ctrl Pts',(-1.65358892572066,-72.3192209236691,
0.));
#131298=CARTESIAN_POINT('Ctrl Pts',(-1.64436262891078,-72.2963913932811,
0.));
#131299=CARTESIAN_POINT('Ctrl Pts',(-1.63517366796459,-72.2735910279149,
0.));
#131300=CARTESIAN_POINT('Ctrl Pts',(-1.62602203111924,-72.2508199539325,
0.));
#131301=CARTESIAN_POINT('Ctrl Pts',(-1.61690770647536,-72.2280782981941,
0.));
#131302=CARTESIAN_POINT('Ctrl Pts',(-1.60783068199662,-72.2053661880611,
0.));
#131303=CARTESIAN_POINT('Ctrl Pts',(-1.5987909455085,-72.1826837514,0.));
#131304=CARTESIAN_POINT('Ctrl Pts',(-1.58978848469128,-72.1600311165813,
0.));
#131305=CARTESIAN_POINT('Ctrl Pts',(-1.58082328707808,-72.1374084124829,
0.));
#131306=CARTESIAN_POINT('Ctrl Pts',(-1.57189534006043,-72.1148157684987,
0.));
#131307=CARTESIAN_POINT('Ctrl Pts',(-1.56300463088811,-72.092253314543,
0.));
#131308=CARTESIAN_POINT('Ctrl Pts',(-1.55415114666774,-72.0697211810548,
0.));
#131309=CARTESIAN_POINT('Ctrl Pts',(-1.54533487435626,-72.0472194989968,
0.));
#131310=CARTESIAN_POINT('Ctrl Pts',(-1.53655580075814,-72.0247483998582,
0.));
#131311=CARTESIAN_POINT('Ctrl Pts',(-1.52781391253103,-72.0023080156647,
0.));
#131312=CARTESIAN_POINT('Ctrl Pts',(-1.51910919618567,-71.9798984789828,
0.));
#131313=CARTESIAN_POINT('Ctrl Pts',(-1.51044163808455,-71.9575199229241,
0.));
#131314=CARTESIAN_POINT('Ctrl Pts',(-1.50181122443535,-71.935172481145,
0.));
#131315=CARTESIAN_POINT('Ctrl Pts',(-1.493217941288,-71.9128562878491,0.));
#131316=CARTESIAN_POINT('Ctrl Pts',(-1.48466177454021,-71.8905714777972,
0.));
#131317=CARTESIAN_POINT('Ctrl Pts',(-1.4761427099373,-71.8683181863123,
0.));
#131318=CARTESIAN_POINT('Ctrl Pts',(-1.46766073307089,-71.8460965492836,
0.));
#131319=CARTESIAN_POINT('Ctrl Pts',(-1.45921582937229,-71.8239067031664,
0.));
#131320=CARTESIAN_POINT('Ctrl Pts',(-1.45080798410957,-71.8017487849865,
0.));
#131321=CARTESIAN_POINT('Ctrl Pts',(-1.44243718239305,-71.7796229323496,
0.));
#131322=CARTESIAN_POINT('Ctrl Pts',(-1.43410340917489,-71.7575292834456,
0.));
#131323=CARTESIAN_POINT('Ctrl Pts',(-1.42580664924774,-71.7354679770537,
0.));
#131324=CARTESIAN_POINT('Ctrl Pts',(-1.41754688723791,-71.7134391525417,
0.));
#131325=CARTESIAN_POINT('Ctrl Pts',(-1.40932410760275,-71.6914429498702,
0.));
#131326=CARTESIAN_POINT('Ctrl Pts',(-1.401138294636,-71.6694795096034,0.));
#131327=CARTESIAN_POINT('Ctrl Pts',(-1.39298943246731,-71.6475489729149,
0.));
#131328=CARTESIAN_POINT('Ctrl Pts',(-1.38487750506076,-71.6256514815918,
0.));
#131329=CARTESIAN_POINT('Ctrl Pts',(-1.37680249620763,-71.6037871780347,
0.));
#131330=CARTESIAN_POINT('Ctrl Pts',(-1.36876438952449,-71.5819562052613,
0.));
#131331=CARTESIAN_POINT('Ctrl Pts',(-1.36076316845806,-71.5601587069175,
0.));
#131332=CARTESIAN_POINT('Ctrl Pts',(-1.35279881628453,-71.538394827283,
0.));
#131333=CARTESIAN_POINT('Ctrl Pts',(-1.34487131610785,-71.5166647112766,
0.));
#131334=CARTESIAN_POINT('Ctrl Pts',(-1.33698065085228,-71.4949685044559,
0.));
#131335=CARTESIAN_POINT('Ctrl Pts',(-1.32912680326131,-71.4733063530227,
0.));
#131336=CARTESIAN_POINT('Ctrl Pts',(-1.32130975590231,-71.4516784038346,
0.));
#131337=CARTESIAN_POINT('Ctrl Pts',(-1.31352949116539,-71.4300848044095,
0.));
#131338=CARTESIAN_POINT('Ctrl Pts',(-1.30578599126139,-71.4085257029308,
0.));
#131339=CARTESIAN_POINT('Ctrl Pts',(-1.29807923821414,-71.3870012482474,
0.));
#131340=CARTESIAN_POINT('Ctrl Pts',(-1.29040921386061,-71.3655115898801,
0.));
#131341=CARTESIAN_POINT('Ctrl Pts',(-1.28277589985475,-71.344056878033,
0.));
#131342=CARTESIAN_POINT('Ctrl Pts',(-1.27517927766611,-71.3226372635993,
0.));
#131343=CARTESIAN_POINT('Ctrl Pts',(-1.26761932857723,-71.301252898167,
0.));
#131344=CARTESIAN_POINT('Ctrl Pts',(-1.26009603367565,-71.2799039340191,
0.));
#131345=CARTESIAN_POINT('Ctrl Pts',(-1.25260937385561,-71.2585905241422,
0.));
#131346=CARTESIAN_POINT('Ctrl Pts',(-1.24515932982108,-71.2373128222359,
0.));
#131347=CARTESIAN_POINT('Ctrl Pts',(-1.23774588208427,-71.2160709827189,
0.));
#131348=CARTESIAN_POINT('Ctrl Pts',(-1.23036901096246,-71.1948651607319,
0.));
#131349=CARTESIAN_POINT('Ctrl Pts',(-1.22302869657028,-71.1736955121361,
0.));
#131350=CARTESIAN_POINT('Ctrl Pts',(-1.21572491882273,-71.1525621935266,
0.));
#131351=CARTESIAN_POINT('Ctrl Pts',(-1.20845765743654,-71.1314653622442,
0.));
#131352=CARTESIAN_POINT('Ctrl Pts',(-1.20122689192836,-71.1104051763839,
0.));
#131353=CARTESIAN_POINT('Ctrl Pts',(-1.19403260160998,-71.089381794801,
0.));
#131354=CARTESIAN_POINT('Ctrl Pts',(-1.18687476558127,-71.0683953771147,
0.));
#131355=CARTESIAN_POINT('Ctrl Pts',(-1.179753362735,-71.0474460837157,0.));
#131356=CARTESIAN_POINT('Ctrl Pts',(-1.17266837175776,-71.0265340757697,
0.));
#131357=CARTESIAN_POINT('Ctrl Pts',(-1.16561977112882,-71.0056595152204,
0.));
#131358=CARTESIAN_POINT('Ctrl Pts',(-1.1586075391149,-70.9848225647876,
0.));
#131359=CARTESIAN_POINT('Ctrl Pts',(-1.1516316537653,-70.9640233879671,
0.));
#131360=CARTESIAN_POINT('Ctrl Pts',(-1.14469209291494,-70.943262149058,
0.));
#131361=CARTESIAN_POINT('Ctrl Pts',(-1.13778883418216,-70.9225390131835,
0.));
#131362=CARTESIAN_POINT('Ctrl Pts',(-1.13092185496563,-70.9018541463083,
0.));
#131363=CARTESIAN_POINT('Ctrl Pts',(-1.12409113243511,-70.8812077152564,
0.));
#131364=CARTESIAN_POINT('Ctrl Pts',(-1.1172966435299,-70.860599887712,0.));
#131365=CARTESIAN_POINT('Ctrl Pts',(-1.11053836496638,-70.8400308322013,
0.));
#131366=CARTESIAN_POINT('Ctrl Pts',(-1.10381627323946,-70.8195007180739,
0.));
#131367=CARTESIAN_POINT('Ctrl Pts',(-1.0971303446227,-70.7990097154855,
0.));
#131368=CARTESIAN_POINT('Ctrl Pts',(-1.09048055516434,-70.7785579953611,
0.));
#131369=CARTESIAN_POINT('Ctrl Pts',(-1.08386688068349,-70.7581457294475,
0.));
#131370=CARTESIAN_POINT('Ctrl Pts',(-1.07728929676412,-70.737773090397,
0.));
#131371=CARTESIAN_POINT('Ctrl Pts',(-1.07074777874596,-70.7174402518378,
0.));
#131372=CARTESIAN_POINT('Ctrl Pts',(-1.0642423017128,-70.6971473884443,
0.));
#131373=CARTESIAN_POINT('Ctrl Pts',(-1.05777284047728,-70.6768946760063,
0.));
#131374=CARTESIAN_POINT('Ctrl Pts',(-1.05133936960069,-70.6566822912965,
0.));
#131375=CARTESIAN_POINT('Ctrl Pts',(-1.04494186341156,-70.6365104119238,
0.));
#131376=CARTESIAN_POINT('Ctrl Pts',(-1.03858029601906,-70.6163792162079,
0.));
#131377=CARTESIAN_POINT('Ctrl Pts',(-1.03225464132872,-70.5962888829958,
0.));
#131378=CARTESIAN_POINT('Ctrl Pts',(-1.02596487304049,-70.5762395916412,
0.));
#131379=CARTESIAN_POINT('Ctrl Pts',(-1.01971096460599,-70.5562315224219,
0.));
#131380=CARTESIAN_POINT('Ctrl Pts',(-1.0134928891854,-70.5362648569072,
0.));
#131381=CARTESIAN_POINT('Ctrl Pts',(-1.00731061960968,-70.5163397782699,
0.));
#131382=CARTESIAN_POINT('Ctrl Pts',(-1.00116412831438,-70.4964564717917,
0.));
#131383=CARTESIAN_POINT('Ctrl Pts',(-0.995053387379681,-70.476615124517,
0.));
#131384=CARTESIAN_POINT('Ctrl Pts',(-0.98897836864359,-70.4568159243131,
0.));
#131385=CARTESIAN_POINT('Ctrl Pts',(-0.982939043792158,-70.4370590590839,
0.));
#131386=CARTESIAN_POINT('Ctrl Pts',(-0.976935384450128,-70.41734471596,
0.));
#131387=CARTESIAN_POINT('Ctrl Pts',(-0.970967362281301,-70.3976730803664,
0.));
#131388=CARTESIAN_POINT('Ctrl Pts',(-0.965034948786559,-70.3780443378003,
0.));
#131389=CARTESIAN_POINT('Ctrl Pts',(-0.959138115058886,-70.3584586759561,
0.));
#131390=CARTESIAN_POINT('Ctrl Pts',(-0.953276831581232,-70.338916286457,
0.));
#131391=CARTESIAN_POINT('Ctrl Pts',(-0.947451067929564,-70.3194173673635,
0.));
#131392=CARTESIAN_POINT('Ctrl Pts',(-0.941660792742953,-70.2999621233938,
0.));
#131393=CARTESIAN_POINT('Ctrl Pts',(-0.935905974336492,-70.2805507606832,
0.));
#131394=CARTESIAN_POINT('Ctrl Pts',(-0.930186581235576,-70.2611834821711,
0.));
#131395=CARTESIAN_POINT('Ctrl Pts',(-0.924502582639453,-70.241860483586,
0.));
#131396=CARTESIAN_POINT('Ctrl Pts',(-0.918853949157045,-70.2225819470306,
0.));
#131397=CARTESIAN_POINT('Ctrl Pts',(-0.913240652090839,-70.2033480471749,
0.));
#131398=CARTESIAN_POINT('Ctrl Pts',(-0.90766266201565,-70.184158963563,
0.));
#131399=CARTESIAN_POINT('Ctrl Pts',(-0.902119947629773,-70.1650148905109,
0.));
#131400=CARTESIAN_POINT('Ctrl Pts',(-0.896612474372085,-70.1459160490366,
0.));
#131401=CARTESIAN_POINT('Ctrl Pts',(-0.891140203464724,-70.1268626950031,
0.));
#131402=CARTESIAN_POINT('Ctrl Pts',(-0.885703094803086,-70.1078550938801,
0.));
#131403=CARTESIAN_POINT('Ctrl Pts',(-0.880301109661037,-70.0888934967772,
0.));
#131404=CARTESIAN_POINT('Ctrl Pts',(-0.87493421325557,-70.0699781184013,
0.));
#131405=CARTESIAN_POINT('Ctrl Pts',(-0.869602377870139,-70.0511091083285,
0.));
#131406=CARTESIAN_POINT('Ctrl Pts',(-0.86430558366009,-70.0322865493339,
0.));
#131407=CARTESIAN_POINT('Ctrl Pts',(-0.860096170667398,-70.0172656934192,
0.));
#131408=CARTESIAN_POINT('Ctrl Pts',(-0.856954870258371,-70.0060209754332,
0.));
#131409=CARTESIAN_POINT('Ctrl Pts',(-0.854867673848293,-69.9985337959499,
0.));
#131410=CARTESIAN_POINT('Ctrl Pts',(-0.853825826608993,-69.9947925310006,
0.));
#131411=CARTESIAN_POINT('Ctrl Pts',(-9.10443154852688,-73.9415940197274,
0.));
#131412=CARTESIAN_POINT('Ctrl Pts',(-9.10443154852688,-73.9415940197274,
12.));
#131413=CARTESIAN_POINT('Ctrl Pts',(-9.10148558516537,-73.9368365074299,
0.));
#131414=CARTESIAN_POINT('Ctrl Pts',(-9.10148558516537,-73.9368365074299,
12.));
#131415=CARTESIAN_POINT('Ctrl Pts',(-9.09559760529042,-73.9273231219835,
0.));
#131416=CARTESIAN_POINT('Ctrl Pts',(-9.09559760529042,-73.9273231219835,
12.));
#131417=CARTESIAN_POINT('Ctrl Pts',(-9.08677747602205,-73.9130579612604,
0.));
#131418=CARTESIAN_POINT('Ctrl Pts',(-9.08677747602205,-73.9130579612604,
12.));
#131419=CARTESIAN_POINT('Ctrl Pts',(-9.07504098571707,-73.8940475822492,
0.));
#131420=CARTESIAN_POINT('Ctrl Pts',(-9.07504098571707,-73.8940475822492,
12.));
#131421=CARTESIAN_POINT('Ctrl Pts',(-9.06040984890246,-73.8703010078091,
0.));
#131422=CARTESIAN_POINT('Ctrl Pts',(-9.06040984890246,-73.8703010078091,
12.));
#131423=CARTESIAN_POINT('Ctrl Pts',(-9.04581819646984,-73.8465708501057,
0.));
#131424=CARTESIAN_POINT('Ctrl Pts',(-9.04581819646984,-73.8465708501057,
12.));
#131425=CARTESIAN_POINT('Ctrl Pts',(-9.03126603778125,-73.8228571411697,
0.));
#131426=CARTESIAN_POINT('Ctrl Pts',(-9.03126603778125,-73.8228571411697,
12.));
#131427=CARTESIAN_POINT('Ctrl Pts',(-9.01675338208004,-73.7991599312592,
0.));
#131428=CARTESIAN_POINT('Ctrl Pts',(-9.01675338208004,-73.7991599312592,
12.));
#131429=CARTESIAN_POINT('Ctrl Pts',(-9.00228023701055,-73.7754792943665,
0.));
#131430=CARTESIAN_POINT('Ctrl Pts',(-9.00228023701055,-73.7754792943665,
12.));
#131431=CARTESIAN_POINT('Ctrl Pts',(-8.98784660837397,-73.7518153261981,
0.));
#131432=CARTESIAN_POINT('Ctrl Pts',(-8.98784660837397,-73.7518153261981,
12.));
#131433=CARTESIAN_POINT('Ctrl Pts',(-8.97345250083601,-73.728168136383,
0.));
#131434=CARTESIAN_POINT('Ctrl Pts',(-8.97345250083601,-73.728168136383,
12.));
#131435=CARTESIAN_POINT('Ctrl Pts',(-8.95909791836152,-73.7045378422686,
0.));
#131436=CARTESIAN_POINT('Ctrl Pts',(-8.95909791836152,-73.7045378422686,
12.));
#131437=CARTESIAN_POINT('Ctrl Pts',(-8.94478286474419,-73.6809245622383,
0.));
#131438=CARTESIAN_POINT('Ctrl Pts',(-8.94478286474419,-73.6809245622383,
12.));
#131439=CARTESIAN_POINT('Ctrl Pts',(-8.93050734412124,-73.6573284088184,
0.));
#131440=CARTESIAN_POINT('Ctrl Pts',(-8.93050734412124,-73.6573284088184,
12.));
#131441=CARTESIAN_POINT('Ctrl Pts',(-8.91627136140084,-73.633749483097,
0.));
#131442=CARTESIAN_POINT('Ctrl Pts',(-8.91627136140084,-73.633749483097,
12.));
#131443=CARTESIAN_POINT('Ctrl Pts',(-8.90207492199043,-73.6101878785976,
0.));
#131444=CARTESIAN_POINT('Ctrl Pts',(-8.90207492199043,-73.6101878785976,
12.));
#131445=CARTESIAN_POINT('Ctrl Pts',(-8.88791803160442,-73.5866436840556,
0.));
#131446=CARTESIAN_POINT('Ctrl Pts',(-8.88791803160442,-73.5866436840556,
12.));
#131447=CARTESIAN_POINT('Ctrl Pts',(-8.8738006960297,-73.5631169867122,
0.));
#131448=CARTESIAN_POINT('Ctrl Pts',(-8.8738006960297,-73.5631169867122,
12.));
#131449=CARTESIAN_POINT('Ctrl Pts',(-8.8597229209213,-73.5396078751639,
0.));
#131450=CARTESIAN_POINT('Ctrl Pts',(-8.8597229209213,-73.5396078751639,
12.));
#131451=CARTESIAN_POINT('Ctrl Pts',(-8.84568471153805,-73.5161164429709,
0.));
#131452=CARTESIAN_POINT('Ctrl Pts',(-8.84568471153805,-73.5161164429709,
12.));
#131453=CARTESIAN_POINT('Ctrl Pts',(-8.83168607277325,-73.492642788273,
0.));
#131454=CARTESIAN_POINT('Ctrl Pts',(-8.83168607277325,-73.492642788273,
12.));
#131455=CARTESIAN_POINT('Ctrl Pts',(-8.8177270092753,-73.4691870121567,
0.));
#131456=CARTESIAN_POINT('Ctrl Pts',(-8.8177270092753,-73.4691870121567,
12.));
#131457=CARTESIAN_POINT('Ctrl Pts',(-8.80380752553691,-73.4457492173933,
0.));
#131458=CARTESIAN_POINT('Ctrl Pts',(-8.80380752553691,-73.4457492173933,
12.));
#131459=CARTESIAN_POINT('Ctrl Pts',(-8.78992762598756,-73.422329507113,
0.));
#131460=CARTESIAN_POINT('Ctrl Pts',(-8.78992762598756,-73.422329507113,
12.));
#131461=CARTESIAN_POINT('Ctrl Pts',(-8.77608731509347,-73.3989279832835,
0.));
#131462=CARTESIAN_POINT('Ctrl Pts',(-8.77608731509347,-73.3989279832835,
12.));
#131463=CARTESIAN_POINT('Ctrl Pts',(-8.76228659740357,-73.3755447460269,
0.));
#131464=CARTESIAN_POINT('Ctrl Pts',(-8.76228659740357,-73.3755447460269,
12.));
#131465=CARTESIAN_POINT('Ctrl Pts',(-8.74852547749778,-73.3521798944622,
0.));
#131466=CARTESIAN_POINT('Ctrl Pts',(-8.74852547749778,-73.3521798944622,
12.));
#131467=CARTESIAN_POINT('Ctrl Pts',(-8.7348039599538,-73.3288335272002,
0.));
#131468=CARTESIAN_POINT('Ctrl Pts',(-8.7348039599538,-73.3288335272002,
12.));
#131469=CARTESIAN_POINT('Ctrl Pts',(-8.72112204930231,-73.3055057429742,
0.));
#131470=CARTESIAN_POINT('Ctrl Pts',(-8.72112204930231,-73.3055057429742,
12.));
#131471=CARTESIAN_POINT('Ctrl Pts',(-8.70747974998229,-73.2821966412148,
0.));
#131472=CARTESIAN_POINT('Ctrl Pts',(-8.70747974998229,-73.2821966412148,
12.));
#131473=CARTESIAN_POINT('Ctrl Pts',(-8.69387706629285,-73.2589063226358,
0.));
#131474=CARTESIAN_POINT('Ctrl Pts',(-8.69387706629285,-73.2589063226358,
12.));
#131475=CARTESIAN_POINT('Ctrl Pts',(-8.68031400241871,-73.2356348889693,
0.));
#131476=CARTESIAN_POINT('Ctrl Pts',(-8.68031400241871,-73.2356348889693,
12.));
#131477=CARTESIAN_POINT('Ctrl Pts',(-8.66679056245091,-73.2123824427208,
0.));
#131478=CARTESIAN_POINT('Ctrl Pts',(-8.66679056245091,-73.2123824427208,
12.));
#131479=CARTESIAN_POINT('Ctrl Pts',(-8.65330675040536,-73.1891490869056,
0.));
#131480=CARTESIAN_POINT('Ctrl Pts',(-8.65330675040536,-73.1891490869056,
12.));
#131481=CARTESIAN_POINT('Ctrl Pts',(-8.63986257023738,-73.1659349248132,
0.));
#131482=CARTESIAN_POINT('Ctrl Pts',(-8.63986257023738,-73.1659349248132,
12.));
#131483=CARTESIAN_POINT('Ctrl Pts',(-8.62645802585483,-73.1427400597037,
0.));
#131484=CARTESIAN_POINT('Ctrl Pts',(-8.62645802585483,-73.1427400597037,
12.));
#131485=CARTESIAN_POINT('Ctrl Pts',(-8.61309312112001,-73.1195645948178,
0.));
#131486=CARTESIAN_POINT('Ctrl Pts',(-8.61309312112001,-73.1195645948178,
12.));
#131487=CARTESIAN_POINT('Ctrl Pts',(-8.59976785984551,-73.0964086335235,
0.));
#131488=CARTESIAN_POINT('Ctrl Pts',(-8.59976785984551,-73.0964086335235,
12.));
#131489=CARTESIAN_POINT('Ctrl Pts',(-8.58648224578731,-73.0732722794195,
0.));
#131490=CARTESIAN_POINT('Ctrl Pts',(-8.58648224578731,-73.0732722794195,
12.));
#131491=CARTESIAN_POINT('Ctrl Pts',(-8.57323628263593,-73.0501556364479,
0.));
#131492=CARTESIAN_POINT('Ctrl Pts',(-8.57323628263593,-73.0501556364479,
12.));
#131493=CARTESIAN_POINT('Ctrl Pts',(-8.56002997400083,-73.0270588090183,
0.));
#131494=CARTESIAN_POINT('Ctrl Pts',(-8.56002997400083,-73.0270588090183,
12.));
#131495=CARTESIAN_POINT('Ctrl Pts',(-8.54686332340417,-73.0039819020648,
0.));
#131496=CARTESIAN_POINT('Ctrl Pts',(-8.54686332340417,-73.0039819020648,
12.));
#131497=CARTESIAN_POINT('Ctrl Pts',(-8.5337363342928,-72.9809250209828,
0.));
#131498=CARTESIAN_POINT('Ctrl Pts',(-8.5337363342928,-72.9809250209828,
12.));
#131499=CARTESIAN_POINT('Ctrl Pts',(-8.52064901004227,-72.9578882715912,
0.));
#131500=CARTESIAN_POINT('Ctrl Pts',(-8.52064901004227,-72.9578882715912,
12.));
#131501=CARTESIAN_POINT('Ctrl Pts',(-8.50760135395983,-72.9348717600838,
0.));
#131502=CARTESIAN_POINT('Ctrl Pts',(-8.50760135395983,-72.9348717600838,
12.));
#131503=CARTESIAN_POINT('Ctrl Pts',(-8.49459336928295,-72.9118755929795,
0.));
#131504=CARTESIAN_POINT('Ctrl Pts',(-8.49459336928295,-72.9118755929795,
12.));
#131505=CARTESIAN_POINT('Ctrl Pts',(-8.48162505917657,-72.8888998770785,
0.));
#131506=CARTESIAN_POINT('Ctrl Pts',(-8.48162505917657,-72.8888998770785,
12.));
#131507=CARTESIAN_POINT('Ctrl Pts',(-8.46869642673794,-72.8659447194933,
0.));
#131508=CARTESIAN_POINT('Ctrl Pts',(-8.46869642673794,-72.8659447194933,
12.));
#131509=CARTESIAN_POINT('Ctrl Pts',(-8.45580747499793,-72.8430102276713,
0.));
#131510=CARTESIAN_POINT('Ctrl Pts',(-8.45580747499793,-72.8430102276713,
12.));
#131511=CARTESIAN_POINT('Ctrl Pts',(-8.44295820691911,-72.8200965094199,
0.));
#131512=CARTESIAN_POINT('Ctrl Pts',(-8.44295820691911,-72.8200965094199,
12.));
#131513=CARTESIAN_POINT('Ctrl Pts',(-8.43014862539157,-72.7972036729276,
0.));
#131514=CARTESIAN_POINT('Ctrl Pts',(-8.43014862539157,-72.7972036729276,
12.));
#131515=CARTESIAN_POINT('Ctrl Pts',(-8.41737873322329,-72.7743318267865,
0.));
#131516=CARTESIAN_POINT('Ctrl Pts',(-8.41737873322329,-72.7743318267865,
12.));
#131517=CARTESIAN_POINT('Ctrl Pts',(-8.40464853314468,-72.751481079992,
0.));
#131518=CARTESIAN_POINT('Ctrl Pts',(-8.40464853314468,-72.751481079992,
12.));
#131519=CARTESIAN_POINT('Ctrl Pts',(-8.3919580278139,-72.7286515419373,
0.));
#131520=CARTESIAN_POINT('Ctrl Pts',(-8.3919580278139,-72.7286515419373,
12.));
#131521=CARTESIAN_POINT('Ctrl Pts',(-8.37930721981731,-72.705843322407,
0.));
#131522=CARTESIAN_POINT('Ctrl Pts',(-8.37930721981731,-72.705843322407,
12.));
#131523=CARTESIAN_POINT('Ctrl Pts',(-8.36669611166842,-72.6830565315703,
0.));
#131524=CARTESIAN_POINT('Ctrl Pts',(-8.36669611166842,-72.6830565315703,
12.));
#131525=CARTESIAN_POINT('Ctrl Pts',(-8.35412470580101,-72.6602912799696,
0.));
#131526=CARTESIAN_POINT('Ctrl Pts',(-8.35412470580101,-72.6602912799696,
12.));
#131527=CARTESIAN_POINT('Ctrl Pts',(-8.34159300456986,-72.6375476785215,
0.));
#131528=CARTESIAN_POINT('Ctrl Pts',(-8.34159300456986,-72.6375476785215,
12.));
#131529=CARTESIAN_POINT('Ctrl Pts',(-8.3291010102567,-72.6148258385296,
0.));
#131530=CARTESIAN_POINT('Ctrl Pts',(-8.3291010102567,-72.6148258385296,
12.));
#131531=CARTESIAN_POINT('Ctrl Pts',(-8.31664872507016,-72.5921258716901,
0.));
#131532=CARTESIAN_POINT('Ctrl Pts',(-8.31664872507016,-72.5921258716901,
12.));
#131533=CARTESIAN_POINT('Ctrl Pts',(-8.30423615114452,-72.5694478900982,
0.));
#131534=CARTESIAN_POINT('Ctrl Pts',(-8.30423615114452,-72.5694478900982,
12.));
#131535=CARTESIAN_POINT('Ctrl Pts',(-8.29186329053279,-72.5467920062521,
0.));
#131536=CARTESIAN_POINT('Ctrl Pts',(-8.29186329053279,-72.5467920062521,
12.));
#131537=CARTESIAN_POINT('Ctrl Pts',(-8.27953014520376,-72.5241583330562,
0.));
#131538=CARTESIAN_POINT('Ctrl Pts',(-8.27953014520376,-72.5241583330562,
12.));
#131539=CARTESIAN_POINT('Ctrl Pts',(-8.26723671704919,-72.5015469838254,
0.));
#131540=CARTESIAN_POINT('Ctrl Pts',(-8.26723671704919,-72.5015469838254,
12.));
#131541=CARTESIAN_POINT('Ctrl Pts',(-8.25498300788493,-72.4789580722875,
0.));
#131542=CARTESIAN_POINT('Ctrl Pts',(-8.25498300788493,-72.4789580722875,
12.));
#131543=CARTESIAN_POINT('Ctrl Pts',(-8.2427690194504,-72.4563917125842,
0.));
#131544=CARTESIAN_POINT('Ctrl Pts',(-8.2427690194504,-72.4563917125842,
12.));
#131545=CARTESIAN_POINT('Ctrl Pts',(-8.23059475340356,-72.4338480192695,
0.));
#131546=CARTESIAN_POINT('Ctrl Pts',(-8.23059475340356,-72.4338480192695,
12.));
#131547=CARTESIAN_POINT('Ctrl Pts',(-8.2184602113156,-72.4113271073079,
0.));
#131548=CARTESIAN_POINT('Ctrl Pts',(-8.2184602113156,-72.4113271073079,
12.));
#131549=CARTESIAN_POINT('Ctrl Pts',(-8.20636539467776,-72.3888290920832,
0.));
#131550=CARTESIAN_POINT('Ctrl Pts',(-8.20636539467776,-72.3888290920832,
12.));
#131551=CARTESIAN_POINT('Ctrl Pts',(-8.19431030490314,-72.3663540894026,
0.));
#131552=CARTESIAN_POINT('Ctrl Pts',(-8.19431030490314,-72.3663540894026,
12.));
#131553=CARTESIAN_POINT('Ctrl Pts',(-8.18229494332623,-72.3439022155007,
0.));
#131554=CARTESIAN_POINT('Ctrl Pts',(-8.18229494332623,-72.3439022155007,
12.));
#131555=CARTESIAN_POINT('Ctrl Pts',(-8.1703193111989,-72.3214735870409,
0.));
#131556=CARTESIAN_POINT('Ctrl Pts',(-8.1703193111989,-72.3214735870409,
12.));
#131557=CARTESIAN_POINT('Ctrl Pts',(-8.15838340968335,-72.2990683211162,
0.));
#131558=CARTESIAN_POINT('Ctrl Pts',(-8.15838340968335,-72.2990683211162,
12.));
#131559=CARTESIAN_POINT('Ctrl Pts',(-8.14648723985797,-72.2766865352555,
0.));
#131560=CARTESIAN_POINT('Ctrl Pts',(-8.14648723985797,-72.2766865352555,
12.));
#131561=CARTESIAN_POINT('Ctrl Pts',(-8.13463080272028,-72.2543283474278,
0.));
#131562=CARTESIAN_POINT('Ctrl Pts',(-8.13463080272028,-72.2543283474278,
12.));
#131563=CARTESIAN_POINT('Ctrl Pts',(-8.1228140991866,-72.2319938760449,
0.));
#131564=CARTESIAN_POINT('Ctrl Pts',(-8.1228140991866,-72.2319938760449,
12.));
#131565=CARTESIAN_POINT('Ctrl Pts',(-8.11103713008928,-72.209683239963,
0.));
#131566=CARTESIAN_POINT('Ctrl Pts',(-8.11103713008928,-72.209683239963,
12.));
#131567=CARTESIAN_POINT('Ctrl Pts',(-8.09929989616889,-72.1873965584813,
0.));
#131568=CARTESIAN_POINT('Ctrl Pts',(-8.09929989616889,-72.1873965584813,
12.));
#131569=CARTESIAN_POINT('Ctrl Pts',(-8.08760239807836,-72.1651339513477,
0.));
#131570=CARTESIAN_POINT('Ctrl Pts',(-8.08760239807836,-72.1651339513477,
12.));
#131571=CARTESIAN_POINT('Ctrl Pts',(-8.07594463638719,-72.1428955387663,
0.));
#131572=CARTESIAN_POINT('Ctrl Pts',(-8.07594463638719,-72.1428955387663,
12.));
#131573=CARTESIAN_POINT('Ctrl Pts',(-8.06432661158095,-72.1206814413988,
0.));
#131574=CARTESIAN_POINT('Ctrl Pts',(-8.06432661158095,-72.1206814413988,
12.));
#131575=CARTESIAN_POINT('Ctrl Pts',(-8.05274832405948,-72.0984917803693,
0.));
#131576=CARTESIAN_POINT('Ctrl Pts',(-8.05274832405948,-72.0984917803693,
12.));
#131577=CARTESIAN_POINT('Ctrl Pts',(-8.04120977412872,-72.0763266772615,
0.));
#131578=CARTESIAN_POINT('Ctrl Pts',(-8.04120977412872,-72.0763266772615,
12.));
#131579=CARTESIAN_POINT('Ctrl Pts',(-8.02971096200307,-72.0541862541243,
0.));
#131580=CARTESIAN_POINT('Ctrl Pts',(-8.02971096200307,-72.0541862541243,
12.));
#131581=CARTESIAN_POINT('Ctrl Pts',(-8.01825188781056,-72.032070633479,
0.));
#131582=CARTESIAN_POINT('Ctrl Pts',(-8.01825188781056,-72.032070633479,
12.));
#131583=CARTESIAN_POINT('Ctrl Pts',(-8.00683255159247,-72.0099799383213,
0.));
#131584=CARTESIAN_POINT('Ctrl Pts',(-8.00683255159247,-72.0099799383213,
12.));
#131585=CARTESIAN_POINT('Ctrl Pts',(-7.99545295330191,-71.9879142921254,
0.));
#131586=CARTESIAN_POINT('Ctrl Pts',(-7.99545295330191,-71.9879142921254,
12.));
#131587=CARTESIAN_POINT('Ctrl Pts',(-7.98411309279612,-71.965873818843,
0.));
#131588=CARTESIAN_POINT('Ctrl Pts',(-7.98411309279612,-71.965873818843,
12.));
#131589=CARTESIAN_POINT('Ctrl Pts',(-7.97281296983717,-71.9438586429081,
0.));
#131590=CARTESIAN_POINT('Ctrl Pts',(-7.97281296983717,-71.9438586429081,
12.));
#131591=CARTESIAN_POINT('Ctrl Pts',(-7.96155258409763,-71.9218688892431,
0.));
#131592=CARTESIAN_POINT('Ctrl Pts',(-7.96155258409763,-71.9218688892431,
12.));
#131593=CARTESIAN_POINT('Ctrl Pts',(-7.9503319351605,-71.8999046832643,
0.));
#131594=CARTESIAN_POINT('Ctrl Pts',(-7.9503319351605,-71.8999046832643,
12.));
#131595=CARTESIAN_POINT('Ctrl Pts',(-7.93915102251794,-71.8779661508832,
0.));
#131596=CARTESIAN_POINT('Ctrl Pts',(-7.93915102251794,-71.8779661508832,
12.));
#131597=CARTESIAN_POINT('Ctrl Pts',(-7.92800984556395,-71.8560534185071,
0.));
#131598=CARTESIAN_POINT('Ctrl Pts',(-7.92800984556395,-71.8560534185071,
12.));
#131599=CARTESIAN_POINT('Ctrl Pts',(-7.91690840359367,-71.8341666130426,
0.));
#131600=CARTESIAN_POINT('Ctrl Pts',(-7.91690840359367,-71.8341666130426,
12.));
#131601=CARTESIAN_POINT('Ctrl Pts',(-7.90584669580955,-71.8123058619042,
0.));
#131602=CARTESIAN_POINT('Ctrl Pts',(-7.90584669580955,-71.8123058619042,
12.));
#131603=CARTESIAN_POINT('Ctrl Pts',(-7.89482472132137,-71.7904712930175,
0.));
#131604=CARTESIAN_POINT('Ctrl Pts',(-7.89482472132137,-71.7904712930175,
12.));
#131605=CARTESIAN_POINT('Ctrl Pts',(-7.88384247914523,-71.7686630348238,
0.));
#131606=CARTESIAN_POINT('Ctrl Pts',(-7.88384247914523,-71.7686630348238,
12.));
#131607=CARTESIAN_POINT('Ctrl Pts',(-7.87289996819653,-71.7468812162788,
0.));
#131608=CARTESIAN_POINT('Ctrl Pts',(-7.87289996819653,-71.7468812162788,
12.));
#131609=CARTESIAN_POINT('Ctrl Pts',(-7.86199718728826,-71.7251259668563,
0.));
#131610=CARTESIAN_POINT('Ctrl Pts',(-7.86199718728826,-71.7251259668563,
12.));
#131611=CARTESIAN_POINT('Ctrl Pts',(-7.85113413513735,-71.7033974165568,
0.));
#131612=CARTESIAN_POINT('Ctrl Pts',(-7.85113413513735,-71.7033974165568,
12.));
#131613=CARTESIAN_POINT('Ctrl Pts',(-7.84031081036489,-71.6816956959117,
0.));
#131614=CARTESIAN_POINT('Ctrl Pts',(-7.84031081036489,-71.6816956959117,
12.));
#131615=CARTESIAN_POINT('Ctrl Pts',(-7.82952721149507,-71.6600209359872,
0.));
#131616=CARTESIAN_POINT('Ctrl Pts',(-7.82952721149507,-71.6600209359872,
12.));
#131617=CARTESIAN_POINT('Ctrl Pts',(-7.8187833369486,-71.6383732683844,
0.));
#131618=CARTESIAN_POINT('Ctrl Pts',(-7.8187833369486,-71.6383732683844,
12.));
#131619=CARTESIAN_POINT('Ctrl Pts',(-7.80807918504021,-71.6167528252423,
0.));
#131620=CARTESIAN_POINT('Ctrl Pts',(-7.80807918504021,-71.6167528252423,
12.));
#131621=CARTESIAN_POINT('Ctrl Pts',(-7.79741475398513,-71.5951597392471,
0.));
#131622=CARTESIAN_POINT('Ctrl Pts',(-7.79741475398513,-71.5951597392471,
12.));
#131623=CARTESIAN_POINT('Ctrl Pts',(-7.78679004189934,-71.5735941436364,
0.));
#131624=CARTESIAN_POINT('Ctrl Pts',(-7.78679004189934,-71.5735941436364,
12.));
#131625=CARTESIAN_POINT('Ctrl Pts',(-7.77620504679869,-71.5520561722039,
0.));
#131626=CARTESIAN_POINT('Ctrl Pts',(-7.77620504679869,-71.5520561722039,
12.));
#131627=CARTESIAN_POINT('Ctrl Pts',(-7.76565976659226,-71.5305459592994,
0.));
#131628=CARTESIAN_POINT('Ctrl Pts',(-7.76565976659226,-71.5305459592994,
12.));
#131629=CARTESIAN_POINT('Ctrl Pts',(-7.75515419907966,-71.5090636398318,
0.));
#131630=CARTESIAN_POINT('Ctrl Pts',(-7.75515419907966,-71.5090636398318,
12.));
#131631=CARTESIAN_POINT('Ctrl Pts',(-7.74468834195746,-71.4876093492781,
0.));
#131632=CARTESIAN_POINT('Ctrl Pts',(-7.74468834195746,-71.4876093492781,
12.));
#131633=CARTESIAN_POINT('Ctrl Pts',(-7.7342621928194,-71.4661832236888,
0.));
#131634=CARTESIAN_POINT('Ctrl Pts',(-7.7342621928194,-71.4661832236888,
12.));
#131635=CARTESIAN_POINT('Ctrl Pts',(-7.72387574915544,-71.4447853996916,
0.));
#131636=CARTESIAN_POINT('Ctrl Pts',(-7.72387574915544,-71.4447853996916,
12.));
#131637=CARTESIAN_POINT('Ctrl Pts',(-7.7135290083452,-71.4234160144925,
0.));
#131638=CARTESIAN_POINT('Ctrl Pts',(-7.7135290083452,-71.4234160144925,
12.));
#131639=CARTESIAN_POINT('Ctrl Pts',(-7.70322196765538,-71.4020752058796,
0.));
#131640=CARTESIAN_POINT('Ctrl Pts',(-7.70322196765538,-71.4020752058796,
12.));
#131641=CARTESIAN_POINT('Ctrl Pts',(-7.69295462424611,-71.3807631122331,
0.));
#131642=CARTESIAN_POINT('Ctrl Pts',(-7.69295462424611,-71.3807631122331,
12.));
#131643=CARTESIAN_POINT('Ctrl Pts',(-7.68272697517086,-71.3594798725281,
0.));
#131644=CARTESIAN_POINT('Ctrl Pts',(-7.68272697517086,-71.3594798725281,
12.));
#131645=CARTESIAN_POINT('Ctrl Pts',(-7.67253901737552,-71.3382256263414,
0.));
#131646=CARTESIAN_POINT('Ctrl Pts',(-7.67253901737552,-71.3382256263414,
12.));
#131647=CARTESIAN_POINT('Ctrl Pts',(-7.66239074769163,-71.3170005138502,
0.));
#131648=CARTESIAN_POINT('Ctrl Pts',(-7.66239074769163,-71.3170005138502,
12.));
#131649=CARTESIAN_POINT('Ctrl Pts',(-7.65228216283403,-71.2958046758372,
0.));
#131650=CARTESIAN_POINT('Ctrl Pts',(-7.65228216283403,-71.2958046758372,
12.));
#131651=CARTESIAN_POINT('Ctrl Pts',(-7.64221325940724,-71.2746382537007,
0.));
#131652=CARTESIAN_POINT('Ctrl Pts',(-7.64221325940724,-71.2746382537007,
12.));
#131653=CARTESIAN_POINT('Ctrl Pts',(-7.63218403390537,-71.2535013894602,
0.));
#131654=CARTESIAN_POINT('Ctrl Pts',(-7.63218403390537,-71.2535013894602,
12.));
#131655=CARTESIAN_POINT('Ctrl Pts',(-7.62219448271109,-71.2323942257609,
0.));
#131656=CARTESIAN_POINT('Ctrl Pts',(-7.62219448271109,-71.2323942257609,
12.));
#131657=CARTESIAN_POINT('Ctrl Pts',(-7.61224460208837,-71.211316905874,
0.));
#131658=CARTESIAN_POINT('Ctrl Pts',(-7.61224460208837,-71.211316905874,
12.));
#131659=CARTESIAN_POINT('Ctrl Pts',(-7.60233438818096,-71.1902695737013,
0.));
#131660=CARTESIAN_POINT('Ctrl Pts',(-7.60233438818096,-71.1902695737013,
12.));
#131661=CARTESIAN_POINT('Ctrl Pts',(-7.59246383701813,-71.1692523737844,
0.));
#131662=CARTESIAN_POINT('Ctrl Pts',(-7.59246383701813,-71.1692523737844,
12.));
#131663=CARTESIAN_POINT('Ctrl Pts',(-7.58263294451451,-71.1482654513119,
0.));
#131664=CARTESIAN_POINT('Ctrl Pts',(-7.58263294451451,-71.1482654513119,
12.));
#131665=CARTESIAN_POINT('Ctrl Pts',(-7.57284170646886,-71.1273089521234,
0.));
#131666=CARTESIAN_POINT('Ctrl Pts',(-7.57284170646886,-71.1273089521234,
12.));
#131667=CARTESIAN_POINT('Ctrl Pts',(-7.56309011855657,-71.106383022711,
0.));
#131668=CARTESIAN_POINT('Ctrl Pts',(-7.56309011855657,-71.106383022711,
12.));
#131669=CARTESIAN_POINT('Ctrl Pts',(-7.55337817632916,-71.0854878102243,
0.));
#131670=CARTESIAN_POINT('Ctrl Pts',(-7.55337817632916,-71.0854878102243,
12.));
#131671=CARTESIAN_POINT('Ctrl Pts',(-7.54370587521979,-71.0646234624811,
0.));
#131672=CARTESIAN_POINT('Ctrl Pts',(-7.54370587521979,-71.0646234624811,
12.));
#131673=CARTESIAN_POINT('Ctrl Pts',(-7.53407321054262,-71.043790127973,
0.));
#131674=CARTESIAN_POINT('Ctrl Pts',(-7.53407321054262,-71.043790127973,
12.));
#131675=CARTESIAN_POINT('Ctrl Pts',(-7.52448017749124,-71.0229879558699,
0.));
#131676=CARTESIAN_POINT('Ctrl Pts',(-7.52448017749124,-71.0229879558699,
12.));
#131677=CARTESIAN_POINT('Ctrl Pts',(-7.5149267711309,-71.002217096021,0.));
#131678=CARTESIAN_POINT('Ctrl Pts',(-7.5149267711309,-71.002217096021,12.));
#131679=CARTESIAN_POINT('Ctrl Pts',(-7.50541298639928,-70.9814776989612,
0.));
#131680=CARTESIAN_POINT('Ctrl Pts',(-7.50541298639928,-70.9814776989612,
12.));
#131681=CARTESIAN_POINT('Ctrl Pts',(-7.4959388181113,-70.9607699159218,
0.));
#131682=CARTESIAN_POINT('Ctrl Pts',(-7.4959388181113,-70.9607699159218,
12.));
#131683=CARTESIAN_POINT('Ctrl Pts',(-7.48650426095823,-70.940093898837,
0.));
#131684=CARTESIAN_POINT('Ctrl Pts',(-7.48650426095823,-70.940093898837,
12.));
#131685=CARTESIAN_POINT('Ctrl Pts',(-7.47710930950562,-70.9194498003493,
0.));
#131686=CARTESIAN_POINT('Ctrl Pts',(-7.47710930950562,-70.9194498003493,
12.));
#131687=CARTESIAN_POINT('Ctrl Pts',(-7.46775395818527,-70.8988377738104,
0.));
#131688=CARTESIAN_POINT('Ctrl Pts',(-7.46775395818527,-70.8988377738104,
12.));
#131689=CARTESIAN_POINT('Ctrl Pts',(-7.45843820129782,-70.87825797329,0.));
#131690=CARTESIAN_POINT('Ctrl Pts',(-7.45843820129782,-70.87825797329,12.));
#131691=CARTESIAN_POINT('Ctrl Pts',(-7.44916203301647,-70.8577105535848,
0.));
#131692=CARTESIAN_POINT('Ctrl Pts',(-7.44916203301647,-70.8577105535848,
12.));
#131693=CARTESIAN_POINT('Ctrl Pts',(-7.43992544738605,-70.8371956702241,
0.));
#131694=CARTESIAN_POINT('Ctrl Pts',(-7.43992544738605,-70.8371956702241,
12.));
#131695=CARTESIAN_POINT('Ctrl Pts',(-7.43072843832014,-70.8167134794737,
0.));
#131696=CARTESIAN_POINT('Ctrl Pts',(-7.43072843832014,-70.8167134794737,
12.));
#131697=CARTESIAN_POINT('Ctrl Pts',(-7.42157099959326,-70.796264138335,
0.));
#131698=CARTESIAN_POINT('Ctrl Pts',(-7.42157099959326,-70.796264138335,
12.));
#131699=CARTESIAN_POINT('Ctrl Pts',(-7.41245312484497,-70.7758478045576,
0.));
#131700=CARTESIAN_POINT('Ctrl Pts',(-7.41245312484497,-70.7758478045576,
12.));
#131701=CARTESIAN_POINT('Ctrl Pts',(-7.40337480758237,-70.7554646366514,
0.));
#131702=CARTESIAN_POINT('Ctrl Pts',(-7.40337480758237,-70.7554646366514,
12.));
#131703=CARTESIAN_POINT('Ctrl Pts',(-7.39433604117891,-70.735114793895,
0.));
#131704=CARTESIAN_POINT('Ctrl Pts',(-7.39433604117891,-70.735114793895,
12.));
#131705=CARTESIAN_POINT('Ctrl Pts',(-7.38533681887027,-70.7147984363423,
0.));
#131706=CARTESIAN_POINT('Ctrl Pts',(-7.38533681887027,-70.7147984363423,
12.));
#131707=CARTESIAN_POINT('Ctrl Pts',(-7.3763771337476,-70.6945157248269,
0.));
#131708=CARTESIAN_POINT('Ctrl Pts',(-7.3763771337476,-70.6945157248269,
12.));
#131709=CARTESIAN_POINT('Ctrl Pts',(-7.36745697876295,-70.6742668209685,
0.));
#131710=CARTESIAN_POINT('Ctrl Pts',(-7.36745697876295,-70.6742668209685,
12.));
#131711=CARTESIAN_POINT('Ctrl Pts',(-7.35857634673051,-70.6540518871772,
0.));
#131712=CARTESIAN_POINT('Ctrl Pts',(-7.35857634673051,-70.6540518871772,
12.));
#131713=CARTESIAN_POINT('Ctrl Pts',(-7.3497352303258,-70.6338710866562,
0.));
#131714=CARTESIAN_POINT('Ctrl Pts',(-7.3497352303258,-70.6338710866562,
12.));
#131715=CARTESIAN_POINT('Ctrl Pts',(-7.34093362208017,-70.6137245834002,
0.));
#131716=CARTESIAN_POINT('Ctrl Pts',(-7.34093362208017,-70.6137245834002,
12.));
#131717=CARTESIAN_POINT('Ctrl Pts',(-7.33217151437608,-70.5936125421958,
0.));
#131718=CARTESIAN_POINT('Ctrl Pts',(-7.33217151437608,-70.5936125421958,
12.));
#131719=CARTESIAN_POINT('Ctrl Pts',(-7.32344889945237,-70.573535128649,
0.));
#131720=CARTESIAN_POINT('Ctrl Pts',(-7.32344889945237,-70.573535128649,
12.));
#131721=CARTESIAN_POINT('Ctrl Pts',(-7.31476576940403,-70.5534925092053,
0.));
#131722=CARTESIAN_POINT('Ctrl Pts',(-7.31476576940403,-70.5534925092053,
12.));
#131723=CARTESIAN_POINT('Ctrl Pts',(-7.30612211618047,-70.5334848511675,
0.));
#131724=CARTESIAN_POINT('Ctrl Pts',(-7.30612211618047,-70.5334848511675,
12.));
#131725=CARTESIAN_POINT('Ctrl Pts',(-7.29751793157801,-70.5135123227147,
0.));
#131726=CARTESIAN_POINT('Ctrl Pts',(-7.29751793157801,-70.5135123227147,
12.));
#131727=CARTESIAN_POINT('Ctrl Pts',(-7.28895320723835,-70.4935750929029,
0.));
#131728=CARTESIAN_POINT('Ctrl Pts',(-7.28895320723835,-70.4935750929029,
12.));
#131729=CARTESIAN_POINT('Ctrl Pts',(-7.28042793465449,-70.4736733316463,
0.));
#131730=CARTESIAN_POINT('Ctrl Pts',(-7.28042793465449,-70.4736733316463,
12.));
#131731=CARTESIAN_POINT('Ctrl Pts',(-7.27194210517057,-70.4538072096986,
0.));
#131732=CARTESIAN_POINT('Ctrl Pts',(-7.27194210517057,-70.4538072096986,
12.));
#131733=CARTESIAN_POINT('Ctrl Pts',(-7.2634957099805,-70.433976898636,0.));
#131734=CARTESIAN_POINT('Ctrl Pts',(-7.2634957099805,-70.433976898636,12.));
#131735=CARTESIAN_POINT('Ctrl Pts',(-7.25508874012075,-70.4141825708207,
0.));
#131736=CARTESIAN_POINT('Ctrl Pts',(-7.25508874012075,-70.4141825708207,
12.));
#131737=CARTESIAN_POINT('Ctrl Pts',(-7.24672118647116,-70.3944243994532,
0.));
#131738=CARTESIAN_POINT('Ctrl Pts',(-7.24672118647116,-70.3944243994532,
12.));
#131739=CARTESIAN_POINT('Ctrl Pts',(-7.23839303975626,-70.3747025586569,
0.));
#131740=CARTESIAN_POINT('Ctrl Pts',(-7.23839303975626,-70.3747025586569,
12.));
#131741=CARTESIAN_POINT('Ctrl Pts',(-7.2301042905423,-70.3550172235486,
0.));
#131742=CARTESIAN_POINT('Ctrl Pts',(-7.2301042905423,-70.3550172235486,
12.));
#131743=CARTESIAN_POINT('Ctrl Pts',(-7.22185492923177,-70.3353685703097,
0.));
#131744=CARTESIAN_POINT('Ctrl Pts',(-7.22185492923177,-70.3353685703097,
12.));
#131745=CARTESIAN_POINT('Ctrl Pts',(-7.21364494605424,-70.3157567762561,
0.));
#131746=CARTESIAN_POINT('Ctrl Pts',(-7.21364494605424,-70.3157567762561,
12.));
#131747=CARTESIAN_POINT('Ctrl Pts',(-7.20547433107457,-70.2961820197051,
0.));
#131748=CARTESIAN_POINT('Ctrl Pts',(-7.20547433107457,-70.2961820197051,
12.));
#131749=CARTESIAN_POINT('Ctrl Pts',(-7.1973430741986,-70.276644479827,0.));
#131750=CARTESIAN_POINT('Ctrl Pts',(-7.1973430741986,-70.276644479827,12.));
#131751=CARTESIAN_POINT('Ctrl Pts',(-7.18925116517562,-70.2571443365198,
0.));
#131752=CARTESIAN_POINT('Ctrl Pts',(-7.18925116517562,-70.2571443365198,
12.));
#131753=CARTESIAN_POINT('Ctrl Pts',(-7.181198593598,-70.2376817702239,0.));
#131754=CARTESIAN_POINT('Ctrl Pts',(-7.181198593598,-70.2376817702239,12.));
#131755=CARTESIAN_POINT('Ctrl Pts',(-7.17318534889747,-70.2182569619028,
0.));
#131756=CARTESIAN_POINT('Ctrl Pts',(-7.17318534889747,-70.2182569619028,
12.));
#131757=CARTESIAN_POINT('Ctrl Pts',(-7.16521142033892,-70.1988700934622,
0.));
#131758=CARTESIAN_POINT('Ctrl Pts',(-7.16521142033892,-70.1988700934622,
12.));
#131759=CARTESIAN_POINT('Ctrl Pts',(-7.15727679700946,-70.1795213481196,
0.));
#131760=CARTESIAN_POINT('Ctrl Pts',(-7.15727679700946,-70.1795213481196,
12.));
#131761=CARTESIAN_POINT('Ctrl Pts',(-7.14938146780801,-70.1602109107188,
0.));
#131762=CARTESIAN_POINT('Ctrl Pts',(-7.14938146780801,-70.1602109107188,
12.));
#131763=CARTESIAN_POINT('Ctrl Pts',(-7.14152542142338,-70.1409389682389,
0.));
#131764=CARTESIAN_POINT('Ctrl Pts',(-7.14152542142338,-70.1409389682389,
12.));
#131765=CARTESIAN_POINT('Ctrl Pts',(-7.13370864634398,-70.1217057094456,
0.));
#131766=CARTESIAN_POINT('Ctrl Pts',(-7.13370864634398,-70.1217057094456,
12.));
#131767=CARTESIAN_POINT('Ctrl Pts',(-7.1259311308887,-70.1025113239463,
0.));
#131768=CARTESIAN_POINT('Ctrl Pts',(-7.1259311308887,-70.1025113239463,
12.));
#131769=CARTESIAN_POINT('Ctrl Pts',(-7.11819286322823,-70.0833560013971,
0.));
#131770=CARTESIAN_POINT('Ctrl Pts',(-7.11819286322823,-70.0833560013971,
12.));
#131771=CARTESIAN_POINT('Ctrl Pts',(-7.11049383140481,-70.06423993069,0.));
#131772=CARTESIAN_POINT('Ctrl Pts',(-7.11049383140481,-70.06423993069,12.));
#131773=CARTESIAN_POINT('Ctrl Pts',(-7.10283402335091,-70.0451632990137,
0.));
#131774=CARTESIAN_POINT('Ctrl Pts',(-7.10283402335091,-70.0451632990137,
12.));
#131775=CARTESIAN_POINT('Ctrl Pts',(-7.09521342684301,-70.0261262936435,
0.));
#131776=CARTESIAN_POINT('Ctrl Pts',(-7.09521342684301,-70.0261262936435,
12.));
#131777=CARTESIAN_POINT('Ctrl Pts',(-7.08763202944274,-70.0071291040791,
0.));
#131778=CARTESIAN_POINT('Ctrl Pts',(-7.08763202944274,-70.0071291040791,
12.));
#131779=CARTESIAN_POINT('Ctrl Pts',(-7.08008981844642,-69.988171923787,
0.));
#131780=CARTESIAN_POINT('Ctrl Pts',(-7.08008981844642,-69.988171923787,
12.));
#131781=CARTESIAN_POINT('Ctrl Pts',(-7.07258678080792,-69.9692549527256,
0.));
#131782=CARTESIAN_POINT('Ctrl Pts',(-7.07258678080792,-69.9692549527256,
12.));
#131783=CARTESIAN_POINT('Ctrl Pts',(-7.06512290312802,-69.9503783975676,
0.));
#131784=CARTESIAN_POINT('Ctrl Pts',(-7.06512290312802,-69.9503783975676,
12.));
#131785=CARTESIAN_POINT('Ctrl Pts',(-7.05769817180824,-69.9315424664252,
0.));
#131786=CARTESIAN_POINT('Ctrl Pts',(-7.05769817180824,-69.9315424664252,
12.));
#131787=CARTESIAN_POINT('Ctrl Pts',(-7.05031257318107,-69.9127473642087,
0.));
#131788=CARTESIAN_POINT('Ctrl Pts',(-7.05031257318107,-69.9127473642087,
12.));
#131789=CARTESIAN_POINT('Ctrl Pts',(-7.04296609362186,-69.8939932885864,
0.));
#131790=CARTESIAN_POINT('Ctrl Pts',(-7.04296609362186,-69.8939932885864,
12.));
#131791=CARTESIAN_POINT('Ctrl Pts',(-7.03565871972265,-69.8752804235296,
0.));
#131792=CARTESIAN_POINT('Ctrl Pts',(-7.03565871972265,-69.8752804235296,
12.));
#131793=CARTESIAN_POINT('Ctrl Pts',(-7.02839043811862,-69.8566089455448,
0.));
#131794=CARTESIAN_POINT('Ctrl Pts',(-7.02839043811862,-69.8566089455448,
12.));
#131795=CARTESIAN_POINT('Ctrl Pts',(-7.02116123514487,-69.8379790360574,
0.));
#131796=CARTESIAN_POINT('Ctrl Pts',(-7.02116123514487,-69.8379790360574,
12.));
#131797=CARTESIAN_POINT('Ctrl Pts',(-7.01397109655455,-69.8193908913722,
0.));
#131798=CARTESIAN_POINT('Ctrl Pts',(-7.01397109655455,-69.8193908913722,
12.));
#131799=CARTESIAN_POINT('Ctrl Pts',(-7.00682000718104,-69.8008447346782,
0.));
#131800=CARTESIAN_POINT('Ctrl Pts',(-7.00682000718104,-69.8008447346782,
12.));
#131801=CARTESIAN_POINT('Ctrl Pts',(-6.99970795069399,-69.7823408242446,
0.));
#131802=CARTESIAN_POINT('Ctrl Pts',(-6.99970795069399,-69.7823408242446,
12.));
#131803=CARTESIAN_POINT('Ctrl Pts',(-6.99263491027859,-69.7638794280263,
0.));
#131804=CARTESIAN_POINT('Ctrl Pts',(-6.99263491027859,-69.7638794280263,
12.));
#131805=CARTESIAN_POINT('Ctrl Pts',(-6.98560086924172,-69.7454607995524,
0.));
#131806=CARTESIAN_POINT('Ctrl Pts',(-6.98560086924172,-69.7454607995524,
12.));
#131807=CARTESIAN_POINT('Ctrl Pts',(-6.97860581164568,-69.7270851557443,
0.));
#131808=CARTESIAN_POINT('Ctrl Pts',(-6.97860581164568,-69.7270851557443,
12.));
#131809=CARTESIAN_POINT('Ctrl Pts',(-6.97164972291581,-69.7087526480249,
0.));
#131810=CARTESIAN_POINT('Ctrl Pts',(-6.97164972291581,-69.7087526480249,
12.));
#131811=CARTESIAN_POINT('Ctrl Pts',(-6.96473259049729,-69.6904633605834,
0.));
#131812=CARTESIAN_POINT('Ctrl Pts',(-6.96473259049729,-69.6904633605834,
12.));
#131813=CARTESIAN_POINT('Ctrl Pts',(-6.95923004173795,-69.6758665380764,
0.));
#131814=CARTESIAN_POINT('Ctrl Pts',(-6.95923004173795,-69.6758665380764,
12.));
#131815=CARTESIAN_POINT('Ctrl Pts',(-6.9551206531773,-69.6649383920075,
0.));
#131816=CARTESIAN_POINT('Ctrl Pts',(-6.9551206531773,-69.6649383920075,
12.));
#131817=CARTESIAN_POINT('Ctrl Pts',(-6.95238884849075,-69.6576616146559,
0.));
#131818=CARTESIAN_POINT('Ctrl Pts',(-6.95238884849075,-69.6576616146559,
12.));
#131819=CARTESIAN_POINT('Ctrl Pts',(-6.95102489306927,-69.6540253893193,
0.));
#131820=CARTESIAN_POINT('Ctrl Pts',(-6.95102489306927,-69.6540253893193,
12.));
#131821=CARTESIAN_POINT('',(-6.95102489306927,-69.6540253893193,12.));
#131822=CARTESIAN_POINT('Ctrl Pts',(-6.95102489306927,-69.6540253893193,
12.));
#131823=CARTESIAN_POINT('Ctrl Pts',(-6.95238884849075,-69.6576616146559,
12.));
#131824=CARTESIAN_POINT('Ctrl Pts',(-6.9551206531773,-69.6649383920075,
12.));
#131825=CARTESIAN_POINT('Ctrl Pts',(-6.95923004173795,-69.6758665380764,
12.));
#131826=CARTESIAN_POINT('Ctrl Pts',(-6.96473259049729,-69.6904633605834,
12.));
#131827=CARTESIAN_POINT('Ctrl Pts',(-6.97164972291581,-69.7087526480249,
12.));
#131828=CARTESIAN_POINT('Ctrl Pts',(-6.97860581164568,-69.7270851557443,
12.));
#131829=CARTESIAN_POINT('Ctrl Pts',(-6.98560086924172,-69.7454607995524,
12.));
#131830=CARTESIAN_POINT('Ctrl Pts',(-6.99263491027859,-69.7638794280263,
12.));
#131831=CARTESIAN_POINT('Ctrl Pts',(-6.99970795069399,-69.7823408242446,
12.));
#131832=CARTESIAN_POINT('Ctrl Pts',(-7.00682000718104,-69.8008447346782,
12.));
#131833=CARTESIAN_POINT('Ctrl Pts',(-7.01397109655455,-69.8193908913722,
12.));
#131834=CARTESIAN_POINT('Ctrl Pts',(-7.02116123514487,-69.8379790360574,
12.));
#131835=CARTESIAN_POINT('Ctrl Pts',(-7.02839043811862,-69.8566089455448,
12.));
#131836=CARTESIAN_POINT('Ctrl Pts',(-7.03565871972265,-69.8752804235296,
12.));
#131837=CARTESIAN_POINT('Ctrl Pts',(-7.04296609362186,-69.8939932885864,
12.));
#131838=CARTESIAN_POINT('Ctrl Pts',(-7.05031257318107,-69.9127473642087,
12.));
#131839=CARTESIAN_POINT('Ctrl Pts',(-7.05769817180824,-69.9315424664252,
12.));
#131840=CARTESIAN_POINT('Ctrl Pts',(-7.06512290312802,-69.9503783975676,
12.));
#131841=CARTESIAN_POINT('Ctrl Pts',(-7.07258678080792,-69.9692549527256,
12.));
#131842=CARTESIAN_POINT('Ctrl Pts',(-7.08008981844642,-69.988171923787,
12.));
#131843=CARTESIAN_POINT('Ctrl Pts',(-7.08763202944274,-70.0071291040791,
12.));
#131844=CARTESIAN_POINT('Ctrl Pts',(-7.09521342684301,-70.0261262936435,
12.));
#131845=CARTESIAN_POINT('Ctrl Pts',(-7.10283402335091,-70.0451632990137,
12.));
#131846=CARTESIAN_POINT('Ctrl Pts',(-7.11049383140481,-70.06423993069,12.));
#131847=CARTESIAN_POINT('Ctrl Pts',(-7.11819286322823,-70.0833560013971,
12.));
#131848=CARTESIAN_POINT('Ctrl Pts',(-7.1259311308887,-70.1025113239463,
12.));
#131849=CARTESIAN_POINT('Ctrl Pts',(-7.13370864634398,-70.1217057094456,
12.));
#131850=CARTESIAN_POINT('Ctrl Pts',(-7.14152542142338,-70.1409389682389,
12.));
#131851=CARTESIAN_POINT('Ctrl Pts',(-7.14938146780801,-70.1602109107188,
12.));
#131852=CARTESIAN_POINT('Ctrl Pts',(-7.15727679700946,-70.1795213481196,
12.));
#131853=CARTESIAN_POINT('Ctrl Pts',(-7.16521142033892,-70.1988700934622,
12.));
#131854=CARTESIAN_POINT('Ctrl Pts',(-7.17318534889747,-70.2182569619028,
12.));
#131855=CARTESIAN_POINT('Ctrl Pts',(-7.181198593598,-70.2376817702239,12.));
#131856=CARTESIAN_POINT('Ctrl Pts',(-7.18925116517562,-70.2571443365198,
12.));
#131857=CARTESIAN_POINT('Ctrl Pts',(-7.1973430741986,-70.276644479827,12.));
#131858=CARTESIAN_POINT('Ctrl Pts',(-7.20547433107457,-70.2961820197051,
12.));
#131859=CARTESIAN_POINT('Ctrl Pts',(-7.21364494605424,-70.3157567762561,
12.));
#131860=CARTESIAN_POINT('Ctrl Pts',(-7.22185492923177,-70.3353685703097,
12.));
#131861=CARTESIAN_POINT('Ctrl Pts',(-7.2301042905423,-70.3550172235486,
12.));
#131862=CARTESIAN_POINT('Ctrl Pts',(-7.23839303975626,-70.3747025586569,
12.));
#131863=CARTESIAN_POINT('Ctrl Pts',(-7.24672118647116,-70.3944243994532,
12.));
#131864=CARTESIAN_POINT('Ctrl Pts',(-7.25508874012075,-70.4141825708207,
12.));
#131865=CARTESIAN_POINT('Ctrl Pts',(-7.2634957099805,-70.433976898636,12.));
#131866=CARTESIAN_POINT('Ctrl Pts',(-7.27194210517057,-70.4538072096986,
12.));
#131867=CARTESIAN_POINT('Ctrl Pts',(-7.28042793465449,-70.4736733316463,
12.));
#131868=CARTESIAN_POINT('Ctrl Pts',(-7.28895320723835,-70.4935750929029,
12.));
#131869=CARTESIAN_POINT('Ctrl Pts',(-7.29751793157801,-70.5135123227147,
12.));
#131870=CARTESIAN_POINT('Ctrl Pts',(-7.30612211618047,-70.5334848511675,
12.));
#131871=CARTESIAN_POINT('Ctrl Pts',(-7.31476576940403,-70.5534925092053,
12.));
#131872=CARTESIAN_POINT('Ctrl Pts',(-7.32344889945237,-70.573535128649,
12.));
#131873=CARTESIAN_POINT('Ctrl Pts',(-7.33217151437608,-70.5936125421958,
12.));
#131874=CARTESIAN_POINT('Ctrl Pts',(-7.34093362208017,-70.6137245834002,
12.));
#131875=CARTESIAN_POINT('Ctrl Pts',(-7.3497352303258,-70.6338710866562,
12.));
#131876=CARTESIAN_POINT('Ctrl Pts',(-7.35857634673051,-70.6540518871772,
12.));
#131877=CARTESIAN_POINT('Ctrl Pts',(-7.36745697876295,-70.6742668209685,
12.));
#131878=CARTESIAN_POINT('Ctrl Pts',(-7.3763771337476,-70.6945157248269,
12.));
#131879=CARTESIAN_POINT('Ctrl Pts',(-7.38533681887027,-70.7147984363423,
12.));
#131880=CARTESIAN_POINT('Ctrl Pts',(-7.39433604117891,-70.735114793895,
12.));
#131881=CARTESIAN_POINT('Ctrl Pts',(-7.40337480758237,-70.7554646366514,
12.));
#131882=CARTESIAN_POINT('Ctrl Pts',(-7.41245312484497,-70.7758478045576,
12.));
#131883=CARTESIAN_POINT('Ctrl Pts',(-7.42157099959326,-70.796264138335,
12.));
#131884=CARTESIAN_POINT('Ctrl Pts',(-7.43072843832014,-70.8167134794737,
12.));
#131885=CARTESIAN_POINT('Ctrl Pts',(-7.43992544738605,-70.8371956702241,
12.));
#131886=CARTESIAN_POINT('Ctrl Pts',(-7.44916203301647,-70.8577105535848,
12.));
#131887=CARTESIAN_POINT('Ctrl Pts',(-7.45843820129782,-70.87825797329,12.));
#131888=CARTESIAN_POINT('Ctrl Pts',(-7.46775395818527,-70.8988377738104,
12.));
#131889=CARTESIAN_POINT('Ctrl Pts',(-7.47710930950562,-70.9194498003493,
12.));
#131890=CARTESIAN_POINT('Ctrl Pts',(-7.48650426095823,-70.940093898837,
12.));
#131891=CARTESIAN_POINT('Ctrl Pts',(-7.4959388181113,-70.9607699159218,
12.));
#131892=CARTESIAN_POINT('Ctrl Pts',(-7.50541298639928,-70.9814776989612,
12.));
#131893=CARTESIAN_POINT('Ctrl Pts',(-7.5149267711309,-71.002217096021,12.));
#131894=CARTESIAN_POINT('Ctrl Pts',(-7.52448017749124,-71.0229879558699,
12.));
#131895=CARTESIAN_POINT('Ctrl Pts',(-7.53407321054262,-71.043790127973,
12.));
#131896=CARTESIAN_POINT('Ctrl Pts',(-7.54370587521979,-71.0646234624811,
12.));
#131897=CARTESIAN_POINT('Ctrl Pts',(-7.55337817632916,-71.0854878102243,
12.));
#131898=CARTESIAN_POINT('Ctrl Pts',(-7.56309011855657,-71.106383022711,
12.));
#131899=CARTESIAN_POINT('Ctrl Pts',(-7.57284170646886,-71.1273089521234,
12.));
#131900=CARTESIAN_POINT('Ctrl Pts',(-7.58263294451451,-71.1482654513119,
12.));
#131901=CARTESIAN_POINT('Ctrl Pts',(-7.59246383701813,-71.1692523737844,
12.));
#131902=CARTESIAN_POINT('Ctrl Pts',(-7.60233438818096,-71.1902695737013,
12.));
#131903=CARTESIAN_POINT('Ctrl Pts',(-7.61224460208837,-71.211316905874,
12.));
#131904=CARTESIAN_POINT('Ctrl Pts',(-7.62219448271109,-71.2323942257609,
12.));
#131905=CARTESIAN_POINT('Ctrl Pts',(-7.63218403390537,-71.2535013894602,
12.));
#131906=CARTESIAN_POINT('Ctrl Pts',(-7.64221325940724,-71.2746382537007,
12.));
#131907=CARTESIAN_POINT('Ctrl Pts',(-7.65228216283403,-71.2958046758372,
12.));
#131908=CARTESIAN_POINT('Ctrl Pts',(-7.66239074769163,-71.3170005138502,
12.));
#131909=CARTESIAN_POINT('Ctrl Pts',(-7.67253901737552,-71.3382256263414,
12.));
#131910=CARTESIAN_POINT('Ctrl Pts',(-7.68272697517086,-71.3594798725281,
12.));
#131911=CARTESIAN_POINT('Ctrl Pts',(-7.69295462424611,-71.3807631122331,
12.));
#131912=CARTESIAN_POINT('Ctrl Pts',(-7.70322196765538,-71.4020752058796,
12.));
#131913=CARTESIAN_POINT('Ctrl Pts',(-7.7135290083452,-71.4234160144925,
12.));
#131914=CARTESIAN_POINT('Ctrl Pts',(-7.72387574915544,-71.4447853996916,
12.));
#131915=CARTESIAN_POINT('Ctrl Pts',(-7.7342621928194,-71.4661832236888,
12.));
#131916=CARTESIAN_POINT('Ctrl Pts',(-7.74468834195746,-71.4876093492781,
12.));
#131917=CARTESIAN_POINT('Ctrl Pts',(-7.75515419907966,-71.5090636398318,
12.));
#131918=CARTESIAN_POINT('Ctrl Pts',(-7.76565976659226,-71.5305459592994,
12.));
#131919=CARTESIAN_POINT('Ctrl Pts',(-7.77620504679869,-71.5520561722039,
12.));
#131920=CARTESIAN_POINT('Ctrl Pts',(-7.78679004189934,-71.5735941436364,
12.));
#131921=CARTESIAN_POINT('Ctrl Pts',(-7.79741475398513,-71.5951597392471,
12.));
#131922=CARTESIAN_POINT('Ctrl Pts',(-7.80807918504021,-71.6167528252423,
12.));
#131923=CARTESIAN_POINT('Ctrl Pts',(-7.8187833369486,-71.6383732683844,
12.));
#131924=CARTESIAN_POINT('Ctrl Pts',(-7.82952721149507,-71.6600209359872,
12.));
#131925=CARTESIAN_POINT('Ctrl Pts',(-7.84031081036489,-71.6816956959117,
12.));
#131926=CARTESIAN_POINT('Ctrl Pts',(-7.85113413513735,-71.7033974165568,
12.));
#131927=CARTESIAN_POINT('Ctrl Pts',(-7.86199718728826,-71.7251259668563,
12.));
#131928=CARTESIAN_POINT('Ctrl Pts',(-7.87289996819653,-71.7468812162788,
12.));
#131929=CARTESIAN_POINT('Ctrl Pts',(-7.88384247914523,-71.7686630348238,
12.));
#131930=CARTESIAN_POINT('Ctrl Pts',(-7.89482472132137,-71.7904712930175,
12.));
#131931=CARTESIAN_POINT('Ctrl Pts',(-7.90584669580955,-71.8123058619042,
12.));
#131932=CARTESIAN_POINT('Ctrl Pts',(-7.91690840359367,-71.8341666130426,
12.));
#131933=CARTESIAN_POINT('Ctrl Pts',(-7.92800984556395,-71.8560534185071,
12.));
#131934=CARTESIAN_POINT('Ctrl Pts',(-7.93915102251794,-71.8779661508832,
12.));
#131935=CARTESIAN_POINT('Ctrl Pts',(-7.9503319351605,-71.8999046832643,
12.));
#131936=CARTESIAN_POINT('Ctrl Pts',(-7.96155258409763,-71.9218688892431,
12.));
#131937=CARTESIAN_POINT('Ctrl Pts',(-7.97281296983717,-71.9438586429081,
12.));
#131938=CARTESIAN_POINT('Ctrl Pts',(-7.98411309279612,-71.965873818843,
12.));
#131939=CARTESIAN_POINT('Ctrl Pts',(-7.99545295330191,-71.9879142921254,
12.));
#131940=CARTESIAN_POINT('Ctrl Pts',(-8.00683255159247,-72.0099799383213,
12.));
#131941=CARTESIAN_POINT('Ctrl Pts',(-8.01825188781056,-72.032070633479,
12.));
#131942=CARTESIAN_POINT('Ctrl Pts',(-8.02971096200307,-72.0541862541243,
12.));
#131943=CARTESIAN_POINT('Ctrl Pts',(-8.04120977412872,-72.0763266772615,
12.));
#131944=CARTESIAN_POINT('Ctrl Pts',(-8.05274832405948,-72.0984917803693,
12.));
#131945=CARTESIAN_POINT('Ctrl Pts',(-8.06432661158095,-72.1206814413988,
12.));
#131946=CARTESIAN_POINT('Ctrl Pts',(-8.07594463638719,-72.1428955387663,
12.));
#131947=CARTESIAN_POINT('Ctrl Pts',(-8.08760239807836,-72.1651339513477,
12.));
#131948=CARTESIAN_POINT('Ctrl Pts',(-8.09929989616889,-72.1873965584813,
12.));
#131949=CARTESIAN_POINT('Ctrl Pts',(-8.11103713008928,-72.209683239963,
12.));
#131950=CARTESIAN_POINT('Ctrl Pts',(-8.1228140991866,-72.2319938760449,
12.));
#131951=CARTESIAN_POINT('Ctrl Pts',(-8.13463080272028,-72.2543283474278,
12.));
#131952=CARTESIAN_POINT('Ctrl Pts',(-8.14648723985797,-72.2766865352555,
12.));
#131953=CARTESIAN_POINT('Ctrl Pts',(-8.15838340968335,-72.2990683211162,
12.));
#131954=CARTESIAN_POINT('Ctrl Pts',(-8.1703193111989,-72.3214735870409,
12.));
#131955=CARTESIAN_POINT('Ctrl Pts',(-8.18229494332623,-72.3439022155007,
12.));
#131956=CARTESIAN_POINT('Ctrl Pts',(-8.19431030490314,-72.3663540894026,
12.));
#131957=CARTESIAN_POINT('Ctrl Pts',(-8.20636539467776,-72.3888290920832,
12.));
#131958=CARTESIAN_POINT('Ctrl Pts',(-8.2184602113156,-72.4113271073079,
12.));
#131959=CARTESIAN_POINT('Ctrl Pts',(-8.23059475340356,-72.4338480192695,
12.));
#131960=CARTESIAN_POINT('Ctrl Pts',(-8.2427690194504,-72.4563917125842,
12.));
#131961=CARTESIAN_POINT('Ctrl Pts',(-8.25498300788493,-72.4789580722875,
12.));
#131962=CARTESIAN_POINT('Ctrl Pts',(-8.26723671704919,-72.5015469838254,
12.));
#131963=CARTESIAN_POINT('Ctrl Pts',(-8.27953014520376,-72.5241583330562,
12.));
#131964=CARTESIAN_POINT('Ctrl Pts',(-8.29186329053279,-72.5467920062521,
12.));
#131965=CARTESIAN_POINT('Ctrl Pts',(-8.30423615114452,-72.5694478900982,
12.));
#131966=CARTESIAN_POINT('Ctrl Pts',(-8.31664872507016,-72.5921258716901,
12.));
#131967=CARTESIAN_POINT('Ctrl Pts',(-8.3291010102567,-72.6148258385296,
12.));
#131968=CARTESIAN_POINT('Ctrl Pts',(-8.34159300456986,-72.6375476785215,
12.));
#131969=CARTESIAN_POINT('Ctrl Pts',(-8.35412470580101,-72.6602912799696,
12.));
#131970=CARTESIAN_POINT('Ctrl Pts',(-8.36669611166842,-72.6830565315703,
12.));
#131971=CARTESIAN_POINT('Ctrl Pts',(-8.37930721981731,-72.705843322407,
12.));
#131972=CARTESIAN_POINT('Ctrl Pts',(-8.3919580278139,-72.7286515419373,
12.));
#131973=CARTESIAN_POINT('Ctrl Pts',(-8.40464853314468,-72.751481079992,
12.));
#131974=CARTESIAN_POINT('Ctrl Pts',(-8.41737873322329,-72.7743318267865,
12.));
#131975=CARTESIAN_POINT('Ctrl Pts',(-8.43014862539157,-72.7972036729276,
12.));
#131976=CARTESIAN_POINT('Ctrl Pts',(-8.44295820691911,-72.8200965094199,
12.));
#131977=CARTESIAN_POINT('Ctrl Pts',(-8.45580747499793,-72.8430102276713,
12.));
#131978=CARTESIAN_POINT('Ctrl Pts',(-8.46869642673794,-72.8659447194933,
12.));
#131979=CARTESIAN_POINT('Ctrl Pts',(-8.48162505917657,-72.8888998770785,
12.));
#131980=CARTESIAN_POINT('Ctrl Pts',(-8.49459336928295,-72.9118755929795,
12.));
#131981=CARTESIAN_POINT('Ctrl Pts',(-8.50760135395983,-72.9348717600838,
12.));
#131982=CARTESIAN_POINT('Ctrl Pts',(-8.52064901004227,-72.9578882715912,
12.));
#131983=CARTESIAN_POINT('Ctrl Pts',(-8.5337363342928,-72.9809250209828,
12.));
#131984=CARTESIAN_POINT('Ctrl Pts',(-8.54686332340417,-73.0039819020648,
12.));
#131985=CARTESIAN_POINT('Ctrl Pts',(-8.56002997400083,-73.0270588090183,
12.));
#131986=CARTESIAN_POINT('Ctrl Pts',(-8.57323628263593,-73.0501556364479,
12.));
#131987=CARTESIAN_POINT('Ctrl Pts',(-8.58648224578731,-73.0732722794195,
12.));
#131988=CARTESIAN_POINT('Ctrl Pts',(-8.59976785984551,-73.0964086335235,
12.));
#131989=CARTESIAN_POINT('Ctrl Pts',(-8.61309312112001,-73.1195645948178,
12.));
#131990=CARTESIAN_POINT('Ctrl Pts',(-8.62645802585483,-73.1427400597037,
12.));
#131991=CARTESIAN_POINT('Ctrl Pts',(-8.63986257023738,-73.1659349248132,
12.));
#131992=CARTESIAN_POINT('Ctrl Pts',(-8.65330675040536,-73.1891490869056,
12.));
#131993=CARTESIAN_POINT('Ctrl Pts',(-8.66679056245091,-73.2123824427208,
12.));
#131994=CARTESIAN_POINT('Ctrl Pts',(-8.68031400241871,-73.2356348889693,
12.));
#131995=CARTESIAN_POINT('Ctrl Pts',(-8.69387706629285,-73.2589063226358,
12.));
#131996=CARTESIAN_POINT('Ctrl Pts',(-8.70747974998229,-73.2821966412148,
12.));
#131997=CARTESIAN_POINT('Ctrl Pts',(-8.72112204930231,-73.3055057429742,
12.));
#131998=CARTESIAN_POINT('Ctrl Pts',(-8.7348039599538,-73.3288335272002,
12.));
#131999=CARTESIAN_POINT('Ctrl Pts',(-8.74852547749778,-73.3521798944622,
12.));
#132000=CARTESIAN_POINT('Ctrl Pts',(-8.76228659740357,-73.3755447460269,
12.));
#132001=CARTESIAN_POINT('Ctrl Pts',(-8.77608731509347,-73.3989279832835,
12.));
#132002=CARTESIAN_POINT('Ctrl Pts',(-8.78992762598756,-73.422329507113,
12.));
#132003=CARTESIAN_POINT('Ctrl Pts',(-8.80380752553691,-73.4457492173933,
12.));
#132004=CARTESIAN_POINT('Ctrl Pts',(-8.8177270092753,-73.4691870121567,
12.));
#132005=CARTESIAN_POINT('Ctrl Pts',(-8.83168607277325,-73.492642788273,
12.));
#132006=CARTESIAN_POINT('Ctrl Pts',(-8.84568471153805,-73.5161164429709,
12.));
#132007=CARTESIAN_POINT('Ctrl Pts',(-8.8597229209213,-73.5396078751639,
12.));
#132008=CARTESIAN_POINT('Ctrl Pts',(-8.8738006960297,-73.5631169867122,
12.));
#132009=CARTESIAN_POINT('Ctrl Pts',(-8.88791803160442,-73.5866436840556,
12.));
#132010=CARTESIAN_POINT('Ctrl Pts',(-8.90207492199043,-73.6101878785976,
12.));
#132011=CARTESIAN_POINT('Ctrl Pts',(-8.91424402151604,-73.630384739363,
12.));
#132012=CARTESIAN_POINT('Ctrl Pts',(-8.92359518178502,-73.6458786306025,
12.));
#132013=CARTESIAN_POINT('Ctrl Pts',(-8.93011088817333,-73.6566618622077,
12.));
#132014=CARTESIAN_POINT('Ctrl Pts',(-8.93377955965658,-73.6627293782592,
12.));
#132015=CARTESIAN_POINT('Ctrl Pts',(-8.93459554657871,-73.6640787198061,
12.));
#132016=CARTESIAN_POINT('',(-6.95102489306927,-69.6540253893193,0.));
#132017=CARTESIAN_POINT('',(-6.95102489306927,-69.6540253893193,0.));
#132018=CARTESIAN_POINT('Ctrl Pts',(-8.93459554657871,-73.6640787198061,
0.));
#132019=CARTESIAN_POINT('Ctrl Pts',(-8.93377955965658,-73.6627293782592,
0.));
#132020=CARTESIAN_POINT('Ctrl Pts',(-8.93011088817333,-73.6566618622077,
0.));
#132021=CARTESIAN_POINT('Ctrl Pts',(-8.92359518178502,-73.6458786306025,
0.));
#132022=CARTESIAN_POINT('Ctrl Pts',(-8.91424402151604,-73.630384739363,
0.));
#132023=CARTESIAN_POINT('Ctrl Pts',(-8.90207492199043,-73.6101878785976,
0.));
#132024=CARTESIAN_POINT('Ctrl Pts',(-8.88791803160442,-73.5866436840556,
0.));
#132025=CARTESIAN_POINT('Ctrl Pts',(-8.8738006960297,-73.5631169867122,
0.));
#132026=CARTESIAN_POINT('Ctrl Pts',(-8.8597229209213,-73.5396078751639,
0.));
#132027=CARTESIAN_POINT('Ctrl Pts',(-8.84568471153805,-73.5161164429709,
0.));
#132028=CARTESIAN_POINT('Ctrl Pts',(-8.83168607277325,-73.492642788273,
0.));
#132029=CARTESIAN_POINT('Ctrl Pts',(-8.8177270092753,-73.4691870121567,
0.));
#132030=CARTESIAN_POINT('Ctrl Pts',(-8.80380752553691,-73.4457492173933,
0.));
#132031=CARTESIAN_POINT('Ctrl Pts',(-8.78992762598756,-73.422329507113,
0.));
#132032=CARTESIAN_POINT('Ctrl Pts',(-8.77608731509347,-73.3989279832835,
0.));
#132033=CARTESIAN_POINT('Ctrl Pts',(-8.76228659740357,-73.3755447460269,
0.));
#132034=CARTESIAN_POINT('Ctrl Pts',(-8.74852547749778,-73.3521798944622,
0.));
#132035=CARTESIAN_POINT('Ctrl Pts',(-8.7348039599538,-73.3288335272002,
0.));
#132036=CARTESIAN_POINT('Ctrl Pts',(-8.72112204930231,-73.3055057429742,
0.));
#132037=CARTESIAN_POINT('Ctrl Pts',(-8.70747974998229,-73.2821966412148,
0.));
#132038=CARTESIAN_POINT('Ctrl Pts',(-8.69387706629285,-73.2589063226358,
0.));
#132039=CARTESIAN_POINT('Ctrl Pts',(-8.68031400241871,-73.2356348889693,
0.));
#132040=CARTESIAN_POINT('Ctrl Pts',(-8.66679056245091,-73.2123824427208,
0.));
#132041=CARTESIAN_POINT('Ctrl Pts',(-8.65330675040536,-73.1891490869056,
0.));
#132042=CARTESIAN_POINT('Ctrl Pts',(-8.63986257023738,-73.1659349248132,
0.));
#132043=CARTESIAN_POINT('Ctrl Pts',(-8.62645802585483,-73.1427400597037,
0.));
#132044=CARTESIAN_POINT('Ctrl Pts',(-8.61309312112001,-73.1195645948178,
0.));
#132045=CARTESIAN_POINT('Ctrl Pts',(-8.59976785984551,-73.0964086335235,
0.));
#132046=CARTESIAN_POINT('Ctrl Pts',(-8.58648224578731,-73.0732722794195,
0.));
#132047=CARTESIAN_POINT('Ctrl Pts',(-8.57323628263593,-73.0501556364479,
0.));
#132048=CARTESIAN_POINT('Ctrl Pts',(-8.56002997400083,-73.0270588090183,
0.));
#132049=CARTESIAN_POINT('Ctrl Pts',(-8.54686332340417,-73.0039819020648,
0.));
#132050=CARTESIAN_POINT('Ctrl Pts',(-8.5337363342928,-72.9809250209828,
0.));
#132051=CARTESIAN_POINT('Ctrl Pts',(-8.52064901004227,-72.9578882715912,
0.));
#132052=CARTESIAN_POINT('Ctrl Pts',(-8.50760135395983,-72.9348717600838,
0.));
#132053=CARTESIAN_POINT('Ctrl Pts',(-8.49459336928295,-72.9118755929795,
0.));
#132054=CARTESIAN_POINT('Ctrl Pts',(-8.48162505917657,-72.8888998770785,
0.));
#132055=CARTESIAN_POINT('Ctrl Pts',(-8.46869642673794,-72.8659447194933,
0.));
#132056=CARTESIAN_POINT('Ctrl Pts',(-8.45580747499793,-72.8430102276713,
0.));
#132057=CARTESIAN_POINT('Ctrl Pts',(-8.44295820691911,-72.8200965094199,
0.));
#132058=CARTESIAN_POINT('Ctrl Pts',(-8.43014862539157,-72.7972036729276,
0.));
#132059=CARTESIAN_POINT('Ctrl Pts',(-8.41737873322329,-72.7743318267865,
0.));
#132060=CARTESIAN_POINT('Ctrl Pts',(-8.40464853314468,-72.751481079992,
0.));
#132061=CARTESIAN_POINT('Ctrl Pts',(-8.3919580278139,-72.7286515419373,
0.));
#132062=CARTESIAN_POINT('Ctrl Pts',(-8.37930721981731,-72.705843322407,
0.));
#132063=CARTESIAN_POINT('Ctrl Pts',(-8.36669611166842,-72.6830565315703,
0.));
#132064=CARTESIAN_POINT('Ctrl Pts',(-8.35412470580101,-72.6602912799696,
0.));
#132065=CARTESIAN_POINT('Ctrl Pts',(-8.34159300456986,-72.6375476785215,
0.));
#132066=CARTESIAN_POINT('Ctrl Pts',(-8.3291010102567,-72.6148258385296,
0.));
#132067=CARTESIAN_POINT('Ctrl Pts',(-8.31664872507016,-72.5921258716901,
0.));
#132068=CARTESIAN_POINT('Ctrl Pts',(-8.30423615114452,-72.5694478900982,
0.));
#132069=CARTESIAN_POINT('Ctrl Pts',(-8.29186329053279,-72.5467920062521,
0.));
#132070=CARTESIAN_POINT('Ctrl Pts',(-8.27953014520376,-72.5241583330562,
0.));
#132071=CARTESIAN_POINT('Ctrl Pts',(-8.26723671704919,-72.5015469838254,
0.));
#132072=CARTESIAN_POINT('Ctrl Pts',(-8.25498300788493,-72.4789580722875,
0.));
#132073=CARTESIAN_POINT('Ctrl Pts',(-8.2427690194504,-72.4563917125842,
0.));
#132074=CARTESIAN_POINT('Ctrl Pts',(-8.23059475340356,-72.4338480192695,
0.));
#132075=CARTESIAN_POINT('Ctrl Pts',(-8.2184602113156,-72.4113271073079,
0.));
#132076=CARTESIAN_POINT('Ctrl Pts',(-8.20636539467776,-72.3888290920832,
0.));
#132077=CARTESIAN_POINT('Ctrl Pts',(-8.19431030490314,-72.3663540894026,
0.));
#132078=CARTESIAN_POINT('Ctrl Pts',(-8.18229494332623,-72.3439022155007,
0.));
#132079=CARTESIAN_POINT('Ctrl Pts',(-8.1703193111989,-72.3214735870409,
0.));
#132080=CARTESIAN_POINT('Ctrl Pts',(-8.15838340968335,-72.2990683211162,
0.));
#132081=CARTESIAN_POINT('Ctrl Pts',(-8.14648723985797,-72.2766865352555,
0.));
#132082=CARTESIAN_POINT('Ctrl Pts',(-8.13463080272028,-72.2543283474278,
0.));
#132083=CARTESIAN_POINT('Ctrl Pts',(-8.1228140991866,-72.2319938760449,
0.));
#132084=CARTESIAN_POINT('Ctrl Pts',(-8.11103713008928,-72.209683239963,
0.));
#132085=CARTESIAN_POINT('Ctrl Pts',(-8.09929989616889,-72.1873965584813,
0.));
#132086=CARTESIAN_POINT('Ctrl Pts',(-8.08760239807836,-72.1651339513477,
0.));
#132087=CARTESIAN_POINT('Ctrl Pts',(-8.07594463638719,-72.1428955387663,
0.));
#132088=CARTESIAN_POINT('Ctrl Pts',(-8.06432661158095,-72.1206814413988,
0.));
#132089=CARTESIAN_POINT('Ctrl Pts',(-8.05274832405948,-72.0984917803693,
0.));
#132090=CARTESIAN_POINT('Ctrl Pts',(-8.04120977412872,-72.0763266772615,
0.));
#132091=CARTESIAN_POINT('Ctrl Pts',(-8.02971096200307,-72.0541862541243,
0.));
#132092=CARTESIAN_POINT('Ctrl Pts',(-8.01825188781056,-72.032070633479,
0.));
#132093=CARTESIAN_POINT('Ctrl Pts',(-8.00683255159247,-72.0099799383213,
0.));
#132094=CARTESIAN_POINT('Ctrl Pts',(-7.99545295330191,-71.9879142921254,
0.));
#132095=CARTESIAN_POINT('Ctrl Pts',(-7.98411309279612,-71.965873818843,
0.));
#132096=CARTESIAN_POINT('Ctrl Pts',(-7.97281296983717,-71.9438586429081,
0.));
#132097=CARTESIAN_POINT('Ctrl Pts',(-7.96155258409763,-71.9218688892431,
0.));
#132098=CARTESIAN_POINT('Ctrl Pts',(-7.9503319351605,-71.8999046832643,
0.));
#132099=CARTESIAN_POINT('Ctrl Pts',(-7.93915102251794,-71.8779661508832,
0.));
#132100=CARTESIAN_POINT('Ctrl Pts',(-7.92800984556395,-71.8560534185071,
0.));
#132101=CARTESIAN_POINT('Ctrl Pts',(-7.91690840359367,-71.8341666130426,
0.));
#132102=CARTESIAN_POINT('Ctrl Pts',(-7.90584669580955,-71.8123058619042,
0.));
#132103=CARTESIAN_POINT('Ctrl Pts',(-7.89482472132137,-71.7904712930175,
0.));
#132104=CARTESIAN_POINT('Ctrl Pts',(-7.88384247914523,-71.7686630348238,
0.));
#132105=CARTESIAN_POINT('Ctrl Pts',(-7.87289996819653,-71.7468812162788,
0.));
#132106=CARTESIAN_POINT('Ctrl Pts',(-7.86199718728826,-71.7251259668563,
0.));
#132107=CARTESIAN_POINT('Ctrl Pts',(-7.85113413513735,-71.7033974165568,
0.));
#132108=CARTESIAN_POINT('Ctrl Pts',(-7.84031081036489,-71.6816956959117,
0.));
#132109=CARTESIAN_POINT('Ctrl Pts',(-7.82952721149507,-71.6600209359872,
0.));
#132110=CARTESIAN_POINT('Ctrl Pts',(-7.8187833369486,-71.6383732683844,
0.));
#132111=CARTESIAN_POINT('Ctrl Pts',(-7.80807918504021,-71.6167528252423,
0.));
#132112=CARTESIAN_POINT('Ctrl Pts',(-7.79741475398513,-71.5951597392471,
0.));
#132113=CARTESIAN_POINT('Ctrl Pts',(-7.78679004189934,-71.5735941436364,
0.));
#132114=CARTESIAN_POINT('Ctrl Pts',(-7.77620504679869,-71.5520561722039,
0.));
#132115=CARTESIAN_POINT('Ctrl Pts',(-7.76565976659226,-71.5305459592994,
0.));
#132116=CARTESIAN_POINT('Ctrl Pts',(-7.75515419907966,-71.5090636398318,
0.));
#132117=CARTESIAN_POINT('Ctrl Pts',(-7.74468834195746,-71.4876093492781,
0.));
#132118=CARTESIAN_POINT('Ctrl Pts',(-7.7342621928194,-71.4661832236888,
0.));
#132119=CARTESIAN_POINT('Ctrl Pts',(-7.72387574915544,-71.4447853996916,
0.));
#132120=CARTESIAN_POINT('Ctrl Pts',(-7.7135290083452,-71.4234160144925,
0.));
#132121=CARTESIAN_POINT('Ctrl Pts',(-7.70322196765538,-71.4020752058796,
0.));
#132122=CARTESIAN_POINT('Ctrl Pts',(-7.69295462424611,-71.3807631122331,
0.));
#132123=CARTESIAN_POINT('Ctrl Pts',(-7.68272697517086,-71.3594798725281,
0.));
#132124=CARTESIAN_POINT('Ctrl Pts',(-7.67253901737552,-71.3382256263414,
0.));
#132125=CARTESIAN_POINT('Ctrl Pts',(-7.66239074769163,-71.3170005138502,
0.));
#132126=CARTESIAN_POINT('Ctrl Pts',(-7.65228216283403,-71.2958046758372,
0.));
#132127=CARTESIAN_POINT('Ctrl Pts',(-7.64221325940724,-71.2746382537007,
0.));
#132128=CARTESIAN_POINT('Ctrl Pts',(-7.63218403390537,-71.2535013894602,
0.));
#132129=CARTESIAN_POINT('Ctrl Pts',(-7.62219448271109,-71.2323942257609,
0.));
#132130=CARTESIAN_POINT('Ctrl Pts',(-7.61224460208837,-71.211316905874,
0.));
#132131=CARTESIAN_POINT('Ctrl Pts',(-7.60233438818096,-71.1902695737013,
0.));
#132132=CARTESIAN_POINT('Ctrl Pts',(-7.59246383701813,-71.1692523737844,
0.));
#132133=CARTESIAN_POINT('Ctrl Pts',(-7.58263294451451,-71.1482654513119,
0.));
#132134=CARTESIAN_POINT('Ctrl Pts',(-7.57284170646886,-71.1273089521234,
0.));
#132135=CARTESIAN_POINT('Ctrl Pts',(-7.56309011855657,-71.106383022711,
0.));
#132136=CARTESIAN_POINT('Ctrl Pts',(-7.55337817632916,-71.0854878102243,
0.));
#132137=CARTESIAN_POINT('Ctrl Pts',(-7.54370587521979,-71.0646234624811,
0.));
#132138=CARTESIAN_POINT('Ctrl Pts',(-7.53407321054262,-71.043790127973,
0.));
#132139=CARTESIAN_POINT('Ctrl Pts',(-7.52448017749124,-71.0229879558699,
0.));
#132140=CARTESIAN_POINT('Ctrl Pts',(-7.5149267711309,-71.002217096021,0.));
#132141=CARTESIAN_POINT('Ctrl Pts',(-7.50541298639928,-70.9814776989612,
0.));
#132142=CARTESIAN_POINT('Ctrl Pts',(-7.4959388181113,-70.9607699159218,
0.));
#132143=CARTESIAN_POINT('Ctrl Pts',(-7.48650426095823,-70.940093898837,
0.));
#132144=CARTESIAN_POINT('Ctrl Pts',(-7.47710930950562,-70.9194498003493,
0.));
#132145=CARTESIAN_POINT('Ctrl Pts',(-7.46775395818527,-70.8988377738104,
0.));
#132146=CARTESIAN_POINT('Ctrl Pts',(-7.45843820129782,-70.87825797329,0.));
#132147=CARTESIAN_POINT('Ctrl Pts',(-7.44916203301647,-70.8577105535848,
0.));
#132148=CARTESIAN_POINT('Ctrl Pts',(-7.43992544738605,-70.8371956702241,
0.));
#132149=CARTESIAN_POINT('Ctrl Pts',(-7.43072843832014,-70.8167134794737,
0.));
#132150=CARTESIAN_POINT('Ctrl Pts',(-7.42157099959326,-70.796264138335,
0.));
#132151=CARTESIAN_POINT('Ctrl Pts',(-7.41245312484497,-70.7758478045576,
0.));
#132152=CARTESIAN_POINT('Ctrl Pts',(-7.40337480758237,-70.7554646366514,
0.));
#132153=CARTESIAN_POINT('Ctrl Pts',(-7.39433604117891,-70.735114793895,
0.));
#132154=CARTESIAN_POINT('Ctrl Pts',(-7.38533681887027,-70.7147984363423,
0.));
#132155=CARTESIAN_POINT('Ctrl Pts',(-7.3763771337476,-70.6945157248269,
0.));
#132156=CARTESIAN_POINT('Ctrl Pts',(-7.36745697876295,-70.6742668209685,
0.));
#132157=CARTESIAN_POINT('Ctrl Pts',(-7.35857634673051,-70.6540518871772,
0.));
#132158=CARTESIAN_POINT('Ctrl Pts',(-7.3497352303258,-70.6338710866562,
0.));
#132159=CARTESIAN_POINT('Ctrl Pts',(-7.34093362208017,-70.6137245834002,
0.));
#132160=CARTESIAN_POINT('Ctrl Pts',(-7.33217151437608,-70.5936125421958,
0.));
#132161=CARTESIAN_POINT('Ctrl Pts',(-7.32344889945237,-70.573535128649,
0.));
#132162=CARTESIAN_POINT('Ctrl Pts',(-7.31476576940403,-70.5534925092053,
0.));
#132163=CARTESIAN_POINT('Ctrl Pts',(-7.30612211618047,-70.5334848511675,
0.));
#132164=CARTESIAN_POINT('Ctrl Pts',(-7.29751793157801,-70.5135123227147,
0.));
#132165=CARTESIAN_POINT('Ctrl Pts',(-7.28895320723835,-70.4935750929029,
0.));
#132166=CARTESIAN_POINT('Ctrl Pts',(-7.28042793465449,-70.4736733316463,
0.));
#132167=CARTESIAN_POINT('Ctrl Pts',(-7.27194210517057,-70.4538072096986,
0.));
#132168=CARTESIAN_POINT('Ctrl Pts',(-7.2634957099805,-70.433976898636,0.));
#132169=CARTESIAN_POINT('Ctrl Pts',(-7.25508874012075,-70.4141825708207,
0.));
#132170=CARTESIAN_POINT('Ctrl Pts',(-7.24672118647116,-70.3944243994532,
0.));
#132171=CARTESIAN_POINT('Ctrl Pts',(-7.23839303975626,-70.3747025586569,
0.));
#132172=CARTESIAN_POINT('Ctrl Pts',(-7.2301042905423,-70.3550172235486,
0.));
#132173=CARTESIAN_POINT('Ctrl Pts',(-7.22185492923177,-70.3353685703097,
0.));
#132174=CARTESIAN_POINT('Ctrl Pts',(-7.21364494605424,-70.3157567762561,
0.));
#132175=CARTESIAN_POINT('Ctrl Pts',(-7.20547433107457,-70.2961820197051,
0.));
#132176=CARTESIAN_POINT('Ctrl Pts',(-7.1973430741986,-70.276644479827,0.));
#132177=CARTESIAN_POINT('Ctrl Pts',(-7.18925116517562,-70.2571443365198,
0.));
#132178=CARTESIAN_POINT('Ctrl Pts',(-7.181198593598,-70.2376817702239,0.));
#132179=CARTESIAN_POINT('Ctrl Pts',(-7.17318534889747,-70.2182569619028,
0.));
#132180=CARTESIAN_POINT('Ctrl Pts',(-7.16521142033892,-70.1988700934622,
0.));
#132181=CARTESIAN_POINT('Ctrl Pts',(-7.15727679700946,-70.1795213481196,
0.));
#132182=CARTESIAN_POINT('Ctrl Pts',(-7.14938146780801,-70.1602109107188,
0.));
#132183=CARTESIAN_POINT('Ctrl Pts',(-7.14152542142338,-70.1409389682389,
0.));
#132184=CARTESIAN_POINT('Ctrl Pts',(-7.13370864634398,-70.1217057094456,
0.));
#132185=CARTESIAN_POINT('Ctrl Pts',(-7.1259311308887,-70.1025113239463,
0.));
#132186=CARTESIAN_POINT('Ctrl Pts',(-7.11819286322823,-70.0833560013971,
0.));
#132187=CARTESIAN_POINT('Ctrl Pts',(-7.11049383140481,-70.06423993069,0.));
#132188=CARTESIAN_POINT('Ctrl Pts',(-7.10283402335091,-70.0451632990137,
0.));
#132189=CARTESIAN_POINT('Ctrl Pts',(-7.09521342684301,-70.0261262936435,
0.));
#132190=CARTESIAN_POINT('Ctrl Pts',(-7.08763202944274,-70.0071291040791,
0.));
#132191=CARTESIAN_POINT('Ctrl Pts',(-7.08008981844642,-69.988171923787,
0.));
#132192=CARTESIAN_POINT('Ctrl Pts',(-7.07258678080792,-69.9692549527256,
0.));
#132193=CARTESIAN_POINT('Ctrl Pts',(-7.06512290312802,-69.9503783975676,
0.));
#132194=CARTESIAN_POINT('Ctrl Pts',(-7.05769817180824,-69.9315424664252,
0.));
#132195=CARTESIAN_POINT('Ctrl Pts',(-7.05031257318107,-69.9127473642087,
0.));
#132196=CARTESIAN_POINT('Ctrl Pts',(-7.04296609362186,-69.8939932885864,
0.));
#132197=CARTESIAN_POINT('Ctrl Pts',(-7.03565871972265,-69.8752804235296,
0.));
#132198=CARTESIAN_POINT('Ctrl Pts',(-7.02839043811862,-69.8566089455448,
0.));
#132199=CARTESIAN_POINT('Ctrl Pts',(-7.02116123514487,-69.8379790360574,
0.));
#132200=CARTESIAN_POINT('Ctrl Pts',(-7.01397109655455,-69.8193908913722,
0.));
#132201=CARTESIAN_POINT('Ctrl Pts',(-7.00682000718104,-69.8008447346782,
0.));
#132202=CARTESIAN_POINT('Ctrl Pts',(-6.99970795069399,-69.7823408242446,
0.));
#132203=CARTESIAN_POINT('Ctrl Pts',(-6.99263491027859,-69.7638794280263,
0.));
#132204=CARTESIAN_POINT('Ctrl Pts',(-6.98560086924172,-69.7454607995524,
0.));
#132205=CARTESIAN_POINT('Ctrl Pts',(-6.97860581164568,-69.7270851557443,
0.));
#132206=CARTESIAN_POINT('Ctrl Pts',(-6.97164972291581,-69.7087526480249,
0.));
#132207=CARTESIAN_POINT('Ctrl Pts',(-6.96473259049729,-69.6904633605834,
0.));
#132208=CARTESIAN_POINT('Ctrl Pts',(-6.95923004173795,-69.6758665380764,
0.));
#132209=CARTESIAN_POINT('Ctrl Pts',(-6.9551206531773,-69.6649383920075,
0.));
#132210=CARTESIAN_POINT('Ctrl Pts',(-6.95238884849075,-69.6576616146559,
0.));
#132211=CARTESIAN_POINT('Ctrl Pts',(-6.95102489306927,-69.6540253893193,
0.));
#132212=CARTESIAN_POINT('Ctrl Pts',(-15.5142209845168,-72.8667204369977,
0.));
#132213=CARTESIAN_POINT('Ctrl Pts',(-15.5142209845168,-72.8667204369977,
12.));
#132214=CARTESIAN_POINT('Ctrl Pts',(-15.5108715869174,-72.8622377860957,
0.));
#132215=CARTESIAN_POINT('Ctrl Pts',(-15.5108715869174,-72.8622377860957,
12.));
#132216=CARTESIAN_POINT('Ctrl Pts',(-15.5041768664089,-72.8532737732124,
0.));
#132217=CARTESIAN_POINT('Ctrl Pts',(-15.5041768664089,-72.8532737732124,
12.));
#132218=CARTESIAN_POINT('Ctrl Pts',(-15.494147009717,-72.8398316206501,
0.));
#132219=CARTESIAN_POINT('Ctrl Pts',(-15.494147009717,-72.8398316206501,
12.));
#132220=CARTESIAN_POINT('Ctrl Pts',(-15.4807983165983,-72.8219164844002,
0.));
#132221=CARTESIAN_POINT('Ctrl Pts',(-15.4807983165983,-72.8219164844002,
12.));
#132222=CARTESIAN_POINT('Ctrl Pts',(-15.4641532053435,-72.7995354604414,
0.));
#132223=CARTESIAN_POINT('Ctrl Pts',(-15.4641532053435,-72.7995354604414,
12.));
#132224=CARTESIAN_POINT('Ctrl Pts',(-15.4475488590336,-72.7771673494582,
0.));
#132225=CARTESIAN_POINT('Ctrl Pts',(-15.4475488590336,-72.7771673494582,
12.));
#132226=CARTESIAN_POINT('Ctrl Pts',(-15.4309852897866,-72.7548121825431,
0.));
#132227=CARTESIAN_POINT('Ctrl Pts',(-15.4309852897866,-72.7548121825431,
12.));
#132228=CARTESIAN_POINT('Ctrl Pts',(-15.4144625111911,-72.7324700089576,
0.));
#132229=CARTESIAN_POINT('Ctrl Pts',(-15.4144625111911,-72.7324700089576,
12.));
#132230=CARTESIAN_POINT('Ctrl Pts',(-15.397980537311,-72.710140901746,0.));
#132231=CARTESIAN_POINT('Ctrl Pts',(-15.397980537311,-72.710140901746,12.));
#132232=CARTESIAN_POINT('Ctrl Pts',(-15.3815393822669,-72.6878249557452,
0.));
#132233=CARTESIAN_POINT('Ctrl Pts',(-15.3815393822669,-72.6878249557452,
12.));
#132234=CARTESIAN_POINT('Ctrl Pts',(-15.3651390602616,-72.6655222797603,
0.));
#132235=CARTESIAN_POINT('Ctrl Pts',(-15.3651390602616,-72.6655222797603,
12.));
#132236=CARTESIAN_POINT('Ctrl Pts',(-15.3487795854723,-72.6432329903466,
0.));
#132237=CARTESIAN_POINT('Ctrl Pts',(-15.3487795854723,-72.6432329903466,
12.));
#132238=CARTESIAN_POINT('Ctrl Pts',(-15.3324609719961,-72.6209572051064,
0.));
#132239=CARTESIAN_POINT('Ctrl Pts',(-15.3324609719961,-72.6209572051064,
12.));
#132240=CARTESIAN_POINT('Ctrl Pts',(-15.3161832337617,-72.5986950357771,
0.));
#132241=CARTESIAN_POINT('Ctrl Pts',(-15.3161832337617,-72.5986950357771,
12.));
#132242=CARTESIAN_POINT('Ctrl Pts',(-15.2999463844691,-72.5764465826345,
0.));
#132243=CARTESIAN_POINT('Ctrl Pts',(-15.2999463844691,-72.5764465826345,
12.));
#132244=CARTESIAN_POINT('Ctrl Pts',(-15.2837504376562,-72.5542119383748,
0.));
#132245=CARTESIAN_POINT('Ctrl Pts',(-15.2837504376562,-72.5542119383748,
12.));
#132246=CARTESIAN_POINT('Ctrl Pts',(-15.2675954067495,-72.5319911908978,
0.));
#132247=CARTESIAN_POINT('Ctrl Pts',(-15.2675954067495,-72.5319911908978,
12.));
#132248=CARTESIAN_POINT('Ctrl Pts',(-15.2514813051174,-72.5097844266083,
0.));
#132249=CARTESIAN_POINT('Ctrl Pts',(-15.2514813051174,-72.5097844266083,
12.));
#132250=CARTESIAN_POINT('Ctrl Pts',(-15.2354081461151,-72.4875917332729,
0.));
#132251=CARTESIAN_POINT('Ctrl Pts',(-15.2354081461151,-72.4875917332729,
12.));
#132252=CARTESIAN_POINT('Ctrl Pts',(-15.2193759431359,-72.4654132036373,
0.));
#132253=CARTESIAN_POINT('Ctrl Pts',(-15.2193759431359,-72.4654132036373,
12.));
#132254=CARTESIAN_POINT('Ctrl Pts',(-15.2033847096077,-72.4432489350415,
0.));
#132255=CARTESIAN_POINT('Ctrl Pts',(-15.2033847096077,-72.4432489350415,
12.));
#132256=CARTESIAN_POINT('Ctrl Pts',(-15.1874344589715,-72.4210990277819,
0.));
#132257=CARTESIAN_POINT('Ctrl Pts',(-15.1874344589715,-72.4210990277819,
12.));
#132258=CARTESIAN_POINT('Ctrl Pts',(-15.1715252046602,-72.3989635838476,
0.));
#132259=CARTESIAN_POINT('Ctrl Pts',(-15.1715252046602,-72.3989635838476,
12.));
#132260=CARTESIAN_POINT('Ctrl Pts',(-15.1556569600747,-72.37684270559,0.));
#132261=CARTESIAN_POINT('Ctrl Pts',(-15.1556569600747,-72.37684270559,12.));
#132262=CARTESIAN_POINT('Ctrl Pts',(-15.1398297385513,-72.3547364941996,
0.));
#132263=CARTESIAN_POINT('Ctrl Pts',(-15.1398297385513,-72.3547364941996,
12.));
#132264=CARTESIAN_POINT('Ctrl Pts',(-15.1240435533478,-72.332645049021,
0.));
#132265=CARTESIAN_POINT('Ctrl Pts',(-15.1240435533478,-72.332645049021,
12.));
#132266=CARTESIAN_POINT('Ctrl Pts',(-15.1082984176655,-72.3105684683971,
0.));
#132267=CARTESIAN_POINT('Ctrl Pts',(-15.1082984176655,-72.3105684683971,
12.));
#132268=CARTESIAN_POINT('Ctrl Pts',(-15.0925943446593,-72.2885068501641,
0.));
#132269=CARTESIAN_POINT('Ctrl Pts',(-15.0925943446593,-72.2885068501641,
12.));
#132270=CARTESIAN_POINT('Ctrl Pts',(-15.0769313474476,-72.266460292285,
0.));
#132271=CARTESIAN_POINT('Ctrl Pts',(-15.0769313474476,-72.266460292285,
12.));
#132272=CARTESIAN_POINT('Ctrl Pts',(-15.0613094391186,-72.244428893425,
0.));
#132273=CARTESIAN_POINT('Ctrl Pts',(-15.0613094391186,-72.244428893425,
12.));
#132274=CARTESIAN_POINT('Ctrl Pts',(-15.0457286327328,-72.2224127535401,
0.));
#132275=CARTESIAN_POINT('Ctrl Pts',(-15.0457286327328,-72.2224127535401,
12.));
#132276=CARTESIAN_POINT('Ctrl Pts',(-15.0301889413255,-72.2004119736104,
0.));
#132277=CARTESIAN_POINT('Ctrl Pts',(-15.0301889413255,-72.2004119736104,
12.));
#132278=CARTESIAN_POINT('Ctrl Pts',(-15.0146903779061,-72.1784266553948,
0.));
#132279=CARTESIAN_POINT('Ctrl Pts',(-15.0146903779061,-72.1784266553948,
12.));
#132280=CARTESIAN_POINT('Ctrl Pts',(-14.9992329554537,-72.1564569011668,
0.));
#132281=CARTESIAN_POINT('Ctrl Pts',(-14.9992329554537,-72.1564569011668,
12.));
#132282=CARTESIAN_POINT('Ctrl Pts',(-14.9838166869107,-72.1345028134779,
0.));
#132283=CARTESIAN_POINT('Ctrl Pts',(-14.9838166869107,-72.1345028134779,
12.));
#132284=CARTESIAN_POINT('Ctrl Pts',(-14.9684415851699,-72.1125644948547,
0.));
#132285=CARTESIAN_POINT('Ctrl Pts',(-14.9684415851699,-72.1125644948547,
12.));
#132286=CARTESIAN_POINT('Ctrl Pts',(-14.953107663077,-72.0906420478085,
0.));
#132287=CARTESIAN_POINT('Ctrl Pts',(-14.953107663077,-72.0906420478085,
12.));
#132288=CARTESIAN_POINT('Ctrl Pts',(-14.937814933439,-72.0687355749815,
0.));
#132289=CARTESIAN_POINT('Ctrl Pts',(-14.937814933439,-72.0687355749815,
12.));
#132290=CARTESIAN_POINT('Ctrl Pts',(-14.9225634090269,-72.046845179251,
0.));
#132291=CARTESIAN_POINT('Ctrl Pts',(-14.9225634090269,-72.046845179251,
12.));
#132292=CARTESIAN_POINT('Ctrl Pts',(-14.9073531025763,-72.0249709638419,
0.));
#132293=CARTESIAN_POINT('Ctrl Pts',(-14.9073531025763,-72.0249709638419,
12.));
#132294=CARTESIAN_POINT('Ctrl Pts',(-14.8921840267829,-72.0031130324519,
0.));
#132295=CARTESIAN_POINT('Ctrl Pts',(-14.8921840267829,-72.0031130324519,
12.));
#132296=CARTESIAN_POINT('Ctrl Pts',(-14.8770561943011,-71.9812714893087,
0.));
#132297=CARTESIAN_POINT('Ctrl Pts',(-14.8770561943011,-71.9812714893087,
12.));
#132298=CARTESIAN_POINT('Ctrl Pts',(-14.8619696177503,-71.9594464391063,
0.));
#132299=CARTESIAN_POINT('Ctrl Pts',(-14.8619696177503,-71.9594464391063,
12.));
#132300=CARTESIAN_POINT('Ctrl Pts',(-14.846924309716,-71.9376379869668,
0.));
#132301=CARTESIAN_POINT('Ctrl Pts',(-14.846924309716,-71.9376379869668,
12.));
#132302=CARTESIAN_POINT('Ctrl Pts',(-14.8319202827482,-71.9158462383915,
0.));
#132303=CARTESIAN_POINT('Ctrl Pts',(-14.8319202827482,-71.9158462383915,
12.));
#132304=CARTESIAN_POINT('Ctrl Pts',(-14.8169575493559,-71.8940712992119,
0.));
#132305=CARTESIAN_POINT('Ctrl Pts',(-14.8169575493559,-71.8940712992119,
12.));
#132306=CARTESIAN_POINT('Ctrl Pts',(-14.8020361220002,-71.872313275546,
0.));
#132307=CARTESIAN_POINT('Ctrl Pts',(-14.8020361220002,-71.872313275546,
12.));
#132308=CARTESIAN_POINT('Ctrl Pts',(-14.7871560131021,-71.8505722738286,
0.));
#132309=CARTESIAN_POINT('Ctrl Pts',(-14.7871560131021,-71.8505722738286,
12.));
#132310=CARTESIAN_POINT('Ctrl Pts',(-14.7723172350454,-71.8288484008343,
0.));
#132311=CARTESIAN_POINT('Ctrl Pts',(-14.7723172350454,-71.8288484008343,
12.));
#132312=CARTESIAN_POINT('Ctrl Pts',(-14.7575198001776,-71.8071417637019,
0.));
#132313=CARTESIAN_POINT('Ctrl Pts',(-14.7575198001776,-71.8071417637019,
12.));
#132314=CARTESIAN_POINT('Ctrl Pts',(-14.742763720807,-71.7854524699563,
0.));
#132315=CARTESIAN_POINT('Ctrl Pts',(-14.742763720807,-71.7854524699563,
12.));
#132316=CARTESIAN_POINT('Ctrl Pts',(-14.7280490091954,-71.7637806275316,
0.));
#132317=CARTESIAN_POINT('Ctrl Pts',(-14.7280490091954,-71.7637806275316,
12.));
#132318=CARTESIAN_POINT('Ctrl Pts',(-14.7133756775622,-71.7421263447707,
0.));
#132319=CARTESIAN_POINT('Ctrl Pts',(-14.7133756775622,-71.7421263447707,
12.));
#132320=CARTESIAN_POINT('Ctrl Pts',(-14.6987437380898,-71.7204897304186,
0.));
#132321=CARTESIAN_POINT('Ctrl Pts',(-14.6987437380898,-71.7204897304186,
12.));
#132322=CARTESIAN_POINT('Ctrl Pts',(-14.6841532029231,-71.698870893617,
0.));
#132323=CARTESIAN_POINT('Ctrl Pts',(-14.6841532029231,-71.698870893617,
12.));
#132324=CARTESIAN_POINT('Ctrl Pts',(-14.6696040841679,-71.6772699438966,
0.));
#132325=CARTESIAN_POINT('Ctrl Pts',(-14.6696040841679,-71.6772699438966,
12.));
#132326=CARTESIAN_POINT('Ctrl Pts',(-14.6550963938832,-71.6556869911669,
0.));
#132327=CARTESIAN_POINT('Ctrl Pts',(-14.6550963938832,-71.6556869911669,
12.));
#132328=CARTESIAN_POINT('Ctrl Pts',(-14.6406301440817,-71.6341221457175,
0.));
#132329=CARTESIAN_POINT('Ctrl Pts',(-14.6406301440817,-71.6341221457175,
12.));
#132330=CARTESIAN_POINT('Ctrl Pts',(-14.6262053467372,-71.6125755182295,
0.));
#132331=CARTESIAN_POINT('Ctrl Pts',(-14.6262053467372,-71.6125755182295,
12.));
#132332=CARTESIAN_POINT('Ctrl Pts',(-14.611822013785,-71.5910472197815,
0.));
#132333=CARTESIAN_POINT('Ctrl Pts',(-14.611822013785,-71.5910472197815,
12.));
#132334=CARTESIAN_POINT('Ctrl Pts',(-14.5974801571209,-71.569537361856,
0.));
#132335=CARTESIAN_POINT('Ctrl Pts',(-14.5974801571209,-71.569537361856,
12.));
#132336=CARTESIAN_POINT('Ctrl Pts',(-14.5831797885951,-71.5480460563445,
0.));
#132337=CARTESIAN_POINT('Ctrl Pts',(-14.5831797885951,-71.5480460563445,
12.));
#132338=CARTESIAN_POINT('Ctrl Pts',(-14.568920920009,-71.52657341555,0.));
#132339=CARTESIAN_POINT('Ctrl Pts',(-14.568920920009,-71.52657341555,12.));
#132340=CARTESIAN_POINT('Ctrl Pts',(-14.5547035631233,-71.5051195521914,
0.));
#132341=CARTESIAN_POINT('Ctrl Pts',(-14.5547035631233,-71.5051195521914,
12.));
#132342=CARTESIAN_POINT('Ctrl Pts',(-14.540527729659,-71.4836845794052,
0.));
#132343=CARTESIAN_POINT('Ctrl Pts',(-14.540527729659,-71.4836845794052,
12.));
#132344=CARTESIAN_POINT('Ctrl Pts',(-14.5263934312969,-71.4622686107475,
0.));
#132345=CARTESIAN_POINT('Ctrl Pts',(-14.5263934312969,-71.4622686107475,
12.));
#132346=CARTESIAN_POINT('Ctrl Pts',(-14.5123006796728,-71.4408717601917,
0.));
#132347=CARTESIAN_POINT('Ctrl Pts',(-14.5123006796728,-71.4408717601917,
12.));
#132348=CARTESIAN_POINT('Ctrl Pts',(-14.4982494863716,-71.4194941421279,
0.));
#132349=CARTESIAN_POINT('Ctrl Pts',(-14.4982494863716,-71.4194941421279,
12.));
#132350=CARTESIAN_POINT('Ctrl Pts',(-14.4842398629353,-71.398135871371,
0.));
#132351=CARTESIAN_POINT('Ctrl Pts',(-14.4842398629353,-71.398135871371,
12.));
#132352=CARTESIAN_POINT('Ctrl Pts',(-14.470271820865,-71.3767970631642,
0.));
#132353=CARTESIAN_POINT('Ctrl Pts',(-14.470271820865,-71.3767970631642,
12.));
#132354=CARTESIAN_POINT('Ctrl Pts',(-14.4563453716204,-71.3554778331835,
0.));
#132355=CARTESIAN_POINT('Ctrl Pts',(-14.4563453716204,-71.3554778331835,
12.));
#132356=CARTESIAN_POINT('Ctrl Pts',(-14.4424605266166,-71.3341782975393,
0.));
#132357=CARTESIAN_POINT('Ctrl Pts',(-14.4424605266166,-71.3341782975393,
12.));
#132358=CARTESIAN_POINT('Ctrl Pts',(-14.4286172972168,-71.3128985727777,
0.));
#132359=CARTESIAN_POINT('Ctrl Pts',(-14.4286172972168,-71.3128985727777,
12.));
#132360=CARTESIAN_POINT('Ctrl Pts',(-14.4148156947384,-71.2916387758864,
0.));
#132361=CARTESIAN_POINT('Ctrl Pts',(-14.4148156947384,-71.2916387758864,
12.));
#132362=CARTESIAN_POINT('Ctrl Pts',(-14.401055730457,-71.2703990242986,
0.));
#132363=CARTESIAN_POINT('Ctrl Pts',(-14.401055730457,-71.2703990242986,
12.));
#132364=CARTESIAN_POINT('Ctrl Pts',(-14.3873374156056,-71.2491794358956,
0.));
#132365=CARTESIAN_POINT('Ctrl Pts',(-14.3873374156056,-71.2491794358956,
12.));
#132366=CARTESIAN_POINT('Ctrl Pts',(-14.3736607613723,-71.2279801290088,
0.));
#132367=CARTESIAN_POINT('Ctrl Pts',(-14.3736607613723,-71.2279801290088,
12.));
#132368=CARTESIAN_POINT('Ctrl Pts',(-14.3600257788927,-71.2068012224187,
0.));
#132369=CARTESIAN_POINT('Ctrl Pts',(-14.3600257788927,-71.2068012224187,
12.));
#132370=CARTESIAN_POINT('Ctrl Pts',(-14.3464324792537,-71.185642835361,
0.));
#132371=CARTESIAN_POINT('Ctrl Pts',(-14.3464324792537,-71.185642835361,
12.));
#132372=CARTESIAN_POINT('Ctrl Pts',(-14.3328808734993,-71.1645050875323,
0.));
#132373=CARTESIAN_POINT('Ctrl Pts',(-14.3328808734993,-71.1645050875323,
12.));
#132374=CARTESIAN_POINT('Ctrl Pts',(-14.3193709726295,-71.1433880990932,
0.));
#132375=CARTESIAN_POINT('Ctrl Pts',(-14.3193709726295,-71.1433880990932,
12.));
#132376=CARTESIAN_POINT('Ctrl Pts',(-14.3059027875992,-71.1222919906718,
0.));
#132377=CARTESIAN_POINT('Ctrl Pts',(-14.3059027875992,-71.1222919906718,
12.));
#132378=CARTESIAN_POINT('Ctrl Pts',(-14.2924763293101,-71.1012168833626,
0.));
#132379=CARTESIAN_POINT('Ctrl Pts',(-14.2924763293101,-71.1012168833626,
12.));
#132380=CARTESIAN_POINT('Ctrl Pts',(-14.2790916086129,-71.0801628987314,
0.));
#132381=CARTESIAN_POINT('Ctrl Pts',(-14.2790916086129,-71.0801628987314,
12.));
#132382=CARTESIAN_POINT('Ctrl Pts',(-14.2657486363136,-71.059130158822,
0.));
#132383=CARTESIAN_POINT('Ctrl Pts',(-14.2657486363136,-71.059130158822,
12.));
#132384=CARTESIAN_POINT('Ctrl Pts',(-14.2524474231732,-71.0381187861585,
0.));
#132385=CARTESIAN_POINT('Ctrl Pts',(-14.2524474231732,-71.0381187861585,
12.));
#132386=CARTESIAN_POINT('Ctrl Pts',(-14.2391879799063,-71.0171289037493,
0.));
#132387=CARTESIAN_POINT('Ctrl Pts',(-14.2391879799063,-71.0171289037493,
12.));
#132388=CARTESIAN_POINT('Ctrl Pts',(-14.2259703171739,-70.996160635087,
0.));
#132389=CARTESIAN_POINT('Ctrl Pts',(-14.2259703171739,-70.996160635087,
12.));
#132390=CARTESIAN_POINT('Ctrl Pts',(-14.2127944455841,-70.9752141041527,
0.));
#132391=CARTESIAN_POINT('Ctrl Pts',(-14.2127944455841,-70.9752141041527,
12.));
#132392=CARTESIAN_POINT('Ctrl Pts',(-14.1996603756984,-70.9542894354221,
0.));
#132393=CARTESIAN_POINT('Ctrl Pts',(-14.1996603756984,-70.9542894354221,
12.));
#132394=CARTESIAN_POINT('Ctrl Pts',(-14.1865681180321,-70.9333867538705,
0.));
#132395=CARTESIAN_POINT('Ctrl Pts',(-14.1865681180321,-70.9333867538705,
12.));
#132396=CARTESIAN_POINT('Ctrl Pts',(-14.1735176830533,-70.9125061849744,
0.));
#132397=CARTESIAN_POINT('Ctrl Pts',(-14.1735176830533,-70.9125061849744,
12.));
#132398=CARTESIAN_POINT('Ctrl Pts',(-14.1605090811753,-70.8916478547131,
0.));
#132399=CARTESIAN_POINT('Ctrl Pts',(-14.1605090811753,-70.8916478547131,
12.));
#132400=CARTESIAN_POINT('Ctrl Pts',(-14.1475423227567,-70.8708118895718,
0.));
#132401=CARTESIAN_POINT('Ctrl Pts',(-14.1475423227567,-70.8708118895718,
12.));
#132402=CARTESIAN_POINT('Ctrl Pts',(-14.1346174181079,-70.8499984165493,
0.));
#132403=CARTESIAN_POINT('Ctrl Pts',(-14.1346174181079,-70.8499984165493,
12.));
#132404=CARTESIAN_POINT('Ctrl Pts',(-14.1217343774914,-70.8292075631624,
0.));
#132405=CARTESIAN_POINT('Ctrl Pts',(-14.1217343774914,-70.8292075631624,
12.));
#132406=CARTESIAN_POINT('Ctrl Pts',(-14.1088932111214,-70.8084394574491,
0.));
#132407=CARTESIAN_POINT('Ctrl Pts',(-14.1088932111214,-70.8084394574491,
12.));
#132408=CARTESIAN_POINT('Ctrl Pts',(-14.0960939291568,-70.787694227969,
0.));
#132409=CARTESIAN_POINT('Ctrl Pts',(-14.0960939291568,-70.787694227969,
12.));
#132410=CARTESIAN_POINT('Ctrl Pts',(-14.0833365416995,-70.7669720038067,
0.));
#132411=CARTESIAN_POINT('Ctrl Pts',(-14.0833365416995,-70.7669720038067,
12.));
#132412=CARTESIAN_POINT('Ctrl Pts',(-14.0706210588015,-70.7462729145799,
0.));
#132413=CARTESIAN_POINT('Ctrl Pts',(-14.0706210588015,-70.7462729145799,
12.));
#132414=CARTESIAN_POINT('Ctrl Pts',(-14.0579474904657,-70.7255970904433,
0.));
#132415=CARTESIAN_POINT('Ctrl Pts',(-14.0579474904657,-70.7255970904433,
12.));
#132416=CARTESIAN_POINT('Ctrl Pts',(-14.0453158466451,-70.7049446620931,
0.));
#132417=CARTESIAN_POINT('Ctrl Pts',(-14.0453158466451,-70.7049446620931,
12.));
#132418=CARTESIAN_POINT('Ctrl Pts',(-14.0327261372363,-70.6843157607672,
0.));
#132419=CARTESIAN_POINT('Ctrl Pts',(-14.0327261372363,-70.6843157607672,
12.));
#132420=CARTESIAN_POINT('Ctrl Pts',(-14.020178372077,-70.6637105182487,
0.));
#132421=CARTESIAN_POINT('Ctrl Pts',(-14.020178372077,-70.6637105182487,
12.));
#132422=CARTESIAN_POINT('Ctrl Pts',(-14.0076725609536,-70.6431290668744,
0.));
#132423=CARTESIAN_POINT('Ctrl Pts',(-14.0076725609536,-70.6431290668744,
12.));
#132424=CARTESIAN_POINT('Ctrl Pts',(-13.9952087136018,-70.6225715395392,
0.));
#132425=CARTESIAN_POINT('Ctrl Pts',(-13.9952087136018,-70.6225715395392,
12.));
#132426=CARTESIAN_POINT('Ctrl Pts',(-13.9827868397057,-70.6020380697004,
0.));
#132427=CARTESIAN_POINT('Ctrl Pts',(-13.9827868397057,-70.6020380697004,
12.));
#132428=CARTESIAN_POINT('Ctrl Pts',(-13.9704069488918,-70.5815287913791,
0.));
#132429=CARTESIAN_POINT('Ctrl Pts',(-13.9704069488918,-70.5815287913791,
12.));
#132430=CARTESIAN_POINT('Ctrl Pts',(-13.9580690507262,-70.5610438391622,
0.));
#132431=CARTESIAN_POINT('Ctrl Pts',(-13.9580690507262,-70.5610438391622,
12.));
#132432=CARTESIAN_POINT('Ctrl Pts',(-13.9457731547217,-70.5405833482123,
0.));
#132433=CARTESIAN_POINT('Ctrl Pts',(-13.9457731547217,-70.5405833482123,
12.));
#132434=CARTESIAN_POINT('Ctrl Pts',(-13.9335192703389,-70.5201474542717,
0.));
#132435=CARTESIAN_POINT('Ctrl Pts',(-13.9335192703389,-70.5201474542717,
12.));
#132436=CARTESIAN_POINT('Ctrl Pts',(-13.9213074069852,-70.4997362936671,
0.));
#132437=CARTESIAN_POINT('Ctrl Pts',(-13.9213074069852,-70.4997362936671,
12.));
#132438=CARTESIAN_POINT('Ctrl Pts',(-13.9091375740084,-70.4793500033106,
0.));
#132439=CARTESIAN_POINT('Ctrl Pts',(-13.9091375740084,-70.4793500033106,
12.));
#132440=CARTESIAN_POINT('Ctrl Pts',(-13.8970097806947,-70.4589887207043,
0.));
#132441=CARTESIAN_POINT('Ctrl Pts',(-13.8970097806947,-70.4589887207043,
12.));
#132442=CARTESIAN_POINT('Ctrl Pts',(-13.8849240362757,-70.4386525839492,
0.));
#132443=CARTESIAN_POINT('Ctrl Pts',(-13.8849240362757,-70.4386525839492,
12.));
#132444=CARTESIAN_POINT('Ctrl Pts',(-13.8728803499284,-70.4183417317486,
0.));
#132445=CARTESIAN_POINT('Ctrl Pts',(-13.8728803499284,-70.4183417317486,
12.));
#132446=CARTESIAN_POINT('Ctrl Pts',(-13.8608787307753,-70.3980563034142,
0.));
#132447=CARTESIAN_POINT('Ctrl Pts',(-13.8608787307753,-70.3980563034142,
12.));
#132448=CARTESIAN_POINT('Ctrl Pts',(-13.8489191878774,-70.377796438866,
0.));
#132449=CARTESIAN_POINT('Ctrl Pts',(-13.8489191878774,-70.377796438866,
12.));
#132450=CARTESIAN_POINT('Ctrl Pts',(-13.8370017302318,-70.3575622786373,
0.));
#132451=CARTESIAN_POINT('Ctrl Pts',(-13.8370017302318,-70.3575622786373,
12.));
#132452=CARTESIAN_POINT('Ctrl Pts',(-13.8251263667799,-70.3373539638841,
0.));
#132453=CARTESIAN_POINT('Ctrl Pts',(-13.8251263667799,-70.3373539638841,
12.));
#132454=CARTESIAN_POINT('Ctrl Pts',(-13.8132931064067,-70.3171716363912,
0.));
#132455=CARTESIAN_POINT('Ctrl Pts',(-13.8132931064067,-70.3171716363912,
12.));
#132456=CARTESIAN_POINT('Ctrl Pts',(-13.8015019579411,-70.2970154385763,
0.));
#132457=CARTESIAN_POINT('Ctrl Pts',(-13.8015019579411,-70.2970154385763,
12.));
#132458=CARTESIAN_POINT('Ctrl Pts',(-13.7897529301482,-70.2768855134909,
0.));
#132459=CARTESIAN_POINT('Ctrl Pts',(-13.7897529301482,-70.2768855134909,
12.));
#132460=CARTESIAN_POINT('Ctrl Pts',(-13.7780460317284,-70.2567820048253,
0.));
#132461=CARTESIAN_POINT('Ctrl Pts',(-13.7780460317284,-70.2567820048253,
12.));
#132462=CARTESIAN_POINT('Ctrl Pts',(-13.7663812713235,-70.2367050569174,
0.));
#132463=CARTESIAN_POINT('Ctrl Pts',(-13.7663812713235,-70.2367050569174,
12.));
#132464=CARTESIAN_POINT('Ctrl Pts',(-13.7547586575178,-70.216654814759,
0.));
#132465=CARTESIAN_POINT('Ctrl Pts',(-13.7547586575178,-70.216654814759,
12.));
#132466=CARTESIAN_POINT('Ctrl Pts',(-13.7431781988368,-70.1966314240012,
0.));
#132467=CARTESIAN_POINT('Ctrl Pts',(-13.7431781988368,-70.1966314240012,
12.));
#132468=CARTESIAN_POINT('Ctrl Pts',(-13.73163990374,-70.1766350309554,0.));
#132469=CARTESIAN_POINT('Ctrl Pts',(-13.73163990374,-70.1766350309554,12.));
#132470=CARTESIAN_POINT('Ctrl Pts',(-13.7201437806207,-70.1566657825989,
0.));
#132471=CARTESIAN_POINT('Ctrl Pts',(-13.7201437806207,-70.1566657825989,
12.));
#132472=CARTESIAN_POINT('Ctrl Pts',(-13.7086898378127,-70.1367238265853,
0.));
#132473=CARTESIAN_POINT('Ctrl Pts',(-13.7086898378127,-70.1367238265853,
12.));
#132474=CARTESIAN_POINT('Ctrl Pts',(-13.6972780835898,-70.1168093112493,
0.));
#132475=CARTESIAN_POINT('Ctrl Pts',(-13.6972780835898,-70.1168093112493,
12.));
#132476=CARTESIAN_POINT('Ctrl Pts',(-13.685908526165,-70.0969223856123,
0.));
#132477=CARTESIAN_POINT('Ctrl Pts',(-13.685908526165,-70.0969223856123,
12.));
#132478=CARTESIAN_POINT('Ctrl Pts',(-13.6745811736825,-70.0770631993831,
0.));
#132479=CARTESIAN_POINT('Ctrl Pts',(-13.6745811736825,-70.0770631993831,
12.));
#132480=CARTESIAN_POINT('Ctrl Pts',(-13.6632960342192,-70.057231902965,
0.));
#132481=CARTESIAN_POINT('Ctrl Pts',(-13.6632960342192,-70.057231902965,
12.));
#132482=CARTESIAN_POINT('Ctrl Pts',(-13.6520531157904,-70.037428647466,
0.));
#132483=CARTESIAN_POINT('Ctrl Pts',(-13.6520531157904,-70.037428647466,
12.));
#132484=CARTESIAN_POINT('Ctrl Pts',(-13.6408524263496,-70.0176535847047,
0.));
#132485=CARTESIAN_POINT('Ctrl Pts',(-13.6408524263496,-70.0176535847047,
12.));
#132486=CARTESIAN_POINT('Ctrl Pts',(-13.6296939737866,-69.9979068672163,
0.));
#132487=CARTESIAN_POINT('Ctrl Pts',(-13.6296939737866,-69.9979068672163,
12.));
#132488=CARTESIAN_POINT('Ctrl Pts',(-13.61857776592,-69.9781886482543,0.));
#132489=CARTESIAN_POINT('Ctrl Pts',(-13.61857776592,-69.9781886482543,12.));
#132490=CARTESIAN_POINT('Ctrl Pts',(-13.6075038105,-69.9584990817989,0.));
#132491=CARTESIAN_POINT('Ctrl Pts',(-13.6075038105,-69.9584990817989,12.));
#132492=CARTESIAN_POINT('Ctrl Pts',(-13.5964721152136,-69.9388383225655,
0.));
#132493=CARTESIAN_POINT('Ctrl Pts',(-13.5964721152136,-69.9388383225655,
12.));
#132494=CARTESIAN_POINT('Ctrl Pts',(-13.5854826876834,-69.9192065260107,
0.));
#132495=CARTESIAN_POINT('Ctrl Pts',(-13.5854826876834,-69.9192065260107,
12.));
#132496=CARTESIAN_POINT('Ctrl Pts',(-13.5745355354657,-69.899603848336,
0.));
#132497=CARTESIAN_POINT('Ctrl Pts',(-13.5745355354657,-69.899603848336,
12.));
#132498=CARTESIAN_POINT('Ctrl Pts',(-13.5636306660422,-69.880030446488,
0.));
#132499=CARTESIAN_POINT('Ctrl Pts',(-13.5636306660422,-69.880030446488,
12.));
#132500=CARTESIAN_POINT('Ctrl Pts',(-13.5527680868256,-69.8604864781705,
0.));
#132501=CARTESIAN_POINT('Ctrl Pts',(-13.5527680868256,-69.8604864781705,
12.));
#132502=CARTESIAN_POINT('Ctrl Pts',(-13.5419478051626,-69.840972101856,
0.));
#132503=CARTESIAN_POINT('Ctrl Pts',(-13.5419478051626,-69.840972101856,
12.));
#132504=CARTESIAN_POINT('Ctrl Pts',(-13.5311698283339,-69.8214874767944,
0.));
#132505=CARTESIAN_POINT('Ctrl Pts',(-13.5311698283339,-69.8214874767944,
12.));
#132506=CARTESIAN_POINT('Ctrl Pts',(-13.5204341635507,-69.8020327630204,
0.));
#132507=CARTESIAN_POINT('Ctrl Pts',(-13.5204341635507,-69.8020327630204,
12.));
#132508=CARTESIAN_POINT('Ctrl Pts',(-13.5097408179478,-69.7826081213575,
0.));
#132509=CARTESIAN_POINT('Ctrl Pts',(-13.5097408179478,-69.7826081213575,
12.));
#132510=CARTESIAN_POINT('Ctrl Pts',(-13.4990897985903,-69.7632137134247,
0.));
#132511=CARTESIAN_POINT('Ctrl Pts',(-13.4990897985903,-69.7632137134247,
12.));
#132512=CARTESIAN_POINT('Ctrl Pts',(-13.4884811124748,-69.7438497016404,
0.));
#132513=CARTESIAN_POINT('Ctrl Pts',(-13.4884811124748,-69.7438497016404,
12.));
#132514=CARTESIAN_POINT('Ctrl Pts',(-13.4779147665285,-69.7245162492251,
0.));
#132515=CARTESIAN_POINT('Ctrl Pts',(-13.4779147665285,-69.7245162492251,
12.));
#132516=CARTESIAN_POINT('Ctrl Pts',(-13.4673907676045,-69.7052135202003,
0.));
#132517=CARTESIAN_POINT('Ctrl Pts',(-13.4673907676045,-69.7052135202003,
12.));
#132518=CARTESIAN_POINT('Ctrl Pts',(-13.4569091224762,-69.6859416793898,
0.));
#132519=CARTESIAN_POINT('Ctrl Pts',(-13.4569091224762,-69.6859416793898,
12.));
#132520=CARTESIAN_POINT('Ctrl Pts',(-13.4464698378456,-69.6667008924454,
0.));
#132521=CARTESIAN_POINT('Ctrl Pts',(-13.4464698378456,-69.6667008924454,
12.));
#132522=CARTESIAN_POINT('Ctrl Pts',(-13.4360729203444,-69.6474913258684,
0.));
#132523=CARTESIAN_POINT('Ctrl Pts',(-13.4360729203444,-69.6474913258684,
12.));
#132524=CARTESIAN_POINT('Ctrl Pts',(-13.425718376534,-69.6283131470267,
0.));
#132525=CARTESIAN_POINT('Ctrl Pts',(-13.425718376534,-69.6283131470267,
12.));
#132526=CARTESIAN_POINT('Ctrl Pts',(-13.4154062128998,-69.6091665241743,
0.));
#132527=CARTESIAN_POINT('Ctrl Pts',(-13.4154062128998,-69.6091665241743,
12.));
#132528=CARTESIAN_POINT('Ctrl Pts',(-13.4051364358494,-69.5900516264524,
0.));
#132529=CARTESIAN_POINT('Ctrl Pts',(-13.4051364358494,-69.5900516264524,
12.));
#132530=CARTESIAN_POINT('Ctrl Pts',(-13.3949090517173,-69.5709686238701,
0.));
#132531=CARTESIAN_POINT('Ctrl Pts',(-13.3949090517173,-69.5709686238701,
12.));
#132532=CARTESIAN_POINT('Ctrl Pts',(-13.3847240667626,-69.5519176872857,
0.));
#132533=CARTESIAN_POINT('Ctrl Pts',(-13.3847240667626,-69.5519176872857,
12.));
#132534=CARTESIAN_POINT('Ctrl Pts',(-13.3745814871667,-69.5328989883899,
0.));
#132535=CARTESIAN_POINT('Ctrl Pts',(-13.3745814871667,-69.5328989883899,
12.));
#132536=CARTESIAN_POINT('Ctrl Pts',(-13.3644813190225,-69.5139126996703,
0.));
#132537=CARTESIAN_POINT('Ctrl Pts',(-13.3644813190225,-69.5139126996703,
12.));
#132538=CARTESIAN_POINT('Ctrl Pts',(-13.3544235683399,-69.4949589944633,
0.));
#132539=CARTESIAN_POINT('Ctrl Pts',(-13.3544235683399,-69.4949589944633,
12.));
#132540=CARTESIAN_POINT('Ctrl Pts',(-13.3444082410546,-69.4760380470382,
0.));
#132541=CARTESIAN_POINT('Ctrl Pts',(-13.3444082410546,-69.4760380470382,
12.));
#132542=CARTESIAN_POINT('Ctrl Pts',(-13.3344353430313,-69.4571500326673,
0.));
#132543=CARTESIAN_POINT('Ctrl Pts',(-13.3344353430313,-69.4571500326673,
12.));
#132544=CARTESIAN_POINT('Ctrl Pts',(-13.3245048800641,-69.4382951276983,
0.));
#132545=CARTESIAN_POINT('Ctrl Pts',(-13.3245048800641,-69.4382951276983,
12.));
#132546=CARTESIAN_POINT('Ctrl Pts',(-13.3146168578738,-69.4194735096238,
0.));
#132547=CARTESIAN_POINT('Ctrl Pts',(-13.3146168578738,-69.4194735096238,
12.));
#132548=CARTESIAN_POINT('Ctrl Pts',(-13.3047712821046,-69.4006853569485,
0.));
#132549=CARTESIAN_POINT('Ctrl Pts',(-13.3047712821046,-69.4006853569485,
12.));
#132550=CARTESIAN_POINT('Ctrl Pts',(-13.2949681583164,-69.3819308490408,
0.));
#132551=CARTESIAN_POINT('Ctrl Pts',(-13.2949681583164,-69.3819308490408,
12.));
#132552=CARTESIAN_POINT('Ctrl Pts',(-13.2852074919767,-69.3632101660072,
0.));
#132553=CARTESIAN_POINT('Ctrl Pts',(-13.2852074919767,-69.3632101660072,
12.));
#132554=CARTESIAN_POINT('Ctrl Pts',(-13.2754892884437,-69.3445234885088,
0.));
#132555=CARTESIAN_POINT('Ctrl Pts',(-13.2754892884437,-69.3445234885088,
12.));
#132556=CARTESIAN_POINT('Ctrl Pts',(-13.2658135529616,-69.3258709977416,
0.));
#132557=CARTESIAN_POINT('Ctrl Pts',(-13.2658135529616,-69.3258709977416,
12.));
#132558=CARTESIAN_POINT('Ctrl Pts',(-13.2561802906901,-69.3072528758546,
0.));
#132559=CARTESIAN_POINT('Ctrl Pts',(-13.2561802906901,-69.3072528758546,
12.));
#132560=CARTESIAN_POINT('Ctrl Pts',(-13.2465895067264,-69.2886693063193,
0.));
#132561=CARTESIAN_POINT('Ctrl Pts',(-13.2465895067264,-69.2886693063193,
12.));
#132562=CARTESIAN_POINT('Ctrl Pts',(-13.2370412061218,-69.2701204742436,
0.));
#132563=CARTESIAN_POINT('Ctrl Pts',(-13.2370412061218,-69.2701204742436,
12.));
#132564=CARTESIAN_POINT('Ctrl Pts',(-13.2275353939044,-69.2516065668809,
0.));
#132565=CARTESIAN_POINT('Ctrl Pts',(-13.2275353939044,-69.2516065668809,
12.));
#132566=CARTESIAN_POINT('Ctrl Pts',(-13.2180720750585,-69.2331277732819,
0.));
#132567=CARTESIAN_POINT('Ctrl Pts',(-13.2180720750585,-69.2331277732819,
12.));
#132568=CARTESIAN_POINT('Ctrl Pts',(-13.2086512544729,-69.2146842833506,
0.));
#132569=CARTESIAN_POINT('Ctrl Pts',(-13.2086512544729,-69.2146842833506,
12.));
#132570=CARTESIAN_POINT('Ctrl Pts',(-13.1992729368928,-69.1962762870524,
0.));
#132571=CARTESIAN_POINT('Ctrl Pts',(-13.1992729368928,-69.1962762870524,
12.));
#132572=CARTESIAN_POINT('Ctrl Pts',(-13.1899371268689,-69.1779039736026,
0.));
#132573=CARTESIAN_POINT('Ctrl Pts',(-13.1899371268689,-69.1779039736026,
12.));
#132574=CARTESIAN_POINT('Ctrl Pts',(-13.1806438286944,-69.1595675305294,
0.));
#132575=CARTESIAN_POINT('Ctrl Pts',(-13.1806438286944,-69.1595675305294,
12.));
#132576=CARTESIAN_POINT('Ctrl Pts',(-13.1713930465142,-69.141267145461,
0.));
#132577=CARTESIAN_POINT('Ctrl Pts',(-13.1713930465142,-69.141267145461,
12.));
#132578=CARTESIAN_POINT('Ctrl Pts',(-13.1621847844533,-69.1230030082597,
0.));
#132579=CARTESIAN_POINT('Ctrl Pts',(-13.1621847844533,-69.1230030082597,
12.));
#132580=CARTESIAN_POINT('Ctrl Pts',(-13.1530190467181,-69.1047753127633,
0.));
#132581=CARTESIAN_POINT('Ctrl Pts',(-13.1530190467181,-69.1047753127633,
12.));
#132582=CARTESIAN_POINT('Ctrl Pts',(-13.1438958377397,-69.0865842593063,
0.));
#132583=CARTESIAN_POINT('Ctrl Pts',(-13.1438958377397,-69.0865842593063,
12.));
#132584=CARTESIAN_POINT('Ctrl Pts',(-13.1348151621824,-69.0684300549426,
0.));
#132585=CARTESIAN_POINT('Ctrl Pts',(-13.1348151621824,-69.0684300549426,
12.));
#132586=CARTESIAN_POINT('Ctrl Pts',(-13.1257770246378,-69.0503129081778,
0.));
#132587=CARTESIAN_POINT('Ctrl Pts',(-13.1257770246378,-69.0503129081778,
12.));
#132588=CARTESIAN_POINT('Ctrl Pts',(-13.1167814293495,-69.0322330243336,
0.));
#132589=CARTESIAN_POINT('Ctrl Pts',(-13.1167814293495,-69.0322330243336,
12.));
#132590=CARTESIAN_POINT('Ctrl Pts',(-13.1078283799726,-69.0141906015137,
0.));
#132591=CARTESIAN_POINT('Ctrl Pts',(-13.1078283799726,-69.0141906015137,
12.));
#132592=CARTESIAN_POINT('Ctrl Pts',(-13.0989178791843,-68.9961858241577,
0.));
#132593=CARTESIAN_POINT('Ctrl Pts',(-13.0989178791843,-68.9961858241577,
12.));
#132594=CARTESIAN_POINT('Ctrl Pts',(-13.0900499290541,-68.9782188692654,
0.));
#132595=CARTESIAN_POINT('Ctrl Pts',(-13.0900499290541,-68.9782188692654,
12.));
#132596=CARTESIAN_POINT('Ctrl Pts',(-13.0812245317816,-68.9602899187628,
0.));
#132597=CARTESIAN_POINT('Ctrl Pts',(-13.0812245317816,-68.9602899187628,
12.));
#132598=CARTESIAN_POINT('Ctrl Pts',(-13.072441690283,-68.9423991694493,
0.));
#132599=CARTESIAN_POINT('Ctrl Pts',(-13.072441690283,-68.9423991694493,
12.));
#132600=CARTESIAN_POINT('Ctrl Pts',(-13.0637014089018,-68.9245468449865,
0.));
#132601=CARTESIAN_POINT('Ctrl Pts',(-13.0637014089018,-68.9245468449865,
12.));
#132602=CARTESIAN_POINT('Ctrl Pts',(-13.0550036938793,-68.9067332040842,
0.));
#132603=CARTESIAN_POINT('Ctrl Pts',(-13.0550036938793,-68.9067332040842,
12.));
#132604=CARTESIAN_POINT('Ctrl Pts',(-13.0463485518185,-68.8889585151431,
0.));
#132605=CARTESIAN_POINT('Ctrl Pts',(-13.0463485518185,-68.8889585151431,
12.));
#132606=CARTESIAN_POINT('Ctrl Pts',(-13.0377359881863,-68.8712230321823,
0.));
#132607=CARTESIAN_POINT('Ctrl Pts',(-13.0377359881863,-68.8712230321823,
12.));
#132608=CARTESIAN_POINT('Ctrl Pts',(-13.0291660060118,-68.8535269726871,
0.));
#132609=CARTESIAN_POINT('Ctrl Pts',(-13.0291660060118,-68.8535269726871,
12.));
#132610=CARTESIAN_POINT('Ctrl Pts',(-13.0206386039729,-68.835870488774,
0.));
#132611=CARTESIAN_POINT('Ctrl Pts',(-13.0206386039729,-68.835870488774,
12.));
#132612=CARTESIAN_POINT('Ctrl Pts',(-13.0121537769003,-68.8182536654067,
0.));
#132613=CARTESIAN_POINT('Ctrl Pts',(-13.0121537769003,-68.8182536654067,
12.));
#132614=CARTESIAN_POINT('Ctrl Pts',(-13.0053999700929,-68.8041919669403,
0.));
#132615=CARTESIAN_POINT('Ctrl Pts',(-13.0053999700929,-68.8041919669403,
12.));
#132616=CARTESIAN_POINT('Ctrl Pts',(-13.0003537683089,-68.7936635625788,
0.));
#132617=CARTESIAN_POINT('Ctrl Pts',(-13.0003537683089,-68.7936635625788,
12.));
#132618=CARTESIAN_POINT('Ctrl Pts',(-12.996998146029,-68.7866525680284,
0.));
#132619=CARTESIAN_POINT('Ctrl Pts',(-12.996998146029,-68.7866525680284,
12.));
#132620=CARTESIAN_POINT('Ctrl Pts',(-12.9953224629497,-68.7831490561748,
0.));
#132621=CARTESIAN_POINT('Ctrl Pts',(-12.9953224629497,-68.7831490561748,
12.));
#132622=CARTESIAN_POINT('',(-12.9953224629497,-68.7831490561748,12.));
#132623=CARTESIAN_POINT('Ctrl Pts',(-12.9953224629497,-68.7831490561748,
12.));
#132624=CARTESIAN_POINT('Ctrl Pts',(-12.996998146029,-68.7866525680284,
12.));
#132625=CARTESIAN_POINT('Ctrl Pts',(-13.0003537683089,-68.7936635625788,
12.));
#132626=CARTESIAN_POINT('Ctrl Pts',(-13.0053999700929,-68.8041919669403,
12.));
#132627=CARTESIAN_POINT('Ctrl Pts',(-13.0121537769003,-68.8182536654067,
12.));
#132628=CARTESIAN_POINT('Ctrl Pts',(-13.0206386039729,-68.835870488774,
12.));
#132629=CARTESIAN_POINT('Ctrl Pts',(-13.0291660060118,-68.8535269726871,
12.));
#132630=CARTESIAN_POINT('Ctrl Pts',(-13.0377359881863,-68.8712230321823,
12.));
#132631=CARTESIAN_POINT('Ctrl Pts',(-13.0463485518185,-68.8889585151431,
12.));
#132632=CARTESIAN_POINT('Ctrl Pts',(-13.0550036938793,-68.9067332040842,
12.));
#132633=CARTESIAN_POINT('Ctrl Pts',(-13.0637014089018,-68.9245468449865,
12.));
#132634=CARTESIAN_POINT('Ctrl Pts',(-13.072441690283,-68.9423991694493,
12.));
#132635=CARTESIAN_POINT('Ctrl Pts',(-13.0812245317816,-68.9602899187628,
12.));
#132636=CARTESIAN_POINT('Ctrl Pts',(-13.0900499290541,-68.9782188692654,
12.));
#132637=CARTESIAN_POINT('Ctrl Pts',(-13.0989178791843,-68.9961858241577,
12.));
#132638=CARTESIAN_POINT('Ctrl Pts',(-13.1078283799726,-69.0141906015137,
12.));
#132639=CARTESIAN_POINT('Ctrl Pts',(-13.1167814293495,-69.0322330243336,
12.));
#132640=CARTESIAN_POINT('Ctrl Pts',(-13.1257770246378,-69.0503129081778,
12.));
#132641=CARTESIAN_POINT('Ctrl Pts',(-13.1348151621824,-69.0684300549426,
12.));
#132642=CARTESIAN_POINT('Ctrl Pts',(-13.1438958377397,-69.0865842593063,
12.));
#132643=CARTESIAN_POINT('Ctrl Pts',(-13.1530190467181,-69.1047753127633,
12.));
#132644=CARTESIAN_POINT('Ctrl Pts',(-13.1621847844533,-69.1230030082597,
12.));
#132645=CARTESIAN_POINT('Ctrl Pts',(-13.1713930465142,-69.141267145461,
12.));
#132646=CARTESIAN_POINT('Ctrl Pts',(-13.1806438286944,-69.1595675305294,
12.));
#132647=CARTESIAN_POINT('Ctrl Pts',(-13.1899371268689,-69.1779039736026,
12.));
#132648=CARTESIAN_POINT('Ctrl Pts',(-13.1992729368928,-69.1962762870524,
12.));
#132649=CARTESIAN_POINT('Ctrl Pts',(-13.2086512544729,-69.2146842833506,
12.));
#132650=CARTESIAN_POINT('Ctrl Pts',(-13.2180720750585,-69.2331277732819,
12.));
#132651=CARTESIAN_POINT('Ctrl Pts',(-13.2275353939044,-69.2516065668809,
12.));
#132652=CARTESIAN_POINT('Ctrl Pts',(-13.2370412061218,-69.2701204742436,
12.));
#132653=CARTESIAN_POINT('Ctrl Pts',(-13.2465895067264,-69.2886693063193,
12.));
#132654=CARTESIAN_POINT('Ctrl Pts',(-13.2561802906901,-69.3072528758546,
12.));
#132655=CARTESIAN_POINT('Ctrl Pts',(-13.2658135529616,-69.3258709977416,
12.));
#132656=CARTESIAN_POINT('Ctrl Pts',(-13.2754892884437,-69.3445234885088,
12.));
#132657=CARTESIAN_POINT('Ctrl Pts',(-13.2852074919767,-69.3632101660072,
12.));
#132658=CARTESIAN_POINT('Ctrl Pts',(-13.2949681583164,-69.3819308490408,
12.));
#132659=CARTESIAN_POINT('Ctrl Pts',(-13.3047712821046,-69.4006853569485,
12.));
#132660=CARTESIAN_POINT('Ctrl Pts',(-13.3146168578738,-69.4194735096238,
12.));
#132661=CARTESIAN_POINT('Ctrl Pts',(-13.3245048800641,-69.4382951276983,
12.));
#132662=CARTESIAN_POINT('Ctrl Pts',(-13.3344353430313,-69.4571500326673,
12.));
#132663=CARTESIAN_POINT('Ctrl Pts',(-13.3444082410546,-69.4760380470382,
12.));
#132664=CARTESIAN_POINT('Ctrl Pts',(-13.3544235683399,-69.4949589944633,
12.));
#132665=CARTESIAN_POINT('Ctrl Pts',(-13.3644813190225,-69.5139126996703,
12.));
#132666=CARTESIAN_POINT('Ctrl Pts',(-13.3745814871667,-69.5328989883899,
12.));
#132667=CARTESIAN_POINT('Ctrl Pts',(-13.3847240667626,-69.5519176872857,
12.));
#132668=CARTESIAN_POINT('Ctrl Pts',(-13.3949090517173,-69.5709686238701,
12.));
#132669=CARTESIAN_POINT('Ctrl Pts',(-13.4051364358494,-69.5900516264524,
12.));
#132670=CARTESIAN_POINT('Ctrl Pts',(-13.4154062128998,-69.6091665241743,
12.));
#132671=CARTESIAN_POINT('Ctrl Pts',(-13.425718376534,-69.6283131470267,
12.));
#132672=CARTESIAN_POINT('Ctrl Pts',(-13.4360729203444,-69.6474913258684,
12.));
#132673=CARTESIAN_POINT('Ctrl Pts',(-13.4464698378456,-69.6667008924454,
12.));
#132674=CARTESIAN_POINT('Ctrl Pts',(-13.4569091224762,-69.6859416793898,
12.));
#132675=CARTESIAN_POINT('Ctrl Pts',(-13.4673907676045,-69.7052135202003,
12.));
#132676=CARTESIAN_POINT('Ctrl Pts',(-13.4779147665285,-69.7245162492251,
12.));
#132677=CARTESIAN_POINT('Ctrl Pts',(-13.4884811124748,-69.7438497016404,
12.));
#132678=CARTESIAN_POINT('Ctrl Pts',(-13.4990897985903,-69.7632137134247,
12.));
#132679=CARTESIAN_POINT('Ctrl Pts',(-13.5097408179478,-69.7826081213575,
12.));
#132680=CARTESIAN_POINT('Ctrl Pts',(-13.5204341635507,-69.8020327630204,
12.));
#132681=CARTESIAN_POINT('Ctrl Pts',(-13.5311698283339,-69.8214874767944,
12.));
#132682=CARTESIAN_POINT('Ctrl Pts',(-13.5419478051626,-69.840972101856,
12.));
#132683=CARTESIAN_POINT('Ctrl Pts',(-13.5527680868256,-69.8604864781705,
12.));
#132684=CARTESIAN_POINT('Ctrl Pts',(-13.5636306660422,-69.880030446488,
12.));
#132685=CARTESIAN_POINT('Ctrl Pts',(-13.5745355354657,-69.899603848336,
12.));
#132686=CARTESIAN_POINT('Ctrl Pts',(-13.5854826876834,-69.9192065260107,
12.));
#132687=CARTESIAN_POINT('Ctrl Pts',(-13.5964721152136,-69.9388383225655,
12.));
#132688=CARTESIAN_POINT('Ctrl Pts',(-13.6075038105,-69.9584990817989,12.));
#132689=CARTESIAN_POINT('Ctrl Pts',(-13.61857776592,-69.9781886482543,12.));
#132690=CARTESIAN_POINT('Ctrl Pts',(-13.6296939737866,-69.9979068672163,
12.));
#132691=CARTESIAN_POINT('Ctrl Pts',(-13.6408524263496,-70.0176535847047,
12.));
#132692=CARTESIAN_POINT('Ctrl Pts',(-13.6520531157904,-70.037428647466,
12.));
#132693=CARTESIAN_POINT('Ctrl Pts',(-13.6632960342192,-70.057231902965,
12.));
#132694=CARTESIAN_POINT('Ctrl Pts',(-13.6745811736825,-70.0770631993831,
12.));
#132695=CARTESIAN_POINT('Ctrl Pts',(-13.685908526165,-70.0969223856123,
12.));
#132696=CARTESIAN_POINT('Ctrl Pts',(-13.6972780835898,-70.1168093112493,
12.));
#132697=CARTESIAN_POINT('Ctrl Pts',(-13.7086898378127,-70.1367238265853,
12.));
#132698=CARTESIAN_POINT('Ctrl Pts',(-13.7201437806207,-70.1566657825989,
12.));
#132699=CARTESIAN_POINT('Ctrl Pts',(-13.73163990374,-70.1766350309554,12.));
#132700=CARTESIAN_POINT('Ctrl Pts',(-13.7431781988368,-70.1966314240012,
12.));
#132701=CARTESIAN_POINT('Ctrl Pts',(-13.7547586575178,-70.216654814759,
12.));
#132702=CARTESIAN_POINT('Ctrl Pts',(-13.7663812713235,-70.2367050569174,
12.));
#132703=CARTESIAN_POINT('Ctrl Pts',(-13.7780460317284,-70.2567820048253,
12.));
#132704=CARTESIAN_POINT('Ctrl Pts',(-13.7897529301482,-70.2768855134909,
12.));
#132705=CARTESIAN_POINT('Ctrl Pts',(-13.8015019579411,-70.2970154385763,
12.));
#132706=CARTESIAN_POINT('Ctrl Pts',(-13.8132931064067,-70.3171716363912,
12.));
#132707=CARTESIAN_POINT('Ctrl Pts',(-13.8251263667799,-70.3373539638841,
12.));
#132708=CARTESIAN_POINT('Ctrl Pts',(-13.8370017302318,-70.3575622786373,
12.));
#132709=CARTESIAN_POINT('Ctrl Pts',(-13.8489191878774,-70.377796438866,
12.));
#132710=CARTESIAN_POINT('Ctrl Pts',(-13.8608787307753,-70.3980563034142,
12.));
#132711=CARTESIAN_POINT('Ctrl Pts',(-13.8728803499284,-70.4183417317486,
12.));
#132712=CARTESIAN_POINT('Ctrl Pts',(-13.8849240362757,-70.4386525839492,
12.));
#132713=CARTESIAN_POINT('Ctrl Pts',(-13.8970097806947,-70.4589887207043,
12.));
#132714=CARTESIAN_POINT('Ctrl Pts',(-13.9091375740084,-70.4793500033106,
12.));
#132715=CARTESIAN_POINT('Ctrl Pts',(-13.9213074069852,-70.4997362936671,
12.));
#132716=CARTESIAN_POINT('Ctrl Pts',(-13.9335192703389,-70.5201474542717,
12.));
#132717=CARTESIAN_POINT('Ctrl Pts',(-13.9457731547217,-70.5405833482123,
12.));
#132718=CARTESIAN_POINT('Ctrl Pts',(-13.9580690507262,-70.5610438391622,
12.));
#132719=CARTESIAN_POINT('Ctrl Pts',(-13.9704069488918,-70.5815287913791,
12.));
#132720=CARTESIAN_POINT('Ctrl Pts',(-13.9827868397057,-70.6020380697004,
12.));
#132721=CARTESIAN_POINT('Ctrl Pts',(-13.9952087136018,-70.6225715395392,
12.));
#132722=CARTESIAN_POINT('Ctrl Pts',(-14.0076725609536,-70.6431290668744,
12.));
#132723=CARTESIAN_POINT('Ctrl Pts',(-14.020178372077,-70.6637105182487,
12.));
#132724=CARTESIAN_POINT('Ctrl Pts',(-14.0327261372363,-70.6843157607672,
12.));
#132725=CARTESIAN_POINT('Ctrl Pts',(-14.0453158466451,-70.7049446620931,
12.));
#132726=CARTESIAN_POINT('Ctrl Pts',(-14.0579474904657,-70.7255970904433,
12.));
#132727=CARTESIAN_POINT('Ctrl Pts',(-14.0706210588015,-70.7462729145799,
12.));
#132728=CARTESIAN_POINT('Ctrl Pts',(-14.0833365416995,-70.7669720038067,
12.));
#132729=CARTESIAN_POINT('Ctrl Pts',(-14.0960939291568,-70.787694227969,
12.));
#132730=CARTESIAN_POINT('Ctrl Pts',(-14.1088932111214,-70.8084394574491,
12.));
#132731=CARTESIAN_POINT('Ctrl Pts',(-14.1217343774914,-70.8292075631624,
12.));
#132732=CARTESIAN_POINT('Ctrl Pts',(-14.1346174181079,-70.8499984165493,
12.));
#132733=CARTESIAN_POINT('Ctrl Pts',(-14.1475423227567,-70.8708118895718,
12.));
#132734=CARTESIAN_POINT('Ctrl Pts',(-14.1605090811753,-70.8916478547131,
12.));
#132735=CARTESIAN_POINT('Ctrl Pts',(-14.1735176830533,-70.9125061849744,
12.));
#132736=CARTESIAN_POINT('Ctrl Pts',(-14.1865681180321,-70.9333867538705,
12.));
#132737=CARTESIAN_POINT('Ctrl Pts',(-14.1996603756984,-70.9542894354221,
12.));
#132738=CARTESIAN_POINT('Ctrl Pts',(-14.2127944455841,-70.9752141041527,
12.));
#132739=CARTESIAN_POINT('Ctrl Pts',(-14.2259703171739,-70.996160635087,
12.));
#132740=CARTESIAN_POINT('Ctrl Pts',(-14.2391879799063,-71.0171289037493,
12.));
#132741=CARTESIAN_POINT('Ctrl Pts',(-14.2524474231732,-71.0381187861585,
12.));
#132742=CARTESIAN_POINT('Ctrl Pts',(-14.2657486363136,-71.059130158822,
12.));
#132743=CARTESIAN_POINT('Ctrl Pts',(-14.2790916086129,-71.0801628987314,
12.));
#132744=CARTESIAN_POINT('Ctrl Pts',(-14.2924763293101,-71.1012168833626,
12.));
#132745=CARTESIAN_POINT('Ctrl Pts',(-14.3059027875992,-71.1222919906718,
12.));
#132746=CARTESIAN_POINT('Ctrl Pts',(-14.3193709726295,-71.1433880990932,
12.));
#132747=CARTESIAN_POINT('Ctrl Pts',(-14.3328808734993,-71.1645050875323,
12.));
#132748=CARTESIAN_POINT('Ctrl Pts',(-14.3464324792537,-71.185642835361,
12.));
#132749=CARTESIAN_POINT('Ctrl Pts',(-14.3600257788927,-71.2068012224187,
12.));
#132750=CARTESIAN_POINT('Ctrl Pts',(-14.3736607613723,-71.2279801290088,
12.));
#132751=CARTESIAN_POINT('Ctrl Pts',(-14.3873374156056,-71.2491794358956,
12.));
#132752=CARTESIAN_POINT('Ctrl Pts',(-14.401055730457,-71.2703990242986,
12.));
#132753=CARTESIAN_POINT('Ctrl Pts',(-14.4148156947384,-71.2916387758864,
12.));
#132754=CARTESIAN_POINT('Ctrl Pts',(-14.4286172972168,-71.3128985727777,
12.));
#132755=CARTESIAN_POINT('Ctrl Pts',(-14.4424605266166,-71.3341782975393,
12.));
#132756=CARTESIAN_POINT('Ctrl Pts',(-14.4563453716204,-71.3554778331835,
12.));
#132757=CARTESIAN_POINT('Ctrl Pts',(-14.470271820865,-71.3767970631642,
12.));
#132758=CARTESIAN_POINT('Ctrl Pts',(-14.4842398629353,-71.398135871371,
12.));
#132759=CARTESIAN_POINT('Ctrl Pts',(-14.4982494863716,-71.4194941421279,
12.));
#132760=CARTESIAN_POINT('Ctrl Pts',(-14.5123006796728,-71.4408717601917,
12.));
#132761=CARTESIAN_POINT('Ctrl Pts',(-14.5263934312969,-71.4622686107475,
12.));
#132762=CARTESIAN_POINT('Ctrl Pts',(-14.540527729659,-71.4836845794052,
12.));
#132763=CARTESIAN_POINT('Ctrl Pts',(-14.5547035631233,-71.5051195521914,
12.));
#132764=CARTESIAN_POINT('Ctrl Pts',(-14.568920920009,-71.52657341555,12.));
#132765=CARTESIAN_POINT('Ctrl Pts',(-14.5831797885951,-71.5480460563445,
12.));
#132766=CARTESIAN_POINT('Ctrl Pts',(-14.5974801571209,-71.569537361856,
12.));
#132767=CARTESIAN_POINT('Ctrl Pts',(-14.611822013785,-71.5910472197815,
12.));
#132768=CARTESIAN_POINT('Ctrl Pts',(-14.6262053467372,-71.6125755182295,
12.));
#132769=CARTESIAN_POINT('Ctrl Pts',(-14.6406301440817,-71.6341221457175,
12.));
#132770=CARTESIAN_POINT('Ctrl Pts',(-14.6550963938832,-71.6556869911669,
12.));
#132771=CARTESIAN_POINT('Ctrl Pts',(-14.6696040841679,-71.6772699438966,
12.));
#132772=CARTESIAN_POINT('Ctrl Pts',(-14.6841532029231,-71.698870893617,
12.));
#132773=CARTESIAN_POINT('Ctrl Pts',(-14.6987437380898,-71.7204897304186,
12.));
#132774=CARTESIAN_POINT('Ctrl Pts',(-14.7133756775622,-71.7421263447707,
12.));
#132775=CARTESIAN_POINT('Ctrl Pts',(-14.7280490091954,-71.7637806275316,
12.));
#132776=CARTESIAN_POINT('Ctrl Pts',(-14.742763720807,-71.7854524699563,
12.));
#132777=CARTESIAN_POINT('Ctrl Pts',(-14.7575198001776,-71.8071417637019,
12.));
#132778=CARTESIAN_POINT('Ctrl Pts',(-14.7723172350454,-71.8288484008343,
12.));
#132779=CARTESIAN_POINT('Ctrl Pts',(-14.7871560131021,-71.8505722738286,
12.));
#132780=CARTESIAN_POINT('Ctrl Pts',(-14.8020361220002,-71.872313275546,
12.));
#132781=CARTESIAN_POINT('Ctrl Pts',(-14.8169575493559,-71.8940712992119,
12.));
#132782=CARTESIAN_POINT('Ctrl Pts',(-14.8319202827482,-71.9158462383915,
12.));
#132783=CARTESIAN_POINT('Ctrl Pts',(-14.846924309716,-71.9376379869668,
12.));
#132784=CARTESIAN_POINT('Ctrl Pts',(-14.8619696177503,-71.9594464391063,
12.));
#132785=CARTESIAN_POINT('Ctrl Pts',(-14.8770561943011,-71.9812714893087,
12.));
#132786=CARTESIAN_POINT('Ctrl Pts',(-14.8921840267829,-72.0031130324519,
12.));
#132787=CARTESIAN_POINT('Ctrl Pts',(-14.9073531025763,-72.0249709638419,
12.));
#132788=CARTESIAN_POINT('Ctrl Pts',(-14.9225634090269,-72.046845179251,
12.));
#132789=CARTESIAN_POINT('Ctrl Pts',(-14.937814933439,-72.0687355749815,
12.));
#132790=CARTESIAN_POINT('Ctrl Pts',(-14.953107663077,-72.0906420478085,
12.));
#132791=CARTESIAN_POINT('Ctrl Pts',(-14.9684415851699,-72.1125644948547,
12.));
#132792=CARTESIAN_POINT('Ctrl Pts',(-14.9838166869107,-72.1345028134779,
12.));
#132793=CARTESIAN_POINT('Ctrl Pts',(-14.9992329554537,-72.1564569011668,
12.));
#132794=CARTESIAN_POINT('Ctrl Pts',(-15.0146903779061,-72.1784266553948,
12.));
#132795=CARTESIAN_POINT('Ctrl Pts',(-15.0301889413255,-72.2004119736104,
12.));
#132796=CARTESIAN_POINT('Ctrl Pts',(-15.0457286327328,-72.2224127535401,
12.));
#132797=CARTESIAN_POINT('Ctrl Pts',(-15.0613094391186,-72.244428893425,
12.));
#132798=CARTESIAN_POINT('Ctrl Pts',(-15.0769313474476,-72.266460292285,
12.));
#132799=CARTESIAN_POINT('Ctrl Pts',(-15.0925943446593,-72.2885068501641,
12.));
#132800=CARTESIAN_POINT('Ctrl Pts',(-15.1082984176655,-72.3105684683971,
12.));
#132801=CARTESIAN_POINT('Ctrl Pts',(-15.1240435533478,-72.332645049021,
12.));
#132802=CARTESIAN_POINT('Ctrl Pts',(-15.1398297385513,-72.3547364941996,
12.));
#132803=CARTESIAN_POINT('Ctrl Pts',(-15.1556569600747,-72.37684270559,12.));
#132804=CARTESIAN_POINT('Ctrl Pts',(-15.1715252046602,-72.3989635838476,
12.));
#132805=CARTESIAN_POINT('Ctrl Pts',(-15.1874344589715,-72.4210990277819,
12.));
#132806=CARTESIAN_POINT('Ctrl Pts',(-15.2033847096077,-72.4432489350415,
12.));
#132807=CARTESIAN_POINT('Ctrl Pts',(-15.2193759431359,-72.4654132036373,
12.));
#132808=CARTESIAN_POINT('Ctrl Pts',(-15.2354081461151,-72.4875917332729,
12.));
#132809=CARTESIAN_POINT('Ctrl Pts',(-15.2514813051174,-72.5097844266083,
12.));
#132810=CARTESIAN_POINT('Ctrl Pts',(-15.2675954067495,-72.5319911908978,
12.));
#132811=CARTESIAN_POINT('Ctrl Pts',(-15.2837504376562,-72.5542119383748,
12.));
#132812=CARTESIAN_POINT('Ctrl Pts',(-15.2976335024853,-72.5732713370796,
12.));
#132813=CARTESIAN_POINT('Ctrl Pts',(-15.3082994603652,-72.5878912620663,
12.));
#132814=CARTESIAN_POINT('Ctrl Pts',(-15.3157301930832,-72.5980655789898,
12.));
#132815=CARTESIAN_POINT('Ctrl Pts',(-15.3199137230319,-72.6037902605228,
12.));
#132816=CARTESIAN_POINT('Ctrl Pts',(-15.3208442077421,-72.6050633494713,
12.));
#132817=CARTESIAN_POINT('',(-12.9953224629497,-68.7831490561748,0.));
#132818=CARTESIAN_POINT('',(-12.9953224629497,-68.7831490561748,0.));
#132819=CARTESIAN_POINT('Ctrl Pts',(-15.3208442077421,-72.6050633494713,
0.));
#132820=CARTESIAN_POINT('Ctrl Pts',(-15.3199137230319,-72.6037902605228,
0.));
#132821=CARTESIAN_POINT('Ctrl Pts',(-15.3157301930832,-72.5980655789898,
0.));
#132822=CARTESIAN_POINT('Ctrl Pts',(-15.3082994603652,-72.5878912620663,
0.));
#132823=CARTESIAN_POINT('Ctrl Pts',(-15.2976335024853,-72.5732713370796,
0.));
#132824=CARTESIAN_POINT('Ctrl Pts',(-15.2837504376562,-72.5542119383748,
0.));
#132825=CARTESIAN_POINT('Ctrl Pts',(-15.2675954067495,-72.5319911908978,
0.));
#132826=CARTESIAN_POINT('Ctrl Pts',(-15.2514813051174,-72.5097844266083,
0.));
#132827=CARTESIAN_POINT('Ctrl Pts',(-15.2354081461151,-72.4875917332729,
0.));
#132828=CARTESIAN_POINT('Ctrl Pts',(-15.2193759431359,-72.4654132036373,
0.));
#132829=CARTESIAN_POINT('Ctrl Pts',(-15.2033847096077,-72.4432489350415,
0.));
#132830=CARTESIAN_POINT('Ctrl Pts',(-15.1874344589715,-72.4210990277819,
0.));
#132831=CARTESIAN_POINT('Ctrl Pts',(-15.1715252046602,-72.3989635838476,
0.));
#132832=CARTESIAN_POINT('Ctrl Pts',(-15.1556569600747,-72.37684270559,0.));
#132833=CARTESIAN_POINT('Ctrl Pts',(-15.1398297385513,-72.3547364941996,
0.));
#132834=CARTESIAN_POINT('Ctrl Pts',(-15.1240435533478,-72.332645049021,
0.));
#132835=CARTESIAN_POINT('Ctrl Pts',(-15.1082984176655,-72.3105684683971,
0.));
#132836=CARTESIAN_POINT('Ctrl Pts',(-15.0925943446593,-72.2885068501641,
0.));
#132837=CARTESIAN_POINT('Ctrl Pts',(-15.0769313474476,-72.266460292285,
0.));
#132838=CARTESIAN_POINT('Ctrl Pts',(-15.0613094391186,-72.244428893425,
0.));
#132839=CARTESIAN_POINT('Ctrl Pts',(-15.0457286327328,-72.2224127535401,
0.));
#132840=CARTESIAN_POINT('Ctrl Pts',(-15.0301889413255,-72.2004119736104,
0.));
#132841=CARTESIAN_POINT('Ctrl Pts',(-15.0146903779061,-72.1784266553948,
0.));
#132842=CARTESIAN_POINT('Ctrl Pts',(-14.9992329554537,-72.1564569011668,
0.));
#132843=CARTESIAN_POINT('Ctrl Pts',(-14.9838166869107,-72.1345028134779,
0.));
#132844=CARTESIAN_POINT('Ctrl Pts',(-14.9684415851699,-72.1125644948547,
0.));
#132845=CARTESIAN_POINT('Ctrl Pts',(-14.953107663077,-72.0906420478085,
0.));
#132846=CARTESIAN_POINT('Ctrl Pts',(-14.937814933439,-72.0687355749815,
0.));
#132847=CARTESIAN_POINT('Ctrl Pts',(-14.9225634090269,-72.046845179251,
0.));
#132848=CARTESIAN_POINT('Ctrl Pts',(-14.9073531025763,-72.0249709638419,
0.));
#132849=CARTESIAN_POINT('Ctrl Pts',(-14.8921840267829,-72.0031130324519,
0.));
#132850=CARTESIAN_POINT('Ctrl Pts',(-14.8770561943011,-71.9812714893087,
0.));
#132851=CARTESIAN_POINT('Ctrl Pts',(-14.8619696177503,-71.9594464391063,
0.));
#132852=CARTESIAN_POINT('Ctrl Pts',(-14.846924309716,-71.9376379869668,
0.));
#132853=CARTESIAN_POINT('Ctrl Pts',(-14.8319202827482,-71.9158462383915,
0.));
#132854=CARTESIAN_POINT('Ctrl Pts',(-14.8169575493559,-71.8940712992119,
0.));
#132855=CARTESIAN_POINT('Ctrl Pts',(-14.8020361220002,-71.872313275546,
0.));
#132856=CARTESIAN_POINT('Ctrl Pts',(-14.7871560131021,-71.8505722738286,
0.));
#132857=CARTESIAN_POINT('Ctrl Pts',(-14.7723172350454,-71.8288484008343,
0.));
#132858=CARTESIAN_POINT('Ctrl Pts',(-14.7575198001776,-71.8071417637019,
0.));
#132859=CARTESIAN_POINT('Ctrl Pts',(-14.742763720807,-71.7854524699563,
0.));
#132860=CARTESIAN_POINT('Ctrl Pts',(-14.7280490091954,-71.7637806275316,
0.));
#132861=CARTESIAN_POINT('Ctrl Pts',(-14.7133756775622,-71.7421263447707,
0.));
#132862=CARTESIAN_POINT('Ctrl Pts',(-14.6987437380898,-71.7204897304186,
0.));
#132863=CARTESIAN_POINT('Ctrl Pts',(-14.6841532029231,-71.698870893617,
0.));
#132864=CARTESIAN_POINT('Ctrl Pts',(-14.6696040841679,-71.6772699438966,
0.));
#132865=CARTESIAN_POINT('Ctrl Pts',(-14.6550963938832,-71.6556869911669,
0.));
#132866=CARTESIAN_POINT('Ctrl Pts',(-14.6406301440817,-71.6341221457175,
0.));
#132867=CARTESIAN_POINT('Ctrl Pts',(-14.6262053467372,-71.6125755182295,
0.));
#132868=CARTESIAN_POINT('Ctrl Pts',(-14.611822013785,-71.5910472197815,
0.));
#132869=CARTESIAN_POINT('Ctrl Pts',(-14.5974801571209,-71.569537361856,
0.));
#132870=CARTESIAN_POINT('Ctrl Pts',(-14.5831797885951,-71.5480460563445,
0.));
#132871=CARTESIAN_POINT('Ctrl Pts',(-14.568920920009,-71.52657341555,0.));
#132872=CARTESIAN_POINT('Ctrl Pts',(-14.5547035631233,-71.5051195521914,
0.));
#132873=CARTESIAN_POINT('Ctrl Pts',(-14.540527729659,-71.4836845794052,
0.));
#132874=CARTESIAN_POINT('Ctrl Pts',(-14.5263934312969,-71.4622686107475,
0.));
#132875=CARTESIAN_POINT('Ctrl Pts',(-14.5123006796728,-71.4408717601917,
0.));
#132876=CARTESIAN_POINT('Ctrl Pts',(-14.4982494863716,-71.4194941421279,
0.));
#132877=CARTESIAN_POINT('Ctrl Pts',(-14.4842398629353,-71.398135871371,
0.));
#132878=CARTESIAN_POINT('Ctrl Pts',(-14.470271820865,-71.3767970631642,
0.));
#132879=CARTESIAN_POINT('Ctrl Pts',(-14.4563453716204,-71.3554778331835,
0.));
#132880=CARTESIAN_POINT('Ctrl Pts',(-14.4424605266166,-71.3341782975393,
0.));
#132881=CARTESIAN_POINT('Ctrl Pts',(-14.4286172972168,-71.3128985727777,
0.));
#132882=CARTESIAN_POINT('Ctrl Pts',(-14.4148156947384,-71.2916387758864,
0.));
#132883=CARTESIAN_POINT('Ctrl Pts',(-14.401055730457,-71.2703990242986,
0.));
#132884=CARTESIAN_POINT('Ctrl Pts',(-14.3873374156056,-71.2491794358956,
0.));
#132885=CARTESIAN_POINT('Ctrl Pts',(-14.3736607613723,-71.2279801290088,
0.));
#132886=CARTESIAN_POINT('Ctrl Pts',(-14.3600257788927,-71.2068012224187,
0.));
#132887=CARTESIAN_POINT('Ctrl Pts',(-14.3464324792537,-71.185642835361,
0.));
#132888=CARTESIAN_POINT('Ctrl Pts',(-14.3328808734993,-71.1645050875323,
0.));
#132889=CARTESIAN_POINT('Ctrl Pts',(-14.3193709726295,-71.1433880990932,
0.));
#132890=CARTESIAN_POINT('Ctrl Pts',(-14.3059027875992,-71.1222919906718,
0.));
#132891=CARTESIAN_POINT('Ctrl Pts',(-14.2924763293101,-71.1012168833626,
0.));
#132892=CARTESIAN_POINT('Ctrl Pts',(-14.2790916086129,-71.0801628987314,
0.));
#132893=CARTESIAN_POINT('Ctrl Pts',(-14.2657486363136,-71.059130158822,
0.));
#132894=CARTESIAN_POINT('Ctrl Pts',(-14.2524474231732,-71.0381187861585,
0.));
#132895=CARTESIAN_POINT('Ctrl Pts',(-14.2391879799063,-71.0171289037493,
0.));
#132896=CARTESIAN_POINT('Ctrl Pts',(-14.2259703171739,-70.996160635087,
0.));
#132897=CARTESIAN_POINT('Ctrl Pts',(-14.2127944455841,-70.9752141041527,
0.));
#132898=CARTESIAN_POINT('Ctrl Pts',(-14.1996603756984,-70.9542894354221,
0.));
#132899=CARTESIAN_POINT('Ctrl Pts',(-14.1865681180321,-70.9333867538705,
0.));
#132900=CARTESIAN_POINT('Ctrl Pts',(-14.1735176830533,-70.9125061849744,
0.));
#132901=CARTESIAN_POINT('Ctrl Pts',(-14.1605090811753,-70.8916478547131,
0.));
#132902=CARTESIAN_POINT('Ctrl Pts',(-14.1475423227567,-70.8708118895718,
0.));
#132903=CARTESIAN_POINT('Ctrl Pts',(-14.1346174181079,-70.8499984165493,
0.));
#132904=CARTESIAN_POINT('Ctrl Pts',(-14.1217343774914,-70.8292075631624,
0.));
#132905=CARTESIAN_POINT('Ctrl Pts',(-14.1088932111214,-70.8084394574491,
0.));
#132906=CARTESIAN_POINT('Ctrl Pts',(-14.0960939291568,-70.787694227969,
0.));
#132907=CARTESIAN_POINT('Ctrl Pts',(-14.0833365416995,-70.7669720038067,
0.));
#132908=CARTESIAN_POINT('Ctrl Pts',(-14.0706210588015,-70.7462729145799,
0.));
#132909=CARTESIAN_POINT('Ctrl Pts',(-14.0579474904657,-70.7255970904433,
0.));
#132910=CARTESIAN_POINT('Ctrl Pts',(-14.0453158466451,-70.7049446620931,
0.));
#132911=CARTESIAN_POINT('Ctrl Pts',(-14.0327261372363,-70.6843157607672,
0.));
#132912=CARTESIAN_POINT('Ctrl Pts',(-14.020178372077,-70.6637105182487,
0.));
#132913=CARTESIAN_POINT('Ctrl Pts',(-14.0076725609536,-70.6431290668744,
0.));
#132914=CARTESIAN_POINT('Ctrl Pts',(-13.9952087136018,-70.6225715395392,
0.));
#132915=CARTESIAN_POINT('Ctrl Pts',(-13.9827868397057,-70.6020380697004,
0.));
#132916=CARTESIAN_POINT('Ctrl Pts',(-13.9704069488918,-70.5815287913791,
0.));
#132917=CARTESIAN_POINT('Ctrl Pts',(-13.9580690507262,-70.5610438391622,
0.));
#132918=CARTESIAN_POINT('Ctrl Pts',(-13.9457731547217,-70.5405833482123,
0.));
#132919=CARTESIAN_POINT('Ctrl Pts',(-13.9335192703389,-70.5201474542717,
0.));
#132920=CARTESIAN_POINT('Ctrl Pts',(-13.9213074069852,-70.4997362936671,
0.));
#132921=CARTESIAN_POINT('Ctrl Pts',(-13.9091375740084,-70.4793500033106,
0.));
#132922=CARTESIAN_POINT('Ctrl Pts',(-13.8970097806947,-70.4589887207043,
0.));
#132923=CARTESIAN_POINT('Ctrl Pts',(-13.8849240362757,-70.4386525839492,
0.));
#132924=CARTESIAN_POINT('Ctrl Pts',(-13.8728803499284,-70.4183417317486,
0.));
#132925=CARTESIAN_POINT('Ctrl Pts',(-13.8608787307753,-70.3980563034142,
0.));
#132926=CARTESIAN_POINT('Ctrl Pts',(-13.8489191878774,-70.377796438866,
0.));
#132927=CARTESIAN_POINT('Ctrl Pts',(-13.8370017302318,-70.3575622786373,
0.));
#132928=CARTESIAN_POINT('Ctrl Pts',(-13.8251263667799,-70.3373539638841,
0.));
#132929=CARTESIAN_POINT('Ctrl Pts',(-13.8132931064067,-70.3171716363912,
0.));
#132930=CARTESIAN_POINT('Ctrl Pts',(-13.8015019579411,-70.2970154385763,
0.));
#132931=CARTESIAN_POINT('Ctrl Pts',(-13.7897529301482,-70.2768855134909,
0.));
#132932=CARTESIAN_POINT('Ctrl Pts',(-13.7780460317284,-70.2567820048253,
0.));
#132933=CARTESIAN_POINT('Ctrl Pts',(-13.7663812713235,-70.2367050569174,
0.));
#132934=CARTESIAN_POINT('Ctrl Pts',(-13.7547586575178,-70.216654814759,
0.));
#132935=CARTESIAN_POINT('Ctrl Pts',(-13.7431781988368,-70.1966314240012,
0.));
#132936=CARTESIAN_POINT('Ctrl Pts',(-13.73163990374,-70.1766350309554,0.));
#132937=CARTESIAN_POINT('Ctrl Pts',(-13.7201437806207,-70.1566657825989,
0.));
#132938=CARTESIAN_POINT('Ctrl Pts',(-13.7086898378127,-70.1367238265853,
0.));
#132939=CARTESIAN_POINT('Ctrl Pts',(-13.6972780835898,-70.1168093112493,
0.));
#132940=CARTESIAN_POINT('Ctrl Pts',(-13.685908526165,-70.0969223856123,
0.));
#132941=CARTESIAN_POINT('Ctrl Pts',(-13.6745811736825,-70.0770631993831,
0.));
#132942=CARTESIAN_POINT('Ctrl Pts',(-13.6632960342192,-70.057231902965,
0.));
#132943=CARTESIAN_POINT('Ctrl Pts',(-13.6520531157904,-70.037428647466,
0.));
#132944=CARTESIAN_POINT('Ctrl Pts',(-13.6408524263496,-70.0176535847047,
0.));
#132945=CARTESIAN_POINT('Ctrl Pts',(-13.6296939737866,-69.9979068672163,
0.));
#132946=CARTESIAN_POINT('Ctrl Pts',(-13.61857776592,-69.9781886482543,0.));
#132947=CARTESIAN_POINT('Ctrl Pts',(-13.6075038105,-69.9584990817989,0.));
#132948=CARTESIAN_POINT('Ctrl Pts',(-13.5964721152136,-69.9388383225655,
0.));
#132949=CARTESIAN_POINT('Ctrl Pts',(-13.5854826876834,-69.9192065260107,
0.));
#132950=CARTESIAN_POINT('Ctrl Pts',(-13.5745355354657,-69.899603848336,
0.));
#132951=CARTESIAN_POINT('Ctrl Pts',(-13.5636306660422,-69.880030446488,
0.));
#132952=CARTESIAN_POINT('Ctrl Pts',(-13.5527680868256,-69.8604864781705,
0.));
#132953=CARTESIAN_POINT('Ctrl Pts',(-13.5419478051626,-69.840972101856,
0.));
#132954=CARTESIAN_POINT('Ctrl Pts',(-13.5311698283339,-69.8214874767944,
0.));
#132955=CARTESIAN_POINT('Ctrl Pts',(-13.5204341635507,-69.8020327630204,
0.));
#132956=CARTESIAN_POINT('Ctrl Pts',(-13.5097408179478,-69.7826081213575,
0.));
#132957=CARTESIAN_POINT('Ctrl Pts',(-13.4990897985903,-69.7632137134247,
0.));
#132958=CARTESIAN_POINT('Ctrl Pts',(-13.4884811124748,-69.7438497016404,
0.));
#132959=CARTESIAN_POINT('Ctrl Pts',(-13.4779147665285,-69.7245162492251,
0.));
#132960=CARTESIAN_POINT('Ctrl Pts',(-13.4673907676045,-69.7052135202003,
0.));
#132961=CARTESIAN_POINT('Ctrl Pts',(-13.4569091224762,-69.6859416793898,
0.));
#132962=CARTESIAN_POINT('Ctrl Pts',(-13.4464698378456,-69.6667008924454,
0.));
#132963=CARTESIAN_POINT('Ctrl Pts',(-13.4360729203444,-69.6474913258684,
0.));
#132964=CARTESIAN_POINT('Ctrl Pts',(-13.425718376534,-69.6283131470267,
0.));
#132965=CARTESIAN_POINT('Ctrl Pts',(-13.4154062128998,-69.6091665241743,
0.));
#132966=CARTESIAN_POINT('Ctrl Pts',(-13.4051364358494,-69.5900516264524,
0.));
#132967=CARTESIAN_POINT('Ctrl Pts',(-13.3949090517173,-69.5709686238701,
0.));
#132968=CARTESIAN_POINT('Ctrl Pts',(-13.3847240667626,-69.5519176872857,
0.));
#132969=CARTESIAN_POINT('Ctrl Pts',(-13.3745814871667,-69.5328989883899,
0.));
#132970=CARTESIAN_POINT('Ctrl Pts',(-13.3644813190225,-69.5139126996703,
0.));
#132971=CARTESIAN_POINT('Ctrl Pts',(-13.3544235683399,-69.4949589944633,
0.));
#132972=CARTESIAN_POINT('Ctrl Pts',(-13.3444082410546,-69.4760380470382,
0.));
#132973=CARTESIAN_POINT('Ctrl Pts',(-13.3344353430313,-69.4571500326673,
0.));
#132974=CARTESIAN_POINT('Ctrl Pts',(-13.3245048800641,-69.4382951276983,
0.));
#132975=CARTESIAN_POINT('Ctrl Pts',(-13.3146168578738,-69.4194735096238,
0.));
#132976=CARTESIAN_POINT('Ctrl Pts',(-13.3047712821046,-69.4006853569485,
0.));
#132977=CARTESIAN_POINT('Ctrl Pts',(-13.2949681583164,-69.3819308490408,
0.));
#132978=CARTESIAN_POINT('Ctrl Pts',(-13.2852074919767,-69.3632101660072,
0.));
#132979=CARTESIAN_POINT('Ctrl Pts',(-13.2754892884437,-69.3445234885088,
0.));
#132980=CARTESIAN_POINT('Ctrl Pts',(-13.2658135529616,-69.3258709977416,
0.));
#132981=CARTESIAN_POINT('Ctrl Pts',(-13.2561802906901,-69.3072528758546,
0.));
#132982=CARTESIAN_POINT('Ctrl Pts',(-13.2465895067264,-69.2886693063193,
0.));
#132983=CARTESIAN_POINT('Ctrl Pts',(-13.2370412061218,-69.2701204742436,
0.));
#132984=CARTESIAN_POINT('Ctrl Pts',(-13.2275353939044,-69.2516065668809,
0.));
#132985=CARTESIAN_POINT('Ctrl Pts',(-13.2180720750585,-69.2331277732819,
0.));
#132986=CARTESIAN_POINT('Ctrl Pts',(-13.2086512544729,-69.2146842833506,
0.));
#132987=CARTESIAN_POINT('Ctrl Pts',(-13.1992729368928,-69.1962762870524,
0.));
#132988=CARTESIAN_POINT('Ctrl Pts',(-13.1899371268689,-69.1779039736026,
0.));
#132989=CARTESIAN_POINT('Ctrl Pts',(-13.1806438286944,-69.1595675305294,
0.));
#132990=CARTESIAN_POINT('Ctrl Pts',(-13.1713930465142,-69.141267145461,
0.));
#132991=CARTESIAN_POINT('Ctrl Pts',(-13.1621847844533,-69.1230030082597,
0.));
#132992=CARTESIAN_POINT('Ctrl Pts',(-13.1530190467181,-69.1047753127633,
0.));
#132993=CARTESIAN_POINT('Ctrl Pts',(-13.1438958377397,-69.0865842593063,
0.));
#132994=CARTESIAN_POINT('Ctrl Pts',(-13.1348151621824,-69.0684300549426,
0.));
#132995=CARTESIAN_POINT('Ctrl Pts',(-13.1257770246378,-69.0503129081778,
0.));
#132996=CARTESIAN_POINT('Ctrl Pts',(-13.1167814293495,-69.0322330243336,
0.));
#132997=CARTESIAN_POINT('Ctrl Pts',(-13.1078283799726,-69.0141906015137,
0.));
#132998=CARTESIAN_POINT('Ctrl Pts',(-13.0989178791843,-68.9961858241577,
0.));
#132999=CARTESIAN_POINT('Ctrl Pts',(-13.0900499290541,-68.9782188692654,
0.));
#133000=CARTESIAN_POINT('Ctrl Pts',(-13.0812245317816,-68.9602899187628,
0.));
#133001=CARTESIAN_POINT('Ctrl Pts',(-13.072441690283,-68.9423991694493,
0.));
#133002=CARTESIAN_POINT('Ctrl Pts',(-13.0637014089018,-68.9245468449865,
0.));
#133003=CARTESIAN_POINT('Ctrl Pts',(-13.0550036938793,-68.9067332040842,
0.));
#133004=CARTESIAN_POINT('Ctrl Pts',(-13.0463485518185,-68.8889585151431,
0.));
#133005=CARTESIAN_POINT('Ctrl Pts',(-13.0377359881863,-68.8712230321823,
0.));
#133006=CARTESIAN_POINT('Ctrl Pts',(-13.0291660060118,-68.8535269726871,
0.));
#133007=CARTESIAN_POINT('Ctrl Pts',(-13.0206386039729,-68.835870488774,
0.));
#133008=CARTESIAN_POINT('Ctrl Pts',(-13.0121537769003,-68.8182536654067,
0.));
#133009=CARTESIAN_POINT('Ctrl Pts',(-13.0053999700929,-68.8041919669403,
0.));
#133010=CARTESIAN_POINT('Ctrl Pts',(-13.0003537683089,-68.7936635625788,
0.));
#133011=CARTESIAN_POINT('Ctrl Pts',(-12.996998146029,-68.7866525680284,
0.));
#133012=CARTESIAN_POINT('Ctrl Pts',(-12.9953224629497,-68.7831490561748,
0.));
#133013=CARTESIAN_POINT('Ctrl Pts',(-21.8059378310719,-71.2372871136136,
0.));
#133014=CARTESIAN_POINT('Ctrl Pts',(-21.8059378310719,-71.2372871136136,
12.));
#133015=CARTESIAN_POINT('Ctrl Pts',(-21.8022104901727,-71.2331134397872,
0.));
#133016=CARTESIAN_POINT('Ctrl Pts',(-21.8022104901727,-71.2331134397872,
12.));
#133017=CARTESIAN_POINT('Ctrl Pts',(-21.7947599798961,-71.2247670210176,
0.));
#133018=CARTESIAN_POINT('Ctrl Pts',(-21.7947599798961,-71.2247670210176,
12.));
#133019=CARTESIAN_POINT('Ctrl Pts',(-21.7835967290463,-71.2122501795138,
0.));
#133020=CARTESIAN_POINT('Ctrl Pts',(-21.7835967290463,-71.2122501795138,
12.));
#133021=CARTESIAN_POINT('Ctrl Pts',(-21.7687374247288,-71.1955666310295,
0.));
#133022=CARTESIAN_POINT('Ctrl Pts',(-21.7687374247288,-71.1955666310295,
12.));
#133023=CARTESIAN_POINT('Ctrl Pts',(-21.750205018381,-71.1747214906585,
0.));
#133024=CARTESIAN_POINT('Ctrl Pts',(-21.750205018381,-71.1747214906585,
12.));
#133025=CARTESIAN_POINT('Ctrl Pts',(-21.7317143472952,-71.1538856612261,
0.));
#133026=CARTESIAN_POINT('Ctrl Pts',(-21.7317143472952,-71.1538856612261,
12.));
#133027=CARTESIAN_POINT('Ctrl Pts',(-21.7132654262531,-71.1330591726506,
0.));
#133028=CARTESIAN_POINT('Ctrl Pts',(-21.7132654262531,-71.1330591726506,
12.));
#133029=CARTESIAN_POINT('Ctrl Pts',(-21.694858273085,-71.1122420728217,
0.));
#133030=CARTESIAN_POINT('Ctrl Pts',(-21.694858273085,-71.1122420728217,
12.));
#133031=CARTESIAN_POINT('Ctrl Pts',(-21.6764929081677,-71.0914344332798,
0.));
#133032=CARTESIAN_POINT('Ctrl Pts',(-21.6764929081677,-71.0914344332798,
12.));
#133033=CARTESIAN_POINT('Ctrl Pts',(-21.6581693538335,-71.0706363472704,
0.));
#133034=CARTESIAN_POINT('Ctrl Pts',(-21.6581693538335,-71.0706363472704,
12.));
#133035=CARTESIAN_POINT('Ctrl Pts',(-21.6398876337141,-71.0498479219467,
0.));
#133036=CARTESIAN_POINT('Ctrl Pts',(-21.6398876337141,-71.0498479219467,
12.));
#133037=CARTESIAN_POINT('Ctrl Pts',(-21.6216477720913,-71.0290692721847,
0.));
#133038=CARTESIAN_POINT('Ctrl Pts',(-21.6216477720913,-71.0290692721847,
12.));
#133039=CARTESIAN_POINT('Ctrl Pts',(-21.6034497932581,-71.0083005139107,
0.));
#133040=CARTESIAN_POINT('Ctrl Pts',(-21.6034497932581,-71.0083005139107,
12.));
#133041=CARTESIAN_POINT('Ctrl Pts',(-21.585293720829,-70.987541757223,0.));
#133042=CARTESIAN_POINT('Ctrl Pts',(-21.585293720829,-70.987541757223,12.));
#133043=CARTESIAN_POINT('Ctrl Pts',(-21.5671795771914,-70.9667931008215,
0.));
#133044=CARTESIAN_POINT('Ctrl Pts',(-21.5671795771914,-70.9667931008215,
12.));
#133045=CARTESIAN_POINT('Ctrl Pts',(-21.5491073839106,-70.94605463587,0.));
#133046=CARTESIAN_POINT('Ctrl Pts',(-21.5491073839106,-70.94605463587,12.));
#133047=CARTESIAN_POINT('Ctrl Pts',(-21.5310771620231,-70.9253264487636,
0.));
#133048=CARTESIAN_POINT('Ctrl Pts',(-21.5310771620231,-70.9253264487636,
12.));
#133049=CARTESIAN_POINT('Ctrl Pts',(-21.513088932377,-70.9046086244131,
0.));
#133050=CARTESIAN_POINT('Ctrl Pts',(-21.513088932377,-70.9046086244131,
12.));
#133051=CARTESIAN_POINT('Ctrl Pts',(-21.4951427159262,-70.8839012490871,
0.));
#133052=CARTESIAN_POINT('Ctrl Pts',(-21.4951427159262,-70.8839012490871,
12.));
#133053=CARTESIAN_POINT('Ctrl Pts',(-21.477238534096,-70.8632044140112,
0.));
#133054=CARTESIAN_POINT('Ctrl Pts',(-21.477238534096,-70.8632044140112,
12.));
#133055=CARTESIAN_POINT('Ctrl Pts',(-21.4593764087474,-70.8425182149846,
0.));
#133056=CARTESIAN_POINT('Ctrl Pts',(-21.4593764087474,-70.8425182149846,
12.));
#133057=CARTESIAN_POINT('Ctrl Pts',(-21.4415563620114,-70.8218427507506,
0.));
#133058=CARTESIAN_POINT('Ctrl Pts',(-21.4415563620114,-70.8218427507506,
12.));
#133059=CARTESIAN_POINT('Ctrl Pts',(-21.4237784161588,-70.8011781217394,
0.));
#133060=CARTESIAN_POINT('Ctrl Pts',(-21.4237784161588,-70.8011781217394,
12.));
#133061=CARTESIAN_POINT('Ctrl Pts',(-21.4060425934599,-70.780524428745,
0.));
#133062=CARTESIAN_POINT('Ctrl Pts',(-21.4060425934599,-70.780524428745,
12.));
#133063=CARTESIAN_POINT('Ctrl Pts',(-21.3883489160196,-70.7598817714105,
0.));
#133064=CARTESIAN_POINT('Ctrl Pts',(-21.3883489160196,-70.7598817714105,
12.));
#133065=CARTESIAN_POINT('Ctrl Pts',(-21.3706974057039,-70.7392502475469,
0.));
#133066=CARTESIAN_POINT('Ctrl Pts',(-21.3706974057039,-70.7392502475469,
12.));
#133067=CARTESIAN_POINT('Ctrl Pts',(-21.3530880842349,-70.7186299539724,
0.));
#133068=CARTESIAN_POINT('Ctrl Pts',(-21.3530880842349,-70.7186299539724,
12.));
#133069=CARTESIAN_POINT('Ctrl Pts',(-21.3355209732443,-70.6980209870045,
0.));
#133070=CARTESIAN_POINT('Ctrl Pts',(-21.3355209732443,-70.6980209870045,
12.));
#133071=CARTESIAN_POINT('Ctrl Pts',(-21.3179960943389,-70.6774234430897,
0.));
#133072=CARTESIAN_POINT('Ctrl Pts',(-21.3179960943389,-70.6774234430897,
12.));
#133073=CARTESIAN_POINT('Ctrl Pts',(-21.300513469156,-70.6568374193774,
0.));
#133074=CARTESIAN_POINT('Ctrl Pts',(-21.300513469156,-70.6568374193774,
12.));
#133075=CARTESIAN_POINT('Ctrl Pts',(-21.2830731194183,-70.6362630143047,
0.));
#133076=CARTESIAN_POINT('Ctrl Pts',(-21.2830731194183,-70.6362630143047,
12.));
#133077=CARTESIAN_POINT('Ctrl Pts',(-21.2656750669126,-70.6157003273316,
0.));
#133078=CARTESIAN_POINT('Ctrl Pts',(-21.2656750669126,-70.6157003273316,
12.));
#133079=CARTESIAN_POINT('Ctrl Pts',(-21.2483193334676,-70.5951494586957,
0.));
#133080=CARTESIAN_POINT('Ctrl Pts',(-21.2483193334676,-70.5951494586957,
12.));
#133081=CARTESIAN_POINT('Ctrl Pts',(-21.2310059409266,-70.5746105091502,
0.));
#133082=CARTESIAN_POINT('Ctrl Pts',(-21.2310059409266,-70.5746105091502,
12.));
#133083=CARTESIAN_POINT('Ctrl Pts',(-21.2137349111208,-70.5540835797283,
0.));
#133084=CARTESIAN_POINT('Ctrl Pts',(-21.2137349111208,-70.5540835797283,
12.));
#133085=CARTESIAN_POINT('Ctrl Pts',(-21.1965062658298,-70.5335687714428,
0.));
#133086=CARTESIAN_POINT('Ctrl Pts',(-21.1965062658298,-70.5335687714428,
12.));
#133087=CARTESIAN_POINT('Ctrl Pts',(-21.1793200267847,-70.5130661852955,
0.));
#133088=CARTESIAN_POINT('Ctrl Pts',(-21.1793200267847,-70.5130661852955,
12.));
#133089=CARTESIAN_POINT('Ctrl Pts',(-21.1621762156897,-70.4925759224216,
0.));
#133090=CARTESIAN_POINT('Ctrl Pts',(-21.1621762156897,-70.4925759224216,
12.));
#133091=CARTESIAN_POINT('Ctrl Pts',(-21.1450748542337,-70.4720980841939,
0.));
#133092=CARTESIAN_POINT('Ctrl Pts',(-21.1450748542337,-70.4720980841939,
12.));
#133093=CARTESIAN_POINT('Ctrl Pts',(-21.1280159641003,-70.4516327723346,
0.));
#133094=CARTESIAN_POINT('Ctrl Pts',(-21.1280159641003,-70.4516327723346,
12.));
#133095=CARTESIAN_POINT('Ctrl Pts',(-21.1109995669747,-70.4311800890401,
0.));
#133096=CARTESIAN_POINT('Ctrl Pts',(-21.1109995669747,-70.4311800890401,
12.));
#133097=CARTESIAN_POINT('Ctrl Pts',(-21.0940256845473,-70.4107401370389,
0.));
#133098=CARTESIAN_POINT('Ctrl Pts',(-21.0940256845473,-70.4107401370389,
12.));
#133099=CARTESIAN_POINT('Ctrl Pts',(-21.0770943385141,-70.3903130195265,
0.));
#133100=CARTESIAN_POINT('Ctrl Pts',(-21.0770943385141,-70.3903130195265,
12.));
#133101=CARTESIAN_POINT('Ctrl Pts',(-21.0602055505748,-70.3698988401281,
0.));
#133102=CARTESIAN_POINT('Ctrl Pts',(-21.0602055505748,-70.3698988401281,
12.));
#133103=CARTESIAN_POINT('Ctrl Pts',(-21.0433593424267,-70.3494977028498,
0.));
#133104=CARTESIAN_POINT('Ctrl Pts',(-21.0433593424267,-70.3494977028498,
12.));
#133105=CARTESIAN_POINT('Ctrl Pts',(-21.0265557357548,-70.3291097120302,
0.));
#133106=CARTESIAN_POINT('Ctrl Pts',(-21.0265557357548,-70.3291097120302,
12.));
#133107=CARTESIAN_POINT('Ctrl Pts',(-21.0097947522218,-70.3087349722973,
0.));
#133108=CARTESIAN_POINT('Ctrl Pts',(-21.0097947522218,-70.3087349722973,
12.));
#133109=CARTESIAN_POINT('Ctrl Pts',(-20.9930764134776,-70.2883735885984,
0.));
#133110=CARTESIAN_POINT('Ctrl Pts',(-20.9930764134776,-70.2883735885984,
12.));
#133111=CARTESIAN_POINT('Ctrl Pts',(-20.9764007411653,-70.2680256662224,
0.));
#133112=CARTESIAN_POINT('Ctrl Pts',(-20.9764007411653,-70.2680256662224,
12.));
#133113=CARTESIAN_POINT('Ctrl Pts',(-20.9597677569228,-70.2476913108244,
0.));
#133114=CARTESIAN_POINT('Ctrl Pts',(-20.9597677569228,-70.2476913108244,
12.));
#133115=CARTESIAN_POINT('Ctrl Pts',(-20.9431774823831,-70.2273706284472,
0.));
#133116=CARTESIAN_POINT('Ctrl Pts',(-20.9431774823831,-70.2273706284472,
12.));
#133117=CARTESIAN_POINT('Ctrl Pts',(-20.9266299391684,-70.2070637255458,
0.));
#133118=CARTESIAN_POINT('Ctrl Pts',(-20.9266299391684,-70.2070637255458,
12.));
#133119=CARTESIAN_POINT('Ctrl Pts',(-20.9101251488944,-70.1867707089854,
0.));
#133120=CARTESIAN_POINT('Ctrl Pts',(-20.9101251488944,-70.1867707089854,
12.));
#133121=CARTESIAN_POINT('Ctrl Pts',(-20.8936631331748,-70.1664916860358,
0.));
#133122=CARTESIAN_POINT('Ctrl Pts',(-20.8936631331748,-70.1664916860358,
12.));
#133123=CARTESIAN_POINT('Ctrl Pts',(-20.8772439136206,-70.1462267643646,
0.));
#133124=CARTESIAN_POINT('Ctrl Pts',(-20.8772439136206,-70.1462267643646,
12.));
#133125=CARTESIAN_POINT('Ctrl Pts',(-20.8608675118379,-70.1259760520309,
0.));
#133126=CARTESIAN_POINT('Ctrl Pts',(-20.8608675118379,-70.1259760520309,
12.));
#133127=CARTESIAN_POINT('Ctrl Pts',(-20.8445339494188,-70.1057396574747,
0.));
#133128=CARTESIAN_POINT('Ctrl Pts',(-20.8445339494188,-70.1057396574747,
12.));
#133129=CARTESIAN_POINT('Ctrl Pts',(-20.8282432479429,-70.0855176895191,
0.));
#133130=CARTESIAN_POINT('Ctrl Pts',(-20.8282432479429,-70.0855176895191,
12.));
#133131=CARTESIAN_POINT('Ctrl Pts',(-20.8119954289849,-70.0653102573803,
0.));
#133132=CARTESIAN_POINT('Ctrl Pts',(-20.8119954289849,-70.0653102573803,
12.));
#133133=CARTESIAN_POINT('Ctrl Pts',(-20.7957905141157,-70.0451174706741,
0.));
#133134=CARTESIAN_POINT('Ctrl Pts',(-20.7957905141157,-70.0451174706741,
12.));
#133135=CARTESIAN_POINT('Ctrl Pts',(-20.7796285249022,-70.024939439422,
0.));
#133136=CARTESIAN_POINT('Ctrl Pts',(-20.7796285249022,-70.024939439422,
12.));
#133137=CARTESIAN_POINT('Ctrl Pts',(-20.7635094829016,-70.0047762740568,
0.));
#133138=CARTESIAN_POINT('Ctrl Pts',(-20.7635094829016,-70.0047762740568,
12.));
#133139=CARTESIAN_POINT('Ctrl Pts',(-20.7474334096581,-69.9846280854257,
0.));
#133140=CARTESIAN_POINT('Ctrl Pts',(-20.7474334096581,-69.9846280854257,
12.));
#133141=CARTESIAN_POINT('Ctrl Pts',(-20.7314003267119,-69.9644949847934,
0.));
#133142=CARTESIAN_POINT('Ctrl Pts',(-20.7314003267119,-69.9644949847934,
12.));
#133143=CARTESIAN_POINT('Ctrl Pts',(-20.7154102555997,-69.9443770838448,
0.));
#133144=CARTESIAN_POINT('Ctrl Pts',(-20.7154102555997,-69.9443770838448,
12.));
#133145=CARTESIAN_POINT('Ctrl Pts',(-20.6994632178552,-69.9242744946854,
0.));
#133146=CARTESIAN_POINT('Ctrl Pts',(-20.6994632178552,-69.9242744946854,
12.));
#133147=CARTESIAN_POINT('Ctrl Pts',(-20.683559235003,-69.904187329841,0.));
#133148=CARTESIAN_POINT('Ctrl Pts',(-20.683559235003,-69.904187329841,12.));
#133149=CARTESIAN_POINT('Ctrl Pts',(-20.667698328554,-69.8841157022568,
0.));
#133150=CARTESIAN_POINT('Ctrl Pts',(-20.667698328554,-69.8841157022568,
12.));
#133151=CARTESIAN_POINT('Ctrl Pts',(-20.6518805200129,-69.8640597253045,
0.));
#133152=CARTESIAN_POINT('Ctrl Pts',(-20.6518805200129,-69.8640597253045,
12.));
#133153=CARTESIAN_POINT('Ctrl Pts',(-20.6361058308811,-69.8440195127866,
0.));
#133154=CARTESIAN_POINT('Ctrl Pts',(-20.6361058308811,-69.8440195127866,
12.));
#133155=CARTESIAN_POINT('Ctrl Pts',(-20.6203742826566,-69.8239951789402,
0.));
#133156=CARTESIAN_POINT('Ctrl Pts',(-20.6203742826566,-69.8239951789402,
12.));
#133157=CARTESIAN_POINT('Ctrl Pts',(-20.6046858968308,-69.8039868384389,
0.));
#133158=CARTESIAN_POINT('Ctrl Pts',(-20.6046858968308,-69.8039868384389,
12.));
#133159=CARTESIAN_POINT('Ctrl Pts',(-20.5890406948811,-69.7839946063949,
0.));
#133160=CARTESIAN_POINT('Ctrl Pts',(-20.5890406948811,-69.7839946063949,
12.));
#133161=CARTESIAN_POINT('Ctrl Pts',(-20.5734386982783,-69.7640185983644,
0.));
#133162=CARTESIAN_POINT('Ctrl Pts',(-20.5734386982783,-69.7640185983644,
12.));
#133163=CARTESIAN_POINT('Ctrl Pts',(-20.5578799284898,-69.744058930351,
0.));
#133164=CARTESIAN_POINT('Ctrl Pts',(-20.5578799284898,-69.744058930351,
12.));
#133165=CARTESIAN_POINT('Ctrl Pts',(-20.54236440698,-69.7241157188083,0.));
#133166=CARTESIAN_POINT('Ctrl Pts',(-20.54236440698,-69.7241157188083,12.));
#133167=CARTESIAN_POINT('Ctrl Pts',(-20.5268921552077,-69.7041890806425,
0.));
#133168=CARTESIAN_POINT('Ctrl Pts',(-20.5268921552077,-69.7041890806425,
12.));
#133169=CARTESIAN_POINT('Ctrl Pts',(-20.5114631946185,-69.6842791332115,
0.));
#133170=CARTESIAN_POINT('Ctrl Pts',(-20.5114631946185,-69.6842791332115,
12.));
#133171=CARTESIAN_POINT('Ctrl Pts',(-20.4960775466492,-69.6643859943308,
0.));
#133172=CARTESIAN_POINT('Ctrl Pts',(-20.4960775466492,-69.6643859943308,
12.));
#133173=CARTESIAN_POINT('Ctrl Pts',(-20.480735232734,-69.6445097822792,
0.));
#133174=CARTESIAN_POINT('Ctrl Pts',(-20.480735232734,-69.6445097822792,
12.));
#133175=CARTESIAN_POINT('Ctrl Pts',(-20.4654362743037,-69.6246506158013,
0.));
#133176=CARTESIAN_POINT('Ctrl Pts',(-20.4654362743037,-69.6246506158013,
12.));
#133177=CARTESIAN_POINT('Ctrl Pts',(-20.4501806927852,-69.6048086141113,
0.));
#133178=CARTESIAN_POINT('Ctrl Pts',(-20.4501806927852,-69.6048086141113,
12.));
#133179=CARTESIAN_POINT('Ctrl Pts',(-20.4349685095924,-69.5849838968928,
0.));
#133180=CARTESIAN_POINT('Ctrl Pts',(-20.4349685095924,-69.5849838968928,
12.));
#133181=CARTESIAN_POINT('Ctrl Pts',(-20.4197997461301,-69.5651765843033,
0.));
#133182=CARTESIAN_POINT('Ctrl Pts',(-20.4197997461301,-69.5651765843033,
12.));
#133183=CARTESIAN_POINT('Ctrl Pts',(-20.4046744237999,-69.5453867969804,
0.));
#133184=CARTESIAN_POINT('Ctrl Pts',(-20.4046744237999,-69.5453867969804,
12.));
#133185=CARTESIAN_POINT('Ctrl Pts',(-20.3895925640005,-69.5256146560441,
0.));
#133186=CARTESIAN_POINT('Ctrl Pts',(-20.3895925640005,-69.5256146560441,
12.));
#133187=CARTESIAN_POINT('Ctrl Pts',(-20.3745541881269,-69.5058602831008,
0.));
#133188=CARTESIAN_POINT('Ctrl Pts',(-20.3745541881269,-69.5058602831008,
12.));
#133189=CARTESIAN_POINT('Ctrl Pts',(-20.3595593175623,-69.4861238002441,
0.));
#133190=CARTESIAN_POINT('Ctrl Pts',(-20.3595593175623,-69.4861238002441,
12.));
#133191=CARTESIAN_POINT('Ctrl Pts',(-20.3446079736802,-69.4664053300587,
0.));
#133192=CARTESIAN_POINT('Ctrl Pts',(-20.3446079736802,-69.4664053300587,
12.));
#133193=CARTESIAN_POINT('Ctrl Pts',(-20.3297001778507,-69.4467049956262,
0.));
#133194=CARTESIAN_POINT('Ctrl Pts',(-20.3297001778507,-69.4467049956262,
12.));
#133195=CARTESIAN_POINT('Ctrl Pts',(-20.3148359514415,-69.4270229205297,
0.));
#133196=CARTESIAN_POINT('Ctrl Pts',(-20.3148359514415,-69.4270229205297,
12.));
#133197=CARTESIAN_POINT('Ctrl Pts',(-20.3000153158167,-69.407359228856,
0.));
#133198=CARTESIAN_POINT('Ctrl Pts',(-20.3000153158167,-69.407359228856,
12.));
#133199=CARTESIAN_POINT('Ctrl Pts',(-20.2852382923299,-69.3877140451975,
0.));
#133200=CARTESIAN_POINT('Ctrl Pts',(-20.2852382923299,-69.3877140451975,
12.));
#133201=CARTESIAN_POINT('Ctrl Pts',(-20.2705049023241,-69.368087494655,
0.));
#133202=CARTESIAN_POINT('Ctrl Pts',(-20.2705049023241,-69.368087494655,
12.));
#133203=CARTESIAN_POINT('Ctrl Pts',(-20.2558151671391,-69.3484797028458,
0.));
#133204=CARTESIAN_POINT('Ctrl Pts',(-20.2558151671391,-69.3484797028458,
12.));
#133205=CARTESIAN_POINT('Ctrl Pts',(-20.2411691081123,-69.3288907959067,
0.));
#133206=CARTESIAN_POINT('Ctrl Pts',(-20.2411691081123,-69.3288907959067,
12.));
#133207=CARTESIAN_POINT('Ctrl Pts',(-20.2265667465784,-69.3093209004984,
0.));
#133208=CARTESIAN_POINT('Ctrl Pts',(-20.2265667465784,-69.3093209004984,
12.));
#133209=CARTESIAN_POINT('Ctrl Pts',(-20.2120081038621,-69.2897701438059,
0.));
#133210=CARTESIAN_POINT('Ctrl Pts',(-20.2120081038621,-69.2897701438059,
12.));
#133211=CARTESIAN_POINT('Ctrl Pts',(-20.1974932012773,-69.2702386535422,
0.));
#133212=CARTESIAN_POINT('Ctrl Pts',(-20.1974932012773,-69.2702386535422,
12.));
#133213=CARTESIAN_POINT('Ctrl Pts',(-20.1830220601349,-69.2507265579554,
0.));
#133214=CARTESIAN_POINT('Ctrl Pts',(-20.1830220601349,-69.2507265579554,
12.));
#133215=CARTESIAN_POINT('Ctrl Pts',(-20.1685947017433,-69.2312339858335,
0.));
#133216=CARTESIAN_POINT('Ctrl Pts',(-20.1685947017433,-69.2312339858335,
12.));
#133217=CARTESIAN_POINT('Ctrl Pts',(-20.1542111474087,-69.2117610665076,
0.));
#133218=CARTESIAN_POINT('Ctrl Pts',(-20.1542111474087,-69.2117610665076,
12.));
#133219=CARTESIAN_POINT('Ctrl Pts',(-20.139871418428,-69.1923079298538,
0.));
#133220=CARTESIAN_POINT('Ctrl Pts',(-20.139871418428,-69.1923079298538,
12.));
#133221=CARTESIAN_POINT('Ctrl Pts',(-20.1255755360872,-69.1728747062963,
0.));
#133222=CARTESIAN_POINT('Ctrl Pts',(-20.1255755360872,-69.1728747062963,
12.));
#133223=CARTESIAN_POINT('Ctrl Pts',(-20.1113235216694,-69.1534615268152,
0.));
#133224=CARTESIAN_POINT('Ctrl Pts',(-20.1113235216694,-69.1534615268152,
12.));
#133225=CARTESIAN_POINT('Ctrl Pts',(-20.0971153964557,-69.1340685229514,
0.));
#133226=CARTESIAN_POINT('Ctrl Pts',(-20.0971153964557,-69.1340685229514,
12.));
#133227=CARTESIAN_POINT('Ctrl Pts',(-20.0829511817251,-69.1146958268104,
0.));
#133228=CARTESIAN_POINT('Ctrl Pts',(-20.0829511817251,-69.1146958268104,
12.));
#133229=CARTESIAN_POINT('Ctrl Pts',(-20.068830898748,-69.095343571064,0.));
#133230=CARTESIAN_POINT('Ctrl Pts',(-20.068830898748,-69.095343571064,12.));
#133231=CARTESIAN_POINT('Ctrl Pts',(-20.0547545687842,-69.0760118889535,
0.));
#133232=CARTESIAN_POINT('Ctrl Pts',(-20.0547545687842,-69.0760118889535,
12.));
#133233=CARTESIAN_POINT('Ctrl Pts',(-20.0407222130906,-69.0567009142978,
0.));
#133234=CARTESIAN_POINT('Ctrl Pts',(-20.0407222130906,-69.0567009142978,
12.));
#133235=CARTESIAN_POINT('Ctrl Pts',(-20.0267338529223,-69.0374107814984,
0.));
#133236=CARTESIAN_POINT('Ctrl Pts',(-20.0267338529223,-69.0374107814984,
12.));
#133237=CARTESIAN_POINT('Ctrl Pts',(-20.0127895095327,-69.0181416255431,
0.));
#133238=CARTESIAN_POINT('Ctrl Pts',(-20.0127895095327,-69.0181416255431,
12.));
#133239=CARTESIAN_POINT('Ctrl Pts',(-19.9988892041666,-68.9988935820084,
0.));
#133240=CARTESIAN_POINT('Ctrl Pts',(-19.9988892041666,-68.9988935820084,
12.));
#133241=CARTESIAN_POINT('Ctrl Pts',(-19.9850329580591,-68.9796667870638,
0.));
#133242=CARTESIAN_POINT('Ctrl Pts',(-19.9850329580591,-68.9796667870638,
12.));
#133243=CARTESIAN_POINT('Ctrl Pts',(-19.9712207924429,-68.9604613774802,
0.));
#133244=CARTESIAN_POINT('Ctrl Pts',(-19.9712207924429,-68.9604613774802,
12.));
#133245=CARTESIAN_POINT('Ctrl Pts',(-19.9574527285488,-68.9412774906333,
0.));
#133246=CARTESIAN_POINT('Ctrl Pts',(-19.9574527285488,-68.9412774906333,
12.));
#133247=CARTESIAN_POINT('Ctrl Pts',(-19.9437287876066,-68.9221152645095,
0.));
#133248=CARTESIAN_POINT('Ctrl Pts',(-19.9437287876066,-68.9221152645095,
12.));
#133249=CARTESIAN_POINT('Ctrl Pts',(-19.9300489908374,-68.9029748377067,
0.));
#133250=CARTESIAN_POINT('Ctrl Pts',(-19.9300489908374,-68.9029748377067,
12.));
#133251=CARTESIAN_POINT('Ctrl Pts',(-19.9164133594526,-68.8838563494393,
0.));
#133252=CARTESIAN_POINT('Ctrl Pts',(-19.9164133594526,-68.8838563494393,
12.));
#133253=CARTESIAN_POINT('Ctrl Pts',(-19.9028219146618,-68.8647599395469,
0.));
#133254=CARTESIAN_POINT('Ctrl Pts',(-19.9028219146618,-68.8647599395469,
12.));
#133255=CARTESIAN_POINT('Ctrl Pts',(-19.8892746776739,-68.8456857485002,
0.));
#133256=CARTESIAN_POINT('Ctrl Pts',(-19.8892746776739,-68.8456857485002,
12.));
#133257=CARTESIAN_POINT('Ctrl Pts',(-19.8757716696965,-68.8266339174056,
0.));
#133258=CARTESIAN_POINT('Ctrl Pts',(-19.8757716696965,-68.8266339174056,
12.));
#133259=CARTESIAN_POINT('Ctrl Pts',(-19.8623129119293,-68.8076045880065,
0.));
#133260=CARTESIAN_POINT('Ctrl Pts',(-19.8623129119293,-68.8076045880065,
12.));
#133261=CARTESIAN_POINT('Ctrl Pts',(-19.8488984255627,-68.7885979026878,
0.));
#133262=CARTESIAN_POINT('Ctrl Pts',(-19.8488984255627,-68.7885979026878,
12.));
#133263=CARTESIAN_POINT('Ctrl Pts',(-19.8355282317858,-68.7696140044851,
0.));
#133264=CARTESIAN_POINT('Ctrl Pts',(-19.8355282317858,-68.7696140044851,
12.));
#133265=CARTESIAN_POINT('Ctrl Pts',(-19.8222023517871,-68.7506530370904,
0.));
#133266=CARTESIAN_POINT('Ctrl Pts',(-19.8222023517871,-68.7506530370904,
12.));
#133267=CARTESIAN_POINT('Ctrl Pts',(-19.8089208067537,-68.7317151448573,
0.));
#133268=CARTESIAN_POINT('Ctrl Pts',(-19.8089208067537,-68.7317151448573,
12.));
#133269=CARTESIAN_POINT('Ctrl Pts',(-19.7956836178651,-68.7128004728033,
0.));
#133270=CARTESIAN_POINT('Ctrl Pts',(-19.7956836178651,-68.7128004728033,
12.));
#133271=CARTESIAN_POINT('Ctrl Pts',(-19.7824908062925,-68.6939091666149,
0.));
#133272=CARTESIAN_POINT('Ctrl Pts',(-19.7824908062925,-68.6939091666149,
12.));
#133273=CARTESIAN_POINT('Ctrl Pts',(-19.7693423932067,-68.6750413726574,
0.));
#133274=CARTESIAN_POINT('Ctrl Pts',(-19.7693423932067,-68.6750413726574,
12.));
#133275=CARTESIAN_POINT('Ctrl Pts',(-19.7562383997784,-68.65619723798,0.));
#133276=CARTESIAN_POINT('Ctrl Pts',(-19.7562383997784,-68.65619723798,12.));
#133277=CARTESIAN_POINT('Ctrl Pts',(-19.7431788471773,-68.6373769103211,
0.));
#133278=CARTESIAN_POINT('Ctrl Pts',(-19.7431788471773,-68.6373769103211,
12.));
#133279=CARTESIAN_POINT('Ctrl Pts',(-19.7301637565646,-68.6185805381102,
0.));
#133280=CARTESIAN_POINT('Ctrl Pts',(-19.7301637565646,-68.6185805381102,
12.));
#133281=CARTESIAN_POINT('Ctrl Pts',(-19.717193149095,-68.5998082704741,
0.));
#133282=CARTESIAN_POINT('Ctrl Pts',(-19.717193149095,-68.5998082704741,
12.));
#133283=CARTESIAN_POINT('Ctrl Pts',(-19.7042670459234,-68.5810602572474,
0.));
#133284=CARTESIAN_POINT('Ctrl Pts',(-19.7042670459234,-68.5810602572474,
12.));
#133285=CARTESIAN_POINT('Ctrl Pts',(-19.6913854682046,-68.5623366489776,
0.));
#133286=CARTESIAN_POINT('Ctrl Pts',(-19.6913854682046,-68.5623366489776,
12.));
#133287=CARTESIAN_POINT('Ctrl Pts',(-19.6785484370929,-68.543637596932,
0.));
#133288=CARTESIAN_POINT('Ctrl Pts',(-19.6785484370929,-68.543637596932,
12.));
#133289=CARTESIAN_POINT('Ctrl Pts',(-19.665755973734,-68.5249632530994,
0.));
#133290=CARTESIAN_POINT('Ctrl Pts',(-19.665755973734,-68.5249632530994,
12.));
#133291=CARTESIAN_POINT('Ctrl Pts',(-19.653008099269,-68.5063137701986,
0.));
#133292=CARTESIAN_POINT('Ctrl Pts',(-19.653008099269,-68.5063137701986,
12.));
#133293=CARTESIAN_POINT('Ctrl Pts',(-19.6403048348397,-68.4876893016863,
0.));
#133294=CARTESIAN_POINT('Ctrl Pts',(-19.6403048348397,-68.4876893016863,
12.));
#133295=CARTESIAN_POINT('Ctrl Pts',(-19.6276462015888,-68.4690900017631,
0.));
#133296=CARTESIAN_POINT('Ctrl Pts',(-19.6276462015888,-68.4690900017631,
12.));
#133297=CARTESIAN_POINT('Ctrl Pts',(-19.6150322206578,-68.4505160253777,
0.));
#133298=CARTESIAN_POINT('Ctrl Pts',(-19.6150322206578,-68.4505160253777,
12.));
#133299=CARTESIAN_POINT('Ctrl Pts',(-19.6024629131786,-68.4319675282273,
0.));
#133300=CARTESIAN_POINT('Ctrl Pts',(-19.6024629131786,-68.4319675282273,
12.));
#133301=CARTESIAN_POINT('Ctrl Pts',(-19.5899383002804,-68.4134446667695,
0.));
#133302=CARTESIAN_POINT('Ctrl Pts',(-19.5899383002804,-68.4134446667695,
12.));
#133303=CARTESIAN_POINT('Ctrl Pts',(-19.5774584030939,-68.3949475982334,
0.));
#133304=CARTESIAN_POINT('Ctrl Pts',(-19.5774584030939,-68.3949475982334,
12.));
#133305=CARTESIAN_POINT('Ctrl Pts',(-19.5650232427516,-68.3764764806287,
0.));
#133306=CARTESIAN_POINT('Ctrl Pts',(-19.5650232427516,-68.3764764806287,
12.));
#133307=CARTESIAN_POINT('Ctrl Pts',(-19.5526328403852,-68.3580314727522,
0.));
#133308=CARTESIAN_POINT('Ctrl Pts',(-19.5526328403852,-68.3580314727522,
12.));
#133309=CARTESIAN_POINT('Ctrl Pts',(-19.540287217119,-68.3396127341938,
0.));
#133310=CARTESIAN_POINT('Ctrl Pts',(-19.540287217119,-68.3396127341938,
12.));
#133311=CARTESIAN_POINT('Ctrl Pts',(-19.5279863940773,-68.3212204253415,
0.));
#133312=CARTESIAN_POINT('Ctrl Pts',(-19.5279863940773,-68.3212204253415,
12.));
#133313=CARTESIAN_POINT('Ctrl Pts',(-19.5157303923856,-68.3028547073862,
0.));
#133314=CARTESIAN_POINT('Ctrl Pts',(-19.5157303923856,-68.3028547073862,
12.));
#133315=CARTESIAN_POINT('Ctrl Pts',(-19.5035192331706,-68.2845157423234,
0.));
#133316=CARTESIAN_POINT('Ctrl Pts',(-19.5035192331706,-68.2845157423234,
12.));
#133317=CARTESIAN_POINT('Ctrl Pts',(-19.4913529375545,-68.2662036929531,
0.));
#133318=CARTESIAN_POINT('Ctrl Pts',(-19.4913529375545,-68.2662036929531,
12.));
#133319=CARTESIAN_POINT('Ctrl Pts',(-19.4792315266505,-68.2479187228815,
0.));
#133320=CARTESIAN_POINT('Ctrl Pts',(-19.4792315266505,-68.2479187228815,
12.));
#133321=CARTESIAN_POINT('Ctrl Pts',(-19.4671550215724,-68.2296609965461,
0.));
#133322=CARTESIAN_POINT('Ctrl Pts',(-19.4671550215724,-68.2296609965461,
12.));
#133323=CARTESIAN_POINT('Ctrl Pts',(-19.4551234434384,-68.2114306792366,
0.));
#133324=CARTESIAN_POINT('Ctrl Pts',(-19.4551234434384,-68.2114306792366,
12.));
#133325=CARTESIAN_POINT('Ctrl Pts',(-19.4431368133718,-68.1932279371121,
0.));
#133326=CARTESIAN_POINT('Ctrl Pts',(-19.4431368133718,-68.1932279371121,
12.));
#133327=CARTESIAN_POINT('Ctrl Pts',(-19.4311951524977,-68.1750529372211,
0.));
#133328=CARTESIAN_POINT('Ctrl Pts',(-19.4311951524977,-68.1750529372211,
12.));
#133329=CARTESIAN_POINT('Ctrl Pts',(-19.4192984819411,-68.1569058475026,
0.));
#133330=CARTESIAN_POINT('Ctrl Pts',(-19.4192984819411,-68.1569058475026,
12.));
#133331=CARTESIAN_POINT('Ctrl Pts',(-19.4074468228294,-68.1387868367668,
0.));
#133332=CARTESIAN_POINT('Ctrl Pts',(-19.4074468228294,-68.1387868367668,
12.));
#133333=CARTESIAN_POINT('Ctrl Pts',(-19.3956401962893,-68.1206960746763,
0.));
#133334=CARTESIAN_POINT('Ctrl Pts',(-19.3956401962893,-68.1206960746763,
12.));
#133335=CARTESIAN_POINT('Ctrl Pts',(-19.3838786234426,-68.1026337317298,
0.));
#133336=CARTESIAN_POINT('Ctrl Pts',(-19.3838786234426,-68.1026337317298,
12.));
#133337=CARTESIAN_POINT('Ctrl Pts',(-19.3721621253921,-68.0845999792274,
0.));
#133338=CARTESIAN_POINT('Ctrl Pts',(-19.3721621253921,-68.0845999792274,
12.));
#133339=CARTESIAN_POINT('Ctrl Pts',(-19.3604907232322,-68.0665949893222,
0.));
#133340=CARTESIAN_POINT('Ctrl Pts',(-19.3604907232322,-68.0665949893222,
12.));
#133341=CARTESIAN_POINT('Ctrl Pts',(-19.3488644380646,-68.0486189351027,
0.));
#133342=CARTESIAN_POINT('Ctrl Pts',(-19.3488644380646,-68.0486189351027,
12.));
#133343=CARTESIAN_POINT('Ctrl Pts',(-19.3372832910077,-68.0306719906636,
0.));
#133344=CARTESIAN_POINT('Ctrl Pts',(-19.3372832910077,-68.0306719906636,
12.));
#133345=CARTESIAN_POINT('Ctrl Pts',(-19.3257473032031,-68.0127543311761,
0.));
#133346=CARTESIAN_POINT('Ctrl Pts',(-19.3257473032031,-68.0127543311761,
12.));
#133347=CARTESIAN_POINT('Ctrl Pts',(-19.3142564958196,-67.9948661329591,
0.));
#133348=CARTESIAN_POINT('Ctrl Pts',(-19.3142564958196,-67.9948661329591,
12.));
#133349=CARTESIAN_POINT('Ctrl Pts',(-19.3028108900374,-67.977007573346,
0.));
#133350=CARTESIAN_POINT('Ctrl Pts',(-19.3028108900374,-67.977007573346,
12.));
#133351=CARTESIAN_POINT('Ctrl Pts',(-19.2914105070283,-67.959178830538,
0.));
#133352=CARTESIAN_POINT('Ctrl Pts',(-19.2914105070283,-67.959178830538,
12.));
#133353=CARTESIAN_POINT('Ctrl Pts',(-19.2800553679362,-67.9413800834798,
0.));
#133354=CARTESIAN_POINT('Ctrl Pts',(-19.2800553679362,-67.9413800834798,
12.));
#133355=CARTESIAN_POINT('Ctrl Pts',(-19.2687454938449,-67.9236115116781,
0.));
#133356=CARTESIAN_POINT('Ctrl Pts',(-19.2687454938449,-67.9236115116781,
12.));
#133357=CARTESIAN_POINT('Ctrl Pts',(-19.2574809057705,-67.9058732951822,
0.));
#133358=CARTESIAN_POINT('Ctrl Pts',(-19.2574809057705,-67.9058732951822,
12.));
#133359=CARTESIAN_POINT('Ctrl Pts',(-19.2462616247287,-67.8881656149983,
0.));
#133360=CARTESIAN_POINT('Ctrl Pts',(-19.2462616247287,-67.8881656149983,
12.));
#133361=CARTESIAN_POINT('Ctrl Pts',(-19.2350876717878,-67.8704886534555,
0.));
#133362=CARTESIAN_POINT('Ctrl Pts',(-19.2350876717878,-67.8704886534555,
12.));
#133363=CARTESIAN_POINT('Ctrl Pts',(-19.223959068113,-67.852842594517,0.));
#133364=CARTESIAN_POINT('Ctrl Pts',(-19.223959068113,-67.852842594517,12.));
#133365=CARTESIAN_POINT('Ctrl Pts',(-19.2128758350336,-67.8352276242856,
0.));
#133366=CARTESIAN_POINT('Ctrl Pts',(-19.2128758350336,-67.8352276242856,
12.));
#133367=CARTESIAN_POINT('Ctrl Pts',(-19.2018379939918,-67.817643930658,
0.));
#133368=CARTESIAN_POINT('Ctrl Pts',(-19.2018379939918,-67.817643930658,
12.));
#133369=CARTESIAN_POINT('Ctrl Pts',(-19.1908455664089,-67.8000917023896,
0.));
#133370=CARTESIAN_POINT('Ctrl Pts',(-19.1908455664089,-67.8000917023896,
12.));
#133371=CARTESIAN_POINT('Ctrl Pts',(-19.1798985735687,-67.7825711283092,
0.));
#133372=CARTESIAN_POINT('Ctrl Pts',(-19.1798985735687,-67.7825711283092,
12.));
#133373=CARTESIAN_POINT('Ctrl Pts',(-19.1689970364959,-67.7650823965156,
0.));
#133374=CARTESIAN_POINT('Ctrl Pts',(-19.1689970364959,-67.7650823965156,
12.));
#133375=CARTESIAN_POINT('Ctrl Pts',(-19.1581409758112,-67.7476256934492,
0.));
#133376=CARTESIAN_POINT('Ctrl Pts',(-19.1581409758112,-67.7476256934492,
12.));
#133377=CARTESIAN_POINT('Ctrl Pts',(-19.1473304119969,-67.7302012056629,
0.));
#133378=CARTESIAN_POINT('Ctrl Pts',(-19.1473304119969,-67.7302012056629,
12.));
#133379=CARTESIAN_POINT('Ctrl Pts',(-19.1365653657098,-67.7128091219372,
0.));
#133380=CARTESIAN_POINT('Ctrl Pts',(-19.1365653657098,-67.7128091219372,
12.));
#133381=CARTESIAN_POINT('Ctrl Pts',(-19.1258458580343,-67.6954496350053,
0.));
#133382=CARTESIAN_POINT('Ctrl Pts',(-19.1258458580343,-67.6954496350053,
12.));
#133383=CARTESIAN_POINT('Ctrl Pts',(-19.115171910845,-67.6781229440535,
0.));
#133384=CARTESIAN_POINT('Ctrl Pts',(-19.115171910845,-67.6781229440535,
12.));
#133385=CARTESIAN_POINT('Ctrl Pts',(-19.1045435468345,-67.6608292549412,
0.));
#133386=CARTESIAN_POINT('Ctrl Pts',(-19.1045435468345,-67.6608292549412,
12.));
#133387=CARTESIAN_POINT('Ctrl Pts',(-19.0939607887492,-67.6435687749803,
0.));
#133388=CARTESIAN_POINT('Ctrl Pts',(-19.0939607887492,-67.6435687749803,
12.));
#133389=CARTESIAN_POINT('Ctrl Pts',(-19.0834236587115,-67.6263417083414,
0.));
#133390=CARTESIAN_POINT('Ctrl Pts',(-19.0834236587115,-67.6263417083414,
12.));
#133391=CARTESIAN_POINT('Ctrl Pts',(-19.0729321776287,-67.6091482520557,
0.));
#133392=CARTESIAN_POINT('Ctrl Pts',(-19.0729321776287,-67.6091482520557,
12.));
#133393=CARTESIAN_POINT('Ctrl Pts',(-19.0624863642425,-67.5919885896278,
0.));
#133394=CARTESIAN_POINT('Ctrl Pts',(-19.0624863642425,-67.5919885896278,
12.));
#133395=CARTESIAN_POINT('Ctrl Pts',(-19.0520862360414,-67.5748628972035,
0.));
#133396=CARTESIAN_POINT('Ctrl Pts',(-19.0520862360414,-67.5748628972035,
12.));
#133397=CARTESIAN_POINT('Ctrl Pts',(-19.0417318110721,-67.5577713558248,
0.));
#133398=CARTESIAN_POINT('Ctrl Pts',(-19.0417318110721,-67.5577713558248,
12.));
#133399=CARTESIAN_POINT('Ctrl Pts',(-19.0314231093924,-67.540714161288,
0.));
#133400=CARTESIAN_POINT('Ctrl Pts',(-19.0314231093924,-67.540714161288,
12.));
#133401=CARTESIAN_POINT('Ctrl Pts',(-19.0211601548222,-67.5236915360253,
0.));
#133402=CARTESIAN_POINT('Ctrl Pts',(-19.0211601548222,-67.5236915360253,
12.));
#133403=CARTESIAN_POINT('Ctrl Pts',(-19.0109429761274,-67.5067037372177,
0.));
#133404=CARTESIAN_POINT('Ctrl Pts',(-19.0109429761274,-67.5067037372177,
12.));
#133405=CARTESIAN_POINT('Ctrl Pts',(-19.0007716032785,-67.4897510316692,
0.));
#133406=CARTESIAN_POINT('Ctrl Pts',(-19.0007716032785,-67.4897510316692,
12.));
#133407=CARTESIAN_POINT('Ctrl Pts',(-18.9906460638607,-67.4728336719558,
0.));
#133408=CARTESIAN_POINT('Ctrl Pts',(-18.9906460638607,-67.4728336719558,
12.));
#133409=CARTESIAN_POINT('Ctrl Pts',(-18.9805663798466,-67.4559518744714,
0.));
#133410=CARTESIAN_POINT('Ctrl Pts',(-18.9805663798466,-67.4559518744714,
12.));
#133411=CARTESIAN_POINT('Ctrl Pts',(-18.9705325631773,-67.4391057908687,
0.));
#133412=CARTESIAN_POINT('Ctrl Pts',(-18.9705325631773,-67.4391057908687,
12.));
#133413=CARTESIAN_POINT('Ctrl Pts',(-18.9605446161079,-67.4222955062385,
0.));
#133414=CARTESIAN_POINT('Ctrl Pts',(-18.9605446161079,-67.4222955062385,
12.));
#133415=CARTESIAN_POINT('Ctrl Pts',(-18.9525909518003,-67.4088759498287,
0.));
#133416=CARTESIAN_POINT('Ctrl Pts',(-18.9525909518003,-67.4088759498287,
12.));
#133417=CARTESIAN_POINT('Ctrl Pts',(-18.9466463414355,-67.398827414689,
0.));
#133418=CARTESIAN_POINT('Ctrl Pts',(-18.9466463414355,-67.398827414689,
12.));
#133419=CARTESIAN_POINT('Ctrl Pts',(-18.942692439874,-67.3921355608417,
0.));
#133420=CARTESIAN_POINT('Ctrl Pts',(-18.942692439874,-67.3921355608417,
12.));
#133421=CARTESIAN_POINT('Ctrl Pts',(-18.9407177820969,-67.3887914263118,
0.));
#133422=CARTESIAN_POINT('Ctrl Pts',(-18.9407177820969,-67.3887914263118,
12.));
#133423=CARTESIAN_POINT('',(-18.9407177820969,-67.3887914263118,12.));
#133424=CARTESIAN_POINT('Ctrl Pts',(-18.9407177820969,-67.3887914263118,
12.));
#133425=CARTESIAN_POINT('Ctrl Pts',(-18.942692439874,-67.3921355608417,
12.));
#133426=CARTESIAN_POINT('Ctrl Pts',(-18.9466463414355,-67.398827414689,
12.));
#133427=CARTESIAN_POINT('Ctrl Pts',(-18.9525909518003,-67.4088759498287,
12.));
#133428=CARTESIAN_POINT('Ctrl Pts',(-18.9605446161079,-67.4222955062385,
12.));
#133429=CARTESIAN_POINT('Ctrl Pts',(-18.9705325631773,-67.4391057908687,
12.));
#133430=CARTESIAN_POINT('Ctrl Pts',(-18.9805663798466,-67.4559518744714,
12.));
#133431=CARTESIAN_POINT('Ctrl Pts',(-18.9906460638607,-67.4728336719558,
12.));
#133432=CARTESIAN_POINT('Ctrl Pts',(-19.0007716032785,-67.4897510316692,
12.));
#133433=CARTESIAN_POINT('Ctrl Pts',(-19.0109429761274,-67.5067037372177,
12.));
#133434=CARTESIAN_POINT('Ctrl Pts',(-19.0211601548222,-67.5236915360253,
12.));
#133435=CARTESIAN_POINT('Ctrl Pts',(-19.0314231093924,-67.540714161288,
12.));
#133436=CARTESIAN_POINT('Ctrl Pts',(-19.0417318110721,-67.5577713558248,
12.));
#133437=CARTESIAN_POINT('Ctrl Pts',(-19.0520862360414,-67.5748628972035,
12.));
#133438=CARTESIAN_POINT('Ctrl Pts',(-19.0624863642425,-67.5919885896278,
12.));
#133439=CARTESIAN_POINT('Ctrl Pts',(-19.0729321776287,-67.6091482520557,
12.));
#133440=CARTESIAN_POINT('Ctrl Pts',(-19.0834236587115,-67.6263417083414,
12.));
#133441=CARTESIAN_POINT('Ctrl Pts',(-19.0939607887492,-67.6435687749803,
12.));
#133442=CARTESIAN_POINT('Ctrl Pts',(-19.1045435468345,-67.6608292549412,
12.));
#133443=CARTESIAN_POINT('Ctrl Pts',(-19.115171910845,-67.6781229440535,
12.));
#133444=CARTESIAN_POINT('Ctrl Pts',(-19.1258458580343,-67.6954496350053,
12.));
#133445=CARTESIAN_POINT('Ctrl Pts',(-19.1365653657098,-67.7128091219372,
12.));
#133446=CARTESIAN_POINT('Ctrl Pts',(-19.1473304119969,-67.7302012056629,
12.));
#133447=CARTESIAN_POINT('Ctrl Pts',(-19.1581409758112,-67.7476256934492,
12.));
#133448=CARTESIAN_POINT('Ctrl Pts',(-19.1689970364959,-67.7650823965156,
12.));
#133449=CARTESIAN_POINT('Ctrl Pts',(-19.1798985735687,-67.7825711283092,
12.));
#133450=CARTESIAN_POINT('Ctrl Pts',(-19.1908455664089,-67.8000917023896,
12.));
#133451=CARTESIAN_POINT('Ctrl Pts',(-19.2018379939918,-67.817643930658,
12.));
#133452=CARTESIAN_POINT('Ctrl Pts',(-19.2128758350336,-67.8352276242856,
12.));
#133453=CARTESIAN_POINT('Ctrl Pts',(-19.223959068113,-67.852842594517,12.));
#133454=CARTESIAN_POINT('Ctrl Pts',(-19.2350876717878,-67.8704886534555,
12.));
#133455=CARTESIAN_POINT('Ctrl Pts',(-19.2462616247287,-67.8881656149983,
12.));
#133456=CARTESIAN_POINT('Ctrl Pts',(-19.2574809057705,-67.9058732951822,
12.));
#133457=CARTESIAN_POINT('Ctrl Pts',(-19.2687454938449,-67.9236115116781,
12.));
#133458=CARTESIAN_POINT('Ctrl Pts',(-19.2800553679362,-67.9413800834798,
12.));
#133459=CARTESIAN_POINT('Ctrl Pts',(-19.2914105070283,-67.959178830538,
12.));
#133460=CARTESIAN_POINT('Ctrl Pts',(-19.3028108900374,-67.977007573346,
12.));
#133461=CARTESIAN_POINT('Ctrl Pts',(-19.3142564958196,-67.9948661329591,
12.));
#133462=CARTESIAN_POINT('Ctrl Pts',(-19.3257473032031,-68.0127543311761,
12.));
#133463=CARTESIAN_POINT('Ctrl Pts',(-19.3372832910077,-68.0306719906636,
12.));
#133464=CARTESIAN_POINT('Ctrl Pts',(-19.3488644380646,-68.0486189351027,
12.));
#133465=CARTESIAN_POINT('Ctrl Pts',(-19.3604907232322,-68.0665949893222,
12.));
#133466=CARTESIAN_POINT('Ctrl Pts',(-19.3721621253921,-68.0845999792274,
12.));
#133467=CARTESIAN_POINT('Ctrl Pts',(-19.3838786234426,-68.1026337317298,
12.));
#133468=CARTESIAN_POINT('Ctrl Pts',(-19.3956401962893,-68.1206960746763,
12.));
#133469=CARTESIAN_POINT('Ctrl Pts',(-19.4074468228294,-68.1387868367668,
12.));
#133470=CARTESIAN_POINT('Ctrl Pts',(-19.4192984819411,-68.1569058475026,
12.));
#133471=CARTESIAN_POINT('Ctrl Pts',(-19.4311951524977,-68.1750529372211,
12.));
#133472=CARTESIAN_POINT('Ctrl Pts',(-19.4431368133718,-68.1932279371121,
12.));
#133473=CARTESIAN_POINT('Ctrl Pts',(-19.4551234434384,-68.2114306792366,
12.));
#133474=CARTESIAN_POINT('Ctrl Pts',(-19.4671550215724,-68.2296609965461,
12.));
#133475=CARTESIAN_POINT('Ctrl Pts',(-19.4792315266505,-68.2479187228815,
12.));
#133476=CARTESIAN_POINT('Ctrl Pts',(-19.4913529375545,-68.2662036929531,
12.));
#133477=CARTESIAN_POINT('Ctrl Pts',(-19.5035192331706,-68.2845157423234,
12.));
#133478=CARTESIAN_POINT('Ctrl Pts',(-19.5157303923856,-68.3028547073862,
12.));
#133479=CARTESIAN_POINT('Ctrl Pts',(-19.5279863940773,-68.3212204253415,
12.));
#133480=CARTESIAN_POINT('Ctrl Pts',(-19.540287217119,-68.3396127341938,
12.));
#133481=CARTESIAN_POINT('Ctrl Pts',(-19.5526328403852,-68.3580314727522,
12.));
#133482=CARTESIAN_POINT('Ctrl Pts',(-19.5650232427516,-68.3764764806287,
12.));
#133483=CARTESIAN_POINT('Ctrl Pts',(-19.5774584030939,-68.3949475982334,
12.));
#133484=CARTESIAN_POINT('Ctrl Pts',(-19.5899383002804,-68.4134446667695,
12.));
#133485=CARTESIAN_POINT('Ctrl Pts',(-19.6024629131786,-68.4319675282273,
12.));
#133486=CARTESIAN_POINT('Ctrl Pts',(-19.6150322206578,-68.4505160253777,
12.));
#133487=CARTESIAN_POINT('Ctrl Pts',(-19.6276462015888,-68.4690900017631,
12.));
#133488=CARTESIAN_POINT('Ctrl Pts',(-19.6403048348397,-68.4876893016863,
12.));
#133489=CARTESIAN_POINT('Ctrl Pts',(-19.653008099269,-68.5063137701986,
12.));
#133490=CARTESIAN_POINT('Ctrl Pts',(-19.665755973734,-68.5249632530994,
12.));
#133491=CARTESIAN_POINT('Ctrl Pts',(-19.6785484370929,-68.543637596932,
12.));
#133492=CARTESIAN_POINT('Ctrl Pts',(-19.6913854682046,-68.5623366489776,
12.));
#133493=CARTESIAN_POINT('Ctrl Pts',(-19.7042670459234,-68.5810602572474,
12.));
#133494=CARTESIAN_POINT('Ctrl Pts',(-19.717193149095,-68.5998082704741,
12.));
#133495=CARTESIAN_POINT('Ctrl Pts',(-19.7301637565646,-68.6185805381102,
12.));
#133496=CARTESIAN_POINT('Ctrl Pts',(-19.7431788471773,-68.6373769103211,
12.));
#133497=CARTESIAN_POINT('Ctrl Pts',(-19.7562383997784,-68.65619723798,12.));
#133498=CARTESIAN_POINT('Ctrl Pts',(-19.7693423932067,-68.6750413726574,
12.));
#133499=CARTESIAN_POINT('Ctrl Pts',(-19.7824908062925,-68.6939091666149,
12.));
#133500=CARTESIAN_POINT('Ctrl Pts',(-19.7956836178651,-68.7128004728033,
12.));
#133501=CARTESIAN_POINT('Ctrl Pts',(-19.8089208067537,-68.7317151448573,
12.));
#133502=CARTESIAN_POINT('Ctrl Pts',(-19.8222023517871,-68.7506530370904,
12.));
#133503=CARTESIAN_POINT('Ctrl Pts',(-19.8355282317858,-68.7696140044851,
12.));
#133504=CARTESIAN_POINT('Ctrl Pts',(-19.8488984255627,-68.7885979026878,
12.));
#133505=CARTESIAN_POINT('Ctrl Pts',(-19.8623129119293,-68.8076045880065,
12.));
#133506=CARTESIAN_POINT('Ctrl Pts',(-19.8757716696965,-68.8266339174056,
12.));
#133507=CARTESIAN_POINT('Ctrl Pts',(-19.8892746776739,-68.8456857485002,
12.));
#133508=CARTESIAN_POINT('Ctrl Pts',(-19.9028219146618,-68.8647599395469,
12.));
#133509=CARTESIAN_POINT('Ctrl Pts',(-19.9164133594526,-68.8838563494393,
12.));
#133510=CARTESIAN_POINT('Ctrl Pts',(-19.9300489908374,-68.9029748377067,
12.));
#133511=CARTESIAN_POINT('Ctrl Pts',(-19.9437287876066,-68.9221152645095,
12.));
#133512=CARTESIAN_POINT('Ctrl Pts',(-19.9574527285488,-68.9412774906333,
12.));
#133513=CARTESIAN_POINT('Ctrl Pts',(-19.9712207924429,-68.9604613774802,
12.));
#133514=CARTESIAN_POINT('Ctrl Pts',(-19.9850329580591,-68.9796667870638,
12.));
#133515=CARTESIAN_POINT('Ctrl Pts',(-19.9988892041666,-68.9988935820084,
12.));
#133516=CARTESIAN_POINT('Ctrl Pts',(-20.0127895095327,-69.0181416255431,
12.));
#133517=CARTESIAN_POINT('Ctrl Pts',(-20.0267338529223,-69.0374107814984,
12.));
#133518=CARTESIAN_POINT('Ctrl Pts',(-20.0407222130906,-69.0567009142978,
12.));
#133519=CARTESIAN_POINT('Ctrl Pts',(-20.0547545687842,-69.0760118889535,
12.));
#133520=CARTESIAN_POINT('Ctrl Pts',(-20.068830898748,-69.095343571064,12.));
#133521=CARTESIAN_POINT('Ctrl Pts',(-20.0829511817251,-69.1146958268104,
12.));
#133522=CARTESIAN_POINT('Ctrl Pts',(-20.0971153964557,-69.1340685229514,
12.));
#133523=CARTESIAN_POINT('Ctrl Pts',(-20.1113235216694,-69.1534615268152,
12.));
#133524=CARTESIAN_POINT('Ctrl Pts',(-20.1255755360872,-69.1728747062963,
12.));
#133525=CARTESIAN_POINT('Ctrl Pts',(-20.139871418428,-69.1923079298538,
12.));
#133526=CARTESIAN_POINT('Ctrl Pts',(-20.1542111474087,-69.2117610665076,
12.));
#133527=CARTESIAN_POINT('Ctrl Pts',(-20.1685947017433,-69.2312339858335,
12.));
#133528=CARTESIAN_POINT('Ctrl Pts',(-20.1830220601349,-69.2507265579554,
12.));
#133529=CARTESIAN_POINT('Ctrl Pts',(-20.1974932012773,-69.2702386535422,
12.));
#133530=CARTESIAN_POINT('Ctrl Pts',(-20.2120081038621,-69.2897701438059,
12.));
#133531=CARTESIAN_POINT('Ctrl Pts',(-20.2265667465784,-69.3093209004984,
12.));
#133532=CARTESIAN_POINT('Ctrl Pts',(-20.2411691081123,-69.3288907959067,
12.));
#133533=CARTESIAN_POINT('Ctrl Pts',(-20.2558151671391,-69.3484797028458,
12.));
#133534=CARTESIAN_POINT('Ctrl Pts',(-20.2705049023241,-69.368087494655,
12.));
#133535=CARTESIAN_POINT('Ctrl Pts',(-20.2852382923299,-69.3877140451975,
12.));
#133536=CARTESIAN_POINT('Ctrl Pts',(-20.3000153158167,-69.407359228856,
12.));
#133537=CARTESIAN_POINT('Ctrl Pts',(-20.3148359514415,-69.4270229205297,
12.));
#133538=CARTESIAN_POINT('Ctrl Pts',(-20.3297001778507,-69.4467049956262,
12.));
#133539=CARTESIAN_POINT('Ctrl Pts',(-20.3446079736802,-69.4664053300587,
12.));
#133540=CARTESIAN_POINT('Ctrl Pts',(-20.3595593175623,-69.4861238002441,
12.));
#133541=CARTESIAN_POINT('Ctrl Pts',(-20.3745541881269,-69.5058602831008,
12.));
#133542=CARTESIAN_POINT('Ctrl Pts',(-20.3895925640005,-69.5256146560441,
12.));
#133543=CARTESIAN_POINT('Ctrl Pts',(-20.4046744237999,-69.5453867969804,
12.));
#133544=CARTESIAN_POINT('Ctrl Pts',(-20.4197997461301,-69.5651765843033,
12.));
#133545=CARTESIAN_POINT('Ctrl Pts',(-20.4349685095924,-69.5849838968928,
12.));
#133546=CARTESIAN_POINT('Ctrl Pts',(-20.4501806927852,-69.6048086141113,
12.));
#133547=CARTESIAN_POINT('Ctrl Pts',(-20.4654362743037,-69.6246506158013,
12.));
#133548=CARTESIAN_POINT('Ctrl Pts',(-20.480735232734,-69.6445097822792,
12.));
#133549=CARTESIAN_POINT('Ctrl Pts',(-20.4960775466492,-69.6643859943308,
12.));
#133550=CARTESIAN_POINT('Ctrl Pts',(-20.5114631946185,-69.6842791332115,
12.));
#133551=CARTESIAN_POINT('Ctrl Pts',(-20.5268921552077,-69.7041890806425,
12.));
#133552=CARTESIAN_POINT('Ctrl Pts',(-20.54236440698,-69.7241157188083,12.));
#133553=CARTESIAN_POINT('Ctrl Pts',(-20.5578799284898,-69.744058930351,
12.));
#133554=CARTESIAN_POINT('Ctrl Pts',(-20.5734386982783,-69.7640185983644,
12.));
#133555=CARTESIAN_POINT('Ctrl Pts',(-20.5890406948811,-69.7839946063949,
12.));
#133556=CARTESIAN_POINT('Ctrl Pts',(-20.6046858968308,-69.8039868384389,
12.));
#133557=CARTESIAN_POINT('Ctrl Pts',(-20.6203742826566,-69.8239951789402,
12.));
#133558=CARTESIAN_POINT('Ctrl Pts',(-20.6361058308811,-69.8440195127866,
12.));
#133559=CARTESIAN_POINT('Ctrl Pts',(-20.6518805200129,-69.8640597253045,
12.));
#133560=CARTESIAN_POINT('Ctrl Pts',(-20.667698328554,-69.8841157022568,
12.));
#133561=CARTESIAN_POINT('Ctrl Pts',(-20.683559235003,-69.904187329841,12.));
#133562=CARTESIAN_POINT('Ctrl Pts',(-20.6994632178552,-69.9242744946854,
12.));
#133563=CARTESIAN_POINT('Ctrl Pts',(-20.7154102555997,-69.9443770838448,
12.));
#133564=CARTESIAN_POINT('Ctrl Pts',(-20.7314003267119,-69.9644949847934,
12.));
#133565=CARTESIAN_POINT('Ctrl Pts',(-20.7474334096581,-69.9846280854257,
12.));
#133566=CARTESIAN_POINT('Ctrl Pts',(-20.7635094829016,-70.0047762740568,
12.));
#133567=CARTESIAN_POINT('Ctrl Pts',(-20.7796285249022,-70.024939439422,
12.));
#133568=CARTESIAN_POINT('Ctrl Pts',(-20.7957905141157,-70.0451174706741,
12.));
#133569=CARTESIAN_POINT('Ctrl Pts',(-20.8119954289849,-70.0653102573803,
12.));
#133570=CARTESIAN_POINT('Ctrl Pts',(-20.8282432479429,-70.0855176895191,
12.));
#133571=CARTESIAN_POINT('Ctrl Pts',(-20.8445339494188,-70.1057396574747,
12.));
#133572=CARTESIAN_POINT('Ctrl Pts',(-20.8608675118379,-70.1259760520309,
12.));
#133573=CARTESIAN_POINT('Ctrl Pts',(-20.8772439136206,-70.1462267643646,
12.));
#133574=CARTESIAN_POINT('Ctrl Pts',(-20.8936631331748,-70.1664916860358,
12.));
#133575=CARTESIAN_POINT('Ctrl Pts',(-20.9101251488944,-70.1867707089854,
12.));
#133576=CARTESIAN_POINT('Ctrl Pts',(-20.9266299391684,-70.2070637255458,
12.));
#133577=CARTESIAN_POINT('Ctrl Pts',(-20.9431774823831,-70.2273706284472,
12.));
#133578=CARTESIAN_POINT('Ctrl Pts',(-20.9597677569228,-70.2476913108244,
12.));
#133579=CARTESIAN_POINT('Ctrl Pts',(-20.9764007411653,-70.2680256662224,
12.));
#133580=CARTESIAN_POINT('Ctrl Pts',(-20.9930764134776,-70.2883735885984,
12.));
#133581=CARTESIAN_POINT('Ctrl Pts',(-21.0097947522218,-70.3087349722973,
12.));
#133582=CARTESIAN_POINT('Ctrl Pts',(-21.0265557357548,-70.3291097120302,
12.));
#133583=CARTESIAN_POINT('Ctrl Pts',(-21.0433593424267,-70.3494977028498,
12.));
#133584=CARTESIAN_POINT('Ctrl Pts',(-21.0602055505748,-70.3698988401281,
12.));
#133585=CARTESIAN_POINT('Ctrl Pts',(-21.0770943385141,-70.3903130195265,
12.));
#133586=CARTESIAN_POINT('Ctrl Pts',(-21.0940256845473,-70.4107401370389,
12.));
#133587=CARTESIAN_POINT('Ctrl Pts',(-21.1109995669747,-70.4311800890401,
12.));
#133588=CARTESIAN_POINT('Ctrl Pts',(-21.1280159641003,-70.4516327723346,
12.));
#133589=CARTESIAN_POINT('Ctrl Pts',(-21.1450748542337,-70.4720980841939,
12.));
#133590=CARTESIAN_POINT('Ctrl Pts',(-21.1621762156897,-70.4925759224216,
12.));
#133591=CARTESIAN_POINT('Ctrl Pts',(-21.1793200267847,-70.5130661852955,
12.));
#133592=CARTESIAN_POINT('Ctrl Pts',(-21.1965062658298,-70.5335687714428,
12.));
#133593=CARTESIAN_POINT('Ctrl Pts',(-21.2137349111208,-70.5540835797283,
12.));
#133594=CARTESIAN_POINT('Ctrl Pts',(-21.2310059409266,-70.5746105091502,
12.));
#133595=CARTESIAN_POINT('Ctrl Pts',(-21.2483193334676,-70.5951494586957,
12.));
#133596=CARTESIAN_POINT('Ctrl Pts',(-21.2656750669126,-70.6157003273316,
12.));
#133597=CARTESIAN_POINT('Ctrl Pts',(-21.2830731194183,-70.6362630143047,
12.));
#133598=CARTESIAN_POINT('Ctrl Pts',(-21.300513469156,-70.6568374193774,
12.));
#133599=CARTESIAN_POINT('Ctrl Pts',(-21.3179960943389,-70.6774234430897,
12.));
#133600=CARTESIAN_POINT('Ctrl Pts',(-21.3355209732443,-70.6980209870045,
12.));
#133601=CARTESIAN_POINT('Ctrl Pts',(-21.3530880842349,-70.7186299539724,
12.));
#133602=CARTESIAN_POINT('Ctrl Pts',(-21.3706974057039,-70.7392502475469,
12.));
#133603=CARTESIAN_POINT('Ctrl Pts',(-21.3883489160196,-70.7598817714105,
12.));
#133604=CARTESIAN_POINT('Ctrl Pts',(-21.4060425934599,-70.780524428745,
12.));
#133605=CARTESIAN_POINT('Ctrl Pts',(-21.4237784161588,-70.8011781217394,
12.));
#133606=CARTESIAN_POINT('Ctrl Pts',(-21.4415563620114,-70.8218427507506,
12.));
#133607=CARTESIAN_POINT('Ctrl Pts',(-21.4593764087474,-70.8425182149846,
12.));
#133608=CARTESIAN_POINT('Ctrl Pts',(-21.477238534096,-70.8632044140112,
12.));
#133609=CARTESIAN_POINT('Ctrl Pts',(-21.4951427159262,-70.8839012490871,
12.));
#133610=CARTESIAN_POINT('Ctrl Pts',(-21.513088932377,-70.9046086244131,
12.));
#133611=CARTESIAN_POINT('Ctrl Pts',(-21.5310771620231,-70.9253264487636,
12.));
#133612=CARTESIAN_POINT('Ctrl Pts',(-21.5491073839106,-70.94605463587,12.));
#133613=CARTESIAN_POINT('Ctrl Pts',(-21.5645987555371,-70.9638315189818,
12.));
#133614=CARTESIAN_POINT('Ctrl Pts',(-21.5764983366483,-70.977466211259,
12.));
#133615=CARTESIAN_POINT('Ctrl Pts',(-21.5847875433335,-70.9869541808058,
12.));
#133616=CARTESIAN_POINT('Ctrl Pts',(-21.5894540925587,-70.9922924595372,
12.));
#133617=CARTESIAN_POINT('Ctrl Pts',(-21.5904919935066,-70.993479606912,
12.));
#133618=CARTESIAN_POINT('',(-18.9407177820969,-67.3887914263118,0.));
#133619=CARTESIAN_POINT('',(-18.9407177820969,-67.3887914263118,0.));
#133620=CARTESIAN_POINT('Ctrl Pts',(-21.5904919935066,-70.993479606912,
0.));
#133621=CARTESIAN_POINT('Ctrl Pts',(-21.5894540925587,-70.9922924595372,
0.));
#133622=CARTESIAN_POINT('Ctrl Pts',(-21.5847875433335,-70.9869541808058,
0.));
#133623=CARTESIAN_POINT('Ctrl Pts',(-21.5764983366483,-70.977466211259,
0.));
#133624=CARTESIAN_POINT('Ctrl Pts',(-21.5645987555371,-70.9638315189818,
0.));
#133625=CARTESIAN_POINT('Ctrl Pts',(-21.5491073839106,-70.94605463587,0.));
#133626=CARTESIAN_POINT('Ctrl Pts',(-21.5310771620231,-70.9253264487636,
0.));
#133627=CARTESIAN_POINT('Ctrl Pts',(-21.513088932377,-70.9046086244131,
0.));
#133628=CARTESIAN_POINT('Ctrl Pts',(-21.4951427159262,-70.8839012490871,
0.));
#133629=CARTESIAN_POINT('Ctrl Pts',(-21.477238534096,-70.8632044140112,
0.));
#133630=CARTESIAN_POINT('Ctrl Pts',(-21.4593764087474,-70.8425182149846,
0.));
#133631=CARTESIAN_POINT('Ctrl Pts',(-21.4415563620114,-70.8218427507506,
0.));
#133632=CARTESIAN_POINT('Ctrl Pts',(-21.4237784161588,-70.8011781217394,
0.));
#133633=CARTESIAN_POINT('Ctrl Pts',(-21.4060425934599,-70.780524428745,
0.));
#133634=CARTESIAN_POINT('Ctrl Pts',(-21.3883489160196,-70.7598817714105,
0.));
#133635=CARTESIAN_POINT('Ctrl Pts',(-21.3706974057039,-70.7392502475469,
0.));
#133636=CARTESIAN_POINT('Ctrl Pts',(-21.3530880842349,-70.7186299539724,
0.));
#133637=CARTESIAN_POINT('Ctrl Pts',(-21.3355209732443,-70.6980209870045,
0.));
#133638=CARTESIAN_POINT('Ctrl Pts',(-21.3179960943389,-70.6774234430897,
0.));
#133639=CARTESIAN_POINT('Ctrl Pts',(-21.300513469156,-70.6568374193774,
0.));
#133640=CARTESIAN_POINT('Ctrl Pts',(-21.2830731194183,-70.6362630143047,
0.));
#133641=CARTESIAN_POINT('Ctrl Pts',(-21.2656750669126,-70.6157003273316,
0.));
#133642=CARTESIAN_POINT('Ctrl Pts',(-21.2483193334676,-70.5951494586957,
0.));
#133643=CARTESIAN_POINT('Ctrl Pts',(-21.2310059409266,-70.5746105091502,
0.));
#133644=CARTESIAN_POINT('Ctrl Pts',(-21.2137349111208,-70.5540835797283,
0.));
#133645=CARTESIAN_POINT('Ctrl Pts',(-21.1965062658298,-70.5335687714428,
0.));
#133646=CARTESIAN_POINT('Ctrl Pts',(-21.1793200267847,-70.5130661852955,
0.));
#133647=CARTESIAN_POINT('Ctrl Pts',(-21.1621762156897,-70.4925759224216,
0.));
#133648=CARTESIAN_POINT('Ctrl Pts',(-21.1450748542337,-70.4720980841939,
0.));
#133649=CARTESIAN_POINT('Ctrl Pts',(-21.1280159641003,-70.4516327723346,
0.));
#133650=CARTESIAN_POINT('Ctrl Pts',(-21.1109995669747,-70.4311800890401,
0.));
#133651=CARTESIAN_POINT('Ctrl Pts',(-21.0940256845473,-70.4107401370389,
0.));
#133652=CARTESIAN_POINT('Ctrl Pts',(-21.0770943385141,-70.3903130195265,
0.));
#133653=CARTESIAN_POINT('Ctrl Pts',(-21.0602055505748,-70.3698988401281,
0.));
#133654=CARTESIAN_POINT('Ctrl Pts',(-21.0433593424267,-70.3494977028498,
0.));
#133655=CARTESIAN_POINT('Ctrl Pts',(-21.0265557357548,-70.3291097120302,
0.));
#133656=CARTESIAN_POINT('Ctrl Pts',(-21.0097947522218,-70.3087349722973,
0.));
#133657=CARTESIAN_POINT('Ctrl Pts',(-20.9930764134776,-70.2883735885984,
0.));
#133658=CARTESIAN_POINT('Ctrl Pts',(-20.9764007411653,-70.2680256662224,
0.));
#133659=CARTESIAN_POINT('Ctrl Pts',(-20.9597677569228,-70.2476913108244,
0.));
#133660=CARTESIAN_POINT('Ctrl Pts',(-20.9431774823831,-70.2273706284472,
0.));
#133661=CARTESIAN_POINT('Ctrl Pts',(-20.9266299391684,-70.2070637255458,
0.));
#133662=CARTESIAN_POINT('Ctrl Pts',(-20.9101251488944,-70.1867707089854,
0.));
#133663=CARTESIAN_POINT('Ctrl Pts',(-20.8936631331748,-70.1664916860358,
0.));
#133664=CARTESIAN_POINT('Ctrl Pts',(-20.8772439136206,-70.1462267643646,
0.));
#133665=CARTESIAN_POINT('Ctrl Pts',(-20.8608675118379,-70.1259760520309,
0.));
#133666=CARTESIAN_POINT('Ctrl Pts',(-20.8445339494188,-70.1057396574747,
0.));
#133667=CARTESIAN_POINT('Ctrl Pts',(-20.8282432479429,-70.0855176895191,
0.));
#133668=CARTESIAN_POINT('Ctrl Pts',(-20.8119954289849,-70.0653102573803,
0.));
#133669=CARTESIAN_POINT('Ctrl Pts',(-20.7957905141157,-70.0451174706741,
0.));
#133670=CARTESIAN_POINT('Ctrl Pts',(-20.7796285249022,-70.024939439422,
0.));
#133671=CARTESIAN_POINT('Ctrl Pts',(-20.7635094829016,-70.0047762740568,
0.));
#133672=CARTESIAN_POINT('Ctrl Pts',(-20.7474334096581,-69.9846280854257,
0.));
#133673=CARTESIAN_POINT('Ctrl Pts',(-20.7314003267119,-69.9644949847934,
0.));
#133674=CARTESIAN_POINT('Ctrl Pts',(-20.7154102555997,-69.9443770838448,
0.));
#133675=CARTESIAN_POINT('Ctrl Pts',(-20.6994632178552,-69.9242744946854,
0.));
#133676=CARTESIAN_POINT('Ctrl Pts',(-20.683559235003,-69.904187329841,0.));
#133677=CARTESIAN_POINT('Ctrl Pts',(-20.667698328554,-69.8841157022568,
0.));
#133678=CARTESIAN_POINT('Ctrl Pts',(-20.6518805200129,-69.8640597253045,
0.));
#133679=CARTESIAN_POINT('Ctrl Pts',(-20.6361058308811,-69.8440195127866,
0.));
#133680=CARTESIAN_POINT('Ctrl Pts',(-20.6203742826566,-69.8239951789402,
0.));
#133681=CARTESIAN_POINT('Ctrl Pts',(-20.6046858968308,-69.8039868384389,
0.));
#133682=CARTESIAN_POINT('Ctrl Pts',(-20.5890406948811,-69.7839946063949,
0.));
#133683=CARTESIAN_POINT('Ctrl Pts',(-20.5734386982783,-69.7640185983644,
0.));
#133684=CARTESIAN_POINT('Ctrl Pts',(-20.5578799284898,-69.744058930351,
0.));
#133685=CARTESIAN_POINT('Ctrl Pts',(-20.54236440698,-69.7241157188083,0.));
#133686=CARTESIAN_POINT('Ctrl Pts',(-20.5268921552077,-69.7041890806425,
0.));
#133687=CARTESIAN_POINT('Ctrl Pts',(-20.5114631946185,-69.6842791332115,
0.));
#133688=CARTESIAN_POINT('Ctrl Pts',(-20.4960775466492,-69.6643859943308,
0.));
#133689=CARTESIAN_POINT('Ctrl Pts',(-20.480735232734,-69.6445097822792,
0.));
#133690=CARTESIAN_POINT('Ctrl Pts',(-20.4654362743037,-69.6246506158013,
0.));
#133691=CARTESIAN_POINT('Ctrl Pts',(-20.4501806927852,-69.6048086141113,
0.));
#133692=CARTESIAN_POINT('Ctrl Pts',(-20.4349685095924,-69.5849838968928,
0.));
#133693=CARTESIAN_POINT('Ctrl Pts',(-20.4197997461301,-69.5651765843033,
0.));
#133694=CARTESIAN_POINT('Ctrl Pts',(-20.4046744237999,-69.5453867969804,
0.));
#133695=CARTESIAN_POINT('Ctrl Pts',(-20.3895925640005,-69.5256146560441,
0.));
#133696=CARTESIAN_POINT('Ctrl Pts',(-20.3745541881269,-69.5058602831008,
0.));
#133697=CARTESIAN_POINT('Ctrl Pts',(-20.3595593175623,-69.4861238002441,
0.));
#133698=CARTESIAN_POINT('Ctrl Pts',(-20.3446079736802,-69.4664053300587,
0.));
#133699=CARTESIAN_POINT('Ctrl Pts',(-20.3297001778507,-69.4467049956262,
0.));
#133700=CARTESIAN_POINT('Ctrl Pts',(-20.3148359514415,-69.4270229205297,
0.));
#133701=CARTESIAN_POINT('Ctrl Pts',(-20.3000153158167,-69.407359228856,
0.));
#133702=CARTESIAN_POINT('Ctrl Pts',(-20.2852382923299,-69.3877140451975,
0.));
#133703=CARTESIAN_POINT('Ctrl Pts',(-20.2705049023241,-69.368087494655,
0.));
#133704=CARTESIAN_POINT('Ctrl Pts',(-20.2558151671391,-69.3484797028458,
0.));
#133705=CARTESIAN_POINT('Ctrl Pts',(-20.2411691081123,-69.3288907959067,
0.));
#133706=CARTESIAN_POINT('Ctrl Pts',(-20.2265667465784,-69.3093209004984,
0.));
#133707=CARTESIAN_POINT('Ctrl Pts',(-20.2120081038621,-69.2897701438059,
0.));
#133708=CARTESIAN_POINT('Ctrl Pts',(-20.1974932012773,-69.2702386535422,
0.));
#133709=CARTESIAN_POINT('Ctrl Pts',(-20.1830220601349,-69.2507265579554,
0.));
#133710=CARTESIAN_POINT('Ctrl Pts',(-20.1685947017433,-69.2312339858335,
0.));
#133711=CARTESIAN_POINT('Ctrl Pts',(-20.1542111474087,-69.2117610665076,
0.));
#133712=CARTESIAN_POINT('Ctrl Pts',(-20.139871418428,-69.1923079298538,
0.));
#133713=CARTESIAN_POINT('Ctrl Pts',(-20.1255755360872,-69.1728747062963,
0.));
#133714=CARTESIAN_POINT('Ctrl Pts',(-20.1113235216694,-69.1534615268152,
0.));
#133715=CARTESIAN_POINT('Ctrl Pts',(-20.0971153964557,-69.1340685229514,
0.));
#133716=CARTESIAN_POINT('Ctrl Pts',(-20.0829511817251,-69.1146958268104,
0.));
#133717=CARTESIAN_POINT('Ctrl Pts',(-20.068830898748,-69.095343571064,0.));
#133718=CARTESIAN_POINT('Ctrl Pts',(-20.0547545687842,-69.0760118889535,
0.));
#133719=CARTESIAN_POINT('Ctrl Pts',(-20.0407222130906,-69.0567009142978,
0.));
#133720=CARTESIAN_POINT('Ctrl Pts',(-20.0267338529223,-69.0374107814984,
0.));
#133721=CARTESIAN_POINT('Ctrl Pts',(-20.0127895095327,-69.0181416255431,
0.));
#133722=CARTESIAN_POINT('Ctrl Pts',(-19.9988892041666,-68.9988935820084,
0.));
#133723=CARTESIAN_POINT('Ctrl Pts',(-19.9850329580591,-68.9796667870638,
0.));
#133724=CARTESIAN_POINT('Ctrl Pts',(-19.9712207924429,-68.9604613774802,
0.));
#133725=CARTESIAN_POINT('Ctrl Pts',(-19.9574527285488,-68.9412774906333,
0.));
#133726=CARTESIAN_POINT('Ctrl Pts',(-19.9437287876066,-68.9221152645095,
0.));
#133727=CARTESIAN_POINT('Ctrl Pts',(-19.9300489908374,-68.9029748377067,
0.));
#133728=CARTESIAN_POINT('Ctrl Pts',(-19.9164133594526,-68.8838563494393,
0.));
#133729=CARTESIAN_POINT('Ctrl Pts',(-19.9028219146618,-68.8647599395469,
0.));
#133730=CARTESIAN_POINT('Ctrl Pts',(-19.8892746776739,-68.8456857485002,
0.));
#133731=CARTESIAN_POINT('Ctrl Pts',(-19.8757716696965,-68.8266339174056,
0.));
#133732=CARTESIAN_POINT('Ctrl Pts',(-19.8623129119293,-68.8076045880065,
0.));
#133733=CARTESIAN_POINT('Ctrl Pts',(-19.8488984255627,-68.7885979026878,
0.));
#133734=CARTESIAN_POINT('Ctrl Pts',(-19.8355282317858,-68.7696140044851,
0.));
#133735=CARTESIAN_POINT('Ctrl Pts',(-19.8222023517871,-68.7506530370904,
0.));
#133736=CARTESIAN_POINT('Ctrl Pts',(-19.8089208067537,-68.7317151448573,
0.));
#133737=CARTESIAN_POINT('Ctrl Pts',(-19.7956836178651,-68.7128004728033,
0.));
#133738=CARTESIAN_POINT('Ctrl Pts',(-19.7824908062925,-68.6939091666149,
0.));
#133739=CARTESIAN_POINT('Ctrl Pts',(-19.7693423932067,-68.6750413726574,
0.));
#133740=CARTESIAN_POINT('Ctrl Pts',(-19.7562383997784,-68.65619723798,0.));
#133741=CARTESIAN_POINT('Ctrl Pts',(-19.7431788471773,-68.6373769103211,
0.));
#133742=CARTESIAN_POINT('Ctrl Pts',(-19.7301637565646,-68.6185805381102,
0.));
#133743=CARTESIAN_POINT('Ctrl Pts',(-19.717193149095,-68.5998082704741,
0.));
#133744=CARTESIAN_POINT('Ctrl Pts',(-19.7042670459234,-68.5810602572474,
0.));
#133745=CARTESIAN_POINT('Ctrl Pts',(-19.6913854682046,-68.5623366489776,
0.));
#133746=CARTESIAN_POINT('Ctrl Pts',(-19.6785484370929,-68.543637596932,
0.));
#133747=CARTESIAN_POINT('Ctrl Pts',(-19.665755973734,-68.5249632530994,
0.));
#133748=CARTESIAN_POINT('Ctrl Pts',(-19.653008099269,-68.5063137701986,
0.));
#133749=CARTESIAN_POINT('Ctrl Pts',(-19.6403048348397,-68.4876893016863,
0.));
#133750=CARTESIAN_POINT('Ctrl Pts',(-19.6276462015888,-68.4690900017631,
0.));
#133751=CARTESIAN_POINT('Ctrl Pts',(-19.6150322206578,-68.4505160253777,
0.));
#133752=CARTESIAN_POINT('Ctrl Pts',(-19.6024629131786,-68.4319675282273,
0.));
#133753=CARTESIAN_POINT('Ctrl Pts',(-19.5899383002804,-68.4134446667695,
0.));
#133754=CARTESIAN_POINT('Ctrl Pts',(-19.5774584030939,-68.3949475982334,
0.));
#133755=CARTESIAN_POINT('Ctrl Pts',(-19.5650232427516,-68.3764764806287,
0.));
#133756=CARTESIAN_POINT('Ctrl Pts',(-19.5526328403852,-68.3580314727522,
0.));
#133757=CARTESIAN_POINT('Ctrl Pts',(-19.540287217119,-68.3396127341938,
0.));
#133758=CARTESIAN_POINT('Ctrl Pts',(-19.5279863940773,-68.3212204253415,
0.));
#133759=CARTESIAN_POINT('Ctrl Pts',(-19.5157303923856,-68.3028547073862,
0.));
#133760=CARTESIAN_POINT('Ctrl Pts',(-19.5035192331706,-68.2845157423234,
0.));
#133761=CARTESIAN_POINT('Ctrl Pts',(-19.4913529375545,-68.2662036929531,
0.));
#133762=CARTESIAN_POINT('Ctrl Pts',(-19.4792315266505,-68.2479187228815,
0.));
#133763=CARTESIAN_POINT('Ctrl Pts',(-19.4671550215724,-68.2296609965461,
0.));
#133764=CARTESIAN_POINT('Ctrl Pts',(-19.4551234434384,-68.2114306792366,
0.));
#133765=CARTESIAN_POINT('Ctrl Pts',(-19.4431368133718,-68.1932279371121,
0.));
#133766=CARTESIAN_POINT('Ctrl Pts',(-19.4311951524977,-68.1750529372211,
0.));
#133767=CARTESIAN_POINT('Ctrl Pts',(-19.4192984819411,-68.1569058475026,
0.));
#133768=CARTESIAN_POINT('Ctrl Pts',(-19.4074468228294,-68.1387868367668,
0.));
#133769=CARTESIAN_POINT('Ctrl Pts',(-19.3956401962893,-68.1206960746763,
0.));
#133770=CARTESIAN_POINT('Ctrl Pts',(-19.3838786234426,-68.1026337317298,
0.));
#133771=CARTESIAN_POINT('Ctrl Pts',(-19.3721621253921,-68.0845999792274,
0.));
#133772=CARTESIAN_POINT('Ctrl Pts',(-19.3604907232322,-68.0665949893222,
0.));
#133773=CARTESIAN_POINT('Ctrl Pts',(-19.3488644380646,-68.0486189351027,
0.));
#133774=CARTESIAN_POINT('Ctrl Pts',(-19.3372832910077,-68.0306719906636,
0.));
#133775=CARTESIAN_POINT('Ctrl Pts',(-19.3257473032031,-68.0127543311761,
0.));
#133776=CARTESIAN_POINT('Ctrl Pts',(-19.3142564958196,-67.9948661329591,
0.));
#133777=CARTESIAN_POINT('Ctrl Pts',(-19.3028108900374,-67.977007573346,
0.));
#133778=CARTESIAN_POINT('Ctrl Pts',(-19.2914105070283,-67.959178830538,
0.));
#133779=CARTESIAN_POINT('Ctrl Pts',(-19.2800553679362,-67.9413800834798,
0.));
#133780=CARTESIAN_POINT('Ctrl Pts',(-19.2687454938449,-67.9236115116781,
0.));
#133781=CARTESIAN_POINT('Ctrl Pts',(-19.2574809057705,-67.9058732951822,
0.));
#133782=CARTESIAN_POINT('Ctrl Pts',(-19.2462616247287,-67.8881656149983,
0.));
#133783=CARTESIAN_POINT('Ctrl Pts',(-19.2350876717878,-67.8704886534555,
0.));
#133784=CARTESIAN_POINT('Ctrl Pts',(-19.223959068113,-67.852842594517,0.));
#133785=CARTESIAN_POINT('Ctrl Pts',(-19.2128758350336,-67.8352276242856,
0.));
#133786=CARTESIAN_POINT('Ctrl Pts',(-19.2018379939918,-67.817643930658,
0.));
#133787=CARTESIAN_POINT('Ctrl Pts',(-19.1908455664089,-67.8000917023896,
0.));
#133788=CARTESIAN_POINT('Ctrl Pts',(-19.1798985735687,-67.7825711283092,
0.));
#133789=CARTESIAN_POINT('Ctrl Pts',(-19.1689970364959,-67.7650823965156,
0.));
#133790=CARTESIAN_POINT('Ctrl Pts',(-19.1581409758112,-67.7476256934492,
0.));
#133791=CARTESIAN_POINT('Ctrl Pts',(-19.1473304119969,-67.7302012056629,
0.));
#133792=CARTESIAN_POINT('Ctrl Pts',(-19.1365653657098,-67.7128091219372,
0.));
#133793=CARTESIAN_POINT('Ctrl Pts',(-19.1258458580343,-67.6954496350053,
0.));
#133794=CARTESIAN_POINT('Ctrl Pts',(-19.115171910845,-67.6781229440535,
0.));
#133795=CARTESIAN_POINT('Ctrl Pts',(-19.1045435468345,-67.6608292549412,
0.));
#133796=CARTESIAN_POINT('Ctrl Pts',(-19.0939607887492,-67.6435687749803,
0.));
#133797=CARTESIAN_POINT('Ctrl Pts',(-19.0834236587115,-67.6263417083414,
0.));
#133798=CARTESIAN_POINT('Ctrl Pts',(-19.0729321776287,-67.6091482520557,
0.));
#133799=CARTESIAN_POINT('Ctrl Pts',(-19.0624863642425,-67.5919885896278,
0.));
#133800=CARTESIAN_POINT('Ctrl Pts',(-19.0520862360414,-67.5748628972035,
0.));
#133801=CARTESIAN_POINT('Ctrl Pts',(-19.0417318110721,-67.5577713558248,
0.));
#133802=CARTESIAN_POINT('Ctrl Pts',(-19.0314231093924,-67.540714161288,
0.));
#133803=CARTESIAN_POINT('Ctrl Pts',(-19.0211601548222,-67.5236915360253,
0.));
#133804=CARTESIAN_POINT('Ctrl Pts',(-19.0109429761274,-67.5067037372177,
0.));
#133805=CARTESIAN_POINT('Ctrl Pts',(-19.0007716032785,-67.4897510316692,
0.));
#133806=CARTESIAN_POINT('Ctrl Pts',(-18.9906460638607,-67.4728336719558,
0.));
#133807=CARTESIAN_POINT('Ctrl Pts',(-18.9805663798466,-67.4559518744714,
0.));
#133808=CARTESIAN_POINT('Ctrl Pts',(-18.9705325631773,-67.4391057908687,
0.));
#133809=CARTESIAN_POINT('Ctrl Pts',(-18.9605446161079,-67.4222955062385,
0.));
#133810=CARTESIAN_POINT('Ctrl Pts',(-18.9525909518003,-67.4088759498287,
0.));
#133811=CARTESIAN_POINT('Ctrl Pts',(-18.9466463414355,-67.398827414689,
0.));
#133812=CARTESIAN_POINT('Ctrl Pts',(-18.942692439874,-67.3921355608417,
0.));
#133813=CARTESIAN_POINT('Ctrl Pts',(-18.9407177820969,-67.3887914263118,
0.));
#133814=CARTESIAN_POINT('Ctrl Pts',(-27.9316983239472,-69.065695021045,
0.));
#133815=CARTESIAN_POINT('Ctrl Pts',(-27.9316983239472,-69.065695021045,
12.));
#133816=CARTESIAN_POINT('Ctrl Pts',(-27.9276214070631,-69.0618620884721,
0.));
#133817=CARTESIAN_POINT('Ctrl Pts',(-27.9276214070631,-69.0618620884721,
12.));
#133818=CARTESIAN_POINT('Ctrl Pts',(-27.9194718099003,-69.0541967851028,
0.));
#133819=CARTESIAN_POINT('Ctrl Pts',(-27.9194718099003,-69.0541967851028,
12.));
#133820=CARTESIAN_POINT('Ctrl Pts',(-27.9072601239722,-69.0427005153791,
0.));
#133821=CARTESIAN_POINT('Ctrl Pts',(-27.9072601239722,-69.0427005153791,
12.));
#133822=CARTESIAN_POINT('Ctrl Pts',(-27.8910032967339,-69.0273755265382,
0.));
#133823=CARTESIAN_POINT('Ctrl Pts',(-27.8910032967339,-69.0273755265382,
12.));
#133824=CARTESIAN_POINT('Ctrl Pts',(-27.8707246380957,-69.0082249138598,
0.));
#133825=CARTESIAN_POINT('Ctrl Pts',(-27.8707246380957,-69.0082249138598,
12.));
#133826=CARTESIAN_POINT('Ctrl Pts',(-27.8504883674059,-68.9890799392213,
0.));
#133827=CARTESIAN_POINT('Ctrl Pts',(-27.8504883674059,-68.9890799392213,
12.));
#133828=CARTESIAN_POINT('Ctrl Pts',(-27.8302945019977,-68.9699406311389,
0.));
#133829=CARTESIAN_POINT('Ctrl Pts',(-27.8302945019977,-68.9699406311389,
12.));
#133830=CARTESIAN_POINT('Ctrl Pts',(-27.8101430638072,-68.9508070357658,
0.));
#133831=CARTESIAN_POINT('Ctrl Pts',(-27.8101430638072,-68.9508070357658,
12.));
#133832=CARTESIAN_POINT('Ctrl Pts',(-27.7900340793689,-68.9316792225946,
0.));
#133833=CARTESIAN_POINT('Ctrl Pts',(-27.7900340793689,-68.9316792225946,
12.));
#133834=CARTESIAN_POINT('Ctrl Pts',(-27.7699675790571,-68.9125572825693,
0.));
#133835=CARTESIAN_POINT('Ctrl Pts',(-27.7699675790571,-68.9125572825693,
12.));
#133836=CARTESIAN_POINT('Ctrl Pts',(-27.7499435957525,-68.8934413203759,
0.));
#133837=CARTESIAN_POINT('Ctrl Pts',(-27.7499435957525,-68.8934413203759,
12.));
#133838=CARTESIAN_POINT('Ctrl Pts',(-27.7299621636566,-68.8743314483369,
0.));
#133839=CARTESIAN_POINT('Ctrl Pts',(-27.7299621636566,-68.8743314483369,
12.));
#133840=CARTESIAN_POINT('Ctrl Pts',(-27.7100233170737,-68.85522777982,0.));
#133841=CARTESIAN_POINT('Ctrl Pts',(-27.7100233170737,-68.85522777982,12.));
#133842=CARTESIAN_POINT('Ctrl Pts',(-27.6901270891241,-68.8361304224467,
0.));
#133843=CARTESIAN_POINT('Ctrl Pts',(-27.6901270891241,-68.8361304224467,
12.));
#133844=CARTESIAN_POINT('Ctrl Pts',(-27.6702735107121,-68.81703947259,0.));
#133845=CARTESIAN_POINT('Ctrl Pts',(-27.6702735107121,-68.81703947259,12.));
#133846=CARTESIAN_POINT('Ctrl Pts',(-27.6504626112666,-68.7979550191872,
0.));
#133847=CARTESIAN_POINT('Ctrl Pts',(-27.6504626112666,-68.7979550191872,
12.));
#133848=CARTESIAN_POINT('Ctrl Pts',(-27.6306944192738,-68.7788771464713,
0.));
#133849=CARTESIAN_POINT('Ctrl Pts',(-27.6306944192738,-68.7788771464713,
12.));
#133850=CARTESIAN_POINT('Ctrl Pts',(-27.6109689629029,-68.7598059372129,
0.));
#133851=CARTESIAN_POINT('Ctrl Pts',(-27.6109689629029,-68.7598059372129,
12.));
#133852=CARTESIAN_POINT('Ctrl Pts',(-27.5912862705469,-68.7407414755259,
0.));
#133853=CARTESIAN_POINT('Ctrl Pts',(-27.5912862705469,-68.7407414755259,
12.));
#133854=CARTESIAN_POINT('Ctrl Pts',(-27.5716463715005,-68.7216838504218,
0.));
#133855=CARTESIAN_POINT('Ctrl Pts',(-27.5716463715005,-68.7216838504218,
12.));
#133856=CARTESIAN_POINT('Ctrl Pts',(-27.5520492958907,-68.7026331554296,
0.));
#133857=CARTESIAN_POINT('Ctrl Pts',(-27.5520492958907,-68.7026331554296,
12.));
#133858=CARTESIAN_POINT('Ctrl Pts',(-27.5324950743706,-68.6835894869882,
0.));
#133859=CARTESIAN_POINT('Ctrl Pts',(-27.5324950743706,-68.6835894869882,
12.));
#133860=CARTESIAN_POINT('Ctrl Pts',(-27.5129837378791,-68.6645529432045,
0.));
#133861=CARTESIAN_POINT('Ctrl Pts',(-27.5129837378791,-68.6645529432045,
12.));
#133862=CARTESIAN_POINT('Ctrl Pts',(-27.4935153173868,-68.645523622548,
0.));
#133863=CARTESIAN_POINT('Ctrl Pts',(-27.4935153173868,-68.645523622548,
12.));
#133864=CARTESIAN_POINT('Ctrl Pts',(-27.4740898435988,-68.6265016223561,
0.));
#133865=CARTESIAN_POINT('Ctrl Pts',(-27.4740898435988,-68.6265016223561,
12.));
#133866=CARTESIAN_POINT('Ctrl Pts',(-27.4547073468227,-68.6074870381619,
0.));
#133867=CARTESIAN_POINT('Ctrl Pts',(-27.4547073468227,-68.6074870381619,
12.));
#133868=CARTESIAN_POINT('Ctrl Pts',(-27.4353678571361,-68.5884799645218,
0.));
#133869=CARTESIAN_POINT('Ctrl Pts',(-27.4353678571361,-68.5884799645218,
12.));
#133870=CARTESIAN_POINT('Ctrl Pts',(-27.4160714044831,-68.5694804955014,
0.));
#133871=CARTESIAN_POINT('Ctrl Pts',(-27.4160714044831,-68.5694804955014,
12.));
#133872=CARTESIAN_POINT('Ctrl Pts',(-27.3968180187941,-68.5504887252975,
0.));
#133873=CARTESIAN_POINT('Ctrl Pts',(-27.3968180187941,-68.5504887252975,
12.));
#133874=CARTESIAN_POINT('Ctrl Pts',(-27.3776077300914,-68.5315047488035,
0.));
#133875=CARTESIAN_POINT('Ctrl Pts',(-27.3776077300914,-68.5315047488035,
12.));
#133876=CARTESIAN_POINT('Ctrl Pts',(-27.3584405685941,-68.5125286621888,
0.));
#133877=CARTESIAN_POINT('Ctrl Pts',(-27.3584405685941,-68.5125286621888,
12.));
#133878=CARTESIAN_POINT('Ctrl Pts',(-27.3393165646748,-68.4935605626361,
0.));
#133879=CARTESIAN_POINT('Ctrl Pts',(-27.3393165646748,-68.4935605626361,
12.));
#133880=CARTESIAN_POINT('Ctrl Pts',(-27.3202357488153,-68.4746005480992,
0.));
#133881=CARTESIAN_POINT('Ctrl Pts',(-27.3202357488153,-68.4746005480992,
12.));
#133882=CARTESIAN_POINT('Ctrl Pts',(-27.301198151557,-68.455648717044,0.));
#133883=CARTESIAN_POINT('Ctrl Pts',(-27.301198151557,-68.455648717044,12.));
#133884=CARTESIAN_POINT('Ctrl Pts',(-27.2822038034539,-68.4367051682166,
0.));
#133885=CARTESIAN_POINT('Ctrl Pts',(-27.2822038034539,-68.4367051682166,
12.));
#133886=CARTESIAN_POINT('Ctrl Pts',(-27.2632527350062,-68.4177700003471,
0.));
#133887=CARTESIAN_POINT('Ctrl Pts',(-27.2632527350062,-68.4177700003471,
12.));
#133888=CARTESIAN_POINT('Ctrl Pts',(-27.2443449766654,-68.3988433121589,
0.));
#133889=CARTESIAN_POINT('Ctrl Pts',(-27.2443449766654,-68.3988433121589,
12.));
#133890=CARTESIAN_POINT('Ctrl Pts',(-27.2254805588677,-68.379925202511,
0.));
#133891=CARTESIAN_POINT('Ctrl Pts',(-27.2254805588677,-68.379925202511,
12.));
#133892=CARTESIAN_POINT('Ctrl Pts',(-27.2066595120544,-68.3610157704999,
0.));
#133893=CARTESIAN_POINT('Ctrl Pts',(-27.2066595120544,-68.3610157704999,
12.));
#133894=CARTESIAN_POINT('Ctrl Pts',(-27.1878818666925,-68.3421151155708,
0.));
#133895=CARTESIAN_POINT('Ctrl Pts',(-27.1878818666925,-68.3421151155708,
12.));
#133896=CARTESIAN_POINT('Ctrl Pts',(-27.1691476532917,-68.3232233376415,
0.));
#133897=CARTESIAN_POINT('Ctrl Pts',(-27.1691476532917,-68.3232233376415,
12.));
#133898=CARTESIAN_POINT('Ctrl Pts',(-27.1504569024131,-68.3043405371589,
0.));
#133899=CARTESIAN_POINT('Ctrl Pts',(-27.1504569024131,-68.3043405371589,
12.));
#133900=CARTESIAN_POINT('Ctrl Pts',(-27.1318096446643,-68.285466815035,
0.));
#133901=CARTESIAN_POINT('Ctrl Pts',(-27.1318096446643,-68.285466815035,
12.));
#133902=CARTESIAN_POINT('Ctrl Pts',(-27.1132059106939,-68.2666022726094,
0.));
#133903=CARTESIAN_POINT('Ctrl Pts',(-27.1132059106939,-68.2666022726094,
12.));
#133904=CARTESIAN_POINT('Ctrl Pts',(-27.0946457311814,-68.2477470116014,
0.));
#133905=CARTESIAN_POINT('Ctrl Pts',(-27.0946457311814,-68.2477470116014,
12.));
#133906=CARTESIAN_POINT('Ctrl Pts',(-27.076129136823,-68.2289011340624,
0.));
#133907=CARTESIAN_POINT('Ctrl Pts',(-27.076129136823,-68.2289011340624,
12.));
#133908=CARTESIAN_POINT('Ctrl Pts',(-27.0576561583179,-68.2100647423345,
0.));
#133909=CARTESIAN_POINT('Ctrl Pts',(-27.0576561583179,-68.2100647423345,
12.));
#133910=CARTESIAN_POINT('Ctrl Pts',(-27.0392268263805,-68.1912379390786,
0.));
#133911=CARTESIAN_POINT('Ctrl Pts',(-27.0392268263805,-68.1912379390786,
12.));
#133912=CARTESIAN_POINT('Ctrl Pts',(-27.0208411717477,-68.1724208272967,
0.));
#133913=CARTESIAN_POINT('Ctrl Pts',(-27.0208411717477,-68.1724208272967,
12.));
#133914=CARTESIAN_POINT('Ctrl Pts',(-27.0024992251839,-68.1536135103558,
0.));
#133915=CARTESIAN_POINT('Ctrl Pts',(-27.0024992251839,-68.1536135103558,
12.));
#133916=CARTESIAN_POINT('Ctrl Pts',(-26.9842010174819,-68.13481609201,0.));
#133917=CARTESIAN_POINT('Ctrl Pts',(-26.9842010174819,-68.13481609201,12.));
#133918=CARTESIAN_POINT('Ctrl Pts',(-26.9659465794596,-68.1160286764244,
0.));
#133919=CARTESIAN_POINT('Ctrl Pts',(-26.9659465794596,-68.1160286764244,
12.));
#133920=CARTESIAN_POINT('Ctrl Pts',(-26.9477359419646,-68.0972513681739,
0.));
#133921=CARTESIAN_POINT('Ctrl Pts',(-26.9477359419646,-68.0972513681739,
12.));
#133922=CARTESIAN_POINT('Ctrl Pts',(-26.9295691358775,-68.0784842722362,
0.));
#133923=CARTESIAN_POINT('Ctrl Pts',(-26.9295691358775,-68.0784842722362,
12.));
#133924=CARTESIAN_POINT('Ctrl Pts',(-26.9114461921109,-68.0597274939857,
0.));
#133925=CARTESIAN_POINT('Ctrl Pts',(-26.9114461921109,-68.0597274939857,
12.));
#133926=CARTESIAN_POINT('Ctrl Pts',(-26.8933671416065,-68.0409811391871,
0.));
#133927=CARTESIAN_POINT('Ctrl Pts',(-26.8933671416065,-68.0409811391871,
12.));
#133928=CARTESIAN_POINT('Ctrl Pts',(-26.8753320153255,-68.0222453139862,
0.));
#133929=CARTESIAN_POINT('Ctrl Pts',(-26.8753320153255,-68.0222453139862,
12.));
#133930=CARTESIAN_POINT('Ctrl Pts',(-26.85734084425,-68.0035201249108,0.));
#133931=CARTESIAN_POINT('Ctrl Pts',(-26.85734084425,-68.0035201249108,12.));
#133932=CARTESIAN_POINT('Ctrl Pts',(-26.8393936593914,-67.9848056788814,
0.));
#133933=CARTESIAN_POINT('Ctrl Pts',(-26.8393936593914,-67.9848056788814,
12.));
#133934=CARTESIAN_POINT('Ctrl Pts',(-26.8214904917922,-67.9661020832165,
0.));
#133935=CARTESIAN_POINT('Ctrl Pts',(-26.8214904917922,-67.9661020832165,
12.));
#133936=CARTESIAN_POINT('Ctrl Pts',(-26.8036313725262,-67.9474094456395,
0.));
#133937=CARTESIAN_POINT('Ctrl Pts',(-26.8036313725262,-67.9474094456395,
12.));
#133938=CARTESIAN_POINT('Ctrl Pts',(-26.7858163326933,-67.9287278742839,
0.));
#133939=CARTESIAN_POINT('Ctrl Pts',(-26.7858163326933,-67.9287278742839,
12.));
#133940=CARTESIAN_POINT('Ctrl Pts',(-26.7680454034169,-67.9100574776974,
0.));
#133941=CARTESIAN_POINT('Ctrl Pts',(-26.7680454034169,-67.9100574776974,
12.));
#133942=CARTESIAN_POINT('Ctrl Pts',(-26.7503186158523,-67.8913983648441,
0.));
#133943=CARTESIAN_POINT('Ctrl Pts',(-26.7503186158523,-67.8913983648441,
12.));
#133944=CARTESIAN_POINT('Ctrl Pts',(-26.7326360011886,-67.8727506451067,
0.));
#133945=CARTESIAN_POINT('Ctrl Pts',(-26.7326360011886,-67.8727506451067,
12.));
#133946=CARTESIAN_POINT('Ctrl Pts',(-26.7149975906478,-67.8541144282875,
0.));
#133947=CARTESIAN_POINT('Ctrl Pts',(-26.7149975906478,-67.8541144282875,
12.));
#133948=CARTESIAN_POINT('Ctrl Pts',(-26.6974034154803,-67.8354898246079,
0.));
#133949=CARTESIAN_POINT('Ctrl Pts',(-26.6974034154803,-67.8354898246079,
12.));
#133950=CARTESIAN_POINT('Ctrl Pts',(-26.6798535069586,-67.8168769447086,
0.));
#133951=CARTESIAN_POINT('Ctrl Pts',(-26.6798535069586,-67.8168769447086,
12.));
#133952=CARTESIAN_POINT('Ctrl Pts',(-26.6623478963867,-67.7982758996557,
0.));
#133953=CARTESIAN_POINT('Ctrl Pts',(-26.6623478963867,-67.7982758996557,
12.));
#133954=CARTESIAN_POINT('Ctrl Pts',(-26.6448866151027,-67.7796868009447,
0.));
#133955=CARTESIAN_POINT('Ctrl Pts',(-26.6448866151027,-67.7796868009447,
12.));
#133956=CARTESIAN_POINT('Ctrl Pts',(-26.6274696944793,-67.7611097605042,
0.));
#133957=CARTESIAN_POINT('Ctrl Pts',(-26.6274696944793,-67.7611097605042,
12.));
#133958=CARTESIAN_POINT('Ctrl Pts',(-26.6100971659205,-67.7425448906983,
0.));
#133959=CARTESIAN_POINT('Ctrl Pts',(-26.6100971659205,-67.7425448906983,
12.));
#133960=CARTESIAN_POINT('Ctrl Pts',(-26.5927690608547,-67.7239923043295,
0.));
#133961=CARTESIAN_POINT('Ctrl Pts',(-26.5927690608547,-67.7239923043295,
12.));
#133962=CARTESIAN_POINT('Ctrl Pts',(-26.5754854107422,-67.7054521146427,
0.));
#133963=CARTESIAN_POINT('Ctrl Pts',(-26.5754854107422,-67.7054521146427,
12.));
#133964=CARTESIAN_POINT('Ctrl Pts',(-26.5582462470794,-67.6869244353292,
0.));
#133965=CARTESIAN_POINT('Ctrl Pts',(-26.5582462470794,-67.6869244353292,
12.));
#133966=CARTESIAN_POINT('Ctrl Pts',(-26.5410516013984,-67.6684093805288,
0.));
#133967=CARTESIAN_POINT('Ctrl Pts',(-26.5410516013984,-67.6684093805288,
12.));
#133968=CARTESIAN_POINT('Ctrl Pts',(-26.5239015052656,-67.6499070648323,
0.));
#133969=CARTESIAN_POINT('Ctrl Pts',(-26.5239015052656,-67.6499070648323,
12.));
#133970=CARTESIAN_POINT('Ctrl Pts',(-26.5067959902731,-67.6314176032823,
0.));
#133971=CARTESIAN_POINT('Ctrl Pts',(-26.5067959902731,-67.6314176032823,
12.));
#133972=CARTESIAN_POINT('Ctrl Pts',(-26.4897350880447,-67.6129411113774,
0.));
#133973=CARTESIAN_POINT('Ctrl Pts',(-26.4897350880447,-67.6129411113774,
12.));
#133974=CARTESIAN_POINT('Ctrl Pts',(-26.4727188302415,-67.5944777050782,
0.));
#133975=CARTESIAN_POINT('Ctrl Pts',(-26.4727188302415,-67.5944777050782,
12.));
#133976=CARTESIAN_POINT('Ctrl Pts',(-26.4557472485622,-67.5760275008096,
0.));
#133977=CARTESIAN_POINT('Ctrl Pts',(-26.4557472485622,-67.5760275008096,
12.));
#133978=CARTESIAN_POINT('Ctrl Pts',(-26.4388203747422,-67.5575906154648,
0.));
#133979=CARTESIAN_POINT('Ctrl Pts',(-26.4388203747422,-67.5575906154648,
12.));
#133980=CARTESIAN_POINT('Ctrl Pts',(-26.4219382405452,-67.5391671664055,
0.));
#133981=CARTESIAN_POINT('Ctrl Pts',(-26.4219382405452,-67.5391671664055,
12.));
#133982=CARTESIAN_POINT('Ctrl Pts',(-26.4051008777669,-67.5207572714666,
0.));
#133983=CARTESIAN_POINT('Ctrl Pts',(-26.4051008777669,-67.5207572714666,
12.));
#133984=CARTESIAN_POINT('Ctrl Pts',(-26.3883083182417,-67.5023610489611,
0.));
#133985=CARTESIAN_POINT('Ctrl Pts',(-26.3883083182417,-67.5023610489611,
12.));
#133986=CARTESIAN_POINT('Ctrl Pts',(-26.3715605938432,-67.4839786176833,
0.));
#133987=CARTESIAN_POINT('Ctrl Pts',(-26.3715605938432,-67.4839786176833,
12.));
#133988=CARTESIAN_POINT('Ctrl Pts',(-26.3548577364835,-67.4656100969121,
0.));
#133989=CARTESIAN_POINT('Ctrl Pts',(-26.3548577364835,-67.4656100969121,
12.));
#133990=CARTESIAN_POINT('Ctrl Pts',(-26.3381997781059,-67.4472556064127,
0.));
#133991=CARTESIAN_POINT('Ctrl Pts',(-26.3381997781059,-67.4472556064127,
12.));
#133992=CARTESIAN_POINT('Ctrl Pts',(-26.3215867506864,-67.4289152664406,
0.));
#133993=CARTESIAN_POINT('Ctrl Pts',(-26.3215867506864,-67.4289152664406,
12.));
#133994=CARTESIAN_POINT('Ctrl Pts',(-26.305018686241,-67.4105891977465,
0.));
#133995=CARTESIAN_POINT('Ctrl Pts',(-26.305018686241,-67.4105891977465,
12.));
#133996=CARTESIAN_POINT('Ctrl Pts',(-26.288495616827,-67.392277521581,0.));
#133997=CARTESIAN_POINT('Ctrl Pts',(-26.288495616827,-67.392277521581,12.));
#133998=CARTESIAN_POINT('Ctrl Pts',(-26.2720175745423,-67.3739803596967,
0.));
#133999=CARTESIAN_POINT('Ctrl Pts',(-26.2720175745423,-67.3739803596967,
12.));
#134000=CARTESIAN_POINT('Ctrl Pts',(-26.255584591518,-67.3556978343506,
0.));
#134001=CARTESIAN_POINT('Ctrl Pts',(-26.255584591518,-67.3556978343506,
12.));
#134002=CARTESIAN_POINT('Ctrl Pts',(-26.2391966999192,-67.3374300683075,
0.));
#134003=CARTESIAN_POINT('Ctrl Pts',(-26.2391966999192,-67.3374300683075,
12.));
#134004=CARTESIAN_POINT('Ctrl Pts',(-26.2228539319528,-67.3191771848468,
0.));
#134005=CARTESIAN_POINT('Ctrl Pts',(-26.2228539319528,-67.3191771848468,
12.));
#134006=CARTESIAN_POINT('Ctrl Pts',(-26.2065563198685,-67.3009393077654,
0.));
#134007=CARTESIAN_POINT('Ctrl Pts',(-26.2065563198685,-67.3009393077654,
12.));
#134008=CARTESIAN_POINT('Ctrl Pts',(-26.1903038959589,-67.2827165613828,
0.));
#134009=CARTESIAN_POINT('Ctrl Pts',(-26.1903038959589,-67.2827165613828,
12.));
#134010=CARTESIAN_POINT('Ctrl Pts',(-26.1740966925527,-67.2645090705414,
0.));
#134011=CARTESIAN_POINT('Ctrl Pts',(-26.1740966925527,-67.2645090705414,
12.));
#134012=CARTESIAN_POINT('Ctrl Pts',(-26.1579347420135,-67.2463169606105,
0.));
#134013=CARTESIAN_POINT('Ctrl Pts',(-26.1579347420135,-67.2463169606105,
12.));
#134014=CARTESIAN_POINT('Ctrl Pts',(-26.1418180767487,-67.228140357493,
0.));
#134015=CARTESIAN_POINT('Ctrl Pts',(-26.1418180767487,-67.228140357493,
12.));
#134016=CARTESIAN_POINT('Ctrl Pts',(-26.1257467292102,-67.2099793876295,
0.));
#134017=CARTESIAN_POINT('Ctrl Pts',(-26.1257467292102,-67.2099793876295,
12.));
#134018=CARTESIAN_POINT('Ctrl Pts',(-26.109720731895,-67.191834178002,0.));
#134019=CARTESIAN_POINT('Ctrl Pts',(-26.109720731895,-67.191834178002,12.));
#134020=CARTESIAN_POINT('Ctrl Pts',(-26.0937401173385,-67.1737048561364,
0.));
#134021=CARTESIAN_POINT('Ctrl Pts',(-26.0937401173385,-67.1737048561364,
12.));
#134022=CARTESIAN_POINT('Ctrl Pts',(-26.077804918113,-67.1555915501052,
0.));
#134023=CARTESIAN_POINT('Ctrl Pts',(-26.077804918113,-67.1555915501052,
12.));
#134024=CARTESIAN_POINT('Ctrl Pts',(-26.0619151668361,-67.1374943885353,
0.));
#134025=CARTESIAN_POINT('Ctrl Pts',(-26.0619151668361,-67.1374943885353,
12.));
#134026=CARTESIAN_POINT('Ctrl Pts',(-26.0460708961725,-67.1194135006121,
0.));
#134027=CARTESIAN_POINT('Ctrl Pts',(-26.0460708961725,-67.1194135006121,
12.));
#134028=CARTESIAN_POINT('Ctrl Pts',(-26.030272138834,-67.101349016084,0.));
#134029=CARTESIAN_POINT('Ctrl Pts',(-26.030272138834,-67.101349016084,12.));
#134030=CARTESIAN_POINT('Ctrl Pts',(-26.0145189275733,-67.083301065264,
0.));
#134031=CARTESIAN_POINT('Ctrl Pts',(-26.0145189275733,-67.083301065264,
12.));
#134032=CARTESIAN_POINT('Ctrl Pts',(-25.9988112951818,-67.0652697790335,
0.));
#134033=CARTESIAN_POINT('Ctrl Pts',(-25.9988112951818,-67.0652697790335,
12.));
#134034=CARTESIAN_POINT('Ctrl Pts',(-25.9831492744988,-67.0472552888495,
0.));
#134035=CARTESIAN_POINT('Ctrl Pts',(-25.9831492744988,-67.0472552888495,
12.));
#134036=CARTESIAN_POINT('Ctrl Pts',(-25.9675328984123,-67.0292577267495,
0.));
#134037=CARTESIAN_POINT('Ctrl Pts',(-25.9675328984123,-67.0292577267495,
12.));
#134038=CARTESIAN_POINT('Ctrl Pts',(-25.9519621998598,-67.0112772253553,
0.));
#134039=CARTESIAN_POINT('Ctrl Pts',(-25.9519621998598,-67.0112772253553,
12.));
#134040=CARTESIAN_POINT('Ctrl Pts',(-25.9364372118216,-66.993313917876,
0.));
#134041=CARTESIAN_POINT('Ctrl Pts',(-25.9364372118216,-66.993313917876,
12.));
#134042=CARTESIAN_POINT('Ctrl Pts',(-25.9209579673198,-66.9753679381122,
0.));
#134043=CARTESIAN_POINT('Ctrl Pts',(-25.9209579673198,-66.9753679381122,
12.));
#134044=CARTESIAN_POINT('Ctrl Pts',(-25.9055244994267,-66.9574394204635,
0.));
#134045=CARTESIAN_POINT('Ctrl Pts',(-25.9055244994267,-66.9574394204635,
12.));
#134046=CARTESIAN_POINT('Ctrl Pts',(-25.8901368412655,-66.9395284999327,
0.));
#134047=CARTESIAN_POINT('Ctrl Pts',(-25.8901368412655,-66.9395284999327,
12.));
#134048=CARTESIAN_POINT('Ctrl Pts',(-25.8747950260114,-66.9216353121308,
0.));
#134049=CARTESIAN_POINT('Ctrl Pts',(-25.8747950260114,-66.9216353121308,
12.));
#134050=CARTESIAN_POINT('Ctrl Pts',(-25.8594990868845,-66.9037599932787,
0.));
#134051=CARTESIAN_POINT('Ctrl Pts',(-25.8594990868845,-66.9037599932787,
12.));
#134052=CARTESIAN_POINT('Ctrl Pts',(-25.8442490571486,-66.8859026802123,
0.));
#134053=CARTESIAN_POINT('Ctrl Pts',(-25.8442490571486,-66.8859026802123,
12.));
#134054=CARTESIAN_POINT('Ctrl Pts',(-25.8290449701207,-66.8680635103907,
0.));
#134055=CARTESIAN_POINT('Ctrl Pts',(-25.8290449701207,-66.8680635103907,
12.));
#134056=CARTESIAN_POINT('Ctrl Pts',(-25.8138868591715,-66.8502426219015,
0.));
#134057=CARTESIAN_POINT('Ctrl Pts',(-25.8138868591715,-66.8502426219015,
12.));
#134058=CARTESIAN_POINT('Ctrl Pts',(-25.7987747577265,-66.8324401534657,
0.));
#134059=CARTESIAN_POINT('Ctrl Pts',(-25.7987747577265,-66.8324401534657,
12.));
#134060=CARTESIAN_POINT('Ctrl Pts',(-25.783708699258,-66.8146562444397,
0.));
#134061=CARTESIAN_POINT('Ctrl Pts',(-25.783708699258,-66.8146562444397,
12.));
#134062=CARTESIAN_POINT('Ctrl Pts',(-25.7686887172859,-66.7968910348199,
0.));
#134063=CARTESIAN_POINT('Ctrl Pts',(-25.7686887172859,-66.7968910348199,
12.));
#134064=CARTESIAN_POINT('Ctrl Pts',(-25.7537148453848,-66.7791446652505,
0.));
#134065=CARTESIAN_POINT('Ctrl Pts',(-25.7537148453848,-66.7791446652505,
12.));
#134066=CARTESIAN_POINT('Ctrl Pts',(-25.7387871171861,-66.7614172770302,
0.));
#134067=CARTESIAN_POINT('Ctrl Pts',(-25.7387871171861,-66.7614172770302,
12.));
#134068=CARTESIAN_POINT('Ctrl Pts',(-25.7239055663778,-66.7437090121168,
0.));
#134069=CARTESIAN_POINT('Ctrl Pts',(-25.7239055663778,-66.7437090121168,
12.));
#134070=CARTESIAN_POINT('Ctrl Pts',(-25.7090702266976,-66.72602001313,0.));
#134071=CARTESIAN_POINT('Ctrl Pts',(-25.7090702266976,-66.72602001313,12.));
#134072=CARTESIAN_POINT('Ctrl Pts',(-25.6942811319337,-66.7083504233566,
0.));
#134073=CARTESIAN_POINT('Ctrl Pts',(-25.6942811319337,-66.7083504233566,
12.));
#134074=CARTESIAN_POINT('Ctrl Pts',(-25.679538315933,-66.6907003867599,
0.));
#134075=CARTESIAN_POINT('Ctrl Pts',(-25.679538315933,-66.6907003867599,
12.));
#134076=CARTESIAN_POINT('Ctrl Pts',(-25.6648418126016,-66.6730700479843,
0.));
#134077=CARTESIAN_POINT('Ctrl Pts',(-25.6648418126016,-66.6730700479843,
12.));
#134078=CARTESIAN_POINT('Ctrl Pts',(-25.6501916559051,-66.6554595523611,
0.));
#134079=CARTESIAN_POINT('Ctrl Pts',(-25.6501916559051,-66.6554595523611,
12.));
#134080=CARTESIAN_POINT('Ctrl Pts',(-25.6355878798605,-66.6378690459105,
0.));
#134081=CARTESIAN_POINT('Ctrl Pts',(-25.6355878798605,-66.6378690459105,
12.));
#134082=CARTESIAN_POINT('Ctrl Pts',(-25.6210305185395,-66.6202986753482,
0.));
#134083=CARTESIAN_POINT('Ctrl Pts',(-25.6210305185395,-66.6202986753482,
12.));
#134084=CARTESIAN_POINT('Ctrl Pts',(-25.606519606075,-66.6027485880947,
0.));
#134085=CARTESIAN_POINT('Ctrl Pts',(-25.606519606075,-66.6027485880947,
12.));
#134086=CARTESIAN_POINT('Ctrl Pts',(-25.5920551766629,-66.585218932281,
0.));
#134087=CARTESIAN_POINT('Ctrl Pts',(-25.5920551766629,-66.585218932281,
12.));
#134088=CARTESIAN_POINT('Ctrl Pts',(-25.5776372645605,-66.567709856755,
0.));
#134089=CARTESIAN_POINT('Ctrl Pts',(-25.5776372645605,-66.567709856755,
12.));
#134090=CARTESIAN_POINT('Ctrl Pts',(-25.5632659040797,-66.5502215110843,
0.));
#134091=CARTESIAN_POINT('Ctrl Pts',(-25.5632659040797,-66.5502215110843,
12.));
#134092=CARTESIAN_POINT('Ctrl Pts',(-25.5489411295916,-66.5327540455638,
0.));
#134093=CARTESIAN_POINT('Ctrl Pts',(-25.5489411295916,-66.5327540455638,
12.));
#134094=CARTESIAN_POINT('Ctrl Pts',(-25.5346629755322,-66.5153076112237,
0.));
#134095=CARTESIAN_POINT('Ctrl Pts',(-25.5346629755322,-66.5153076112237,
12.));
#134096=CARTESIAN_POINT('Ctrl Pts',(-25.5204314764033,-66.4978823598352,
0.));
#134097=CARTESIAN_POINT('Ctrl Pts',(-25.5204314764033,-66.4978823598352,
12.));
#134098=CARTESIAN_POINT('Ctrl Pts',(-25.5062466667703,-66.4804784439146,
0.));
#134099=CARTESIAN_POINT('Ctrl Pts',(-25.5062466667703,-66.4804784439146,
12.));
#134100=CARTESIAN_POINT('Ctrl Pts',(-25.4921085812548,-66.463096016725,
0.));
#134101=CARTESIAN_POINT('Ctrl Pts',(-25.4921085812548,-66.463096016725,
12.));
#134102=CARTESIAN_POINT('Ctrl Pts',(-25.4780172545418,-66.445735232287,
0.));
#134103=CARTESIAN_POINT('Ctrl Pts',(-25.4780172545418,-66.445735232287,
12.));
#134104=CARTESIAN_POINT('Ctrl Pts',(-25.463972721385,-66.4283962453899,
0.));
#134105=CARTESIAN_POINT('Ctrl Pts',(-25.463972721385,-66.4283962453899,
12.));
#134106=CARTESIAN_POINT('Ctrl Pts',(-25.4499750166079,-66.4110792116,0.));
#134107=CARTESIAN_POINT('Ctrl Pts',(-25.4499750166079,-66.4110792116,12.));
#134108=CARTESIAN_POINT('Ctrl Pts',(-25.4360241751017,-66.3937842872684,
0.));
#134109=CARTESIAN_POINT('Ctrl Pts',(-25.4360241751017,-66.3937842872684,
12.));
#134110=CARTESIAN_POINT('Ctrl Pts',(-25.4221202318198,-66.3765116295363,
0.));
#134111=CARTESIAN_POINT('Ctrl Pts',(-25.4221202318198,-66.3765116295363,
12.));
#134112=CARTESIAN_POINT('Ctrl Pts',(-25.4082632217846,-66.3592613963407,
0.));
#134113=CARTESIAN_POINT('Ctrl Pts',(-25.4082632217846,-66.3592613963407,
12.));
#134114=CARTESIAN_POINT('Ctrl Pts',(-25.3944531800901,-66.3420337464176,
0.));
#134115=CARTESIAN_POINT('Ctrl Pts',(-25.3944531800901,-66.3420337464176,
12.));
#134116=CARTESIAN_POINT('Ctrl Pts',(-25.3806901419013,-66.3248288393046,
0.));
#134117=CARTESIAN_POINT('Ctrl Pts',(-25.3806901419013,-66.3248288393046,
12.));
#134118=CARTESIAN_POINT('Ctrl Pts',(-25.3669741424491,-66.3076468353417,
0.));
#134119=CARTESIAN_POINT('Ctrl Pts',(-25.3669741424491,-66.3076468353417,
12.));
#134120=CARTESIAN_POINT('Ctrl Pts',(-25.3533052170254,-66.2904878956721,
0.));
#134121=CARTESIAN_POINT('Ctrl Pts',(-25.3533052170254,-66.2904878956721,
12.));
#134122=CARTESIAN_POINT('Ctrl Pts',(-25.3396834009955,-66.2733521822675,
0.));
#134123=CARTESIAN_POINT('Ctrl Pts',(-25.3396834009955,-66.2733521822675,
12.));
#134124=CARTESIAN_POINT('Ctrl Pts',(-25.326108729803,-66.2562398579479,
0.));
#134125=CARTESIAN_POINT('Ctrl Pts',(-25.326108729803,-66.2562398579479,
12.));
#134126=CARTESIAN_POINT('Ctrl Pts',(-25.3125812389728,-66.2391510863992,
0.));
#134127=CARTESIAN_POINT('Ctrl Pts',(-25.3125812389728,-66.2391510863992,
12.));
#134128=CARTESIAN_POINT('Ctrl Pts',(-25.2991009641087,-66.222086032193,
0.));
#134129=CARTESIAN_POINT('Ctrl Pts',(-25.2991009641087,-66.222086032193,
12.));
#134130=CARTESIAN_POINT('Ctrl Pts',(-25.2856679408921,-66.2050448607883,
0.));
#134131=CARTESIAN_POINT('Ctrl Pts',(-25.2856679408921,-66.2050448607883,
12.));
#134132=CARTESIAN_POINT('Ctrl Pts',(-25.2722822050829,-66.1880277385113,
0.));
#134133=CARTESIAN_POINT('Ctrl Pts',(-25.2722822050829,-66.1880277385113,
12.));
#134134=CARTESIAN_POINT('Ctrl Pts',(-25.2589437925145,-66.1710348325378,
0.));
#134135=CARTESIAN_POINT('Ctrl Pts',(-25.2589437925145,-66.1710348325378,
12.));
#134136=CARTESIAN_POINT('Ctrl Pts',(-25.245652739088,-66.1540663108767,
0.));
#134137=CARTESIAN_POINT('Ctrl Pts',(-25.245652739088,-66.1540663108767,
12.));
#134138=CARTESIAN_POINT('Ctrl Pts',(-25.2324090807561,-66.1371223423371,
0.));
#134139=CARTESIAN_POINT('Ctrl Pts',(-25.2324090807561,-66.1371223423371,
12.));
#134140=CARTESIAN_POINT('Ctrl Pts',(-25.2192128535367,-66.1202030965784,
0.));
#134141=CARTESIAN_POINT('Ctrl Pts',(-25.2192128535367,-66.1202030965784,
12.));
#134142=CARTESIAN_POINT('Ctrl Pts',(-25.2060640935371,-66.1033087441916,
0.));
#134143=CARTESIAN_POINT('Ctrl Pts',(-25.2060640935371,-66.1033087441916,
12.));
#134144=CARTESIAN_POINT('Ctrl Pts',(-25.1929628369685,-66.086439456768,
0.));
#134145=CARTESIAN_POINT('Ctrl Pts',(-25.1929628369685,-66.086439456768,
12.));
#134146=CARTESIAN_POINT('Ctrl Pts',(-25.1799091201594,-66.0695954069698,
0.));
#134147=CARTESIAN_POINT('Ctrl Pts',(-25.1799091201594,-66.0695954069698,
12.));
#134148=CARTESIAN_POINT('Ctrl Pts',(-25.1669029795652,-66.0527767686,0.));
#134149=CARTESIAN_POINT('Ctrl Pts',(-25.1669029795652,-66.0527767686,12.));
#134150=CARTESIAN_POINT('Ctrl Pts',(-25.153944451741,-66.0359837164709,
0.));
#134151=CARTESIAN_POINT('Ctrl Pts',(-25.153944451741,-66.0359837164709,
12.));
#134152=CARTESIAN_POINT('Ctrl Pts',(-25.1410335733094,-66.0192164262607,
0.));
#134153=CARTESIAN_POINT('Ctrl Pts',(-25.1410335733094,-66.0192164262607,
12.));
#134154=CARTESIAN_POINT('Ctrl Pts',(-25.12817038093,-66.0024750743902,0.));
#134155=CARTESIAN_POINT('Ctrl Pts',(-25.12817038093,-66.0024750743902,12.));
#134156=CARTESIAN_POINT('Ctrl Pts',(-25.1153549112512,-65.9857598378455,
0.));
#134157=CARTESIAN_POINT('Ctrl Pts',(-25.1153549112512,-65.9857598378455,
12.));
#134158=CARTESIAN_POINT('Ctrl Pts',(-25.1025872009016,-65.9690708941591,
0.));
#134159=CARTESIAN_POINT('Ctrl Pts',(-25.1025872009016,-65.9690708941591,
12.));
#134160=CARTESIAN_POINT('Ctrl Pts',(-25.0898672865926,-65.9524084218167,
0.));
#134161=CARTESIAN_POINT('Ctrl Pts',(-25.0898672865926,-65.9524084218167,
12.));
#134162=CARTESIAN_POINT('Ctrl Pts',(-25.0771952052033,-65.9357726006174,
0.));
#134163=CARTESIAN_POINT('Ctrl Pts',(-25.0771952052033,-65.9357726006174,
12.));
#134164=CARTESIAN_POINT('Ctrl Pts',(-25.0645709938519,-65.9191636119796,
0.));
#134165=CARTESIAN_POINT('Ctrl Pts',(-25.0645709938519,-65.9191636119796,
12.));
#134166=CARTESIAN_POINT('Ctrl Pts',(-25.0519946900066,-65.9025816394391,
0.));
#134167=CARTESIAN_POINT('Ctrl Pts',(-25.0519946900066,-65.9025816394391,
12.));
#134168=CARTESIAN_POINT('Ctrl Pts',(-25.039466331404,-65.8860268683088,
0.));
#134169=CARTESIAN_POINT('Ctrl Pts',(-25.039466331404,-65.8860268683088,
12.));
#134170=CARTESIAN_POINT('Ctrl Pts',(-25.0269859558351,-65.8694994847586,
0.));
#134171=CARTESIAN_POINT('Ctrl Pts',(-25.0269859558351,-65.8694994847586,
12.));
#134172=CARTESIAN_POINT('Ctrl Pts',(-25.0145536009603,-65.8529996750441,
0.));
#134173=CARTESIAN_POINT('Ctrl Pts',(-25.0145536009603,-65.8529996750441,
12.));
#134174=CARTESIAN_POINT('Ctrl Pts',(-25.0021693041181,-65.8365276247157,
0.));
#134175=CARTESIAN_POINT('Ctrl Pts',(-25.0021693041181,-65.8365276247157,
12.));
#134176=CARTESIAN_POINT('Ctrl Pts',(-24.9898331021002,-65.8200835177071,
0.));
#134177=CARTESIAN_POINT('Ctrl Pts',(-24.9898331021002,-65.8200835177071,
12.));
#134178=CARTESIAN_POINT('Ctrl Pts',(-24.97754503157,-65.8036675380761,0.));
#134179=CARTESIAN_POINT('Ctrl Pts',(-24.97754503157,-65.8036675380761,12.));
#134180=CARTESIAN_POINT('Ctrl Pts',(-24.965305129559,-65.7872798720847,
0.));
#134181=CARTESIAN_POINT('Ctrl Pts',(-24.965305129559,-65.7872798720847,
12.));
#134182=CARTESIAN_POINT('Ctrl Pts',(-24.9531134338693,-65.7709207098949,
0.));
#134183=CARTESIAN_POINT('Ctrl Pts',(-24.9531134338693,-65.7709207098949,
12.));
#134184=CARTESIAN_POINT('Ctrl Pts',(-24.9409699836523,-65.7545902480286,
0.));
#134185=CARTESIAN_POINT('Ctrl Pts',(-24.9409699836523,-65.7545902480286,
12.));
#134186=CARTESIAN_POINT('Ctrl Pts',(-24.9288748194562,-65.7382886895839,
0.));
#134187=CARTESIAN_POINT('Ctrl Pts',(-24.9288748194562,-65.7382886895839,
12.));
#134188=CARTESIAN_POINT('Ctrl Pts',(-24.9168279820093,-65.7220162391016,
0.));
#134189=CARTESIAN_POINT('Ctrl Pts',(-24.9168279820093,-65.7220162391016,
12.));
#134190=CARTESIAN_POINT('Ctrl Pts',(-24.9048295111444,-65.7057730980471,
0.));
#134191=CARTESIAN_POINT('Ctrl Pts',(-24.9048295111444,-65.7057730980471,
12.));
#134192=CARTESIAN_POINT('Ctrl Pts',(-24.8928794448616,-65.6895594608798,
0.));
#134193=CARTESIAN_POINT('Ctrl Pts',(-24.8928794448616,-65.6895594608798,
12.));
#134194=CARTESIAN_POINT('Ctrl Pts',(-24.8809778178248,-65.6733755087723,
0.));
#134195=CARTESIAN_POINT('Ctrl Pts',(-24.8809778178248,-65.6733755087723,
12.));
#134196=CARTESIAN_POINT('Ctrl Pts',(-24.8691246628081,-65.6572214156761,
0.));
#134197=CARTESIAN_POINT('Ctrl Pts',(-24.8691246628081,-65.6572214156761,
12.));
#134198=CARTESIAN_POINT('Ctrl Pts',(-24.8573200135684,-65.6410973603713,
0.));
#134199=CARTESIAN_POINT('Ctrl Pts',(-24.8573200135684,-65.6410973603713,
12.));
#134200=CARTESIAN_POINT('Ctrl Pts',(-24.8455639071517,-65.6250035361612,
0.));
#134201=CARTESIAN_POINT('Ctrl Pts',(-24.8455639071517,-65.6250035361612,
12.));
#134202=CARTESIAN_POINT('Ctrl Pts',(-24.8338563866739,-65.6089401625551,
0.));
#134203=CARTESIAN_POINT('Ctrl Pts',(-24.8338563866739,-65.6089401625551,
12.));
#134204=CARTESIAN_POINT('Ctrl Pts',(-24.8221975032059,-65.5929074932487,
0.));
#134205=CARTESIAN_POINT('Ctrl Pts',(-24.8221975032059,-65.5929074932487,
12.));
#134206=CARTESIAN_POINT('Ctrl Pts',(-24.8105873098578,-65.5769057914184,
0.));
#134207=CARTESIAN_POINT('Ctrl Pts',(-24.8105873098578,-65.5769057914184,
12.));
#134208=CARTESIAN_POINT('Ctrl Pts',(-24.7990258561234,-65.5609353062749,
0.));
#134209=CARTESIAN_POINT('Ctrl Pts',(-24.7990258561234,-65.5609353062749,
12.));
#134210=CARTESIAN_POINT('Ctrl Pts',(-24.7875131827515,-65.5449962514735,
0.));
#134211=CARTESIAN_POINT('Ctrl Pts',(-24.7875131827515,-65.5449962514735,
12.));
#134212=CARTESIAN_POINT('Ctrl Pts',(-24.7760493148551,-65.5290887770493,
0.));
#134213=CARTESIAN_POINT('Ctrl Pts',(-24.7760493148551,-65.5290887770493,
12.));
#134214=CARTESIAN_POINT('Ctrl Pts',(-24.7646342620969,-65.5132129675727,
0.));
#134215=CARTESIAN_POINT('Ctrl Pts',(-24.7646342620969,-65.5132129675727,
12.));
#134216=CARTESIAN_POINT('Ctrl Pts',(-24.7555412724771,-65.5005376841469,
0.));
#134217=CARTESIAN_POINT('Ctrl Pts',(-24.7555412724771,-65.5005376841469,
12.));
#134218=CARTESIAN_POINT('Ctrl Pts',(-24.7487434956058,-65.4910454936487,
0.));
#134219=CARTESIAN_POINT('Ctrl Pts',(-24.7487434956058,-65.4910454936487,
12.));
#134220=CARTESIAN_POINT('Ctrl Pts',(-24.7442214063411,-65.484723709553,
0.));
#134221=CARTESIAN_POINT('Ctrl Pts',(-24.7442214063411,-65.484723709553,
12.));
#134222=CARTESIAN_POINT('Ctrl Pts',(-24.7419628022042,-65.4815644032299,
0.));
#134223=CARTESIAN_POINT('Ctrl Pts',(-24.7419628022042,-65.4815644032299,
12.));
#134224=CARTESIAN_POINT('',(-24.7419628022042,-65.4815644032299,12.));
#134225=CARTESIAN_POINT('Ctrl Pts',(-24.7419628022042,-65.4815644032299,
12.));
#134226=CARTESIAN_POINT('Ctrl Pts',(-24.7442214063411,-65.484723709553,
12.));
#134227=CARTESIAN_POINT('Ctrl Pts',(-24.7487434956058,-65.4910454936487,
12.));
#134228=CARTESIAN_POINT('Ctrl Pts',(-24.7555412724771,-65.5005376841469,
12.));
#134229=CARTESIAN_POINT('Ctrl Pts',(-24.7646342620969,-65.5132129675727,
12.));
#134230=CARTESIAN_POINT('Ctrl Pts',(-24.7760493148551,-65.5290887770493,
12.));
#134231=CARTESIAN_POINT('Ctrl Pts',(-24.7875131827515,-65.5449962514735,
12.));
#134232=CARTESIAN_POINT('Ctrl Pts',(-24.7990258561234,-65.5609353062749,
12.));
#134233=CARTESIAN_POINT('Ctrl Pts',(-24.8105873098578,-65.5769057914184,
12.));
#134234=CARTESIAN_POINT('Ctrl Pts',(-24.8221975032059,-65.5929074932487,
12.));
#134235=CARTESIAN_POINT('Ctrl Pts',(-24.8338563866739,-65.6089401625551,
12.));
#134236=CARTESIAN_POINT('Ctrl Pts',(-24.8455639071517,-65.6250035361612,
12.));
#134237=CARTESIAN_POINT('Ctrl Pts',(-24.8573200135684,-65.6410973603713,
12.));
#134238=CARTESIAN_POINT('Ctrl Pts',(-24.8691246628081,-65.6572214156761,
12.));
#134239=CARTESIAN_POINT('Ctrl Pts',(-24.8809778178248,-65.6733755087723,
12.));
#134240=CARTESIAN_POINT('Ctrl Pts',(-24.8928794448616,-65.6895594608798,
12.));
#134241=CARTESIAN_POINT('Ctrl Pts',(-24.9048295111444,-65.7057730980471,
12.));
#134242=CARTESIAN_POINT('Ctrl Pts',(-24.9168279820093,-65.7220162391016,
12.));
#134243=CARTESIAN_POINT('Ctrl Pts',(-24.9288748194562,-65.7382886895839,
12.));
#134244=CARTESIAN_POINT('Ctrl Pts',(-24.9409699836523,-65.7545902480286,
12.));
#134245=CARTESIAN_POINT('Ctrl Pts',(-24.9531134338693,-65.7709207098949,
12.));
#134246=CARTESIAN_POINT('Ctrl Pts',(-24.965305129559,-65.7872798720847,
12.));
#134247=CARTESIAN_POINT('Ctrl Pts',(-24.97754503157,-65.8036675380761,12.));
#134248=CARTESIAN_POINT('Ctrl Pts',(-24.9898331021002,-65.8200835177071,
12.));
#134249=CARTESIAN_POINT('Ctrl Pts',(-25.0021693041181,-65.8365276247157,
12.));
#134250=CARTESIAN_POINT('Ctrl Pts',(-25.0145536009603,-65.8529996750441,
12.));
#134251=CARTESIAN_POINT('Ctrl Pts',(-25.0269859558351,-65.8694994847586,
12.));
#134252=CARTESIAN_POINT('Ctrl Pts',(-25.039466331404,-65.8860268683088,
12.));
#134253=CARTESIAN_POINT('Ctrl Pts',(-25.0519946900066,-65.9025816394391,
12.));
#134254=CARTESIAN_POINT('Ctrl Pts',(-25.0645709938519,-65.9191636119796,
12.));
#134255=CARTESIAN_POINT('Ctrl Pts',(-25.0771952052033,-65.9357726006174,
12.));
#134256=CARTESIAN_POINT('Ctrl Pts',(-25.0898672865926,-65.9524084218167,
12.));
#134257=CARTESIAN_POINT('Ctrl Pts',(-25.1025872009016,-65.9690708941591,
12.));
#134258=CARTESIAN_POINT('Ctrl Pts',(-25.1153549112512,-65.9857598378455,
12.));
#134259=CARTESIAN_POINT('Ctrl Pts',(-25.12817038093,-66.0024750743902,12.));
#134260=CARTESIAN_POINT('Ctrl Pts',(-25.1410335733094,-66.0192164262607,
12.));
#134261=CARTESIAN_POINT('Ctrl Pts',(-25.153944451741,-66.0359837164709,
12.));
#134262=CARTESIAN_POINT('Ctrl Pts',(-25.1669029795652,-66.0527767686,12.));
#134263=CARTESIAN_POINT('Ctrl Pts',(-25.1799091201594,-66.0695954069698,
12.));
#134264=CARTESIAN_POINT('Ctrl Pts',(-25.1929628369685,-66.086439456768,
12.));
#134265=CARTESIAN_POINT('Ctrl Pts',(-25.2060640935371,-66.1033087441916,
12.));
#134266=CARTESIAN_POINT('Ctrl Pts',(-25.2192128535367,-66.1202030965784,
12.));
#134267=CARTESIAN_POINT('Ctrl Pts',(-25.2324090807561,-66.1371223423371,
12.));
#134268=CARTESIAN_POINT('Ctrl Pts',(-25.245652739088,-66.1540663108767,
12.));
#134269=CARTESIAN_POINT('Ctrl Pts',(-25.2589437925145,-66.1710348325378,
12.));
#134270=CARTESIAN_POINT('Ctrl Pts',(-25.2722822050829,-66.1880277385113,
12.));
#134271=CARTESIAN_POINT('Ctrl Pts',(-25.2856679408921,-66.2050448607883,
12.));
#134272=CARTESIAN_POINT('Ctrl Pts',(-25.2991009641087,-66.222086032193,
12.));
#134273=CARTESIAN_POINT('Ctrl Pts',(-25.3125812389728,-66.2391510863992,
12.));
#134274=CARTESIAN_POINT('Ctrl Pts',(-25.326108729803,-66.2562398579479,
12.));
#134275=CARTESIAN_POINT('Ctrl Pts',(-25.3396834009955,-66.2733521822675,
12.));
#134276=CARTESIAN_POINT('Ctrl Pts',(-25.3533052170254,-66.2904878956721,
12.));
#134277=CARTESIAN_POINT('Ctrl Pts',(-25.3669741424491,-66.3076468353417,
12.));
#134278=CARTESIAN_POINT('Ctrl Pts',(-25.3806901419013,-66.3248288393046,
12.));
#134279=CARTESIAN_POINT('Ctrl Pts',(-25.3944531800901,-66.3420337464176,
12.));
#134280=CARTESIAN_POINT('Ctrl Pts',(-25.4082632217846,-66.3592613963407,
12.));
#134281=CARTESIAN_POINT('Ctrl Pts',(-25.4221202318198,-66.3765116295363,
12.));
#134282=CARTESIAN_POINT('Ctrl Pts',(-25.4360241751017,-66.3937842872684,
12.));
#134283=CARTESIAN_POINT('Ctrl Pts',(-25.4499750166079,-66.4110792116,12.));
#134284=CARTESIAN_POINT('Ctrl Pts',(-25.463972721385,-66.4283962453899,
12.));
#134285=CARTESIAN_POINT('Ctrl Pts',(-25.4780172545418,-66.445735232287,
12.));
#134286=CARTESIAN_POINT('Ctrl Pts',(-25.4921085812548,-66.463096016725,
12.));
#134287=CARTESIAN_POINT('Ctrl Pts',(-25.5062466667703,-66.4804784439146,
12.));
#134288=CARTESIAN_POINT('Ctrl Pts',(-25.5204314764033,-66.4978823598352,
12.));
#134289=CARTESIAN_POINT('Ctrl Pts',(-25.5346629755322,-66.5153076112237,
12.));
#134290=CARTESIAN_POINT('Ctrl Pts',(-25.5489411295916,-66.5327540455638,
12.));
#134291=CARTESIAN_POINT('Ctrl Pts',(-25.5632659040797,-66.5502215110843,
12.));
#134292=CARTESIAN_POINT('Ctrl Pts',(-25.5776372645605,-66.567709856755,
12.));
#134293=CARTESIAN_POINT('Ctrl Pts',(-25.5920551766629,-66.585218932281,
12.));
#134294=CARTESIAN_POINT('Ctrl Pts',(-25.606519606075,-66.6027485880947,
12.));
#134295=CARTESIAN_POINT('Ctrl Pts',(-25.6210305185395,-66.6202986753482,
12.));
#134296=CARTESIAN_POINT('Ctrl Pts',(-25.6355878798605,-66.6378690459105,
12.));
#134297=CARTESIAN_POINT('Ctrl Pts',(-25.6501916559051,-66.6554595523611,
12.));
#134298=CARTESIAN_POINT('Ctrl Pts',(-25.6648418126016,-66.6730700479843,
12.));
#134299=CARTESIAN_POINT('Ctrl Pts',(-25.679538315933,-66.6907003867599,
12.));
#134300=CARTESIAN_POINT('Ctrl Pts',(-25.6942811319337,-66.7083504233566,
12.));
#134301=CARTESIAN_POINT('Ctrl Pts',(-25.7090702266976,-66.72602001313,12.));
#134302=CARTESIAN_POINT('Ctrl Pts',(-25.7239055663778,-66.7437090121168,
12.));
#134303=CARTESIAN_POINT('Ctrl Pts',(-25.7387871171861,-66.7614172770302,
12.));
#134304=CARTESIAN_POINT('Ctrl Pts',(-25.7537148453848,-66.7791446652505,
12.));
#134305=CARTESIAN_POINT('Ctrl Pts',(-25.7686887172859,-66.7968910348199,
12.));
#134306=CARTESIAN_POINT('Ctrl Pts',(-25.783708699258,-66.8146562444397,
12.));
#134307=CARTESIAN_POINT('Ctrl Pts',(-25.7987747577265,-66.8324401534657,
12.));
#134308=CARTESIAN_POINT('Ctrl Pts',(-25.8138868591715,-66.8502426219015,
12.));
#134309=CARTESIAN_POINT('Ctrl Pts',(-25.8290449701207,-66.8680635103907,
12.));
#134310=CARTESIAN_POINT('Ctrl Pts',(-25.8442490571486,-66.8859026802123,
12.));
#134311=CARTESIAN_POINT('Ctrl Pts',(-25.8594990868845,-66.9037599932787,
12.));
#134312=CARTESIAN_POINT('Ctrl Pts',(-25.8747950260114,-66.9216353121308,
12.));
#134313=CARTESIAN_POINT('Ctrl Pts',(-25.8901368412655,-66.9395284999327,
12.));
#134314=CARTESIAN_POINT('Ctrl Pts',(-25.9055244994267,-66.9574394204635,
12.));
#134315=CARTESIAN_POINT('Ctrl Pts',(-25.9209579673198,-66.9753679381122,
12.));
#134316=CARTESIAN_POINT('Ctrl Pts',(-25.9364372118216,-66.993313917876,
12.));
#134317=CARTESIAN_POINT('Ctrl Pts',(-25.9519621998598,-67.0112772253553,
12.));
#134318=CARTESIAN_POINT('Ctrl Pts',(-25.9675328984123,-67.0292577267495,
12.));
#134319=CARTESIAN_POINT('Ctrl Pts',(-25.9831492744988,-67.0472552888495,
12.));
#134320=CARTESIAN_POINT('Ctrl Pts',(-25.9988112951818,-67.0652697790335,
12.));
#134321=CARTESIAN_POINT('Ctrl Pts',(-26.0145189275733,-67.083301065264,
12.));
#134322=CARTESIAN_POINT('Ctrl Pts',(-26.030272138834,-67.101349016084,12.));
#134323=CARTESIAN_POINT('Ctrl Pts',(-26.0460708961725,-67.1194135006121,
12.));
#134324=CARTESIAN_POINT('Ctrl Pts',(-26.0619151668361,-67.1374943885353,
12.));
#134325=CARTESIAN_POINT('Ctrl Pts',(-26.077804918113,-67.1555915501052,
12.));
#134326=CARTESIAN_POINT('Ctrl Pts',(-26.0937401173385,-67.1737048561364,
12.));
#134327=CARTESIAN_POINT('Ctrl Pts',(-26.109720731895,-67.191834178002,12.));
#134328=CARTESIAN_POINT('Ctrl Pts',(-26.1257467292102,-67.2099793876295,
12.));
#134329=CARTESIAN_POINT('Ctrl Pts',(-26.1418180767487,-67.228140357493,
12.));
#134330=CARTESIAN_POINT('Ctrl Pts',(-26.1579347420135,-67.2463169606105,
12.));
#134331=CARTESIAN_POINT('Ctrl Pts',(-26.1740966925527,-67.2645090705414,
12.));
#134332=CARTESIAN_POINT('Ctrl Pts',(-26.1903038959589,-67.2827165613828,
12.));
#134333=CARTESIAN_POINT('Ctrl Pts',(-26.2065563198685,-67.3009393077654,
12.));
#134334=CARTESIAN_POINT('Ctrl Pts',(-26.2228539319528,-67.3191771848468,
12.));
#134335=CARTESIAN_POINT('Ctrl Pts',(-26.2391966999192,-67.3374300683075,
12.));
#134336=CARTESIAN_POINT('Ctrl Pts',(-26.255584591518,-67.3556978343506,
12.));
#134337=CARTESIAN_POINT('Ctrl Pts',(-26.2720175745423,-67.3739803596967,
12.));
#134338=CARTESIAN_POINT('Ctrl Pts',(-26.288495616827,-67.392277521581,12.));
#134339=CARTESIAN_POINT('Ctrl Pts',(-26.305018686241,-67.4105891977465,
12.));
#134340=CARTESIAN_POINT('Ctrl Pts',(-26.3215867506864,-67.4289152664406,
12.));
#134341=CARTESIAN_POINT('Ctrl Pts',(-26.3381997781059,-67.4472556064127,
12.));
#134342=CARTESIAN_POINT('Ctrl Pts',(-26.3548577364835,-67.4656100969121,
12.));
#134343=CARTESIAN_POINT('Ctrl Pts',(-26.3715605938432,-67.4839786176833,
12.));
#134344=CARTESIAN_POINT('Ctrl Pts',(-26.3883083182417,-67.5023610489611,
12.));
#134345=CARTESIAN_POINT('Ctrl Pts',(-26.4051008777669,-67.5207572714666,
12.));
#134346=CARTESIAN_POINT('Ctrl Pts',(-26.4219382405452,-67.5391671664055,
12.));
#134347=CARTESIAN_POINT('Ctrl Pts',(-26.4388203747422,-67.5575906154648,
12.));
#134348=CARTESIAN_POINT('Ctrl Pts',(-26.4557472485622,-67.5760275008096,
12.));
#134349=CARTESIAN_POINT('Ctrl Pts',(-26.4727188302415,-67.5944777050782,
12.));
#134350=CARTESIAN_POINT('Ctrl Pts',(-26.4897350880447,-67.6129411113774,
12.));
#134351=CARTESIAN_POINT('Ctrl Pts',(-26.5067959902731,-67.6314176032823,
12.));
#134352=CARTESIAN_POINT('Ctrl Pts',(-26.5239015052656,-67.6499070648323,
12.));
#134353=CARTESIAN_POINT('Ctrl Pts',(-26.5410516013984,-67.6684093805288,
12.));
#134354=CARTESIAN_POINT('Ctrl Pts',(-26.5582462470794,-67.6869244353292,
12.));
#134355=CARTESIAN_POINT('Ctrl Pts',(-26.5754854107422,-67.7054521146427,
12.));
#134356=CARTESIAN_POINT('Ctrl Pts',(-26.5927690608547,-67.7239923043295,
12.));
#134357=CARTESIAN_POINT('Ctrl Pts',(-26.6100971659205,-67.7425448906983,
12.));
#134358=CARTESIAN_POINT('Ctrl Pts',(-26.6274696944793,-67.7611097605042,
12.));
#134359=CARTESIAN_POINT('Ctrl Pts',(-26.6448866151027,-67.7796868009447,
12.));
#134360=CARTESIAN_POINT('Ctrl Pts',(-26.6623478963867,-67.7982758996557,
12.));
#134361=CARTESIAN_POINT('Ctrl Pts',(-26.6798535069586,-67.8168769447086,
12.));
#134362=CARTESIAN_POINT('Ctrl Pts',(-26.6974034154803,-67.8354898246079,
12.));
#134363=CARTESIAN_POINT('Ctrl Pts',(-26.7149975906478,-67.8541144282875,
12.));
#134364=CARTESIAN_POINT('Ctrl Pts',(-26.7326360011886,-67.8727506451067,
12.));
#134365=CARTESIAN_POINT('Ctrl Pts',(-26.7503186158523,-67.8913983648441,
12.));
#134366=CARTESIAN_POINT('Ctrl Pts',(-26.7680454034169,-67.9100574776974,
12.));
#134367=CARTESIAN_POINT('Ctrl Pts',(-26.7858163326933,-67.9287278742839,
12.));
#134368=CARTESIAN_POINT('Ctrl Pts',(-26.8036313725262,-67.9474094456395,
12.));
#134369=CARTESIAN_POINT('Ctrl Pts',(-26.8214904917922,-67.9661020832165,
12.));
#134370=CARTESIAN_POINT('Ctrl Pts',(-26.8393936593914,-67.9848056788814,
12.));
#134371=CARTESIAN_POINT('Ctrl Pts',(-26.85734084425,-68.0035201249108,12.));
#134372=CARTESIAN_POINT('Ctrl Pts',(-26.8753320153255,-68.0222453139862,
12.));
#134373=CARTESIAN_POINT('Ctrl Pts',(-26.8933671416065,-68.0409811391871,
12.));
#134374=CARTESIAN_POINT('Ctrl Pts',(-26.9114461921109,-68.0597274939857,
12.));
#134375=CARTESIAN_POINT('Ctrl Pts',(-26.9295691358775,-68.0784842722362,
12.));
#134376=CARTESIAN_POINT('Ctrl Pts',(-26.9477359419646,-68.0972513681739,
12.));
#134377=CARTESIAN_POINT('Ctrl Pts',(-26.9659465794596,-68.1160286764244,
12.));
#134378=CARTESIAN_POINT('Ctrl Pts',(-26.9842010174819,-68.13481609201,12.));
#134379=CARTESIAN_POINT('Ctrl Pts',(-27.0024992251839,-68.1536135103558,
12.));
#134380=CARTESIAN_POINT('Ctrl Pts',(-27.0208411717477,-68.1724208272967,
12.));
#134381=CARTESIAN_POINT('Ctrl Pts',(-27.0392268263805,-68.1912379390786,
12.));
#134382=CARTESIAN_POINT('Ctrl Pts',(-27.0576561583179,-68.2100647423345,
12.));
#134383=CARTESIAN_POINT('Ctrl Pts',(-27.076129136823,-68.2289011340624,
12.));
#134384=CARTESIAN_POINT('Ctrl Pts',(-27.0946457311814,-68.2477470116014,
12.));
#134385=CARTESIAN_POINT('Ctrl Pts',(-27.1132059106939,-68.2666022726094,
12.));
#134386=CARTESIAN_POINT('Ctrl Pts',(-27.1318096446643,-68.285466815035,
12.));
#134387=CARTESIAN_POINT('Ctrl Pts',(-27.1504569024131,-68.3043405371589,
12.));
#134388=CARTESIAN_POINT('Ctrl Pts',(-27.1691476532917,-68.3232233376415,
12.));
#134389=CARTESIAN_POINT('Ctrl Pts',(-27.1878818666925,-68.3421151155708,
12.));
#134390=CARTESIAN_POINT('Ctrl Pts',(-27.2066595120544,-68.3610157704999,
12.));
#134391=CARTESIAN_POINT('Ctrl Pts',(-27.2254805588677,-68.379925202511,
12.));
#134392=CARTESIAN_POINT('Ctrl Pts',(-27.2443449766654,-68.3988433121589,
12.));
#134393=CARTESIAN_POINT('Ctrl Pts',(-27.2632527350062,-68.4177700003471,
12.));
#134394=CARTESIAN_POINT('Ctrl Pts',(-27.2822038034539,-68.4367051682166,
12.));
#134395=CARTESIAN_POINT('Ctrl Pts',(-27.301198151557,-68.455648717044,12.));
#134396=CARTESIAN_POINT('Ctrl Pts',(-27.3202357488153,-68.4746005480992,
12.));
#134397=CARTESIAN_POINT('Ctrl Pts',(-27.3393165646748,-68.4935605626361,
12.));
#134398=CARTESIAN_POINT('Ctrl Pts',(-27.3584405685941,-68.5125286621888,
12.));
#134399=CARTESIAN_POINT('Ctrl Pts',(-27.3776077300914,-68.5315047488035,
12.));
#134400=CARTESIAN_POINT('Ctrl Pts',(-27.3968180187941,-68.5504887252975,
12.));
#134401=CARTESIAN_POINT('Ctrl Pts',(-27.4160714044831,-68.5694804955014,
12.));
#134402=CARTESIAN_POINT('Ctrl Pts',(-27.4353678571361,-68.5884799645218,
12.));
#134403=CARTESIAN_POINT('Ctrl Pts',(-27.4547073468227,-68.6074870381619,
12.));
#134404=CARTESIAN_POINT('Ctrl Pts',(-27.4740898435988,-68.6265016223561,
12.));
#134405=CARTESIAN_POINT('Ctrl Pts',(-27.4935153173868,-68.645523622548,
12.));
#134406=CARTESIAN_POINT('Ctrl Pts',(-27.5129837378791,-68.6645529432045,
12.));
#134407=CARTESIAN_POINT('Ctrl Pts',(-27.5324950743706,-68.6835894869882,
12.));
#134408=CARTESIAN_POINT('Ctrl Pts',(-27.5520492958907,-68.7026331554296,
12.));
#134409=CARTESIAN_POINT('Ctrl Pts',(-27.5716463715005,-68.7216838504218,
12.));
#134410=CARTESIAN_POINT('Ctrl Pts',(-27.5912862705469,-68.7407414755259,
12.));
#134411=CARTESIAN_POINT('Ctrl Pts',(-27.6109689629029,-68.7598059372129,
12.));
#134412=CARTESIAN_POINT('Ctrl Pts',(-27.6306944192738,-68.7788771464713,
12.));
#134413=CARTESIAN_POINT('Ctrl Pts',(-27.6504626112666,-68.7979550191872,
12.));
#134414=CARTESIAN_POINT('Ctrl Pts',(-27.6674443909984,-68.8143140938915,
12.));
#134415=CARTESIAN_POINT('Ctrl Pts',(-27.6804870323434,-68.8268597852179,
12.));
#134416=CARTESIAN_POINT('Ctrl Pts',(-27.6895716271275,-68.8355891982106,
12.));
#134417=CARTESIAN_POINT('Ctrl Pts',(-27.6946856803719,-68.840500446616,
12.));
#134418=CARTESIAN_POINT('Ctrl Pts',(-27.6958230985045,-68.8415926175086,
12.));
#134419=CARTESIAN_POINT('',(-24.7419628022042,-65.4815644032299,0.));
#134420=CARTESIAN_POINT('',(-24.7419628022042,-65.4815644032299,0.));
#134421=CARTESIAN_POINT('Ctrl Pts',(-27.6958230985045,-68.8415926175086,
0.));
#134422=CARTESIAN_POINT('Ctrl Pts',(-27.6946856803719,-68.840500446616,
0.));
#134423=CARTESIAN_POINT('Ctrl Pts',(-27.6895716271275,-68.8355891982106,
0.));
#134424=CARTESIAN_POINT('Ctrl Pts',(-27.6804870323434,-68.8268597852179,
0.));
#134425=CARTESIAN_POINT('Ctrl Pts',(-27.6674443909984,-68.8143140938915,
0.));
#134426=CARTESIAN_POINT('Ctrl Pts',(-27.6504626112666,-68.7979550191872,
0.));
#134427=CARTESIAN_POINT('Ctrl Pts',(-27.6306944192738,-68.7788771464713,
0.));
#134428=CARTESIAN_POINT('Ctrl Pts',(-27.6109689629029,-68.7598059372129,
0.));
#134429=CARTESIAN_POINT('Ctrl Pts',(-27.5912862705469,-68.7407414755259,
0.));
#134430=CARTESIAN_POINT('Ctrl Pts',(-27.5716463715005,-68.7216838504218,
0.));
#134431=CARTESIAN_POINT('Ctrl Pts',(-27.5520492958907,-68.7026331554296,
0.));
#134432=CARTESIAN_POINT('Ctrl Pts',(-27.5324950743706,-68.6835894869882,
0.));
#134433=CARTESIAN_POINT('Ctrl Pts',(-27.5129837378791,-68.6645529432045,
0.));
#134434=CARTESIAN_POINT('Ctrl Pts',(-27.4935153173868,-68.645523622548,
0.));
#134435=CARTESIAN_POINT('Ctrl Pts',(-27.4740898435988,-68.6265016223561,
0.));
#134436=CARTESIAN_POINT('Ctrl Pts',(-27.4547073468227,-68.6074870381619,
0.));
#134437=CARTESIAN_POINT('Ctrl Pts',(-27.4353678571361,-68.5884799645218,
0.));
#134438=CARTESIAN_POINT('Ctrl Pts',(-27.4160714044831,-68.5694804955014,
0.));
#134439=CARTESIAN_POINT('Ctrl Pts',(-27.3968180187941,-68.5504887252975,
0.));
#134440=CARTESIAN_POINT('Ctrl Pts',(-27.3776077300914,-68.5315047488035,
0.));
#134441=CARTESIAN_POINT('Ctrl Pts',(-27.3584405685941,-68.5125286621888,
0.));
#134442=CARTESIAN_POINT('Ctrl Pts',(-27.3393165646748,-68.4935605626361,
0.));
#134443=CARTESIAN_POINT('Ctrl Pts',(-27.3202357488153,-68.4746005480992,
0.));
#134444=CARTESIAN_POINT('Ctrl Pts',(-27.301198151557,-68.455648717044,0.));
#134445=CARTESIAN_POINT('Ctrl Pts',(-27.2822038034539,-68.4367051682166,
0.));
#134446=CARTESIAN_POINT('Ctrl Pts',(-27.2632527350062,-68.4177700003471,
0.));
#134447=CARTESIAN_POINT('Ctrl Pts',(-27.2443449766654,-68.3988433121589,
0.));
#134448=CARTESIAN_POINT('Ctrl Pts',(-27.2254805588677,-68.379925202511,
0.));
#134449=CARTESIAN_POINT('Ctrl Pts',(-27.2066595120544,-68.3610157704999,
0.));
#134450=CARTESIAN_POINT('Ctrl Pts',(-27.1878818666925,-68.3421151155708,
0.));
#134451=CARTESIAN_POINT('Ctrl Pts',(-27.1691476532917,-68.3232233376415,
0.));
#134452=CARTESIAN_POINT('Ctrl Pts',(-27.1504569024131,-68.3043405371589,
0.));
#134453=CARTESIAN_POINT('Ctrl Pts',(-27.1318096446643,-68.285466815035,
0.));
#134454=CARTESIAN_POINT('Ctrl Pts',(-27.1132059106939,-68.2666022726094,
0.));
#134455=CARTESIAN_POINT('Ctrl Pts',(-27.0946457311814,-68.2477470116014,
0.));
#134456=CARTESIAN_POINT('Ctrl Pts',(-27.076129136823,-68.2289011340624,
0.));
#134457=CARTESIAN_POINT('Ctrl Pts',(-27.0576561583179,-68.2100647423345,
0.));
#134458=CARTESIAN_POINT('Ctrl Pts',(-27.0392268263805,-68.1912379390786,
0.));
#134459=CARTESIAN_POINT('Ctrl Pts',(-27.0208411717477,-68.1724208272967,
0.));
#134460=CARTESIAN_POINT('Ctrl Pts',(-27.0024992251839,-68.1536135103558,
0.));
#134461=CARTESIAN_POINT('Ctrl Pts',(-26.9842010174819,-68.13481609201,0.));
#134462=CARTESIAN_POINT('Ctrl Pts',(-26.9659465794596,-68.1160286764244,
0.));
#134463=CARTESIAN_POINT('Ctrl Pts',(-26.9477359419646,-68.0972513681739,
0.));
#134464=CARTESIAN_POINT('Ctrl Pts',(-26.9295691358775,-68.0784842722362,
0.));
#134465=CARTESIAN_POINT('Ctrl Pts',(-26.9114461921109,-68.0597274939857,
0.));
#134466=CARTESIAN_POINT('Ctrl Pts',(-26.8933671416065,-68.0409811391871,
0.));
#134467=CARTESIAN_POINT('Ctrl Pts',(-26.8753320153255,-68.0222453139862,
0.));
#134468=CARTESIAN_POINT('Ctrl Pts',(-26.85734084425,-68.0035201249108,0.));
#134469=CARTESIAN_POINT('Ctrl Pts',(-26.8393936593914,-67.9848056788814,
0.));
#134470=CARTESIAN_POINT('Ctrl Pts',(-26.8214904917922,-67.9661020832165,
0.));
#134471=CARTESIAN_POINT('Ctrl Pts',(-26.8036313725262,-67.9474094456395,
0.));
#134472=CARTESIAN_POINT('Ctrl Pts',(-26.7858163326933,-67.9287278742839,
0.));
#134473=CARTESIAN_POINT('Ctrl Pts',(-26.7680454034169,-67.9100574776974,
0.));
#134474=CARTESIAN_POINT('Ctrl Pts',(-26.7503186158523,-67.8913983648441,
0.));
#134475=CARTESIAN_POINT('Ctrl Pts',(-26.7326360011886,-67.8727506451067,
0.));
#134476=CARTESIAN_POINT('Ctrl Pts',(-26.7149975906478,-67.8541144282875,
0.));
#134477=CARTESIAN_POINT('Ctrl Pts',(-26.6974034154803,-67.8354898246079,
0.));
#134478=CARTESIAN_POINT('Ctrl Pts',(-26.6798535069586,-67.8168769447086,
0.));
#134479=CARTESIAN_POINT('Ctrl Pts',(-26.6623478963867,-67.7982758996557,
0.));
#134480=CARTESIAN_POINT('Ctrl Pts',(-26.6448866151027,-67.7796868009447,
0.));
#134481=CARTESIAN_POINT('Ctrl Pts',(-26.6274696944793,-67.7611097605042,
0.));
#134482=CARTESIAN_POINT('Ctrl Pts',(-26.6100971659205,-67.7425448906983,
0.));
#134483=CARTESIAN_POINT('Ctrl Pts',(-26.5927690608547,-67.7239923043295,
0.));
#134484=CARTESIAN_POINT('Ctrl Pts',(-26.5754854107422,-67.7054521146427,
0.));
#134485=CARTESIAN_POINT('Ctrl Pts',(-26.5582462470794,-67.6869244353292,
0.));
#134486=CARTESIAN_POINT('Ctrl Pts',(-26.5410516013984,-67.6684093805288,
0.));
#134487=CARTESIAN_POINT('Ctrl Pts',(-26.5239015052656,-67.6499070648323,
0.));
#134488=CARTESIAN_POINT('Ctrl Pts',(-26.5067959902731,-67.6314176032823,
0.));
#134489=CARTESIAN_POINT('Ctrl Pts',(-26.4897350880447,-67.6129411113774,
0.));
#134490=CARTESIAN_POINT('Ctrl Pts',(-26.4727188302415,-67.5944777050782,
0.));
#134491=CARTESIAN_POINT('Ctrl Pts',(-26.4557472485622,-67.5760275008096,
0.));
#134492=CARTESIAN_POINT('Ctrl Pts',(-26.4388203747422,-67.5575906154648,
0.));
#134493=CARTESIAN_POINT('Ctrl Pts',(-26.4219382405452,-67.5391671664055,
0.));
#134494=CARTESIAN_POINT('Ctrl Pts',(-26.4051008777669,-67.5207572714666,
0.));
#134495=CARTESIAN_POINT('Ctrl Pts',(-26.3883083182417,-67.5023610489611,
0.));
#134496=CARTESIAN_POINT('Ctrl Pts',(-26.3715605938432,-67.4839786176833,
0.));
#134497=CARTESIAN_POINT('Ctrl Pts',(-26.3548577364835,-67.4656100969121,
0.));
#134498=CARTESIAN_POINT('Ctrl Pts',(-26.3381997781059,-67.4472556064127,
0.));
#134499=CARTESIAN_POINT('Ctrl Pts',(-26.3215867506864,-67.4289152664406,
0.));
#134500=CARTESIAN_POINT('Ctrl Pts',(-26.305018686241,-67.4105891977465,
0.));
#134501=CARTESIAN_POINT('Ctrl Pts',(-26.288495616827,-67.392277521581,0.));
#134502=CARTESIAN_POINT('Ctrl Pts',(-26.2720175745423,-67.3739803596967,
0.));
#134503=CARTESIAN_POINT('Ctrl Pts',(-26.255584591518,-67.3556978343506,
0.));
#134504=CARTESIAN_POINT('Ctrl Pts',(-26.2391966999192,-67.3374300683075,
0.));
#134505=CARTESIAN_POINT('Ctrl Pts',(-26.2228539319528,-67.3191771848468,
0.));
#134506=CARTESIAN_POINT('Ctrl Pts',(-26.2065563198685,-67.3009393077654,
0.));
#134507=CARTESIAN_POINT('Ctrl Pts',(-26.1903038959589,-67.2827165613828,
0.));
#134508=CARTESIAN_POINT('Ctrl Pts',(-26.1740966925527,-67.2645090705414,
0.));
#134509=CARTESIAN_POINT('Ctrl Pts',(-26.1579347420135,-67.2463169606105,
0.));
#134510=CARTESIAN_POINT('Ctrl Pts',(-26.1418180767487,-67.228140357493,
0.));
#134511=CARTESIAN_POINT('Ctrl Pts',(-26.1257467292102,-67.2099793876295,
0.));
#134512=CARTESIAN_POINT('Ctrl Pts',(-26.109720731895,-67.191834178002,0.));
#134513=CARTESIAN_POINT('Ctrl Pts',(-26.0937401173385,-67.1737048561364,
0.));
#134514=CARTESIAN_POINT('Ctrl Pts',(-26.077804918113,-67.1555915501052,
0.));
#134515=CARTESIAN_POINT('Ctrl Pts',(-26.0619151668361,-67.1374943885353,
0.));
#134516=CARTESIAN_POINT('Ctrl Pts',(-26.0460708961725,-67.1194135006121,
0.));
#134517=CARTESIAN_POINT('Ctrl Pts',(-26.030272138834,-67.101349016084,0.));
#134518=CARTESIAN_POINT('Ctrl Pts',(-26.0145189275733,-67.083301065264,
0.));
#134519=CARTESIAN_POINT('Ctrl Pts',(-25.9988112951818,-67.0652697790335,
0.));
#134520=CARTESIAN_POINT('Ctrl Pts',(-25.9831492744988,-67.0472552888495,
0.));
#134521=CARTESIAN_POINT('Ctrl Pts',(-25.9675328984123,-67.0292577267495,
0.));
#134522=CARTESIAN_POINT('Ctrl Pts',(-25.9519621998598,-67.0112772253553,
0.));
#134523=CARTESIAN_POINT('Ctrl Pts',(-25.9364372118216,-66.993313917876,
0.));
#134524=CARTESIAN_POINT('Ctrl Pts',(-25.9209579673198,-66.9753679381122,
0.));
#134525=CARTESIAN_POINT('Ctrl Pts',(-25.9055244994267,-66.9574394204635,
0.));
#134526=CARTESIAN_POINT('Ctrl Pts',(-25.8901368412655,-66.9395284999327,
0.));
#134527=CARTESIAN_POINT('Ctrl Pts',(-25.8747950260114,-66.9216353121308,
0.));
#134528=CARTESIAN_POINT('Ctrl Pts',(-25.8594990868845,-66.9037599932787,
0.));
#134529=CARTESIAN_POINT('Ctrl Pts',(-25.8442490571486,-66.8859026802123,
0.));
#134530=CARTESIAN_POINT('Ctrl Pts',(-25.8290449701207,-66.8680635103907,
0.));
#134531=CARTESIAN_POINT('Ctrl Pts',(-25.8138868591715,-66.8502426219015,
0.));
#134532=CARTESIAN_POINT('Ctrl Pts',(-25.7987747577265,-66.8324401534657,
0.));
#134533=CARTESIAN_POINT('Ctrl Pts',(-25.783708699258,-66.8146562444397,
0.));
#134534=CARTESIAN_POINT('Ctrl Pts',(-25.7686887172859,-66.7968910348199,
0.));
#134535=CARTESIAN_POINT('Ctrl Pts',(-25.7537148453848,-66.7791446652505,
0.));
#134536=CARTESIAN_POINT('Ctrl Pts',(-25.7387871171861,-66.7614172770302,
0.));
#134537=CARTESIAN_POINT('Ctrl Pts',(-25.7239055663778,-66.7437090121168,
0.));
#134538=CARTESIAN_POINT('Ctrl Pts',(-25.7090702266976,-66.72602001313,0.));
#134539=CARTESIAN_POINT('Ctrl Pts',(-25.6942811319337,-66.7083504233566,
0.));
#134540=CARTESIAN_POINT('Ctrl Pts',(-25.679538315933,-66.6907003867599,
0.));
#134541=CARTESIAN_POINT('Ctrl Pts',(-25.6648418126016,-66.6730700479843,
0.));
#134542=CARTESIAN_POINT('Ctrl Pts',(-25.6501916559051,-66.6554595523611,
0.));
#134543=CARTESIAN_POINT('Ctrl Pts',(-25.6355878798605,-66.6378690459105,
0.));
#134544=CARTESIAN_POINT('Ctrl Pts',(-25.6210305185395,-66.6202986753482,
0.));
#134545=CARTESIAN_POINT('Ctrl Pts',(-25.606519606075,-66.6027485880947,
0.));
#134546=CARTESIAN_POINT('Ctrl Pts',(-25.5920551766629,-66.585218932281,
0.));
#134547=CARTESIAN_POINT('Ctrl Pts',(-25.5776372645605,-66.567709856755,
0.));
#134548=CARTESIAN_POINT('Ctrl Pts',(-25.5632659040797,-66.5502215110843,
0.));
#134549=CARTESIAN_POINT('Ctrl Pts',(-25.5489411295916,-66.5327540455638,
0.));
#134550=CARTESIAN_POINT('Ctrl Pts',(-25.5346629755322,-66.5153076112237,
0.));
#134551=CARTESIAN_POINT('Ctrl Pts',(-25.5204314764033,-66.4978823598352,
0.));
#134552=CARTESIAN_POINT('Ctrl Pts',(-25.5062466667703,-66.4804784439146,
0.));
#134553=CARTESIAN_POINT('Ctrl Pts',(-25.4921085812548,-66.463096016725,
0.));
#134554=CARTESIAN_POINT('Ctrl Pts',(-25.4780172545418,-66.445735232287,
0.));
#134555=CARTESIAN_POINT('Ctrl Pts',(-25.463972721385,-66.4283962453899,
0.));
#134556=CARTESIAN_POINT('Ctrl Pts',(-25.4499750166079,-66.4110792116,0.));
#134557=CARTESIAN_POINT('Ctrl Pts',(-25.4360241751017,-66.3937842872684,
0.));
#134558=CARTESIAN_POINT('Ctrl Pts',(-25.4221202318198,-66.3765116295363,
0.));
#134559=CARTESIAN_POINT('Ctrl Pts',(-25.4082632217846,-66.3592613963407,
0.));
#134560=CARTESIAN_POINT('Ctrl Pts',(-25.3944531800901,-66.3420337464176,
0.));
#134561=CARTESIAN_POINT('Ctrl Pts',(-25.3806901419013,-66.3248288393046,
0.));
#134562=CARTESIAN_POINT('Ctrl Pts',(-25.3669741424491,-66.3076468353417,
0.));
#134563=CARTESIAN_POINT('Ctrl Pts',(-25.3533052170254,-66.2904878956721,
0.));
#134564=CARTESIAN_POINT('Ctrl Pts',(-25.3396834009955,-66.2733521822675,
0.));
#134565=CARTESIAN_POINT('Ctrl Pts',(-25.326108729803,-66.2562398579479,
0.));
#134566=CARTESIAN_POINT('Ctrl Pts',(-25.3125812389728,-66.2391510863992,
0.));
#134567=CARTESIAN_POINT('Ctrl Pts',(-25.2991009641087,-66.222086032193,
0.));
#134568=CARTESIAN_POINT('Ctrl Pts',(-25.2856679408921,-66.2050448607883,
0.));
#134569=CARTESIAN_POINT('Ctrl Pts',(-25.2722822050829,-66.1880277385113,
0.));
#134570=CARTESIAN_POINT('Ctrl Pts',(-25.2589437925145,-66.1710348325378,
0.));
#134571=CARTESIAN_POINT('Ctrl Pts',(-25.245652739088,-66.1540663108767,
0.));
#134572=CARTESIAN_POINT('Ctrl Pts',(-25.2324090807561,-66.1371223423371,
0.));
#134573=CARTESIAN_POINT('Ctrl Pts',(-25.2192128535367,-66.1202030965784,
0.));
#134574=CARTESIAN_POINT('Ctrl Pts',(-25.2060640935371,-66.1033087441916,
0.));
#134575=CARTESIAN_POINT('Ctrl Pts',(-25.1929628369685,-66.086439456768,
0.));
#134576=CARTESIAN_POINT('Ctrl Pts',(-25.1799091201594,-66.0695954069698,
0.));
#134577=CARTESIAN_POINT('Ctrl Pts',(-25.1669029795652,-66.0527767686,0.));
#134578=CARTESIAN_POINT('Ctrl Pts',(-25.153944451741,-66.0359837164709,
0.));
#134579=CARTESIAN_POINT('Ctrl Pts',(-25.1410335733094,-66.0192164262607,
0.));
#134580=CARTESIAN_POINT('Ctrl Pts',(-25.12817038093,-66.0024750743902,0.));
#134581=CARTESIAN_POINT('Ctrl Pts',(-25.1153549112512,-65.9857598378455,
0.));
#134582=CARTESIAN_POINT('Ctrl Pts',(-25.1025872009016,-65.9690708941591,
0.));
#134583=CARTESIAN_POINT('Ctrl Pts',(-25.0898672865926,-65.9524084218167,
0.));
#134584=CARTESIAN_POINT('Ctrl Pts',(-25.0771952052033,-65.9357726006174,
0.));
#134585=CARTESIAN_POINT('Ctrl Pts',(-25.0645709938519,-65.9191636119796,
0.));
#134586=CARTESIAN_POINT('Ctrl Pts',(-25.0519946900066,-65.9025816394391,
0.));
#134587=CARTESIAN_POINT('Ctrl Pts',(-25.039466331404,-65.8860268683088,
0.));
#134588=CARTESIAN_POINT('Ctrl Pts',(-25.0269859558351,-65.8694994847586,
0.));
#134589=CARTESIAN_POINT('Ctrl Pts',(-25.0145536009603,-65.8529996750441,
0.));
#134590=CARTESIAN_POINT('Ctrl Pts',(-25.0021693041181,-65.8365276247157,
0.));
#134591=CARTESIAN_POINT('Ctrl Pts',(-24.9898331021002,-65.8200835177071,
0.));
#134592=CARTESIAN_POINT('Ctrl Pts',(-24.97754503157,-65.8036675380761,0.));
#134593=CARTESIAN_POINT('Ctrl Pts',(-24.965305129559,-65.7872798720847,
0.));
#134594=CARTESIAN_POINT('Ctrl Pts',(-24.9531134338693,-65.7709207098949,
0.));
#134595=CARTESIAN_POINT('Ctrl Pts',(-24.9409699836523,-65.7545902480286,
0.));
#134596=CARTESIAN_POINT('Ctrl Pts',(-24.9288748194562,-65.7382886895839,
0.));
#134597=CARTESIAN_POINT('Ctrl Pts',(-24.9168279820093,-65.7220162391016,
0.));
#134598=CARTESIAN_POINT('Ctrl Pts',(-24.9048295111444,-65.7057730980471,
0.));
#134599=CARTESIAN_POINT('Ctrl Pts',(-24.8928794448616,-65.6895594608798,
0.));
#134600=CARTESIAN_POINT('Ctrl Pts',(-24.8809778178248,-65.6733755087723,
0.));
#134601=CARTESIAN_POINT('Ctrl Pts',(-24.8691246628081,-65.6572214156761,
0.));
#134602=CARTESIAN_POINT('Ctrl Pts',(-24.8573200135684,-65.6410973603713,
0.));
#134603=CARTESIAN_POINT('Ctrl Pts',(-24.8455639071517,-65.6250035361612,
0.));
#134604=CARTESIAN_POINT('Ctrl Pts',(-24.8338563866739,-65.6089401625551,
0.));
#134605=CARTESIAN_POINT('Ctrl Pts',(-24.8221975032059,-65.5929074932487,
0.));
#134606=CARTESIAN_POINT('Ctrl Pts',(-24.8105873098578,-65.5769057914184,
0.));
#134607=CARTESIAN_POINT('Ctrl Pts',(-24.7990258561234,-65.5609353062749,
0.));
#134608=CARTESIAN_POINT('Ctrl Pts',(-24.7875131827515,-65.5449962514735,
0.));
#134609=CARTESIAN_POINT('Ctrl Pts',(-24.7760493148551,-65.5290887770493,
0.));
#134610=CARTESIAN_POINT('Ctrl Pts',(-24.7646342620969,-65.5132129675727,
0.));
#134611=CARTESIAN_POINT('Ctrl Pts',(-24.7555412724771,-65.5005376841469,
0.));
#134612=CARTESIAN_POINT('Ctrl Pts',(-24.7487434956058,-65.4910454936487,
0.));
#134613=CARTESIAN_POINT('Ctrl Pts',(-24.7442214063411,-65.484723709553,
0.));
#134614=CARTESIAN_POINT('Ctrl Pts',(-24.7419628022042,-65.4815644032299,
0.));
#134615=CARTESIAN_POINT('Ctrl Pts',(-33.8448817269567,-66.3684712863594,
0.));
#134616=CARTESIAN_POINT('Ctrl Pts',(-33.8448817269567,-66.3684712863594,
12.));
#134617=CARTESIAN_POINT('Ctrl Pts',(-33.840486261887,-66.3650082659712,
0.));
#134618=CARTESIAN_POINT('Ctrl Pts',(-33.840486261887,-66.3650082659712,
12.));
#134619=CARTESIAN_POINT('Ctrl Pts',(-33.8316996011932,-66.3580824155893,
0.));
#134620=CARTESIAN_POINT('Ctrl Pts',(-33.8316996011932,-66.3580824155893,
12.));
#134621=CARTESIAN_POINT('Ctrl Pts',(-33.8185324184903,-66.3476942112,0.));
#134622=CARTESIAN_POINT('Ctrl Pts',(-33.8185324184903,-66.3476942112,12.));
#134623=CARTESIAN_POINT('Ctrl Pts',(-33.8010017926027,-66.3338444144211,
0.));
#134624=CARTESIAN_POINT('Ctrl Pts',(-33.8010017926027,-66.3338444144211,
12.));
#134625=CARTESIAN_POINT('Ctrl Pts',(-33.7791312145108,-66.3165340771611,
0.));
#134626=CARTESIAN_POINT('Ctrl Pts',(-33.7791312145108,-66.3165340771611,
12.));
#134627=CARTESIAN_POINT('Ctrl Pts',(-33.7573033544559,-66.2992256621336,
0.));
#134628=CARTESIAN_POINT('Ctrl Pts',(-33.7573033544559,-66.2992256621336,
12.));
#134629=CARTESIAN_POINT('Ctrl Pts',(-33.7355182321907,-66.2819191962353,
0.));
#134630=CARTESIAN_POINT('Ctrl Pts',(-33.7355182321907,-66.2819191962353,
12.));
#134631=CARTESIAN_POINT('Ctrl Pts',(-33.7137758735903,-66.2646147235321,
0.));
#134632=CARTESIAN_POINT('Ctrl Pts',(-33.7137758735903,-66.2646147235321,
12.));
#134633=CARTESIAN_POINT('Ctrl Pts',(-33.6920763111448,-66.2473123109395,
0.));
#134634=CARTESIAN_POINT('Ctrl Pts',(-33.6920763111448,-66.2473123109395,
12.));
#134635=CARTESIAN_POINT('Ctrl Pts',(-33.6704195830392,-66.2300120464082,
0.));
#134636=CARTESIAN_POINT('Ctrl Pts',(-33.6704195830392,-66.2300120464082,
12.));
#134637=CARTESIAN_POINT('Ctrl Pts',(-33.6488057311532,-66.2127140313598,
0.));
#134638=CARTESIAN_POINT('Ctrl Pts',(-33.6488057311532,-66.2127140313598,
12.));
#134639=CARTESIAN_POINT('Ctrl Pts',(-33.6272347993476,-66.1954183747088,
0.));
#134640=CARTESIAN_POINT('Ctrl Pts',(-33.6272347993476,-66.1954183747088,
12.));
#134641=CARTESIAN_POINT('Ctrl Pts',(-33.6057068316769,-66.1781251864017,
0.));
#134642=CARTESIAN_POINT('Ctrl Pts',(-33.6057068316769,-66.1781251864017,
12.));
#134643=CARTESIAN_POINT('Ctrl Pts',(-33.5842218705151,-66.1608345707636,
0.));
#134644=CARTESIAN_POINT('Ctrl Pts',(-33.5842218705151,-66.1608345707636,
12.));
#134645=CARTESIAN_POINT('Ctrl Pts',(-33.5627799550483,-66.1435466211076,
0.));
#134646=CARTESIAN_POINT('Ctrl Pts',(-33.5627799550483,-66.1435466211076,
12.));
#134647=CARTESIAN_POINT('Ctrl Pts',(-33.5413811223451,-66.1262614234674,
0.));
#134648=CARTESIAN_POINT('Ctrl Pts',(-33.5413811223451,-66.1262614234674,
12.));
#134649=CARTESIAN_POINT('Ctrl Pts',(-33.5200254081243,-66.1089790592729,
0.));
#134650=CARTESIAN_POINT('Ctrl Pts',(-33.5200254081243,-66.1089790592729,
12.));
#134651=CARTESIAN_POINT('Ctrl Pts',(-33.4987128476622,-66.0916996085244,
0.));
#134652=CARTESIAN_POINT('Ctrl Pts',(-33.4987128476622,-66.0916996085244,
12.));
#134653=CARTESIAN_POINT('Ctrl Pts',(-33.4774434765746,-66.0744231525415,
0.));
#134654=CARTESIAN_POINT('Ctrl Pts',(-33.4774434765746,-66.0744231525415,
12.));
#134655=CARTESIAN_POINT('Ctrl Pts',(-33.4562173318025,-66.0571497774434,
0.));
#134656=CARTESIAN_POINT('Ctrl Pts',(-33.4562173318025,-66.0571497774434,
12.));
#134657=CARTESIAN_POINT('Ctrl Pts',(-33.4350344515101,-66.0398795737777,
0.));
#134658=CARTESIAN_POINT('Ctrl Pts',(-33.4350344515101,-66.0398795737777,
12.));
#134659=CARTESIAN_POINT('Ctrl Pts',(-33.4138948746388,-66.0226126349446,
0.));
#134660=CARTESIAN_POINT('Ctrl Pts',(-33.4138948746388,-66.0226126349446,
12.));
#134661=CARTESIAN_POINT('Ctrl Pts',(-33.3927986405605,-66.0053490559812,
0.));
#134662=CARTESIAN_POINT('Ctrl Pts',(-33.3927986405605,-66.0053490559812,
12.));
#134663=CARTESIAN_POINT('Ctrl Pts',(-33.37174578871,-65.9880889322831,0.));
#134664=CARTESIAN_POINT('Ctrl Pts',(-33.37174578871,-65.9880889322831,12.));
#134665=CARTESIAN_POINT('Ctrl Pts',(-33.3507363581593,-65.970832358141,
0.));
#134666=CARTESIAN_POINT('Ctrl Pts',(-33.3507363581593,-65.970832358141,
12.));
#134667=CARTESIAN_POINT('Ctrl Pts',(-33.3297703874266,-65.9535794260831,
0.));
#134668=CARTESIAN_POINT('Ctrl Pts',(-33.3297703874266,-65.9535794260831,
12.));
#134669=CARTESIAN_POINT('Ctrl Pts',(-33.3088479147164,-65.9363302276846,
0.));
#134670=CARTESIAN_POINT('Ctrl Pts',(-33.3088479147164,-65.9363302276846,
12.));
#134671=CARTESIAN_POINT('Ctrl Pts',(-33.2879689780573,-65.9190848540433,
0.));
#134672=CARTESIAN_POINT('Ctrl Pts',(-33.2879689780573,-65.9190848540433,
12.));
#134673=CARTESIAN_POINT('Ctrl Pts',(-33.2671336154754,-65.9018433963889,
0.));
#134674=CARTESIAN_POINT('Ctrl Pts',(-33.2671336154754,-65.9018433963889,
12.));
#134675=CARTESIAN_POINT('Ctrl Pts',(-33.2463418651493,-65.8846059466371,
0.));
#134676=CARTESIAN_POINT('Ctrl Pts',(-33.2463418651493,-65.8846059466371,
12.));
#134677=CARTESIAN_POINT('Ctrl Pts',(-33.2255937655649,-65.8673725979577,
0.));
#134678=CARTESIAN_POINT('Ctrl Pts',(-33.2255937655649,-65.8673725979577,
12.));
#134679=CARTESIAN_POINT('Ctrl Pts',(-33.2048893554491,-65.8501434445164,
0.));
#134680=CARTESIAN_POINT('Ctrl Pts',(-33.2048893554491,-65.8501434445164,
12.));
#134681=CARTESIAN_POINT('Ctrl Pts',(-33.1842286737051,-65.8329185812375,
0.));
#134682=CARTESIAN_POINT('Ctrl Pts',(-33.1842286737051,-65.8329185812375,
12.));
#134683=CARTESIAN_POINT('Ctrl Pts',(-33.16361175934,-65.8156981035503,0.));
#134684=CARTESIAN_POINT('Ctrl Pts',(-33.16361175934,-65.8156981035503,12.));
#134685=CARTESIAN_POINT('Ctrl Pts',(-33.1430386513976,-65.7984821071623,
0.));
#134686=CARTESIAN_POINT('Ctrl Pts',(-33.1430386513976,-65.7984821071623,
12.));
#134687=CARTESIAN_POINT('Ctrl Pts',(-33.1225093888672,-65.7812706877696,
0.));
#134688=CARTESIAN_POINT('Ctrl Pts',(-33.1225093888672,-65.7812706877696,
12.));
#134689=CARTESIAN_POINT('Ctrl Pts',(-33.1020240106885,-65.7640639410661,
0.));
#134690=CARTESIAN_POINT('Ctrl Pts',(-33.1020240106885,-65.7640639410661,
12.));
#134691=CARTESIAN_POINT('Ctrl Pts',(-33.081582555798,-65.7468619628815,
0.));
#134692=CARTESIAN_POINT('Ctrl Pts',(-33.081582555798,-65.7468619628815,
12.));
#134693=CARTESIAN_POINT('Ctrl Pts',(-33.0611850631582,-65.7296648492824,
0.));
#134694=CARTESIAN_POINT('Ctrl Pts',(-33.0611850631582,-65.7296648492824,
12.));
#134695=CARTESIAN_POINT('Ctrl Pts',(-33.0408315717873,-65.7124726966802,
0.));
#134696=CARTESIAN_POINT('Ctrl Pts',(-33.0408315717873,-65.7124726966802,
12.));
#134697=CARTESIAN_POINT('Ctrl Pts',(-33.0205221207873,-65.6952856019533,
0.));
#134698=CARTESIAN_POINT('Ctrl Pts',(-33.0205221207873,-65.6952856019533,
12.));
#134699=CARTESIAN_POINT('Ctrl Pts',(-33.0002567493574,-65.6781036625027,
0.));
#134700=CARTESIAN_POINT('Ctrl Pts',(-33.0002567493574,-65.6781036625027,
12.));
#134701=CARTESIAN_POINT('Ctrl Pts',(-32.980035496784,-65.6609269761888,
0.));
#134702=CARTESIAN_POINT('Ctrl Pts',(-32.980035496784,-65.6609269761888,
12.));
#134703=CARTESIAN_POINT('Ctrl Pts',(-32.9598584024313,-65.6437556412946,
0.));
#134704=CARTESIAN_POINT('Ctrl Pts',(-32.9598584024313,-65.6437556412946,
12.));
#134705=CARTESIAN_POINT('Ctrl Pts',(-32.9397255057274,-65.6265897564783,
0.));
#134706=CARTESIAN_POINT('Ctrl Pts',(-32.9397255057274,-65.6265897564783,
12.));
#134707=CARTESIAN_POINT('Ctrl Pts',(-32.9196368461463,-65.6094294207276,
0.));
#134708=CARTESIAN_POINT('Ctrl Pts',(-32.9196368461463,-65.6094294207276,
12.));
#134709=CARTESIAN_POINT('Ctrl Pts',(-32.8995924631898,-65.5922747333194,
0.));
#134710=CARTESIAN_POINT('Ctrl Pts',(-32.8995924631898,-65.5922747333194,
12.));
#134711=CARTESIAN_POINT('Ctrl Pts',(-32.879592396403,-65.5751257938472,
0.));
#134712=CARTESIAN_POINT('Ctrl Pts',(-32.879592396403,-65.5751257938472,
12.));
#134713=CARTESIAN_POINT('Ctrl Pts',(-32.8596366853832,-65.5579827022421,
0.));
#134714=CARTESIAN_POINT('Ctrl Pts',(-32.8596366853832,-65.5579827022421,
12.));
#134715=CARTESIAN_POINT('Ctrl Pts',(-32.8397253697866,-65.5408455587964,
0.));
#134716=CARTESIAN_POINT('Ctrl Pts',(-32.8397253697866,-65.5408455587964,
12.));
#134717=CARTESIAN_POINT('Ctrl Pts',(-32.8198584893316,-65.5237144641857,
0.));
#134718=CARTESIAN_POINT('Ctrl Pts',(-32.8198584893316,-65.5237144641857,
12.));
#134719=CARTESIAN_POINT('Ctrl Pts',(-32.8000360837975,-65.5065895194928,
0.));
#134720=CARTESIAN_POINT('Ctrl Pts',(-32.8000360837975,-65.5065895194928,
12.));
#134721=CARTESIAN_POINT('Ctrl Pts',(-32.7802581930287,-65.489470826206,
0.));
#134722=CARTESIAN_POINT('Ctrl Pts',(-32.7802581930287,-65.489470826206,
12.));
#134723=CARTESIAN_POINT('Ctrl Pts',(-32.7605248569378,-65.4723584862122,
0.));
#134724=CARTESIAN_POINT('Ctrl Pts',(-32.7605248569378,-65.4723584862122,
12.));
#134725=CARTESIAN_POINT('Ctrl Pts',(-32.7408361155037,-65.4552526017905,
0.));
#134726=CARTESIAN_POINT('Ctrl Pts',(-32.7408361155037,-65.4552526017905,
12.));
#134727=CARTESIAN_POINT('Ctrl Pts',(-32.7211920087684,-65.4381532756065,
0.));
#134728=CARTESIAN_POINT('Ctrl Pts',(-32.7211920087684,-65.4381532756065,
12.));
#134729=CARTESIAN_POINT('Ctrl Pts',(-32.7015925768265,-65.4210606107035,
0.));
#134730=CARTESIAN_POINT('Ctrl Pts',(-32.7015925768265,-65.4210606107035,
12.));
#134731=CARTESIAN_POINT('Ctrl Pts',(-32.6820378598267,-65.4039747105038,
0.));
#134732=CARTESIAN_POINT('Ctrl Pts',(-32.6820378598267,-65.4039747105038,
12.));
#134733=CARTESIAN_POINT('Ctrl Pts',(-32.6625278979811,-65.3868956788182,
0.));
#134734=CARTESIAN_POINT('Ctrl Pts',(-32.6625278979811,-65.3868956788182,
12.));
#134735=CARTESIAN_POINT('Ctrl Pts',(-32.6430627315674,-65.3698236198512,
0.));
#134736=CARTESIAN_POINT('Ctrl Pts',(-32.6430627315674,-65.3698236198512,
12.));
#134737=CARTESIAN_POINT('Ctrl Pts',(-32.6236424009301,-65.3527586382081,
0.));
#134738=CARTESIAN_POINT('Ctrl Pts',(-32.6236424009301,-65.3527586382081,
12.));
#134739=CARTESIAN_POINT('Ctrl Pts',(-32.6042669464751,-65.3357008389003,
0.));
#134740=CARTESIAN_POINT('Ctrl Pts',(-32.6042669464751,-65.3357008389003,
12.));
#134741=CARTESIAN_POINT('Ctrl Pts',(-32.5849364086679,-65.31865032735,0.));
#134742=CARTESIAN_POINT('Ctrl Pts',(-32.5849364086679,-65.31865032735,12.));
#134743=CARTESIAN_POINT('Ctrl Pts',(-32.5656508280422,-65.3016072093912,
0.));
#134744=CARTESIAN_POINT('Ctrl Pts',(-32.5656508280422,-65.3016072093912,
12.));
#134745=CARTESIAN_POINT('Ctrl Pts',(-32.5464102452015,-65.2845715912721,
0.));
#134746=CARTESIAN_POINT('Ctrl Pts',(-32.5464102452015,-65.2845715912721,
12.));
#134747=CARTESIAN_POINT('Ctrl Pts',(-32.5272147008191,-65.2675435796558,
0.));
#134748=CARTESIAN_POINT('Ctrl Pts',(-32.5272147008191,-65.2675435796558,
12.));
#134749=CARTESIAN_POINT('Ctrl Pts',(-32.5080642356328,-65.2505232816209,
0.));
#134750=CARTESIAN_POINT('Ctrl Pts',(-32.5080642356328,-65.2505232816209,
12.));
#134751=CARTESIAN_POINT('Ctrl Pts',(-32.4889588904392,-65.2335108046614,
0.));
#134752=CARTESIAN_POINT('Ctrl Pts',(-32.4889588904392,-65.2335108046614,
12.));
#134753=CARTESIAN_POINT('Ctrl Pts',(-32.4698987061032,-65.2165062566924,
0.));
#134754=CARTESIAN_POINT('Ctrl Pts',(-32.4698987061032,-65.2165062566924,
12.));
#134755=CARTESIAN_POINT('Ctrl Pts',(-32.450883723561,-65.1995097460538,
0.));
#134756=CARTESIAN_POINT('Ctrl Pts',(-32.450883723561,-65.1995097460538,
12.));
#134757=CARTESIAN_POINT('Ctrl Pts',(-32.4319139838213,-65.182521381514,
0.));
#134758=CARTESIAN_POINT('Ctrl Pts',(-32.4319139838213,-65.182521381514,
12.));
#134759=CARTESIAN_POINT('Ctrl Pts',(-32.4129895279615,-65.1655412722725,
0.));
#134760=CARTESIAN_POINT('Ctrl Pts',(-32.4129895279615,-65.1655412722725,
12.));
#134761=CARTESIAN_POINT('Ctrl Pts',(-32.3941103971221,-65.1485695279635,
0.));
#134762=CARTESIAN_POINT('Ctrl Pts',(-32.3941103971221,-65.1485695279635,
12.));
#134763=CARTESIAN_POINT('Ctrl Pts',(-32.3752766325136,-65.1316062586588,
0.));
#134764=CARTESIAN_POINT('Ctrl Pts',(-32.3752766325136,-65.1316062586588,
12.));
#134765=CARTESIAN_POINT('Ctrl Pts',(-32.3564882754212,-65.1146515748722,
0.));
#134766=CARTESIAN_POINT('Ctrl Pts',(-32.3564882754212,-65.1146515748722,
12.));
#134767=CARTESIAN_POINT('Ctrl Pts',(-32.3377453672051,-65.0977055875607,
0.));
#134768=CARTESIAN_POINT('Ctrl Pts',(-32.3377453672051,-65.0977055875607,
12.));
#134769=CARTESIAN_POINT('Ctrl Pts',(-32.3190479492987,-65.0807684081281,
0.));
#134770=CARTESIAN_POINT('Ctrl Pts',(-32.3190479492987,-65.0807684081281,
12.));
#134771=CARTESIAN_POINT('Ctrl Pts',(-32.3003960632007,-65.0638401484257,
0.));
#134772=CARTESIAN_POINT('Ctrl Pts',(-32.3003960632007,-65.0638401484257,
12.));
#134773=CARTESIAN_POINT('Ctrl Pts',(-32.2817897504807,-65.0469209207563,
0.));
#134774=CARTESIAN_POINT('Ctrl Pts',(-32.2817897504807,-65.0469209207563,
12.));
#134775=CARTESIAN_POINT('Ctrl Pts',(-32.2632290527862,-65.03001083788,0.));
#134776=CARTESIAN_POINT('Ctrl Pts',(-32.2632290527862,-65.03001083788,12.));
#134777=CARTESIAN_POINT('Ctrl Pts',(-32.2447140118422,-65.0131100130157,
0.));
#134778=CARTESIAN_POINT('Ctrl Pts',(-32.2447140118422,-65.0131100130157,
12.));
#134779=CARTESIAN_POINT('Ctrl Pts',(-32.2262446694513,-64.9962185598461,
0.));
#134780=CARTESIAN_POINT('Ctrl Pts',(-32.2262446694513,-64.9962185598461,
12.));
#134781=CARTESIAN_POINT('Ctrl Pts',(-32.207821067485,-64.9793365925178,
0.));
#134782=CARTESIAN_POINT('Ctrl Pts',(-32.207821067485,-64.9793365925178,
12.));
#134783=CARTESIAN_POINT('Ctrl Pts',(-32.1894432478881,-64.9624642256461,
0.));
#134784=CARTESIAN_POINT('Ctrl Pts',(-32.1894432478881,-64.9624642256461,
12.));
#134785=CARTESIAN_POINT('Ctrl Pts',(-32.1711112526855,-64.9456015743192,
0.));
#134786=CARTESIAN_POINT('Ctrl Pts',(-32.1711112526855,-64.9456015743192,
12.));
#134787=CARTESIAN_POINT('Ctrl Pts',(-32.1528251239831,-64.9287487541015,
0.));
#134788=CARTESIAN_POINT('Ctrl Pts',(-32.1528251239831,-64.9287487541015,
12.));
#134789=CARTESIAN_POINT('Ctrl Pts',(-32.1345849039674,-64.9119058810366,
0.));
#134790=CARTESIAN_POINT('Ctrl Pts',(-32.1345849039674,-64.9119058810366,
12.));
#134791=CARTESIAN_POINT('Ctrl Pts',(-32.1163906348984,-64.8950730716501,
0.));
#134792=CARTESIAN_POINT('Ctrl Pts',(-32.1163906348984,-64.8950730716501,
12.));
#134793=CARTESIAN_POINT('Ctrl Pts',(-32.0982423591113,-64.8782504429527,
0.));
#134794=CARTESIAN_POINT('Ctrl Pts',(-32.0982423591113,-64.8782504429527,
12.));
#134795=CARTESIAN_POINT('Ctrl Pts',(-32.0801401190244,-64.8614381124454,
0.));
#134796=CARTESIAN_POINT('Ctrl Pts',(-32.0801401190244,-64.8614381124454,
12.));
#134797=CARTESIAN_POINT('Ctrl Pts',(-32.0620839571409,-64.8446361981234,
0.));
#134798=CARTESIAN_POINT('Ctrl Pts',(-32.0620839571409,-64.8446361981234,
12.));
#134799=CARTESIAN_POINT('Ctrl Pts',(-32.0440739160477,-64.8278448184785,
0.));
#134800=CARTESIAN_POINT('Ctrl Pts',(-32.0440739160477,-64.8278448184785,
12.));
#134801=CARTESIAN_POINT('Ctrl Pts',(-32.0261100384092,-64.811064092502,
0.));
#134802=CARTESIAN_POINT('Ctrl Pts',(-32.0261100384092,-64.811064092502,
12.));
#134803=CARTESIAN_POINT('Ctrl Pts',(-32.0081923669678,-64.7942941396883,
0.));
#134804=CARTESIAN_POINT('Ctrl Pts',(-32.0081923669678,-64.7942941396883,
12.));
#134805=CARTESIAN_POINT('Ctrl Pts',(-31.9903209445522,-64.7775350800404,
0.));
#134806=CARTESIAN_POINT('Ctrl Pts',(-31.9903209445522,-64.7775350800404,
12.));
#134807=CARTESIAN_POINT('Ctrl Pts',(-31.9724958140791,-64.7607870340738,
0.));
#134808=CARTESIAN_POINT('Ctrl Pts',(-31.9724958140791,-64.7607870340738,
12.));
#134809=CARTESIAN_POINT('Ctrl Pts',(-31.9547170185533,-64.74405012282,0.));
#134810=CARTESIAN_POINT('Ctrl Pts',(-31.9547170185533,-64.74405012282,12.));
#134811=CARTESIAN_POINT('Ctrl Pts',(-31.9369846010613,-64.727324467829,
0.));
#134812=CARTESIAN_POINT('Ctrl Pts',(-31.9369846010613,-64.727324467829,
12.));
#134813=CARTESIAN_POINT('Ctrl Pts',(-31.9192986047702,-64.7106101911722,
0.));
#134814=CARTESIAN_POINT('Ctrl Pts',(-31.9192986047702,-64.7106101911722,
12.));
#134815=CARTESIAN_POINT('Ctrl Pts',(-31.9016590729371,-64.693907415449,
0.));
#134816=CARTESIAN_POINT('Ctrl Pts',(-31.9016590729371,-64.693907415449,
12.));
#134817=CARTESIAN_POINT('Ctrl Pts',(-31.8840660489106,-64.6772162637904,
0.));
#134818=CARTESIAN_POINT('Ctrl Pts',(-31.8840660489106,-64.6772162637904,
12.));
#134819=CARTESIAN_POINT('Ctrl Pts',(-31.8665195761312,-64.6605368598631,
0.));
#134820=CARTESIAN_POINT('Ctrl Pts',(-31.8665195761312,-64.6605368598631,
12.));
#134821=CARTESIAN_POINT('Ctrl Pts',(-31.849019698125,-64.6438693278718,
0.));
#134822=CARTESIAN_POINT('Ctrl Pts',(-31.849019698125,-64.6438693278718,
12.));
#134823=CARTESIAN_POINT('Ctrl Pts',(-31.8315664585027,-64.6272137925629,
0.));
#134824=CARTESIAN_POINT('Ctrl Pts',(-31.8315664585027,-64.6272137925629,
12.));
#134825=CARTESIAN_POINT('Ctrl Pts',(-31.8141599009685,-64.6105703792311,
0.));
#134826=CARTESIAN_POINT('Ctrl Pts',(-31.8141599009685,-64.6105703792311,
12.));
#134827=CARTESIAN_POINT('Ctrl Pts',(-31.7968000693218,-64.5939392137233,
0.));
#134828=CARTESIAN_POINT('Ctrl Pts',(-31.7968000693218,-64.5939392137233,
12.));
#134829=CARTESIAN_POINT('Ctrl Pts',(-31.7794870074584,-64.5773204224429,
0.));
#134830=CARTESIAN_POINT('Ctrl Pts',(-31.7794870074584,-64.5773204224429,
12.));
#134831=CARTESIAN_POINT('Ctrl Pts',(-31.7622207593637,-64.5607141323527,
0.));
#134832=CARTESIAN_POINT('Ctrl Pts',(-31.7622207593637,-64.5607141323527,
12.));
#134833=CARTESIAN_POINT('Ctrl Pts',(-31.7450013691117,-64.5441204709779,
0.));
#134834=CARTESIAN_POINT('Ctrl Pts',(-31.7450013691117,-64.5441204709779,
12.));
#134835=CARTESIAN_POINT('Ctrl Pts',(-31.7278288808736,-64.5275395664134,
0.));
#134836=CARTESIAN_POINT('Ctrl Pts',(-31.7278288808736,-64.5275395664134,
12.));
#134837=CARTESIAN_POINT('Ctrl Pts',(-31.7107033389204,-64.5109715473276,
0.));
#134838=CARTESIAN_POINT('Ctrl Pts',(-31.7107033389204,-64.5109715473276,
12.));
#134839=CARTESIAN_POINT('Ctrl Pts',(-31.6936247876228,-64.4944165429672,
0.));
#134840=CARTESIAN_POINT('Ctrl Pts',(-31.6936247876228,-64.4944165429672,
12.));
#134841=CARTESIAN_POINT('Ctrl Pts',(-31.6765932714456,-64.4778746831597,
0.));
#134842=CARTESIAN_POINT('Ctrl Pts',(-31.6765932714456,-64.4778746831597,
12.));
#134843=CARTESIAN_POINT('Ctrl Pts',(-31.6596088349468,-64.4613460983186,
0.));
#134844=CARTESIAN_POINT('Ctrl Pts',(-31.6596088349468,-64.4613460983186,
12.));
#134845=CARTESIAN_POINT('Ctrl Pts',(-31.6426715227865,-64.4448309194498,
0.));
#134846=CARTESIAN_POINT('Ctrl Pts',(-31.6426715227865,-64.4448309194498,
12.));
#134847=CARTESIAN_POINT('Ctrl Pts',(-31.6257813797282,-64.4283292781553,
0.));
#134848=CARTESIAN_POINT('Ctrl Pts',(-31.6257813797282,-64.4283292781553,
12.));
#134849=CARTESIAN_POINT('Ctrl Pts',(-31.6089384506399,-64.4118413066386,
0.));
#134850=CARTESIAN_POINT('Ctrl Pts',(-31.6089384506399,-64.4118413066386,
12.));
#134851=CARTESIAN_POINT('Ctrl Pts',(-31.5921427804879,-64.3953671377071,
0.));
#134852=CARTESIAN_POINT('Ctrl Pts',(-31.5921427804879,-64.3953671377071,
12.));
#134853=CARTESIAN_POINT('Ctrl Pts',(-31.5753944143355,-64.3789069047768,
0.));
#134854=CARTESIAN_POINT('Ctrl Pts',(-31.5753944143355,-64.3789069047768,
12.));
#134855=CARTESIAN_POINT('Ctrl Pts',(-31.5586933973532,-64.3624607418798,
0.));
#134856=CARTESIAN_POINT('Ctrl Pts',(-31.5586933973532,-64.3624607418798,
12.));
#134857=CARTESIAN_POINT('Ctrl Pts',(-31.5420397748198,-64.34602878367,0.));
#134858=CARTESIAN_POINT('Ctrl Pts',(-31.5420397748198,-64.34602878367,12.));
#134859=CARTESIAN_POINT('Ctrl Pts',(-31.525433592124,-64.3296111654273,
0.));
#134860=CARTESIAN_POINT('Ctrl Pts',(-31.525433592124,-64.3296111654273,
12.));
#134861=CARTESIAN_POINT('Ctrl Pts',(-31.5088748947565,-64.3132080230603,
0.));
#134862=CARTESIAN_POINT('Ctrl Pts',(-31.5088748947565,-64.3132080230603,
12.));
#134863=CARTESIAN_POINT('Ctrl Pts',(-31.4923637283109,-64.2968194931113,
0.));
#134864=CARTESIAN_POINT('Ctrl Pts',(-31.4923637283109,-64.2968194931113,
12.));
#134865=CARTESIAN_POINT('Ctrl Pts',(-31.4759001384923,-64.2804457127633,
0.));
#134866=CARTESIAN_POINT('Ctrl Pts',(-31.4759001384923,-64.2804457127633,
12.));
#134867=CARTESIAN_POINT('Ctrl Pts',(-31.4594841711189,-64.264086819846,
0.));
#134868=CARTESIAN_POINT('Ctrl Pts',(-31.4594841711189,-64.264086819846,
12.));
#134869=CARTESIAN_POINT('Ctrl Pts',(-31.443115872123,-64.2477429528408,
0.));
#134870=CARTESIAN_POINT('Ctrl Pts',(-31.443115872123,-64.2477429528408,
12.));
#134871=CARTESIAN_POINT('Ctrl Pts',(-31.426795287544,-64.2314142508843,
0.));
#134872=CARTESIAN_POINT('Ctrl Pts',(-31.426795287544,-64.2314142508843,
12.));
#134873=CARTESIAN_POINT('Ctrl Pts',(-31.4105224635298,-64.2151008537733,
0.));
#134874=CARTESIAN_POINT('Ctrl Pts',(-31.4105224635298,-64.2151008537733,
12.));
#134875=CARTESIAN_POINT('Ctrl Pts',(-31.3942974463458,-64.1988029019733,
0.));
#134876=CARTESIAN_POINT('Ctrl Pts',(-31.3942974463458,-64.1988029019733,
12.));
#134877=CARTESIAN_POINT('Ctrl Pts',(-31.3781202823758,-64.1825205366231,
0.));
#134878=CARTESIAN_POINT('Ctrl Pts',(-31.3781202823758,-64.1825205366231,
12.));
#134879=CARTESIAN_POINT('Ctrl Pts',(-31.3619910181223,-64.1662538995407,
0.));
#134880=CARTESIAN_POINT('Ctrl Pts',(-31.3619910181223,-64.1662538995407,
12.));
#134881=CARTESIAN_POINT('Ctrl Pts',(-31.3459097001996,-64.150003133226,
0.));
#134882=CARTESIAN_POINT('Ctrl Pts',(-31.3459097001996,-64.150003133226,
12.));
#134883=CARTESIAN_POINT('Ctrl Pts',(-31.3298763753366,-64.1337683808667,
0.));
#134884=CARTESIAN_POINT('Ctrl Pts',(-31.3298763753366,-64.1337683808667,
12.));
#134885=CARTESIAN_POINT('Ctrl Pts',(-31.3138910903852,-64.1175497863475,
0.));
#134886=CARTESIAN_POINT('Ctrl Pts',(-31.3138910903852,-64.1175497863475,
12.));
#134887=CARTESIAN_POINT('Ctrl Pts',(-31.2979538923214,-64.1013474942554,
0.));
#134888=CARTESIAN_POINT('Ctrl Pts',(-31.2979538923214,-64.1013474942554,
12.));
#134889=CARTESIAN_POINT('Ctrl Pts',(-31.2820648282451,-64.0851616498861,
0.));
#134890=CARTESIAN_POINT('Ctrl Pts',(-31.2820648282451,-64.0851616498861,
12.));
#134891=CARTESIAN_POINT('Ctrl Pts',(-31.2662239453734,-64.0689923992474,
0.));
#134892=CARTESIAN_POINT('Ctrl Pts',(-31.2662239453734,-64.0689923992474,
12.));
#134893=CARTESIAN_POINT('Ctrl Pts',(-31.2504312910457,-64.0528398890671,
0.));
#134894=CARTESIAN_POINT('Ctrl Pts',(-31.2504312910457,-64.0528398890671,
12.));
#134895=CARTESIAN_POINT('Ctrl Pts',(-31.23468691273,-64.036704266799,0.));
#134896=CARTESIAN_POINT('Ctrl Pts',(-31.23468691273,-64.036704266799,12.));
#134897=CARTESIAN_POINT('Ctrl Pts',(-31.2189908580245,-64.0205856806298,
0.));
#134898=CARTESIAN_POINT('Ctrl Pts',(-31.2189908580245,-64.0205856806298,
12.));
#134899=CARTESIAN_POINT('Ctrl Pts',(-31.2033431746559,-64.004484279483,
0.));
#134900=CARTESIAN_POINT('Ctrl Pts',(-31.2033431746559,-64.004484279483,
12.));
#134901=CARTESIAN_POINT('Ctrl Pts',(-31.1877439104717,-63.9884002130209,
0.));
#134902=CARTESIAN_POINT('Ctrl Pts',(-31.1877439104717,-63.9884002130209,
12.));
#134903=CARTESIAN_POINT('Ctrl Pts',(-31.1721931134488,-63.972333631655,
0.));
#134904=CARTESIAN_POINT('Ctrl Pts',(-31.1721931134488,-63.972333631655,
12.));
#134905=CARTESIAN_POINT('Ctrl Pts',(-31.1566908316993,-63.9562846865566,
0.));
#134906=CARTESIAN_POINT('Ctrl Pts',(-31.1566908316993,-63.9562846865566,
12.));
#134907=CARTESIAN_POINT('Ctrl Pts',(-31.1412371134727,-63.940253529665,
0.));
#134908=CARTESIAN_POINT('Ctrl Pts',(-31.1412371134727,-63.940253529665,
12.));
#134909=CARTESIAN_POINT('Ctrl Pts',(-31.1258320071545,-63.9242403136954,
0.));
#134910=CARTESIAN_POINT('Ctrl Pts',(-31.1258320071545,-63.9242403136954,
12.));
#134911=CARTESIAN_POINT('Ctrl Pts',(-31.1104755612606,-63.9082451921447,
0.));
#134912=CARTESIAN_POINT('Ctrl Pts',(-31.1104755612606,-63.9082451921447,
12.));
#134913=CARTESIAN_POINT('Ctrl Pts',(-31.0951678244454,-63.8922683192962,
0.));
#134914=CARTESIAN_POINT('Ctrl Pts',(-31.0951678244454,-63.8922683192962,
12.));
#134915=CARTESIAN_POINT('Ctrl Pts',(-31.079908845504,-63.8763098502235,
0.));
#134916=CARTESIAN_POINT('Ctrl Pts',(-31.079908845504,-63.8763098502235,
12.));
#134917=CARTESIAN_POINT('Ctrl Pts',(-31.0646986733724,-63.8603699407922,
0.));
#134918=CARTESIAN_POINT('Ctrl Pts',(-31.0646986733724,-63.8603699407922,
12.));
#134919=CARTESIAN_POINT('Ctrl Pts',(-31.0495373571218,-63.8444487476615,
0.));
#134920=CARTESIAN_POINT('Ctrl Pts',(-31.0495373571218,-63.8444487476615,
12.));
#134921=CARTESIAN_POINT('Ctrl Pts',(-31.0344249459544,-63.8285464282857,
0.));
#134922=CARTESIAN_POINT('Ctrl Pts',(-31.0344249459544,-63.8285464282857,
12.));
#134923=CARTESIAN_POINT('Ctrl Pts',(-31.0193614892177,-63.8126631409376,
0.));
#134924=CARTESIAN_POINT('Ctrl Pts',(-31.0193614892177,-63.8126631409376,
12.));
#134925=CARTESIAN_POINT('Ctrl Pts',(-31.0043470364112,-63.7967990447287,
0.));
#134926=CARTESIAN_POINT('Ctrl Pts',(-31.0043470364112,-63.7967990447287,
12.));
#134927=CARTESIAN_POINT('Ctrl Pts',(-30.9893816371907,-63.7809542996258,
0.));
#134928=CARTESIAN_POINT('Ctrl Pts',(-30.9893816371907,-63.7809542996258,
12.));
#134929=CARTESIAN_POINT('Ctrl Pts',(-30.9744653413679,-63.7651290664713,
0.));
#134930=CARTESIAN_POINT('Ctrl Pts',(-30.9744653413679,-63.7651290664713,
12.));
#134931=CARTESIAN_POINT('Ctrl Pts',(-30.9595981989091,-63.7493235069844,
0.));
#134932=CARTESIAN_POINT('Ctrl Pts',(-30.9595981989091,-63.7493235069844,
12.));
#134933=CARTESIAN_POINT('Ctrl Pts',(-30.9447802599345,-63.733537783742,
0.));
#134934=CARTESIAN_POINT('Ctrl Pts',(-30.9447802599345,-63.733537783742,
12.));
#134935=CARTESIAN_POINT('Ctrl Pts',(-30.9300115747113,-63.7177720601604,
0.));
#134936=CARTESIAN_POINT('Ctrl Pts',(-30.9300115747113,-63.7177720601604,
12.));
#134937=CARTESIAN_POINT('Ctrl Pts',(-30.9152921936471,-63.7020265004805,
0.));
#134938=CARTESIAN_POINT('Ctrl Pts',(-30.9152921936471,-63.7020265004805,
12.));
#134939=CARTESIAN_POINT('Ctrl Pts',(-30.9006221672703,-63.6863012697353,
0.));
#134940=CARTESIAN_POINT('Ctrl Pts',(-30.9006221672703,-63.6863012697353,
12.));
#134941=CARTESIAN_POINT('Ctrl Pts',(-30.8860015462488,-63.6705965337996,
0.));
#134942=CARTESIAN_POINT('Ctrl Pts',(-30.8860015462488,-63.6705965337996,
12.));
#134943=CARTESIAN_POINT('Ctrl Pts',(-30.8714303814202,-63.6549124594681,
0.));
#134944=CARTESIAN_POINT('Ctrl Pts',(-30.8714303814202,-63.6549124594681,
12.));
#134945=CARTESIAN_POINT('Ctrl Pts',(-30.8569087238132,-63.6392492145233,
0.));
#134946=CARTESIAN_POINT('Ctrl Pts',(-30.8569087238132,-63.6392492145233,
12.));
#134947=CARTESIAN_POINT('Ctrl Pts',(-30.8424366246665,-63.6236069678041,
0.));
#134948=CARTESIAN_POINT('Ctrl Pts',(-30.8424366246665,-63.6236069678041,
12.));
#134949=CARTESIAN_POINT('Ctrl Pts',(-30.8280141354448,-63.6079858892746,
0.));
#134950=CARTESIAN_POINT('Ctrl Pts',(-30.8280141354448,-63.6079858892746,
12.));
#134951=CARTESIAN_POINT('Ctrl Pts',(-30.8136413077999,-63.5923861498963,
0.));
#134952=CARTESIAN_POINT('Ctrl Pts',(-30.8136413077999,-63.5923861498963,
12.));
#134953=CARTESIAN_POINT('Ctrl Pts',(-30.7993181935265,-63.5768079214868,
0.));
#134954=CARTESIAN_POINT('Ctrl Pts',(-30.7993181935265,-63.5768079214868,
12.));
#134955=CARTESIAN_POINT('Ctrl Pts',(-30.7850448445207,-63.5612513766005,
0.));
#134956=CARTESIAN_POINT('Ctrl Pts',(-30.7850448445207,-63.5612513766005,
12.));
#134957=CARTESIAN_POINT('Ctrl Pts',(-30.7708213127169,-63.5457166883558,
0.));
#134958=CARTESIAN_POINT('Ctrl Pts',(-30.7708213127169,-63.5457166883558,
12.));
#134959=CARTESIAN_POINT('Ctrl Pts',(-30.7566476500772,-63.5302040304173,
0.));
#134960=CARTESIAN_POINT('Ctrl Pts',(-30.7566476500772,-63.5302040304173,
12.));
#134961=CARTESIAN_POINT('Ctrl Pts',(-30.7425239087294,-63.514713577392,
0.));
#134962=CARTESIAN_POINT('Ctrl Pts',(-30.7425239087294,-63.514713577392,
12.));
#134963=CARTESIAN_POINT('Ctrl Pts',(-30.7284501410827,-63.4992455051805,
0.));
#134964=CARTESIAN_POINT('Ctrl Pts',(-30.7284501410827,-63.4992455051805,
12.));
#134965=CARTESIAN_POINT('Ctrl Pts',(-30.7144263999259,-63.4837999912758,
0.));
#134966=CARTESIAN_POINT('Ctrl Pts',(-30.7144263999259,-63.4837999912758,
12.));
#134967=CARTESIAN_POINT('Ctrl Pts',(-30.7004527385806,-63.4683772152497,
0.));
#134968=CARTESIAN_POINT('Ctrl Pts',(-30.7004527385806,-63.4683772152497,
12.));
#134969=CARTESIAN_POINT('Ctrl Pts',(-30.6865292107911,-63.452977358421,
0.));
#134970=CARTESIAN_POINT('Ctrl Pts',(-30.6865292107911,-63.452977358421,
12.));
#134971=CARTESIAN_POINT('Ctrl Pts',(-30.6726558704302,-63.4376006029575,
0.));
#134972=CARTESIAN_POINT('Ctrl Pts',(-30.6726558704302,-63.4376006029575,
12.));
#134973=CARTESIAN_POINT('Ctrl Pts',(-30.6588327712482,-63.4222471311236,
0.));
#134974=CARTESIAN_POINT('Ctrl Pts',(-30.6588327712482,-63.4222471311236,
12.));
#134975=CARTESIAN_POINT('Ctrl Pts',(-30.6450599666135,-63.4069171245093,
0.));
#134976=CARTESIAN_POINT('Ctrl Pts',(-30.6450599666135,-63.4069171245093,
12.));
#134977=CARTESIAN_POINT('Ctrl Pts',(-30.6313375092085,-63.3916107631421,
0.));
#134978=CARTESIAN_POINT('Ctrl Pts',(-30.6313375092085,-63.3916107631421,
12.));
#134979=CARTESIAN_POINT('Ctrl Pts',(-30.6176654515988,-63.3763282271838,
0.));
#134980=CARTESIAN_POINT('Ctrl Pts',(-30.6176654515988,-63.3763282271838,
12.));
#134981=CARTESIAN_POINT('Ctrl Pts',(-30.604043846909,-63.3610696989599,
0.));
#134982=CARTESIAN_POINT('Ctrl Pts',(-30.604043846909,-63.3610696989599,
12.));
#134983=CARTESIAN_POINT('Ctrl Pts',(-30.5904727493707,-63.3458353646144,
0.));
#134984=CARTESIAN_POINT('Ctrl Pts',(-30.5904727493707,-63.3458353646144,
12.));
#134985=CARTESIAN_POINT('Ctrl Pts',(-30.5769522151147,-63.330625416509,
0.));
#134986=CARTESIAN_POINT('Ctrl Pts',(-30.5769522151147,-63.330625416509,
12.));
#134987=CARTESIAN_POINT('Ctrl Pts',(-30.5634823022358,-63.315440053435,
0.));
#134988=CARTESIAN_POINT('Ctrl Pts',(-30.5634823022358,-63.315440053435,
12.));
#134989=CARTESIAN_POINT('Ctrl Pts',(-30.5500630691343,-63.3002794756049,
0.));
#134990=CARTESIAN_POINT('Ctrl Pts',(-30.5500630691343,-63.3002794756049,
12.));
#134991=CARTESIAN_POINT('Ctrl Pts',(-30.5366945730503,-63.2851438802462,
0.));
#134992=CARTESIAN_POINT('Ctrl Pts',(-30.5366945730503,-63.2851438802462,
12.));
#134993=CARTESIAN_POINT('Ctrl Pts',(-30.5233768687875,-63.2700334577661,
0.));
#134994=CARTESIAN_POINT('Ctrl Pts',(-30.5233768687875,-63.2700334577661,
12.));
#134995=CARTESIAN_POINT('Ctrl Pts',(-30.5101100066683,-63.2549483856268,
0.));
#134996=CARTESIAN_POINT('Ctrl Pts',(-30.5101100066683,-63.2549483856268,
12.));
#134997=CARTESIAN_POINT('Ctrl Pts',(-30.4968940345028,-63.2398888342612,
0.));
#134998=CARTESIAN_POINT('Ctrl Pts',(-30.4968940345028,-63.2398888342612,
12.));
#134999=CARTESIAN_POINT('Ctrl Pts',(-30.4837290015011,-63.2248549788272,
0.));
#135000=CARTESIAN_POINT('Ctrl Pts',(-30.4837290015011,-63.2248549788272,
12.));
#135001=CARTESIAN_POINT('Ctrl Pts',(-30.470614961416,-63.2098470086636,
0.));
#135002=CARTESIAN_POINT('Ctrl Pts',(-30.470614961416,-63.2098470086636,
12.));
#135003=CARTESIAN_POINT('Ctrl Pts',(-30.4575519763305,-63.1948651386868,
0.));
#135004=CARTESIAN_POINT('Ctrl Pts',(-30.4575519763305,-63.1948651386868,
12.));
#135005=CARTESIAN_POINT('Ctrl Pts',(-30.4445401192324,-63.1799096171757,
0.));
#135006=CARTESIAN_POINT('Ctrl Pts',(-30.4445401192324,-63.1799096171757,
12.));
#135007=CARTESIAN_POINT('Ctrl Pts',(-30.431579465967,-63.1649807016766,
0.));
#135008=CARTESIAN_POINT('Ctrl Pts',(-30.431579465967,-63.1649807016766,
12.));
#135009=CARTESIAN_POINT('Ctrl Pts',(-30.4186700875598,-63.1500786361382,
0.));
#135010=CARTESIAN_POINT('Ctrl Pts',(-30.4186700875598,-63.1500786361382,
12.));
#135011=CARTESIAN_POINT('Ctrl Pts',(-30.4058120432259,-63.1352036298512,
0.));
#135012=CARTESIAN_POINT('Ctrl Pts',(-30.4058120432259,-63.1352036298512,
12.));
#135013=CARTESIAN_POINT('Ctrl Pts',(-30.3930053710592,-63.1203558300911,
0.));
#135014=CARTESIAN_POINT('Ctrl Pts',(-30.3930053710592,-63.1203558300911,
12.));
#135015=CARTESIAN_POINT('Ctrl Pts',(-30.3802500880565,-63.1055353202641,
0.));
#135016=CARTESIAN_POINT('Ctrl Pts',(-30.3802500880565,-63.1055353202641,
12.));
#135017=CARTESIAN_POINT('Ctrl Pts',(-30.3700869762658,-63.0937007763826,
0.));
#135018=CARTESIAN_POINT('Ctrl Pts',(-30.3700869762658,-63.0937007763826,
12.));
#135019=CARTESIAN_POINT('Ctrl Pts',(-30.3624877680747,-63.0848371718274,
0.));
#135020=CARTESIAN_POINT('Ctrl Pts',(-30.3624877680747,-63.0848371718274,
12.));
#135021=CARTESIAN_POINT('Ctrl Pts',(-30.3574319069366,-63.0789335700774,
0.));
#135022=CARTESIAN_POINT('Ctrl Pts',(-30.3574319069366,-63.0789335700774,
12.));
#135023=CARTESIAN_POINT('Ctrl Pts',(-30.3549065457811,-63.0759831361898,
0.));
#135024=CARTESIAN_POINT('Ctrl Pts',(-30.3549065457811,-63.0759831361898,
12.));
#135025=CARTESIAN_POINT('',(-30.3549065457811,-63.0759831361898,12.));
#135026=CARTESIAN_POINT('Ctrl Pts',(-30.3549065457811,-63.0759831361898,
12.));
#135027=CARTESIAN_POINT('Ctrl Pts',(-30.3574319069366,-63.0789335700774,
12.));
#135028=CARTESIAN_POINT('Ctrl Pts',(-30.3624877680747,-63.0848371718274,
12.));
#135029=CARTESIAN_POINT('Ctrl Pts',(-30.3700869762658,-63.0937007763826,
12.));
#135030=CARTESIAN_POINT('Ctrl Pts',(-30.3802500880565,-63.1055353202641,
12.));
#135031=CARTESIAN_POINT('Ctrl Pts',(-30.3930053710592,-63.1203558300911,
12.));
#135032=CARTESIAN_POINT('Ctrl Pts',(-30.4058120432259,-63.1352036298512,
12.));
#135033=CARTESIAN_POINT('Ctrl Pts',(-30.4186700875598,-63.1500786361382,
12.));
#135034=CARTESIAN_POINT('Ctrl Pts',(-30.431579465967,-63.1649807016766,
12.));
#135035=CARTESIAN_POINT('Ctrl Pts',(-30.4445401192324,-63.1799096171757,
12.));
#135036=CARTESIAN_POINT('Ctrl Pts',(-30.4575519763305,-63.1948651386868,
12.));
#135037=CARTESIAN_POINT('Ctrl Pts',(-30.470614961416,-63.2098470086636,
12.));
#135038=CARTESIAN_POINT('Ctrl Pts',(-30.4837290015011,-63.2248549788272,
12.));
#135039=CARTESIAN_POINT('Ctrl Pts',(-30.4968940345028,-63.2398888342612,
12.));
#135040=CARTESIAN_POINT('Ctrl Pts',(-30.5101100066683,-63.2549483856268,
12.));
#135041=CARTESIAN_POINT('Ctrl Pts',(-30.5233768687875,-63.2700334577661,
12.));
#135042=CARTESIAN_POINT('Ctrl Pts',(-30.5366945730503,-63.2851438802462,
12.));
#135043=CARTESIAN_POINT('Ctrl Pts',(-30.5500630691343,-63.3002794756049,
12.));
#135044=CARTESIAN_POINT('Ctrl Pts',(-30.5634823022358,-63.315440053435,
12.));
#135045=CARTESIAN_POINT('Ctrl Pts',(-30.5769522151147,-63.330625416509,
12.));
#135046=CARTESIAN_POINT('Ctrl Pts',(-30.5904727493707,-63.3458353646144,
12.));
#135047=CARTESIAN_POINT('Ctrl Pts',(-30.604043846909,-63.3610696989599,
12.));
#135048=CARTESIAN_POINT('Ctrl Pts',(-30.6176654515988,-63.3763282271838,
12.));
#135049=CARTESIAN_POINT('Ctrl Pts',(-30.6313375092085,-63.3916107631421,
12.));
#135050=CARTESIAN_POINT('Ctrl Pts',(-30.6450599666135,-63.4069171245093,
12.));
#135051=CARTESIAN_POINT('Ctrl Pts',(-30.6588327712482,-63.4222471311236,
12.));
#135052=CARTESIAN_POINT('Ctrl Pts',(-30.6726558704302,-63.4376006029575,
12.));
#135053=CARTESIAN_POINT('Ctrl Pts',(-30.6865292107911,-63.452977358421,
12.));
#135054=CARTESIAN_POINT('Ctrl Pts',(-30.7004527385806,-63.4683772152497,
12.));
#135055=CARTESIAN_POINT('Ctrl Pts',(-30.7144263999259,-63.4837999912758,
12.));
#135056=CARTESIAN_POINT('Ctrl Pts',(-30.7284501410827,-63.4992455051805,
12.));
#135057=CARTESIAN_POINT('Ctrl Pts',(-30.7425239087294,-63.514713577392,
12.));
#135058=CARTESIAN_POINT('Ctrl Pts',(-30.7566476500772,-63.5302040304173,
12.));
#135059=CARTESIAN_POINT('Ctrl Pts',(-30.7708213127169,-63.5457166883558,
12.));
#135060=CARTESIAN_POINT('Ctrl Pts',(-30.7850448445207,-63.5612513766005,
12.));
#135061=CARTESIAN_POINT('Ctrl Pts',(-30.7993181935265,-63.5768079214868,
12.));
#135062=CARTESIAN_POINT('Ctrl Pts',(-30.8136413077999,-63.5923861498963,
12.));
#135063=CARTESIAN_POINT('Ctrl Pts',(-30.8280141354448,-63.6079858892746,
12.));
#135064=CARTESIAN_POINT('Ctrl Pts',(-30.8424366246665,-63.6236069678041,
12.));
#135065=CARTESIAN_POINT('Ctrl Pts',(-30.8569087238132,-63.6392492145233,
12.));
#135066=CARTESIAN_POINT('Ctrl Pts',(-30.8714303814202,-63.6549124594681,
12.));
#135067=CARTESIAN_POINT('Ctrl Pts',(-30.8860015462488,-63.6705965337996,
12.));
#135068=CARTESIAN_POINT('Ctrl Pts',(-30.9006221672703,-63.6863012697353,
12.));
#135069=CARTESIAN_POINT('Ctrl Pts',(-30.9152921936471,-63.7020265004805,
12.));
#135070=CARTESIAN_POINT('Ctrl Pts',(-30.9300115747113,-63.7177720601604,
12.));
#135071=CARTESIAN_POINT('Ctrl Pts',(-30.9447802599345,-63.733537783742,
12.));
#135072=CARTESIAN_POINT('Ctrl Pts',(-30.9595981989091,-63.7493235069844,
12.));
#135073=CARTESIAN_POINT('Ctrl Pts',(-30.9744653413679,-63.7651290664713,
12.));
#135074=CARTESIAN_POINT('Ctrl Pts',(-30.9893816371907,-63.7809542996258,
12.));
#135075=CARTESIAN_POINT('Ctrl Pts',(-31.0043470364112,-63.7967990447287,
12.));
#135076=CARTESIAN_POINT('Ctrl Pts',(-31.0193614892177,-63.8126631409376,
12.));
#135077=CARTESIAN_POINT('Ctrl Pts',(-31.0344249459544,-63.8285464282857,
12.));
#135078=CARTESIAN_POINT('Ctrl Pts',(-31.0495373571218,-63.8444487476615,
12.));
#135079=CARTESIAN_POINT('Ctrl Pts',(-31.0646986733724,-63.8603699407922,
12.));
#135080=CARTESIAN_POINT('Ctrl Pts',(-31.079908845504,-63.8763098502235,
12.));
#135081=CARTESIAN_POINT('Ctrl Pts',(-31.0951678244454,-63.8922683192962,
12.));
#135082=CARTESIAN_POINT('Ctrl Pts',(-31.1104755612606,-63.9082451921447,
12.));
#135083=CARTESIAN_POINT('Ctrl Pts',(-31.1258320071545,-63.9242403136954,
12.));
#135084=CARTESIAN_POINT('Ctrl Pts',(-31.1412371134727,-63.940253529665,
12.));
#135085=CARTESIAN_POINT('Ctrl Pts',(-31.1566908316993,-63.9562846865566,
12.));
#135086=CARTESIAN_POINT('Ctrl Pts',(-31.1721931134488,-63.972333631655,
12.));
#135087=CARTESIAN_POINT('Ctrl Pts',(-31.1877439104717,-63.9884002130209,
12.));
#135088=CARTESIAN_POINT('Ctrl Pts',(-31.2033431746559,-64.004484279483,
12.));
#135089=CARTESIAN_POINT('Ctrl Pts',(-31.2189908580245,-64.0205856806298,
12.));
#135090=CARTESIAN_POINT('Ctrl Pts',(-31.23468691273,-64.036704266799,12.));
#135091=CARTESIAN_POINT('Ctrl Pts',(-31.2504312910457,-64.0528398890671,
12.));
#135092=CARTESIAN_POINT('Ctrl Pts',(-31.2662239453734,-64.0689923992474,
12.));
#135093=CARTESIAN_POINT('Ctrl Pts',(-31.2820648282451,-64.0851616498861,
12.));
#135094=CARTESIAN_POINT('Ctrl Pts',(-31.2979538923214,-64.1013474942554,
12.));
#135095=CARTESIAN_POINT('Ctrl Pts',(-31.3138910903852,-64.1175497863475,
12.));
#135096=CARTESIAN_POINT('Ctrl Pts',(-31.3298763753366,-64.1337683808667,
12.));
#135097=CARTESIAN_POINT('Ctrl Pts',(-31.3459097001996,-64.150003133226,
12.));
#135098=CARTESIAN_POINT('Ctrl Pts',(-31.3619910181223,-64.1662538995407,
12.));
#135099=CARTESIAN_POINT('Ctrl Pts',(-31.3781202823758,-64.1825205366231,
12.));
#135100=CARTESIAN_POINT('Ctrl Pts',(-31.3942974463458,-64.1988029019733,
12.));
#135101=CARTESIAN_POINT('Ctrl Pts',(-31.4105224635298,-64.2151008537733,
12.));
#135102=CARTESIAN_POINT('Ctrl Pts',(-31.426795287544,-64.2314142508843,
12.));
#135103=CARTESIAN_POINT('Ctrl Pts',(-31.443115872123,-64.2477429528408,
12.));
#135104=CARTESIAN_POINT('Ctrl Pts',(-31.4594841711189,-64.264086819846,
12.));
#135105=CARTESIAN_POINT('Ctrl Pts',(-31.4759001384923,-64.2804457127633,
12.));
#135106=CARTESIAN_POINT('Ctrl Pts',(-31.4923637283109,-64.2968194931113,
12.));
#135107=CARTESIAN_POINT('Ctrl Pts',(-31.5088748947565,-64.3132080230603,
12.));
#135108=CARTESIAN_POINT('Ctrl Pts',(-31.525433592124,-64.3296111654273,
12.));
#135109=CARTESIAN_POINT('Ctrl Pts',(-31.5420397748198,-64.34602878367,12.));
#135110=CARTESIAN_POINT('Ctrl Pts',(-31.5586933973532,-64.3624607418798,
12.));
#135111=CARTESIAN_POINT('Ctrl Pts',(-31.5753944143355,-64.3789069047768,
12.));
#135112=CARTESIAN_POINT('Ctrl Pts',(-31.5921427804879,-64.3953671377071,
12.));
#135113=CARTESIAN_POINT('Ctrl Pts',(-31.6089384506399,-64.4118413066386,
12.));
#135114=CARTESIAN_POINT('Ctrl Pts',(-31.6257813797282,-64.4283292781553,
12.));
#135115=CARTESIAN_POINT('Ctrl Pts',(-31.6426715227865,-64.4448309194498,
12.));
#135116=CARTESIAN_POINT('Ctrl Pts',(-31.6596088349468,-64.4613460983186,
12.));
#135117=CARTESIAN_POINT('Ctrl Pts',(-31.6765932714456,-64.4778746831597,
12.));
#135118=CARTESIAN_POINT('Ctrl Pts',(-31.6936247876228,-64.4944165429672,
12.));
#135119=CARTESIAN_POINT('Ctrl Pts',(-31.7107033389204,-64.5109715473276,
12.));
#135120=CARTESIAN_POINT('Ctrl Pts',(-31.7278288808736,-64.5275395664134,
12.));
#135121=CARTESIAN_POINT('Ctrl Pts',(-31.7450013691117,-64.5441204709779,
12.));
#135122=CARTESIAN_POINT('Ctrl Pts',(-31.7622207593637,-64.5607141323527,
12.));
#135123=CARTESIAN_POINT('Ctrl Pts',(-31.7794870074584,-64.5773204224429,
12.));
#135124=CARTESIAN_POINT('Ctrl Pts',(-31.7968000693218,-64.5939392137233,
12.));
#135125=CARTESIAN_POINT('Ctrl Pts',(-31.8141599009685,-64.6105703792311,
12.));
#135126=CARTESIAN_POINT('Ctrl Pts',(-31.8315664585027,-64.6272137925629,
12.));
#135127=CARTESIAN_POINT('Ctrl Pts',(-31.849019698125,-64.6438693278718,
12.));
#135128=CARTESIAN_POINT('Ctrl Pts',(-31.8665195761312,-64.6605368598631,
12.));
#135129=CARTESIAN_POINT('Ctrl Pts',(-31.8840660489106,-64.6772162637904,
12.));
#135130=CARTESIAN_POINT('Ctrl Pts',(-31.9016590729371,-64.693907415449,
12.));
#135131=CARTESIAN_POINT('Ctrl Pts',(-31.9192986047702,-64.7106101911722,
12.));
#135132=CARTESIAN_POINT('Ctrl Pts',(-31.9369846010613,-64.727324467829,
12.));
#135133=CARTESIAN_POINT('Ctrl Pts',(-31.9547170185533,-64.74405012282,12.));
#135134=CARTESIAN_POINT('Ctrl Pts',(-31.9724958140791,-64.7607870340738,
12.));
#135135=CARTESIAN_POINT('Ctrl Pts',(-31.9903209445522,-64.7775350800404,
12.));
#135136=CARTESIAN_POINT('Ctrl Pts',(-32.0081923669678,-64.7942941396883,
12.));
#135137=CARTESIAN_POINT('Ctrl Pts',(-32.0261100384092,-64.811064092502,
12.));
#135138=CARTESIAN_POINT('Ctrl Pts',(-32.0440739160477,-64.8278448184785,
12.));
#135139=CARTESIAN_POINT('Ctrl Pts',(-32.0620839571409,-64.8446361981234,
12.));
#135140=CARTESIAN_POINT('Ctrl Pts',(-32.0801401190244,-64.8614381124454,
12.));
#135141=CARTESIAN_POINT('Ctrl Pts',(-32.0982423591113,-64.8782504429527,
12.));
#135142=CARTESIAN_POINT('Ctrl Pts',(-32.1163906348984,-64.8950730716501,
12.));
#135143=CARTESIAN_POINT('Ctrl Pts',(-32.1345849039674,-64.9119058810366,
12.));
#135144=CARTESIAN_POINT('Ctrl Pts',(-32.1528251239831,-64.9287487541015,
12.));
#135145=CARTESIAN_POINT('Ctrl Pts',(-32.1711112526855,-64.9456015743192,
12.));
#135146=CARTESIAN_POINT('Ctrl Pts',(-32.1894432478881,-64.9624642256461,
12.));
#135147=CARTESIAN_POINT('Ctrl Pts',(-32.207821067485,-64.9793365925178,
12.));
#135148=CARTESIAN_POINT('Ctrl Pts',(-32.2262446694513,-64.9962185598461,
12.));
#135149=CARTESIAN_POINT('Ctrl Pts',(-32.2447140118422,-65.0131100130157,
12.));
#135150=CARTESIAN_POINT('Ctrl Pts',(-32.2632290527862,-65.03001083788,12.));
#135151=CARTESIAN_POINT('Ctrl Pts',(-32.2817897504807,-65.0469209207563,
12.));
#135152=CARTESIAN_POINT('Ctrl Pts',(-32.3003960632007,-65.0638401484257,
12.));
#135153=CARTESIAN_POINT('Ctrl Pts',(-32.3190479492987,-65.0807684081281,
12.));
#135154=CARTESIAN_POINT('Ctrl Pts',(-32.3377453672051,-65.0977055875607,
12.));
#135155=CARTESIAN_POINT('Ctrl Pts',(-32.3564882754212,-65.1146515748722,
12.));
#135156=CARTESIAN_POINT('Ctrl Pts',(-32.3752766325136,-65.1316062586588,
12.));
#135157=CARTESIAN_POINT('Ctrl Pts',(-32.3941103971221,-65.1485695279635,
12.));
#135158=CARTESIAN_POINT('Ctrl Pts',(-32.4129895279615,-65.1655412722725,
12.));
#135159=CARTESIAN_POINT('Ctrl Pts',(-32.4319139838213,-65.182521381514,
12.));
#135160=CARTESIAN_POINT('Ctrl Pts',(-32.450883723561,-65.1995097460538,
12.));
#135161=CARTESIAN_POINT('Ctrl Pts',(-32.4698987061032,-65.2165062566924,
12.));
#135162=CARTESIAN_POINT('Ctrl Pts',(-32.4889588904392,-65.2335108046614,
12.));
#135163=CARTESIAN_POINT('Ctrl Pts',(-32.5080642356328,-65.2505232816209,
12.));
#135164=CARTESIAN_POINT('Ctrl Pts',(-32.5272147008191,-65.2675435796558,
12.));
#135165=CARTESIAN_POINT('Ctrl Pts',(-32.5464102452015,-65.2845715912721,
12.));
#135166=CARTESIAN_POINT('Ctrl Pts',(-32.5656508280422,-65.3016072093912,
12.));
#135167=CARTESIAN_POINT('Ctrl Pts',(-32.5849364086679,-65.31865032735,12.));
#135168=CARTESIAN_POINT('Ctrl Pts',(-32.6042669464751,-65.3357008389003,
12.));
#135169=CARTESIAN_POINT('Ctrl Pts',(-32.6236424009301,-65.3527586382081,
12.));
#135170=CARTESIAN_POINT('Ctrl Pts',(-32.6430627315674,-65.3698236198512,
12.));
#135171=CARTESIAN_POINT('Ctrl Pts',(-32.6625278979811,-65.3868956788182,
12.));
#135172=CARTESIAN_POINT('Ctrl Pts',(-32.6820378598267,-65.4039747105038,
12.));
#135173=CARTESIAN_POINT('Ctrl Pts',(-32.7015925768265,-65.4210606107035,
12.));
#135174=CARTESIAN_POINT('Ctrl Pts',(-32.7211920087684,-65.4381532756065,
12.));
#135175=CARTESIAN_POINT('Ctrl Pts',(-32.7408361155037,-65.4552526017905,
12.));
#135176=CARTESIAN_POINT('Ctrl Pts',(-32.7605248569378,-65.4723584862122,
12.));
#135177=CARTESIAN_POINT('Ctrl Pts',(-32.7802581930287,-65.489470826206,
12.));
#135178=CARTESIAN_POINT('Ctrl Pts',(-32.8000360837975,-65.5065895194928,
12.));
#135179=CARTESIAN_POINT('Ctrl Pts',(-32.8198584893316,-65.5237144641857,
12.));
#135180=CARTESIAN_POINT('Ctrl Pts',(-32.8397253697866,-65.5408455587964,
12.));
#135181=CARTESIAN_POINT('Ctrl Pts',(-32.8596366853832,-65.5579827022421,
12.));
#135182=CARTESIAN_POINT('Ctrl Pts',(-32.879592396403,-65.5751257938472,
12.));
#135183=CARTESIAN_POINT('Ctrl Pts',(-32.8995924631898,-65.5922747333194,
12.));
#135184=CARTESIAN_POINT('Ctrl Pts',(-32.9196368461463,-65.6094294207276,
12.));
#135185=CARTESIAN_POINT('Ctrl Pts',(-32.9397255057274,-65.6265897564783,
12.));
#135186=CARTESIAN_POINT('Ctrl Pts',(-32.9598584024313,-65.6437556412946,
12.));
#135187=CARTESIAN_POINT('Ctrl Pts',(-32.980035496784,-65.6609269761888,
12.));
#135188=CARTESIAN_POINT('Ctrl Pts',(-33.0002567493574,-65.6781036625027,
12.));
#135189=CARTESIAN_POINT('Ctrl Pts',(-33.0205221207873,-65.6952856019533,
12.));
#135190=CARTESIAN_POINT('Ctrl Pts',(-33.0408315717873,-65.7124726966802,
12.));
#135191=CARTESIAN_POINT('Ctrl Pts',(-33.0611850631582,-65.7296648492824,
12.));
#135192=CARTESIAN_POINT('Ctrl Pts',(-33.081582555798,-65.7468619628815,
12.));
#135193=CARTESIAN_POINT('Ctrl Pts',(-33.1020240106885,-65.7640639410661,
12.));
#135194=CARTESIAN_POINT('Ctrl Pts',(-33.1225093888672,-65.7812706877696,
12.));
#135195=CARTESIAN_POINT('Ctrl Pts',(-33.1430386513976,-65.7984821071623,
12.));
#135196=CARTESIAN_POINT('Ctrl Pts',(-33.16361175934,-65.8156981035503,12.));
#135197=CARTESIAN_POINT('Ctrl Pts',(-33.1842286737051,-65.8329185812375,
12.));
#135198=CARTESIAN_POINT('Ctrl Pts',(-33.2048893554491,-65.8501434445164,
12.));
#135199=CARTESIAN_POINT('Ctrl Pts',(-33.2255937655649,-65.8673725979577,
12.));
#135200=CARTESIAN_POINT('Ctrl Pts',(-33.2463418651493,-65.8846059466371,
12.));
#135201=CARTESIAN_POINT('Ctrl Pts',(-33.2671336154754,-65.9018433963889,
12.));
#135202=CARTESIAN_POINT('Ctrl Pts',(-33.2879689780573,-65.9190848540433,
12.));
#135203=CARTESIAN_POINT('Ctrl Pts',(-33.3088479147164,-65.9363302276846,
12.));
#135204=CARTESIAN_POINT('Ctrl Pts',(-33.3297703874266,-65.9535794260831,
12.));
#135205=CARTESIAN_POINT('Ctrl Pts',(-33.3507363581593,-65.970832358141,
12.));
#135206=CARTESIAN_POINT('Ctrl Pts',(-33.37174578871,-65.9880889322831,12.));
#135207=CARTESIAN_POINT('Ctrl Pts',(-33.3927986405605,-66.0053490559812,
12.));
#135208=CARTESIAN_POINT('Ctrl Pts',(-33.4138948746388,-66.0226126349446,
12.));
#135209=CARTESIAN_POINT('Ctrl Pts',(-33.4350344515101,-66.0398795737777,
12.));
#135210=CARTESIAN_POINT('Ctrl Pts',(-33.4562173318025,-66.0571497774434,
12.));
#135211=CARTESIAN_POINT('Ctrl Pts',(-33.4774434765746,-66.0744231525415,
12.));
#135212=CARTESIAN_POINT('Ctrl Pts',(-33.4987128476622,-66.0916996085244,
12.));
#135213=CARTESIAN_POINT('Ctrl Pts',(-33.5200254081243,-66.1089790592729,
12.));
#135214=CARTESIAN_POINT('Ctrl Pts',(-33.5413811223451,-66.1262614234674,
12.));
#135215=CARTESIAN_POINT('Ctrl Pts',(-33.5597240685846,-66.1410781873278,
12.));
#135216=CARTESIAN_POINT('Ctrl Pts',(-33.5738105077875,-66.1524393974174,
12.));
#135217=CARTESIAN_POINT('Ctrl Pts',(-33.5836213514189,-66.1603438177522,
12.));
#135218=CARTESIAN_POINT('Ctrl Pts',(-33.5891439876494,-66.1647906582657,
12.));
#135219=CARTESIAN_POINT('Ctrl Pts',(-33.590372266528,-66.1657795405962,
12.));
#135220=CARTESIAN_POINT('',(-30.3549065457811,-63.0759831361898,0.));
#135221=CARTESIAN_POINT('',(-30.3549065457811,-63.0759831361898,0.));
#135222=CARTESIAN_POINT('Ctrl Pts',(-33.590372266528,-66.1657795405962,
0.));
#135223=CARTESIAN_POINT('Ctrl Pts',(-33.5891439876494,-66.1647906582657,
0.));
#135224=CARTESIAN_POINT('Ctrl Pts',(-33.5836213514189,-66.1603438177522,
0.));
#135225=CARTESIAN_POINT('Ctrl Pts',(-33.5738105077875,-66.1524393974174,
0.));
#135226=CARTESIAN_POINT('Ctrl Pts',(-33.5597240685846,-66.1410781873278,
0.));
#135227=CARTESIAN_POINT('Ctrl Pts',(-33.5413811223451,-66.1262614234674,
0.));
#135228=CARTESIAN_POINT('Ctrl Pts',(-33.5200254081243,-66.1089790592729,
0.));
#135229=CARTESIAN_POINT('Ctrl Pts',(-33.4987128476622,-66.0916996085244,
0.));
#135230=CARTESIAN_POINT('Ctrl Pts',(-33.4774434765746,-66.0744231525415,
0.));
#135231=CARTESIAN_POINT('Ctrl Pts',(-33.4562173318025,-66.0571497774434,
0.));
#135232=CARTESIAN_POINT('Ctrl Pts',(-33.4350344515101,-66.0398795737777,
0.));
#135233=CARTESIAN_POINT('Ctrl Pts',(-33.4138948746388,-66.0226126349446,
0.));
#135234=CARTESIAN_POINT('Ctrl Pts',(-33.3927986405605,-66.0053490559812,
0.));
#135235=CARTESIAN_POINT('Ctrl Pts',(-33.37174578871,-65.9880889322831,0.));
#135236=CARTESIAN_POINT('Ctrl Pts',(-33.3507363581593,-65.970832358141,
0.));
#135237=CARTESIAN_POINT('Ctrl Pts',(-33.3297703874266,-65.9535794260831,
0.));
#135238=CARTESIAN_POINT('Ctrl Pts',(-33.3088479147164,-65.9363302276846,
0.));
#135239=CARTESIAN_POINT('Ctrl Pts',(-33.2879689780573,-65.9190848540433,
0.));
#135240=CARTESIAN_POINT('Ctrl Pts',(-33.2671336154754,-65.9018433963889,
0.));
#135241=CARTESIAN_POINT('Ctrl Pts',(-33.2463418651493,-65.8846059466371,
0.));
#135242=CARTESIAN_POINT('Ctrl Pts',(-33.2255937655649,-65.8673725979577,
0.));
#135243=CARTESIAN_POINT('Ctrl Pts',(-33.2048893554491,-65.8501434445164,
0.));
#135244=CARTESIAN_POINT('Ctrl Pts',(-33.1842286737051,-65.8329185812375,
0.));
#135245=CARTESIAN_POINT('Ctrl Pts',(-33.16361175934,-65.8156981035503,0.));
#135246=CARTESIAN_POINT('Ctrl Pts',(-33.1430386513976,-65.7984821071623,
0.));
#135247=CARTESIAN_POINT('Ctrl Pts',(-33.1225093888672,-65.7812706877696,
0.));
#135248=CARTESIAN_POINT('Ctrl Pts',(-33.1020240106885,-65.7640639410661,
0.));
#135249=CARTESIAN_POINT('Ctrl Pts',(-33.081582555798,-65.7468619628815,
0.));
#135250=CARTESIAN_POINT('Ctrl Pts',(-33.0611850631582,-65.7296648492824,
0.));
#135251=CARTESIAN_POINT('Ctrl Pts',(-33.0408315717873,-65.7124726966802,
0.));
#135252=CARTESIAN_POINT('Ctrl Pts',(-33.0205221207873,-65.6952856019533,
0.));
#135253=CARTESIAN_POINT('Ctrl Pts',(-33.0002567493574,-65.6781036625027,
0.));
#135254=CARTESIAN_POINT('Ctrl Pts',(-32.980035496784,-65.6609269761888,
0.));
#135255=CARTESIAN_POINT('Ctrl Pts',(-32.9598584024313,-65.6437556412946,
0.));
#135256=CARTESIAN_POINT('Ctrl Pts',(-32.9397255057274,-65.6265897564783,
0.));
#135257=CARTESIAN_POINT('Ctrl Pts',(-32.9196368461463,-65.6094294207276,
0.));
#135258=CARTESIAN_POINT('Ctrl Pts',(-32.8995924631898,-65.5922747333194,
0.));
#135259=CARTESIAN_POINT('Ctrl Pts',(-32.879592396403,-65.5751257938472,
0.));
#135260=CARTESIAN_POINT('Ctrl Pts',(-32.8596366853832,-65.5579827022421,
0.));
#135261=CARTESIAN_POINT('Ctrl Pts',(-32.8397253697866,-65.5408455587964,
0.));
#135262=CARTESIAN_POINT('Ctrl Pts',(-32.8198584893316,-65.5237144641857,
0.));
#135263=CARTESIAN_POINT('Ctrl Pts',(-32.8000360837975,-65.5065895194928,
0.));
#135264=CARTESIAN_POINT('Ctrl Pts',(-32.7802581930287,-65.489470826206,
0.));
#135265=CARTESIAN_POINT('Ctrl Pts',(-32.7605248569378,-65.4723584862122,
0.));
#135266=CARTESIAN_POINT('Ctrl Pts',(-32.7408361155037,-65.4552526017905,
0.));
#135267=CARTESIAN_POINT('Ctrl Pts',(-32.7211920087684,-65.4381532756065,
0.));
#135268=CARTESIAN_POINT('Ctrl Pts',(-32.7015925768265,-65.4210606107035,
0.));
#135269=CARTESIAN_POINT('Ctrl Pts',(-32.6820378598267,-65.4039747105038,
0.));
#135270=CARTESIAN_POINT('Ctrl Pts',(-32.6625278979811,-65.3868956788182,
0.));
#135271=CARTESIAN_POINT('Ctrl Pts',(-32.6430627315674,-65.3698236198512,
0.));
#135272=CARTESIAN_POINT('Ctrl Pts',(-32.6236424009301,-65.3527586382081,
0.));
#135273=CARTESIAN_POINT('Ctrl Pts',(-32.6042669464751,-65.3357008389003,
0.));
#135274=CARTESIAN_POINT('Ctrl Pts',(-32.5849364086679,-65.31865032735,0.));
#135275=CARTESIAN_POINT('Ctrl Pts',(-32.5656508280422,-65.3016072093912,
0.));
#135276=CARTESIAN_POINT('Ctrl Pts',(-32.5464102452015,-65.2845715912721,
0.));
#135277=CARTESIAN_POINT('Ctrl Pts',(-32.5272147008191,-65.2675435796558,
0.));
#135278=CARTESIAN_POINT('Ctrl Pts',(-32.5080642356328,-65.2505232816209,
0.));
#135279=CARTESIAN_POINT('Ctrl Pts',(-32.4889588904392,-65.2335108046614,
0.));
#135280=CARTESIAN_POINT('Ctrl Pts',(-32.4698987061032,-65.2165062566924,
0.));
#135281=CARTESIAN_POINT('Ctrl Pts',(-32.450883723561,-65.1995097460538,
0.));
#135282=CARTESIAN_POINT('Ctrl Pts',(-32.4319139838213,-65.182521381514,
0.));
#135283=CARTESIAN_POINT('Ctrl Pts',(-32.4129895279615,-65.1655412722725,
0.));
#135284=CARTESIAN_POINT('Ctrl Pts',(-32.3941103971221,-65.1485695279635,
0.));
#135285=CARTESIAN_POINT('Ctrl Pts',(-32.3752766325136,-65.1316062586588,
0.));
#135286=CARTESIAN_POINT('Ctrl Pts',(-32.3564882754212,-65.1146515748722,
0.));
#135287=CARTESIAN_POINT('Ctrl Pts',(-32.3377453672051,-65.0977055875607,
0.));
#135288=CARTESIAN_POINT('Ctrl Pts',(-32.3190479492987,-65.0807684081281,
0.));
#135289=CARTESIAN_POINT('Ctrl Pts',(-32.3003960632007,-65.0638401484257,
0.));
#135290=CARTESIAN_POINT('Ctrl Pts',(-32.2817897504807,-65.0469209207563,
0.));
#135291=CARTESIAN_POINT('Ctrl Pts',(-32.2632290527862,-65.03001083788,0.));
#135292=CARTESIAN_POINT('Ctrl Pts',(-32.2447140118422,-65.0131100130157,
0.));
#135293=CARTESIAN_POINT('Ctrl Pts',(-32.2262446694513,-64.9962185598461,
0.));
#135294=CARTESIAN_POINT('Ctrl Pts',(-32.207821067485,-64.9793365925178,
0.));
#135295=CARTESIAN_POINT('Ctrl Pts',(-32.1894432478881,-64.9624642256461,
0.));
#135296=CARTESIAN_POINT('Ctrl Pts',(-32.1711112526855,-64.9456015743192,
0.));
#135297=CARTESIAN_POINT('Ctrl Pts',(-32.1528251239831,-64.9287487541015,
0.));
#135298=CARTESIAN_POINT('Ctrl Pts',(-32.1345849039674,-64.9119058810366,
0.));
#135299=CARTESIAN_POINT('Ctrl Pts',(-32.1163906348984,-64.8950730716501,
0.));
#135300=CARTESIAN_POINT('Ctrl Pts',(-32.0982423591113,-64.8782504429527,
0.));
#135301=CARTESIAN_POINT('Ctrl Pts',(-32.0801401190244,-64.8614381124454,
0.));
#135302=CARTESIAN_POINT('Ctrl Pts',(-32.0620839571409,-64.8446361981234,
0.));
#135303=CARTESIAN_POINT('Ctrl Pts',(-32.0440739160477,-64.8278448184785,
0.));
#135304=CARTESIAN_POINT('Ctrl Pts',(-32.0261100384092,-64.811064092502,
0.));
#135305=CARTESIAN_POINT('Ctrl Pts',(-32.0081923669678,-64.7942941396883,
0.));
#135306=CARTESIAN_POINT('Ctrl Pts',(-31.9903209445522,-64.7775350800404,
0.));
#135307=CARTESIAN_POINT('Ctrl Pts',(-31.9724958140791,-64.7607870340738,
0.));
#135308=CARTESIAN_POINT('Ctrl Pts',(-31.9547170185533,-64.74405012282,0.));
#135309=CARTESIAN_POINT('Ctrl Pts',(-31.9369846010613,-64.727324467829,
0.));
#135310=CARTESIAN_POINT('Ctrl Pts',(-31.9192986047702,-64.7106101911722,
0.));
#135311=CARTESIAN_POINT('Ctrl Pts',(-31.9016590729371,-64.693907415449,
0.));
#135312=CARTESIAN_POINT('Ctrl Pts',(-31.8840660489106,-64.6772162637904,
0.));
#135313=CARTESIAN_POINT('Ctrl Pts',(-31.8665195761312,-64.6605368598631,
0.));
#135314=CARTESIAN_POINT('Ctrl Pts',(-31.849019698125,-64.6438693278718,
0.));
#135315=CARTESIAN_POINT('Ctrl Pts',(-31.8315664585027,-64.6272137925629,
0.));
#135316=CARTESIAN_POINT('Ctrl Pts',(-31.8141599009685,-64.6105703792311,
0.));
#135317=CARTESIAN_POINT('Ctrl Pts',(-31.7968000693218,-64.5939392137233,
0.));
#135318=CARTESIAN_POINT('Ctrl Pts',(-31.7794870074584,-64.5773204224429,
0.));
#135319=CARTESIAN_POINT('Ctrl Pts',(-31.7622207593637,-64.5607141323527,
0.));
#135320=CARTESIAN_POINT('Ctrl Pts',(-31.7450013691117,-64.5441204709779,
0.));
#135321=CARTESIAN_POINT('Ctrl Pts',(-31.7278288808736,-64.5275395664134,
0.));
#135322=CARTESIAN_POINT('Ctrl Pts',(-31.7107033389204,-64.5109715473276,
0.));
#135323=CARTESIAN_POINT('Ctrl Pts',(-31.6936247876228,-64.4944165429672,
0.));
#135324=CARTESIAN_POINT('Ctrl Pts',(-31.6765932714456,-64.4778746831597,
0.));
#135325=CARTESIAN_POINT('Ctrl Pts',(-31.6596088349468,-64.4613460983186,
0.));
#135326=CARTESIAN_POINT('Ctrl Pts',(-31.6426715227865,-64.4448309194498,
0.));
#135327=CARTESIAN_POINT('Ctrl Pts',(-31.6257813797282,-64.4283292781553,
0.));
#135328=CARTESIAN_POINT('Ctrl Pts',(-31.6089384506399,-64.4118413066386,
0.));
#135329=CARTESIAN_POINT('Ctrl Pts',(-31.5921427804879,-64.3953671377071,
0.));
#135330=CARTESIAN_POINT('Ctrl Pts',(-31.5753944143355,-64.3789069047768,
0.));
#135331=CARTESIAN_POINT('Ctrl Pts',(-31.5586933973532,-64.3624607418798,
0.));
#135332=CARTESIAN_POINT('Ctrl Pts',(-31.5420397748198,-64.34602878367,0.));
#135333=CARTESIAN_POINT('Ctrl Pts',(-31.525433592124,-64.3296111654273,
0.));
#135334=CARTESIAN_POINT('Ctrl Pts',(-31.5088748947565,-64.3132080230603,
0.));
#135335=CARTESIAN_POINT('Ctrl Pts',(-31.4923637283109,-64.2968194931113,
0.));
#135336=CARTESIAN_POINT('Ctrl Pts',(-31.4759001384923,-64.2804457127633,
0.));
#135337=CARTESIAN_POINT('Ctrl Pts',(-31.4594841711189,-64.264086819846,
0.));
#135338=CARTESIAN_POINT('Ctrl Pts',(-31.443115872123,-64.2477429528408,
0.));
#135339=CARTESIAN_POINT('Ctrl Pts',(-31.426795287544,-64.2314142508843,
0.));
#135340=CARTESIAN_POINT('Ctrl Pts',(-31.4105224635298,-64.2151008537733,
0.));
#135341=CARTESIAN_POINT('Ctrl Pts',(-31.3942974463458,-64.1988029019733,
0.));
#135342=CARTESIAN_POINT('Ctrl Pts',(-31.3781202823758,-64.1825205366231,
0.));
#135343=CARTESIAN_POINT('Ctrl Pts',(-31.3619910181223,-64.1662538995407,
0.));
#135344=CARTESIAN_POINT('Ctrl Pts',(-31.3459097001996,-64.150003133226,
0.));
#135345=CARTESIAN_POINT('Ctrl Pts',(-31.3298763753366,-64.1337683808667,
0.));
#135346=CARTESIAN_POINT('Ctrl Pts',(-31.3138910903852,-64.1175497863475,
0.));
#135347=CARTESIAN_POINT('Ctrl Pts',(-31.2979538923214,-64.1013474942554,
0.));
#135348=CARTESIAN_POINT('Ctrl Pts',(-31.2820648282451,-64.0851616498861,
0.));
#135349=CARTESIAN_POINT('Ctrl Pts',(-31.2662239453734,-64.0689923992474,
0.));
#135350=CARTESIAN_POINT('Ctrl Pts',(-31.2504312910457,-64.0528398890671,
0.));
#135351=CARTESIAN_POINT('Ctrl Pts',(-31.23468691273,-64.036704266799,0.));
#135352=CARTESIAN_POINT('Ctrl Pts',(-31.2189908580245,-64.0205856806298,
0.));
#135353=CARTESIAN_POINT('Ctrl Pts',(-31.2033431746559,-64.004484279483,
0.));
#135354=CARTESIAN_POINT('Ctrl Pts',(-31.1877439104717,-63.9884002130209,
0.));
#135355=CARTESIAN_POINT('Ctrl Pts',(-31.1721931134488,-63.972333631655,
0.));
#135356=CARTESIAN_POINT('Ctrl Pts',(-31.1566908316993,-63.9562846865566,
0.));
#135357=CARTESIAN_POINT('Ctrl Pts',(-31.1412371134727,-63.940253529665,
0.));
#135358=CARTESIAN_POINT('Ctrl Pts',(-31.1258320071545,-63.9242403136954,
0.));
#135359=CARTESIAN_POINT('Ctrl Pts',(-31.1104755612606,-63.9082451921447,
0.));
#135360=CARTESIAN_POINT('Ctrl Pts',(-31.0951678244454,-63.8922683192962,
0.));
#135361=CARTESIAN_POINT('Ctrl Pts',(-31.079908845504,-63.8763098502235,
0.));
#135362=CARTESIAN_POINT('Ctrl Pts',(-31.0646986733724,-63.8603699407922,
0.));
#135363=CARTESIAN_POINT('Ctrl Pts',(-31.0495373571218,-63.8444487476615,
0.));
#135364=CARTESIAN_POINT('Ctrl Pts',(-31.0344249459544,-63.8285464282857,
0.));
#135365=CARTESIAN_POINT('Ctrl Pts',(-31.0193614892177,-63.8126631409376,
0.));
#135366=CARTESIAN_POINT('Ctrl Pts',(-31.0043470364112,-63.7967990447287,
0.));
#135367=CARTESIAN_POINT('Ctrl Pts',(-30.9893816371907,-63.7809542996258,
0.));
#135368=CARTESIAN_POINT('Ctrl Pts',(-30.9744653413679,-63.7651290664713,
0.));
#135369=CARTESIAN_POINT('Ctrl Pts',(-30.9595981989091,-63.7493235069844,
0.));
#135370=CARTESIAN_POINT('Ctrl Pts',(-30.9447802599345,-63.733537783742,
0.));
#135371=CARTESIAN_POINT('Ctrl Pts',(-30.9300115747113,-63.7177720601604,
0.));
#135372=CARTESIAN_POINT('Ctrl Pts',(-30.9152921936471,-63.7020265004805,
0.));
#135373=CARTESIAN_POINT('Ctrl Pts',(-30.9006221672703,-63.6863012697353,
0.));
#135374=CARTESIAN_POINT('Ctrl Pts',(-30.8860015462488,-63.6705965337996,
0.));
#135375=CARTESIAN_POINT('Ctrl Pts',(-30.8714303814202,-63.6549124594681,
0.));
#135376=CARTESIAN_POINT('Ctrl Pts',(-30.8569087238132,-63.6392492145233,
0.));
#135377=CARTESIAN_POINT('Ctrl Pts',(-30.8424366246665,-63.6236069678041,
0.));
#135378=CARTESIAN_POINT('Ctrl Pts',(-30.8280141354448,-63.6079858892746,
0.));
#135379=CARTESIAN_POINT('Ctrl Pts',(-30.8136413077999,-63.5923861498963,
0.));
#135380=CARTESIAN_POINT('Ctrl Pts',(-30.7993181935265,-63.5768079214868,
0.));
#135381=CARTESIAN_POINT('Ctrl Pts',(-30.7850448445207,-63.5612513766005,
0.));
#135382=CARTESIAN_POINT('Ctrl Pts',(-30.7708213127169,-63.5457166883558,
0.));
#135383=CARTESIAN_POINT('Ctrl Pts',(-30.7566476500772,-63.5302040304173,
0.));
#135384=CARTESIAN_POINT('Ctrl Pts',(-30.7425239087294,-63.514713577392,
0.));
#135385=CARTESIAN_POINT('Ctrl Pts',(-30.7284501410827,-63.4992455051805,
0.));
#135386=CARTESIAN_POINT('Ctrl Pts',(-30.7144263999259,-63.4837999912758,
0.));
#135387=CARTESIAN_POINT('Ctrl Pts',(-30.7004527385806,-63.4683772152497,
0.));
#135388=CARTESIAN_POINT('Ctrl Pts',(-30.6865292107911,-63.452977358421,
0.));
#135389=CARTESIAN_POINT('Ctrl Pts',(-30.6726558704302,-63.4376006029575,
0.));
#135390=CARTESIAN_POINT('Ctrl Pts',(-30.6588327712482,-63.4222471311236,
0.));
#135391=CARTESIAN_POINT('Ctrl Pts',(-30.6450599666135,-63.4069171245093,
0.));
#135392=CARTESIAN_POINT('Ctrl Pts',(-30.6313375092085,-63.3916107631421,
0.));
#135393=CARTESIAN_POINT('Ctrl Pts',(-30.6176654515988,-63.3763282271838,
0.));
#135394=CARTESIAN_POINT('Ctrl Pts',(-30.604043846909,-63.3610696989599,
0.));
#135395=CARTESIAN_POINT('Ctrl Pts',(-30.5904727493707,-63.3458353646144,
0.));
#135396=CARTESIAN_POINT('Ctrl Pts',(-30.5769522151147,-63.330625416509,
0.));
#135397=CARTESIAN_POINT('Ctrl Pts',(-30.5634823022358,-63.315440053435,
0.));
#135398=CARTESIAN_POINT('Ctrl Pts',(-30.5500630691343,-63.3002794756049,
0.));
#135399=CARTESIAN_POINT('Ctrl Pts',(-30.5366945730503,-63.2851438802462,
0.));
#135400=CARTESIAN_POINT('Ctrl Pts',(-30.5233768687875,-63.2700334577661,
0.));
#135401=CARTESIAN_POINT('Ctrl Pts',(-30.5101100066683,-63.2549483856268,
0.));
#135402=CARTESIAN_POINT('Ctrl Pts',(-30.4968940345028,-63.2398888342612,
0.));
#135403=CARTESIAN_POINT('Ctrl Pts',(-30.4837290015011,-63.2248549788272,
0.));
#135404=CARTESIAN_POINT('Ctrl Pts',(-30.470614961416,-63.2098470086636,
0.));
#135405=CARTESIAN_POINT('Ctrl Pts',(-30.4575519763305,-63.1948651386868,
0.));
#135406=CARTESIAN_POINT('Ctrl Pts',(-30.4445401192324,-63.1799096171757,
0.));
#135407=CARTESIAN_POINT('Ctrl Pts',(-30.431579465967,-63.1649807016766,
0.));
#135408=CARTESIAN_POINT('Ctrl Pts',(-30.4186700875598,-63.1500786361382,
0.));
#135409=CARTESIAN_POINT('Ctrl Pts',(-30.4058120432259,-63.1352036298512,
0.));
#135410=CARTESIAN_POINT('Ctrl Pts',(-30.3930053710592,-63.1203558300911,
0.));
#135411=CARTESIAN_POINT('Ctrl Pts',(-30.3802500880565,-63.1055353202641,
0.));
#135412=CARTESIAN_POINT('Ctrl Pts',(-30.3700869762658,-63.0937007763826,
0.));
#135413=CARTESIAN_POINT('Ctrl Pts',(-30.3624877680747,-63.0848371718274,
0.));
#135414=CARTESIAN_POINT('Ctrl Pts',(-30.3574319069366,-63.0789335700774,
0.));
#135415=CARTESIAN_POINT('Ctrl Pts',(-30.3549065457811,-63.0759831361898,
0.));
#135416=CARTESIAN_POINT('Ctrl Pts',(-39.5004851439258,-63.1661434108059,
0.));
#135417=CARTESIAN_POINT('Ctrl Pts',(-39.5004851439258,-63.1661434108059,
12.));
#135418=CARTESIAN_POINT('Ctrl Pts',(-39.4958045828135,-63.1630766582787,
0.));
#135419=CARTESIAN_POINT('Ctrl Pts',(-39.4958045828135,-63.1630766582787,
12.));
#135420=CARTESIAN_POINT('Ctrl Pts',(-39.4864477303823,-63.1569429707875,
0.));
#135421=CARTESIAN_POINT('Ctrl Pts',(-39.4864477303823,-63.1569429707875,
12.));
#135422=CARTESIAN_POINT('Ctrl Pts',(-39.4724252611155,-63.1477418922405,
0.));
#135423=CARTESIAN_POINT('Ctrl Pts',(-39.4724252611155,-63.1477418922405,
12.));
#135424=CARTESIAN_POINT('Ctrl Pts',(-39.4537542552268,-63.1354726928398,
0.));
#135425=CARTESIAN_POINT('Ctrl Pts',(-39.4537542552268,-63.1354726928398,
12.));
#135426=CARTESIAN_POINT('Ctrl Pts',(-39.4304582059864,-63.1201343731172,
0.));
#135427=CARTESIAN_POINT('Ctrl Pts',(-39.4304582059864,-63.1201343731172,
12.));
#135428=CARTESIAN_POINT('Ctrl Pts',(-39.4072048797616,-63.10479424519,0.));
#135429=CARTESIAN_POINT('Ctrl Pts',(-39.4072048797616,-63.10479424519,12.));
#135430=CARTESIAN_POINT('Ctrl Pts',(-39.383994298574,-63.0894523341314,
0.));
#135431=CARTESIAN_POINT('Ctrl Pts',(-39.383994298574,-63.0894523341314,
12.));
#135432=CARTESIAN_POINT('Ctrl Pts',(-39.3608264920409,-63.0741086815841,
0.));
#135433=CARTESIAN_POINT('Ctrl Pts',(-39.3608264920409,-63.0741086815841,
12.));
#135434=CARTESIAN_POINT('Ctrl Pts',(-39.3377014983609,-63.0587633513774,
0.));
#135435=CARTESIAN_POINT('Ctrl Pts',(-39.3377014983609,-63.0587633513774,
12.));
#135436=CARTESIAN_POINT('Ctrl Pts',(-39.3146193632392,-63.0434164277992,
0.));
#135437=CARTESIAN_POINT('Ctrl Pts',(-39.3146193632392,-63.0434164277992,
12.));
#135438=CARTESIAN_POINT('Ctrl Pts',(-39.2915801372354,-63.0280680082352,
0.));
#135439=CARTESIAN_POINT('Ctrl Pts',(-39.2915801372354,-63.0280680082352,
12.));
#135440=CARTESIAN_POINT('Ctrl Pts',(-39.2685838735361,-63.0127181973628,
0.));
#135441=CARTESIAN_POINT('Ctrl Pts',(-39.2685838735361,-63.0127181973628,
12.));
#135442=CARTESIAN_POINT('Ctrl Pts',(-39.2456306256104,-62.9973671008703,
0.));
#135443=CARTESIAN_POINT('Ctrl Pts',(-39.2456306256104,-62.9973671008703,
12.));
#135444=CARTESIAN_POINT('Ctrl Pts',(-39.2227204447638,-62.9820148189929,
0.));
#135445=CARTESIAN_POINT('Ctrl Pts',(-39.2227204447638,-62.9820148189929,
12.));
#135446=CARTESIAN_POINT('Ctrl Pts',(-39.1998533781661,-62.9666614412731,
0.));
#135447=CARTESIAN_POINT('Ctrl Pts',(-39.1998533781661,-62.9666614412731,
12.));
#135448=CARTESIAN_POINT('Ctrl Pts',(-39.1770294702428,-62.9513070501867,
0.));
#135449=CARTESIAN_POINT('Ctrl Pts',(-39.1770294702428,-62.9513070501867,
12.));
#135450=CARTESIAN_POINT('Ctrl Pts',(-39.1542487636744,-62.9359517237404,
0.));
#135451=CARTESIAN_POINT('Ctrl Pts',(-39.1542487636744,-62.9359517237404,
12.));
#135452=CARTESIAN_POINT('Ctrl Pts',(-39.131511300575,-62.9205955385558,
0.));
#135453=CARTESIAN_POINT('Ctrl Pts',(-39.131511300575,-62.9205955385558,
12.));
#135454=CARTESIAN_POINT('Ctrl Pts',(-39.1088171235125,-62.9052385725387,
0.));
#135455=CARTESIAN_POINT('Ctrl Pts',(-39.1088171235125,-62.9052385725387,
12.));
#135456=CARTESIAN_POINT('Ctrl Pts',(-39.0861662767932,-62.8898809082611,
0.));
#135457=CARTESIAN_POINT('Ctrl Pts',(-39.0861662767932,-62.8898809082611,
12.));
#135458=CARTESIAN_POINT('Ctrl Pts',(-39.0635588063277,-62.8745226325998,
0.));
#135459=CARTESIAN_POINT('Ctrl Pts',(-39.0635588063277,-62.8745226325998,
12.));
#135460=CARTESIAN_POINT('Ctrl Pts',(-39.0409947590497,-62.8591638352055,
0.));
#135461=CARTESIAN_POINT('Ctrl Pts',(-39.0409947590497,-62.8591638352055,
12.));
#135462=CARTESIAN_POINT('Ctrl Pts',(-39.0184741824641,-62.8438046073224,
0.));
#135463=CARTESIAN_POINT('Ctrl Pts',(-39.0184741824641,-62.8438046073224,
12.));
#135464=CARTESIAN_POINT('Ctrl Pts',(-38.9959971241701,-62.8284450405459,
0.));
#135465=CARTESIAN_POINT('Ctrl Pts',(-38.9959971241701,-62.8284450405459,
12.));
#135466=CARTESIAN_POINT('Ctrl Pts',(-38.9735636313089,-62.8130852254027,
0.));
#135467=CARTESIAN_POINT('Ctrl Pts',(-38.9735636313089,-62.8130852254027,
12.));
#135468=CARTESIAN_POINT('Ctrl Pts',(-38.9511737503165,-62.7977252507117,
0.));
#135469=CARTESIAN_POINT('Ctrl Pts',(-38.9511737503165,-62.7977252507117,
12.));
#135470=CARTESIAN_POINT('Ctrl Pts',(-38.9288275272335,-62.78236520437,0.));
#135471=CARTESIAN_POINT('Ctrl Pts',(-38.9288275272335,-62.78236520437,12.));
#135472=CARTESIAN_POINT('Ctrl Pts',(-38.9065250078832,-62.7670051738143,
0.));
#135473=CARTESIAN_POINT('Ctrl Pts',(-38.9065250078832,-62.7670051738143,
12.));
#135474=CARTESIAN_POINT('Ctrl Pts',(-38.8842662380984,-62.7516452466128,
0.));
#135475=CARTESIAN_POINT('Ctrl Pts',(-38.8842662380984,-62.7516452466128,
12.));
#135476=CARTESIAN_POINT('Ctrl Pts',(-38.8620512639233,-62.7362855110042,
0.));
#135477=CARTESIAN_POINT('Ctrl Pts',(-38.8620512639233,-62.7362855110042,
12.));
#135478=CARTESIAN_POINT('Ctrl Pts',(-38.8398801318177,-62.7209260564493,
0.));
#135479=CARTESIAN_POINT('Ctrl Pts',(-38.8398801318177,-62.7209260564493,
12.));
#135480=CARTESIAN_POINT('Ctrl Pts',(-38.8177528885681,-62.7055669733802,
0.));
#135481=CARTESIAN_POINT('Ctrl Pts',(-38.8177528885681,-62.7055669733802,
12.));
#135482=CARTESIAN_POINT('Ctrl Pts',(-38.795669581203,-62.6902083529694,
0.));
#135483=CARTESIAN_POINT('Ctrl Pts',(-38.795669581203,-62.6902083529694,
12.));
#135484=CARTESIAN_POINT('Ctrl Pts',(-38.7736302568982,-62.6748502868835,
0.));
#135485=CARTESIAN_POINT('Ctrl Pts',(-38.7736302568982,-62.6748502868835,
12.));
#135486=CARTESIAN_POINT('Ctrl Pts',(-38.7516349628904,-62.6594928670628,
0.));
#135487=CARTESIAN_POINT('Ctrl Pts',(-38.7516349628904,-62.6594928670628,
12.));
#135488=CARTESIAN_POINT('Ctrl Pts',(-38.7296837463609,-62.6441361854411,
0.));
#135489=CARTESIAN_POINT('Ctrl Pts',(-38.7296837463609,-62.6441361854411,
12.));
#135490=CARTESIAN_POINT('Ctrl Pts',(-38.7077766544416,-62.6287803339542,
0.));
#135491=CARTESIAN_POINT('Ctrl Pts',(-38.7077766544416,-62.6287803339542,
12.));
#135492=CARTESIAN_POINT('Ctrl Pts',(-38.6859137342731,-62.6134254046739,
0.));
#135493=CARTESIAN_POINT('Ctrl Pts',(-38.6859137342731,-62.6134254046739,
12.));
#135494=CARTESIAN_POINT('Ctrl Pts',(-38.6640950330421,-62.5980714899052,
0.));
#135495=CARTESIAN_POINT('Ctrl Pts',(-38.6640950330421,-62.5980714899052,
12.));
#135496=CARTESIAN_POINT('Ctrl Pts',(-38.6423205980213,-62.582718682292,
0.));
#135497=CARTESIAN_POINT('Ctrl Pts',(-38.6423205980213,-62.582718682292,
12.));
#135498=CARTESIAN_POINT('Ctrl Pts',(-38.6205904766073,-62.5673670749361,
0.));
#135499=CARTESIAN_POINT('Ctrl Pts',(-38.6205904766073,-62.5673670749361,
12.));
#135500=CARTESIAN_POINT('Ctrl Pts',(-38.5989047163393,-62.5520167614516,
0.));
#135501=CARTESIAN_POINT('Ctrl Pts',(-38.5989047163393,-62.5520167614516,
12.));
#135502=CARTESIAN_POINT('Ctrl Pts',(-38.5772633648832,-62.5366678359023,
0.));
#135503=CARTESIAN_POINT('Ctrl Pts',(-38.5772633648832,-62.5366678359023,
12.));
#135504=CARTESIAN_POINT('Ctrl Pts',(-38.5556664700195,-62.5213203927663,
0.));
#135505=CARTESIAN_POINT('Ctrl Pts',(-38.5556664700195,-62.5213203927663,
12.));
#135506=CARTESIAN_POINT('Ctrl Pts',(-38.5341140796248,-62.5059745268901,
0.));
#135507=CARTESIAN_POINT('Ctrl Pts',(-38.5341140796248,-62.5059745268901,
12.));
#135508=CARTESIAN_POINT('Ctrl Pts',(-38.5126062416502,-62.4906303334443,
0.));
#135509=CARTESIAN_POINT('Ctrl Pts',(-38.5126062416502,-62.4906303334443,
12.));
#135510=CARTESIAN_POINT('Ctrl Pts',(-38.4911430040997,-62.4752879078854,
0.));
#135511=CARTESIAN_POINT('Ctrl Pts',(-38.4911430040997,-62.4752879078854,
12.));
#135512=CARTESIAN_POINT('Ctrl Pts',(-38.4697244150482,-62.4599473459811,
0.));
#135513=CARTESIAN_POINT('Ctrl Pts',(-38.4697244150482,-62.4599473459811,
12.));
#135514=CARTESIAN_POINT('Ctrl Pts',(-38.4483505226518,-62.4446087438312,
0.));
#135515=CARTESIAN_POINT('Ctrl Pts',(-38.4483505226518,-62.4446087438312,
12.));
#135516=CARTESIAN_POINT('Ctrl Pts',(-38.4270213751568,-62.4292721978901,
0.));
#135517=CARTESIAN_POINT('Ctrl Pts',(-38.4270213751568,-62.4292721978901,
12.));
#135518=CARTESIAN_POINT('Ctrl Pts',(-38.405737020905,-62.4139378049885,
0.));
#135519=CARTESIAN_POINT('Ctrl Pts',(-38.405737020905,-62.4139378049885,
12.));
#135520=CARTESIAN_POINT('Ctrl Pts',(-38.3844975083343,-62.3986056623577,
0.));
#135521=CARTESIAN_POINT('Ctrl Pts',(-38.3844975083343,-62.3986056623577,
12.));
#135522=CARTESIAN_POINT('Ctrl Pts',(-38.3633028859828,-62.3832758676271,
0.));
#135523=CARTESIAN_POINT('Ctrl Pts',(-38.3633028859828,-62.3832758676271,
12.));
#135524=CARTESIAN_POINT('Ctrl Pts',(-38.342153202491,-62.3679485188171,
0.));
#135525=CARTESIAN_POINT('Ctrl Pts',(-38.342153202491,-62.3679485188171,
12.));
#135526=CARTESIAN_POINT('Ctrl Pts',(-38.3210485066001,-62.3526237143336,
0.));
#135527=CARTESIAN_POINT('Ctrl Pts',(-38.3210485066001,-62.3526237143336,
12.));
#135528=CARTESIAN_POINT('Ctrl Pts',(-38.2999888471476,-62.3373015529613,
0.));
#135529=CARTESIAN_POINT('Ctrl Pts',(-38.2999888471476,-62.3373015529613,
12.));
#135530=CARTESIAN_POINT('Ctrl Pts',(-38.2789742730564,-62.3219821338569,
0.));
#135531=CARTESIAN_POINT('Ctrl Pts',(-38.2789742730564,-62.3219821338569,
12.));
#135532=CARTESIAN_POINT('Ctrl Pts',(-38.2580048333361,-62.3066655565503,
0.));
#135533=CARTESIAN_POINT('Ctrl Pts',(-38.2580048333361,-62.3066655565503,
12.));
#135534=CARTESIAN_POINT('Ctrl Pts',(-38.2370805770935,-62.2913519209521,
0.));
#135535=CARTESIAN_POINT('Ctrl Pts',(-38.2370805770935,-62.2913519209521,
12.));
#135536=CARTESIAN_POINT('Ctrl Pts',(-38.2162015535353,-62.2760413273602,
0.));
#135537=CARTESIAN_POINT('Ctrl Pts',(-38.2162015535353,-62.2760413273602,
12.));
#135538=CARTESIAN_POINT('Ctrl Pts',(-38.1953678119691,-62.2607338764654,
0.));
#135539=CARTESIAN_POINT('Ctrl Pts',(-38.1953678119691,-62.2607338764654,
12.));
#135540=CARTESIAN_POINT('Ctrl Pts',(-38.1745794017996,-62.245429669358,
0.));
#135541=CARTESIAN_POINT('Ctrl Pts',(-38.1745794017996,-62.245429669358,
12.));
#135542=CARTESIAN_POINT('Ctrl Pts',(-38.1538363725264,-62.2301288075321,
0.));
#135543=CARTESIAN_POINT('Ctrl Pts',(-38.1538363725264,-62.2301288075321,
12.));
#135544=CARTESIAN_POINT('Ctrl Pts',(-38.133138773753,-62.2148313928863,
0.));
#135545=CARTESIAN_POINT('Ctrl Pts',(-38.133138773753,-62.2148313928863,
12.));
#135546=CARTESIAN_POINT('Ctrl Pts',(-38.1124866551886,-62.1995375277257,
0.));
#135547=CARTESIAN_POINT('Ctrl Pts',(-38.1124866551886,-62.1995375277257,
12.));
#135548=CARTESIAN_POINT('Ctrl Pts',(-38.0918800666479,-62.1842473147626,
0.));
#135549=CARTESIAN_POINT('Ctrl Pts',(-38.0918800666479,-62.1842473147626,
12.));
#135550=CARTESIAN_POINT('Ctrl Pts',(-38.0713190580463,-62.1689608571176,
0.));
#135551=CARTESIAN_POINT('Ctrl Pts',(-38.0713190580463,-62.1689608571176,
12.));
#135552=CARTESIAN_POINT('Ctrl Pts',(-38.0508036793939,-62.1536782583199,
0.));
#135553=CARTESIAN_POINT('Ctrl Pts',(-38.0508036793939,-62.1536782583199,
12.));
#135554=CARTESIAN_POINT('Ctrl Pts',(-38.0303339808053,-62.1383996223124,
0.));
#135555=CARTESIAN_POINT('Ctrl Pts',(-38.0303339808053,-62.1383996223124,
12.));
#135556=CARTESIAN_POINT('Ctrl Pts',(-38.0099100125037,-62.123125053455,
0.));
#135557=CARTESIAN_POINT('Ctrl Pts',(-38.0099100125037,-62.123125053455,
12.));
#135558=CARTESIAN_POINT('Ctrl Pts',(-37.9895318248212,-62.107854656528,
0.));
#135559=CARTESIAN_POINT('Ctrl Pts',(-37.9895318248212,-62.107854656528,
12.));
#135560=CARTESIAN_POINT('Ctrl Pts',(-37.9691994681966,-62.0925885367352,
0.));
#135561=CARTESIAN_POINT('Ctrl Pts',(-37.9691994681966,-62.0925885367352,
12.));
#135562=CARTESIAN_POINT('Ctrl Pts',(-37.9489129931689,-62.0773267997078,
0.));
#135563=CARTESIAN_POINT('Ctrl Pts',(-37.9489129931689,-62.0773267997078,
12.));
#135564=CARTESIAN_POINT('Ctrl Pts',(-37.9286724503851,-62.0620695515074,
0.));
#135565=CARTESIAN_POINT('Ctrl Pts',(-37.9286724503851,-62.0620695515074,
12.));
#135566=CARTESIAN_POINT('Ctrl Pts',(-37.9084778906053,-62.0468168986288,
0.));
#135567=CARTESIAN_POINT('Ctrl Pts',(-37.9084778906053,-62.0468168986288,
12.));
#135568=CARTESIAN_POINT('Ctrl Pts',(-37.8883293647029,-62.031568948002,
0.));
#135569=CARTESIAN_POINT('Ctrl Pts',(-37.8883293647029,-62.031568948002,
12.));
#135570=CARTESIAN_POINT('Ctrl Pts',(-37.868226923663,-62.0163258069957,
0.));
#135571=CARTESIAN_POINT('Ctrl Pts',(-37.868226923663,-62.0163258069957,
12.));
#135572=CARTESIAN_POINT('Ctrl Pts',(-37.8481706185749,-62.0010875834187,
0.));
#135573=CARTESIAN_POINT('Ctrl Pts',(-37.8481706185749,-62.0010875834187,
12.));
#135574=CARTESIAN_POINT('Ctrl Pts',(-37.828160500638,-61.9858543855236,
0.));
#135575=CARTESIAN_POINT('Ctrl Pts',(-37.828160500638,-61.9858543855236,
12.));
#135576=CARTESIAN_POINT('Ctrl Pts',(-37.8081966211689,-61.9706263220114,
0.));
#135577=CARTESIAN_POINT('Ctrl Pts',(-37.8081966211689,-61.9706263220114,
12.));
#135578=CARTESIAN_POINT('Ctrl Pts',(-37.7882790316014,-61.9554035020338,
0.));
#135579=CARTESIAN_POINT('Ctrl Pts',(-37.7882790316014,-61.9554035020338,
12.));
#135580=CARTESIAN_POINT('Ctrl Pts',(-37.7684077834872,-61.9401860351972,
0.));
#135581=CARTESIAN_POINT('Ctrl Pts',(-37.7684077834872,-61.9401860351972,
12.));
#135582=CARTESIAN_POINT('Ctrl Pts',(-37.7485829284871,-61.9249740315649,
0.));
#135583=CARTESIAN_POINT('Ctrl Pts',(-37.7485829284871,-61.9249740315649,
12.));
#135584=CARTESIAN_POINT('Ctrl Pts',(-37.7288045183756,-61.9097676016601,
0.));
#135585=CARTESIAN_POINT('Ctrl Pts',(-37.7288045183756,-61.9097676016601,
12.));
#135586=CARTESIAN_POINT('Ctrl Pts',(-37.7090726050482,-61.8945668564704,
0.));
#135587=CARTESIAN_POINT('Ctrl Pts',(-37.7090726050482,-61.8945668564704,
12.));
#135588=CARTESIAN_POINT('Ctrl Pts',(-37.6893872405228,-61.8793719074507,
0.));
#135589=CARTESIAN_POINT('Ctrl Pts',(-37.6893872405228,-61.8793719074507,
12.));
#135590=CARTESIAN_POINT('Ctrl Pts',(-37.6697484769392,-61.8641828665261,
0.));
#135591=CARTESIAN_POINT('Ctrl Pts',(-37.6697484769392,-61.8641828665261,
12.));
#135592=CARTESIAN_POINT('Ctrl Pts',(-37.6501563665523,-61.8489998460957,
0.));
#135593=CARTESIAN_POINT('Ctrl Pts',(-37.6501563665523,-61.8489998460957,
12.));
#135594=CARTESIAN_POINT('Ctrl Pts',(-37.6306109617346,-61.8338229590352,
0.));
#135595=CARTESIAN_POINT('Ctrl Pts',(-37.6306109617346,-61.8338229590352,
12.));
#135596=CARTESIAN_POINT('Ctrl Pts',(-37.6111123149839,-61.8186523187015,
0.));
#135597=CARTESIAN_POINT('Ctrl Pts',(-37.6111123149839,-61.8186523187015,
12.));
#135598=CARTESIAN_POINT('Ctrl Pts',(-37.5916604789253,-61.8034880389362,
0.));
#135599=CARTESIAN_POINT('Ctrl Pts',(-37.5916604789253,-61.8034880389362,
12.));
#135600=CARTESIAN_POINT('Ctrl Pts',(-37.5722555063111,-61.7883302340687,
0.));
#135601=CARTESIAN_POINT('Ctrl Pts',(-37.5722555063111,-61.7883302340687,
12.));
#135602=CARTESIAN_POINT('Ctrl Pts',(-37.5528974500142,-61.773179018919,
0.));
#135603=CARTESIAN_POINT('Ctrl Pts',(-37.5528974500142,-61.773179018919,
12.));
#135604=CARTESIAN_POINT('Ctrl Pts',(-37.5335863630287,-61.7580345088016,
0.));
#135605=CARTESIAN_POINT('Ctrl Pts',(-37.5335863630287,-61.7580345088016,
12.));
#135606=CARTESIAN_POINT('Ctrl Pts',(-37.5143222984796,-61.7428968195299,
0.));
#135607=CARTESIAN_POINT('Ctrl Pts',(-37.5143222984796,-61.7428968195299,
12.));
#135608=CARTESIAN_POINT('Ctrl Pts',(-37.4951053096237,-61.7277660674205,
0.));
#135609=CARTESIAN_POINT('Ctrl Pts',(-37.4951053096237,-61.7277660674205,
12.));
#135610=CARTESIAN_POINT('Ctrl Pts',(-37.4759354498509,-61.7126423692963,
0.));
#135611=CARTESIAN_POINT('Ctrl Pts',(-37.4759354498509,-61.7126423692963,
12.));
#135612=CARTESIAN_POINT('Ctrl Pts',(-37.4568127726773,-61.6975258424894,
0.));
#135613=CARTESIAN_POINT('Ctrl Pts',(-37.4568127726773,-61.6975258424894,
12.));
#135614=CARTESIAN_POINT('Ctrl Pts',(-37.4377373317451,-61.6824166048444,
0.));
#135615=CARTESIAN_POINT('Ctrl Pts',(-37.4377373317451,-61.6824166048444,
12.));
#135616=CARTESIAN_POINT('Ctrl Pts',(-37.4187091808321,-61.6673147747242,
0.));
#135617=CARTESIAN_POINT('Ctrl Pts',(-37.4187091808321,-61.6673147747242,
12.));
#135618=CARTESIAN_POINT('Ctrl Pts',(-37.3997283738533,-61.6522204710131,
0.));
#135619=CARTESIAN_POINT('Ctrl Pts',(-37.3997283738533,-61.6522204710131,
12.));
#135620=CARTESIAN_POINT('Ctrl Pts',(-37.3807949648624,-61.637133813121,
0.));
#135621=CARTESIAN_POINT('Ctrl Pts',(-37.3807949648624,-61.637133813121,
12.));
#135622=CARTESIAN_POINT('Ctrl Pts',(-37.361909008045,-61.6220549209866,
0.));
#135623=CARTESIAN_POINT('Ctrl Pts',(-37.361909008045,-61.6220549209866,
12.));
#135624=CARTESIAN_POINT('Ctrl Pts',(-37.343070557718,-61.6069839150807,
0.));
#135625=CARTESIAN_POINT('Ctrl Pts',(-37.343070557718,-61.6069839150807,
12.));
#135626=CARTESIAN_POINT('Ctrl Pts',(-37.3242796683395,-61.591920916412,
0.));
#135627=CARTESIAN_POINT('Ctrl Pts',(-37.3242796683395,-61.591920916412,
12.));
#135628=CARTESIAN_POINT('Ctrl Pts',(-37.3055363945107,-61.5768660465311,
0.));
#135629=CARTESIAN_POINT('Ctrl Pts',(-37.3055363945107,-61.5768660465311,
12.));
#135630=CARTESIAN_POINT('Ctrl Pts',(-37.2868407909771,-61.5618194275348,
0.));
#135631=CARTESIAN_POINT('Ctrl Pts',(-37.2868407909771,-61.5618194275348,
12.));
#135632=CARTESIAN_POINT('Ctrl Pts',(-37.2681929126221,-61.5467811820691,
0.));
#135633=CARTESIAN_POINT('Ctrl Pts',(-37.2681929126221,-61.5467811820691,
12.));
#135634=CARTESIAN_POINT('Ctrl Pts',(-37.2495928144667,-61.5317514333328,
0.));
#135635=CARTESIAN_POINT('Ctrl Pts',(-37.2495928144667,-61.5317514333328,
12.));
#135636=CARTESIAN_POINT('Ctrl Pts',(-37.2310405516781,-61.5167303050832,
0.));
#135637=CARTESIAN_POINT('Ctrl Pts',(-37.2310405516781,-61.5167303050832,
12.));
#135638=CARTESIAN_POINT('Ctrl Pts',(-37.2125361795731,-61.501717921641,
0.));
#135639=CARTESIAN_POINT('Ctrl Pts',(-37.2125361795731,-61.501717921641,
12.));
#135640=CARTESIAN_POINT('Ctrl Pts',(-37.1940797536181,-61.4867144078936,
0.));
#135641=CARTESIAN_POINT('Ctrl Pts',(-37.1940797536181,-61.4867144078936,
12.));
#135642=CARTESIAN_POINT('Ctrl Pts',(-37.175671329424,-61.4717198892994,
0.));
#135643=CARTESIAN_POINT('Ctrl Pts',(-37.175671329424,-61.4717198892994,
12.));
#135644=CARTESIAN_POINT('Ctrl Pts',(-37.1573109627454,-61.4567344918919,
0.));
#135645=CARTESIAN_POINT('Ctrl Pts',(-37.1573109627454,-61.4567344918919,
12.));
#135646=CARTESIAN_POINT('Ctrl Pts',(-37.1389987094905,-61.4417583422863,
0.));
#135647=CARTESIAN_POINT('Ctrl Pts',(-37.1389987094905,-61.4417583422863,
12.));
#135648=CARTESIAN_POINT('Ctrl Pts',(-37.1207346257222,-61.4267915676822,
0.));
#135649=CARTESIAN_POINT('Ctrl Pts',(-37.1207346257222,-61.4267915676822,
12.));
#135650=CARTESIAN_POINT('Ctrl Pts',(-37.1025187676602,-61.4118342958697,
0.));
#135651=CARTESIAN_POINT('Ctrl Pts',(-37.1025187676602,-61.4118342958697,
12.));
#135652=CARTESIAN_POINT('Ctrl Pts',(-37.0843511916745,-61.3968866552317,
0.));
#135653=CARTESIAN_POINT('Ctrl Pts',(-37.0843511916745,-61.3968866552317,
12.));
#135654=CARTESIAN_POINT('Ctrl Pts',(-37.0662319542849,-61.381948774749,
0.));
#135655=CARTESIAN_POINT('Ctrl Pts',(-37.0662319542849,-61.381948774749,
12.));
#135656=CARTESIAN_POINT('Ctrl Pts',(-37.0481611121717,-61.3670207840068,
0.));
#135657=CARTESIAN_POINT('Ctrl Pts',(-37.0481611121717,-61.3670207840068,
12.));
#135658=CARTESIAN_POINT('Ctrl Pts',(-37.0301387221774,-61.3521028132003,
0.));
#135659=CARTESIAN_POINT('Ctrl Pts',(-37.0301387221774,-61.3521028132003,
12.));
#135660=CARTESIAN_POINT('Ctrl Pts',(-37.0121648413082,-61.3371949931387,
0.));
#135661=CARTESIAN_POINT('Ctrl Pts',(-37.0121648413082,-61.3371949931387,
12.));
#135662=CARTESIAN_POINT('Ctrl Pts',(-36.994239526727,-61.3222974552486,
0.));
#135663=CARTESIAN_POINT('Ctrl Pts',(-36.994239526727,-61.3222974552486,
12.));
#135664=CARTESIAN_POINT('Ctrl Pts',(-36.9763628357544,-61.3074103315791,
0.));
#135665=CARTESIAN_POINT('Ctrl Pts',(-36.9763628357544,-61.3074103315791,
12.));
#135666=CARTESIAN_POINT('Ctrl Pts',(-36.9585348258776,-61.2925337548077,
0.));
#135667=CARTESIAN_POINT('Ctrl Pts',(-36.9585348258776,-61.2925337548077,
12.));
#135668=CARTESIAN_POINT('Ctrl Pts',(-36.9407555547535,-61.2776678582461,
0.));
#135669=CARTESIAN_POINT('Ctrl Pts',(-36.9407555547535,-61.2776678582461,
12.));
#135670=CARTESIAN_POINT('Ctrl Pts',(-36.9230250802087,-61.2628127758457,
0.));
#135671=CARTESIAN_POINT('Ctrl Pts',(-36.9230250802087,-61.2628127758457,
12.));
#135672=CARTESIAN_POINT('Ctrl Pts',(-36.9053434602343,-61.247968642201,
0.));
#135673=CARTESIAN_POINT('Ctrl Pts',(-36.9053434602343,-61.247968642201,
12.));
#135674=CARTESIAN_POINT('Ctrl Pts',(-36.8877107529865,-61.2331355925547,
0.));
#135675=CARTESIAN_POINT('Ctrl Pts',(-36.8877107529865,-61.2331355925547,
12.));
#135676=CARTESIAN_POINT('Ctrl Pts',(-36.8701270167969,-61.2183137628056,
0.));
#135677=CARTESIAN_POINT('Ctrl Pts',(-36.8701270167969,-61.2183137628056,
12.));
#135678=CARTESIAN_POINT('Ctrl Pts',(-36.852592310174,-61.2035032895127,
0.));
#135679=CARTESIAN_POINT('Ctrl Pts',(-36.852592310174,-61.2035032895127,
12.));
#135680=CARTESIAN_POINT('Ctrl Pts',(-36.8351066918036,-61.1887043099014,
0.));
#135681=CARTESIAN_POINT('Ctrl Pts',(-36.8351066918036,-61.1887043099014,
12.));
#135682=CARTESIAN_POINT('Ctrl Pts',(-36.8176702205423,-61.1739169618666,
0.));
#135683=CARTESIAN_POINT('Ctrl Pts',(-36.8176702205423,-61.1739169618666,
12.));
#135684=CARTESIAN_POINT('Ctrl Pts',(-36.8002829554209,-61.1591413839787,
0.));
#135685=CARTESIAN_POINT('Ctrl Pts',(-36.8002829554209,-61.1591413839787,
12.));
#135686=CARTESIAN_POINT('Ctrl Pts',(-36.7829449556532,-61.1443777154911,
0.));
#135687=CARTESIAN_POINT('Ctrl Pts',(-36.7829449556532,-61.1443777154911,
12.));
#135688=CARTESIAN_POINT('Ctrl Pts',(-36.765656280638,-61.1296260963466,
0.));
#135689=CARTESIAN_POINT('Ctrl Pts',(-36.765656280638,-61.1296260963466,
12.));
#135690=CARTESIAN_POINT('Ctrl Pts',(-36.7484169899596,-61.1148866671829,
0.));
#135691=CARTESIAN_POINT('Ctrl Pts',(-36.7484169899596,-61.1148866671829,
12.));
#135692=CARTESIAN_POINT('Ctrl Pts',(-36.7312271433807,-61.100159569337,
0.));
#135693=CARTESIAN_POINT('Ctrl Pts',(-36.7312271433807,-61.100159569337,
12.));
#135694=CARTESIAN_POINT('Ctrl Pts',(-36.7140868008486,-61.0854449448524,
0.));
#135695=CARTESIAN_POINT('Ctrl Pts',(-36.7140868008486,-61.0854449448524,
12.));
#135696=CARTESIAN_POINT('Ctrl Pts',(-36.6969960225022,-61.0707429364847,
0.));
#135697=CARTESIAN_POINT('Ctrl Pts',(-36.6969960225022,-61.0707429364847,
12.));
#135698=CARTESIAN_POINT('Ctrl Pts',(-36.679954868674,-61.0560536877083,
0.));
#135699=CARTESIAN_POINT('Ctrl Pts',(-36.679954868674,-61.0560536877083,
12.));
#135700=CARTESIAN_POINT('Ctrl Pts',(-36.6629633998886,-61.0413773427203,
0.));
#135701=CARTESIAN_POINT('Ctrl Pts',(-36.6629633998886,-61.0413773427203,
12.));
#135702=CARTESIAN_POINT('Ctrl Pts',(-36.6460216768553,-61.0267140464432,
0.));
#135703=CARTESIAN_POINT('Ctrl Pts',(-36.6460216768553,-61.0267140464432,
12.));
#135704=CARTESIAN_POINT('Ctrl Pts',(-36.6291297604776,-61.0120639445349,
0.));
#135705=CARTESIAN_POINT('Ctrl Pts',(-36.6291297604776,-61.0120639445349,
12.));
#135706=CARTESIAN_POINT('Ctrl Pts',(-36.61228771186,-60.9974271833981,0.));
#135707=CARTESIAN_POINT('Ctrl Pts',(-36.61228771186,-60.9974271833981,12.));
#135708=CARTESIAN_POINT('Ctrl Pts',(-36.595495592311,-60.9828039101887,
0.));
#135709=CARTESIAN_POINT('Ctrl Pts',(-36.595495592311,-60.9828039101887,
12.));
#135710=CARTESIAN_POINT('Ctrl Pts',(-36.5787534633416,-60.9681942728236,
0.));
#135711=CARTESIAN_POINT('Ctrl Pts',(-36.5787534633416,-60.9681942728236,
12.));
#135712=CARTESIAN_POINT('Ctrl Pts',(-36.5620613866615,-60.9535984199873,
0.));
#135713=CARTESIAN_POINT('Ctrl Pts',(-36.5620613866615,-60.9535984199873,
12.));
#135714=CARTESIAN_POINT('Ctrl Pts',(-36.5454194241865,-60.9390165011355,
0.));
#135715=CARTESIAN_POINT('Ctrl Pts',(-36.5454194241865,-60.9390165011355,
12.));
#135716=CARTESIAN_POINT('Ctrl Pts',(-36.5288276380416,-60.9244486664987,
0.));
#135717=CARTESIAN_POINT('Ctrl Pts',(-36.5288276380416,-60.9244486664987,
12.));
#135718=CARTESIAN_POINT('Ctrl Pts',(-36.5122860905612,-60.9098950670847,
0.));
#135719=CARTESIAN_POINT('Ctrl Pts',(-36.5122860905612,-60.9098950670847,
12.));
#135720=CARTESIAN_POINT('Ctrl Pts',(-36.4957948442835,-60.8953558546795,
0.));
#135721=CARTESIAN_POINT('Ctrl Pts',(-36.4957948442835,-60.8953558546795,
12.));
#135722=CARTESIAN_POINT('Ctrl Pts',(-36.4793539619466,-60.8808311818499,
0.));
#135723=CARTESIAN_POINT('Ctrl Pts',(-36.4793539619466,-60.8808311818499,
12.));
#135724=CARTESIAN_POINT('Ctrl Pts',(-36.4629635065045,-60.8663212019657,
0.));
#135725=CARTESIAN_POINT('Ctrl Pts',(-36.4629635065045,-60.8663212019657,
12.));
#135726=CARTESIAN_POINT('Ctrl Pts',(-36.4466235411358,-60.8518260692188,
0.));
#135727=CARTESIAN_POINT('Ctrl Pts',(-36.4466235411358,-60.8518260692188,
12.));
#135728=CARTESIAN_POINT('Ctrl Pts',(-36.4303341292494,-60.8373459386392,
0.));
#135729=CARTESIAN_POINT('Ctrl Pts',(-36.4303341292494,-60.8373459386392,
12.));
#135730=CARTESIAN_POINT('Ctrl Pts',(-36.4140953344858,-60.822880966116,
0.));
#135731=CARTESIAN_POINT('Ctrl Pts',(-36.4140953344858,-60.822880966116,
12.));
#135732=CARTESIAN_POINT('Ctrl Pts',(-36.397907220716,-60.8084313083984,
0.));
#135733=CARTESIAN_POINT('Ctrl Pts',(-36.397907220716,-60.8084313083984,
12.));
#135734=CARTESIAN_POINT('Ctrl Pts',(-36.3817698520388,-60.793997123076,
0.));
#135735=CARTESIAN_POINT('Ctrl Pts',(-36.3817698520388,-60.793997123076,
12.));
#135736=CARTESIAN_POINT('Ctrl Pts',(-36.365683292773,-60.7795785685625,
0.));
#135737=CARTESIAN_POINT('Ctrl Pts',(-36.365683292773,-60.7795785685625,
12.));
#135738=CARTESIAN_POINT('Ctrl Pts',(-36.3496476074488,-60.7651758040803,
0.));
#135739=CARTESIAN_POINT('Ctrl Pts',(-36.3496476074488,-60.7651758040803,
12.));
#135740=CARTESIAN_POINT('Ctrl Pts',(-36.3336628607859,-60.7507889896308,
0.));
#135741=CARTESIAN_POINT('Ctrl Pts',(-36.3336628607859,-60.7507889896308,
12.));
#135742=CARTESIAN_POINT('Ctrl Pts',(-36.3177291177163,-60.7364182860412,
0.));
#135743=CARTESIAN_POINT('Ctrl Pts',(-36.3177291177163,-60.7364182860412,
12.));
#135744=CARTESIAN_POINT('Ctrl Pts',(-36.3018464434214,-60.722063855041,
0.));
#135745=CARTESIAN_POINT('Ctrl Pts',(-36.3018464434214,-60.722063855041,
12.));
#135746=CARTESIAN_POINT('Ctrl Pts',(-36.2860149033587,-60.7077258593268,
0.));
#135747=CARTESIAN_POINT('Ctrl Pts',(-36.2860149033587,-60.7077258593268,
12.));
#135748=CARTESIAN_POINT('Ctrl Pts',(-36.2702345632875,-60.6934044626291,
0.));
#135749=CARTESIAN_POINT('Ctrl Pts',(-36.2702345632875,-60.6934044626291,
12.));
#135750=CARTESIAN_POINT('Ctrl Pts',(-36.2545054892897,-60.67909982978,0.));
#135751=CARTESIAN_POINT('Ctrl Pts',(-36.2545054892897,-60.67909982978,12.));
#135752=CARTESIAN_POINT('Ctrl Pts',(-36.2388277477212,-60.6648121265885,
0.));
#135753=CARTESIAN_POINT('Ctrl Pts',(-36.2388277477212,-60.6648121265885,
12.));
#135754=CARTESIAN_POINT('Ctrl Pts',(-36.2232014051541,-60.6505415197042,
0.));
#135755=CARTESIAN_POINT('Ctrl Pts',(-36.2232014051541,-60.6505415197042,
12.));
#135756=CARTESIAN_POINT('Ctrl Pts',(-36.2076265283264,-60.6362881765019,
0.));
#135757=CARTESIAN_POINT('Ctrl Pts',(-36.2076265283264,-60.6362881765019,
12.));
#135758=CARTESIAN_POINT('Ctrl Pts',(-36.192103184063,-60.6220522649149,
0.));
#135759=CARTESIAN_POINT('Ctrl Pts',(-36.192103184063,-60.6220522649149,
12.));
#135760=CARTESIAN_POINT('Ctrl Pts',(-36.1766314392641,-60.6078339534181,
0.));
#135761=CARTESIAN_POINT('Ctrl Pts',(-36.1766314392641,-60.6078339534181,
12.));
#135762=CARTESIAN_POINT('Ctrl Pts',(-36.1612113610773,-60.5936334114108,
0.));
#135763=CARTESIAN_POINT('Ctrl Pts',(-36.1612113610773,-60.5936334114108,
12.));
#135764=CARTESIAN_POINT('Ctrl Pts',(-36.1458430170431,-60.5794508095564,
0.));
#135765=CARTESIAN_POINT('Ctrl Pts',(-36.1458430170431,-60.5794508095564,
12.));
#135766=CARTESIAN_POINT('Ctrl Pts',(-36.1305264752188,-60.565286320072,
0.));
#135767=CARTESIAN_POINT('Ctrl Pts',(-36.1305264752188,-60.565286320072,
12.));
#135768=CARTESIAN_POINT('Ctrl Pts',(-36.1152618043739,-60.5511401171984,
0.));
#135769=CARTESIAN_POINT('Ctrl Pts',(-36.1152618043739,-60.5511401171984,
12.));
#135770=CARTESIAN_POINT('Ctrl Pts',(-36.100049073851,-60.5370123768804,
0.));
#135771=CARTESIAN_POINT('Ctrl Pts',(-36.100049073851,-60.5370123768804,
12.));
#135772=CARTESIAN_POINT('Ctrl Pts',(-36.0848883531952,-60.5229032758973,
0.));
#135773=CARTESIAN_POINT('Ctrl Pts',(-36.0848883531952,-60.5229032758973,
12.));
#135774=CARTESIAN_POINT('Ctrl Pts',(-36.0697797118376,-60.5088129911354,
0.));
#135775=CARTESIAN_POINT('Ctrl Pts',(-36.0697797118376,-60.5088129911354,
12.));
#135776=CARTESIAN_POINT('Ctrl Pts',(-36.0547232187698,-60.4947416988422,
0.));
#135777=CARTESIAN_POINT('Ctrl Pts',(-36.0547232187698,-60.4947416988422,
12.));
#135778=CARTESIAN_POINT('Ctrl Pts',(-36.0397189421644,-60.4806895737686,
0.));
#135779=CARTESIAN_POINT('Ctrl Pts',(-36.0397189421644,-60.4806895737686,
12.));
#135780=CARTESIAN_POINT('Ctrl Pts',(-36.0247669500891,-60.4666567908093,
0.));
#135781=CARTESIAN_POINT('Ctrl Pts',(-36.0247669500891,-60.4666567908093,
12.));
#135782=CARTESIAN_POINT('Ctrl Pts',(-36.009867311357,-60.4526435269662,
0.));
#135783=CARTESIAN_POINT('Ctrl Pts',(-36.009867311357,-60.4526435269662,
12.));
#135784=CARTESIAN_POINT('Ctrl Pts',(-35.995020096217,-60.4386499629481,
0.));
#135785=CARTESIAN_POINT('Ctrl Pts',(-35.995020096217,-60.4386499629481,
12.));
#135786=CARTESIAN_POINT('Ctrl Pts',(-35.9802253773515,-60.4246762854926,
0.));
#135787=CARTESIAN_POINT('Ctrl Pts',(-35.9802253773515,-60.4246762854926,
12.));
#135788=CARTESIAN_POINT('Ctrl Pts',(-35.9654832299601,-60.4107226875714,
0.));
#135789=CARTESIAN_POINT('Ctrl Pts',(-35.9654832299601,-60.4107226875714,
12.));
#135790=CARTESIAN_POINT('Ctrl Pts',(-35.9507937296707,-60.3967893635452,
0.));
#135791=CARTESIAN_POINT('Ctrl Pts',(-35.9507937296707,-60.3967893635452,
12.));
#135792=CARTESIAN_POINT('Ctrl Pts',(-35.936156950695,-60.3828765049019,
0.));
#135793=CARTESIAN_POINT('Ctrl Pts',(-35.936156950695,-60.3828765049019,
12.));
#135794=CARTESIAN_POINT('Ctrl Pts',(-35.9215729642231,-60.3689842965481,
0.));
#135795=CARTESIAN_POINT('Ctrl Pts',(-35.9215729642231,-60.3689842965481,
12.));
#135796=CARTESIAN_POINT('Ctrl Pts',(-35.907041835853,-60.3551129108845,
0.));
#135797=CARTESIAN_POINT('Ctrl Pts',(-35.907041835853,-60.3551129108845,
12.));
#135798=CARTESIAN_POINT('Ctrl Pts',(-35.8925636280668,-60.3412625135287,
0.));
#135799=CARTESIAN_POINT('Ctrl Pts',(-35.8925636280668,-60.3412625135287,
12.));
#135800=CARTESIAN_POINT('Ctrl Pts',(-35.8781384051537,-60.327433274683,
0.));
#135801=CARTESIAN_POINT('Ctrl Pts',(-35.8781384051537,-60.327433274683,
12.));
#135802=CARTESIAN_POINT('Ctrl Pts',(-35.8637662371635,-60.3136253782809,
0.));
#135803=CARTESIAN_POINT('Ctrl Pts',(-35.8637662371635,-60.3136253782809,
12.));
#135804=CARTESIAN_POINT('Ctrl Pts',(-35.8494472046745,-60.2998390330102,
0.));
#135805=CARTESIAN_POINT('Ctrl Pts',(-35.8494472046745,-60.2998390330102,
12.));
#135806=CARTESIAN_POINT('Ctrl Pts',(-35.8351814020357,-60.2860744798436,
0.));
#135807=CARTESIAN_POINT('Ctrl Pts',(-35.8351814020357,-60.2860744798436,
12.));
#135808=CARTESIAN_POINT('Ctrl Pts',(-35.8209689272501,-60.2723319687369,
0.));
#135809=CARTESIAN_POINT('Ctrl Pts',(-35.8209689272501,-60.2723319687369,
12.));
#135810=CARTESIAN_POINT('Ctrl Pts',(-35.8068098723347,-60.2586117365205,
0.));
#135811=CARTESIAN_POINT('Ctrl Pts',(-35.8068098723347,-60.2586117365205,
12.));
#135812=CARTESIAN_POINT('Ctrl Pts',(-35.7927043145201,-60.2449139865274,
0.));
#135813=CARTESIAN_POINT('Ctrl Pts',(-35.7927043145201,-60.2449139865274,
12.));
#135814=CARTESIAN_POINT('Ctrl Pts',(-35.7786523045912,-60.2312388621529,
0.));
#135815=CARTESIAN_POINT('Ctrl Pts',(-35.7786523045912,-60.2312388621529,
12.));
#135816=CARTESIAN_POINT('Ctrl Pts',(-35.7646538667493,-60.2175864450043,
0.));
#135817=CARTESIAN_POINT('Ctrl Pts',(-35.7646538667493,-60.2175864450043,
12.));
#135818=CARTESIAN_POINT('Ctrl Pts',(-35.7534979802053,-60.206682708692,
0.));
#135819=CARTESIAN_POINT('Ctrl Pts',(-35.7534979802053,-60.206682708692,
12.));
#135820=CARTESIAN_POINT('Ctrl Pts',(-35.7451551752572,-60.1985151474623,
0.));
#135821=CARTESIAN_POINT('Ctrl Pts',(-35.7451551752572,-60.1985151474623,
12.));
#135822=CARTESIAN_POINT('Ctrl Pts',(-35.7396040204017,-60.193074658032,
0.));
#135823=CARTESIAN_POINT('Ctrl Pts',(-35.7396040204017,-60.193074658032,
12.));
#135824=CARTESIAN_POINT('Ctrl Pts',(-35.736831121751,-60.1903555511633,
0.));
#135825=CARTESIAN_POINT('Ctrl Pts',(-35.736831121751,-60.1903555511633,
12.));
#135826=CARTESIAN_POINT('',(-35.736831121751,-60.1903555511633,12.));
#135827=CARTESIAN_POINT('Ctrl Pts',(-35.736831121751,-60.1903555511633,
12.));
#135828=CARTESIAN_POINT('Ctrl Pts',(-35.7396040204017,-60.193074658032,
12.));
#135829=CARTESIAN_POINT('Ctrl Pts',(-35.7451551752572,-60.1985151474623,
12.));
#135830=CARTESIAN_POINT('Ctrl Pts',(-35.7534979802053,-60.206682708692,
12.));
#135831=CARTESIAN_POINT('Ctrl Pts',(-35.7646538667493,-60.2175864450043,
12.));
#135832=CARTESIAN_POINT('Ctrl Pts',(-35.7786523045912,-60.2312388621529,
12.));
#135833=CARTESIAN_POINT('Ctrl Pts',(-35.7927043145201,-60.2449139865274,
12.));
#135834=CARTESIAN_POINT('Ctrl Pts',(-35.8068098723347,-60.2586117365205,
12.));
#135835=CARTESIAN_POINT('Ctrl Pts',(-35.8209689272501,-60.2723319687369,
12.));
#135836=CARTESIAN_POINT('Ctrl Pts',(-35.8351814020357,-60.2860744798436,
12.));
#135837=CARTESIAN_POINT('Ctrl Pts',(-35.8494472046745,-60.2998390330102,
12.));
#135838=CARTESIAN_POINT('Ctrl Pts',(-35.8637662371635,-60.3136253782809,
12.));
#135839=CARTESIAN_POINT('Ctrl Pts',(-35.8781384051537,-60.327433274683,
12.));
#135840=CARTESIAN_POINT('Ctrl Pts',(-35.8925636280668,-60.3412625135287,
12.));
#135841=CARTESIAN_POINT('Ctrl Pts',(-35.907041835853,-60.3551129108845,
12.));
#135842=CARTESIAN_POINT('Ctrl Pts',(-35.9215729642231,-60.3689842965481,
12.));
#135843=CARTESIAN_POINT('Ctrl Pts',(-35.936156950695,-60.3828765049019,
12.));
#135844=CARTESIAN_POINT('Ctrl Pts',(-35.9507937296707,-60.3967893635452,
12.));
#135845=CARTESIAN_POINT('Ctrl Pts',(-35.9654832299601,-60.4107226875714,
12.));
#135846=CARTESIAN_POINT('Ctrl Pts',(-35.9802253773515,-60.4246762854926,
12.));
#135847=CARTESIAN_POINT('Ctrl Pts',(-35.995020096217,-60.4386499629481,
12.));
#135848=CARTESIAN_POINT('Ctrl Pts',(-36.009867311357,-60.4526435269662,
12.));
#135849=CARTESIAN_POINT('Ctrl Pts',(-36.0247669500891,-60.4666567908093,
12.));
#135850=CARTESIAN_POINT('Ctrl Pts',(-36.0397189421644,-60.4806895737686,
12.));
#135851=CARTESIAN_POINT('Ctrl Pts',(-36.0547232187698,-60.4947416988422,
12.));
#135852=CARTESIAN_POINT('Ctrl Pts',(-36.0697797118376,-60.5088129911354,
12.));
#135853=CARTESIAN_POINT('Ctrl Pts',(-36.0848883531952,-60.5229032758973,
12.));
#135854=CARTESIAN_POINT('Ctrl Pts',(-36.100049073851,-60.5370123768804,
12.));
#135855=CARTESIAN_POINT('Ctrl Pts',(-36.1152618043739,-60.5511401171984,
12.));
#135856=CARTESIAN_POINT('Ctrl Pts',(-36.1305264752188,-60.565286320072,
12.));
#135857=CARTESIAN_POINT('Ctrl Pts',(-36.1458430170431,-60.5794508095564,
12.));
#135858=CARTESIAN_POINT('Ctrl Pts',(-36.1612113610773,-60.5936334114108,
12.));
#135859=CARTESIAN_POINT('Ctrl Pts',(-36.1766314392641,-60.6078339534181,
12.));
#135860=CARTESIAN_POINT('Ctrl Pts',(-36.192103184063,-60.6220522649149,
12.));
#135861=CARTESIAN_POINT('Ctrl Pts',(-36.2076265283264,-60.6362881765019,
12.));
#135862=CARTESIAN_POINT('Ctrl Pts',(-36.2232014051541,-60.6505415197042,
12.));
#135863=CARTESIAN_POINT('Ctrl Pts',(-36.2388277477212,-60.6648121265885,
12.));
#135864=CARTESIAN_POINT('Ctrl Pts',(-36.2545054892897,-60.67909982978,12.));
#135865=CARTESIAN_POINT('Ctrl Pts',(-36.2702345632875,-60.6934044626291,
12.));
#135866=CARTESIAN_POINT('Ctrl Pts',(-36.2860149033587,-60.7077258593268,
12.));
#135867=CARTESIAN_POINT('Ctrl Pts',(-36.3018464434214,-60.722063855041,
12.));
#135868=CARTESIAN_POINT('Ctrl Pts',(-36.3177291177163,-60.7364182860412,
12.));
#135869=CARTESIAN_POINT('Ctrl Pts',(-36.3336628607859,-60.7507889896308,
12.));
#135870=CARTESIAN_POINT('Ctrl Pts',(-36.3496476074488,-60.7651758040803,
12.));
#135871=CARTESIAN_POINT('Ctrl Pts',(-36.365683292773,-60.7795785685625,
12.));
#135872=CARTESIAN_POINT('Ctrl Pts',(-36.3817698520388,-60.793997123076,
12.));
#135873=CARTESIAN_POINT('Ctrl Pts',(-36.397907220716,-60.8084313083984,
12.));
#135874=CARTESIAN_POINT('Ctrl Pts',(-36.4140953344858,-60.822880966116,
12.));
#135875=CARTESIAN_POINT('Ctrl Pts',(-36.4303341292494,-60.8373459386392,
12.));
#135876=CARTESIAN_POINT('Ctrl Pts',(-36.4466235411358,-60.8518260692188,
12.));
#135877=CARTESIAN_POINT('Ctrl Pts',(-36.4629635065045,-60.8663212019657,
12.));
#135878=CARTESIAN_POINT('Ctrl Pts',(-36.4793539619466,-60.8808311818499,
12.));
#135879=CARTESIAN_POINT('Ctrl Pts',(-36.4957948442835,-60.8953558546795,
12.));
#135880=CARTESIAN_POINT('Ctrl Pts',(-36.5122860905612,-60.9098950670847,
12.));
#135881=CARTESIAN_POINT('Ctrl Pts',(-36.5288276380416,-60.9244486664987,
12.));
#135882=CARTESIAN_POINT('Ctrl Pts',(-36.5454194241865,-60.9390165011355,
12.));
#135883=CARTESIAN_POINT('Ctrl Pts',(-36.5620613866615,-60.9535984199873,
12.));
#135884=CARTESIAN_POINT('Ctrl Pts',(-36.5787534633416,-60.9681942728236,
12.));
#135885=CARTESIAN_POINT('Ctrl Pts',(-36.595495592311,-60.9828039101887,
12.));
#135886=CARTESIAN_POINT('Ctrl Pts',(-36.61228771186,-60.9974271833981,12.));
#135887=CARTESIAN_POINT('Ctrl Pts',(-36.6291297604776,-61.0120639445349,
12.));
#135888=CARTESIAN_POINT('Ctrl Pts',(-36.6460216768553,-61.0267140464432,
12.));
#135889=CARTESIAN_POINT('Ctrl Pts',(-36.6629633998886,-61.0413773427203,
12.));
#135890=CARTESIAN_POINT('Ctrl Pts',(-36.679954868674,-61.0560536877083,
12.));
#135891=CARTESIAN_POINT('Ctrl Pts',(-36.6969960225022,-61.0707429364847,
12.));
#135892=CARTESIAN_POINT('Ctrl Pts',(-36.7140868008486,-61.0854449448524,
12.));
#135893=CARTESIAN_POINT('Ctrl Pts',(-36.7312271433807,-61.100159569337,
12.));
#135894=CARTESIAN_POINT('Ctrl Pts',(-36.7484169899596,-61.1148866671829,
12.));
#135895=CARTESIAN_POINT('Ctrl Pts',(-36.765656280638,-61.1296260963466,
12.));
#135896=CARTESIAN_POINT('Ctrl Pts',(-36.7829449556532,-61.1443777154911,
12.));
#135897=CARTESIAN_POINT('Ctrl Pts',(-36.8002829554209,-61.1591413839787,
12.));
#135898=CARTESIAN_POINT('Ctrl Pts',(-36.8176702205423,-61.1739169618666,
12.));
#135899=CARTESIAN_POINT('Ctrl Pts',(-36.8351066918036,-61.1887043099014,
12.));
#135900=CARTESIAN_POINT('Ctrl Pts',(-36.852592310174,-61.2035032895127,
12.));
#135901=CARTESIAN_POINT('Ctrl Pts',(-36.8701270167969,-61.2183137628056,
12.));
#135902=CARTESIAN_POINT('Ctrl Pts',(-36.8877107529865,-61.2331355925547,
12.));
#135903=CARTESIAN_POINT('Ctrl Pts',(-36.9053434602343,-61.247968642201,
12.));
#135904=CARTESIAN_POINT('Ctrl Pts',(-36.9230250802087,-61.2628127758457,
12.));
#135905=CARTESIAN_POINT('Ctrl Pts',(-36.9407555547535,-61.2776678582461,
12.));
#135906=CARTESIAN_POINT('Ctrl Pts',(-36.9585348258776,-61.2925337548077,
12.));
#135907=CARTESIAN_POINT('Ctrl Pts',(-36.9763628357544,-61.3074103315791,
12.));
#135908=CARTESIAN_POINT('Ctrl Pts',(-36.994239526727,-61.3222974552486,
12.));
#135909=CARTESIAN_POINT('Ctrl Pts',(-37.0121648413082,-61.3371949931387,
12.));
#135910=CARTESIAN_POINT('Ctrl Pts',(-37.0301387221774,-61.3521028132003,
12.));
#135911=CARTESIAN_POINT('Ctrl Pts',(-37.0481611121717,-61.3670207840068,
12.));
#135912=CARTESIAN_POINT('Ctrl Pts',(-37.0662319542849,-61.381948774749,
12.));
#135913=CARTESIAN_POINT('Ctrl Pts',(-37.0843511916745,-61.3968866552317,
12.));
#135914=CARTESIAN_POINT('Ctrl Pts',(-37.1025187676602,-61.4118342958697,
12.));
#135915=CARTESIAN_POINT('Ctrl Pts',(-37.1207346257222,-61.4267915676822,
12.));
#135916=CARTESIAN_POINT('Ctrl Pts',(-37.1389987094905,-61.4417583422863,
12.));
#135917=CARTESIAN_POINT('Ctrl Pts',(-37.1573109627454,-61.4567344918919,
12.));
#135918=CARTESIAN_POINT('Ctrl Pts',(-37.175671329424,-61.4717198892994,
12.));
#135919=CARTESIAN_POINT('Ctrl Pts',(-37.1940797536181,-61.4867144078936,
12.));
#135920=CARTESIAN_POINT('Ctrl Pts',(-37.2125361795731,-61.501717921641,
12.));
#135921=CARTESIAN_POINT('Ctrl Pts',(-37.2310405516781,-61.5167303050832,
12.));
#135922=CARTESIAN_POINT('Ctrl Pts',(-37.2495928144667,-61.5317514333328,
12.));
#135923=CARTESIAN_POINT('Ctrl Pts',(-37.2681929126221,-61.5467811820691,
12.));
#135924=CARTESIAN_POINT('Ctrl Pts',(-37.2868407909771,-61.5618194275348,
12.));
#135925=CARTESIAN_POINT('Ctrl Pts',(-37.3055363945107,-61.5768660465311,
12.));
#135926=CARTESIAN_POINT('Ctrl Pts',(-37.3242796683395,-61.591920916412,
12.));
#135927=CARTESIAN_POINT('Ctrl Pts',(-37.343070557718,-61.6069839150807,
12.));
#135928=CARTESIAN_POINT('Ctrl Pts',(-37.361909008045,-61.6220549209866,
12.));
#135929=CARTESIAN_POINT('Ctrl Pts',(-37.3807949648624,-61.637133813121,
12.));
#135930=CARTESIAN_POINT('Ctrl Pts',(-37.3997283738533,-61.6522204710131,
12.));
#135931=CARTESIAN_POINT('Ctrl Pts',(-37.4187091808321,-61.6673147747242,
12.));
#135932=CARTESIAN_POINT('Ctrl Pts',(-37.4377373317451,-61.6824166048444,
12.));
#135933=CARTESIAN_POINT('Ctrl Pts',(-37.4568127726773,-61.6975258424894,
12.));
#135934=CARTESIAN_POINT('Ctrl Pts',(-37.4759354498509,-61.7126423692963,
12.));
#135935=CARTESIAN_POINT('Ctrl Pts',(-37.4951053096237,-61.7277660674205,
12.));
#135936=CARTESIAN_POINT('Ctrl Pts',(-37.5143222984796,-61.7428968195299,
12.));
#135937=CARTESIAN_POINT('Ctrl Pts',(-37.5335863630287,-61.7580345088016,
12.));
#135938=CARTESIAN_POINT('Ctrl Pts',(-37.5528974500142,-61.773179018919,
12.));
#135939=CARTESIAN_POINT('Ctrl Pts',(-37.5722555063111,-61.7883302340687,
12.));
#135940=CARTESIAN_POINT('Ctrl Pts',(-37.5916604789253,-61.8034880389362,
12.));
#135941=CARTESIAN_POINT('Ctrl Pts',(-37.6111123149839,-61.8186523187015,
12.));
#135942=CARTESIAN_POINT('Ctrl Pts',(-37.6306109617346,-61.8338229590352,
12.));
#135943=CARTESIAN_POINT('Ctrl Pts',(-37.6501563665523,-61.8489998460957,
12.));
#135944=CARTESIAN_POINT('Ctrl Pts',(-37.6697484769392,-61.8641828665261,
12.));
#135945=CARTESIAN_POINT('Ctrl Pts',(-37.6893872405228,-61.8793719074507,
12.));
#135946=CARTESIAN_POINT('Ctrl Pts',(-37.7090726050482,-61.8945668564704,
12.));
#135947=CARTESIAN_POINT('Ctrl Pts',(-37.7288045183756,-61.9097676016601,
12.));
#135948=CARTESIAN_POINT('Ctrl Pts',(-37.7485829284871,-61.9249740315649,
12.));
#135949=CARTESIAN_POINT('Ctrl Pts',(-37.7684077834872,-61.9401860351972,
12.));
#135950=CARTESIAN_POINT('Ctrl Pts',(-37.7882790316014,-61.9554035020338,
12.));
#135951=CARTESIAN_POINT('Ctrl Pts',(-37.8081966211689,-61.9706263220114,
12.));
#135952=CARTESIAN_POINT('Ctrl Pts',(-37.828160500638,-61.9858543855236,
12.));
#135953=CARTESIAN_POINT('Ctrl Pts',(-37.8481706185749,-62.0010875834187,
12.));
#135954=CARTESIAN_POINT('Ctrl Pts',(-37.868226923663,-62.0163258069957,
12.));
#135955=CARTESIAN_POINT('Ctrl Pts',(-37.8883293647029,-62.031568948002,
12.));
#135956=CARTESIAN_POINT('Ctrl Pts',(-37.9084778906053,-62.0468168986288,
12.));
#135957=CARTESIAN_POINT('Ctrl Pts',(-37.9286724503851,-62.0620695515074,
12.));
#135958=CARTESIAN_POINT('Ctrl Pts',(-37.9489129931689,-62.0773267997078,
12.));
#135959=CARTESIAN_POINT('Ctrl Pts',(-37.9691994681966,-62.0925885367352,
12.));
#135960=CARTESIAN_POINT('Ctrl Pts',(-37.9895318248212,-62.107854656528,
12.));
#135961=CARTESIAN_POINT('Ctrl Pts',(-38.0099100125037,-62.123125053455,
12.));
#135962=CARTESIAN_POINT('Ctrl Pts',(-38.0303339808053,-62.1383996223124,
12.));
#135963=CARTESIAN_POINT('Ctrl Pts',(-38.0508036793939,-62.1536782583199,
12.));
#135964=CARTESIAN_POINT('Ctrl Pts',(-38.0713190580463,-62.1689608571176,
12.));
#135965=CARTESIAN_POINT('Ctrl Pts',(-38.0918800666479,-62.1842473147626,
12.));
#135966=CARTESIAN_POINT('Ctrl Pts',(-38.1124866551886,-62.1995375277257,
12.));
#135967=CARTESIAN_POINT('Ctrl Pts',(-38.133138773753,-62.2148313928863,
12.));
#135968=CARTESIAN_POINT('Ctrl Pts',(-38.1538363725264,-62.2301288075321,
12.));
#135969=CARTESIAN_POINT('Ctrl Pts',(-38.1745794017996,-62.245429669358,
12.));
#135970=CARTESIAN_POINT('Ctrl Pts',(-38.1953678119691,-62.2607338764654,
12.));
#135971=CARTESIAN_POINT('Ctrl Pts',(-38.2162015535353,-62.2760413273602,
12.));
#135972=CARTESIAN_POINT('Ctrl Pts',(-38.2370805770935,-62.2913519209521,
12.));
#135973=CARTESIAN_POINT('Ctrl Pts',(-38.2580048333361,-62.3066655565503,
12.));
#135974=CARTESIAN_POINT('Ctrl Pts',(-38.2789742730564,-62.3219821338569,
12.));
#135975=CARTESIAN_POINT('Ctrl Pts',(-38.2999888471476,-62.3373015529613,
12.));
#135976=CARTESIAN_POINT('Ctrl Pts',(-38.3210485066001,-62.3526237143336,
12.));
#135977=CARTESIAN_POINT('Ctrl Pts',(-38.342153202491,-62.3679485188171,
12.));
#135978=CARTESIAN_POINT('Ctrl Pts',(-38.3633028859828,-62.3832758676271,
12.));
#135979=CARTESIAN_POINT('Ctrl Pts',(-38.3844975083343,-62.3986056623577,
12.));
#135980=CARTESIAN_POINT('Ctrl Pts',(-38.405737020905,-62.4139378049885,
12.));
#135981=CARTESIAN_POINT('Ctrl Pts',(-38.4270213751568,-62.4292721978901,
12.));
#135982=CARTESIAN_POINT('Ctrl Pts',(-38.4483505226518,-62.4446087438312,
12.));
#135983=CARTESIAN_POINT('Ctrl Pts',(-38.4697244150482,-62.4599473459811,
12.));
#135984=CARTESIAN_POINT('Ctrl Pts',(-38.4911430040997,-62.4752879078854,
12.));
#135985=CARTESIAN_POINT('Ctrl Pts',(-38.5126062416502,-62.4906303334443,
12.));
#135986=CARTESIAN_POINT('Ctrl Pts',(-38.5341140796248,-62.5059745268901,
12.));
#135987=CARTESIAN_POINT('Ctrl Pts',(-38.5556664700195,-62.5213203927663,
12.));
#135988=CARTESIAN_POINT('Ctrl Pts',(-38.5772633648832,-62.5366678359023,
12.));
#135989=CARTESIAN_POINT('Ctrl Pts',(-38.5989047163393,-62.5520167614516,
12.));
#135990=CARTESIAN_POINT('Ctrl Pts',(-38.6205904766073,-62.5673670749361,
12.));
#135991=CARTESIAN_POINT('Ctrl Pts',(-38.6423205980213,-62.582718682292,
12.));
#135992=CARTESIAN_POINT('Ctrl Pts',(-38.6640950330421,-62.5980714899052,
12.));
#135993=CARTESIAN_POINT('Ctrl Pts',(-38.6859137342731,-62.6134254046739,
12.));
#135994=CARTESIAN_POINT('Ctrl Pts',(-38.7077766544416,-62.6287803339542,
12.));
#135995=CARTESIAN_POINT('Ctrl Pts',(-38.7296837463609,-62.6441361854411,
12.));
#135996=CARTESIAN_POINT('Ctrl Pts',(-38.7516349628904,-62.6594928670628,
12.));
#135997=CARTESIAN_POINT('Ctrl Pts',(-38.7736302568982,-62.6748502868835,
12.));
#135998=CARTESIAN_POINT('Ctrl Pts',(-38.795669581203,-62.6902083529694,
12.));
#135999=CARTESIAN_POINT('Ctrl Pts',(-38.8177528885681,-62.7055669733802,
12.));
#136000=CARTESIAN_POINT('Ctrl Pts',(-38.8398801318177,-62.7209260564493,
12.));
#136001=CARTESIAN_POINT('Ctrl Pts',(-38.8620512639233,-62.7362855110042,
12.));
#136002=CARTESIAN_POINT('Ctrl Pts',(-38.8842662380984,-62.7516452466128,
12.));
#136003=CARTESIAN_POINT('Ctrl Pts',(-38.9065250078832,-62.7670051738143,
12.));
#136004=CARTESIAN_POINT('Ctrl Pts',(-38.9288275272335,-62.78236520437,12.));
#136005=CARTESIAN_POINT('Ctrl Pts',(-38.9511737503165,-62.7977252507117,
12.));
#136006=CARTESIAN_POINT('Ctrl Pts',(-38.9735636313089,-62.8130852254027,
12.));
#136007=CARTESIAN_POINT('Ctrl Pts',(-38.9959971241701,-62.8284450405459,
12.));
#136008=CARTESIAN_POINT('Ctrl Pts',(-39.0184741824641,-62.8438046073224,
12.));
#136009=CARTESIAN_POINT('Ctrl Pts',(-39.0409947590497,-62.8591638352055,
12.));
#136010=CARTESIAN_POINT('Ctrl Pts',(-39.0635588063277,-62.8745226325998,
12.));
#136011=CARTESIAN_POINT('Ctrl Pts',(-39.0861662767932,-62.8898809082611,
12.));
#136012=CARTESIAN_POINT('Ctrl Pts',(-39.1088171235125,-62.9052385725387,
12.));
#136013=CARTESIAN_POINT('Ctrl Pts',(-39.131511300575,-62.9205955385558,
12.));
#136014=CARTESIAN_POINT('Ctrl Pts',(-39.1542487636744,-62.9359517237404,
12.));
#136015=CARTESIAN_POINT('Ctrl Pts',(-39.1770294702428,-62.9513070501867,
12.));
#136016=CARTESIAN_POINT('Ctrl Pts',(-39.1965939820934,-62.9644687386836,
12.));
#136017=CARTESIAN_POINT('Ctrl Pts',(-39.2116170128463,-62.9745590018674,
12.));
#136018=CARTESIAN_POINT('Ctrl Pts',(-39.222079438881,-62.9815782721328,
12.));
#136019=CARTESIAN_POINT('Ctrl Pts',(-39.2279686275011,-62.985526861613,
12.));
#136020=CARTESIAN_POINT('Ctrl Pts',(-39.2292784191818,-62.9864049293897,
12.));
#136021=CARTESIAN_POINT('',(-35.736831121751,-60.1903555511633,0.));
#136022=CARTESIAN_POINT('',(-35.736831121751,-60.1903555511633,0.));
#136023=CARTESIAN_POINT('Ctrl Pts',(-39.2292784191817,-62.9864049293896,
0.));
#136024=CARTESIAN_POINT('Ctrl Pts',(-39.227968627501,-62.985526861613,0.));
#136025=CARTESIAN_POINT('Ctrl Pts',(-39.2220794388809,-62.9815782721327,
0.));
#136026=CARTESIAN_POINT('Ctrl Pts',(-39.2116170128462,-62.9745590018674,
0.));
#136027=CARTESIAN_POINT('Ctrl Pts',(-39.1965939820934,-62.9644687386836,
0.));
#136028=CARTESIAN_POINT('Ctrl Pts',(-39.1770294702428,-62.9513070501867,
0.));
#136029=CARTESIAN_POINT('Ctrl Pts',(-39.1542487636744,-62.9359517237404,
0.));
#136030=CARTESIAN_POINT('Ctrl Pts',(-39.131511300575,-62.9205955385558,
0.));
#136031=CARTESIAN_POINT('Ctrl Pts',(-39.1088171235125,-62.9052385725387,
0.));
#136032=CARTESIAN_POINT('Ctrl Pts',(-39.0861662767932,-62.8898809082611,
0.));
#136033=CARTESIAN_POINT('Ctrl Pts',(-39.0635588063277,-62.8745226325998,
0.));
#136034=CARTESIAN_POINT('Ctrl Pts',(-39.0409947590497,-62.8591638352055,
0.));
#136035=CARTESIAN_POINT('Ctrl Pts',(-39.0184741824641,-62.8438046073224,
0.));
#136036=CARTESIAN_POINT('Ctrl Pts',(-38.9959971241701,-62.8284450405459,
0.));
#136037=CARTESIAN_POINT('Ctrl Pts',(-38.9735636313089,-62.8130852254027,
0.));
#136038=CARTESIAN_POINT('Ctrl Pts',(-38.9511737503165,-62.7977252507117,
0.));
#136039=CARTESIAN_POINT('Ctrl Pts',(-38.9288275272335,-62.78236520437,0.));
#136040=CARTESIAN_POINT('Ctrl Pts',(-38.9065250078832,-62.7670051738143,
0.));
#136041=CARTESIAN_POINT('Ctrl Pts',(-38.8842662380984,-62.7516452466128,
0.));
#136042=CARTESIAN_POINT('Ctrl Pts',(-38.8620512639233,-62.7362855110042,
0.));
#136043=CARTESIAN_POINT('Ctrl Pts',(-38.8398801318177,-62.7209260564493,
0.));
#136044=CARTESIAN_POINT('Ctrl Pts',(-38.8177528885681,-62.7055669733802,
0.));
#136045=CARTESIAN_POINT('Ctrl Pts',(-38.795669581203,-62.6902083529694,
0.));
#136046=CARTESIAN_POINT('Ctrl Pts',(-38.7736302568982,-62.6748502868835,
0.));
#136047=CARTESIAN_POINT('Ctrl Pts',(-38.7516349628904,-62.6594928670628,
0.));
#136048=CARTESIAN_POINT('Ctrl Pts',(-38.7296837463609,-62.6441361854411,
0.));
#136049=CARTESIAN_POINT('Ctrl Pts',(-38.7077766544416,-62.6287803339542,
0.));
#136050=CARTESIAN_POINT('Ctrl Pts',(-38.6859137342731,-62.6134254046739,
0.));
#136051=CARTESIAN_POINT('Ctrl Pts',(-38.6640950330421,-62.5980714899052,
0.));
#136052=CARTESIAN_POINT('Ctrl Pts',(-38.6423205980213,-62.582718682292,
0.));
#136053=CARTESIAN_POINT('Ctrl Pts',(-38.6205904766073,-62.5673670749361,
0.));
#136054=CARTESIAN_POINT('Ctrl Pts',(-38.5989047163393,-62.5520167614516,
0.));
#136055=CARTESIAN_POINT('Ctrl Pts',(-38.5772633648832,-62.5366678359023,
0.));
#136056=CARTESIAN_POINT('Ctrl Pts',(-38.5556664700195,-62.5213203927663,
0.));
#136057=CARTESIAN_POINT('Ctrl Pts',(-38.5341140796248,-62.5059745268901,
0.));
#136058=CARTESIAN_POINT('Ctrl Pts',(-38.5126062416502,-62.4906303334443,
0.));
#136059=CARTESIAN_POINT('Ctrl Pts',(-38.4911430040997,-62.4752879078854,
0.));
#136060=CARTESIAN_POINT('Ctrl Pts',(-38.4697244150482,-62.4599473459811,
0.));
#136061=CARTESIAN_POINT('Ctrl Pts',(-38.4483505226518,-62.4446087438312,
0.));
#136062=CARTESIAN_POINT('Ctrl Pts',(-38.4270213751568,-62.4292721978901,
0.));
#136063=CARTESIAN_POINT('Ctrl Pts',(-38.405737020905,-62.4139378049885,
0.));
#136064=CARTESIAN_POINT('Ctrl Pts',(-38.3844975083343,-62.3986056623577,
0.));
#136065=CARTESIAN_POINT('Ctrl Pts',(-38.3633028859828,-62.3832758676271,
0.));
#136066=CARTESIAN_POINT('Ctrl Pts',(-38.342153202491,-62.3679485188171,
0.));
#136067=CARTESIAN_POINT('Ctrl Pts',(-38.3210485066001,-62.3526237143336,
0.));
#136068=CARTESIAN_POINT('Ctrl Pts',(-38.2999888471476,-62.3373015529613,
0.));
#136069=CARTESIAN_POINT('Ctrl Pts',(-38.2789742730564,-62.3219821338569,
0.));
#136070=CARTESIAN_POINT('Ctrl Pts',(-38.2580048333361,-62.3066655565503,
0.));
#136071=CARTESIAN_POINT('Ctrl Pts',(-38.2370805770935,-62.2913519209521,
0.));
#136072=CARTESIAN_POINT('Ctrl Pts',(-38.2162015535353,-62.2760413273602,
0.));
#136073=CARTESIAN_POINT('Ctrl Pts',(-38.1953678119691,-62.2607338764654,
0.));
#136074=CARTESIAN_POINT('Ctrl Pts',(-38.1745794017996,-62.245429669358,
0.));
#136075=CARTESIAN_POINT('Ctrl Pts',(-38.1538363725264,-62.2301288075321,
0.));
#136076=CARTESIAN_POINT('Ctrl Pts',(-38.133138773753,-62.2148313928863,
0.));
#136077=CARTESIAN_POINT('Ctrl Pts',(-38.1124866551886,-62.1995375277257,
0.));
#136078=CARTESIAN_POINT('Ctrl Pts',(-38.0918800666479,-62.1842473147626,
0.));
#136079=CARTESIAN_POINT('Ctrl Pts',(-38.0713190580463,-62.1689608571176,
0.));
#136080=CARTESIAN_POINT('Ctrl Pts',(-38.0508036793939,-62.1536782583199,
0.));
#136081=CARTESIAN_POINT('Ctrl Pts',(-38.0303339808053,-62.1383996223124,
0.));
#136082=CARTESIAN_POINT('Ctrl Pts',(-38.0099100125037,-62.123125053455,
0.));
#136083=CARTESIAN_POINT('Ctrl Pts',(-37.9895318248212,-62.107854656528,
0.));
#136084=CARTESIAN_POINT('Ctrl Pts',(-37.9691994681966,-62.0925885367352,
0.));
#136085=CARTESIAN_POINT('Ctrl Pts',(-37.9489129931689,-62.0773267997078,
0.));
#136086=CARTESIAN_POINT('Ctrl Pts',(-37.9286724503851,-62.0620695515074,
0.));
#136087=CARTESIAN_POINT('Ctrl Pts',(-37.9084778906053,-62.0468168986288,
0.));
#136088=CARTESIAN_POINT('Ctrl Pts',(-37.8883293647029,-62.031568948002,
0.));
#136089=CARTESIAN_POINT('Ctrl Pts',(-37.868226923663,-62.0163258069957,
0.));
#136090=CARTESIAN_POINT('Ctrl Pts',(-37.8481706185749,-62.0010875834187,
0.));
#136091=CARTESIAN_POINT('Ctrl Pts',(-37.828160500638,-61.9858543855236,
0.));
#136092=CARTESIAN_POINT('Ctrl Pts',(-37.8081966211689,-61.9706263220114,
0.));
#136093=CARTESIAN_POINT('Ctrl Pts',(-37.7882790316014,-61.9554035020338,
0.));
#136094=CARTESIAN_POINT('Ctrl Pts',(-37.7684077834872,-61.9401860351972,
0.));
#136095=CARTESIAN_POINT('Ctrl Pts',(-37.7485829284871,-61.9249740315649,
0.));
#136096=CARTESIAN_POINT('Ctrl Pts',(-37.7288045183756,-61.9097676016601,
0.));
#136097=CARTESIAN_POINT('Ctrl Pts',(-37.7090726050482,-61.8945668564704,
0.));
#136098=CARTESIAN_POINT('Ctrl Pts',(-37.6893872405228,-61.8793719074507,
0.));
#136099=CARTESIAN_POINT('Ctrl Pts',(-37.6697484769392,-61.8641828665261,
0.));
#136100=CARTESIAN_POINT('Ctrl Pts',(-37.6501563665523,-61.8489998460957,
0.));
#136101=CARTESIAN_POINT('Ctrl Pts',(-37.6306109617346,-61.8338229590352,
0.));
#136102=CARTESIAN_POINT('Ctrl Pts',(-37.6111123149839,-61.8186523187015,
0.));
#136103=CARTESIAN_POINT('Ctrl Pts',(-37.5916604789253,-61.8034880389362,
0.));
#136104=CARTESIAN_POINT('Ctrl Pts',(-37.5722555063111,-61.7883302340687,
0.));
#136105=CARTESIAN_POINT('Ctrl Pts',(-37.5528974500142,-61.773179018919,
0.));
#136106=CARTESIAN_POINT('Ctrl Pts',(-37.5335863630287,-61.7580345088016,
0.));
#136107=CARTESIAN_POINT('Ctrl Pts',(-37.5143222984796,-61.7428968195299,
0.));
#136108=CARTESIAN_POINT('Ctrl Pts',(-37.4951053096237,-61.7277660674205,
0.));
#136109=CARTESIAN_POINT('Ctrl Pts',(-37.4759354498509,-61.7126423692963,
0.));
#136110=CARTESIAN_POINT('Ctrl Pts',(-37.4568127726773,-61.6975258424894,
0.));
#136111=CARTESIAN_POINT('Ctrl Pts',(-37.4377373317451,-61.6824166048444,
0.));
#136112=CARTESIAN_POINT('Ctrl Pts',(-37.4187091808321,-61.6673147747242,
0.));
#136113=CARTESIAN_POINT('Ctrl Pts',(-37.3997283738533,-61.6522204710131,
0.));
#136114=CARTESIAN_POINT('Ctrl Pts',(-37.3807949648624,-61.637133813121,
0.));
#136115=CARTESIAN_POINT('Ctrl Pts',(-37.361909008045,-61.6220549209866,
0.));
#136116=CARTESIAN_POINT('Ctrl Pts',(-37.343070557718,-61.6069839150807,
0.));
#136117=CARTESIAN_POINT('Ctrl Pts',(-37.3242796683395,-61.591920916412,
0.));
#136118=CARTESIAN_POINT('Ctrl Pts',(-37.3055363945107,-61.5768660465311,
0.));
#136119=CARTESIAN_POINT('Ctrl Pts',(-37.2868407909771,-61.5618194275348,
0.));
#136120=CARTESIAN_POINT('Ctrl Pts',(-37.2681929126221,-61.5467811820691,
0.));
#136121=CARTESIAN_POINT('Ctrl Pts',(-37.2495928144667,-61.5317514333328,
0.));
#136122=CARTESIAN_POINT('Ctrl Pts',(-37.2310405516781,-61.5167303050832,
0.));
#136123=CARTESIAN_POINT('Ctrl Pts',(-37.2125361795731,-61.501717921641,
0.));
#136124=CARTESIAN_POINT('Ctrl Pts',(-37.1940797536181,-61.4867144078936,
0.));
#136125=CARTESIAN_POINT('Ctrl Pts',(-37.175671329424,-61.4717198892994,
0.));
#136126=CARTESIAN_POINT('Ctrl Pts',(-37.1573109627454,-61.4567344918919,
0.));
#136127=CARTESIAN_POINT('Ctrl Pts',(-37.1389987094905,-61.4417583422863,
0.));
#136128=CARTESIAN_POINT('Ctrl Pts',(-37.1207346257222,-61.4267915676822,
0.));
#136129=CARTESIAN_POINT('Ctrl Pts',(-37.1025187676602,-61.4118342958697,
0.));
#136130=CARTESIAN_POINT('Ctrl Pts',(-37.0843511916745,-61.3968866552317,
0.));
#136131=CARTESIAN_POINT('Ctrl Pts',(-37.0662319542849,-61.381948774749,
0.));
#136132=CARTESIAN_POINT('Ctrl Pts',(-37.0481611121717,-61.3670207840068,
0.));
#136133=CARTESIAN_POINT('Ctrl Pts',(-37.0301387221774,-61.3521028132003,
0.));
#136134=CARTESIAN_POINT('Ctrl Pts',(-37.0121648413082,-61.3371949931387,
0.));
#136135=CARTESIAN_POINT('Ctrl Pts',(-36.994239526727,-61.3222974552486,
0.));
#136136=CARTESIAN_POINT('Ctrl Pts',(-36.9763628357544,-61.3074103315791,
0.));
#136137=CARTESIAN_POINT('Ctrl Pts',(-36.9585348258776,-61.2925337548077,
0.));
#136138=CARTESIAN_POINT('Ctrl Pts',(-36.9407555547535,-61.2776678582461,
0.));
#136139=CARTESIAN_POINT('Ctrl Pts',(-36.9230250802087,-61.2628127758457,
0.));
#136140=CARTESIAN_POINT('Ctrl Pts',(-36.9053434602343,-61.247968642201,
0.));
#136141=CARTESIAN_POINT('Ctrl Pts',(-36.8877107529865,-61.2331355925547,
0.));
#136142=CARTESIAN_POINT('Ctrl Pts',(-36.8701270167969,-61.2183137628056,
0.));
#136143=CARTESIAN_POINT('Ctrl Pts',(-36.852592310174,-61.2035032895127,
0.));
#136144=CARTESIAN_POINT('Ctrl Pts',(-36.8351066918036,-61.1887043099014,
0.));
#136145=CARTESIAN_POINT('Ctrl Pts',(-36.8176702205423,-61.1739169618666,
0.));
#136146=CARTESIAN_POINT('Ctrl Pts',(-36.8002829554209,-61.1591413839787,
0.));
#136147=CARTESIAN_POINT('Ctrl Pts',(-36.7829449556532,-61.1443777154911,
0.));
#136148=CARTESIAN_POINT('Ctrl Pts',(-36.765656280638,-61.1296260963466,
0.));
#136149=CARTESIAN_POINT('Ctrl Pts',(-36.7484169899596,-61.1148866671829,
0.));
#136150=CARTESIAN_POINT('Ctrl Pts',(-36.7312271433807,-61.100159569337,
0.));
#136151=CARTESIAN_POINT('Ctrl Pts',(-36.7140868008486,-61.0854449448524,
0.));
#136152=CARTESIAN_POINT('Ctrl Pts',(-36.6969960225022,-61.0707429364847,
0.));
#136153=CARTESIAN_POINT('Ctrl Pts',(-36.679954868674,-61.0560536877083,
0.));
#136154=CARTESIAN_POINT('Ctrl Pts',(-36.6629633998886,-61.0413773427203,
0.));
#136155=CARTESIAN_POINT('Ctrl Pts',(-36.6460216768553,-61.0267140464432,
0.));
#136156=CARTESIAN_POINT('Ctrl Pts',(-36.6291297604776,-61.0120639445349,
0.));
#136157=CARTESIAN_POINT('Ctrl Pts',(-36.61228771186,-60.9974271833981,0.));
#136158=CARTESIAN_POINT('Ctrl Pts',(-36.595495592311,-60.9828039101887,
0.));
#136159=CARTESIAN_POINT('Ctrl Pts',(-36.5787534633416,-60.9681942728236,
0.));
#136160=CARTESIAN_POINT('Ctrl Pts',(-36.5620613866615,-60.9535984199873,
0.));
#136161=CARTESIAN_POINT('Ctrl Pts',(-36.5454194241865,-60.9390165011355,
0.));
#136162=CARTESIAN_POINT('Ctrl Pts',(-36.5288276380416,-60.9244486664987,
0.));
#136163=CARTESIAN_POINT('Ctrl Pts',(-36.5122860905612,-60.9098950670847,
0.));
#136164=CARTESIAN_POINT('Ctrl Pts',(-36.4957948442835,-60.8953558546795,
0.));
#136165=CARTESIAN_POINT('Ctrl Pts',(-36.4793539619466,-60.8808311818499,
0.));
#136166=CARTESIAN_POINT('Ctrl Pts',(-36.4629635065045,-60.8663212019657,
0.));
#136167=CARTESIAN_POINT('Ctrl Pts',(-36.4466235411358,-60.8518260692188,
0.));
#136168=CARTESIAN_POINT('Ctrl Pts',(-36.4303341292494,-60.8373459386392,
0.));
#136169=CARTESIAN_POINT('Ctrl Pts',(-36.4140953344858,-60.822880966116,
0.));
#136170=CARTESIAN_POINT('Ctrl Pts',(-36.397907220716,-60.8084313083984,
0.));
#136171=CARTESIAN_POINT('Ctrl Pts',(-36.3817698520388,-60.793997123076,
0.));
#136172=CARTESIAN_POINT('Ctrl Pts',(-36.365683292773,-60.7795785685625,
0.));
#136173=CARTESIAN_POINT('Ctrl Pts',(-36.3496476074488,-60.7651758040803,
0.));
#136174=CARTESIAN_POINT('Ctrl Pts',(-36.3336628607859,-60.7507889896308,
0.));
#136175=CARTESIAN_POINT('Ctrl Pts',(-36.3177291177163,-60.7364182860412,
0.));
#136176=CARTESIAN_POINT('Ctrl Pts',(-36.3018464434214,-60.722063855041,
0.));
#136177=CARTESIAN_POINT('Ctrl Pts',(-36.2860149033587,-60.7077258593268,
0.));
#136178=CARTESIAN_POINT('Ctrl Pts',(-36.2702345632875,-60.6934044626291,
0.));
#136179=CARTESIAN_POINT('Ctrl Pts',(-36.2545054892897,-60.67909982978,0.));
#136180=CARTESIAN_POINT('Ctrl Pts',(-36.2388277477212,-60.6648121265885,
0.));
#136181=CARTESIAN_POINT('Ctrl Pts',(-36.2232014051541,-60.6505415197042,
0.));
#136182=CARTESIAN_POINT('Ctrl Pts',(-36.2076265283264,-60.6362881765019,
0.));
#136183=CARTESIAN_POINT('Ctrl Pts',(-36.192103184063,-60.6220522649149,
0.));
#136184=CARTESIAN_POINT('Ctrl Pts',(-36.1766314392641,-60.6078339534181,
0.));
#136185=CARTESIAN_POINT('Ctrl Pts',(-36.1612113610773,-60.5936334114108,
0.));
#136186=CARTESIAN_POINT('Ctrl Pts',(-36.1458430170431,-60.5794508095564,
0.));
#136187=CARTESIAN_POINT('Ctrl Pts',(-36.1305264752188,-60.565286320072,
0.));
#136188=CARTESIAN_POINT('Ctrl Pts',(-36.1152618043739,-60.5511401171984,
0.));
#136189=CARTESIAN_POINT('Ctrl Pts',(-36.100049073851,-60.5370123768804,
0.));
#136190=CARTESIAN_POINT('Ctrl Pts',(-36.0848883531952,-60.5229032758973,
0.));
#136191=CARTESIAN_POINT('Ctrl Pts',(-36.0697797118376,-60.5088129911354,
0.));
#136192=CARTESIAN_POINT('Ctrl Pts',(-36.0547232187698,-60.4947416988422,
0.));
#136193=CARTESIAN_POINT('Ctrl Pts',(-36.0397189421644,-60.4806895737686,
0.));
#136194=CARTESIAN_POINT('Ctrl Pts',(-36.0247669500891,-60.4666567908093,
0.));
#136195=CARTESIAN_POINT('Ctrl Pts',(-36.009867311357,-60.4526435269662,
0.));
#136196=CARTESIAN_POINT('Ctrl Pts',(-35.995020096217,-60.4386499629481,
0.));
#136197=CARTESIAN_POINT('Ctrl Pts',(-35.9802253773515,-60.4246762854926,
0.));
#136198=CARTESIAN_POINT('Ctrl Pts',(-35.9654832299601,-60.4107226875714,
0.));
#136199=CARTESIAN_POINT('Ctrl Pts',(-35.9507937296707,-60.3967893635452,
0.));
#136200=CARTESIAN_POINT('Ctrl Pts',(-35.936156950695,-60.3828765049019,
0.));
#136201=CARTESIAN_POINT('Ctrl Pts',(-35.9215729642231,-60.3689842965481,
0.));
#136202=CARTESIAN_POINT('Ctrl Pts',(-35.907041835853,-60.3551129108845,
0.));
#136203=CARTESIAN_POINT('Ctrl Pts',(-35.8925636280668,-60.3412625135287,
0.));
#136204=CARTESIAN_POINT('Ctrl Pts',(-35.8781384051537,-60.327433274683,
0.));
#136205=CARTESIAN_POINT('Ctrl Pts',(-35.8637662371635,-60.3136253782809,
0.));
#136206=CARTESIAN_POINT('Ctrl Pts',(-35.8494472046745,-60.2998390330102,
0.));
#136207=CARTESIAN_POINT('Ctrl Pts',(-35.8351814020357,-60.2860744798436,
0.));
#136208=CARTESIAN_POINT('Ctrl Pts',(-35.8209689272501,-60.2723319687369,
0.));
#136209=CARTESIAN_POINT('Ctrl Pts',(-35.8068098723347,-60.2586117365205,
0.));
#136210=CARTESIAN_POINT('Ctrl Pts',(-35.7927043145201,-60.2449139865274,
0.));
#136211=CARTESIAN_POINT('Ctrl Pts',(-35.7786523045912,-60.2312388621529,
0.));
#136212=CARTESIAN_POINT('Ctrl Pts',(-35.7646538667493,-60.2175864450043,
0.));
#136213=CARTESIAN_POINT('Ctrl Pts',(-35.7534979802053,-60.206682708692,
0.));
#136214=CARTESIAN_POINT('Ctrl Pts',(-35.7451551752572,-60.1985151474623,
0.));
#136215=CARTESIAN_POINT('Ctrl Pts',(-35.7396040204017,-60.193074658032,
0.));
#136216=CARTESIAN_POINT('Ctrl Pts',(-35.736831121751,-60.1903555511633,
0.));
#136217=CARTESIAN_POINT('Ctrl Pts',(-44.8554660179045,-59.483083043136,
0.));
#136218=CARTESIAN_POINT('Ctrl Pts',(-44.8554660179045,-59.483083043136,
12.));
#136219=CARTESIAN_POINT('Ctrl Pts',(-44.8505359826461,-59.4804358983083,
0.));
#136220=CARTESIAN_POINT('Ctrl Pts',(-44.8505359826461,-59.4804358983083,
12.));
#136221=CARTESIAN_POINT('Ctrl Pts',(-44.8406801497742,-59.4751410547732,
0.));
#136222=CARTESIAN_POINT('Ctrl Pts',(-44.8406801497742,-59.4751410547732,
12.));
#136223=CARTESIAN_POINT('Ctrl Pts',(-44.8259091134016,-59.4671971278321,
0.));
#136224=CARTESIAN_POINT('Ctrl Pts',(-44.8259091134016,-59.4671971278321,
12.));
#136225=CARTESIAN_POINT('Ctrl Pts',(-44.8062398251406,-59.4566019018254,
0.));
#136226=CARTESIAN_POINT('Ctrl Pts',(-44.8062398251406,-59.4566019018254,
12.));
#136227=CARTESIAN_POINT('Ctrl Pts',(-44.7816956017528,-59.4433523335147,
0.));
#136228=CARTESIAN_POINT('Ctrl Pts',(-44.7816956017528,-59.4433523335147,
12.));
#136229=CARTESIAN_POINT('Ctrl Pts',(-44.7571937812113,-59.430097240324,
0.));
#136230=CARTESIAN_POINT('Ctrl Pts',(-44.7571937812113,-59.430097240324,
12.));
#136231=CARTESIAN_POINT('Ctrl Pts',(-44.7327343876391,-59.4168366453118,
0.));
#136232=CARTESIAN_POINT('Ctrl Pts',(-44.7327343876391,-59.4168366453118,
12.));
#136233=CARTESIAN_POINT('Ctrl Pts',(-44.7083174541702,-59.4035705873811,
0.));
#136234=CARTESIAN_POINT('Ctrl Pts',(-44.7083174541702,-59.4035705873811,
12.));
#136235=CARTESIAN_POINT('Ctrl Pts',(-44.683943024421,-59.3902991267889,
0.));
#136236=CARTESIAN_POINT('Ctrl Pts',(-44.683943024421,-59.3902991267889,
12.));
#136237=CARTESIAN_POINT('Ctrl Pts',(-44.6596111512687,-59.377022343519,
0.));
#136238=CARTESIAN_POINT('Ctrl Pts',(-44.6596111512687,-59.377022343519,
12.));
#136239=CARTESIAN_POINT('Ctrl Pts',(-44.6353218935685,-59.3637403301801,
0.));
#136240=CARTESIAN_POINT('Ctrl Pts',(-44.6353218935685,-59.3637403301801,
12.));
#136241=CARTESIAN_POINT('Ctrl Pts',(-44.6110753134277,-59.3504531864154,
0.));
#136242=CARTESIAN_POINT('Ctrl Pts',(-44.6110753134277,-59.3504531864154,
12.));
#136243=CARTESIAN_POINT('Ctrl Pts',(-44.5868714733234,-59.3371610128511,
0.));
#136244=CARTESIAN_POINT('Ctrl Pts',(-44.5868714733234,-59.3371610128511,
12.));
#136245=CARTESIAN_POINT('Ctrl Pts',(-44.5627104331017,-59.3238639048694,
0.));
#136246=CARTESIAN_POINT('Ctrl Pts',(-44.5627104331017,-59.3238639048694,
12.));
#136247=CARTESIAN_POINT('Ctrl Pts',(-44.5385922475573,-59.3105619475609,
0.));
#136248=CARTESIAN_POINT('Ctrl Pts',(-44.5385922475573,-59.3105619475609,
12.));
#136249=CARTESIAN_POINT('Ctrl Pts',(-44.5145169681349,-59.2972552192156,
0.));
#136250=CARTESIAN_POINT('Ctrl Pts',(-44.5145169681349,-59.2972552192156,
12.));
#136251=CARTESIAN_POINT('Ctrl Pts',(-44.490484644151,-59.2839437938237,
0.));
#136252=CARTESIAN_POINT('Ctrl Pts',(-44.490484644151,-59.2839437938237,
12.));
#136253=CARTESIAN_POINT('Ctrl Pts',(-44.4664953242379,-59.2706277440445,
0.));
#136254=CARTESIAN_POINT('Ctrl Pts',(-44.4664953242379,-59.2706277440445,
12.));
#136255=CARTESIAN_POINT('Ctrl Pts',(-44.4425490575911,-59.2573071437774,
0.));
#136256=CARTESIAN_POINT('Ctrl Pts',(-44.4425490575911,-59.2573071437774,
12.));
#136257=CARTESIAN_POINT('Ctrl Pts',(-44.4186458955451,-59.2439820714187,
0.));
#136258=CARTESIAN_POINT('Ctrl Pts',(-44.4186458955451,-59.2439820714187,
12.));
#136259=CARTESIAN_POINT('Ctrl Pts',(-44.3947858914074,-59.2306526095131,
0.));
#136260=CARTESIAN_POINT('Ctrl Pts',(-44.3947858914074,-59.2306526095131,
12.));
#136261=CARTESIAN_POINT('Ctrl Pts',(-44.3709690997469,-59.2173188432798,
0.));
#136262=CARTESIAN_POINT('Ctrl Pts',(-44.3709690997469,-59.2173188432798,
12.));
#136263=CARTESIAN_POINT('Ctrl Pts',(-44.3471955758403,-59.2039808594752,
0.));
#136264=CARTESIAN_POINT('Ctrl Pts',(-44.3471955758403,-59.2039808594752,
12.));
#136265=CARTESIAN_POINT('Ctrl Pts',(-44.3234653750884,-59.1906387451979,
0.));
#136266=CARTESIAN_POINT('Ctrl Pts',(-44.3234653750884,-59.1906387451979,
12.));
#136267=CARTESIAN_POINT('Ctrl Pts',(-44.2997785523431,-59.1772925865213,
0.));
#136268=CARTESIAN_POINT('Ctrl Pts',(-44.2997785523431,-59.1772925865213,
12.));
#136269=CARTESIAN_POINT('Ctrl Pts',(-44.2761351616048,-59.1639424678793,
0.));
#136270=CARTESIAN_POINT('Ctrl Pts',(-44.2761351616048,-59.1639424678793,
12.));
#136271=CARTESIAN_POINT('Ctrl Pts',(-44.2525352563996,-59.1505884728215,
0.));
#136272=CARTESIAN_POINT('Ctrl Pts',(-44.2525352563996,-59.1505884728215,
12.));
#136273=CARTESIAN_POINT('Ctrl Pts',(-44.228978889997,-59.1372306844586,
0.));
#136274=CARTESIAN_POINT('Ctrl Pts',(-44.228978889997,-59.1372306844586,
12.));
#136275=CARTESIAN_POINT('Ctrl Pts',(-44.2054661156875,-59.1238691860306,
0.));
#136276=CARTESIAN_POINT('Ctrl Pts',(-44.2054661156875,-59.1238691860306,
12.));
#136277=CARTESIAN_POINT('Ctrl Pts',(-44.1819969870307,-59.1105040614276,
0.));
#136278=CARTESIAN_POINT('Ctrl Pts',(-44.1819969870307,-59.1105040614276,
12.));
#136279=CARTESIAN_POINT('Ctrl Pts',(-44.1585715581064,-59.0971353957206,
0.));
#136280=CARTESIAN_POINT('Ctrl Pts',(-44.1585715581064,-59.0971353957206,
12.));
#136281=CARTESIAN_POINT('Ctrl Pts',(-44.1351898834051,-59.08376327492,0.));
#136282=CARTESIAN_POINT('Ctrl Pts',(-44.1351898834051,-59.08376327492,12.));
#136283=CARTESIAN_POINT('Ctrl Pts',(-44.1118520177221,-59.0703877857526,
0.));
#136284=CARTESIAN_POINT('Ctrl Pts',(-44.1118520177221,-59.0703877857526,
12.));
#136285=CARTESIAN_POINT('Ctrl Pts',(-44.0885580160432,-59.0570090154243,
0.));
#136286=CARTESIAN_POINT('Ctrl Pts',(-44.0885580160432,-59.0570090154243,
12.));
#136287=CARTESIAN_POINT('Ctrl Pts',(-44.0653079334385,-59.0436270514087,
0.));
#136288=CARTESIAN_POINT('Ctrl Pts',(-44.0653079334385,-59.0436270514087,
12.));
#136289=CARTESIAN_POINT('Ctrl Pts',(-44.0421018249223,-59.0302419811777,
0.));
#136290=CARTESIAN_POINT('Ctrl Pts',(-44.0421018249223,-59.0302419811777,
12.));
#136291=CARTESIAN_POINT('Ctrl Pts',(-44.0189397454599,-59.0168538922095,
0.));
#136292=CARTESIAN_POINT('Ctrl Pts',(-44.0189397454599,-59.0168538922095,
12.));
#136293=CARTESIAN_POINT('Ctrl Pts',(-43.9958217500369,-59.0034628721168,
0.));
#136294=CARTESIAN_POINT('Ctrl Pts',(-43.9958217500369,-59.0034628721168,
12.));
#136295=CARTESIAN_POINT('Ctrl Pts',(-43.9727478937056,-58.9900690087408,
0.));
#136296=CARTESIAN_POINT('Ctrl Pts',(-43.9727478937056,-58.9900690087408,
12.));
#136297=CARTESIAN_POINT('Ctrl Pts',(-43.9497182316331,-58.9766723902529,
0.));
#136298=CARTESIAN_POINT('Ctrl Pts',(-43.9497182316331,-58.9766723902529,
12.));
#136299=CARTESIAN_POINT('Ctrl Pts',(-43.9267328191501,-58.9632731052696,
0.));
#136300=CARTESIAN_POINT('Ctrl Pts',(-43.9267328191501,-58.9632731052696,
12.));
#136301=CARTESIAN_POINT('Ctrl Pts',(-43.9037917117739,-58.9498712429054,
0.));
#136302=CARTESIAN_POINT('Ctrl Pts',(-43.9037917117739,-58.9498712429054,
12.));
#136303=CARTESIAN_POINT('Ctrl Pts',(-43.8808949651873,-58.936466892712,
0.));
#136304=CARTESIAN_POINT('Ctrl Pts',(-43.8808949651873,-58.936466892712,
12.));
#136305=CARTESIAN_POINT('Ctrl Pts',(-43.858042635223,-58.9230601446436,
0.));
#136306=CARTESIAN_POINT('Ctrl Pts',(-43.858042635223,-58.9230601446436,
12.));
#136307=CARTESIAN_POINT('Ctrl Pts',(-43.835234777842,-58.9096510890129,
0.));
#136308=CARTESIAN_POINT('Ctrl Pts',(-43.835234777842,-58.9096510890129,
12.));
#136309=CARTESIAN_POINT('Ctrl Pts',(-43.8124714491076,-58.8962398164493,
0.));
#136310=CARTESIAN_POINT('Ctrl Pts',(-43.8124714491076,-58.8962398164493,
12.));
#136311=CARTESIAN_POINT('Ctrl Pts',(-43.7897527051609,-58.8828264178621,
0.));
#136312=CARTESIAN_POINT('Ctrl Pts',(-43.7897527051609,-58.8828264178621,
12.));
#136313=CARTESIAN_POINT('Ctrl Pts',(-43.7670786022402,-58.8694109844648,
0.));
#136314=CARTESIAN_POINT('Ctrl Pts',(-43.7670786022402,-58.8694109844648,
12.));
#136315=CARTESIAN_POINT('Ctrl Pts',(-43.7444491966942,-58.855993607794,
0.));
#136316=CARTESIAN_POINT('Ctrl Pts',(-43.7444491966942,-58.855993607794,
12.));
#136317=CARTESIAN_POINT('Ctrl Pts',(-43.7218645449922,-58.8425743797326,
0.));
#136318=CARTESIAN_POINT('Ctrl Pts',(-43.7218645449922,-58.8425743797326,
12.));
#136319=CARTESIAN_POINT('Ctrl Pts',(-43.6993247037314,-58.8291533925293,
0.));
#136320=CARTESIAN_POINT('Ctrl Pts',(-43.6993247037314,-58.8291533925293,
12.));
#136321=CARTESIAN_POINT('Ctrl Pts',(-43.6768297296395,-58.8157307388238,
0.));
#136322=CARTESIAN_POINT('Ctrl Pts',(-43.6768297296395,-58.8157307388238,
12.));
#136323=CARTESIAN_POINT('Ctrl Pts',(-43.6543796795789,-58.8023065116436,
0.));
#136324=CARTESIAN_POINT('Ctrl Pts',(-43.6543796795789,-58.8023065116436,
12.));
#136325=CARTESIAN_POINT('Ctrl Pts',(-43.6319746105482,-58.788880804397,
0.));
#136326=CARTESIAN_POINT('Ctrl Pts',(-43.6319746105482,-58.788880804397,
12.));
#136327=CARTESIAN_POINT('Ctrl Pts',(-43.6096145796797,-58.775453710867,
0.));
#136328=CARTESIAN_POINT('Ctrl Pts',(-43.6096145796797,-58.775453710867,
12.));
#136329=CARTESIAN_POINT('Ctrl Pts',(-43.5872996442345,-58.7620253252062,
0.));
#136330=CARTESIAN_POINT('Ctrl Pts',(-43.5872996442345,-58.7620253252062,
12.));
#136331=CARTESIAN_POINT('Ctrl Pts',(-43.5650298615917,-58.74859574193,0.));
#136332=CARTESIAN_POINT('Ctrl Pts',(-43.5650298615917,-58.74859574193,12.));
#136333=CARTESIAN_POINT('Ctrl Pts',(-43.5428052892488,-58.735165055918,
0.));
#136334=CARTESIAN_POINT('Ctrl Pts',(-43.5428052892488,-58.735165055918,
12.));
#136335=CARTESIAN_POINT('Ctrl Pts',(-43.5206259848337,-58.7217333624209,
0.));
#136336=CARTESIAN_POINT('Ctrl Pts',(-43.5206259848337,-58.7217333624209,
12.));
#136337=CARTESIAN_POINT('Ctrl Pts',(-43.4984920061073,-58.7083007570661,
0.));
#136338=CARTESIAN_POINT('Ctrl Pts',(-43.4984920061073,-58.7083007570661,
12.));
#136339=CARTESIAN_POINT('Ctrl Pts',(-43.4764034109654,-58.6948673358638,
0.));
#136340=CARTESIAN_POINT('Ctrl Pts',(-43.4764034109654,-58.6948673358638,
12.));
#136341=CARTESIAN_POINT('Ctrl Pts',(-43.4543602574351,-58.6814331952138,
0.));
#136342=CARTESIAN_POINT('Ctrl Pts',(-43.4543602574351,-58.6814331952138,
12.));
#136343=CARTESIAN_POINT('Ctrl Pts',(-43.4323626036737,-58.6679984319097,
0.));
#136344=CARTESIAN_POINT('Ctrl Pts',(-43.4323626036737,-58.6679984319097,
12.));
#136345=CARTESIAN_POINT('Ctrl Pts',(-43.4104105079768,-58.6545631431393,
0.));
#136346=CARTESIAN_POINT('Ctrl Pts',(-43.4104105079768,-58.6545631431393,
12.));
#136347=CARTESIAN_POINT('Ctrl Pts',(-43.388504028781,-58.6411274264857,
0.));
#136348=CARTESIAN_POINT('Ctrl Pts',(-43.388504028781,-58.6411274264857,
12.));
#136349=CARTESIAN_POINT('Ctrl Pts',(-43.3666432246635,-58.627691379929,
0.));
#136350=CARTESIAN_POINT('Ctrl Pts',(-43.3666432246635,-58.627691379929,
12.));
#136351=CARTESIAN_POINT('Ctrl Pts',(-43.3448281543371,-58.6142551018467,
0.));
#136352=CARTESIAN_POINT('Ctrl Pts',(-43.3448281543371,-58.6142551018467,
12.));
#136353=CARTESIAN_POINT('Ctrl Pts',(-43.3230588766449,-58.6008186910156,
0.));
#136354=CARTESIAN_POINT('Ctrl Pts',(-43.3230588766449,-58.6008186910156,
12.));
#136355=CARTESIAN_POINT('Ctrl Pts',(-43.3013354505701,-58.5873822466152,
0.));
#136356=CARTESIAN_POINT('Ctrl Pts',(-43.3013354505701,-58.5873822466152,
12.));
#136357=CARTESIAN_POINT('Ctrl Pts',(-43.27965793524,-58.573945868231,0.));
#136358=CARTESIAN_POINT('Ctrl Pts',(-43.27965793524,-58.573945868231,12.));
#136359=CARTESIAN_POINT('Ctrl Pts',(-43.2580263899278,-58.5605096558578,
0.));
#136360=CARTESIAN_POINT('Ctrl Pts',(-43.2580263899278,-58.5605096558578,
12.));
#136361=CARTESIAN_POINT('Ctrl Pts',(-43.2364408740493,-58.5470737099032,
0.));
#136362=CARTESIAN_POINT('Ctrl Pts',(-43.2364408740493,-58.5470737099032,
12.));
#136363=CARTESIAN_POINT('Ctrl Pts',(-43.2149014471574,-58.5336381311917,
0.));
#136364=CARTESIAN_POINT('Ctrl Pts',(-43.2149014471574,-58.5336381311917,
12.));
#136365=CARTESIAN_POINT('Ctrl Pts',(-43.1934081689505,-58.5202030209669,
0.));
#136366=CARTESIAN_POINT('Ctrl Pts',(-43.1934081689505,-58.5202030209669,
12.));
#136367=CARTESIAN_POINT('Ctrl Pts',(-43.1719610992771,-58.5067684808944,
0.));
#136368=CARTESIAN_POINT('Ctrl Pts',(-43.1719610992771,-58.5067684808944,
12.));
#136369=CARTESIAN_POINT('Ctrl Pts',(-43.1505602981365,-58.4933346130636,
0.));
#136370=CARTESIAN_POINT('Ctrl Pts',(-43.1505602981365,-58.4933346130636,
12.));
#136371=CARTESIAN_POINT('Ctrl Pts',(-43.1292058256777,-58.4799015199907,
0.));
#136372=CARTESIAN_POINT('Ctrl Pts',(-43.1292058256777,-58.4799015199907,
12.));
#136373=CARTESIAN_POINT('Ctrl Pts',(-43.1078977421916,-58.4664693046217,
0.));
#136374=CARTESIAN_POINT('Ctrl Pts',(-43.1078977421916,-58.4664693046217,
12.));
#136375=CARTESIAN_POINT('Ctrl Pts',(-43.0866361081177,-58.4530380703348,
0.));
#136376=CARTESIAN_POINT('Ctrl Pts',(-43.0866361081177,-58.4530380703348,
12.));
#136377=CARTESIAN_POINT('Ctrl Pts',(-43.0654209840511,-58.439607920945,
0.));
#136378=CARTESIAN_POINT('Ctrl Pts',(-43.0654209840511,-58.439607920945,
12.));
#136379=CARTESIAN_POINT('Ctrl Pts',(-43.0442524307434,-58.4261789607058,
0.));
#136380=CARTESIAN_POINT('Ctrl Pts',(-43.0442524307434,-58.4261789607058,
12.));
#136381=CARTESIAN_POINT('Ctrl Pts',(-43.0231305091027,-58.4127512943136,
0.));
#136382=CARTESIAN_POINT('Ctrl Pts',(-43.0231305091027,-58.4127512943136,
12.));
#136383=CARTESIAN_POINT('Ctrl Pts',(-43.0020552801859,-58.3993250269101,
0.));
#136384=CARTESIAN_POINT('Ctrl Pts',(-43.0020552801859,-58.3993250269101,
12.));
#136385=CARTESIAN_POINT('Ctrl Pts',(-42.9810268052032,-58.3859002640856,
0.));
#136386=CARTESIAN_POINT('Ctrl Pts',(-42.9810268052032,-58.3859002640856,
12.));
#136387=CARTESIAN_POINT('Ctrl Pts',(-42.960045145526,-58.3724771118826,
0.));
#136388=CARTESIAN_POINT('Ctrl Pts',(-42.960045145526,-58.3724771118826,
12.));
#136389=CARTESIAN_POINT('Ctrl Pts',(-42.9391103626879,-58.3590556767978,
0.));
#136390=CARTESIAN_POINT('Ctrl Pts',(-42.9391103626879,-58.3590556767978,
12.));
#136391=CARTESIAN_POINT('Ctrl Pts',(-42.9182225183855,-58.3456360657865,
0.));
#136392=CARTESIAN_POINT('Ctrl Pts',(-42.9182225183855,-58.3456360657865,
12.));
#136393=CARTESIAN_POINT('Ctrl Pts',(-42.8973816744709,-58.3322183862654,
0.));
#136394=CARTESIAN_POINT('Ctrl Pts',(-42.8973816744709,-58.3322183862654,
12.));
#136395=CARTESIAN_POINT('Ctrl Pts',(-42.8765878929551,-58.3188027461164,
0.));
#136396=CARTESIAN_POINT('Ctrl Pts',(-42.8765878929551,-58.3188027461164,
12.));
#136397=CARTESIAN_POINT('Ctrl Pts',(-42.8558412360158,-58.3053892536894,
0.));
#136398=CARTESIAN_POINT('Ctrl Pts',(-42.8558412360158,-58.3053892536894,
12.));
#136399=CARTESIAN_POINT('Ctrl Pts',(-42.8351417659999,-58.2919780178064,
0.));
#136400=CARTESIAN_POINT('Ctrl Pts',(-42.8351417659999,-58.2919780178064,
12.));
#136401=CARTESIAN_POINT('Ctrl Pts',(-42.8144895454233,-58.2785691477638,
0.));
#136402=CARTESIAN_POINT('Ctrl Pts',(-42.8144895454233,-58.2785691477638,
12.));
#136403=CARTESIAN_POINT('Ctrl Pts',(-42.7938846369651,-58.2651627533368,
0.));
#136404=CARTESIAN_POINT('Ctrl Pts',(-42.7938846369651,-58.2651627533368,
12.));
#136405=CARTESIAN_POINT('Ctrl Pts',(-42.7733271034679,-58.251758944782,
0.));
#136406=CARTESIAN_POINT('Ctrl Pts',(-42.7733271034679,-58.251758944782,
12.));
#136407=CARTESIAN_POINT('Ctrl Pts',(-42.7528170079484,-58.2383578328424,
0.));
#136408=CARTESIAN_POINT('Ctrl Pts',(-42.7528170079484,-58.2383578328424,
12.));
#136409=CARTESIAN_POINT('Ctrl Pts',(-42.7323544135985,-58.22495952875,0.));
#136410=CARTESIAN_POINT('Ctrl Pts',(-42.7323544135985,-58.22495952875,12.));
#136411=CARTESIAN_POINT('Ctrl Pts',(-42.7119393837866,-58.21156414423,0.));
#136412=CARTESIAN_POINT('Ctrl Pts',(-42.7119393837866,-58.21156414423,12.));
#136413=CARTESIAN_POINT('Ctrl Pts',(-42.6915719820513,-58.1981717915037,
0.));
#136414=CARTESIAN_POINT('Ctrl Pts',(-42.6915719820513,-58.1981717915037,
12.));
#136415=CARTESIAN_POINT('Ctrl Pts',(-42.6712522721016,-58.1847825832923,
0.));
#136416=CARTESIAN_POINT('Ctrl Pts',(-42.6712522721016,-58.1847825832923,
12.));
#136417=CARTESIAN_POINT('Ctrl Pts',(-42.6509803178265,-58.171396632821,
0.));
#136418=CARTESIAN_POINT('Ctrl Pts',(-42.6509803178265,-58.171396632821,
12.));
#136419=CARTESIAN_POINT('Ctrl Pts',(-42.6307561832976,-58.1580140538228,
0.));
#136420=CARTESIAN_POINT('Ctrl Pts',(-42.6307561832976,-58.1580140538228,
12.));
#136421=CARTESIAN_POINT('Ctrl Pts',(-42.6105799327699,-58.1446349605421,
0.));
#136422=CARTESIAN_POINT('Ctrl Pts',(-42.6105799327699,-58.1446349605421,
12.));
#136423=CARTESIAN_POINT('Ctrl Pts',(-42.5904516306762,-58.1312594677386,
0.));
#136424=CARTESIAN_POINT('Ctrl Pts',(-42.5904516306762,-58.1312594677386,
12.));
#136425=CARTESIAN_POINT('Ctrl Pts',(-42.5703713416265,-58.1178876906907,
0.));
#136426=CARTESIAN_POINT('Ctrl Pts',(-42.5703713416265,-58.1178876906907,
12.));
#136427=CARTESIAN_POINT('Ctrl Pts',(-42.5503391304183,-58.1045197452002,
0.));
#136428=CARTESIAN_POINT('Ctrl Pts',(-42.5503391304183,-58.1045197452002,
12.));
#136429=CARTESIAN_POINT('Ctrl Pts',(-42.5303550620387,-58.0911557475965,
0.));
#136430=CARTESIAN_POINT('Ctrl Pts',(-42.5303550620387,-58.0911557475965,
12.));
#136431=CARTESIAN_POINT('Ctrl Pts',(-42.5104192016664,-58.0777958147403,
0.));
#136432=CARTESIAN_POINT('Ctrl Pts',(-42.5104192016664,-58.0777958147403,
12.));
#136433=CARTESIAN_POINT('Ctrl Pts',(-42.4905316146653,-58.0644400640275,
0.));
#136434=CARTESIAN_POINT('Ctrl Pts',(-42.4905316146653,-58.0644400640275,
12.));
#136435=CARTESIAN_POINT('Ctrl Pts',(-42.4706923665845,-58.0510886133926,
0.));
#136436=CARTESIAN_POINT('Ctrl Pts',(-42.4706923665845,-58.0510886133926,
12.));
#136437=CARTESIAN_POINT('Ctrl Pts',(-42.4509015231674,-58.037741581314,
0.));
#136438=CARTESIAN_POINT('Ctrl Pts',(-42.4509015231674,-58.037741581314,
12.));
#136439=CARTESIAN_POINT('Ctrl Pts',(-42.4311591503555,-58.0243990868181,
0.));
#136440=CARTESIAN_POINT('Ctrl Pts',(-42.4311591503555,-58.0243990868181,
12.));
#136441=CARTESIAN_POINT('Ctrl Pts',(-42.411465314289,-58.0110612494828,
0.));
#136442=CARTESIAN_POINT('Ctrl Pts',(-42.411465314289,-58.0110612494828,
12.));
#136443=CARTESIAN_POINT('Ctrl Pts',(-42.3918200813014,-57.9977281894422,
0.));
#136444=CARTESIAN_POINT('Ctrl Pts',(-42.3918200813014,-57.9977281894422,
12.));
#136445=CARTESIAN_POINT('Ctrl Pts',(-42.3722235179197,-57.9844000273911,
0.));
#136446=CARTESIAN_POINT('Ctrl Pts',(-42.3722235179197,-57.9844000273911,
12.));
#136447=CARTESIAN_POINT('Ctrl Pts',(-42.3526756908746,-57.9710768845899,
0.));
#136448=CARTESIAN_POINT('Ctrl Pts',(-42.3526756908746,-57.9710768845899,
12.));
#136449=CARTESIAN_POINT('Ctrl Pts',(-42.333176667102,-57.9577588828682,
0.));
#136450=CARTESIAN_POINT('Ctrl Pts',(-42.333176667102,-57.9577588828682,
12.));
#136451=CARTESIAN_POINT('Ctrl Pts',(-42.3137265137452,-57.9444461446299,
0.));
#136452=CARTESIAN_POINT('Ctrl Pts',(-42.3137265137452,-57.9444461446299,
12.));
#136453=CARTESIAN_POINT('Ctrl Pts',(-42.2943252981489,-57.9311387928563,
0.));
#136454=CARTESIAN_POINT('Ctrl Pts',(-42.2943252981489,-57.9311387928563,
12.));
#136455=CARTESIAN_POINT('Ctrl Pts',(-42.2749730878594,-57.9178369511114,
0.));
#136456=CARTESIAN_POINT('Ctrl Pts',(-42.2749730878594,-57.9178369511114,
12.));
#136457=CARTESIAN_POINT('Ctrl Pts',(-42.2556699506353,-57.9045407435474,
0.));
#136458=CARTESIAN_POINT('Ctrl Pts',(-42.2556699506353,-57.9045407435474,
12.));
#136459=CARTESIAN_POINT('Ctrl Pts',(-42.2364159544501,-57.8912502949096,
0.));
#136460=CARTESIAN_POINT('Ctrl Pts',(-42.2364159544501,-57.8912502949096,
12.));
#136461=CARTESIAN_POINT('Ctrl Pts',(-42.2172111674938,-57.8779657305413,
0.));
#136462=CARTESIAN_POINT('Ctrl Pts',(-42.2172111674938,-57.8779657305413,
12.));
#136463=CARTESIAN_POINT('Ctrl Pts',(-42.1980556581665,-57.864687176387,
0.));
#136464=CARTESIAN_POINT('Ctrl Pts',(-42.1980556581665,-57.864687176387,
12.));
#136465=CARTESIAN_POINT('Ctrl Pts',(-42.1789494950794,-57.8514147589972,
0.));
#136466=CARTESIAN_POINT('Ctrl Pts',(-42.1789494950794,-57.8514147589972,
12.));
#136467=CARTESIAN_POINT('Ctrl Pts',(-42.1598927470646,-57.8381486055342,
0.));
#136468=CARTESIAN_POINT('Ctrl Pts',(-42.1598927470646,-57.8381486055342,
12.));
#136469=CARTESIAN_POINT('Ctrl Pts',(-42.1408854831783,-57.8248888437775,
0.));
#136470=CARTESIAN_POINT('Ctrl Pts',(-42.1408854831783,-57.8248888437775,
12.));
#136471=CARTESIAN_POINT('Ctrl Pts',(-42.1219277727021,-57.8116356021288,
0.));
#136472=CARTESIAN_POINT('Ctrl Pts',(-42.1219277727021,-57.8116356021288,
12.));
#136473=CARTESIAN_POINT('Ctrl Pts',(-42.1030196851366,-57.798389009616,
0.));
#136474=CARTESIAN_POINT('Ctrl Pts',(-42.1030196851366,-57.798389009616,
12.));
#136475=CARTESIAN_POINT('Ctrl Pts',(-42.0841612902042,-57.7851491958987,
0.));
#136476=CARTESIAN_POINT('Ctrl Pts',(-42.0841612902042,-57.7851491958987,
12.));
#136477=CARTESIAN_POINT('Ctrl Pts',(-42.0653526578588,-57.7719162912744,
0.));
#136478=CARTESIAN_POINT('Ctrl Pts',(-42.0653526578588,-57.7719162912744,
12.));
#136479=CARTESIAN_POINT('Ctrl Pts',(-42.0465938582882,-57.7586904266834,
0.));
#136480=CARTESIAN_POINT('Ctrl Pts',(-42.0465938582882,-57.7586904266834,
12.));
#136481=CARTESIAN_POINT('Ctrl Pts',(-42.0278849619148,-57.745471733714,
0.));
#136482=CARTESIAN_POINT('Ctrl Pts',(-42.0278849619148,-57.745471733714,
12.));
#136483=CARTESIAN_POINT('Ctrl Pts',(-42.0092260393897,-57.7322603446066,
0.));
#136484=CARTESIAN_POINT('Ctrl Pts',(-42.0092260393897,-57.7322603446066,
12.));
#136485=CARTESIAN_POINT('Ctrl Pts',(-41.990617161596,-57.7190563922593,
0.));
#136486=CARTESIAN_POINT('Ctrl Pts',(-41.990617161596,-57.7190563922593,
12.));
#136487=CARTESIAN_POINT('Ctrl Pts',(-41.9720583996592,-57.7058600102351,
0.));
#136488=CARTESIAN_POINT('Ctrl Pts',(-41.9720583996592,-57.7058600102351,
12.));
#136489=CARTESIAN_POINT('Ctrl Pts',(-41.9535498249488,-57.6926713327672,
0.));
#136490=CARTESIAN_POINT('Ctrl Pts',(-41.9535498249488,-57.6926713327672,
12.));
#136491=CARTESIAN_POINT('Ctrl Pts',(-41.9350915090796,-57.6794904947649,
0.));
#136492=CARTESIAN_POINT('Ctrl Pts',(-41.9350915090796,-57.6794904947649,
12.));
#136493=CARTESIAN_POINT('Ctrl Pts',(-41.9166835239054,-57.6663176318189,
0.));
#136494=CARTESIAN_POINT('Ctrl Pts',(-41.9166835239054,-57.6663176318189,
12.));
#136495=CARTESIAN_POINT('Ctrl Pts',(-41.8983259415253,-57.6531528802072,
0.));
#136496=CARTESIAN_POINT('Ctrl Pts',(-41.8983259415253,-57.6531528802072,
12.));
#136497=CARTESIAN_POINT('Ctrl Pts',(-41.8800188342912,-57.6399963769009,
0.));
#136498=CARTESIAN_POINT('Ctrl Pts',(-41.8800188342912,-57.6399963769009,
12.));
#136499=CARTESIAN_POINT('Ctrl Pts',(-41.8617622748107,-57.6268482595701,
0.));
#136500=CARTESIAN_POINT('Ctrl Pts',(-41.8617622748107,-57.6268482595701,
12.));
#136501=CARTESIAN_POINT('Ctrl Pts',(-41.8435563359456,-57.613708666588,
0.));
#136502=CARTESIAN_POINT('Ctrl Pts',(-41.8435563359456,-57.613708666588,
12.));
#136503=CARTESIAN_POINT('Ctrl Pts',(-41.8254010908051,-57.6005777370347,
0.));
#136504=CARTESIAN_POINT('Ctrl Pts',(-41.8254010908051,-57.6005777370347,
12.));
#136505=CARTESIAN_POINT('Ctrl Pts',(-41.8072966127559,-57.5874556107054,
0.));
#136506=CARTESIAN_POINT('Ctrl Pts',(-41.8072966127559,-57.5874556107054,
12.));
#136507=CARTESIAN_POINT('Ctrl Pts',(-41.7892429754298,-57.5743424281204,
0.));
#136508=CARTESIAN_POINT('Ctrl Pts',(-41.7892429754298,-57.5743424281204,
12.));
#136509=CARTESIAN_POINT('Ctrl Pts',(-41.7712402527273,-57.561238330532,
0.));
#136510=CARTESIAN_POINT('Ctrl Pts',(-41.7712402527273,-57.561238330532,
12.));
#136511=CARTESIAN_POINT('Ctrl Pts',(-41.7532885188174,-57.5481434599334,
0.));
#136512=CARTESIAN_POINT('Ctrl Pts',(-41.7532885188174,-57.5481434599334,
12.));
#136513=CARTESIAN_POINT('Ctrl Pts',(-41.7353878481336,-57.5350579590648,
0.));
#136514=CARTESIAN_POINT('Ctrl Pts',(-41.7353878481336,-57.5350579590648,
12.));
#136515=CARTESIAN_POINT('Ctrl Pts',(-41.7175383153819,-57.5219819714169,
0.));
#136516=CARTESIAN_POINT('Ctrl Pts',(-41.7175383153819,-57.5219819714169,
12.));
#136517=CARTESIAN_POINT('Ctrl Pts',(-41.6997399955445,-57.5089156412341,
0.));
#136518=CARTESIAN_POINT('Ctrl Pts',(-41.6997399955445,-57.5089156412341,
12.));
#136519=CARTESIAN_POINT('Ctrl Pts',(-41.6819929638797,-57.4958591135165,
0.));
#136520=CARTESIAN_POINT('Ctrl Pts',(-41.6819929638797,-57.4958591135165,
12.));
#136521=CARTESIAN_POINT('Ctrl Pts',(-41.6642972959168,-57.4828125340222,
0.));
#136522=CARTESIAN_POINT('Ctrl Pts',(-41.6642972959168,-57.4828125340222,
12.));
#136523=CARTESIAN_POINT('Ctrl Pts',(-41.6466530674522,-57.4697760492693,
0.));
#136524=CARTESIAN_POINT('Ctrl Pts',(-41.6466530674522,-57.4697760492693,
12.));
#136525=CARTESIAN_POINT('Ctrl Pts',(-41.6290603545674,-57.4567498065573,
0.));
#136526=CARTESIAN_POINT('Ctrl Pts',(-41.6290603545674,-57.4567498065573,
12.));
#136527=CARTESIAN_POINT('Ctrl Pts',(-41.6115192336393,-57.4437339539848,
0.));
#136528=CARTESIAN_POINT('Ctrl Pts',(-41.6115192336393,-57.4437339539848,
12.));
#136529=CARTESIAN_POINT('Ctrl Pts',(-41.5940297813474,-57.4307286404656,
0.));
#136530=CARTESIAN_POINT('Ctrl Pts',(-41.5940297813474,-57.4307286404656,
12.));
#136531=CARTESIAN_POINT('Ctrl Pts',(-41.5765920746764,-57.417734015749,
0.));
#136532=CARTESIAN_POINT('Ctrl Pts',(-41.5765920746764,-57.417734015749,
12.));
#136533=CARTESIAN_POINT('Ctrl Pts',(-41.5592061909159,-57.4047502304207,
0.));
#136534=CARTESIAN_POINT('Ctrl Pts',(-41.5592061909159,-57.4047502304207,
12.));
#136535=CARTESIAN_POINT('Ctrl Pts',(-41.5418722076558,-57.3917774358844,
0.));
#136536=CARTESIAN_POINT('Ctrl Pts',(-41.5418722076558,-57.3917774358844,
12.));
#136537=CARTESIAN_POINT('Ctrl Pts',(-41.5245902027767,-57.378815784345,
0.));
#136538=CARTESIAN_POINT('Ctrl Pts',(-41.5245902027767,-57.378815784345,
12.));
#136539=CARTESIAN_POINT('Ctrl Pts',(-41.5073602544404,-57.3658654287948,
0.));
#136540=CARTESIAN_POINT('Ctrl Pts',(-41.5073602544404,-57.3658654287948,
12.));
#136541=CARTESIAN_POINT('Ctrl Pts',(-41.4901824410654,-57.3529265229858,
0.));
#136542=CARTESIAN_POINT('Ctrl Pts',(-41.4901824410654,-57.3529265229858,
12.));
#136543=CARTESIAN_POINT('Ctrl Pts',(-41.4730568413535,-57.339999221474,
0.));
#136544=CARTESIAN_POINT('Ctrl Pts',(-41.4730568413535,-57.339999221474,
12.));
#136545=CARTESIAN_POINT('Ctrl Pts',(-41.4559835343338,-57.3270836796925,
0.));
#136546=CARTESIAN_POINT('Ctrl Pts',(-41.4559835343338,-57.3270836796925,
12.));
#136547=CARTESIAN_POINT('Ctrl Pts',(-41.4389625993948,-57.3141800540137,
0.));
#136548=CARTESIAN_POINT('Ctrl Pts',(-41.4389625993948,-57.3141800540137,
12.));
#136549=CARTESIAN_POINT('Ctrl Pts',(-41.4219941163154,-57.3012885018139,
0.));
#136550=CARTESIAN_POINT('Ctrl Pts',(-41.4219941163154,-57.3012885018139,
12.));
#136551=CARTESIAN_POINT('Ctrl Pts',(-41.4050781652923,-57.2884091815385,
0.));
#136552=CARTESIAN_POINT('Ctrl Pts',(-41.4050781652923,-57.2884091815385,
12.));
#136553=CARTESIAN_POINT('Ctrl Pts',(-41.3882148268798,-57.2755422525822,
0.));
#136554=CARTESIAN_POINT('Ctrl Pts',(-41.3882148268798,-57.2755422525822,
12.));
#136555=CARTESIAN_POINT('Ctrl Pts',(-41.3714041819215,-57.2626878751584,
0.));
#136556=CARTESIAN_POINT('Ctrl Pts',(-41.3714041819215,-57.2626878751584,
12.));
#136557=CARTESIAN_POINT('Ctrl Pts',(-41.3546463114889,-57.2498462101883,
0.));
#136558=CARTESIAN_POINT('Ctrl Pts',(-41.3546463114889,-57.2498462101883,
12.));
#136559=CARTESIAN_POINT('Ctrl Pts',(-41.3379412967889,-57.237017419142,
0.));
#136560=CARTESIAN_POINT('Ctrl Pts',(-41.3379412967889,-57.237017419142,
12.));
#136561=CARTESIAN_POINT('Ctrl Pts',(-41.321289219151,-57.2242016640226,
0.));
#136562=CARTESIAN_POINT('Ctrl Pts',(-41.321289219151,-57.2242016640226,
12.));
#136563=CARTESIAN_POINT('Ctrl Pts',(-41.304690160231,-57.2113991077325,
0.));
#136564=CARTESIAN_POINT('Ctrl Pts',(-41.304690160231,-57.2113991077325,
12.));
#136565=CARTESIAN_POINT('Ctrl Pts',(-41.2881442021869,-57.1986099143992,
0.));
#136566=CARTESIAN_POINT('Ctrl Pts',(-41.2881442021869,-57.1986099143992,
12.));
#136567=CARTESIAN_POINT('Ctrl Pts',(-41.2716514278268,-57.1858342496526,
0.));
#136568=CARTESIAN_POINT('Ctrl Pts',(-41.2716514278268,-57.1858342496526,
12.));
#136569=CARTESIAN_POINT('Ctrl Pts',(-41.2552119208445,-57.1730722810771,
0.));
#136570=CARTESIAN_POINT('Ctrl Pts',(-41.2552119208445,-57.1730722810771,
12.));
#136571=CARTESIAN_POINT('Ctrl Pts',(-41.2388257656534,-57.1603241779042,
0.));
#136572=CARTESIAN_POINT('Ctrl Pts',(-41.2388257656534,-57.1603241779042,
12.));
#136573=CARTESIAN_POINT('Ctrl Pts',(-41.2224930469412,-57.1475901101795,
0.));
#136574=CARTESIAN_POINT('Ctrl Pts',(-41.2224930469412,-57.1475901101795,
12.));
#136575=CARTESIAN_POINT('Ctrl Pts',(-41.2062138492913,-57.1348702480644,
0.));
#136576=CARTESIAN_POINT('Ctrl Pts',(-41.2062138492913,-57.1348702480644,
12.));
#136577=CARTESIAN_POINT('Ctrl Pts',(-41.1899882567941,-57.1221647611231,
0.));
#136578=CARTESIAN_POINT('Ctrl Pts',(-41.1899882567941,-57.1221647611231,
12.));
#136579=CARTESIAN_POINT('Ctrl Pts',(-41.1738163525931,-57.1094738174998,
0.));
#136580=CARTESIAN_POINT('Ctrl Pts',(-41.1738163525931,-57.1094738174998,
12.));
#136581=CARTESIAN_POINT('Ctrl Pts',(-41.1576982197402,-57.0967975854912,
0.));
#136582=CARTESIAN_POINT('Ctrl Pts',(-41.1576982197402,-57.0967975854912,
12.));
#136583=CARTESIAN_POINT('Ctrl Pts',(-41.1416339422132,-57.0841362354281,
0.));
#136584=CARTESIAN_POINT('Ctrl Pts',(-41.1416339422132,-57.0841362354281,
12.));
#136585=CARTESIAN_POINT('Ctrl Pts',(-41.1256236057436,-57.0714899412091,
0.));
#136586=CARTESIAN_POINT('Ctrl Pts',(-41.1256236057436,-57.0714899412091,
12.));
#136587=CARTESIAN_POINT('Ctrl Pts',(-41.1096672990125,-57.0588588825266,
0.));
#136588=CARTESIAN_POINT('Ctrl Pts',(-41.1096672990125,-57.0588588825266,
12.));
#136589=CARTESIAN_POINT('Ctrl Pts',(-41.0937651137519,-57.0462432450637,
0.));
#136590=CARTESIAN_POINT('Ctrl Pts',(-41.0937651137519,-57.0462432450637,
12.));
#136591=CARTESIAN_POINT('Ctrl Pts',(-41.0779171422415,-57.0336432158503,
0.));
#136592=CARTESIAN_POINT('Ctrl Pts',(-41.0779171422415,-57.0336432158503,
12.));
#136593=CARTESIAN_POINT('Ctrl Pts',(-41.0621234751,-57.0210589791777,0.));
#136594=CARTESIAN_POINT('Ctrl Pts',(-41.0621234751,-57.0210589791777,12.));
#136595=CARTESIAN_POINT('Ctrl Pts',(-41.0463841993622,-57.008490713044,
0.));
#136596=CARTESIAN_POINT('Ctrl Pts',(-41.0463841993622,-57.008490713044,
12.));
#136597=CARTESIAN_POINT('Ctrl Pts',(-41.0306993954021,-56.9959385834768,
0.));
#136598=CARTESIAN_POINT('Ctrl Pts',(-41.0306993954021,-56.9959385834768,
12.));
#136599=CARTESIAN_POINT('Ctrl Pts',(-41.0150691398988,-56.9834027500178,
0.));
#136600=CARTESIAN_POINT('Ctrl Pts',(-41.0150691398988,-56.9834027500178,
12.));
#136601=CARTESIAN_POINT('Ctrl Pts',(-40.9994935117307,-56.9708833766183,
0.));
#136602=CARTESIAN_POINT('Ctrl Pts',(-40.9994935117307,-56.9708833766183,
12.));
#136603=CARTESIAN_POINT('Ctrl Pts',(-40.9839725967121,-56.9583806404069,
0.));
#136604=CARTESIAN_POINT('Ctrl Pts',(-40.9839725967121,-56.9583806404069,
12.));
#136605=CARTESIAN_POINT('Ctrl Pts',(-40.968506493303,-56.9458947422541,
0.));
#136606=CARTESIAN_POINT('Ctrl Pts',(-40.968506493303,-56.9458947422541,
12.));
#136607=CARTESIAN_POINT('Ctrl Pts',(-40.9530953164952,-56.9334259139928,
0.));
#136608=CARTESIAN_POINT('Ctrl Pts',(-40.9530953164952,-56.9334259139928,
12.));
#136609=CARTESIAN_POINT('Ctrl Pts',(-40.9377391857044,-56.9209743960861,
0.));
#136610=CARTESIAN_POINT('Ctrl Pts',(-40.9377391857044,-56.9209743960861,
12.));
#136611=CARTESIAN_POINT('Ctrl Pts',(-40.9224382132382,-56.9085404164432,
0.));
#136612=CARTESIAN_POINT('Ctrl Pts',(-40.9224382132382,-56.9085404164432,
12.));
#136613=CARTESIAN_POINT('Ctrl Pts',(-40.9071924937551,-56.8961241708926,
0.));
#136614=CARTESIAN_POINT('Ctrl Pts',(-40.9071924937551,-56.8961241708926,
12.));
#136615=CARTESIAN_POINT('Ctrl Pts',(-40.8920020903443,-56.8837257978574,
0.));
#136616=CARTESIAN_POINT('Ctrl Pts',(-40.8920020903443,-56.8837257978574,
12.));
#136617=CARTESIAN_POINT('Ctrl Pts',(-40.8768670342278,-56.8713453765252,
0.));
#136618=CARTESIAN_POINT('Ctrl Pts',(-40.8768670342278,-56.8713453765252,
12.));
#136619=CARTESIAN_POINT('Ctrl Pts',(-40.8648032759631,-56.8614554317993,
0.));
#136620=CARTESIAN_POINT('Ctrl Pts',(-40.8648032759631,-56.8614554317993,
12.));
#136621=CARTESIAN_POINT('Ctrl Pts',(-40.8557803680411,-56.8540460739677,
0.));
#136622=CARTESIAN_POINT('Ctrl Pts',(-40.8557803680411,-56.8540460739677,
12.));
#136623=CARTESIAN_POINT('Ctrl Pts',(-40.8497761671086,-56.8491101022668,
0.));
#136624=CARTESIAN_POINT('Ctrl Pts',(-40.8497761671086,-56.8491101022668,
12.));
#136625=CARTESIAN_POINT('Ctrl Pts',(-40.8467768343956,-56.8466430164621,
0.));
#136626=CARTESIAN_POINT('Ctrl Pts',(-40.8467768343956,-56.8466430164621,
12.));
#136627=CARTESIAN_POINT('',(-40.8467768343956,-56.8466430164621,12.));
#136628=CARTESIAN_POINT('Ctrl Pts',(-40.8467768343956,-56.8466430164621,
12.));
#136629=CARTESIAN_POINT('Ctrl Pts',(-40.8497761671086,-56.8491101022668,
12.));
#136630=CARTESIAN_POINT('Ctrl Pts',(-40.8557803680411,-56.8540460739677,
12.));
#136631=CARTESIAN_POINT('Ctrl Pts',(-40.8648032759631,-56.8614554317993,
12.));
#136632=CARTESIAN_POINT('Ctrl Pts',(-40.8768670342278,-56.8713453765252,
12.));
#136633=CARTESIAN_POINT('Ctrl Pts',(-40.8920020903443,-56.8837257978574,
12.));
#136634=CARTESIAN_POINT('Ctrl Pts',(-40.9071924937551,-56.8961241708926,
12.));
#136635=CARTESIAN_POINT('Ctrl Pts',(-40.9224382132382,-56.9085404164432,
12.));
#136636=CARTESIAN_POINT('Ctrl Pts',(-40.9377391857044,-56.9209743960861,
12.));
#136637=CARTESIAN_POINT('Ctrl Pts',(-40.9530953164952,-56.9334259139928,
12.));
#136638=CARTESIAN_POINT('Ctrl Pts',(-40.968506493303,-56.9458947422541,
12.));
#136639=CARTESIAN_POINT('Ctrl Pts',(-40.9839725967121,-56.9583806404069,
12.));
#136640=CARTESIAN_POINT('Ctrl Pts',(-40.9994935117307,-56.9708833766183,
12.));
#136641=CARTESIAN_POINT('Ctrl Pts',(-41.0150691398988,-56.9834027500178,
12.));
#136642=CARTESIAN_POINT('Ctrl Pts',(-41.0306993954021,-56.9959385834768,
12.));
#136643=CARTESIAN_POINT('Ctrl Pts',(-41.0463841993622,-57.008490713044,
12.));
#136644=CARTESIAN_POINT('Ctrl Pts',(-41.0621234751,-57.0210589791777,12.));
#136645=CARTESIAN_POINT('Ctrl Pts',(-41.0779171422415,-57.0336432158503,
12.));
#136646=CARTESIAN_POINT('Ctrl Pts',(-41.0937651137519,-57.0462432450637,
12.));
#136647=CARTESIAN_POINT('Ctrl Pts',(-41.1096672990125,-57.0588588825266,
12.));
#136648=CARTESIAN_POINT('Ctrl Pts',(-41.1256236057436,-57.0714899412091,
12.));
#136649=CARTESIAN_POINT('Ctrl Pts',(-41.1416339422132,-57.0841362354281,
12.));
#136650=CARTESIAN_POINT('Ctrl Pts',(-41.1576982197402,-57.0967975854912,
12.));
#136651=CARTESIAN_POINT('Ctrl Pts',(-41.1738163525931,-57.1094738174998,
12.));
#136652=CARTESIAN_POINT('Ctrl Pts',(-41.1899882567941,-57.1221647611231,
12.));
#136653=CARTESIAN_POINT('Ctrl Pts',(-41.2062138492913,-57.1348702480644,
12.));
#136654=CARTESIAN_POINT('Ctrl Pts',(-41.2224930469412,-57.1475901101795,
12.));
#136655=CARTESIAN_POINT('Ctrl Pts',(-41.2388257656534,-57.1603241779042,
12.));
#136656=CARTESIAN_POINT('Ctrl Pts',(-41.2552119208445,-57.1730722810771,
12.));
#136657=CARTESIAN_POINT('Ctrl Pts',(-41.2716514278268,-57.1858342496526,
12.));
#136658=CARTESIAN_POINT('Ctrl Pts',(-41.2881442021869,-57.1986099143992,
12.));
#136659=CARTESIAN_POINT('Ctrl Pts',(-41.304690160231,-57.2113991077325,
12.));
#136660=CARTESIAN_POINT('Ctrl Pts',(-41.321289219151,-57.2242016640226,
12.));
#136661=CARTESIAN_POINT('Ctrl Pts',(-41.3379412967889,-57.237017419142,
12.));
#136662=CARTESIAN_POINT('Ctrl Pts',(-41.3546463114889,-57.2498462101883,
12.));
#136663=CARTESIAN_POINT('Ctrl Pts',(-41.3714041819215,-57.2626878751584,
12.));
#136664=CARTESIAN_POINT('Ctrl Pts',(-41.3882148268798,-57.2755422525822,
12.));
#136665=CARTESIAN_POINT('Ctrl Pts',(-41.4050781652923,-57.2884091815385,
12.));
#136666=CARTESIAN_POINT('Ctrl Pts',(-41.4219941163154,-57.3012885018139,
12.));
#136667=CARTESIAN_POINT('Ctrl Pts',(-41.4389625993948,-57.3141800540137,
12.));
#136668=CARTESIAN_POINT('Ctrl Pts',(-41.4559835343338,-57.3270836796925,
12.));
#136669=CARTESIAN_POINT('Ctrl Pts',(-41.4730568413535,-57.339999221474,
12.));
#136670=CARTESIAN_POINT('Ctrl Pts',(-41.4901824410654,-57.3529265229858,
12.));
#136671=CARTESIAN_POINT('Ctrl Pts',(-41.5073602544404,-57.3658654287948,
12.));
#136672=CARTESIAN_POINT('Ctrl Pts',(-41.5245902027767,-57.378815784345,
12.));
#136673=CARTESIAN_POINT('Ctrl Pts',(-41.5418722076558,-57.3917774358844,
12.));
#136674=CARTESIAN_POINT('Ctrl Pts',(-41.5592061909159,-57.4047502304207,
12.));
#136675=CARTESIAN_POINT('Ctrl Pts',(-41.5765920746764,-57.417734015749,
12.));
#136676=CARTESIAN_POINT('Ctrl Pts',(-41.5940297813474,-57.4307286404656,
12.));
#136677=CARTESIAN_POINT('Ctrl Pts',(-41.6115192336393,-57.4437339539848,
12.));
#136678=CARTESIAN_POINT('Ctrl Pts',(-41.6290603545674,-57.4567498065573,
12.));
#136679=CARTESIAN_POINT('Ctrl Pts',(-41.6466530674522,-57.4697760492693,
12.));
#136680=CARTESIAN_POINT('Ctrl Pts',(-41.6642972959168,-57.4828125340222,
12.));
#136681=CARTESIAN_POINT('Ctrl Pts',(-41.6819929638797,-57.4958591135165,
12.));
#136682=CARTESIAN_POINT('Ctrl Pts',(-41.6997399955445,-57.5089156412341,
12.));
#136683=CARTESIAN_POINT('Ctrl Pts',(-41.7175383153819,-57.5219819714169,
12.));
#136684=CARTESIAN_POINT('Ctrl Pts',(-41.7353878481336,-57.5350579590648,
12.));
#136685=CARTESIAN_POINT('Ctrl Pts',(-41.7532885188174,-57.5481434599334,
12.));
#136686=CARTESIAN_POINT('Ctrl Pts',(-41.7712402527273,-57.561238330532,
12.));
#136687=CARTESIAN_POINT('Ctrl Pts',(-41.7892429754298,-57.5743424281204,
12.));
#136688=CARTESIAN_POINT('Ctrl Pts',(-41.8072966127559,-57.5874556107054,
12.));
#136689=CARTESIAN_POINT('Ctrl Pts',(-41.8254010908051,-57.6005777370347,
12.));
#136690=CARTESIAN_POINT('Ctrl Pts',(-41.8435563359456,-57.613708666588,
12.));
#136691=CARTESIAN_POINT('Ctrl Pts',(-41.8617622748107,-57.6268482595701,
12.));
#136692=CARTESIAN_POINT('Ctrl Pts',(-41.8800188342912,-57.6399963769009,
12.));
#136693=CARTESIAN_POINT('Ctrl Pts',(-41.8983259415253,-57.6531528802072,
12.));
#136694=CARTESIAN_POINT('Ctrl Pts',(-41.9166835239054,-57.6663176318189,
12.));
#136695=CARTESIAN_POINT('Ctrl Pts',(-41.9350915090796,-57.6794904947649,
12.));
#136696=CARTESIAN_POINT('Ctrl Pts',(-41.9535498249488,-57.6926713327672,
12.));
#136697=CARTESIAN_POINT('Ctrl Pts',(-41.9720583996592,-57.7058600102351,
12.));
#136698=CARTESIAN_POINT('Ctrl Pts',(-41.990617161596,-57.7190563922593,
12.));
#136699=CARTESIAN_POINT('Ctrl Pts',(-42.0092260393897,-57.7322603446066,
12.));
#136700=CARTESIAN_POINT('Ctrl Pts',(-42.0278849619148,-57.745471733714,
12.));
#136701=CARTESIAN_POINT('Ctrl Pts',(-42.0465938582882,-57.7586904266834,
12.));
#136702=CARTESIAN_POINT('Ctrl Pts',(-42.0653526578588,-57.7719162912744,
12.));
#136703=CARTESIAN_POINT('Ctrl Pts',(-42.0841612902042,-57.7851491958987,
12.));
#136704=CARTESIAN_POINT('Ctrl Pts',(-42.1030196851366,-57.798389009616,
12.));
#136705=CARTESIAN_POINT('Ctrl Pts',(-42.1219277727021,-57.8116356021288,
12.));
#136706=CARTESIAN_POINT('Ctrl Pts',(-42.1408854831783,-57.8248888437775,
12.));
#136707=CARTESIAN_POINT('Ctrl Pts',(-42.1598927470646,-57.8381486055342,
12.));
#136708=CARTESIAN_POINT('Ctrl Pts',(-42.1789494950794,-57.8514147589972,
12.));
#136709=CARTESIAN_POINT('Ctrl Pts',(-42.1980556581665,-57.864687176387,
12.));
#136710=CARTESIAN_POINT('Ctrl Pts',(-42.2172111674938,-57.8779657305413,
12.));
#136711=CARTESIAN_POINT('Ctrl Pts',(-42.2364159544501,-57.8912502949096,
12.));
#136712=CARTESIAN_POINT('Ctrl Pts',(-42.2556699506353,-57.9045407435474,
12.));
#136713=CARTESIAN_POINT('Ctrl Pts',(-42.2749730878594,-57.9178369511114,
12.));
#136714=CARTESIAN_POINT('Ctrl Pts',(-42.2943252981489,-57.9311387928563,
12.));
#136715=CARTESIAN_POINT('Ctrl Pts',(-42.3137265137452,-57.9444461446299,
12.));
#136716=CARTESIAN_POINT('Ctrl Pts',(-42.333176667102,-57.9577588828682,
12.));
#136717=CARTESIAN_POINT('Ctrl Pts',(-42.3526756908746,-57.9710768845899,
12.));
#136718=CARTESIAN_POINT('Ctrl Pts',(-42.3722235179197,-57.9844000273911,
12.));
#136719=CARTESIAN_POINT('Ctrl Pts',(-42.3918200813014,-57.9977281894422,
12.));
#136720=CARTESIAN_POINT('Ctrl Pts',(-42.411465314289,-58.0110612494828,
12.));
#136721=CARTESIAN_POINT('Ctrl Pts',(-42.4311591503555,-58.0243990868181,
12.));
#136722=CARTESIAN_POINT('Ctrl Pts',(-42.4509015231674,-58.037741581314,
12.));
#136723=CARTESIAN_POINT('Ctrl Pts',(-42.4706923665845,-58.0510886133926,
12.));
#136724=CARTESIAN_POINT('Ctrl Pts',(-42.4905316146653,-58.0644400640275,
12.));
#136725=CARTESIAN_POINT('Ctrl Pts',(-42.5104192016664,-58.0777958147403,
12.));
#136726=CARTESIAN_POINT('Ctrl Pts',(-42.5303550620387,-58.0911557475965,
12.));
#136727=CARTESIAN_POINT('Ctrl Pts',(-42.5503391304183,-58.1045197452002,
12.));
#136728=CARTESIAN_POINT('Ctrl Pts',(-42.5703713416265,-58.1178876906907,
12.));
#136729=CARTESIAN_POINT('Ctrl Pts',(-42.5904516306762,-58.1312594677386,
12.));
#136730=CARTESIAN_POINT('Ctrl Pts',(-42.6105799327699,-58.1446349605421,
12.));
#136731=CARTESIAN_POINT('Ctrl Pts',(-42.6307561832976,-58.1580140538228,
12.));
#136732=CARTESIAN_POINT('Ctrl Pts',(-42.6509803178265,-58.171396632821,
12.));
#136733=CARTESIAN_POINT('Ctrl Pts',(-42.6712522721016,-58.1847825832923,
12.));
#136734=CARTESIAN_POINT('Ctrl Pts',(-42.6915719820513,-58.1981717915037,
12.));
#136735=CARTESIAN_POINT('Ctrl Pts',(-42.7119393837866,-58.21156414423,12.));
#136736=CARTESIAN_POINT('Ctrl Pts',(-42.7323544135985,-58.22495952875,12.));
#136737=CARTESIAN_POINT('Ctrl Pts',(-42.7528170079484,-58.2383578328424,
12.));
#136738=CARTESIAN_POINT('Ctrl Pts',(-42.7733271034679,-58.251758944782,
12.));
#136739=CARTESIAN_POINT('Ctrl Pts',(-42.7938846369651,-58.2651627533368,
12.));
#136740=CARTESIAN_POINT('Ctrl Pts',(-42.8144895454233,-58.2785691477638,
12.));
#136741=CARTESIAN_POINT('Ctrl Pts',(-42.8351417659999,-58.2919780178064,
12.));
#136742=CARTESIAN_POINT('Ctrl Pts',(-42.8558412360158,-58.3053892536894,
12.));
#136743=CARTESIAN_POINT('Ctrl Pts',(-42.8765878929551,-58.3188027461164,
12.));
#136744=CARTESIAN_POINT('Ctrl Pts',(-42.8973816744709,-58.3322183862654,
12.));
#136745=CARTESIAN_POINT('Ctrl Pts',(-42.9182225183855,-58.3456360657865,
12.));
#136746=CARTESIAN_POINT('Ctrl Pts',(-42.9391103626879,-58.3590556767978,
12.));
#136747=CARTESIAN_POINT('Ctrl Pts',(-42.960045145526,-58.3724771118826,
12.));
#136748=CARTESIAN_POINT('Ctrl Pts',(-42.9810268052032,-58.3859002640856,
12.));
#136749=CARTESIAN_POINT('Ctrl Pts',(-43.0020552801859,-58.3993250269101,
12.));
#136750=CARTESIAN_POINT('Ctrl Pts',(-43.0231305091027,-58.4127512943136,
12.));
#136751=CARTESIAN_POINT('Ctrl Pts',(-43.0442524307434,-58.4261789607058,
12.));
#136752=CARTESIAN_POINT('Ctrl Pts',(-43.0654209840511,-58.439607920945,
12.));
#136753=CARTESIAN_POINT('Ctrl Pts',(-43.0866361081177,-58.4530380703348,
12.));
#136754=CARTESIAN_POINT('Ctrl Pts',(-43.1078977421916,-58.4664693046217,
12.));
#136755=CARTESIAN_POINT('Ctrl Pts',(-43.1292058256777,-58.4799015199907,
12.));
#136756=CARTESIAN_POINT('Ctrl Pts',(-43.1505602981365,-58.4933346130636,
12.));
#136757=CARTESIAN_POINT('Ctrl Pts',(-43.1719610992771,-58.5067684808944,
12.));
#136758=CARTESIAN_POINT('Ctrl Pts',(-43.1934081689505,-58.5202030209669,
12.));
#136759=CARTESIAN_POINT('Ctrl Pts',(-43.2149014471574,-58.5336381311917,
12.));
#136760=CARTESIAN_POINT('Ctrl Pts',(-43.2364408740493,-58.5470737099032,
12.));
#136761=CARTESIAN_POINT('Ctrl Pts',(-43.2580263899278,-58.5605096558578,
12.));
#136762=CARTESIAN_POINT('Ctrl Pts',(-43.27965793524,-58.573945868231,12.));
#136763=CARTESIAN_POINT('Ctrl Pts',(-43.3013354505701,-58.5873822466152,
12.));
#136764=CARTESIAN_POINT('Ctrl Pts',(-43.3230588766449,-58.6008186910156,
12.));
#136765=CARTESIAN_POINT('Ctrl Pts',(-43.3448281543371,-58.6142551018467,
12.));
#136766=CARTESIAN_POINT('Ctrl Pts',(-43.3666432246635,-58.627691379929,
12.));
#136767=CARTESIAN_POINT('Ctrl Pts',(-43.388504028781,-58.6411274264857,
12.));
#136768=CARTESIAN_POINT('Ctrl Pts',(-43.4104105079768,-58.6545631431393,
12.));
#136769=CARTESIAN_POINT('Ctrl Pts',(-43.4323626036737,-58.6679984319097,
12.));
#136770=CARTESIAN_POINT('Ctrl Pts',(-43.4543602574351,-58.6814331952138,
12.));
#136771=CARTESIAN_POINT('Ctrl Pts',(-43.4764034109654,-58.6948673358638,
12.));
#136772=CARTESIAN_POINT('Ctrl Pts',(-43.4984920061073,-58.7083007570661,
12.));
#136773=CARTESIAN_POINT('Ctrl Pts',(-43.5206259848337,-58.7217333624209,
12.));
#136774=CARTESIAN_POINT('Ctrl Pts',(-43.5428052892488,-58.735165055918,
12.));
#136775=CARTESIAN_POINT('Ctrl Pts',(-43.5650298615917,-58.74859574193,12.));
#136776=CARTESIAN_POINT('Ctrl Pts',(-43.5872996442345,-58.7620253252062,
12.));
#136777=CARTESIAN_POINT('Ctrl Pts',(-43.6096145796797,-58.775453710867,
12.));
#136778=CARTESIAN_POINT('Ctrl Pts',(-43.6319746105482,-58.788880804397,
12.));
#136779=CARTESIAN_POINT('Ctrl Pts',(-43.6543796795789,-58.8023065116436,
12.));
#136780=CARTESIAN_POINT('Ctrl Pts',(-43.6768297296395,-58.8157307388238,
12.));
#136781=CARTESIAN_POINT('Ctrl Pts',(-43.6993247037314,-58.8291533925293,
12.));
#136782=CARTESIAN_POINT('Ctrl Pts',(-43.7218645449922,-58.8425743797326,
12.));
#136783=CARTESIAN_POINT('Ctrl Pts',(-43.7444491966942,-58.855993607794,
12.));
#136784=CARTESIAN_POINT('Ctrl Pts',(-43.7670786022402,-58.8694109844648,
12.));
#136785=CARTESIAN_POINT('Ctrl Pts',(-43.7897527051609,-58.8828264178621,
12.));
#136786=CARTESIAN_POINT('Ctrl Pts',(-43.8124714491076,-58.8962398164493,
12.));
#136787=CARTESIAN_POINT('Ctrl Pts',(-43.835234777842,-58.9096510890129,
12.));
#136788=CARTESIAN_POINT('Ctrl Pts',(-43.858042635223,-58.9230601446436,
12.));
#136789=CARTESIAN_POINT('Ctrl Pts',(-43.8808949651873,-58.936466892712,
12.));
#136790=CARTESIAN_POINT('Ctrl Pts',(-43.9037917117739,-58.9498712429054,
12.));
#136791=CARTESIAN_POINT('Ctrl Pts',(-43.9267328191501,-58.9632731052696,
12.));
#136792=CARTESIAN_POINT('Ctrl Pts',(-43.9497182316331,-58.9766723902529,
12.));
#136793=CARTESIAN_POINT('Ctrl Pts',(-43.9727478937056,-58.9900690087408,
12.));
#136794=CARTESIAN_POINT('Ctrl Pts',(-43.9958217500369,-59.0034628721168,
12.));
#136795=CARTESIAN_POINT('Ctrl Pts',(-44.0189397454599,-59.0168538922095,
12.));
#136796=CARTESIAN_POINT('Ctrl Pts',(-44.0421018249223,-59.0302419811777,
12.));
#136797=CARTESIAN_POINT('Ctrl Pts',(-44.0653079334385,-59.0436270514087,
12.));
#136798=CARTESIAN_POINT('Ctrl Pts',(-44.0885580160432,-59.0570090154243,
12.));
#136799=CARTESIAN_POINT('Ctrl Pts',(-44.1118520177221,-59.0703877857526,
12.));
#136800=CARTESIAN_POINT('Ctrl Pts',(-44.1351898834051,-59.08376327492,12.));
#136801=CARTESIAN_POINT('Ctrl Pts',(-44.1585715581064,-59.0971353957206,
12.));
#136802=CARTESIAN_POINT('Ctrl Pts',(-44.1819969870307,-59.1105040614276,
12.));
#136803=CARTESIAN_POINT('Ctrl Pts',(-44.2054661156875,-59.1238691860306,
12.));
#136804=CARTESIAN_POINT('Ctrl Pts',(-44.228978889997,-59.1372306844586,
12.));
#136805=CARTESIAN_POINT('Ctrl Pts',(-44.2525352563996,-59.1505884728215,
12.));
#136806=CARTESIAN_POINT('Ctrl Pts',(-44.2761351616048,-59.1639424678793,
12.));
#136807=CARTESIAN_POINT('Ctrl Pts',(-44.2997785523431,-59.1772925865213,
12.));
#136808=CARTESIAN_POINT('Ctrl Pts',(-44.3234653750884,-59.1906387451979,
12.));
#136809=CARTESIAN_POINT('Ctrl Pts',(-44.3471955758403,-59.2039808594752,
12.));
#136810=CARTESIAN_POINT('Ctrl Pts',(-44.3709690997469,-59.2173188432798,
12.));
#136811=CARTESIAN_POINT('Ctrl Pts',(-44.3947858914074,-59.2306526095131,
12.));
#136812=CARTESIAN_POINT('Ctrl Pts',(-44.4186458955451,-59.2439820714187,
12.));
#136813=CARTESIAN_POINT('Ctrl Pts',(-44.4425490575911,-59.2573071437774,
12.));
#136814=CARTESIAN_POINT('Ctrl Pts',(-44.4664953242379,-59.2706277440445,
12.));
#136815=CARTESIAN_POINT('Ctrl Pts',(-44.490484644151,-59.2839437938237,
12.));
#136816=CARTESIAN_POINT('Ctrl Pts',(-44.5145169681349,-59.2972552192156,
12.));
#136817=CARTESIAN_POINT('Ctrl Pts',(-44.5351541478479,-59.3086616639523,
12.));
#136818=CARTESIAN_POINT('Ctrl Pts',(-44.5509994358154,-59.3174041872347,
12.));
#136819=CARTESIAN_POINT('Ctrl Pts',(-44.5620338188738,-59.3234848865455,
12.));
#136820=CARTESIAN_POINT('Ctrl Pts',(-44.5682447396021,-59.3269051738423,
12.));
#136821=CARTESIAN_POINT('Ctrl Pts',(-44.5696260757792,-59.3276657444392,
12.));
#136822=CARTESIAN_POINT('',(-40.8467768343956,-56.8466430164621,0.));
#136823=CARTESIAN_POINT('',(-40.8467768343956,-56.8466430164621,0.));
#136824=CARTESIAN_POINT('Ctrl Pts',(-44.5696260757791,-59.3276657444392,
0.));
#136825=CARTESIAN_POINT('Ctrl Pts',(-44.5682447396021,-59.3269051738423,
0.));
#136826=CARTESIAN_POINT('Ctrl Pts',(-44.5620338188738,-59.3234848865455,
0.));
#136827=CARTESIAN_POINT('Ctrl Pts',(-44.5509994358154,-59.3174041872347,
0.));
#136828=CARTESIAN_POINT('Ctrl Pts',(-44.5351541478479,-59.3086616639523,
0.));
#136829=CARTESIAN_POINT('Ctrl Pts',(-44.5145169681349,-59.2972552192156,
0.));
#136830=CARTESIAN_POINT('Ctrl Pts',(-44.490484644151,-59.2839437938237,
0.));
#136831=CARTESIAN_POINT('Ctrl Pts',(-44.4664953242379,-59.2706277440445,
0.));
#136832=CARTESIAN_POINT('Ctrl Pts',(-44.4425490575911,-59.2573071437774,
0.));
#136833=CARTESIAN_POINT('Ctrl Pts',(-44.4186458955451,-59.2439820714187,
0.));
#136834=CARTESIAN_POINT('Ctrl Pts',(-44.3947858914074,-59.2306526095131,
0.));
#136835=CARTESIAN_POINT('Ctrl Pts',(-44.3709690997469,-59.2173188432798,
0.));
#136836=CARTESIAN_POINT('Ctrl Pts',(-44.3471955758403,-59.2039808594752,
0.));
#136837=CARTESIAN_POINT('Ctrl Pts',(-44.3234653750884,-59.1906387451979,
0.));
#136838=CARTESIAN_POINT('Ctrl Pts',(-44.2997785523431,-59.1772925865213,
0.));
#136839=CARTESIAN_POINT('Ctrl Pts',(-44.2761351616048,-59.1639424678793,
0.));
#136840=CARTESIAN_POINT('Ctrl Pts',(-44.2525352563996,-59.1505884728215,
0.));
#136841=CARTESIAN_POINT('Ctrl Pts',(-44.228978889997,-59.1372306844586,
0.));
#136842=CARTESIAN_POINT('Ctrl Pts',(-44.2054661156875,-59.1238691860306,
0.));
#136843=CARTESIAN_POINT('Ctrl Pts',(-44.1819969870307,-59.1105040614276,
0.));
#136844=CARTESIAN_POINT('Ctrl Pts',(-44.1585715581064,-59.0971353957206,
0.));
#136845=CARTESIAN_POINT('Ctrl Pts',(-44.1351898834051,-59.08376327492,0.));
#136846=CARTESIAN_POINT('Ctrl Pts',(-44.1118520177221,-59.0703877857526,
0.));
#136847=CARTESIAN_POINT('Ctrl Pts',(-44.0885580160432,-59.0570090154243,
0.));
#136848=CARTESIAN_POINT('Ctrl Pts',(-44.0653079334385,-59.0436270514087,
0.));
#136849=CARTESIAN_POINT('Ctrl Pts',(-44.0421018249223,-59.0302419811777,
0.));
#136850=CARTESIAN_POINT('Ctrl Pts',(-44.0189397454599,-59.0168538922095,
0.));
#136851=CARTESIAN_POINT('Ctrl Pts',(-43.9958217500369,-59.0034628721168,
0.));
#136852=CARTESIAN_POINT('Ctrl Pts',(-43.9727478937056,-58.9900690087408,
0.));
#136853=CARTESIAN_POINT('Ctrl Pts',(-43.9497182316331,-58.9766723902529,
0.));
#136854=CARTESIAN_POINT('Ctrl Pts',(-43.9267328191501,-58.9632731052696,
0.));
#136855=CARTESIAN_POINT('Ctrl Pts',(-43.9037917117739,-58.9498712429054,
0.));
#136856=CARTESIAN_POINT('Ctrl Pts',(-43.8808949651873,-58.936466892712,
0.));
#136857=CARTESIAN_POINT('Ctrl Pts',(-43.858042635223,-58.9230601446436,
0.));
#136858=CARTESIAN_POINT('Ctrl Pts',(-43.835234777842,-58.9096510890129,
0.));
#136859=CARTESIAN_POINT('Ctrl Pts',(-43.8124714491076,-58.8962398164493,
0.));
#136860=CARTESIAN_POINT('Ctrl Pts',(-43.7897527051609,-58.8828264178621,
0.));
#136861=CARTESIAN_POINT('Ctrl Pts',(-43.7670786022402,-58.8694109844648,
0.));
#136862=CARTESIAN_POINT('Ctrl Pts',(-43.7444491966942,-58.855993607794,
0.));
#136863=CARTESIAN_POINT('Ctrl Pts',(-43.7218645449922,-58.8425743797326,
0.));
#136864=CARTESIAN_POINT('Ctrl Pts',(-43.6993247037314,-58.8291533925293,
0.));
#136865=CARTESIAN_POINT('Ctrl Pts',(-43.6768297296395,-58.8157307388238,
0.));
#136866=CARTESIAN_POINT('Ctrl Pts',(-43.6543796795789,-58.8023065116436,
0.));
#136867=CARTESIAN_POINT('Ctrl Pts',(-43.6319746105482,-58.788880804397,
0.));
#136868=CARTESIAN_POINT('Ctrl Pts',(-43.6096145796797,-58.775453710867,
0.));
#136869=CARTESIAN_POINT('Ctrl Pts',(-43.5872996442345,-58.7620253252062,
0.));
#136870=CARTESIAN_POINT('Ctrl Pts',(-43.5650298615917,-58.74859574193,0.));
#136871=CARTESIAN_POINT('Ctrl Pts',(-43.5428052892488,-58.735165055918,
0.));
#136872=CARTESIAN_POINT('Ctrl Pts',(-43.5206259848337,-58.7217333624209,
0.));
#136873=CARTESIAN_POINT('Ctrl Pts',(-43.4984920061073,-58.7083007570661,
0.));
#136874=CARTESIAN_POINT('Ctrl Pts',(-43.4764034109654,-58.6948673358638,
0.));
#136875=CARTESIAN_POINT('Ctrl Pts',(-43.4543602574351,-58.6814331952138,
0.));
#136876=CARTESIAN_POINT('Ctrl Pts',(-43.4323626036737,-58.6679984319097,
0.));
#136877=CARTESIAN_POINT('Ctrl Pts',(-43.4104105079768,-58.6545631431393,
0.));
#136878=CARTESIAN_POINT('Ctrl Pts',(-43.388504028781,-58.6411274264857,
0.));
#136879=CARTESIAN_POINT('Ctrl Pts',(-43.3666432246635,-58.627691379929,
0.));
#136880=CARTESIAN_POINT('Ctrl Pts',(-43.3448281543371,-58.6142551018467,
0.));
#136881=CARTESIAN_POINT('Ctrl Pts',(-43.3230588766449,-58.6008186910156,
0.));
#136882=CARTESIAN_POINT('Ctrl Pts',(-43.3013354505701,-58.5873822466152,
0.));
#136883=CARTESIAN_POINT('Ctrl Pts',(-43.27965793524,-58.573945868231,0.));
#136884=CARTESIAN_POINT('Ctrl Pts',(-43.2580263899278,-58.5605096558578,
0.));
#136885=CARTESIAN_POINT('Ctrl Pts',(-43.2364408740493,-58.5470737099032,
0.));
#136886=CARTESIAN_POINT('Ctrl Pts',(-43.2149014471574,-58.5336381311917,
0.));
#136887=CARTESIAN_POINT('Ctrl Pts',(-43.1934081689505,-58.5202030209669,
0.));
#136888=CARTESIAN_POINT('Ctrl Pts',(-43.1719610992771,-58.5067684808944,
0.));
#136889=CARTESIAN_POINT('Ctrl Pts',(-43.1505602981365,-58.4933346130636,
0.));
#136890=CARTESIAN_POINT('Ctrl Pts',(-43.1292058256777,-58.4799015199907,
0.));
#136891=CARTESIAN_POINT('Ctrl Pts',(-43.1078977421916,-58.4664693046217,
0.));
#136892=CARTESIAN_POINT('Ctrl Pts',(-43.0866361081177,-58.4530380703348,
0.));
#136893=CARTESIAN_POINT('Ctrl Pts',(-43.0654209840511,-58.439607920945,
0.));
#136894=CARTESIAN_POINT('Ctrl Pts',(-43.0442524307434,-58.4261789607058,
0.));
#136895=CARTESIAN_POINT('Ctrl Pts',(-43.0231305091027,-58.4127512943136,
0.));
#136896=CARTESIAN_POINT('Ctrl Pts',(-43.0020552801859,-58.3993250269101,
0.));
#136897=CARTESIAN_POINT('Ctrl Pts',(-42.9810268052032,-58.3859002640856,
0.));
#136898=CARTESIAN_POINT('Ctrl Pts',(-42.960045145526,-58.3724771118826,
0.));
#136899=CARTESIAN_POINT('Ctrl Pts',(-42.9391103626879,-58.3590556767978,
0.));
#136900=CARTESIAN_POINT('Ctrl Pts',(-42.9182225183855,-58.3456360657865,
0.));
#136901=CARTESIAN_POINT('Ctrl Pts',(-42.8973816744709,-58.3322183862654,
0.));
#136902=CARTESIAN_POINT('Ctrl Pts',(-42.8765878929551,-58.3188027461164,
0.));
#136903=CARTESIAN_POINT('Ctrl Pts',(-42.8558412360158,-58.3053892536894,
0.));
#136904=CARTESIAN_POINT('Ctrl Pts',(-42.8351417659999,-58.2919780178064,
0.));
#136905=CARTESIAN_POINT('Ctrl Pts',(-42.8144895454233,-58.2785691477638,
0.));
#136906=CARTESIAN_POINT('Ctrl Pts',(-42.7938846369651,-58.2651627533368,
0.));
#136907=CARTESIAN_POINT('Ctrl Pts',(-42.7733271034679,-58.251758944782,
0.));
#136908=CARTESIAN_POINT('Ctrl Pts',(-42.7528170079484,-58.2383578328424,
0.));
#136909=CARTESIAN_POINT('Ctrl Pts',(-42.7323544135985,-58.22495952875,0.));
#136910=CARTESIAN_POINT('Ctrl Pts',(-42.7119393837866,-58.21156414423,0.));
#136911=CARTESIAN_POINT('Ctrl Pts',(-42.6915719820513,-58.1981717915037,
0.));
#136912=CARTESIAN_POINT('Ctrl Pts',(-42.6712522721016,-58.1847825832923,
0.));
#136913=CARTESIAN_POINT('Ctrl Pts',(-42.6509803178265,-58.171396632821,
0.));
#136914=CARTESIAN_POINT('Ctrl Pts',(-42.6307561832976,-58.1580140538228,
0.));
#136915=CARTESIAN_POINT('Ctrl Pts',(-42.6105799327699,-58.1446349605421,
0.));
#136916=CARTESIAN_POINT('Ctrl Pts',(-42.5904516306762,-58.1312594677386,
0.));
#136917=CARTESIAN_POINT('Ctrl Pts',(-42.5703713416265,-58.1178876906907,
0.));
#136918=CARTESIAN_POINT('Ctrl Pts',(-42.5503391304183,-58.1045197452002,
0.));
#136919=CARTESIAN_POINT('Ctrl Pts',(-42.5303550620387,-58.0911557475965,
0.));
#136920=CARTESIAN_POINT('Ctrl Pts',(-42.5104192016664,-58.0777958147403,
0.));
#136921=CARTESIAN_POINT('Ctrl Pts',(-42.4905316146653,-58.0644400640275,
0.));
#136922=CARTESIAN_POINT('Ctrl Pts',(-42.4706923665845,-58.0510886133926,
0.));
#136923=CARTESIAN_POINT('Ctrl Pts',(-42.4509015231674,-58.037741581314,
0.));
#136924=CARTESIAN_POINT('Ctrl Pts',(-42.4311591503555,-58.0243990868181,
0.));
#136925=CARTESIAN_POINT('Ctrl Pts',(-42.411465314289,-58.0110612494828,
0.));
#136926=CARTESIAN_POINT('Ctrl Pts',(-42.3918200813014,-57.9977281894422,
0.));
#136927=CARTESIAN_POINT('Ctrl Pts',(-42.3722235179197,-57.9844000273911,
0.));
#136928=CARTESIAN_POINT('Ctrl Pts',(-42.3526756908746,-57.9710768845899,
0.));
#136929=CARTESIAN_POINT('Ctrl Pts',(-42.333176667102,-57.9577588828682,
0.));
#136930=CARTESIAN_POINT('Ctrl Pts',(-42.3137265137452,-57.9444461446299,
0.));
#136931=CARTESIAN_POINT('Ctrl Pts',(-42.2943252981489,-57.9311387928563,
0.));
#136932=CARTESIAN_POINT('Ctrl Pts',(-42.2749730878594,-57.9178369511114,
0.));
#136933=CARTESIAN_POINT('Ctrl Pts',(-42.2556699506353,-57.9045407435474,
0.));
#136934=CARTESIAN_POINT('Ctrl Pts',(-42.2364159544501,-57.8912502949096,
0.));
#136935=CARTESIAN_POINT('Ctrl Pts',(-42.2172111674938,-57.8779657305413,
0.));
#136936=CARTESIAN_POINT('Ctrl Pts',(-42.1980556581665,-57.864687176387,
0.));
#136937=CARTESIAN_POINT('Ctrl Pts',(-42.1789494950794,-57.8514147589972,
0.));
#136938=CARTESIAN_POINT('Ctrl Pts',(-42.1598927470646,-57.8381486055342,
0.));
#136939=CARTESIAN_POINT('Ctrl Pts',(-42.1408854831783,-57.8248888437775,
0.));
#136940=CARTESIAN_POINT('Ctrl Pts',(-42.1219277727021,-57.8116356021288,
0.));
#136941=CARTESIAN_POINT('Ctrl Pts',(-42.1030196851366,-57.798389009616,
0.));
#136942=CARTESIAN_POINT('Ctrl Pts',(-42.0841612902042,-57.7851491958987,
0.));
#136943=CARTESIAN_POINT('Ctrl Pts',(-42.0653526578588,-57.7719162912744,
0.));
#136944=CARTESIAN_POINT('Ctrl Pts',(-42.0465938582882,-57.7586904266834,
0.));
#136945=CARTESIAN_POINT('Ctrl Pts',(-42.0278849619148,-57.745471733714,
0.));
#136946=CARTESIAN_POINT('Ctrl Pts',(-42.0092260393897,-57.7322603446066,
0.));
#136947=CARTESIAN_POINT('Ctrl Pts',(-41.990617161596,-57.7190563922593,
0.));
#136948=CARTESIAN_POINT('Ctrl Pts',(-41.9720583996592,-57.7058600102351,
0.));
#136949=CARTESIAN_POINT('Ctrl Pts',(-41.9535498249488,-57.6926713327672,
0.));
#136950=CARTESIAN_POINT('Ctrl Pts',(-41.9350915090796,-57.6794904947649,
0.));
#136951=CARTESIAN_POINT('Ctrl Pts',(-41.9166835239054,-57.6663176318189,
0.));
#136952=CARTESIAN_POINT('Ctrl Pts',(-41.8983259415253,-57.6531528802072,
0.));
#136953=CARTESIAN_POINT('Ctrl Pts',(-41.8800188342912,-57.6399963769009,
0.));
#136954=CARTESIAN_POINT('Ctrl Pts',(-41.8617622748107,-57.6268482595701,
0.));
#136955=CARTESIAN_POINT('Ctrl Pts',(-41.8435563359456,-57.613708666588,
0.));
#136956=CARTESIAN_POINT('Ctrl Pts',(-41.8254010908051,-57.6005777370347,
0.));
#136957=CARTESIAN_POINT('Ctrl Pts',(-41.8072966127559,-57.5874556107054,
0.));
#136958=CARTESIAN_POINT('Ctrl Pts',(-41.7892429754298,-57.5743424281204,
0.));
#136959=CARTESIAN_POINT('Ctrl Pts',(-41.7712402527273,-57.561238330532,
0.));
#136960=CARTESIAN_POINT('Ctrl Pts',(-41.7532885188174,-57.5481434599334,
0.));
#136961=CARTESIAN_POINT('Ctrl Pts',(-41.7353878481336,-57.5350579590648,
0.));
#136962=CARTESIAN_POINT('Ctrl Pts',(-41.7175383153819,-57.5219819714169,
0.));
#136963=CARTESIAN_POINT('Ctrl Pts',(-41.6997399955445,-57.5089156412341,
0.));
#136964=CARTESIAN_POINT('Ctrl Pts',(-41.6819929638797,-57.4958591135165,
0.));
#136965=CARTESIAN_POINT('Ctrl Pts',(-41.6642972959168,-57.4828125340222,
0.));
#136966=CARTESIAN_POINT('Ctrl Pts',(-41.6466530674522,-57.4697760492693,
0.));
#136967=CARTESIAN_POINT('Ctrl Pts',(-41.6290603545674,-57.4567498065573,
0.));
#136968=CARTESIAN_POINT('Ctrl Pts',(-41.6115192336393,-57.4437339539848,
0.));
#136969=CARTESIAN_POINT('Ctrl Pts',(-41.5940297813474,-57.4307286404656,
0.));
#136970=CARTESIAN_POINT('Ctrl Pts',(-41.5765920746764,-57.417734015749,
0.));
#136971=CARTESIAN_POINT('Ctrl Pts',(-41.5592061909159,-57.4047502304207,
0.));
#136972=CARTESIAN_POINT('Ctrl Pts',(-41.5418722076558,-57.3917774358844,
0.));
#136973=CARTESIAN_POINT('Ctrl Pts',(-41.5245902027767,-57.378815784345,
0.));
#136974=CARTESIAN_POINT('Ctrl Pts',(-41.5073602544404,-57.3658654287948,
0.));
#136975=CARTESIAN_POINT('Ctrl Pts',(-41.4901824410654,-57.3529265229858,
0.));
#136976=CARTESIAN_POINT('Ctrl Pts',(-41.4730568413535,-57.339999221474,
0.));
#136977=CARTESIAN_POINT('Ctrl Pts',(-41.4559835343338,-57.3270836796925,
0.));
#136978=CARTESIAN_POINT('Ctrl Pts',(-41.4389625993948,-57.3141800540137,
0.));
#136979=CARTESIAN_POINT('Ctrl Pts',(-41.4219941163154,-57.3012885018139,
0.));
#136980=CARTESIAN_POINT('Ctrl Pts',(-41.4050781652923,-57.2884091815385,
0.));
#136981=CARTESIAN_POINT('Ctrl Pts',(-41.3882148268798,-57.2755422525822,
0.));
#136982=CARTESIAN_POINT('Ctrl Pts',(-41.3714041819215,-57.2626878751584,
0.));
#136983=CARTESIAN_POINT('Ctrl Pts',(-41.3546463114889,-57.2498462101883,
0.));
#136984=CARTESIAN_POINT('Ctrl Pts',(-41.3379412967889,-57.237017419142,
0.));
#136985=CARTESIAN_POINT('Ctrl Pts',(-41.321289219151,-57.2242016640226,
0.));
#136986=CARTESIAN_POINT('Ctrl Pts',(-41.304690160231,-57.2113991077325,
0.));
#136987=CARTESIAN_POINT('Ctrl Pts',(-41.2881442021869,-57.1986099143992,
0.));
#136988=CARTESIAN_POINT('Ctrl Pts',(-41.2716514278268,-57.1858342496526,
0.));
#136989=CARTESIAN_POINT('Ctrl Pts',(-41.2552119208445,-57.1730722810771,
0.));
#136990=CARTESIAN_POINT('Ctrl Pts',(-41.2388257656534,-57.1603241779042,
0.));
#136991=CARTESIAN_POINT('Ctrl Pts',(-41.2224930469412,-57.1475901101795,
0.));
#136992=CARTESIAN_POINT('Ctrl Pts',(-41.2062138492913,-57.1348702480644,
0.));
#136993=CARTESIAN_POINT('Ctrl Pts',(-41.1899882567941,-57.1221647611231,
0.));
#136994=CARTESIAN_POINT('Ctrl Pts',(-41.1738163525931,-57.1094738174998,
0.));
#136995=CARTESIAN_POINT('Ctrl Pts',(-41.1576982197402,-57.0967975854912,
0.));
#136996=CARTESIAN_POINT('Ctrl Pts',(-41.1416339422132,-57.0841362354281,
0.));
#136997=CARTESIAN_POINT('Ctrl Pts',(-41.1256236057436,-57.0714899412091,
0.));
#136998=CARTESIAN_POINT('Ctrl Pts',(-41.1096672990125,-57.0588588825266,
0.));
#136999=CARTESIAN_POINT('Ctrl Pts',(-41.0937651137519,-57.0462432450637,
0.));
#137000=CARTESIAN_POINT('Ctrl Pts',(-41.0779171422415,-57.0336432158503,
0.));
#137001=CARTESIAN_POINT('Ctrl Pts',(-41.0621234751,-57.0210589791777,0.));
#137002=CARTESIAN_POINT('Ctrl Pts',(-41.0463841993622,-57.008490713044,
0.));
#137003=CARTESIAN_POINT('Ctrl Pts',(-41.0306993954021,-56.9959385834768,
0.));
#137004=CARTESIAN_POINT('Ctrl Pts',(-41.0150691398988,-56.9834027500178,
0.));
#137005=CARTESIAN_POINT('Ctrl Pts',(-40.9994935117307,-56.9708833766183,
0.));
#137006=CARTESIAN_POINT('Ctrl Pts',(-40.9839725967121,-56.9583806404069,
0.));
#137007=CARTESIAN_POINT('Ctrl Pts',(-40.968506493303,-56.9458947422541,
0.));
#137008=CARTESIAN_POINT('Ctrl Pts',(-40.9530953164952,-56.9334259139928,
0.));
#137009=CARTESIAN_POINT('Ctrl Pts',(-40.9377391857044,-56.9209743960861,
0.));
#137010=CARTESIAN_POINT('Ctrl Pts',(-40.9224382132382,-56.9085404164432,
0.));
#137011=CARTESIAN_POINT('Ctrl Pts',(-40.9071924937551,-56.8961241708926,
0.));
#137012=CARTESIAN_POINT('Ctrl Pts',(-40.8920020903443,-56.8837257978574,
0.));
#137013=CARTESIAN_POINT('Ctrl Pts',(-40.8768670342278,-56.8713453765252,
0.));
#137014=CARTESIAN_POINT('Ctrl Pts',(-40.8648032759631,-56.8614554317993,
0.));
#137015=CARTESIAN_POINT('Ctrl Pts',(-40.8557803680411,-56.8540460739677,
0.));
#137016=CARTESIAN_POINT('Ctrl Pts',(-40.8497761671086,-56.8491101022668,
0.));
#137017=CARTESIAN_POINT('Ctrl Pts',(-40.8467768343956,-56.8466430164621,
0.));
#137018=CARTESIAN_POINT('Ctrl Pts',(-49.8690697110161,-55.3473204966403,
0.));
#137019=CARTESIAN_POINT('Ctrl Pts',(-49.8690697110161,-55.3473204966403,
12.));
#137020=CARTESIAN_POINT('Ctrl Pts',(-49.8639277221566,-55.3451131058826,
0.));
#137021=CARTESIAN_POINT('Ctrl Pts',(-49.8639277221566,-55.3451131058826,
12.));
#137022=CARTESIAN_POINT('Ctrl Pts',(-49.8536479176833,-55.34069740326,0.));
#137023=CARTESIAN_POINT('Ctrl Pts',(-49.8536479176833,-55.34069740326,12.));
#137024=CARTESIAN_POINT('Ctrl Pts',(-49.8382407307107,-55.3340710860055,
0.));
#137025=CARTESIAN_POINT('Ctrl Pts',(-49.8382407307107,-55.3340710860055,
12.));
#137026=CARTESIAN_POINT('Ctrl Pts',(-49.8177228552377,-55.3252304694602,
0.));
#137027=CARTESIAN_POINT('Ctrl Pts',(-49.8177228552377,-55.3252304694602,
12.));
#137028=CARTESIAN_POINT('Ctrl Pts',(-49.7921172540628,-55.3141704897766,
0.));
#137029=CARTESIAN_POINT('Ctrl Pts',(-49.7921172540628,-55.3141704897766,
12.));
#137030=CARTESIAN_POINT('Ctrl Pts',(-49.7665534128535,-55.3031013105853,
0.));
#137031=CARTESIAN_POINT('Ctrl Pts',(-49.7665534128535,-55.3031013105853,
12.));
#137032=CARTESIAN_POINT('Ctrl Pts',(-49.7410313576508,-55.2920229527546,
0.));
#137033=CARTESIAN_POINT('Ctrl Pts',(-49.7410313576508,-55.2920229527546,
12.));
#137034=CARTESIAN_POINT('Ctrl Pts',(-49.7155511248531,-55.2809354521515,
0.));
#137035=CARTESIAN_POINT('Ctrl Pts',(-49.7155511248531,-55.2809354521515,
12.));
#137036=CARTESIAN_POINT('Ctrl Pts',(-49.6901127631627,-55.2698388650025,
0.));
#137037=CARTESIAN_POINT('Ctrl Pts',(-49.6901127631627,-55.2698388650025,
12.));
#137038=CARTESIAN_POINT('Ctrl Pts',(-49.6647163322266,-55.2587332663783,
0.));
#137039=CARTESIAN_POINT('Ctrl Pts',(-49.6647163322266,-55.2587332663783,
12.));
#137040=CARTESIAN_POINT('Ctrl Pts',(-49.6393618987473,-55.2476187434057,
0.));
#137041=CARTESIAN_POINT('Ctrl Pts',(-49.6393618987473,-55.2476187434057,
12.));
#137042=CARTESIAN_POINT('Ctrl Pts',(-49.6140495332804,-55.2364953899358,
0.));
#137043=CARTESIAN_POINT('Ctrl Pts',(-49.6140495332804,-55.2364953899358,
12.));
#137044=CARTESIAN_POINT('Ctrl Pts',(-49.5887793068352,-55.2253633007666,
0.));
#137045=CARTESIAN_POINT('Ctrl Pts',(-49.5887793068352,-55.2253633007666,
12.));
#137046=CARTESIAN_POINT('Ctrl Pts',(-49.5635512873435,-55.2142225657013,
0.));
#137047=CARTESIAN_POINT('Ctrl Pts',(-49.5635512873435,-55.2142225657013,
12.));
#137048=CARTESIAN_POINT('Ctrl Pts',(-49.5383655368074,-55.2030732647312,
0.));
#137049=CARTESIAN_POINT('Ctrl Pts',(-49.5383655368074,-55.2030732647312,
12.));
#137050=CARTESIAN_POINT('Ctrl Pts',(-49.5132221132992,-55.1919154713647,
0.));
#137051=CARTESIAN_POINT('Ctrl Pts',(-49.5132221132992,-55.1919154713647,
12.));
#137052=CARTESIAN_POINT('Ctrl Pts',(-49.4881210723966,-55.1807492550119,
0.));
#137053=CARTESIAN_POINT('Ctrl Pts',(-49.4881210723966,-55.1807492550119,
12.));
#137054=CARTESIAN_POINT('Ctrl Pts',(-49.4630624688793,-55.1695746838174,
0.));
#137055=CARTESIAN_POINT('Ctrl Pts',(-49.4630624688793,-55.1695746838174,
12.));
#137056=CARTESIAN_POINT('Ctrl Pts',(-49.4380463581965,-55.1583918271116,
0.));
#137057=CARTESIAN_POINT('Ctrl Pts',(-49.4380463581965,-55.1583918271116,
12.));
#137058=CARTESIAN_POINT('Ctrl Pts',(-49.4130727983201,-55.1472007585183,
0.));
#137059=CARTESIAN_POINT('Ctrl Pts',(-49.4130727983201,-55.1472007585183,
12.));
#137060=CARTESIAN_POINT('Ctrl Pts',(-49.3881418495489,-55.1360015556221,
0.));
#137061=CARTESIAN_POINT('Ctrl Pts',(-49.3881418495489,-55.1360015556221,
12.));
#137062=CARTESIAN_POINT('Ctrl Pts',(-49.3632535736715,-55.1247942985619,
0.));
#137063=CARTESIAN_POINT('Ctrl Pts',(-49.3632535736715,-55.1247942985619,
12.));
#137064=CARTESIAN_POINT('Ctrl Pts',(-49.3384080333155,-55.1135790689464,
0.));
#137065=CARTESIAN_POINT('Ctrl Pts',(-49.3384080333155,-55.1135790689464,
12.));
#137066=CARTESIAN_POINT('Ctrl Pts',(-49.3136052912622,-55.102355948714,
0.));
#137067=CARTESIAN_POINT('Ctrl Pts',(-49.3136052912622,-55.102355948714,
12.));
#137068=CARTESIAN_POINT('Ctrl Pts',(-49.2888454096563,-55.0911250188302,
0.));
#137069=CARTESIAN_POINT('Ctrl Pts',(-49.2888454096563,-55.0911250188302,
12.));
#137070=CARTESIAN_POINT('Ctrl Pts',(-49.264128449652,-55.079886358701,0.));
#137071=CARTESIAN_POINT('Ctrl Pts',(-49.264128449652,-55.079886358701,12.));
#137072=CARTESIAN_POINT('Ctrl Pts',(-49.2394544718531,-55.0686400468931,
0.));
#137073=CARTESIAN_POINT('Ctrl Pts',(-49.2394544718531,-55.0686400468931,
12.));
#137074=CARTESIAN_POINT('Ctrl Pts',(-49.2148235365704,-55.0573861615579,
0.));
#137075=CARTESIAN_POINT('Ctrl Pts',(-49.2148235365704,-55.0573861615579,
12.));
#137076=CARTESIAN_POINT('Ctrl Pts',(-49.1902357041461,-55.0461247809744,
0.));
#137077=CARTESIAN_POINT('Ctrl Pts',(-49.1902357041461,-55.0461247809744,
12.));
#137078=CARTESIAN_POINT('Ctrl Pts',(-49.1656910352476,-55.0348559840453,
0.));
#137079=CARTESIAN_POINT('Ctrl Pts',(-49.1656910352476,-55.0348559840453,
12.));
#137080=CARTESIAN_POINT('Ctrl Pts',(-49.1411895911635,-55.0235798508045,
0.));
#137081=CARTESIAN_POINT('Ctrl Pts',(-49.1411895911635,-55.0235798508045,
12.));
#137082=CARTESIAN_POINT('Ctrl Pts',(-49.116731433673,-55.012296462186,0.));
#137083=CARTESIAN_POINT('Ctrl Pts',(-49.116731433673,-55.012296462186,12.));
#137084=CARTESIAN_POINT('Ctrl Pts',(-49.0923166249219,-55.0010058998107,
0.));
#137085=CARTESIAN_POINT('Ctrl Pts',(-49.0923166249219,-55.0010058998107,
12.));
#137086=CARTESIAN_POINT('Ctrl Pts',(-49.067945227287,-54.9897082457606,
0.));
#137087=CARTESIAN_POINT('Ctrl Pts',(-49.067945227287,-54.9897082457606,
12.));
#137088=CARTESIAN_POINT('Ctrl Pts',(-49.0436173032528,-54.9784035823766,
0.));
#137089=CARTESIAN_POINT('Ctrl Pts',(-49.0436173032528,-54.9784035823766,
12.));
#137090=CARTESIAN_POINT('Ctrl Pts',(-49.0193329152479,-54.9670919920029,
0.));
#137091=CARTESIAN_POINT('Ctrl Pts',(-49.0193329152479,-54.9670919920029,
12.));
#137092=CARTESIAN_POINT('Ctrl Pts',(-48.9950921256527,-54.9557735569943,
0.));
#137093=CARTESIAN_POINT('Ctrl Pts',(-48.9950921256527,-54.9557735569943,
12.));
#137094=CARTESIAN_POINT('Ctrl Pts',(-48.9708949968795,-54.9444483598378,
0.));
#137095=CARTESIAN_POINT('Ctrl Pts',(-48.9708949968795,-54.9444483598378,
12.));
#137096=CARTESIAN_POINT('Ctrl Pts',(-48.9467415914269,-54.9331164832424,
0.));
#137097=CARTESIAN_POINT('Ctrl Pts',(-48.9467415914269,-54.9331164832424,
12.));
#137098=CARTESIAN_POINT('Ctrl Pts',(-48.9226319719369,-54.9217780102355,
0.));
#137099=CARTESIAN_POINT('Ctrl Pts',(-48.9226319719369,-54.9217780102355,
12.));
#137100=CARTESIAN_POINT('Ctrl Pts',(-48.8985662012528,-54.9104330242742,
0.));
#137101=CARTESIAN_POINT('Ctrl Pts',(-48.8985662012528,-54.9104330242742,
12.));
#137102=CARTESIAN_POINT('Ctrl Pts',(-48.8745443424477,-54.8990816092953,
0.));
#137103=CARTESIAN_POINT('Ctrl Pts',(-48.8745443424477,-54.8990816092953,
12.));
#137104=CARTESIAN_POINT('Ctrl Pts',(-48.8505664587974,-54.8877238496566,
0.));
#137105=CARTESIAN_POINT('Ctrl Pts',(-48.8505664587974,-54.8877238496566,
12.));
#137106=CARTESIAN_POINT('Ctrl Pts',(-48.8266326137622,-54.8763598301037,
0.));
#137107=CARTESIAN_POINT('Ctrl Pts',(-48.8266326137622,-54.8763598301037,
12.));
#137108=CARTESIAN_POINT('Ctrl Pts',(-48.8027428709614,-54.8649896357285,
0.));
#137109=CARTESIAN_POINT('Ctrl Pts',(-48.8027428709614,-54.8649896357285,
12.));
#137110=CARTESIAN_POINT('Ctrl Pts',(-48.7788972941438,-54.8536133519292,
0.));
#137111=CARTESIAN_POINT('Ctrl Pts',(-48.7788972941438,-54.8536133519292,
12.));
#137112=CARTESIAN_POINT('Ctrl Pts',(-48.7550959471601,-54.8422310643763,
0.));
#137113=CARTESIAN_POINT('Ctrl Pts',(-48.7550959471601,-54.8422310643763,
12.));
#137114=CARTESIAN_POINT('Ctrl Pts',(-48.7313388939845,-54.8308428590344,
0.));
#137115=CARTESIAN_POINT('Ctrl Pts',(-48.7313388939845,-54.8308428590344,
12.));
#137116=CARTESIAN_POINT('Ctrl Pts',(-48.7076261987292,-54.819448822181,
0.));
#137117=CARTESIAN_POINT('Ctrl Pts',(-48.7076261987292,-54.819448822181,
12.));
#137118=CARTESIAN_POINT('Ctrl Pts',(-48.6839579256566,-54.8080490404275,
0.));
#137119=CARTESIAN_POINT('Ctrl Pts',(-48.6839579256566,-54.8080490404275,
12.));
#137120=CARTESIAN_POINT('Ctrl Pts',(-48.6603341391886,-54.796643600739,
0.));
#137121=CARTESIAN_POINT('Ctrl Pts',(-48.6603341391886,-54.796643600739,
12.));
#137122=CARTESIAN_POINT('Ctrl Pts',(-48.6367549039112,-54.7852325904583,
0.));
#137123=CARTESIAN_POINT('Ctrl Pts',(-48.6367549039112,-54.7852325904583,
12.));
#137124=CARTESIAN_POINT('Ctrl Pts',(-48.6132202845783,-54.7738160973032,
0.));
#137125=CARTESIAN_POINT('Ctrl Pts',(-48.6132202845783,-54.7738160973032,
12.));
#137126=CARTESIAN_POINT('Ctrl Pts',(-48.5897303461125,-54.7623942093586,
0.));
#137127=CARTESIAN_POINT('Ctrl Pts',(-48.5897303461125,-54.7623942093586,
12.));
#137128=CARTESIAN_POINT('Ctrl Pts',(-48.5662851536026,-54.7509670150714,
0.));
#137129=CARTESIAN_POINT('Ctrl Pts',(-48.5662851536026,-54.7509670150714,
12.));
#137130=CARTESIAN_POINT('Ctrl Pts',(-48.5428847722977,-54.7395346032453,
0.));
#137131=CARTESIAN_POINT('Ctrl Pts',(-48.5428847722977,-54.7395346032453,
12.));
#137132=CARTESIAN_POINT('Ctrl Pts',(-48.519529267596,-54.7280970630351,
0.));
#137133=CARTESIAN_POINT('Ctrl Pts',(-48.519529267596,-54.7280970630351,
12.));
#137134=CARTESIAN_POINT('Ctrl Pts',(-48.4962187050457,-54.716654483948,
0.));
#137135=CARTESIAN_POINT('Ctrl Pts',(-48.4962187050457,-54.716654483948,
12.));
#137136=CARTESIAN_POINT('Ctrl Pts',(-48.472953150357,-54.7052069558497,
0.));
#137137=CARTESIAN_POINT('Ctrl Pts',(-48.472953150357,-54.7052069558497,
12.));
#137138=CARTESIAN_POINT('Ctrl Pts',(-48.4497326694052,-54.6937545689695,
0.));
#137139=CARTESIAN_POINT('Ctrl Pts',(-48.4497326694052,-54.6937545689695,
12.));
#137140=CARTESIAN_POINT('Ctrl Pts',(-48.426557328234,-54.6822974139064,
0.));
#137141=CARTESIAN_POINT('Ctrl Pts',(-48.426557328234,-54.6822974139064,
12.));
#137142=CARTESIAN_POINT('Ctrl Pts',(-48.4034271930514,-54.6708355816358,
0.));
#137143=CARTESIAN_POINT('Ctrl Pts',(-48.4034271930514,-54.6708355816358,
12.));
#137144=CARTESIAN_POINT('Ctrl Pts',(-48.3803423302294,-54.6593691635145,
0.));
#137145=CARTESIAN_POINT('Ctrl Pts',(-48.3803423302294,-54.6593691635145,
12.));
#137146=CARTESIAN_POINT('Ctrl Pts',(-48.3573028063124,-54.6478982512794,
0.));
#137147=CARTESIAN_POINT('Ctrl Pts',(-48.3573028063124,-54.6478982512794,
12.));
#137148=CARTESIAN_POINT('Ctrl Pts',(-48.3343086880194,-54.6364229370494,
0.));
#137149=CARTESIAN_POINT('Ctrl Pts',(-48.3343086880194,-54.6364229370494,
12.));
#137150=CARTESIAN_POINT('Ctrl Pts',(-48.3113600422443,-54.6249433133261,
0.));
#137151=CARTESIAN_POINT('Ctrl Pts',(-48.3113600422443,-54.6249433133261,
12.));
#137152=CARTESIAN_POINT('Ctrl Pts',(-48.2884569360506,-54.6134594729959,
0.));
#137153=CARTESIAN_POINT('Ctrl Pts',(-48.2884569360506,-54.6134594729959,
12.));
#137154=CARTESIAN_POINT('Ctrl Pts',(-48.2655994366665,-54.6019715093309,
0.));
#137155=CARTESIAN_POINT('Ctrl Pts',(-48.2655994366665,-54.6019715093309,
12.));
#137156=CARTESIAN_POINT('Ctrl Pts',(-48.2427876114947,-54.5904795159926,
0.));
#137157=CARTESIAN_POINT('Ctrl Pts',(-48.2427876114947,-54.5904795159926,
12.));
#137158=CARTESIAN_POINT('Ctrl Pts',(-48.2200215281173,-54.5789835870342,
0.));
#137159=CARTESIAN_POINT('Ctrl Pts',(-48.2200215281173,-54.5789835870342,
12.));
#137160=CARTESIAN_POINT('Ctrl Pts',(-48.1973012542966,-54.5674838169041,
0.));
#137161=CARTESIAN_POINT('Ctrl Pts',(-48.1973012542966,-54.5674838169041,
12.));
#137162=CARTESIAN_POINT('Ctrl Pts',(-48.1746268579736,-54.5559803004492,
0.));
#137163=CARTESIAN_POINT('Ctrl Pts',(-48.1746268579736,-54.5559803004492,
12.));
#137164=CARTESIAN_POINT('Ctrl Pts',(-48.1519984072622,-54.5444731329201,
0.));
#137165=CARTESIAN_POINT('Ctrl Pts',(-48.1519984072622,-54.5444731329201,
12.));
#137166=CARTESIAN_POINT('Ctrl Pts',(-48.1294159704573,-54.5329624099721,
0.));
#137167=CARTESIAN_POINT('Ctrl Pts',(-48.1294159704573,-54.5329624099721,
12.));
#137168=CARTESIAN_POINT('Ctrl Pts',(-48.1068796160405,-54.5214482276678,
0.));
#137169=CARTESIAN_POINT('Ctrl Pts',(-48.1068796160405,-54.5214482276678,
12.));
#137170=CARTESIAN_POINT('Ctrl Pts',(-48.0843894126806,-54.5099306824786,
0.));
#137171=CARTESIAN_POINT('Ctrl Pts',(-48.0843894126806,-54.5099306824786,
12.));
#137172=CARTESIAN_POINT('Ctrl Pts',(-48.0619454292324,-54.4984098712886,
0.));
#137173=CARTESIAN_POINT('Ctrl Pts',(-48.0619454292324,-54.4984098712886,
12.));
#137174=CARTESIAN_POINT('Ctrl Pts',(-48.0395477347298,-54.4868858913971,
0.));
#137175=CARTESIAN_POINT('Ctrl Pts',(-48.0395477347298,-54.4868858913971,
12.));
#137176=CARTESIAN_POINT('Ctrl Pts',(-48.0171963983924,-54.4753588405215,
0.));
#137177=CARTESIAN_POINT('Ctrl Pts',(-48.0171963983924,-54.4753588405215,
12.));
#137178=CARTESIAN_POINT('Ctrl Pts',(-47.9948914896326,-54.4638288168003,
0.));
#137179=CARTESIAN_POINT('Ctrl Pts',(-47.9948914896326,-54.4638288168003,
12.));
#137180=CARTESIAN_POINT('Ctrl Pts',(-47.9726330780572,-54.4522959187955,
0.));
#137181=CARTESIAN_POINT('Ctrl Pts',(-47.9726330780572,-54.4522959187955,
12.));
#137182=CARTESIAN_POINT('Ctrl Pts',(-47.9504212334675,-54.4407602454967,
0.));
#137183=CARTESIAN_POINT('Ctrl Pts',(-47.9504212334675,-54.4407602454967,
12.));
#137184=CARTESIAN_POINT('Ctrl Pts',(-47.9282560258516,-54.429221896324,
0.));
#137185=CARTESIAN_POINT('Ctrl Pts',(-47.9282560258516,-54.429221896324,
12.));
#137186=CARTESIAN_POINT('Ctrl Pts',(-47.9061375253897,-54.4176809711311,
0.));
#137187=CARTESIAN_POINT('Ctrl Pts',(-47.9061375253897,-54.4176809711311,
12.));
#137188=CARTESIAN_POINT('Ctrl Pts',(-47.8840658024618,-54.4061375702079,
0.));
#137189=CARTESIAN_POINT('Ctrl Pts',(-47.8840658024618,-54.4061375702079,
12.));
#137190=CARTESIAN_POINT('Ctrl Pts',(-47.8620409276493,-54.3945917942832,
0.));
#137191=CARTESIAN_POINT('Ctrl Pts',(-47.8620409276493,-54.3945917942832,
12.));
#137192=CARTESIAN_POINT('Ctrl Pts',(-47.8400629717355,-54.3830437445279,
0.));
#137193=CARTESIAN_POINT('Ctrl Pts',(-47.8400629717355,-54.3830437445279,
12.));
#137194=CARTESIAN_POINT('Ctrl Pts',(-47.8181320056995,-54.3714935225591,
0.));
#137195=CARTESIAN_POINT('Ctrl Pts',(-47.8181320056995,-54.3714935225591,
12.));
#137196=CARTESIAN_POINT('Ctrl Pts',(-47.7962481007185,-54.3599412304438,
0.));
#137197=CARTESIAN_POINT('Ctrl Pts',(-47.7962481007185,-54.3599412304438,
12.));
#137198=CARTESIAN_POINT('Ctrl Pts',(-47.7744113281771,-54.3483869707002,
0.));
#137199=CARTESIAN_POINT('Ctrl Pts',(-47.7744113281771,-54.3483869707002,
12.));
#137200=CARTESIAN_POINT('Ctrl Pts',(-47.7526217596694,-54.3368308463023,
0.));
#137201=CARTESIAN_POINT('Ctrl Pts',(-47.7526217596694,-54.3368308463023,
12.));
#137202=CARTESIAN_POINT('Ctrl Pts',(-47.7308794669993,-54.3252729606823,
0.));
#137203=CARTESIAN_POINT('Ctrl Pts',(-47.7308794669993,-54.3252729606823,
12.));
#137204=CARTESIAN_POINT('Ctrl Pts',(-47.7091845221747,-54.3137134177345,
0.));
#137205=CARTESIAN_POINT('Ctrl Pts',(-47.7091845221747,-54.3137134177345,
12.));
#137206=CARTESIAN_POINT('Ctrl Pts',(-47.6875369974087,-54.302152321819,
0.));
#137207=CARTESIAN_POINT('Ctrl Pts',(-47.6875369974087,-54.302152321819,
12.));
#137208=CARTESIAN_POINT('Ctrl Pts',(-47.6659369651301,-54.290589777765,
0.));
#137209=CARTESIAN_POINT('Ctrl Pts',(-47.6659369651301,-54.290589777765,
12.));
#137210=CARTESIAN_POINT('Ctrl Pts',(-47.6443844979848,-54.2790258908738,
0.));
#137211=CARTESIAN_POINT('Ctrl Pts',(-47.6443844979848,-54.2790258908738,
12.));
#137212=CARTESIAN_POINT('Ctrl Pts',(-47.6228796688375,-54.2674607669226,
0.));
#137213=CARTESIAN_POINT('Ctrl Pts',(-47.6228796688375,-54.2674607669226,
12.));
#137214=CARTESIAN_POINT('Ctrl Pts',(-47.6014225507659,-54.2558945121678,
0.));
#137215=CARTESIAN_POINT('Ctrl Pts',(-47.6014225507659,-54.2558945121678,
12.));
#137216=CARTESIAN_POINT('Ctrl Pts',(-47.5800132170608,-54.244327233349,
0.));
#137217=CARTESIAN_POINT('Ctrl Pts',(-47.5800132170608,-54.244327233349,
12.));
#137218=CARTESIAN_POINT('Ctrl Pts',(-47.5586517412363,-54.2327590376924,
0.));
#137219=CARTESIAN_POINT('Ctrl Pts',(-47.5586517412363,-54.2327590376924,
12.));
#137220=CARTESIAN_POINT('Ctrl Pts',(-47.5373381970326,-54.2211900329138,
0.));
#137221=CARTESIAN_POINT('Ctrl Pts',(-47.5373381970326,-54.2211900329138,
12.));
#137222=CARTESIAN_POINT('Ctrl Pts',(-47.5160726584174,-54.209620327223,
0.));
#137223=CARTESIAN_POINT('Ctrl Pts',(-47.5160726584174,-54.209620327223,
12.));
#137224=CARTESIAN_POINT('Ctrl Pts',(-47.4948551995801,-54.198050029327,
0.));
#137225=CARTESIAN_POINT('Ctrl Pts',(-47.4948551995801,-54.198050029327,
12.));
#137226=CARTESIAN_POINT('Ctrl Pts',(-47.4736858949322,-54.1864792484345,
0.));
#137227=CARTESIAN_POINT('Ctrl Pts',(-47.4736858949322,-54.1864792484345,
12.));
#137228=CARTESIAN_POINT('Ctrl Pts',(-47.4525648191173,-54.1749080942593,
0.));
#137229=CARTESIAN_POINT('Ctrl Pts',(-47.4525648191173,-54.1749080942593,
12.));
#137230=CARTESIAN_POINT('Ctrl Pts',(-47.4314920470141,-54.1633366770239,
0.));
#137231=CARTESIAN_POINT('Ctrl Pts',(-47.4314920470141,-54.1633366770239,
12.));
#137232=CARTESIAN_POINT('Ctrl Pts',(-47.4104676537381,-54.1517651074637,
0.));
#137233=CARTESIAN_POINT('Ctrl Pts',(-47.4104676537381,-54.1517651074637,
12.));
#137234=CARTESIAN_POINT('Ctrl Pts',(-47.3894917146365,-54.1401934968311,
0.));
#137235=CARTESIAN_POINT('Ctrl Pts',(-47.3894917146365,-54.1401934968311,
12.));
#137236=CARTESIAN_POINT('Ctrl Pts',(-47.3685643052874,-54.1286219568989,
0.));
#137237=CARTESIAN_POINT('Ctrl Pts',(-47.3685643052874,-54.1286219568989,
12.));
#137238=CARTESIAN_POINT('Ctrl Pts',(-47.3476855015102,-54.1170505999645,
0.));
#137239=CARTESIAN_POINT('Ctrl Pts',(-47.3476855015102,-54.1170505999645,
12.));
#137240=CARTESIAN_POINT('Ctrl Pts',(-47.3268553793694,-54.1054795388543,
0.));
#137241=CARTESIAN_POINT('Ctrl Pts',(-47.3268553793694,-54.1054795388543,
12.));
#137242=CARTESIAN_POINT('Ctrl Pts',(-47.3060740151752,-54.0939088869269,
0.));
#137243=CARTESIAN_POINT('Ctrl Pts',(-47.3060740151752,-54.0939088869269,
12.));
#137244=CARTESIAN_POINT('Ctrl Pts',(-47.2853414854793,-54.0823387580776,
0.));
#137245=CARTESIAN_POINT('Ctrl Pts',(-47.2853414854793,-54.0823387580776,
12.));
#137246=CARTESIAN_POINT('Ctrl Pts',(-47.2646578670746,-54.0707692667438,
0.));
#137247=CARTESIAN_POINT('Ctrl Pts',(-47.2646578670746,-54.0707692667438,
12.));
#137248=CARTESIAN_POINT('Ctrl Pts',(-47.2440232370065,-54.0592005279086,
0.));
#137249=CARTESIAN_POINT('Ctrl Pts',(-47.2440232370065,-54.0592005279086,
12.));
#137250=CARTESIAN_POINT('Ctrl Pts',(-47.2234376725743,-54.047632657104,
0.));
#137251=CARTESIAN_POINT('Ctrl Pts',(-47.2234376725743,-54.047632657104,
12.));
#137252=CARTESIAN_POINT('Ctrl Pts',(-47.202901251334,-54.0360657704163,
0.));
#137253=CARTESIAN_POINT('Ctrl Pts',(-47.202901251334,-54.0360657704163,
12.));
#137254=CARTESIAN_POINT('Ctrl Pts',(-47.1824140510926,-54.0244999844893,
0.));
#137255=CARTESIAN_POINT('Ctrl Pts',(-47.1824140510926,-54.0244999844893,
12.));
#137256=CARTESIAN_POINT('Ctrl Pts',(-47.1619761499087,-54.0129354165297,
0.));
#137257=CARTESIAN_POINT('Ctrl Pts',(-47.1619761499087,-54.0129354165297,
12.));
#137258=CARTESIAN_POINT('Ctrl Pts',(-47.1415876261035,-54.0013721843118,
0.));
#137259=CARTESIAN_POINT('Ctrl Pts',(-47.1415876261035,-54.0013721843118,
12.));
#137260=CARTESIAN_POINT('Ctrl Pts',(-47.1212485582643,-53.989810406182,
0.));
#137261=CARTESIAN_POINT('Ctrl Pts',(-47.1212485582643,-53.989810406182,
12.));
#137262=CARTESIAN_POINT('Ctrl Pts',(-47.1009590252458,-53.9782502010634,
0.));
#137263=CARTESIAN_POINT('Ctrl Pts',(-47.1009590252458,-53.9782502010634,
12.));
#137264=CARTESIAN_POINT('Ctrl Pts',(-47.0807191061648,-53.9666916884596,
0.));
#137265=CARTESIAN_POINT('Ctrl Pts',(-47.0807191061648,-53.9666916884596,
12.));
#137266=CARTESIAN_POINT('Ctrl Pts',(-47.0605288804008,-53.95513498846,0.));
#137267=CARTESIAN_POINT('Ctrl Pts',(-47.0605288804008,-53.95513498846,12.));
#137268=CARTESIAN_POINT('Ctrl Pts',(-47.0403884276072,-53.9435802217436,
0.));
#137269=CARTESIAN_POINT('Ctrl Pts',(-47.0403884276072,-53.9435802217436,
12.));
#137270=CARTESIAN_POINT('Ctrl Pts',(-47.0202978277138,-53.9320275095853,
0.));
#137271=CARTESIAN_POINT('Ctrl Pts',(-47.0202978277138,-53.9320275095853,
12.));
#137272=CARTESIAN_POINT('Ctrl Pts',(-47.0002571609297,-53.9204769738596,
0.));
#137273=CARTESIAN_POINT('Ctrl Pts',(-47.0002571609297,-53.9204769738596,
12.));
#137274=CARTESIAN_POINT('Ctrl Pts',(-46.9802665077366,-53.9089287370463,
0.));
#137275=CARTESIAN_POINT('Ctrl Pts',(-46.9802665077366,-53.9089287370463,
12.));
#137276=CARTESIAN_POINT('Ctrl Pts',(-46.9603259488921,-53.8973829222348,
0.));
#137277=CARTESIAN_POINT('Ctrl Pts',(-46.9603259488921,-53.8973829222348,
12.));
#137278=CARTESIAN_POINT('Ctrl Pts',(-46.94043556544,-53.8858396531298,0.));
#137279=CARTESIAN_POINT('Ctrl Pts',(-46.94043556544,-53.8858396531298,12.));
#137280=CARTESIAN_POINT('Ctrl Pts',(-46.9205954387133,-53.8742990540563,
0.));
#137281=CARTESIAN_POINT('Ctrl Pts',(-46.9205954387133,-53.8742990540563,
12.));
#137282=CARTESIAN_POINT('Ctrl Pts',(-46.9008056503351,-53.8627612499638,
0.));
#137283=CARTESIAN_POINT('Ctrl Pts',(-46.9008056503351,-53.8627612499638,
12.));
#137284=CARTESIAN_POINT('Ctrl Pts',(-46.881066282213,-53.8512263664321,
0.));
#137285=CARTESIAN_POINT('Ctrl Pts',(-46.881066282213,-53.8512263664321,
12.));
#137286=CARTESIAN_POINT('Ctrl Pts',(-46.8613774165435,-53.8396945296757,
0.));
#137287=CARTESIAN_POINT('Ctrl Pts',(-46.8613774165435,-53.8396945296757,
12.));
#137288=CARTESIAN_POINT('Ctrl Pts',(-46.841739135822,-53.8281658665503,
0.));
#137289=CARTESIAN_POINT('Ctrl Pts',(-46.841739135822,-53.8281658665503,
12.));
#137290=CARTESIAN_POINT('Ctrl Pts',(-46.8221515228457,-53.816640504558,
0.));
#137291=CARTESIAN_POINT('Ctrl Pts',(-46.8221515228457,-53.816640504558,
12.));
#137292=CARTESIAN_POINT('Ctrl Pts',(-46.802614660715,-53.8051185718532,
0.));
#137293=CARTESIAN_POINT('Ctrl Pts',(-46.802614660715,-53.8051185718532,
12.));
#137294=CARTESIAN_POINT('Ctrl Pts',(-46.7831286328278,-53.793600197248,
0.));
#137295=CARTESIAN_POINT('Ctrl Pts',(-46.7831286328278,-53.793600197248,
12.));
#137296=CARTESIAN_POINT('Ctrl Pts',(-46.763693522886,-53.7820855102182,
0.));
#137297=CARTESIAN_POINT('Ctrl Pts',(-46.763693522886,-53.7820855102182,
12.));
#137298=CARTESIAN_POINT('Ctrl Pts',(-46.7443094149045,-53.7705746409076,
0.));
#137299=CARTESIAN_POINT('Ctrl Pts',(-46.7443094149045,-53.7705746409076,
12.));
#137300=CARTESIAN_POINT('Ctrl Pts',(-46.7249763932129,-53.7590677201342,
0.));
#137301=CARTESIAN_POINT('Ctrl Pts',(-46.7249763932129,-53.7590677201342,
12.));
#137302=CARTESIAN_POINT('Ctrl Pts',(-46.7056945424559,-53.7475648793946,
0.));
#137303=CARTESIAN_POINT('Ctrl Pts',(-46.7056945424559,-53.7475648793946,
12.));
#137304=CARTESIAN_POINT('Ctrl Pts',(-46.6864639475862,-53.7360662508675,
0.));
#137305=CARTESIAN_POINT('Ctrl Pts',(-46.6864639475862,-53.7360662508675,
12.));
#137306=CARTESIAN_POINT('Ctrl Pts',(-46.6672846938752,-53.7245719674221,
0.));
#137307=CARTESIAN_POINT('Ctrl Pts',(-46.6672846938752,-53.7245719674221,
12.));
#137308=CARTESIAN_POINT('Ctrl Pts',(-46.6481568669217,-53.7130821626262,
0.));
#137309=CARTESIAN_POINT('Ctrl Pts',(-46.6481568669217,-53.7130821626262,
12.));
#137310=CARTESIAN_POINT('Ctrl Pts',(-46.6290805526559,-53.7015969707541,
0.));
#137311=CARTESIAN_POINT('Ctrl Pts',(-46.6290805526559,-53.7015969707541,
12.));
#137312=CARTESIAN_POINT('Ctrl Pts',(-46.6100558373401,-53.690116526794,
0.));
#137313=CARTESIAN_POINT('Ctrl Pts',(-46.6100558373401,-53.690116526794,
12.));
#137314=CARTESIAN_POINT('Ctrl Pts',(-46.5910828075652,-53.678640966456,
0.));
#137315=CARTESIAN_POINT('Ctrl Pts',(-46.5910828075652,-53.678640966456,
12.));
#137316=CARTESIAN_POINT('Ctrl Pts',(-46.572161550259,-53.6671704261735,
0.));
#137317=CARTESIAN_POINT('Ctrl Pts',(-46.572161550259,-53.6671704261735,
12.));
#137318=CARTESIAN_POINT('Ctrl Pts',(-46.5532921526899,-53.6557050431069,
0.));
#137319=CARTESIAN_POINT('Ctrl Pts',(-46.5532921526899,-53.6557050431069,
12.));
#137320=CARTESIAN_POINT('Ctrl Pts',(-46.5344747024677,-53.6442449551455,
0.));
#137321=CARTESIAN_POINT('Ctrl Pts',(-46.5344747024677,-53.6442449551455,
12.));
#137322=CARTESIAN_POINT('Ctrl Pts',(-46.5157092875377,-53.6327903009098,
0.));
#137323=CARTESIAN_POINT('Ctrl Pts',(-46.5157092875377,-53.6327903009098,
12.));
#137324=CARTESIAN_POINT('Ctrl Pts',(-46.4969959961779,-53.6213412197542,
0.));
#137325=CARTESIAN_POINT('Ctrl Pts',(-46.4969959961779,-53.6213412197542,
12.));
#137326=CARTESIAN_POINT('Ctrl Pts',(-46.4783349170182,-53.6098978517869,
0.));
#137327=CARTESIAN_POINT('Ctrl Pts',(-46.4783349170182,-53.6098978517869,
12.));
#137328=CARTESIAN_POINT('Ctrl Pts',(-46.4597261390526,-53.5984603378862,
0.));
#137329=CARTESIAN_POINT('Ctrl Pts',(-46.4597261390526,-53.5984603378862,
12.));
#137330=CARTESIAN_POINT('Ctrl Pts',(-46.4411697516474,-53.5870288197161,
0.));
#137331=CARTESIAN_POINT('Ctrl Pts',(-46.4411697516474,-53.5870288197161,
12.));
#137332=CARTESIAN_POINT('Ctrl Pts',(-46.422665844546,-53.5756034397464,
0.));
#137333=CARTESIAN_POINT('Ctrl Pts',(-46.422665844546,-53.5756034397464,
12.));
#137334=CARTESIAN_POINT('Ctrl Pts',(-46.4042145078682,-53.5641843412537,
0.));
#137335=CARTESIAN_POINT('Ctrl Pts',(-46.4042145078682,-53.5641843412537,
12.));
#137336=CARTESIAN_POINT('Ctrl Pts',(-46.3858158321044,-53.552771668303,
0.));
#137337=CARTESIAN_POINT('Ctrl Pts',(-46.3858158321044,-53.552771668303,
12.));
#137338=CARTESIAN_POINT('Ctrl Pts',(-46.3674699081043,-53.5413655657323,
0.));
#137339=CARTESIAN_POINT('Ctrl Pts',(-46.3674699081043,-53.5413655657323,
12.));
#137340=CARTESIAN_POINT('Ctrl Pts',(-46.3491768270664,-53.5299661791396,
0.));
#137341=CARTESIAN_POINT('Ctrl Pts',(-46.3491768270664,-53.5299661791396,
12.));
#137342=CARTESIAN_POINT('Ctrl Pts',(-46.3309366805112,-53.518573654857,
0.));
#137343=CARTESIAN_POINT('Ctrl Pts',(-46.3309366805112,-53.518573654857,
12.));
#137344=CARTESIAN_POINT('Ctrl Pts',(-46.3127495603117,-53.5071881399932,
0.));
#137345=CARTESIAN_POINT('Ctrl Pts',(-46.3127495603117,-53.5071881399932,
12.));
#137346=CARTESIAN_POINT('Ctrl Pts',(-46.2946155587428,-53.4958097825019,
0.));
#137347=CARTESIAN_POINT('Ctrl Pts',(-46.2946155587428,-53.4958097825019,
12.));
#137348=CARTESIAN_POINT('Ctrl Pts',(-46.2765347685198,-53.4844387312414,
0.));
#137349=CARTESIAN_POINT('Ctrl Pts',(-46.2765347685198,-53.4844387312414,
12.));
#137350=CARTESIAN_POINT('Ctrl Pts',(-46.2585072828343,-53.4730751360359,
0.));
#137351=CARTESIAN_POINT('Ctrl Pts',(-46.2585072828343,-53.4730751360359,
12.));
#137352=CARTESIAN_POINT('Ctrl Pts',(-46.2405331953872,-53.4617191477382,
0.));
#137353=CARTESIAN_POINT('Ctrl Pts',(-46.2405331953872,-53.4617191477382,
12.));
#137354=CARTESIAN_POINT('Ctrl Pts',(-46.2226126003185,-53.4503709181158,
0.));
#137355=CARTESIAN_POINT('Ctrl Pts',(-46.2226126003185,-53.4503709181158,
12.));
#137356=CARTESIAN_POINT('Ctrl Pts',(-46.2047455921276,-53.4390305997263,
0.));
#137357=CARTESIAN_POINT('Ctrl Pts',(-46.2047455921276,-53.4390305997263,
12.));
#137358=CARTESIAN_POINT('Ctrl Pts',(-46.1869322656027,-53.4276983458129,
0.));
#137359=CARTESIAN_POINT('Ctrl Pts',(-46.1869322656027,-53.4276983458129,
12.));
#137360=CARTESIAN_POINT('Ctrl Pts',(-46.1691727157149,-53.4163743101535,
0.));
#137361=CARTESIAN_POINT('Ctrl Pts',(-46.1691727157149,-53.4163743101535,
12.));
#137362=CARTESIAN_POINT('Ctrl Pts',(-46.1514670376035,-53.4050586470463,
0.));
#137363=CARTESIAN_POINT('Ctrl Pts',(-46.1514670376035,-53.4050586470463,
12.));
#137364=CARTESIAN_POINT('Ctrl Pts',(-46.1338153268116,-53.3937515116572,
0.));
#137365=CARTESIAN_POINT('Ctrl Pts',(-46.1338153268116,-53.3937515116572,
12.));
#137366=CARTESIAN_POINT('Ctrl Pts',(-46.1162176794891,-53.3824530603284,
0.));
#137367=CARTESIAN_POINT('Ctrl Pts',(-46.1162176794891,-53.3824530603284,
12.));
#137368=CARTESIAN_POINT('Ctrl Pts',(-46.0986741925646,-53.3711634508426,
0.));
#137369=CARTESIAN_POINT('Ctrl Pts',(-46.0986741925646,-53.3711634508426,
12.));
#137370=CARTESIAN_POINT('Ctrl Pts',(-46.0811849640195,-53.3598828428519,
0.));
#137371=CARTESIAN_POINT('Ctrl Pts',(-46.0811849640195,-53.3598828428519,
12.));
#137372=CARTESIAN_POINT('Ctrl Pts',(-46.0637500926954,-53.3486113975868,
0.));
#137373=CARTESIAN_POINT('Ctrl Pts',(-46.0637500926954,-53.3486113975868,
12.));
#137374=CARTESIAN_POINT('Ctrl Pts',(-46.046369677778,-53.3373492770647,
0.));
#137375=CARTESIAN_POINT('Ctrl Pts',(-46.046369677778,-53.3373492770647,
12.));
#137376=CARTESIAN_POINT('Ctrl Pts',(-46.0290438183598,-53.3260966434277,
0.));
#137377=CARTESIAN_POINT('Ctrl Pts',(-46.0290438183598,-53.3260966434277,
12.));
#137378=CARTESIAN_POINT('Ctrl Pts',(-46.0117726129893,-53.3148536582658,
0.));
#137379=CARTESIAN_POINT('Ctrl Pts',(-46.0117726129893,-53.3148536582658,
12.));
#137380=CARTESIAN_POINT('Ctrl Pts',(-45.9945561591486,-53.3036204818367,
0.));
#137381=CARTESIAN_POINT('Ctrl Pts',(-45.9945561591486,-53.3036204818367,
12.));
#137382=CARTESIAN_POINT('Ctrl Pts',(-45.9773945542415,-53.2923972745585,
0.));
#137383=CARTESIAN_POINT('Ctrl Pts',(-45.9773945542415,-53.2923972745585,
12.));
#137384=CARTESIAN_POINT('Ctrl Pts',(-45.9602878967715,-53.2811841987945,
0.));
#137385=CARTESIAN_POINT('Ctrl Pts',(-45.9602878967715,-53.2811841987945,
12.));
#137386=CARTESIAN_POINT('Ctrl Pts',(-45.9432362873001,-53.2699814203097,
0.));
#137387=CARTESIAN_POINT('Ctrl Pts',(-45.9432362873001,-53.2699814203097,
12.));
#137388=CARTESIAN_POINT('Ctrl Pts',(-45.9262398298323,-53.2587891103835,
0.));
#137389=CARTESIAN_POINT('Ctrl Pts',(-45.9262398298323,-53.2587891103835,
12.));
#137390=CARTESIAN_POINT('Ctrl Pts',(-45.9092986319343,-53.2476074459977,
0.));
#137391=CARTESIAN_POINT('Ctrl Pts',(-45.9092986319343,-53.2476074459977,
12.));
#137392=CARTESIAN_POINT('Ctrl Pts',(-45.8924128018354,-53.2364366054276,
0.));
#137393=CARTESIAN_POINT('Ctrl Pts',(-45.8924128018354,-53.2364366054276,
12.));
#137394=CARTESIAN_POINT('Ctrl Pts',(-45.8755824458715,-53.2252767643652,
0.));
#137395=CARTESIAN_POINT('Ctrl Pts',(-45.8755824458715,-53.2252767643652,
12.));
#137396=CARTESIAN_POINT('Ctrl Pts',(-45.8588076662598,-53.2141280925458,
0.));
#137397=CARTESIAN_POINT('Ctrl Pts',(-45.8588076662598,-53.2141280925458,
12.));
#137398=CARTESIAN_POINT('Ctrl Pts',(-45.8420885575386,-53.2029907483602,
0.));
#137399=CARTESIAN_POINT('Ctrl Pts',(-45.8420885575386,-53.2029907483602,
12.));
#137400=CARTESIAN_POINT('Ctrl Pts',(-45.8254252100003,-53.1918648840598,
0.));
#137401=CARTESIAN_POINT('Ctrl Pts',(-45.8254252100003,-53.1918648840598,
12.));
#137402=CARTESIAN_POINT('Ctrl Pts',(-45.8088177165124,-53.1807506560977,
0.));
#137403=CARTESIAN_POINT('Ctrl Pts',(-45.8088177165124,-53.1807506560977,
12.));
#137404=CARTESIAN_POINT('Ctrl Pts',(-45.7922661780005,-53.1696482334487,
0.));
#137405=CARTESIAN_POINT('Ctrl Pts',(-45.7922661780005,-53.1696482334487,
12.));
#137406=CARTESIAN_POINT('Ctrl Pts',(-45.7757707100568,-53.158557807638,
0.));
#137407=CARTESIAN_POINT('Ctrl Pts',(-45.7757707100568,-53.158557807638,
12.));
#137408=CARTESIAN_POINT('Ctrl Pts',(-45.7593314474413,-53.147479599594,
0.));
#137409=CARTESIAN_POINT('Ctrl Pts',(-45.7593314474413,-53.147479599594,
12.));
#137410=CARTESIAN_POINT('Ctrl Pts',(-45.7429485300727,-53.136413838457,
0.));
#137411=CARTESIAN_POINT('Ctrl Pts',(-45.7429485300727,-53.136413838457,
12.));
#137412=CARTESIAN_POINT('Ctrl Pts',(-45.7266220896951,-53.1253607414806,
0.));
#137413=CARTESIAN_POINT('Ctrl Pts',(-45.7266220896951,-53.1253607414806,
12.));
#137414=CARTESIAN_POINT('Ctrl Pts',(-45.7103522376744,-53.1143204954981,
0.));
#137415=CARTESIAN_POINT('Ctrl Pts',(-45.7103522376744,-53.1143204954981,
12.));
#137416=CARTESIAN_POINT('Ctrl Pts',(-45.6941390489239,-53.1032932329074,
0.));
#137417=CARTESIAN_POINT('Ctrl Pts',(-45.6941390489239,-53.1032932329074,
12.));
#137418=CARTESIAN_POINT('Ctrl Pts',(-45.6779825614486,-53.0922790298736,
0.));
#137419=CARTESIAN_POINT('Ctrl Pts',(-45.6779825614486,-53.0922790298736,
12.));
#137420=CARTESIAN_POINT('Ctrl Pts',(-45.6651027439479,-53.083478145185,
0.));
#137421=CARTESIAN_POINT('Ctrl Pts',(-45.6651027439479,-53.083478145185,
12.));
#137422=CARTESIAN_POINT('Ctrl Pts',(-45.6554684028296,-53.0768833804386,
0.));
#137423=CARTESIAN_POINT('Ctrl Pts',(-45.6554684028296,-53.0768833804386,
12.));
#137424=CARTESIAN_POINT('Ctrl Pts',(-45.6490568514146,-53.0724894921921,
0.));
#137425=CARTESIAN_POINT('Ctrl Pts',(-45.6490568514146,-53.0724894921921,
12.));
#137426=CARTESIAN_POINT('Ctrl Pts',(-45.6458539113724,-53.0702932034641,
0.));
#137427=CARTESIAN_POINT('Ctrl Pts',(-45.6458539113724,-53.0702932034641,
12.));
#137428=CARTESIAN_POINT('',(-45.6458539113724,-53.0702932034641,12.));
#137429=CARTESIAN_POINT('Ctrl Pts',(-45.6458539113724,-53.0702932034641,
12.));
#137430=CARTESIAN_POINT('Ctrl Pts',(-45.6490568514146,-53.0724894921921,
12.));
#137431=CARTESIAN_POINT('Ctrl Pts',(-45.6554684028296,-53.0768833804386,
12.));
#137432=CARTESIAN_POINT('Ctrl Pts',(-45.6651027439479,-53.083478145185,
12.));
#137433=CARTESIAN_POINT('Ctrl Pts',(-45.6779825614486,-53.0922790298736,
12.));
#137434=CARTESIAN_POINT('Ctrl Pts',(-45.6941390489239,-53.1032932329074,
12.));
#137435=CARTESIAN_POINT('Ctrl Pts',(-45.7103522376744,-53.1143204954981,
12.));
#137436=CARTESIAN_POINT('Ctrl Pts',(-45.7266220896951,-53.1253607414806,
12.));
#137437=CARTESIAN_POINT('Ctrl Pts',(-45.7429485300727,-53.136413838457,
12.));
#137438=CARTESIAN_POINT('Ctrl Pts',(-45.7593314474413,-53.147479599594,
12.));
#137439=CARTESIAN_POINT('Ctrl Pts',(-45.7757707100568,-53.158557807638,
12.));
#137440=CARTESIAN_POINT('Ctrl Pts',(-45.7922661780005,-53.1696482334487,
12.));
#137441=CARTESIAN_POINT('Ctrl Pts',(-45.8088177165124,-53.1807506560977,
12.));
#137442=CARTESIAN_POINT('Ctrl Pts',(-45.8254252100003,-53.1918648840598,
12.));
#137443=CARTESIAN_POINT('Ctrl Pts',(-45.8420885575386,-53.2029907483602,
12.));
#137444=CARTESIAN_POINT('Ctrl Pts',(-45.8588076662598,-53.2141280925458,
12.));
#137445=CARTESIAN_POINT('Ctrl Pts',(-45.8755824458715,-53.2252767643652,
12.));
#137446=CARTESIAN_POINT('Ctrl Pts',(-45.8924128018354,-53.2364366054276,
12.));
#137447=CARTESIAN_POINT('Ctrl Pts',(-45.9092986319343,-53.2476074459977,
12.));
#137448=CARTESIAN_POINT('Ctrl Pts',(-45.9262398298323,-53.2587891103835,
12.));
#137449=CARTESIAN_POINT('Ctrl Pts',(-45.9432362873001,-53.2699814203097,
12.));
#137450=CARTESIAN_POINT('Ctrl Pts',(-45.9602878967715,-53.2811841987945,
12.));
#137451=CARTESIAN_POINT('Ctrl Pts',(-45.9773945542415,-53.2923972745585,
12.));
#137452=CARTESIAN_POINT('Ctrl Pts',(-45.9945561591486,-53.3036204818367,
12.));
#137453=CARTESIAN_POINT('Ctrl Pts',(-46.0117726129893,-53.3148536582658,
12.));
#137454=CARTESIAN_POINT('Ctrl Pts',(-46.0290438183598,-53.3260966434277,
12.));
#137455=CARTESIAN_POINT('Ctrl Pts',(-46.046369677778,-53.3373492770647,
12.));
#137456=CARTESIAN_POINT('Ctrl Pts',(-46.0637500926954,-53.3486113975868,
12.));
#137457=CARTESIAN_POINT('Ctrl Pts',(-46.0811849640195,-53.3598828428519,
12.));
#137458=CARTESIAN_POINT('Ctrl Pts',(-46.0986741925646,-53.3711634508426,
12.));
#137459=CARTESIAN_POINT('Ctrl Pts',(-46.1162176794891,-53.3824530603284,
12.));
#137460=CARTESIAN_POINT('Ctrl Pts',(-46.1338153268116,-53.3937515116572,
12.));
#137461=CARTESIAN_POINT('Ctrl Pts',(-46.1514670376035,-53.4050586470463,
12.));
#137462=CARTESIAN_POINT('Ctrl Pts',(-46.1691727157149,-53.4163743101535,
12.));
#137463=CARTESIAN_POINT('Ctrl Pts',(-46.1869322656027,-53.4276983458129,
12.));
#137464=CARTESIAN_POINT('Ctrl Pts',(-46.2047455921276,-53.4390305997263,
12.));
#137465=CARTESIAN_POINT('Ctrl Pts',(-46.2226126003185,-53.4503709181158,
12.));
#137466=CARTESIAN_POINT('Ctrl Pts',(-46.2405331953872,-53.4617191477382,
12.));
#137467=CARTESIAN_POINT('Ctrl Pts',(-46.2585072828343,-53.4730751360359,
12.));
#137468=CARTESIAN_POINT('Ctrl Pts',(-46.2765347685198,-53.4844387312414,
12.));
#137469=CARTESIAN_POINT('Ctrl Pts',(-46.2946155587428,-53.4958097825019,
12.));
#137470=CARTESIAN_POINT('Ctrl Pts',(-46.3127495603117,-53.5071881399932,
12.));
#137471=CARTESIAN_POINT('Ctrl Pts',(-46.3309366805112,-53.518573654857,
12.));
#137472=CARTESIAN_POINT('Ctrl Pts',(-46.3491768270664,-53.5299661791396,
12.));
#137473=CARTESIAN_POINT('Ctrl Pts',(-46.3674699081043,-53.5413655657323,
12.));
#137474=CARTESIAN_POINT('Ctrl Pts',(-46.3858158321044,-53.552771668303,
12.));
#137475=CARTESIAN_POINT('Ctrl Pts',(-46.4042145078682,-53.5641843412537,
12.));
#137476=CARTESIAN_POINT('Ctrl Pts',(-46.422665844546,-53.5756034397464,
12.));
#137477=CARTESIAN_POINT('Ctrl Pts',(-46.4411697516474,-53.5870288197161,
12.));
#137478=CARTESIAN_POINT('Ctrl Pts',(-46.4597261390526,-53.5984603378862,
12.));
#137479=CARTESIAN_POINT('Ctrl Pts',(-46.4783349170182,-53.6098978517869,
12.));
#137480=CARTESIAN_POINT('Ctrl Pts',(-46.4969959961779,-53.6213412197542,
12.));
#137481=CARTESIAN_POINT('Ctrl Pts',(-46.5157092875377,-53.6327903009098,
12.));
#137482=CARTESIAN_POINT('Ctrl Pts',(-46.5344747024677,-53.6442449551455,
12.));
#137483=CARTESIAN_POINT('Ctrl Pts',(-46.5532921526899,-53.6557050431069,
12.));
#137484=CARTESIAN_POINT('Ctrl Pts',(-46.572161550259,-53.6671704261735,
12.));
#137485=CARTESIAN_POINT('Ctrl Pts',(-46.5910828075652,-53.678640966456,
12.));
#137486=CARTESIAN_POINT('Ctrl Pts',(-46.6100558373401,-53.690116526794,
12.));
#137487=CARTESIAN_POINT('Ctrl Pts',(-46.6290805526559,-53.7015969707541,
12.));
#137488=CARTESIAN_POINT('Ctrl Pts',(-46.6481568669217,-53.7130821626262,
12.));
#137489=CARTESIAN_POINT('Ctrl Pts',(-46.6672846938752,-53.7245719674221,
12.));
#137490=CARTESIAN_POINT('Ctrl Pts',(-46.6864639475862,-53.7360662508675,
12.));
#137491=CARTESIAN_POINT('Ctrl Pts',(-46.7056945424559,-53.7475648793946,
12.));
#137492=CARTESIAN_POINT('Ctrl Pts',(-46.7249763932129,-53.7590677201342,
12.));
#137493=CARTESIAN_POINT('Ctrl Pts',(-46.7443094149045,-53.7705746409076,
12.));
#137494=CARTESIAN_POINT('Ctrl Pts',(-46.763693522886,-53.7820855102182,
12.));
#137495=CARTESIAN_POINT('Ctrl Pts',(-46.7831286328278,-53.793600197248,
12.));
#137496=CARTESIAN_POINT('Ctrl Pts',(-46.802614660715,-53.8051185718532,
12.));
#137497=CARTESIAN_POINT('Ctrl Pts',(-46.8221515228457,-53.816640504558,
12.));
#137498=CARTESIAN_POINT('Ctrl Pts',(-46.841739135822,-53.8281658665503,
12.));
#137499=CARTESIAN_POINT('Ctrl Pts',(-46.8613774165435,-53.8396945296757,
12.));
#137500=CARTESIAN_POINT('Ctrl Pts',(-46.881066282213,-53.8512263664321,
12.));
#137501=CARTESIAN_POINT('Ctrl Pts',(-46.9008056503351,-53.8627612499638,
12.));
#137502=CARTESIAN_POINT('Ctrl Pts',(-46.9205954387133,-53.8742990540563,
12.));
#137503=CARTESIAN_POINT('Ctrl Pts',(-46.94043556544,-53.8858396531298,12.));
#137504=CARTESIAN_POINT('Ctrl Pts',(-46.9603259488921,-53.8973829222348,
12.));
#137505=CARTESIAN_POINT('Ctrl Pts',(-46.9802665077366,-53.9089287370463,
12.));
#137506=CARTESIAN_POINT('Ctrl Pts',(-47.0002571609297,-53.9204769738596,
12.));
#137507=CARTESIAN_POINT('Ctrl Pts',(-47.0202978277138,-53.9320275095853,
12.));
#137508=CARTESIAN_POINT('Ctrl Pts',(-47.0403884276072,-53.9435802217436,
12.));
#137509=CARTESIAN_POINT('Ctrl Pts',(-47.0605288804008,-53.95513498846,12.));
#137510=CARTESIAN_POINT('Ctrl Pts',(-47.0807191061648,-53.9666916884596,
12.));
#137511=CARTESIAN_POINT('Ctrl Pts',(-47.1009590252458,-53.9782502010634,
12.));
#137512=CARTESIAN_POINT('Ctrl Pts',(-47.1212485582643,-53.989810406182,
12.));
#137513=CARTESIAN_POINT('Ctrl Pts',(-47.1415876261035,-54.0013721843118,
12.));
#137514=CARTESIAN_POINT('Ctrl Pts',(-47.1619761499087,-54.0129354165297,
12.));
#137515=CARTESIAN_POINT('Ctrl Pts',(-47.1824140510926,-54.0244999844893,
12.));
#137516=CARTESIAN_POINT('Ctrl Pts',(-47.202901251334,-54.0360657704163,
12.));
#137517=CARTESIAN_POINT('Ctrl Pts',(-47.2234376725743,-54.047632657104,
12.));
#137518=CARTESIAN_POINT('Ctrl Pts',(-47.2440232370065,-54.0592005279086,
12.));
#137519=CARTESIAN_POINT('Ctrl Pts',(-47.2646578670746,-54.0707692667438,
12.));
#137520=CARTESIAN_POINT('Ctrl Pts',(-47.2853414854793,-54.0823387580776,
12.));
#137521=CARTESIAN_POINT('Ctrl Pts',(-47.3060740151752,-54.0939088869269,
12.));
#137522=CARTESIAN_POINT('Ctrl Pts',(-47.3268553793694,-54.1054795388543,
12.));
#137523=CARTESIAN_POINT('Ctrl Pts',(-47.3476855015102,-54.1170505999645,
12.));
#137524=CARTESIAN_POINT('Ctrl Pts',(-47.3685643052874,-54.1286219568989,
12.));
#137525=CARTESIAN_POINT('Ctrl Pts',(-47.3894917146365,-54.1401934968311,
12.));
#137526=CARTESIAN_POINT('Ctrl Pts',(-47.4104676537381,-54.1517651074637,
12.));
#137527=CARTESIAN_POINT('Ctrl Pts',(-47.4314920470141,-54.1633366770239,
12.));
#137528=CARTESIAN_POINT('Ctrl Pts',(-47.4525648191173,-54.1749080942593,
12.));
#137529=CARTESIAN_POINT('Ctrl Pts',(-47.4736858949322,-54.1864792484345,
12.));
#137530=CARTESIAN_POINT('Ctrl Pts',(-47.4948551995801,-54.198050029327,
12.));
#137531=CARTESIAN_POINT('Ctrl Pts',(-47.5160726584174,-54.209620327223,
12.));
#137532=CARTESIAN_POINT('Ctrl Pts',(-47.5373381970326,-54.2211900329138,
12.));
#137533=CARTESIAN_POINT('Ctrl Pts',(-47.5586517412363,-54.2327590376924,
12.));
#137534=CARTESIAN_POINT('Ctrl Pts',(-47.5800132170608,-54.244327233349,
12.));
#137535=CARTESIAN_POINT('Ctrl Pts',(-47.6014225507659,-54.2558945121678,
12.));
#137536=CARTESIAN_POINT('Ctrl Pts',(-47.6228796688375,-54.2674607669226,
12.));
#137537=CARTESIAN_POINT('Ctrl Pts',(-47.6443844979848,-54.2790258908738,
12.));
#137538=CARTESIAN_POINT('Ctrl Pts',(-47.6659369651301,-54.290589777765,
12.));
#137539=CARTESIAN_POINT('Ctrl Pts',(-47.6875369974087,-54.302152321819,
12.));
#137540=CARTESIAN_POINT('Ctrl Pts',(-47.7091845221747,-54.3137134177345,
12.));
#137541=CARTESIAN_POINT('Ctrl Pts',(-47.7308794669993,-54.3252729606823,
12.));
#137542=CARTESIAN_POINT('Ctrl Pts',(-47.7526217596694,-54.3368308463023,
12.));
#137543=CARTESIAN_POINT('Ctrl Pts',(-47.7744113281771,-54.3483869707002,
12.));
#137544=CARTESIAN_POINT('Ctrl Pts',(-47.7962481007185,-54.3599412304438,
12.));
#137545=CARTESIAN_POINT('Ctrl Pts',(-47.8181320056995,-54.3714935225591,
12.));
#137546=CARTESIAN_POINT('Ctrl Pts',(-47.8400629717355,-54.3830437445279,
12.));
#137547=CARTESIAN_POINT('Ctrl Pts',(-47.8620409276493,-54.3945917942832,
12.));
#137548=CARTESIAN_POINT('Ctrl Pts',(-47.8840658024618,-54.4061375702079,
12.));
#137549=CARTESIAN_POINT('Ctrl Pts',(-47.9061375253897,-54.4176809711311,
12.));
#137550=CARTESIAN_POINT('Ctrl Pts',(-47.9282560258516,-54.429221896324,
12.));
#137551=CARTESIAN_POINT('Ctrl Pts',(-47.9504212334675,-54.4407602454967,
12.));
#137552=CARTESIAN_POINT('Ctrl Pts',(-47.9726330780572,-54.4522959187955,
12.));
#137553=CARTESIAN_POINT('Ctrl Pts',(-47.9948914896326,-54.4638288168003,
12.));
#137554=CARTESIAN_POINT('Ctrl Pts',(-48.0171963983924,-54.4753588405215,
12.));
#137555=CARTESIAN_POINT('Ctrl Pts',(-48.0395477347298,-54.4868858913971,
12.));
#137556=CARTESIAN_POINT('Ctrl Pts',(-48.0619454292324,-54.4984098712886,
12.));
#137557=CARTESIAN_POINT('Ctrl Pts',(-48.0843894126806,-54.5099306824786,
12.));
#137558=CARTESIAN_POINT('Ctrl Pts',(-48.1068796160405,-54.5214482276678,
12.));
#137559=CARTESIAN_POINT('Ctrl Pts',(-48.1294159704573,-54.5329624099721,
12.));
#137560=CARTESIAN_POINT('Ctrl Pts',(-48.1519984072622,-54.5444731329201,
12.));
#137561=CARTESIAN_POINT('Ctrl Pts',(-48.1746268579736,-54.5559803004492,
12.));
#137562=CARTESIAN_POINT('Ctrl Pts',(-48.1973012542966,-54.5674838169041,
12.));
#137563=CARTESIAN_POINT('Ctrl Pts',(-48.2200215281173,-54.5789835870342,
12.));
#137564=CARTESIAN_POINT('Ctrl Pts',(-48.2427876114947,-54.5904795159926,
12.));
#137565=CARTESIAN_POINT('Ctrl Pts',(-48.2655994366665,-54.6019715093309,
12.));
#137566=CARTESIAN_POINT('Ctrl Pts',(-48.2884569360506,-54.6134594729959,
12.));
#137567=CARTESIAN_POINT('Ctrl Pts',(-48.3113600422443,-54.6249433133261,
12.));
#137568=CARTESIAN_POINT('Ctrl Pts',(-48.3343086880194,-54.6364229370494,
12.));
#137569=CARTESIAN_POINT('Ctrl Pts',(-48.3573028063124,-54.6478982512794,
12.));
#137570=CARTESIAN_POINT('Ctrl Pts',(-48.3803423302294,-54.6593691635145,
12.));
#137571=CARTESIAN_POINT('Ctrl Pts',(-48.4034271930514,-54.6708355816358,
12.));
#137572=CARTESIAN_POINT('Ctrl Pts',(-48.426557328234,-54.6822974139064,
12.));
#137573=CARTESIAN_POINT('Ctrl Pts',(-48.4497326694052,-54.6937545689695,
12.));
#137574=CARTESIAN_POINT('Ctrl Pts',(-48.472953150357,-54.7052069558497,
12.));
#137575=CARTESIAN_POINT('Ctrl Pts',(-48.4962187050457,-54.716654483948,
12.));
#137576=CARTESIAN_POINT('Ctrl Pts',(-48.519529267596,-54.7280970630351,
12.));
#137577=CARTESIAN_POINT('Ctrl Pts',(-48.5428847722977,-54.7395346032453,
12.));
#137578=CARTESIAN_POINT('Ctrl Pts',(-48.5662851536026,-54.7509670150714,
12.));
#137579=CARTESIAN_POINT('Ctrl Pts',(-48.5897303461125,-54.7623942093586,
12.));
#137580=CARTESIAN_POINT('Ctrl Pts',(-48.6132202845783,-54.7738160973032,
12.));
#137581=CARTESIAN_POINT('Ctrl Pts',(-48.6367549039112,-54.7852325904583,
12.));
#137582=CARTESIAN_POINT('Ctrl Pts',(-48.6603341391886,-54.796643600739,
12.));
#137583=CARTESIAN_POINT('Ctrl Pts',(-48.6839579256566,-54.8080490404275,
12.));
#137584=CARTESIAN_POINT('Ctrl Pts',(-48.7076261987292,-54.819448822181,
12.));
#137585=CARTESIAN_POINT('Ctrl Pts',(-48.7313388939845,-54.8308428590344,
12.));
#137586=CARTESIAN_POINT('Ctrl Pts',(-48.7550959471601,-54.8422310643763,
12.));
#137587=CARTESIAN_POINT('Ctrl Pts',(-48.7788972941438,-54.8536133519292,
12.));
#137588=CARTESIAN_POINT('Ctrl Pts',(-48.8027428709614,-54.8649896357285,
12.));
#137589=CARTESIAN_POINT('Ctrl Pts',(-48.8266326137622,-54.8763598301037,
12.));
#137590=CARTESIAN_POINT('Ctrl Pts',(-48.8505664587974,-54.8877238496566,
12.));
#137591=CARTESIAN_POINT('Ctrl Pts',(-48.8745443424477,-54.8990816092953,
12.));
#137592=CARTESIAN_POINT('Ctrl Pts',(-48.8985662012528,-54.9104330242742,
12.));
#137593=CARTESIAN_POINT('Ctrl Pts',(-48.9226319719369,-54.9217780102355,
12.));
#137594=CARTESIAN_POINT('Ctrl Pts',(-48.9467415914269,-54.9331164832424,
12.));
#137595=CARTESIAN_POINT('Ctrl Pts',(-48.9708949968795,-54.9444483598378,
12.));
#137596=CARTESIAN_POINT('Ctrl Pts',(-48.9950921256527,-54.9557735569943,
12.));
#137597=CARTESIAN_POINT('Ctrl Pts',(-49.0193329152479,-54.9670919920029,
12.));
#137598=CARTESIAN_POINT('Ctrl Pts',(-49.0436173032528,-54.9784035823766,
12.));
#137599=CARTESIAN_POINT('Ctrl Pts',(-49.067945227287,-54.9897082457606,
12.));
#137600=CARTESIAN_POINT('Ctrl Pts',(-49.0923166249219,-55.0010058998107,
12.));
#137601=CARTESIAN_POINT('Ctrl Pts',(-49.116731433673,-55.012296462186,12.));
#137602=CARTESIAN_POINT('Ctrl Pts',(-49.1411895911635,-55.0235798508045,
12.));
#137603=CARTESIAN_POINT('Ctrl Pts',(-49.1656910352476,-55.0348559840453,
12.));
#137604=CARTESIAN_POINT('Ctrl Pts',(-49.1902357041461,-55.0461247809744,
12.));
#137605=CARTESIAN_POINT('Ctrl Pts',(-49.2148235365704,-55.0573861615579,
12.));
#137606=CARTESIAN_POINT('Ctrl Pts',(-49.2394544718531,-55.0686400468931,
12.));
#137607=CARTESIAN_POINT('Ctrl Pts',(-49.264128449652,-55.079886358701,12.));
#137608=CARTESIAN_POINT('Ctrl Pts',(-49.2888454096563,-55.0911250188302,
12.));
#137609=CARTESIAN_POINT('Ctrl Pts',(-49.3136052912622,-55.102355948714,
12.));
#137610=CARTESIAN_POINT('Ctrl Pts',(-49.3384080333155,-55.1135790689464,
12.));
#137611=CARTESIAN_POINT('Ctrl Pts',(-49.3632535736715,-55.1247942985619,
12.));
#137612=CARTESIAN_POINT('Ctrl Pts',(-49.3881418495489,-55.1360015556221,
12.));
#137613=CARTESIAN_POINT('Ctrl Pts',(-49.4130727983201,-55.1472007585183,
12.));
#137614=CARTESIAN_POINT('Ctrl Pts',(-49.4380463581965,-55.1583918271116,
12.));
#137615=CARTESIAN_POINT('Ctrl Pts',(-49.4630624688793,-55.1695746838174,
12.));
#137616=CARTESIAN_POINT('Ctrl Pts',(-49.4881210723966,-55.1807492550119,
12.));
#137617=CARTESIAN_POINT('Ctrl Pts',(-49.5132221132992,-55.1919154713647,
12.));
#137618=CARTESIAN_POINT('Ctrl Pts',(-49.5347748994759,-55.2014798624093,
12.));
#137619=CARTESIAN_POINT('Ctrl Pts',(-49.551321852449,-55.2088081099093,
12.));
#137620=CARTESIAN_POINT('Ctrl Pts',(-49.5628442142132,-55.2139039604721,
12.));
#137621=CARTESIAN_POINT('Ctrl Pts',(-49.5693295981927,-55.2167699151339,
12.));
#137622=CARTESIAN_POINT('Ctrl Pts',(-49.5707719660638,-55.2174072001495,
12.));
#137623=CARTESIAN_POINT('',(-45.6458539113724,-53.0702932034641,0.));
#137624=CARTESIAN_POINT('',(-45.6458539113724,-53.0702932034641,0.));
#137625=CARTESIAN_POINT('Ctrl Pts',(-49.5707719660638,-55.2174072001495,
0.));
#137626=CARTESIAN_POINT('Ctrl Pts',(-49.5693295981927,-55.2167699151339,
0.));
#137627=CARTESIAN_POINT('Ctrl Pts',(-49.5628442142132,-55.2139039604721,
0.));
#137628=CARTESIAN_POINT('Ctrl Pts',(-49.551321852449,-55.2088081099093,
0.));
#137629=CARTESIAN_POINT('Ctrl Pts',(-49.5347748994759,-55.2014798624093,
0.));
#137630=CARTESIAN_POINT('Ctrl Pts',(-49.5132221132992,-55.1919154713647,
0.));
#137631=CARTESIAN_POINT('Ctrl Pts',(-49.4881210723966,-55.1807492550119,
0.));
#137632=CARTESIAN_POINT('Ctrl Pts',(-49.4630624688793,-55.1695746838174,
0.));
#137633=CARTESIAN_POINT('Ctrl Pts',(-49.4380463581965,-55.1583918271116,
0.));
#137634=CARTESIAN_POINT('Ctrl Pts',(-49.4130727983201,-55.1472007585183,
0.));
#137635=CARTESIAN_POINT('Ctrl Pts',(-49.3881418495489,-55.1360015556221,
0.));
#137636=CARTESIAN_POINT('Ctrl Pts',(-49.3632535736715,-55.1247942985619,
0.));
#137637=CARTESIAN_POINT('Ctrl Pts',(-49.3384080333155,-55.1135790689464,
0.));
#137638=CARTESIAN_POINT('Ctrl Pts',(-49.3136052912622,-55.102355948714,
0.));
#137639=CARTESIAN_POINT('Ctrl Pts',(-49.2888454096563,-55.0911250188302,
0.));
#137640=CARTESIAN_POINT('Ctrl Pts',(-49.264128449652,-55.079886358701,0.));
#137641=CARTESIAN_POINT('Ctrl Pts',(-49.2394544718531,-55.0686400468931,
0.));
#137642=CARTESIAN_POINT('Ctrl Pts',(-49.2148235365704,-55.0573861615579,
0.));
#137643=CARTESIAN_POINT('Ctrl Pts',(-49.1902357041461,-55.0461247809744,
0.));
#137644=CARTESIAN_POINT('Ctrl Pts',(-49.1656910352476,-55.0348559840453,
0.));
#137645=CARTESIAN_POINT('Ctrl Pts',(-49.1411895911635,-55.0235798508045,
0.));
#137646=CARTESIAN_POINT('Ctrl Pts',(-49.116731433673,-55.012296462186,0.));
#137647=CARTESIAN_POINT('Ctrl Pts',(-49.0923166249219,-55.0010058998107,
0.));
#137648=CARTESIAN_POINT('Ctrl Pts',(-49.067945227287,-54.9897082457606,
0.));
#137649=CARTESIAN_POINT('Ctrl Pts',(-49.0436173032528,-54.9784035823766,
0.));
#137650=CARTESIAN_POINT('Ctrl Pts',(-49.0193329152479,-54.9670919920029,
0.));
#137651=CARTESIAN_POINT('Ctrl Pts',(-48.9950921256527,-54.9557735569943,
0.));
#137652=CARTESIAN_POINT('Ctrl Pts',(-48.9708949968795,-54.9444483598378,
0.));
#137653=CARTESIAN_POINT('Ctrl Pts',(-48.9467415914269,-54.9331164832424,
0.));
#137654=CARTESIAN_POINT('Ctrl Pts',(-48.9226319719369,-54.9217780102355,
0.));
#137655=CARTESIAN_POINT('Ctrl Pts',(-48.8985662012528,-54.9104330242742,
0.));
#137656=CARTESIAN_POINT('Ctrl Pts',(-48.8745443424477,-54.8990816092953,
0.));
#137657=CARTESIAN_POINT('Ctrl Pts',(-48.8505664587974,-54.8877238496566,
0.));
#137658=CARTESIAN_POINT('Ctrl Pts',(-48.8266326137622,-54.8763598301037,
0.));
#137659=CARTESIAN_POINT('Ctrl Pts',(-48.8027428709614,-54.8649896357285,
0.));
#137660=CARTESIAN_POINT('Ctrl Pts',(-48.7788972941438,-54.8536133519292,
0.));
#137661=CARTESIAN_POINT('Ctrl Pts',(-48.7550959471601,-54.8422310643763,
0.));
#137662=CARTESIAN_POINT('Ctrl Pts',(-48.7313388939845,-54.8308428590344,
0.));
#137663=CARTESIAN_POINT('Ctrl Pts',(-48.7076261987292,-54.819448822181,
0.));
#137664=CARTESIAN_POINT('Ctrl Pts',(-48.6839579256566,-54.8080490404275,
0.));
#137665=CARTESIAN_POINT('Ctrl Pts',(-48.6603341391886,-54.796643600739,
0.));
#137666=CARTESIAN_POINT('Ctrl Pts',(-48.6367549039112,-54.7852325904583,
0.));
#137667=CARTESIAN_POINT('Ctrl Pts',(-48.6132202845783,-54.7738160973032,
0.));
#137668=CARTESIAN_POINT('Ctrl Pts',(-48.5897303461125,-54.7623942093586,
0.));
#137669=CARTESIAN_POINT('Ctrl Pts',(-48.5662851536026,-54.7509670150714,
0.));
#137670=CARTESIAN_POINT('Ctrl Pts',(-48.5428847722977,-54.7395346032453,
0.));
#137671=CARTESIAN_POINT('Ctrl Pts',(-48.519529267596,-54.7280970630351,
0.));
#137672=CARTESIAN_POINT('Ctrl Pts',(-48.4962187050457,-54.716654483948,
0.));
#137673=CARTESIAN_POINT('Ctrl Pts',(-48.472953150357,-54.7052069558497,
0.));
#137674=CARTESIAN_POINT('Ctrl Pts',(-48.4497326694052,-54.6937545689695,
0.));
#137675=CARTESIAN_POINT('Ctrl Pts',(-48.426557328234,-54.6822974139064,
0.));
#137676=CARTESIAN_POINT('Ctrl Pts',(-48.4034271930514,-54.6708355816358,
0.));
#137677=CARTESIAN_POINT('Ctrl Pts',(-48.3803423302294,-54.6593691635145,
0.));
#137678=CARTESIAN_POINT('Ctrl Pts',(-48.3573028063124,-54.6478982512794,
0.));
#137679=CARTESIAN_POINT('Ctrl Pts',(-48.3343086880194,-54.6364229370494,
0.));
#137680=CARTESIAN_POINT('Ctrl Pts',(-48.3113600422443,-54.6249433133261,
0.));
#137681=CARTESIAN_POINT('Ctrl Pts',(-48.2884569360506,-54.6134594729959,
0.));
#137682=CARTESIAN_POINT('Ctrl Pts',(-48.2655994366665,-54.6019715093309,
0.));
#137683=CARTESIAN_POINT('Ctrl Pts',(-48.2427876114947,-54.5904795159926,
0.));
#137684=CARTESIAN_POINT('Ctrl Pts',(-48.2200215281173,-54.5789835870342,
0.));
#137685=CARTESIAN_POINT('Ctrl Pts',(-48.1973012542966,-54.5674838169041,
0.));
#137686=CARTESIAN_POINT('Ctrl Pts',(-48.1746268579736,-54.5559803004492,
0.));
#137687=CARTESIAN_POINT('Ctrl Pts',(-48.1519984072622,-54.5444731329201,
0.));
#137688=CARTESIAN_POINT('Ctrl Pts',(-48.1294159704573,-54.5329624099721,
0.));
#137689=CARTESIAN_POINT('Ctrl Pts',(-48.1068796160405,-54.5214482276678,
0.));
#137690=CARTESIAN_POINT('Ctrl Pts',(-48.0843894126806,-54.5099306824786,
0.));
#137691=CARTESIAN_POINT('Ctrl Pts',(-48.0619454292324,-54.4984098712886,
0.));
#137692=CARTESIAN_POINT('Ctrl Pts',(-48.0395477347298,-54.4868858913971,
0.));
#137693=CARTESIAN_POINT('Ctrl Pts',(-48.0171963983924,-54.4753588405215,
0.));
#137694=CARTESIAN_POINT('Ctrl Pts',(-47.9948914896326,-54.4638288168003,
0.));
#137695=CARTESIAN_POINT('Ctrl Pts',(-47.9726330780572,-54.4522959187955,
0.));
#137696=CARTESIAN_POINT('Ctrl Pts',(-47.9504212334675,-54.4407602454967,
0.));
#137697=CARTESIAN_POINT('Ctrl Pts',(-47.9282560258516,-54.429221896324,
0.));
#137698=CARTESIAN_POINT('Ctrl Pts',(-47.9061375253897,-54.4176809711311,
0.));
#137699=CARTESIAN_POINT('Ctrl Pts',(-47.8840658024618,-54.4061375702079,
0.));
#137700=CARTESIAN_POINT('Ctrl Pts',(-47.8620409276493,-54.3945917942832,
0.));
#137701=CARTESIAN_POINT('Ctrl Pts',(-47.8400629717355,-54.3830437445279,
0.));
#137702=CARTESIAN_POINT('Ctrl Pts',(-47.8181320056995,-54.3714935225591,
0.));
#137703=CARTESIAN_POINT('Ctrl Pts',(-47.7962481007185,-54.3599412304438,
0.));
#137704=CARTESIAN_POINT('Ctrl Pts',(-47.7744113281771,-54.3483869707002,
0.));
#137705=CARTESIAN_POINT('Ctrl Pts',(-47.7526217596694,-54.3368308463023,
0.));
#137706=CARTESIAN_POINT('Ctrl Pts',(-47.7308794669993,-54.3252729606823,
0.));
#137707=CARTESIAN_POINT('Ctrl Pts',(-47.7091845221747,-54.3137134177345,
0.));
#137708=CARTESIAN_POINT('Ctrl Pts',(-47.6875369974087,-54.302152321819,
0.));
#137709=CARTESIAN_POINT('Ctrl Pts',(-47.6659369651301,-54.290589777765,
0.));
#137710=CARTESIAN_POINT('Ctrl Pts',(-47.6443844979848,-54.2790258908738,
0.));
#137711=CARTESIAN_POINT('Ctrl Pts',(-47.6228796688375,-54.2674607669226,
0.));
#137712=CARTESIAN_POINT('Ctrl Pts',(-47.6014225507659,-54.2558945121678,
0.));
#137713=CARTESIAN_POINT('Ctrl Pts',(-47.5800132170608,-54.244327233349,
0.));
#137714=CARTESIAN_POINT('Ctrl Pts',(-47.5586517412363,-54.2327590376924,
0.));
#137715=CARTESIAN_POINT('Ctrl Pts',(-47.5373381970326,-54.2211900329138,
0.));
#137716=CARTESIAN_POINT('Ctrl Pts',(-47.5160726584174,-54.209620327223,
0.));
#137717=CARTESIAN_POINT('Ctrl Pts',(-47.4948551995801,-54.198050029327,
0.));
#137718=CARTESIAN_POINT('Ctrl Pts',(-47.4736858949322,-54.1864792484345,
0.));
#137719=CARTESIAN_POINT('Ctrl Pts',(-47.4525648191173,-54.1749080942593,
0.));
#137720=CARTESIAN_POINT('Ctrl Pts',(-47.4314920470141,-54.1633366770239,
0.));
#137721=CARTESIAN_POINT('Ctrl Pts',(-47.4104676537381,-54.1517651074637,
0.));
#137722=CARTESIAN_POINT('Ctrl Pts',(-47.3894917146365,-54.1401934968311,
0.));
#137723=CARTESIAN_POINT('Ctrl Pts',(-47.3685643052874,-54.1286219568989,
0.));
#137724=CARTESIAN_POINT('Ctrl Pts',(-47.3476855015102,-54.1170505999645,
0.));
#137725=CARTESIAN_POINT('Ctrl Pts',(-47.3268553793694,-54.1054795388543,
0.));
#137726=CARTESIAN_POINT('Ctrl Pts',(-47.3060740151752,-54.0939088869269,
0.));
#137727=CARTESIAN_POINT('Ctrl Pts',(-47.2853414854793,-54.0823387580776,
0.));
#137728=CARTESIAN_POINT('Ctrl Pts',(-47.2646578670746,-54.0707692667438,
0.));
#137729=CARTESIAN_POINT('Ctrl Pts',(-47.2440232370065,-54.0592005279086,
0.));
#137730=CARTESIAN_POINT('Ctrl Pts',(-47.2234376725743,-54.047632657104,
0.));
#137731=CARTESIAN_POINT('Ctrl Pts',(-47.202901251334,-54.0360657704163,
0.));
#137732=CARTESIAN_POINT('Ctrl Pts',(-47.1824140510926,-54.0244999844893,
0.));
#137733=CARTESIAN_POINT('Ctrl Pts',(-47.1619761499087,-54.0129354165297,
0.));
#137734=CARTESIAN_POINT('Ctrl Pts',(-47.1415876261035,-54.0013721843118,
0.));
#137735=CARTESIAN_POINT('Ctrl Pts',(-47.1212485582643,-53.989810406182,
0.));
#137736=CARTESIAN_POINT('Ctrl Pts',(-47.1009590252458,-53.9782502010634,
0.));
#137737=CARTESIAN_POINT('Ctrl Pts',(-47.0807191061648,-53.9666916884596,
0.));
#137738=CARTESIAN_POINT('Ctrl Pts',(-47.0605288804008,-53.95513498846,0.));
#137739=CARTESIAN_POINT('Ctrl Pts',(-47.0403884276072,-53.9435802217436,
0.));
#137740=CARTESIAN_POINT('Ctrl Pts',(-47.0202978277138,-53.9320275095853,
0.));
#137741=CARTESIAN_POINT('Ctrl Pts',(-47.0002571609297,-53.9204769738596,
0.));
#137742=CARTESIAN_POINT('Ctrl Pts',(-46.9802665077366,-53.9089287370463,
0.));
#137743=CARTESIAN_POINT('Ctrl Pts',(-46.9603259488921,-53.8973829222348,
0.));
#137744=CARTESIAN_POINT('Ctrl Pts',(-46.94043556544,-53.8858396531298,0.));
#137745=CARTESIAN_POINT('Ctrl Pts',(-46.9205954387133,-53.8742990540563,
0.));
#137746=CARTESIAN_POINT('Ctrl Pts',(-46.9008056503351,-53.8627612499638,
0.));
#137747=CARTESIAN_POINT('Ctrl Pts',(-46.881066282213,-53.8512263664321,
0.));
#137748=CARTESIAN_POINT('Ctrl Pts',(-46.8613774165435,-53.8396945296757,
0.));
#137749=CARTESIAN_POINT('Ctrl Pts',(-46.841739135822,-53.8281658665503,
0.));
#137750=CARTESIAN_POINT('Ctrl Pts',(-46.8221515228457,-53.816640504558,
0.));
#137751=CARTESIAN_POINT('Ctrl Pts',(-46.802614660715,-53.8051185718532,
0.));
#137752=CARTESIAN_POINT('Ctrl Pts',(-46.7831286328278,-53.793600197248,
0.));
#137753=CARTESIAN_POINT('Ctrl Pts',(-46.763693522886,-53.7820855102182,
0.));
#137754=CARTESIAN_POINT('Ctrl Pts',(-46.7443094149045,-53.7705746409076,
0.));
#137755=CARTESIAN_POINT('Ctrl Pts',(-46.7249763932129,-53.7590677201342,
0.));
#137756=CARTESIAN_POINT('Ctrl Pts',(-46.7056945424559,-53.7475648793946,
0.));
#137757=CARTESIAN_POINT('Ctrl Pts',(-46.6864639475862,-53.7360662508675,
0.));
#137758=CARTESIAN_POINT('Ctrl Pts',(-46.6672846938752,-53.7245719674221,
0.));
#137759=CARTESIAN_POINT('Ctrl Pts',(-46.6481568669217,-53.7130821626262,
0.));
#137760=CARTESIAN_POINT('Ctrl Pts',(-46.6290805526559,-53.7015969707541,
0.));
#137761=CARTESIAN_POINT('Ctrl Pts',(-46.6100558373401,-53.690116526794,
0.));
#137762=CARTESIAN_POINT('Ctrl Pts',(-46.5910828075652,-53.678640966456,
0.));
#137763=CARTESIAN_POINT('Ctrl Pts',(-46.572161550259,-53.6671704261735,
0.));
#137764=CARTESIAN_POINT('Ctrl Pts',(-46.5532921526899,-53.6557050431069,
0.));
#137765=CARTESIAN_POINT('Ctrl Pts',(-46.5344747024677,-53.6442449551455,
0.));
#137766=CARTESIAN_POINT('Ctrl Pts',(-46.5157092875377,-53.6327903009098,
0.));
#137767=CARTESIAN_POINT('Ctrl Pts',(-46.4969959961779,-53.6213412197542,
0.));
#137768=CARTESIAN_POINT('Ctrl Pts',(-46.4783349170182,-53.6098978517869,
0.));
#137769=CARTESIAN_POINT('Ctrl Pts',(-46.4597261390526,-53.5984603378862,
0.));
#137770=CARTESIAN_POINT('Ctrl Pts',(-46.4411697516474,-53.5870288197161,
0.));
#137771=CARTESIAN_POINT('Ctrl Pts',(-46.422665844546,-53.5756034397464,
0.));
#137772=CARTESIAN_POINT('Ctrl Pts',(-46.4042145078682,-53.5641843412537,
0.));
#137773=CARTESIAN_POINT('Ctrl Pts',(-46.3858158321044,-53.552771668303,
0.));
#137774=CARTESIAN_POINT('Ctrl Pts',(-46.3674699081043,-53.5413655657323,
0.));
#137775=CARTESIAN_POINT('Ctrl Pts',(-46.3491768270664,-53.5299661791396,
0.));
#137776=CARTESIAN_POINT('Ctrl Pts',(-46.3309366805112,-53.518573654857,
0.));
#137777=CARTESIAN_POINT('Ctrl Pts',(-46.3127495603117,-53.5071881399932,
0.));
#137778=CARTESIAN_POINT('Ctrl Pts',(-46.2946155587428,-53.4958097825019,
0.));
#137779=CARTESIAN_POINT('Ctrl Pts',(-46.2765347685198,-53.4844387312414,
0.));
#137780=CARTESIAN_POINT('Ctrl Pts',(-46.2585072828343,-53.4730751360359,
0.));
#137781=CARTESIAN_POINT('Ctrl Pts',(-46.2405331953872,-53.4617191477382,
0.));
#137782=CARTESIAN_POINT('Ctrl Pts',(-46.2226126003185,-53.4503709181158,
0.));
#137783=CARTESIAN_POINT('Ctrl Pts',(-46.2047455921276,-53.4390305997263,
0.));
#137784=CARTESIAN_POINT('Ctrl Pts',(-46.1869322656027,-53.4276983458129,
0.));
#137785=CARTESIAN_POINT('Ctrl Pts',(-46.1691727157149,-53.4163743101535,
0.));
#137786=CARTESIAN_POINT('Ctrl Pts',(-46.1514670376035,-53.4050586470463,
0.));
#137787=CARTESIAN_POINT('Ctrl Pts',(-46.1338153268116,-53.3937515116572,
0.));
#137788=CARTESIAN_POINT('Ctrl Pts',(-46.1162176794891,-53.3824530603284,
0.));
#137789=CARTESIAN_POINT('Ctrl Pts',(-46.0986741925646,-53.3711634508426,
0.));
#137790=CARTESIAN_POINT('Ctrl Pts',(-46.0811849640195,-53.3598828428519,
0.));
#137791=CARTESIAN_POINT('Ctrl Pts',(-46.0637500926954,-53.3486113975868,
0.));
#137792=CARTESIAN_POINT('Ctrl Pts',(-46.046369677778,-53.3373492770647,
0.));
#137793=CARTESIAN_POINT('Ctrl Pts',(-46.0290438183598,-53.3260966434277,
0.));
#137794=CARTESIAN_POINT('Ctrl Pts',(-46.0117726129893,-53.3148536582658,
0.));
#137795=CARTESIAN_POINT('Ctrl Pts',(-45.9945561591486,-53.3036204818367,
0.));
#137796=CARTESIAN_POINT('Ctrl Pts',(-45.9773945542415,-53.2923972745585,
0.));
#137797=CARTESIAN_POINT('Ctrl Pts',(-45.9602878967715,-53.2811841987945,
0.));
#137798=CARTESIAN_POINT('Ctrl Pts',(-45.9432362873001,-53.2699814203097,
0.));
#137799=CARTESIAN_POINT('Ctrl Pts',(-45.9262398298323,-53.2587891103835,
0.));
#137800=CARTESIAN_POINT('Ctrl Pts',(-45.9092986319343,-53.2476074459977,
0.));
#137801=CARTESIAN_POINT('Ctrl Pts',(-45.8924128018354,-53.2364366054276,
0.));
#137802=CARTESIAN_POINT('Ctrl Pts',(-45.8755824458715,-53.2252767643652,
0.));
#137803=CARTESIAN_POINT('Ctrl Pts',(-45.8588076662598,-53.2141280925458,
0.));
#137804=CARTESIAN_POINT('Ctrl Pts',(-45.8420885575386,-53.2029907483602,
0.));
#137805=CARTESIAN_POINT('Ctrl Pts',(-45.8254252100003,-53.1918648840598,
0.));
#137806=CARTESIAN_POINT('Ctrl Pts',(-45.8088177165124,-53.1807506560977,
0.));
#137807=CARTESIAN_POINT('Ctrl Pts',(-45.7922661780005,-53.1696482334487,
0.));
#137808=CARTESIAN_POINT('Ctrl Pts',(-45.7757707100568,-53.158557807638,
0.));
#137809=CARTESIAN_POINT('Ctrl Pts',(-45.7593314474413,-53.147479599594,
0.));
#137810=CARTESIAN_POINT('Ctrl Pts',(-45.7429485300727,-53.136413838457,
0.));
#137811=CARTESIAN_POINT('Ctrl Pts',(-45.7266220896951,-53.1253607414806,
0.));
#137812=CARTESIAN_POINT('Ctrl Pts',(-45.7103522376744,-53.1143204954981,
0.));
#137813=CARTESIAN_POINT('Ctrl Pts',(-45.6941390489239,-53.1032932329074,
0.));
#137814=CARTESIAN_POINT('Ctrl Pts',(-45.6779825614486,-53.0922790298736,
0.));
#137815=CARTESIAN_POINT('Ctrl Pts',(-45.6651027439479,-53.083478145185,
0.));
#137816=CARTESIAN_POINT('Ctrl Pts',(-45.6554684028296,-53.0768833804386,
0.));
#137817=CARTESIAN_POINT('Ctrl Pts',(-45.6490568514146,-53.0724894921921,
0.));
#137818=CARTESIAN_POINT('Ctrl Pts',(-45.6458539113724,-53.0702932034641,
0.));
#137819=CARTESIAN_POINT('Ctrl Pts',(-54.5031396718592,-50.7903314215393,
0.));
#137820=CARTESIAN_POINT('Ctrl Pts',(-54.5031396718592,-50.7903314215393,
12.));
#137821=CARTESIAN_POINT('Ctrl Pts',(-54.4978248630387,-50.7885805844281,
0.));
#137822=CARTESIAN_POINT('Ctrl Pts',(-54.4978248630387,-50.7885805844281,
12.));
#137823=CARTESIAN_POINT('Ctrl Pts',(-54.4871993224832,-50.7850776288814,
0.));
#137824=CARTESIAN_POINT('Ctrl Pts',(-54.4871993224832,-50.7850776288814,
12.));
#137825=CARTESIAN_POINT('Ctrl Pts',(-54.4712732429066,-50.7798193515888,
0.));
#137826=CARTESIAN_POINT('Ctrl Pts',(-54.4712732429066,-50.7798193515888,
12.));
#137827=CARTESIAN_POINT('Ctrl Pts',(-54.4500629336429,-50.7728006269349,
0.));
#137828=CARTESIAN_POINT('Ctrl Pts',(-54.4500629336429,-50.7728006269349,
12.));
#137829=CARTESIAN_POINT('Ctrl Pts',(-54.423590828767,-50.764014409002,0.));
#137830=CARTESIAN_POINT('Ctrl Pts',(-54.423590828767,-50.764014409002,12.));
#137831=CARTESIAN_POINT('Ctrl Pts',(-54.3971595231574,-50.7552153869475,
0.));
#137832=CARTESIAN_POINT('Ctrl Pts',(-54.3971595231574,-50.7552153869475,
12.));
#137833=CARTESIAN_POINT('Ctrl Pts',(-54.3707690445749,-50.7464035792906,
0.));
#137834=CARTESIAN_POINT('Ctrl Pts',(-54.3707690445749,-50.7464035792906,
12.));
#137835=CARTESIAN_POINT('Ctrl Pts',(-54.3444194324054,-50.7375790185896,
0.));
#137836=CARTESIAN_POINT('Ctrl Pts',(-54.3444194324054,-50.7375790185896,
12.));
#137837=CARTESIAN_POINT('Ctrl Pts',(-54.3181107400663,-50.7287417566123,
0.));
#137838=CARTESIAN_POINT('Ctrl Pts',(-54.3181107400663,-50.7287417566123,
12.));
#137839=CARTESIAN_POINT('Ctrl Pts',(-54.2918430335206,-50.7198918629451,
0.));
#137840=CARTESIAN_POINT('Ctrl Pts',(-54.2918430335206,-50.7198918629451,
12.));
#137841=CARTESIAN_POINT('Ctrl Pts',(-54.2656163868104,-50.7110294185698,
0.));
#137842=CARTESIAN_POINT('Ctrl Pts',(-54.2656163868104,-50.7110294185698,
12.));
#137843=CARTESIAN_POINT('Ctrl Pts',(-54.2394308784026,-50.7021545108311,
0.));
#137844=CARTESIAN_POINT('Ctrl Pts',(-54.2394308784026,-50.7021545108311,
12.));
#137845=CARTESIAN_POINT('Ctrl Pts',(-54.2132865872985,-50.6932672279772,
0.));
#137846=CARTESIAN_POINT('Ctrl Pts',(-54.2132865872985,-50.6932672279772,
12.));
#137847=CARTESIAN_POINT('Ctrl Pts',(-54.1871835889981,-50.6843676535492,
0.));
#137848=CARTESIAN_POINT('Ctrl Pts',(-54.1871835889981,-50.6843676535492,
12.));
#137849=CARTESIAN_POINT('Ctrl Pts',(-54.1611219522394,-50.67545586183,0.));
#137850=CARTESIAN_POINT('Ctrl Pts',(-54.1611219522394,-50.67545586183,12.));
#137851=CARTESIAN_POINT('Ctrl Pts',(-54.1351017412804,-50.6665319209869,
0.));
#137852=CARTESIAN_POINT('Ctrl Pts',(-54.1351017412804,-50.6665319209869,
12.));
#137853=CARTESIAN_POINT('Ctrl Pts',(-54.1091230175367,-50.6575958953221,
0.));
#137854=CARTESIAN_POINT('Ctrl Pts',(-54.1091230175367,-50.6575958953221,
12.));
#137855=CARTESIAN_POINT('Ctrl Pts',(-54.0831858415189,-50.6486478479465,
0.));
#137856=CARTESIAN_POINT('Ctrl Pts',(-54.0831858415189,-50.6486478479465,
12.));
#137857=CARTESIAN_POINT('Ctrl Pts',(-54.0572902745076,-50.6396878430939,
0.));
#137858=CARTESIAN_POINT('Ctrl Pts',(-54.0572902745076,-50.6396878430939,
12.));
#137859=CARTESIAN_POINT('Ctrl Pts',(-54.0314363806708,-50.6307159490553,
0.));
#137860=CARTESIAN_POINT('Ctrl Pts',(-54.0314363806708,-50.6307159490553,
12.));
#137861=CARTESIAN_POINT('Ctrl Pts',(-54.0056242268399,-50.6217322378648,
0.));
#137862=CARTESIAN_POINT('Ctrl Pts',(-54.0056242268399,-50.6217322378648,
12.));
#137863=CARTESIAN_POINT('Ctrl Pts',(-53.979853881553,-50.6127367839711,
0.));
#137864=CARTESIAN_POINT('Ctrl Pts',(-53.979853881553,-50.6127367839711,
12.));
#137865=CARTESIAN_POINT('Ctrl Pts',(-53.9541254143119,-50.603729663214,
0.));
#137866=CARTESIAN_POINT('Ctrl Pts',(-53.9541254143119,-50.603729663214,
12.));
#137867=CARTESIAN_POINT('Ctrl Pts',(-53.9284388948004,-50.5947109517483,
0.));
#137868=CARTESIAN_POINT('Ctrl Pts',(-53.9284388948004,-50.5947109517483,
12.));
#137869=CARTESIAN_POINT('Ctrl Pts',(-53.9027943919836,-50.5856807248151,
0.));
#137870=CARTESIAN_POINT('Ctrl Pts',(-53.9027943919836,-50.5856807248151,
12.));
#137871=CARTESIAN_POINT('Ctrl Pts',(-53.8771919737032,-50.5766390561884,
0.));
#137872=CARTESIAN_POINT('Ctrl Pts',(-53.8771919737032,-50.5766390561884,
12.));
#137873=CARTESIAN_POINT('Ctrl Pts',(-53.8516317071804,-50.5675860188538,
0.));
#137874=CARTESIAN_POINT('Ctrl Pts',(-53.8516317071804,-50.5675860188538,
12.));
#137875=CARTESIAN_POINT('Ctrl Pts',(-53.8261136593075,-50.5585216854091,
0.));
#137876=CARTESIAN_POINT('Ctrl Pts',(-53.8261136593075,-50.5585216854091,
12.));
#137877=CARTESIAN_POINT('Ctrl Pts',(-53.8006378970197,-50.5494461285761,
0.));
#137878=CARTESIAN_POINT('Ctrl Pts',(-53.8006378970197,-50.5494461285761,
12.));
#137879=CARTESIAN_POINT('Ctrl Pts',(-53.7752044876304,-50.5403594216698,
0.));
#137880=CARTESIAN_POINT('Ctrl Pts',(-53.7752044876304,-50.5403594216698,
12.));
#137881=CARTESIAN_POINT('Ctrl Pts',(-53.7498134991703,-50.5312616390779,
0.));
#137882=CARTESIAN_POINT('Ctrl Pts',(-53.7498134991703,-50.5312616390779,
12.));
#137883=CARTESIAN_POINT('Ctrl Pts',(-53.7244650002374,-50.522152856042,
0.));
#137884=CARTESIAN_POINT('Ctrl Pts',(-53.7244650002374,-50.522152856042,
12.));
#137885=CARTESIAN_POINT('Ctrl Pts',(-53.6991590598548,-50.513033148456,
0.));
#137886=CARTESIAN_POINT('Ctrl Pts',(-53.6991590598548,-50.513033148456,
12.));
#137887=CARTESIAN_POINT('Ctrl Pts',(-53.6738957473158,-50.503902592653,
0.));
#137888=CARTESIAN_POINT('Ctrl Pts',(-53.6738957473158,-50.503902592653,
12.));
#137889=CARTESIAN_POINT('Ctrl Pts',(-53.6486751320436,-50.4947612652149,
0.));
#137890=CARTESIAN_POINT('Ctrl Pts',(-53.6486751320436,-50.4947612652149,
12.));
#137891=CARTESIAN_POINT('Ctrl Pts',(-53.623497283406,-50.4856092427314,
0.));
#137892=CARTESIAN_POINT('Ctrl Pts',(-53.623497283406,-50.4856092427314,
12.));
#137893=CARTESIAN_POINT('Ctrl Pts',(-53.5983622707238,-50.4764466018071,
0.));
#137894=CARTESIAN_POINT('Ctrl Pts',(-53.5983622707238,-50.4764466018071,
12.));
#137895=CARTESIAN_POINT('Ctrl Pts',(-53.5732701633609,-50.4672734191756,
0.));
#137896=CARTESIAN_POINT('Ctrl Pts',(-53.5732701633609,-50.4672734191756,
12.));
#137897=CARTESIAN_POINT('Ctrl Pts',(-53.5482210307868,-50.4580897717838,
0.));
#137898=CARTESIAN_POINT('Ctrl Pts',(-53.5482210307868,-50.4580897717838,
12.));
#137899=CARTESIAN_POINT('Ctrl Pts',(-53.5232149426413,-50.4488957368839,
0.));
#137900=CARTESIAN_POINT('Ctrl Pts',(-53.5232149426413,-50.4488957368839,
12.));
#137901=CARTESIAN_POINT('Ctrl Pts',(-53.4982519688024,-50.4396913921382,
0.));
#137902=CARTESIAN_POINT('Ctrl Pts',(-53.4982519688024,-50.4396913921382,
12.));
#137903=CARTESIAN_POINT('Ctrl Pts',(-53.4733321794188,-50.4304768156667,
0.));
#137904=CARTESIAN_POINT('Ctrl Pts',(-53.4733321794188,-50.4304768156667,
12.));
#137905=CARTESIAN_POINT('Ctrl Pts',(-53.4484556448776,-50.4212520859914,
0.));
#137906=CARTESIAN_POINT('Ctrl Pts',(-53.4484556448776,-50.4212520859914,
12.));
#137907=CARTESIAN_POINT('Ctrl Pts',(-53.4236224357838,-50.4120172820047,
0.));
#137908=CARTESIAN_POINT('Ctrl Pts',(-53.4236224357838,-50.4120172820047,
12.));
#137909=CARTESIAN_POINT('Ctrl Pts',(-53.398832622931,-50.4027724829297,
0.));
#137910=CARTESIAN_POINT('Ctrl Pts',(-53.398832622931,-50.4027724829297,
12.));
#137911=CARTESIAN_POINT('Ctrl Pts',(-53.3740862772681,-50.3935177682837,
0.));
#137912=CARTESIAN_POINT('Ctrl Pts',(-53.3740862772681,-50.3935177682837,
12.));
#137913=CARTESIAN_POINT('Ctrl Pts',(-53.3493834698697,-50.384253217846,
0.));
#137914=CARTESIAN_POINT('Ctrl Pts',(-53.3493834698697,-50.384253217846,
12.));
#137915=CARTESIAN_POINT('Ctrl Pts',(-53.3247242719587,-50.3749789116786,
0.));
#137916=CARTESIAN_POINT('Ctrl Pts',(-53.3247242719587,-50.3749789116786,
12.));
#137917=CARTESIAN_POINT('Ctrl Pts',(-53.300108754923,-50.365694930143,0.));
#137918=CARTESIAN_POINT('Ctrl Pts',(-53.300108754923,-50.365694930143,12.));
#137919=CARTESIAN_POINT('Ctrl Pts',(-53.2755369903293,-50.3564013539199,
0.));
#137920=CARTESIAN_POINT('Ctrl Pts',(-53.2755369903293,-50.3564013539199,
12.));
#137921=CARTESIAN_POINT('Ctrl Pts',(-53.2510090499336,-50.3470982640289,
0.));
#137922=CARTESIAN_POINT('Ctrl Pts',(-53.2510090499336,-50.3470982640289,
12.));
#137923=CARTESIAN_POINT('Ctrl Pts',(-53.2265250056887,-50.3377857418515,
0.));
#137924=CARTESIAN_POINT('Ctrl Pts',(-53.2265250056887,-50.3377857418515,
12.));
#137925=CARTESIAN_POINT('Ctrl Pts',(-53.2020849297471,-50.3284638691278,
0.));
#137926=CARTESIAN_POINT('Ctrl Pts',(-53.2020849297471,-50.3284638691278,
12.));
#137927=CARTESIAN_POINT('Ctrl Pts',(-53.1776888944616,-50.3191327279493,
0.));
#137928=CARTESIAN_POINT('Ctrl Pts',(-53.1776888944616,-50.3191327279493,
12.));
#137929=CARTESIAN_POINT('Ctrl Pts',(-53.1533369723818,-50.3097924007534,
0.));
#137930=CARTESIAN_POINT('Ctrl Pts',(-53.1533369723818,-50.3097924007534,
12.));
#137931=CARTESIAN_POINT('Ctrl Pts',(-53.1290292362485,-50.300442970319,
0.));
#137932=CARTESIAN_POINT('Ctrl Pts',(-53.1290292362485,-50.300442970319,
12.));
#137933=CARTESIAN_POINT('Ctrl Pts',(-53.1047657589812,-50.2910845197619,
0.));
#137934=CARTESIAN_POINT('Ctrl Pts',(-53.1047657589812,-50.2910845197619,
12.));
#137935=CARTESIAN_POINT('Ctrl Pts',(-53.0805466136798,-50.2817171325358,
0.));
#137936=CARTESIAN_POINT('Ctrl Pts',(-53.0805466136798,-50.2817171325358,
12.));
#137937=CARTESIAN_POINT('Ctrl Pts',(-53.0563718736366,-50.2723408924373,
0.));
#137938=CARTESIAN_POINT('Ctrl Pts',(-53.0563718736366,-50.2723408924373,
12.));
#137939=CARTESIAN_POINT('Ctrl Pts',(-53.0322416123406,-50.2629558836111,
0.));
#137940=CARTESIAN_POINT('Ctrl Pts',(-53.0322416123406,-50.2629558836111,
12.));
#137941=CARTESIAN_POINT('Ctrl Pts',(-53.0081559034801,-50.2535621905552,
0.));
#137942=CARTESIAN_POINT('Ctrl Pts',(-53.0081559034801,-50.2535621905552,
12.));
#137943=CARTESIAN_POINT('Ctrl Pts',(-52.9841148209402,-50.2441598981286,
0.));
#137944=CARTESIAN_POINT('Ctrl Pts',(-52.9841148209402,-50.2441598981286,
12.));
#137945=CARTESIAN_POINT('Ctrl Pts',(-52.9601184388028,-50.2347490915555,
0.));
#137946=CARTESIAN_POINT('Ctrl Pts',(-52.9601184388028,-50.2347490915555,
12.));
#137947=CARTESIAN_POINT('Ctrl Pts',(-52.9361668313542,-50.2253298564241,
0.));
#137948=CARTESIAN_POINT('Ctrl Pts',(-52.9361668313542,-50.2253298564241,
12.));
#137949=CARTESIAN_POINT('Ctrl Pts',(-52.9122600730884,-50.2159022786879,
0.));
#137950=CARTESIAN_POINT('Ctrl Pts',(-52.9122600730884,-50.2159022786879,
12.));
#137951=CARTESIAN_POINT('Ctrl Pts',(-52.8883982387068,-50.2064664446663,
0.));
#137952=CARTESIAN_POINT('Ctrl Pts',(-52.8883982387068,-50.2064664446663,
12.));
#137953=CARTESIAN_POINT('Ctrl Pts',(-52.8645814031133,-50.1970224410471,
0.));
#137954=CARTESIAN_POINT('Ctrl Pts',(-52.8645814031133,-50.1970224410471,
12.));
#137955=CARTESIAN_POINT('Ctrl Pts',(-52.8408096414093,-50.1875703548884,
0.));
#137956=CARTESIAN_POINT('Ctrl Pts',(-52.8408096414093,-50.1875703548884,
12.));
#137957=CARTESIAN_POINT('Ctrl Pts',(-52.8170830289044,-50.1781102736205,
0.));
#137958=CARTESIAN_POINT('Ctrl Pts',(-52.8170830289044,-50.1781102736205,
12.));
#137959=CARTESIAN_POINT('Ctrl Pts',(-52.7934016411205,-50.1686422850488,
0.));
#137960=CARTESIAN_POINT('Ctrl Pts',(-52.7934016411205,-50.1686422850488,
12.));
#137961=CARTESIAN_POINT('Ctrl Pts',(-52.769765553794,-50.1591664773561,
0.));
#137962=CARTESIAN_POINT('Ctrl Pts',(-52.769765553794,-50.1591664773561,
12.));
#137963=CARTESIAN_POINT('Ctrl Pts',(-52.7461748428738,-50.1496829391073,
0.));
#137964=CARTESIAN_POINT('Ctrl Pts',(-52.7461748428738,-50.1496829391073,
12.));
#137965=CARTESIAN_POINT('Ctrl Pts',(-52.7226295845161,-50.1401917592537,
0.));
#137966=CARTESIAN_POINT('Ctrl Pts',(-52.7226295845161,-50.1401917592537,
12.));
#137967=CARTESIAN_POINT('Ctrl Pts',(-52.699129855093,-50.1306930271345,
0.));
#137968=CARTESIAN_POINT('Ctrl Pts',(-52.699129855093,-50.1306930271345,
12.));
#137969=CARTESIAN_POINT('Ctrl Pts',(-52.6756757311978,-50.1211868324781,
0.));
#137970=CARTESIAN_POINT('Ctrl Pts',(-52.6756757311978,-50.1211868324781,
12.));
#137971=CARTESIAN_POINT('Ctrl Pts',(-52.652267289646,-50.111673265404,0.));
#137972=CARTESIAN_POINT('Ctrl Pts',(-52.652267289646,-50.111673265404,12.));
#137973=CARTESIAN_POINT('Ctrl Pts',(-52.6289046074746,-50.1021524164264,
0.));
#137974=CARTESIAN_POINT('Ctrl Pts',(-52.6289046074746,-50.1021524164264,
12.));
#137975=CARTESIAN_POINT('Ctrl Pts',(-52.6055877619348,-50.0926243764578,
0.));
#137976=CARTESIAN_POINT('Ctrl Pts',(-52.6055877619348,-50.0926243764578,
12.));
#137977=CARTESIAN_POINT('Ctrl Pts',(-52.5823168304994,-50.0830892368107,
0.));
#137978=CARTESIAN_POINT('Ctrl Pts',(-52.5823168304994,-50.0830892368107,
12.));
#137979=CARTESIAN_POINT('Ctrl Pts',(-52.5590918908702,-50.0735470892007,
0.));
#137980=CARTESIAN_POINT('Ctrl Pts',(-52.5590918908702,-50.0735470892007,
12.));
#137981=CARTESIAN_POINT('Ctrl Pts',(-52.5359130209792,-50.0639980257479,
0.));
#137982=CARTESIAN_POINT('Ctrl Pts',(-52.5359130209792,-50.0639980257479,
12.));
#137983=CARTESIAN_POINT('Ctrl Pts',(-52.5127802989896,-50.0544421389818,
0.));
#137984=CARTESIAN_POINT('Ctrl Pts',(-52.5127802989896,-50.0544421389818,
12.));
#137985=CARTESIAN_POINT('Ctrl Pts',(-52.4896938032884,-50.0448795218441,
0.));
#137986=CARTESIAN_POINT('Ctrl Pts',(-52.4896938032884,-50.0448795218441,
12.));
#137987=CARTESIAN_POINT('Ctrl Pts',(-52.4666536124913,-50.0353102676921,
0.));
#137988=CARTESIAN_POINT('Ctrl Pts',(-52.4666536124913,-50.0353102676921,
12.));
#137989=CARTESIAN_POINT('Ctrl Pts',(-52.4436598054515,-50.0257344703,0.));
#137990=CARTESIAN_POINT('Ctrl Pts',(-52.4436598054515,-50.0257344703,12.));
#137991=CARTESIAN_POINT('Ctrl Pts',(-52.4207124612608,-50.0161522238616,
0.));
#137992=CARTESIAN_POINT('Ctrl Pts',(-52.4207124612608,-50.0161522238616,
12.));
#137993=CARTESIAN_POINT('Ctrl Pts',(-52.3978116592509,-50.0065636229938,
0.));
#137994=CARTESIAN_POINT('Ctrl Pts',(-52.3978116592509,-50.0065636229938,
12.));
#137995=CARTESIAN_POINT('Ctrl Pts',(-52.3749574789871,-49.9969687627408,
0.));
#137996=CARTESIAN_POINT('Ctrl Pts',(-52.3749574789871,-49.9969687627408,
12.));
#137997=CARTESIAN_POINT('Ctrl Pts',(-52.3521500002718,-49.9873677385775,
0.));
#137998=CARTESIAN_POINT('Ctrl Pts',(-52.3521500002718,-49.9873677385775,
12.));
#137999=CARTESIAN_POINT('Ctrl Pts',(-52.3293893031528,-49.9777606464106,
0.));
#138000=CARTESIAN_POINT('Ctrl Pts',(-52.3293893031528,-49.9777606464106,
12.));
#138001=CARTESIAN_POINT('Ctrl Pts',(-52.3066754679265,-49.9681475825824,
0.));
#138002=CARTESIAN_POINT('Ctrl Pts',(-52.3066754679265,-49.9681475825824,
12.));
#138003=CARTESIAN_POINT('Ctrl Pts',(-52.2840085751384,-49.9585286438733,
0.));
#138004=CARTESIAN_POINT('Ctrl Pts',(-52.2840085751384,-49.9585286438733,
12.));
#138005=CARTESIAN_POINT('Ctrl Pts',(-52.2613887055773,-49.9489039275064,
0.));
#138006=CARTESIAN_POINT('Ctrl Pts',(-52.2613887055773,-49.9489039275064,
12.));
#138007=CARTESIAN_POINT('Ctrl Pts',(-52.2388159402771,-49.9392735311509,
0.));
#138008=CARTESIAN_POINT('Ctrl Pts',(-52.2388159402771,-49.9392735311509,
12.));
#138009=CARTESIAN_POINT('Ctrl Pts',(-52.2162903605275,-49.9296375529245,
0.));
#138010=CARTESIAN_POINT('Ctrl Pts',(-52.2162903605275,-49.9296375529245,
12.));
#138011=CARTESIAN_POINT('Ctrl Pts',(-52.1938120478754,-49.9199960913962,
0.));
#138012=CARTESIAN_POINT('Ctrl Pts',(-52.1938120478754,-49.9199960913962,
12.));
#138013=CARTESIAN_POINT('Ctrl Pts',(-52.1713810841276,-49.9103492455902,
0.));
#138014=CARTESIAN_POINT('Ctrl Pts',(-52.1713810841276,-49.9103492455902,
12.));
#138015=CARTESIAN_POINT('Ctrl Pts',(-52.1489975513445,-49.9006971149895,
0.));
#138016=CARTESIAN_POINT('Ctrl Pts',(-52.1489975513445,-49.9006971149895,
12.));
#138017=CARTESIAN_POINT('Ctrl Pts',(-52.1266615318407,-49.8910397995397,
0.));
#138018=CARTESIAN_POINT('Ctrl Pts',(-52.1266615318407,-49.8910397995397,
12.));
#138019=CARTESIAN_POINT('Ctrl Pts',(-52.1043731081962,-49.8813773996517,
0.));
#138020=CARTESIAN_POINT('Ctrl Pts',(-52.1043731081962,-49.8813773996517,
12.));
#138021=CARTESIAN_POINT('Ctrl Pts',(-52.0821323632587,-49.8717100162048,
0.));
#138022=CARTESIAN_POINT('Ctrl Pts',(-52.0821323632587,-49.8717100162048,
12.));
#138023=CARTESIAN_POINT('Ctrl Pts',(-52.0599393801452,-49.86203775055,0.));
#138024=CARTESIAN_POINT('Ctrl Pts',(-52.0599393801452,-49.86203775055,12.));
#138025=CARTESIAN_POINT('Ctrl Pts',(-52.0377942422376,-49.8523607045149,
0.));
#138026=CARTESIAN_POINT('Ctrl Pts',(-52.0377942422376,-49.8523607045149,
12.));
#138027=CARTESIAN_POINT('Ctrl Pts',(-52.0156970331823,-49.8426789804071,
0.));
#138028=CARTESIAN_POINT('Ctrl Pts',(-52.0156970331823,-49.8426789804071,
12.));
#138029=CARTESIAN_POINT('Ctrl Pts',(-51.9936478369008,-49.8329926810172,
0.));
#138030=CARTESIAN_POINT('Ctrl Pts',(-51.9936478369008,-49.8329926810172,
12.));
#138031=CARTESIAN_POINT('Ctrl Pts',(-51.9716467375937,-49.8233019096222,
0.));
#138032=CARTESIAN_POINT('Ctrl Pts',(-51.9716467375937,-49.8233019096222,
12.));
#138033=CARTESIAN_POINT('Ctrl Pts',(-51.9496938197418,-49.8136067699896,
0.));
#138034=CARTESIAN_POINT('Ctrl Pts',(-51.9496938197418,-49.8136067699896,
12.));
#138035=CARTESIAN_POINT('Ctrl Pts',(-51.9277891681018,-49.8039073663812,
0.));
#138036=CARTESIAN_POINT('Ctrl Pts',(-51.9277891681018,-49.8039073663812,
12.));
#138037=CARTESIAN_POINT('Ctrl Pts',(-51.9059328677059,-49.7942038035576,
0.));
#138038=CARTESIAN_POINT('Ctrl Pts',(-51.9059328677059,-49.7942038035576,
12.));
#138039=CARTESIAN_POINT('Ctrl Pts',(-51.8841250038724,-49.7844961867808,
0.));
#138040=CARTESIAN_POINT('Ctrl Pts',(-51.8841250038724,-49.7844961867808,
12.));
#138041=CARTESIAN_POINT('Ctrl Pts',(-51.8623656622097,-49.7747846218182,
0.));
#138042=CARTESIAN_POINT('Ctrl Pts',(-51.8623656622097,-49.7747846218182,
12.));
#138043=CARTESIAN_POINT('Ctrl Pts',(-51.8406549286175,-49.7650692149462,
0.));
#138044=CARTESIAN_POINT('Ctrl Pts',(-51.8406549286175,-49.7650692149462,
12.));
#138045=CARTESIAN_POINT('Ctrl Pts',(-51.8189928892828,-49.755350072955,
0.));
#138046=CARTESIAN_POINT('Ctrl Pts',(-51.8189928892828,-49.755350072955,
12.));
#138047=CARTESIAN_POINT('Ctrl Pts',(-51.7973796306803,-49.7456273031534,
0.));
#138048=CARTESIAN_POINT('Ctrl Pts',(-51.7973796306803,-49.7456273031534,
12.));
#138049=CARTESIAN_POINT('Ctrl Pts',(-51.7758152395836,-49.7359010133721,
0.));
#138050=CARTESIAN_POINT('Ctrl Pts',(-51.7758152395836,-49.7359010133721,
12.));
#138051=CARTESIAN_POINT('Ctrl Pts',(-51.754299803067,-49.7261713119663,
0.));
#138052=CARTESIAN_POINT('Ctrl Pts',(-51.754299803067,-49.7261713119663,
12.));
#138053=CARTESIAN_POINT('Ctrl Pts',(-51.7328334085091,-49.7164383078212,
0.));
#138054=CARTESIAN_POINT('Ctrl Pts',(-51.7328334085091,-49.7164383078212,
12.));
#138055=CARTESIAN_POINT('Ctrl Pts',(-51.7114161435869,-49.7067021103553,
0.));
#138056=CARTESIAN_POINT('Ctrl Pts',(-51.7114161435869,-49.7067021103553,
12.));
#138057=CARTESIAN_POINT('Ctrl Pts',(-51.6900480962773,-49.6969628295262,
0.));
#138058=CARTESIAN_POINT('Ctrl Pts',(-51.6900480962773,-49.6969628295262,
12.));
#138059=CARTESIAN_POINT('Ctrl Pts',(-51.6687293548682,-49.6872205758336,
0.));
#138060=CARTESIAN_POINT('Ctrl Pts',(-51.6687293548682,-49.6872205758336,
12.));
#138061=CARTESIAN_POINT('Ctrl Pts',(-51.6474600079622,-49.6774754603245,
0.));
#138062=CARTESIAN_POINT('Ctrl Pts',(-51.6474600079622,-49.6774754603245,
12.));
#138063=CARTESIAN_POINT('Ctrl Pts',(-51.626240144479,-49.6677275945967,
0.));
#138064=CARTESIAN_POINT('Ctrl Pts',(-51.626240144479,-49.6677275945967,
12.));
#138065=CARTESIAN_POINT('Ctrl Pts',(-51.6050698536496,-49.6579770908037,
0.));
#138066=CARTESIAN_POINT('Ctrl Pts',(-51.6050698536496,-49.6579770908037,
12.));
#138067=CARTESIAN_POINT('Ctrl Pts',(-51.5839492250181,-49.6482240616593,
0.));
#138068=CARTESIAN_POINT('Ctrl Pts',(-51.5839492250181,-49.6482240616593,
12.));
#138069=CARTESIAN_POINT('Ctrl Pts',(-51.5628783484525,-49.6384686204413,
0.));
#138070=CARTESIAN_POINT('Ctrl Pts',(-51.5628783484525,-49.6384686204413,
12.));
#138071=CARTESIAN_POINT('Ctrl Pts',(-51.5418573141484,-49.6287108809966,
0.));
#138072=CARTESIAN_POINT('Ctrl Pts',(-51.5418573141484,-49.6287108809966,
12.));
#138073=CARTESIAN_POINT('Ctrl Pts',(-51.5208862126315,-49.6189509577452,
0.));
#138074=CARTESIAN_POINT('Ctrl Pts',(-51.5208862126315,-49.6189509577452,
12.));
#138075=CARTESIAN_POINT('Ctrl Pts',(-51.4999651347523,-49.6091889656866,
0.));
#138076=CARTESIAN_POINT('Ctrl Pts',(-51.4999651347523,-49.6091889656866,
12.));
#138077=CARTESIAN_POINT('Ctrl Pts',(-51.4790941716888,-49.5994250204031,
0.));
#138078=CARTESIAN_POINT('Ctrl Pts',(-51.4790941716888,-49.5994250204031,
12.));
#138079=CARTESIAN_POINT('Ctrl Pts',(-51.4582734149583,-49.5896592380654,
0.));
#138080=CARTESIAN_POINT('Ctrl Pts',(-51.4582734149583,-49.5896592380654,
12.));
#138081=CARTESIAN_POINT('Ctrl Pts',(-51.4375029564197,-49.5798917354366,
0.));
#138082=CARTESIAN_POINT('Ctrl Pts',(-51.4375029564197,-49.5798917354366,
12.));
#138083=CARTESIAN_POINT('Ctrl Pts',(-51.4167828882756,-49.5701226298769,
0.));
#138084=CARTESIAN_POINT('Ctrl Pts',(-51.4167828882756,-49.5701226298769,
12.));
#138085=CARTESIAN_POINT('Ctrl Pts',(-51.396113303067,-49.5603520393496,
0.));
#138086=CARTESIAN_POINT('Ctrl Pts',(-51.396113303067,-49.5603520393496,
12.));
#138087=CARTESIAN_POINT('Ctrl Pts',(-51.3754942936778,-49.550580082425,
0.));
#138088=CARTESIAN_POINT('Ctrl Pts',(-51.3754942936778,-49.550580082425,
12.));
#138089=CARTESIAN_POINT('Ctrl Pts',(-51.3549259533458,-49.5408068782859,
0.));
#138090=CARTESIAN_POINT('Ctrl Pts',(-51.3549259533458,-49.5408068782859,
12.));
#138091=CARTESIAN_POINT('Ctrl Pts',(-51.3344083756657,-49.5310325467332,
0.));
#138092=CARTESIAN_POINT('Ctrl Pts',(-51.3344083756657,-49.5310325467332,
12.));
#138093=CARTESIAN_POINT('Ctrl Pts',(-51.313941654591,-49.5212572081908,
0.));
#138094=CARTESIAN_POINT('Ctrl Pts',(-51.313941654591,-49.5212572081908,
12.));
#138095=CARTESIAN_POINT('Ctrl Pts',(-51.2935258844289,-49.5114809837122,
0.));
#138096=CARTESIAN_POINT('Ctrl Pts',(-51.2935258844289,-49.5114809837122,
12.));
#138097=CARTESIAN_POINT('Ctrl Pts',(-51.2731611598475,-49.5017039949852,
0.));
#138098=CARTESIAN_POINT('Ctrl Pts',(-51.2731611598475,-49.5017039949852,
12.));
#138099=CARTESIAN_POINT('Ctrl Pts',(-51.2528475758846,-49.4919263643362,
0.));
#138100=CARTESIAN_POINT('Ctrl Pts',(-51.2528475758846,-49.4919263643362,
12.));
#138101=CARTESIAN_POINT('Ctrl Pts',(-51.2325852279506,-49.4821482147356,
0.));
#138102=CARTESIAN_POINT('Ctrl Pts',(-51.2325852279506,-49.4821482147356,
12.));
#138103=CARTESIAN_POINT('Ctrl Pts',(-51.2123742118287,-49.4723696698021,
0.));
#138104=CARTESIAN_POINT('Ctrl Pts',(-51.2123742118287,-49.4723696698021,
12.));
#138105=CARTESIAN_POINT('Ctrl Pts',(-51.1922146236686,-49.4625908538074,
0.));
#138106=CARTESIAN_POINT('Ctrl Pts',(-51.1922146236686,-49.4625908538074,
12.));
#138107=CARTESIAN_POINT('Ctrl Pts',(-51.1721065599973,-49.4528118916832,
0.));
#138108=CARTESIAN_POINT('Ctrl Pts',(-51.1721065599973,-49.4528118916832,
12.));
#138109=CARTESIAN_POINT('Ctrl Pts',(-51.1520501177291,-49.4430329090287,
0.));
#138110=CARTESIAN_POINT('Ctrl Pts',(-51.1520501177291,-49.4430329090287,
12.));
#138111=CARTESIAN_POINT('Ctrl Pts',(-51.1320453941702,-49.4332540321178,
0.));
#138112=CARTESIAN_POINT('Ctrl Pts',(-51.1320453941702,-49.4332540321178,
12.));
#138113=CARTESIAN_POINT('Ctrl Pts',(-51.1120924870195,-49.423475387907,
0.));
#138114=CARTESIAN_POINT('Ctrl Pts',(-51.1120924870195,-49.423475387907,
12.));
#138115=CARTESIAN_POINT('Ctrl Pts',(-51.0921914943662,-49.4136971040428,
0.));
#138116=CARTESIAN_POINT('Ctrl Pts',(-51.0921914943662,-49.4136971040428,
12.));
#138117=CARTESIAN_POINT('Ctrl Pts',(-51.0723425146985,-49.4039193088634,
0.));
#138118=CARTESIAN_POINT('Ctrl Pts',(-51.0723425146985,-49.4039193088634,
12.));
#138119=CARTESIAN_POINT('Ctrl Pts',(-51.052545646907,-49.3941421314013,
0.));
#138120=CARTESIAN_POINT('Ctrl Pts',(-51.052545646907,-49.3941421314013,
12.));
#138121=CARTESIAN_POINT('Ctrl Pts',(-51.0328009902858,-49.3843657013852,
0.));
#138122=CARTESIAN_POINT('Ctrl Pts',(-51.0328009902858,-49.3843657013852,
12.));
#138123=CARTESIAN_POINT('Ctrl Pts',(-51.0131086445272,-49.3745901492432,
0.));
#138124=CARTESIAN_POINT('Ctrl Pts',(-51.0131086445272,-49.3745901492432,
12.));
#138125=CARTESIAN_POINT('Ctrl Pts',(-50.9934687097188,-49.3648156061058,
0.));
#138126=CARTESIAN_POINT('Ctrl Pts',(-50.9934687097188,-49.3648156061058,
12.));
#138127=CARTESIAN_POINT('Ctrl Pts',(-50.9738812863646,-49.355042203823,
0.));
#138128=CARTESIAN_POINT('Ctrl Pts',(-50.9738812863646,-49.355042203823,
12.));
#138129=CARTESIAN_POINT('Ctrl Pts',(-50.9543464753981,-49.345270074981,
0.));
#138130=CARTESIAN_POINT('Ctrl Pts',(-50.9543464753981,-49.345270074981,
12.));
#138131=CARTESIAN_POINT('Ctrl Pts',(-50.9348643781924,-49.3354993529159,
0.));
#138132=CARTESIAN_POINT('Ctrl Pts',(-50.9348643781924,-49.3354993529159,
12.));
#138133=CARTESIAN_POINT('Ctrl Pts',(-50.9154350965666,-49.3257301717335,
0.));
#138134=CARTESIAN_POINT('Ctrl Pts',(-50.9154350965666,-49.3257301717335,
12.));
#138135=CARTESIAN_POINT('Ctrl Pts',(-50.8960587327848,-49.3159626663109,
0.));
#138136=CARTESIAN_POINT('Ctrl Pts',(-50.8960587327848,-49.3159626663109,
12.));
#138137=CARTESIAN_POINT('Ctrl Pts',(-50.8767353895492,-49.3061969722781,
0.));
#138138=CARTESIAN_POINT('Ctrl Pts',(-50.8767353895492,-49.3061969722781,
12.));
#138139=CARTESIAN_POINT('Ctrl Pts',(-50.8574651699873,-49.2964332260039,
0.));
#138140=CARTESIAN_POINT('Ctrl Pts',(-50.8574651699873,-49.2964332260039,
12.));
#138141=CARTESIAN_POINT('Ctrl Pts',(-50.8382481776403,-49.2866715645838,
0.));
#138142=CARTESIAN_POINT('Ctrl Pts',(-50.8382481776403,-49.2866715645838,
12.));
#138143=CARTESIAN_POINT('Ctrl Pts',(-50.819084516434,-49.2769121258164,
0.));
#138144=CARTESIAN_POINT('Ctrl Pts',(-50.819084516434,-49.2769121258164,
12.));
#138145=CARTESIAN_POINT('Ctrl Pts',(-50.7999742907131,-49.2671550482435,
0.));
#138146=CARTESIAN_POINT('Ctrl Pts',(-50.7999742907131,-49.2671550482435,
12.));
#138147=CARTESIAN_POINT('Ctrl Pts',(-50.7809176052966,-49.2574004712134,
0.));
#138148=CARTESIAN_POINT('Ctrl Pts',(-50.7809176052966,-49.2574004712134,
12.));
#138149=CARTESIAN_POINT('Ctrl Pts',(-50.7619145655207,-49.2476485349373,
0.));
#138150=CARTESIAN_POINT('Ctrl Pts',(-50.7619145655207,-49.2476485349373,
12.));
#138151=CARTESIAN_POINT('Ctrl Pts',(-50.7429652772805,-49.2378993805471,
0.));
#138152=CARTESIAN_POINT('Ctrl Pts',(-50.7429652772805,-49.2378993805471,
12.));
#138153=CARTESIAN_POINT('Ctrl Pts',(-50.7240698470679,-49.228153150155,
0.));
#138154=CARTESIAN_POINT('Ctrl Pts',(-50.7240698470679,-49.228153150155,
12.));
#138155=CARTESIAN_POINT('Ctrl Pts',(-50.7052283818922,-49.2184099867461,
0.));
#138156=CARTESIAN_POINT('Ctrl Pts',(-50.7052283818922,-49.2184099867461,
12.));
#138157=CARTESIAN_POINT('Ctrl Pts',(-50.6864409891895,-49.2086700340614,
0.));
#138158=CARTESIAN_POINT('Ctrl Pts',(-50.6864409891895,-49.2086700340614,
12.));
#138159=CARTESIAN_POINT('Ctrl Pts',(-50.6677077767432,-49.1989334364996,
0.));
#138160=CARTESIAN_POINT('Ctrl Pts',(-50.6677077767432,-49.1989334364996,
12.));
#138161=CARTESIAN_POINT('Ctrl Pts',(-50.6490288525656,-49.189200338976,
0.));
#138162=CARTESIAN_POINT('Ctrl Pts',(-50.6490288525656,-49.189200338976,
12.));
#138163=CARTESIAN_POINT('Ctrl Pts',(-50.6304043248821,-49.1794708869099,
0.));
#138164=CARTESIAN_POINT('Ctrl Pts',(-50.6304043248821,-49.1794708869099,
12.));
#138165=CARTESIAN_POINT('Ctrl Pts',(-50.6118343023958,-49.1697452265494,
0.));
#138166=CARTESIAN_POINT('Ctrl Pts',(-50.6118343023958,-49.1697452265494,
12.));
#138167=CARTESIAN_POINT('Ctrl Pts',(-50.5933188945168,-49.1600235052621,
0.));
#138168=CARTESIAN_POINT('Ctrl Pts',(-50.5933188945168,-49.1600235052621,
12.));
#138169=CARTESIAN_POINT('Ctrl Pts',(-50.5748582115565,-49.1503058717821,
0.));
#138170=CARTESIAN_POINT('Ctrl Pts',(-50.5748582115565,-49.1503058717821,
12.));
#138171=CARTESIAN_POINT('Ctrl Pts',(-50.556452365038,-49.1405924766144,
0.));
#138172=CARTESIAN_POINT('Ctrl Pts',(-50.556452365038,-49.1405924766144,
12.));
#138173=CARTESIAN_POINT('Ctrl Pts',(-50.5381014674791,-49.1308834717615,
0.));
#138174=CARTESIAN_POINT('Ctrl Pts',(-50.5381014674791,-49.1308834717615,
12.));
#138175=CARTESIAN_POINT('Ctrl Pts',(-50.5198056318089,-49.1211790099795,
0.));
#138176=CARTESIAN_POINT('Ctrl Pts',(-50.5198056318089,-49.1211790099795,
12.));
#138177=CARTESIAN_POINT('Ctrl Pts',(-50.501564970874,-49.1114792441571,
0.));
#138178=CARTESIAN_POINT('Ctrl Pts',(-50.501564970874,-49.1114792441571,
12.));
#138179=CARTESIAN_POINT('Ctrl Pts',(-50.4833795969318,-49.1017843266803,
0.));
#138180=CARTESIAN_POINT('Ctrl Pts',(-50.4833795969318,-49.1017843266803,
12.));
#138181=CARTESIAN_POINT('Ctrl Pts',(-50.4652496210607,-49.0920944087008,
0.));
#138182=CARTESIAN_POINT('Ctrl Pts',(-50.4652496210607,-49.0920944087008,
12.));
#138183=CARTESIAN_POINT('Ctrl Pts',(-50.4471751542751,-49.0824096415371,
0.));
#138184=CARTESIAN_POINT('Ctrl Pts',(-50.4471751542751,-49.0824096415371,
12.));
#138185=CARTESIAN_POINT('Ctrl Pts',(-50.4291563088547,-49.0727301783494,
0.));
#138186=CARTESIAN_POINT('Ctrl Pts',(-50.4291563088547,-49.0727301783494,
12.));
#138187=CARTESIAN_POINT('Ctrl Pts',(-50.4111931994257,-49.0630561755075,
0.));
#138188=CARTESIAN_POINT('Ctrl Pts',(-50.4111931994257,-49.0630561755075,
12.));
#138189=CARTESIAN_POINT('Ctrl Pts',(-50.3932859445252,-49.0533877945744,
0.));
#138190=CARTESIAN_POINT('Ctrl Pts',(-50.3932859445252,-49.0533877945744,
12.));
#138191=CARTESIAN_POINT('Ctrl Pts',(-50.3754346667353,-49.0437252024832,
0.));
#138192=CARTESIAN_POINT('Ctrl Pts',(-50.3754346667353,-49.0437252024832,
12.));
#138193=CARTESIAN_POINT('Ctrl Pts',(-50.3576394894108,-49.0340685673982,
0.));
#138194=CARTESIAN_POINT('Ctrl Pts',(-50.3576394894108,-49.0340685673982,
12.));
#138195=CARTESIAN_POINT('Ctrl Pts',(-50.3399005337958,-49.024418055075,
0.));
#138196=CARTESIAN_POINT('Ctrl Pts',(-50.3399005337958,-49.024418055075,
12.));
#138197=CARTESIAN_POINT('Ctrl Pts',(-50.3222179165119,-49.0147738256942,
0.));
#138198=CARTESIAN_POINT('Ctrl Pts',(-50.3222179165119,-49.0147738256942,
12.));
#138199=CARTESIAN_POINT('Ctrl Pts',(-50.3045917455424,-49.0051360288044,
0.));
#138200=CARTESIAN_POINT('Ctrl Pts',(-50.3045917455424,-49.0051360288044,
12.));
#138201=CARTESIAN_POINT('Ctrl Pts',(-50.2870221241054,-48.9955048082081,
0.));
#138202=CARTESIAN_POINT('Ctrl Pts',(-50.2870221241054,-48.9955048082081,
12.));
#138203=CARTESIAN_POINT('Ctrl Pts',(-50.2695091583511,-48.9858803116689,
0.));
#138204=CARTESIAN_POINT('Ctrl Pts',(-50.2695091583511,-48.9858803116689,
12.));
#138205=CARTESIAN_POINT('Ctrl Pts',(-50.252052963548,-48.9762626987227,
0.));
#138206=CARTESIAN_POINT('Ctrl Pts',(-50.252052963548,-48.9762626987227,
12.));
#138207=CARTESIAN_POINT('Ctrl Pts',(-50.234653671541,-48.9666521500911,
0.));
#138208=CARTESIAN_POINT('Ctrl Pts',(-50.234653671541,-48.9666521500911,
12.));
#138209=CARTESIAN_POINT('Ctrl Pts',(-50.2173114358325,-48.9570488741167,
0.));
#138210=CARTESIAN_POINT('Ctrl Pts',(-50.2173114358325,-48.9570488741167,
12.));
#138211=CARTESIAN_POINT('Ctrl Pts',(-50.2000264157797,-48.9474530868733,
0.));
#138212=CARTESIAN_POINT('Ctrl Pts',(-50.2000264157797,-48.9474530868733,
12.));
#138213=CARTESIAN_POINT('Ctrl Pts',(-50.1827987615602,-48.9378649933055,
0.));
#138214=CARTESIAN_POINT('Ctrl Pts',(-50.1827987615602,-48.9378649933055,
12.));
#138215=CARTESIAN_POINT('Ctrl Pts',(-50.1656286003997,-48.9282847698294,
0.));
#138216=CARTESIAN_POINT('Ctrl Pts',(-50.1656286003997,-48.9282847698294,
12.));
#138217=CARTESIAN_POINT('Ctrl Pts',(-50.1485160184657,-48.9187125418099,
0.));
#138218=CARTESIAN_POINT('Ctrl Pts',(-50.1485160184657,-48.9187125418099,
12.));
#138219=CARTESIAN_POINT('Ctrl Pts',(-50.1314610602569,-48.90914838181,0.));
#138220=CARTESIAN_POINT('Ctrl Pts',(-50.1314610602569,-48.90914838181,12.));
#138221=CARTESIAN_POINT('Ctrl Pts',(-50.1178632067084,-48.9015035372055,
0.));
#138222=CARTESIAN_POINT('Ctrl Pts',(-50.1178632067084,-48.9015035372055,
12.));
#138223=CARTESIAN_POINT('Ctrl Pts',(-50.1076907555471,-48.895773555686,
0.));
#138224=CARTESIAN_POINT('Ctrl Pts',(-50.1076907555471,-48.895773555686,
12.));
#138225=CARTESIAN_POINT('Ctrl Pts',(-50.1009206494272,-48.8919551910366,
0.));
#138226=CARTESIAN_POINT('Ctrl Pts',(-50.1009206494272,-48.8919551910366,
12.));
#138227=CARTESIAN_POINT('Ctrl Pts',(-50.0975384783635,-48.8900464144686,
0.));
#138228=CARTESIAN_POINT('Ctrl Pts',(-50.0975384783635,-48.8900464144686,
12.));
#138229=CARTESIAN_POINT('',(-50.0975384783635,-48.8900464144686,12.));
#138230=CARTESIAN_POINT('Ctrl Pts',(-50.0975384783635,-48.8900464144686,
12.));
#138231=CARTESIAN_POINT('Ctrl Pts',(-50.1009206494272,-48.8919551910366,
12.));
#138232=CARTESIAN_POINT('Ctrl Pts',(-50.1076907555471,-48.895773555686,
12.));
#138233=CARTESIAN_POINT('Ctrl Pts',(-50.1178632067084,-48.9015035372055,
12.));
#138234=CARTESIAN_POINT('Ctrl Pts',(-50.1314610602569,-48.90914838181,12.));
#138235=CARTESIAN_POINT('Ctrl Pts',(-50.1485160184657,-48.9187125418099,
12.));
#138236=CARTESIAN_POINT('Ctrl Pts',(-50.1656286003997,-48.9282847698294,
12.));
#138237=CARTESIAN_POINT('Ctrl Pts',(-50.1827987615602,-48.9378649933055,
12.));
#138238=CARTESIAN_POINT('Ctrl Pts',(-50.2000264157797,-48.9474530868733,
12.));
#138239=CARTESIAN_POINT('Ctrl Pts',(-50.2173114358325,-48.9570488741167,
12.));
#138240=CARTESIAN_POINT('Ctrl Pts',(-50.234653671541,-48.9666521500911,
12.));
#138241=CARTESIAN_POINT('Ctrl Pts',(-50.252052963548,-48.9762626987227,
12.));
#138242=CARTESIAN_POINT('Ctrl Pts',(-50.2695091583511,-48.9858803116689,
12.));
#138243=CARTESIAN_POINT('Ctrl Pts',(-50.2870221241054,-48.9955048082081,
12.));
#138244=CARTESIAN_POINT('Ctrl Pts',(-50.3045917455424,-49.0051360288044,
12.));
#138245=CARTESIAN_POINT('Ctrl Pts',(-50.3222179165119,-49.0147738256942,
12.));
#138246=CARTESIAN_POINT('Ctrl Pts',(-50.3399005337958,-49.024418055075,
12.));
#138247=CARTESIAN_POINT('Ctrl Pts',(-50.3576394894108,-49.0340685673982,
12.));
#138248=CARTESIAN_POINT('Ctrl Pts',(-50.3754346667353,-49.0437252024832,
12.));
#138249=CARTESIAN_POINT('Ctrl Pts',(-50.3932859445252,-49.0533877945744,
12.));
#138250=CARTESIAN_POINT('Ctrl Pts',(-50.4111931994257,-49.0630561755075,
12.));
#138251=CARTESIAN_POINT('Ctrl Pts',(-50.4291563088547,-49.0727301783494,
12.));
#138252=CARTESIAN_POINT('Ctrl Pts',(-50.4471751542751,-49.0824096415371,
12.));
#138253=CARTESIAN_POINT('Ctrl Pts',(-50.4652496210607,-49.0920944087008,
12.));
#138254=CARTESIAN_POINT('Ctrl Pts',(-50.4833795969318,-49.1017843266803,
12.));
#138255=CARTESIAN_POINT('Ctrl Pts',(-50.501564970874,-49.1114792441571,
12.));
#138256=CARTESIAN_POINT('Ctrl Pts',(-50.5198056318089,-49.1211790099795,
12.));
#138257=CARTESIAN_POINT('Ctrl Pts',(-50.5381014674791,-49.1308834717615,
12.));
#138258=CARTESIAN_POINT('Ctrl Pts',(-50.556452365038,-49.1405924766144,
12.));
#138259=CARTESIAN_POINT('Ctrl Pts',(-50.5748582115565,-49.1503058717821,
12.));
#138260=CARTESIAN_POINT('Ctrl Pts',(-50.5933188945168,-49.1600235052621,
12.));
#138261=CARTESIAN_POINT('Ctrl Pts',(-50.6118343023958,-49.1697452265494,
12.));
#138262=CARTESIAN_POINT('Ctrl Pts',(-50.6304043248821,-49.1794708869099,
12.));
#138263=CARTESIAN_POINT('Ctrl Pts',(-50.6490288525656,-49.189200338976,
12.));
#138264=CARTESIAN_POINT('Ctrl Pts',(-50.6677077767432,-49.1989334364996,
12.));
#138265=CARTESIAN_POINT('Ctrl Pts',(-50.6864409891895,-49.2086700340614,
12.));
#138266=CARTESIAN_POINT('Ctrl Pts',(-50.7052283818922,-49.2184099867461,
12.));
#138267=CARTESIAN_POINT('Ctrl Pts',(-50.7240698470679,-49.228153150155,
12.));
#138268=CARTESIAN_POINT('Ctrl Pts',(-50.7429652772805,-49.2378993805471,
12.));
#138269=CARTESIAN_POINT('Ctrl Pts',(-50.7619145655207,-49.2476485349373,
12.));
#138270=CARTESIAN_POINT('Ctrl Pts',(-50.7809176052966,-49.2574004712134,
12.));
#138271=CARTESIAN_POINT('Ctrl Pts',(-50.7999742907131,-49.2671550482435,
12.));
#138272=CARTESIAN_POINT('Ctrl Pts',(-50.819084516434,-49.2769121258164,
12.));
#138273=CARTESIAN_POINT('Ctrl Pts',(-50.8382481776403,-49.2866715645838,
12.));
#138274=CARTESIAN_POINT('Ctrl Pts',(-50.8574651699873,-49.2964332260039,
12.));
#138275=CARTESIAN_POINT('Ctrl Pts',(-50.8767353895492,-49.3061969722781,
12.));
#138276=CARTESIAN_POINT('Ctrl Pts',(-50.8960587327848,-49.3159626663109,
12.));
#138277=CARTESIAN_POINT('Ctrl Pts',(-50.9154350965666,-49.3257301717335,
12.));
#138278=CARTESIAN_POINT('Ctrl Pts',(-50.9348643781924,-49.3354993529159,
12.));
#138279=CARTESIAN_POINT('Ctrl Pts',(-50.9543464753981,-49.345270074981,
12.));
#138280=CARTESIAN_POINT('Ctrl Pts',(-50.9738812863646,-49.355042203823,
12.));
#138281=CARTESIAN_POINT('Ctrl Pts',(-50.9934687097188,-49.3648156061058,
12.));
#138282=CARTESIAN_POINT('Ctrl Pts',(-51.0131086445272,-49.3745901492432,
12.));
#138283=CARTESIAN_POINT('Ctrl Pts',(-51.0328009902858,-49.3843657013852,
12.));
#138284=CARTESIAN_POINT('Ctrl Pts',(-51.052545646907,-49.3941421314013,
12.));
#138285=CARTESIAN_POINT('Ctrl Pts',(-51.0723425146985,-49.4039193088634,
12.));
#138286=CARTESIAN_POINT('Ctrl Pts',(-51.0921914943662,-49.4136971040428,
12.));
#138287=CARTESIAN_POINT('Ctrl Pts',(-51.1120924870195,-49.423475387907,
12.));
#138288=CARTESIAN_POINT('Ctrl Pts',(-51.1320453941702,-49.4332540321178,
12.));
#138289=CARTESIAN_POINT('Ctrl Pts',(-51.1520501177291,-49.4430329090287,
12.));
#138290=CARTESIAN_POINT('Ctrl Pts',(-51.1721065599973,-49.4528118916832,
12.));
#138291=CARTESIAN_POINT('Ctrl Pts',(-51.1922146236686,-49.4625908538074,
12.));
#138292=CARTESIAN_POINT('Ctrl Pts',(-51.2123742118287,-49.4723696698021,
12.));
#138293=CARTESIAN_POINT('Ctrl Pts',(-51.2325852279506,-49.4821482147356,
12.));
#138294=CARTESIAN_POINT('Ctrl Pts',(-51.2528475758846,-49.4919263643362,
12.));
#138295=CARTESIAN_POINT('Ctrl Pts',(-51.2731611598475,-49.5017039949852,
12.));
#138296=CARTESIAN_POINT('Ctrl Pts',(-51.2935258844289,-49.5114809837122,
12.));
#138297=CARTESIAN_POINT('Ctrl Pts',(-51.313941654591,-49.5212572081908,
12.));
#138298=CARTESIAN_POINT('Ctrl Pts',(-51.3344083756657,-49.5310325467332,
12.));
#138299=CARTESIAN_POINT('Ctrl Pts',(-51.3549259533458,-49.5408068782859,
12.));
#138300=CARTESIAN_POINT('Ctrl Pts',(-51.3754942936778,-49.550580082425,
12.));
#138301=CARTESIAN_POINT('Ctrl Pts',(-51.396113303067,-49.5603520393496,
12.));
#138302=CARTESIAN_POINT('Ctrl Pts',(-51.4167828882756,-49.5701226298769,
12.));
#138303=CARTESIAN_POINT('Ctrl Pts',(-51.4375029564197,-49.5798917354366,
12.));
#138304=CARTESIAN_POINT('Ctrl Pts',(-51.4582734149583,-49.5896592380654,
12.));
#138305=CARTESIAN_POINT('Ctrl Pts',(-51.4790941716888,-49.5994250204031,
12.));
#138306=CARTESIAN_POINT('Ctrl Pts',(-51.4999651347523,-49.6091889656866,
12.));
#138307=CARTESIAN_POINT('Ctrl Pts',(-51.5208862126315,-49.6189509577452,
12.));
#138308=CARTESIAN_POINT('Ctrl Pts',(-51.5418573141484,-49.6287108809966,
12.));
#138309=CARTESIAN_POINT('Ctrl Pts',(-51.5628783484525,-49.6384686204413,
12.));
#138310=CARTESIAN_POINT('Ctrl Pts',(-51.5839492250181,-49.6482240616593,
12.));
#138311=CARTESIAN_POINT('Ctrl Pts',(-51.6050698536496,-49.6579770908037,
12.));
#138312=CARTESIAN_POINT('Ctrl Pts',(-51.626240144479,-49.6677275945967,
12.));
#138313=CARTESIAN_POINT('Ctrl Pts',(-51.6474600079622,-49.6774754603245,
12.));
#138314=CARTESIAN_POINT('Ctrl Pts',(-51.6687293548682,-49.6872205758336,
12.));
#138315=CARTESIAN_POINT('Ctrl Pts',(-51.6900480962773,-49.6969628295262,
12.));
#138316=CARTESIAN_POINT('Ctrl Pts',(-51.7114161435869,-49.7067021103553,
12.));
#138317=CARTESIAN_POINT('Ctrl Pts',(-51.7328334085091,-49.7164383078212,
12.));
#138318=CARTESIAN_POINT('Ctrl Pts',(-51.754299803067,-49.7261713119663,
12.));
#138319=CARTESIAN_POINT('Ctrl Pts',(-51.7758152395836,-49.7359010133721,
12.));
#138320=CARTESIAN_POINT('Ctrl Pts',(-51.7973796306803,-49.7456273031534,
12.));
#138321=CARTESIAN_POINT('Ctrl Pts',(-51.8189928892828,-49.755350072955,
12.));
#138322=CARTESIAN_POINT('Ctrl Pts',(-51.8406549286175,-49.7650692149462,
12.));
#138323=CARTESIAN_POINT('Ctrl Pts',(-51.8623656622097,-49.7747846218182,
12.));
#138324=CARTESIAN_POINT('Ctrl Pts',(-51.8841250038724,-49.7844961867808,
12.));
#138325=CARTESIAN_POINT('Ctrl Pts',(-51.9059328677059,-49.7942038035576,
12.));
#138326=CARTESIAN_POINT('Ctrl Pts',(-51.9277891681018,-49.8039073663812,
12.));
#138327=CARTESIAN_POINT('Ctrl Pts',(-51.9496938197418,-49.8136067699896,
12.));
#138328=CARTESIAN_POINT('Ctrl Pts',(-51.9716467375937,-49.8233019096222,
12.));
#138329=CARTESIAN_POINT('Ctrl Pts',(-51.9936478369008,-49.8329926810172,
12.));
#138330=CARTESIAN_POINT('Ctrl Pts',(-52.0156970331823,-49.8426789804071,
12.));
#138331=CARTESIAN_POINT('Ctrl Pts',(-52.0377942422376,-49.8523607045149,
12.));
#138332=CARTESIAN_POINT('Ctrl Pts',(-52.0599393801452,-49.86203775055,12.));
#138333=CARTESIAN_POINT('Ctrl Pts',(-52.0821323632587,-49.8717100162048,
12.));
#138334=CARTESIAN_POINT('Ctrl Pts',(-52.1043731081962,-49.8813773996517,
12.));
#138335=CARTESIAN_POINT('Ctrl Pts',(-52.1266615318407,-49.8910397995397,
12.));
#138336=CARTESIAN_POINT('Ctrl Pts',(-52.1489975513445,-49.9006971149895,
12.));
#138337=CARTESIAN_POINT('Ctrl Pts',(-52.1713810841276,-49.9103492455902,
12.));
#138338=CARTESIAN_POINT('Ctrl Pts',(-52.1938120478754,-49.9199960913962,
12.));
#138339=CARTESIAN_POINT('Ctrl Pts',(-52.2162903605275,-49.9296375529245,
12.));
#138340=CARTESIAN_POINT('Ctrl Pts',(-52.2388159402771,-49.9392735311509,
12.));
#138341=CARTESIAN_POINT('Ctrl Pts',(-52.2613887055773,-49.9489039275064,
12.));
#138342=CARTESIAN_POINT('Ctrl Pts',(-52.2840085751384,-49.9585286438733,
12.));
#138343=CARTESIAN_POINT('Ctrl Pts',(-52.3066754679265,-49.9681475825824,
12.));
#138344=CARTESIAN_POINT('Ctrl Pts',(-52.3293893031528,-49.9777606464106,
12.));
#138345=CARTESIAN_POINT('Ctrl Pts',(-52.3521500002718,-49.9873677385775,
12.));
#138346=CARTESIAN_POINT('Ctrl Pts',(-52.3749574789871,-49.9969687627408,
12.));
#138347=CARTESIAN_POINT('Ctrl Pts',(-52.3978116592509,-50.0065636229938,
12.));
#138348=CARTESIAN_POINT('Ctrl Pts',(-52.4207124612608,-50.0161522238616,
12.));
#138349=CARTESIAN_POINT('Ctrl Pts',(-52.4436598054515,-50.0257344703,12.));
#138350=CARTESIAN_POINT('Ctrl Pts',(-52.4666536124913,-50.0353102676921,
12.));
#138351=CARTESIAN_POINT('Ctrl Pts',(-52.4896938032884,-50.0448795218441,
12.));
#138352=CARTESIAN_POINT('Ctrl Pts',(-52.5127802989896,-50.0544421389818,
12.));
#138353=CARTESIAN_POINT('Ctrl Pts',(-52.5359130209792,-50.0639980257479,
12.));
#138354=CARTESIAN_POINT('Ctrl Pts',(-52.5590918908702,-50.0735470892007,
12.));
#138355=CARTESIAN_POINT('Ctrl Pts',(-52.5823168304994,-50.0830892368107,
12.));
#138356=CARTESIAN_POINT('Ctrl Pts',(-52.6055877619348,-50.0926243764578,
12.));
#138357=CARTESIAN_POINT('Ctrl Pts',(-52.6289046074746,-50.1021524164264,
12.));
#138358=CARTESIAN_POINT('Ctrl Pts',(-52.652267289646,-50.111673265404,12.));
#138359=CARTESIAN_POINT('Ctrl Pts',(-52.6756757311978,-50.1211868324781,
12.));
#138360=CARTESIAN_POINT('Ctrl Pts',(-52.699129855093,-50.1306930271345,
12.));
#138361=CARTESIAN_POINT('Ctrl Pts',(-52.7226295845161,-50.1401917592537,
12.));
#138362=CARTESIAN_POINT('Ctrl Pts',(-52.7461748428738,-50.1496829391073,
12.));
#138363=CARTESIAN_POINT('Ctrl Pts',(-52.769765553794,-50.1591664773561,
12.));
#138364=CARTESIAN_POINT('Ctrl Pts',(-52.7934016411205,-50.1686422850488,
12.));
#138365=CARTESIAN_POINT('Ctrl Pts',(-52.8170830289044,-50.1781102736205,
12.));
#138366=CARTESIAN_POINT('Ctrl Pts',(-52.8408096414093,-50.1875703548884,
12.));
#138367=CARTESIAN_POINT('Ctrl Pts',(-52.8645814031133,-50.1970224410471,
12.));
#138368=CARTESIAN_POINT('Ctrl Pts',(-52.8883982387068,-50.2064664446663,
12.));
#138369=CARTESIAN_POINT('Ctrl Pts',(-52.9122600730884,-50.2159022786879,
12.));
#138370=CARTESIAN_POINT('Ctrl Pts',(-52.9361668313542,-50.2253298564241,
12.));
#138371=CARTESIAN_POINT('Ctrl Pts',(-52.9601184388028,-50.2347490915555,
12.));
#138372=CARTESIAN_POINT('Ctrl Pts',(-52.9841148209402,-50.2441598981286,
12.));
#138373=CARTESIAN_POINT('Ctrl Pts',(-53.0081559034801,-50.2535621905552,
12.));
#138374=CARTESIAN_POINT('Ctrl Pts',(-53.0322416123406,-50.2629558836111,
12.));
#138375=CARTESIAN_POINT('Ctrl Pts',(-53.0563718736366,-50.2723408924373,
12.));
#138376=CARTESIAN_POINT('Ctrl Pts',(-53.0805466136798,-50.2817171325358,
12.));
#138377=CARTESIAN_POINT('Ctrl Pts',(-53.1047657589812,-50.2910845197619,
12.));
#138378=CARTESIAN_POINT('Ctrl Pts',(-53.1290292362485,-50.300442970319,
12.));
#138379=CARTESIAN_POINT('Ctrl Pts',(-53.1533369723818,-50.3097924007534,
12.));
#138380=CARTESIAN_POINT('Ctrl Pts',(-53.1776888944616,-50.3191327279493,
12.));
#138381=CARTESIAN_POINT('Ctrl Pts',(-53.2020849297471,-50.3284638691278,
12.));
#138382=CARTESIAN_POINT('Ctrl Pts',(-53.2265250056887,-50.3377857418515,
12.));
#138383=CARTESIAN_POINT('Ctrl Pts',(-53.2510090499336,-50.3470982640289,
12.));
#138384=CARTESIAN_POINT('Ctrl Pts',(-53.2755369903293,-50.3564013539199,
12.));
#138385=CARTESIAN_POINT('Ctrl Pts',(-53.300108754923,-50.365694930143,12.));
#138386=CARTESIAN_POINT('Ctrl Pts',(-53.3247242719587,-50.3749789116786,
12.));
#138387=CARTESIAN_POINT('Ctrl Pts',(-53.3493834698697,-50.384253217846,
12.));
#138388=CARTESIAN_POINT('Ctrl Pts',(-53.3740862772681,-50.3935177682837,
12.));
#138389=CARTESIAN_POINT('Ctrl Pts',(-53.398832622931,-50.4027724829297,
12.));
#138390=CARTESIAN_POINT('Ctrl Pts',(-53.4236224357838,-50.4120172820047,
12.));
#138391=CARTESIAN_POINT('Ctrl Pts',(-53.4484556448776,-50.4212520859914,
12.));
#138392=CARTESIAN_POINT('Ctrl Pts',(-53.4733321794188,-50.4304768156667,
12.));
#138393=CARTESIAN_POINT('Ctrl Pts',(-53.4982519688024,-50.4396913921382,
12.));
#138394=CARTESIAN_POINT('Ctrl Pts',(-53.5232149426413,-50.4488957368839,
12.));
#138395=CARTESIAN_POINT('Ctrl Pts',(-53.5482210307868,-50.4580897717838,
12.));
#138396=CARTESIAN_POINT('Ctrl Pts',(-53.5732701633609,-50.4672734191756,
12.));
#138397=CARTESIAN_POINT('Ctrl Pts',(-53.5983622707238,-50.4764466018071,
12.));
#138398=CARTESIAN_POINT('Ctrl Pts',(-53.623497283406,-50.4856092427314,
12.));
#138399=CARTESIAN_POINT('Ctrl Pts',(-53.6486751320436,-50.4947612652149,
12.));
#138400=CARTESIAN_POINT('Ctrl Pts',(-53.6738957473158,-50.503902592653,
12.));
#138401=CARTESIAN_POINT('Ctrl Pts',(-53.6991590598548,-50.513033148456,
12.));
#138402=CARTESIAN_POINT('Ctrl Pts',(-53.7244650002374,-50.522152856042,
12.));
#138403=CARTESIAN_POINT('Ctrl Pts',(-53.7498134991703,-50.5312616390779,
12.));
#138404=CARTESIAN_POINT('Ctrl Pts',(-53.7752044876304,-50.5403594216698,
12.));
#138405=CARTESIAN_POINT('Ctrl Pts',(-53.8006378970197,-50.5494461285761,
12.));
#138406=CARTESIAN_POINT('Ctrl Pts',(-53.8261136593075,-50.5585216854091,
12.));
#138407=CARTESIAN_POINT('Ctrl Pts',(-53.8516317071804,-50.5675860188538,
12.));
#138408=CARTESIAN_POINT('Ctrl Pts',(-53.8771919737032,-50.5766390561884,
12.));
#138409=CARTESIAN_POINT('Ctrl Pts',(-53.9027943919836,-50.5856807248151,
12.));
#138410=CARTESIAN_POINT('Ctrl Pts',(-53.9284388948004,-50.5947109517483,
12.));
#138411=CARTESIAN_POINT('Ctrl Pts',(-53.9541254143119,-50.603729663214,
12.));
#138412=CARTESIAN_POINT('Ctrl Pts',(-53.979853881553,-50.6127367839711,
12.));
#138413=CARTESIAN_POINT('Ctrl Pts',(-54.0056242268399,-50.6217322378648,
12.));
#138414=CARTESIAN_POINT('Ctrl Pts',(-54.0314363806708,-50.6307159490553,
12.));
#138415=CARTESIAN_POINT('Ctrl Pts',(-54.0572902745076,-50.6396878430939,
12.));
#138416=CARTESIAN_POINT('Ctrl Pts',(-54.0831858415189,-50.6486478479465,
12.));
#138417=CARTESIAN_POINT('Ctrl Pts',(-54.1091230175367,-50.6575958953221,
12.));
#138418=CARTESIAN_POINT('Ctrl Pts',(-54.1351017412804,-50.6665319209869,
12.));
#138419=CARTESIAN_POINT('Ctrl Pts',(-54.1574061042043,-50.6741814675486,
12.));
#138420=CARTESIAN_POINT('Ctrl Pts',(-54.1745287898797,-50.6800396668778,
12.));
#138421=CARTESIAN_POINT('Ctrl Pts',(-54.1864514382196,-50.6841118861931,
12.));
#138422=CARTESIAN_POINT('Ctrl Pts',(-54.1931619277624,-50.6864016965744,
12.));
#138423=CARTESIAN_POINT('Ctrl Pts',(-54.1946543500373,-50.6869108458851,
12.));
#138424=CARTESIAN_POINT('',(-50.0975384783635,-48.8900464144686,0.));
#138425=CARTESIAN_POINT('',(-50.0975384783634,-48.8900464144686,0.));
#138426=CARTESIAN_POINT('Ctrl Pts',(-54.1946543500373,-50.6869108458851,
0.));
#138427=CARTESIAN_POINT('Ctrl Pts',(-54.1931619277624,-50.6864016965744,
0.));
#138428=CARTESIAN_POINT('Ctrl Pts',(-54.1864514382196,-50.6841118861931,
0.));
#138429=CARTESIAN_POINT('Ctrl Pts',(-54.1745287898797,-50.6800396668778,
0.));
#138430=CARTESIAN_POINT('Ctrl Pts',(-54.1574061042043,-50.6741814675486,
0.));
#138431=CARTESIAN_POINT('Ctrl Pts',(-54.1351017412804,-50.6665319209869,
0.));
#138432=CARTESIAN_POINT('Ctrl Pts',(-54.1091230175367,-50.6575958953221,
0.));
#138433=CARTESIAN_POINT('Ctrl Pts',(-54.0831858415189,-50.6486478479465,
0.));
#138434=CARTESIAN_POINT('Ctrl Pts',(-54.0572902745076,-50.6396878430939,
0.));
#138435=CARTESIAN_POINT('Ctrl Pts',(-54.0314363806708,-50.6307159490553,
0.));
#138436=CARTESIAN_POINT('Ctrl Pts',(-54.0056242268399,-50.6217322378648,
0.));
#138437=CARTESIAN_POINT('Ctrl Pts',(-53.979853881553,-50.6127367839711,
0.));
#138438=CARTESIAN_POINT('Ctrl Pts',(-53.9541254143119,-50.603729663214,
0.));
#138439=CARTESIAN_POINT('Ctrl Pts',(-53.9284388948004,-50.5947109517483,
0.));
#138440=CARTESIAN_POINT('Ctrl Pts',(-53.9027943919836,-50.5856807248151,
0.));
#138441=CARTESIAN_POINT('Ctrl Pts',(-53.8771919737032,-50.5766390561884,
0.));
#138442=CARTESIAN_POINT('Ctrl Pts',(-53.8516317071804,-50.5675860188538,
0.));
#138443=CARTESIAN_POINT('Ctrl Pts',(-53.8261136593075,-50.5585216854091,
0.));
#138444=CARTESIAN_POINT('Ctrl Pts',(-53.8006378970197,-50.5494461285761,
0.));
#138445=CARTESIAN_POINT('Ctrl Pts',(-53.7752044876304,-50.5403594216698,
0.));
#138446=CARTESIAN_POINT('Ctrl Pts',(-53.7498134991703,-50.5312616390779,
0.));
#138447=CARTESIAN_POINT('Ctrl Pts',(-53.7244650002374,-50.522152856042,
0.));
#138448=CARTESIAN_POINT('Ctrl Pts',(-53.6991590598548,-50.513033148456,
0.));
#138449=CARTESIAN_POINT('Ctrl Pts',(-53.6738957473158,-50.503902592653,
0.));
#138450=CARTESIAN_POINT('Ctrl Pts',(-53.6486751320436,-50.4947612652149,
0.));
#138451=CARTESIAN_POINT('Ctrl Pts',(-53.623497283406,-50.4856092427314,
0.));
#138452=CARTESIAN_POINT('Ctrl Pts',(-53.5983622707238,-50.4764466018071,
0.));
#138453=CARTESIAN_POINT('Ctrl Pts',(-53.5732701633609,-50.4672734191756,
0.));
#138454=CARTESIAN_POINT('Ctrl Pts',(-53.5482210307868,-50.4580897717838,
0.));
#138455=CARTESIAN_POINT('Ctrl Pts',(-53.5232149426413,-50.4488957368839,
0.));
#138456=CARTESIAN_POINT('Ctrl Pts',(-53.4982519688024,-50.4396913921382,
0.));
#138457=CARTESIAN_POINT('Ctrl Pts',(-53.4733321794188,-50.4304768156667,
0.));
#138458=CARTESIAN_POINT('Ctrl Pts',(-53.4484556448776,-50.4212520859914,
0.));
#138459=CARTESIAN_POINT('Ctrl Pts',(-53.4236224357838,-50.4120172820047,
0.));
#138460=CARTESIAN_POINT('Ctrl Pts',(-53.398832622931,-50.4027724829297,
0.));
#138461=CARTESIAN_POINT('Ctrl Pts',(-53.3740862772681,-50.3935177682837,
0.));
#138462=CARTESIAN_POINT('Ctrl Pts',(-53.3493834698697,-50.384253217846,
0.));
#138463=CARTESIAN_POINT('Ctrl Pts',(-53.3247242719587,-50.3749789116786,
0.));
#138464=CARTESIAN_POINT('Ctrl Pts',(-53.300108754923,-50.365694930143,0.));
#138465=CARTESIAN_POINT('Ctrl Pts',(-53.2755369903293,-50.3564013539199,
0.));
#138466=CARTESIAN_POINT('Ctrl Pts',(-53.2510090499336,-50.3470982640289,
0.));
#138467=CARTESIAN_POINT('Ctrl Pts',(-53.2265250056887,-50.3377857418515,
0.));
#138468=CARTESIAN_POINT('Ctrl Pts',(-53.2020849297471,-50.3284638691278,
0.));
#138469=CARTESIAN_POINT('Ctrl Pts',(-53.1776888944616,-50.3191327279493,
0.));
#138470=CARTESIAN_POINT('Ctrl Pts',(-53.1533369723818,-50.3097924007534,
0.));
#138471=CARTESIAN_POINT('Ctrl Pts',(-53.1290292362485,-50.300442970319,
0.));
#138472=CARTESIAN_POINT('Ctrl Pts',(-53.1047657589812,-50.2910845197619,
0.));
#138473=CARTESIAN_POINT('Ctrl Pts',(-53.0805466136798,-50.2817171325358,
0.));
#138474=CARTESIAN_POINT('Ctrl Pts',(-53.0563718736366,-50.2723408924373,
0.));
#138475=CARTESIAN_POINT('Ctrl Pts',(-53.0322416123406,-50.2629558836111,
0.));
#138476=CARTESIAN_POINT('Ctrl Pts',(-53.0081559034801,-50.2535621905552,
0.));
#138477=CARTESIAN_POINT('Ctrl Pts',(-52.9841148209402,-50.2441598981286,
0.));
#138478=CARTESIAN_POINT('Ctrl Pts',(-52.9601184388028,-50.2347490915555,
0.));
#138479=CARTESIAN_POINT('Ctrl Pts',(-52.9361668313542,-50.2253298564241,
0.));
#138480=CARTESIAN_POINT('Ctrl Pts',(-52.9122600730884,-50.2159022786879,
0.));
#138481=CARTESIAN_POINT('Ctrl Pts',(-52.8883982387068,-50.2064664446663,
0.));
#138482=CARTESIAN_POINT('Ctrl Pts',(-52.8645814031133,-50.1970224410471,
0.));
#138483=CARTESIAN_POINT('Ctrl Pts',(-52.8408096414093,-50.1875703548884,
0.));
#138484=CARTESIAN_POINT('Ctrl Pts',(-52.8170830289044,-50.1781102736205,
0.));
#138485=CARTESIAN_POINT('Ctrl Pts',(-52.7934016411205,-50.1686422850488,
0.));
#138486=CARTESIAN_POINT('Ctrl Pts',(-52.769765553794,-50.1591664773561,
0.));
#138487=CARTESIAN_POINT('Ctrl Pts',(-52.7461748428738,-50.1496829391073,
0.));
#138488=CARTESIAN_POINT('Ctrl Pts',(-52.7226295845161,-50.1401917592537,
0.));
#138489=CARTESIAN_POINT('Ctrl Pts',(-52.699129855093,-50.1306930271345,
0.));
#138490=CARTESIAN_POINT('Ctrl Pts',(-52.6756757311978,-50.1211868324781,
0.));
#138491=CARTESIAN_POINT('Ctrl Pts',(-52.652267289646,-50.111673265404,0.));
#138492=CARTESIAN_POINT('Ctrl Pts',(-52.6289046074746,-50.1021524164264,
0.));
#138493=CARTESIAN_POINT('Ctrl Pts',(-52.6055877619348,-50.0926243764578,
0.));
#138494=CARTESIAN_POINT('Ctrl Pts',(-52.5823168304994,-50.0830892368107,
0.));
#138495=CARTESIAN_POINT('Ctrl Pts',(-52.5590918908702,-50.0735470892007,
0.));
#138496=CARTESIAN_POINT('Ctrl Pts',(-52.5359130209792,-50.0639980257479,
0.));
#138497=CARTESIAN_POINT('Ctrl Pts',(-52.5127802989896,-50.0544421389818,
0.));
#138498=CARTESIAN_POINT('Ctrl Pts',(-52.4896938032884,-50.0448795218441,
0.));
#138499=CARTESIAN_POINT('Ctrl Pts',(-52.4666536124913,-50.0353102676921,
0.));
#138500=CARTESIAN_POINT('Ctrl Pts',(-52.4436598054515,-50.0257344703,0.));
#138501=CARTESIAN_POINT('Ctrl Pts',(-52.4207124612608,-50.0161522238616,
0.));
#138502=CARTESIAN_POINT('Ctrl Pts',(-52.3978116592509,-50.0065636229938,
0.));
#138503=CARTESIAN_POINT('Ctrl Pts',(-52.3749574789871,-49.9969687627408,
0.));
#138504=CARTESIAN_POINT('Ctrl Pts',(-52.3521500002718,-49.9873677385775,
0.));
#138505=CARTESIAN_POINT('Ctrl Pts',(-52.3293893031528,-49.9777606464106,
0.));
#138506=CARTESIAN_POINT('Ctrl Pts',(-52.3066754679265,-49.9681475825824,
0.));
#138507=CARTESIAN_POINT('Ctrl Pts',(-52.2840085751384,-49.9585286438733,
0.));
#138508=CARTESIAN_POINT('Ctrl Pts',(-52.2613887055773,-49.9489039275064,
0.));
#138509=CARTESIAN_POINT('Ctrl Pts',(-52.2388159402771,-49.9392735311509,
0.));
#138510=CARTESIAN_POINT('Ctrl Pts',(-52.2162903605275,-49.9296375529245,
0.));
#138511=CARTESIAN_POINT('Ctrl Pts',(-52.1938120478754,-49.9199960913962,
0.));
#138512=CARTESIAN_POINT('Ctrl Pts',(-52.1713810841276,-49.9103492455902,
0.));
#138513=CARTESIAN_POINT('Ctrl Pts',(-52.1489975513445,-49.9006971149895,
0.));
#138514=CARTESIAN_POINT('Ctrl Pts',(-52.1266615318407,-49.8910397995397,
0.));
#138515=CARTESIAN_POINT('Ctrl Pts',(-52.1043731081962,-49.8813773996517,
0.));
#138516=CARTESIAN_POINT('Ctrl Pts',(-52.0821323632587,-49.8717100162048,
0.));
#138517=CARTESIAN_POINT('Ctrl Pts',(-52.0599393801452,-49.86203775055,0.));
#138518=CARTESIAN_POINT('Ctrl Pts',(-52.0377942422376,-49.8523607045149,
0.));
#138519=CARTESIAN_POINT('Ctrl Pts',(-52.0156970331823,-49.8426789804071,
0.));
#138520=CARTESIAN_POINT('Ctrl Pts',(-51.9936478369008,-49.8329926810172,
0.));
#138521=CARTESIAN_POINT('Ctrl Pts',(-51.9716467375937,-49.8233019096222,
0.));
#138522=CARTESIAN_POINT('Ctrl Pts',(-51.9496938197418,-49.8136067699896,
0.));
#138523=CARTESIAN_POINT('Ctrl Pts',(-51.9277891681018,-49.8039073663812,
0.));
#138524=CARTESIAN_POINT('Ctrl Pts',(-51.9059328677059,-49.7942038035576,
0.));
#138525=CARTESIAN_POINT('Ctrl Pts',(-51.8841250038724,-49.7844961867808,
0.));
#138526=CARTESIAN_POINT('Ctrl Pts',(-51.8623656622097,-49.7747846218182,
0.));
#138527=CARTESIAN_POINT('Ctrl Pts',(-51.8406549286175,-49.7650692149462,
0.));
#138528=CARTESIAN_POINT('Ctrl Pts',(-51.8189928892828,-49.755350072955,
0.));
#138529=CARTESIAN_POINT('Ctrl Pts',(-51.7973796306803,-49.7456273031534,
0.));
#138530=CARTESIAN_POINT('Ctrl Pts',(-51.7758152395836,-49.7359010133721,
0.));
#138531=CARTESIAN_POINT('Ctrl Pts',(-51.754299803067,-49.7261713119663,
0.));
#138532=CARTESIAN_POINT('Ctrl Pts',(-51.7328334085091,-49.7164383078212,
0.));
#138533=CARTESIAN_POINT('Ctrl Pts',(-51.7114161435869,-49.7067021103553,
0.));
#138534=CARTESIAN_POINT('Ctrl Pts',(-51.6900480962773,-49.6969628295262,
0.));
#138535=CARTESIAN_POINT('Ctrl Pts',(-51.6687293548682,-49.6872205758336,
0.));
#138536=CARTESIAN_POINT('Ctrl Pts',(-51.6474600079622,-49.6774754603245,
0.));
#138537=CARTESIAN_POINT('Ctrl Pts',(-51.626240144479,-49.6677275945967,
0.));
#138538=CARTESIAN_POINT('Ctrl Pts',(-51.6050698536496,-49.6579770908037,
0.));
#138539=CARTESIAN_POINT('Ctrl Pts',(-51.5839492250181,-49.6482240616593,
0.));
#138540=CARTESIAN_POINT('Ctrl Pts',(-51.5628783484525,-49.6384686204413,
0.));
#138541=CARTESIAN_POINT('Ctrl Pts',(-51.5418573141484,-49.6287108809966,
0.));
#138542=CARTESIAN_POINT('Ctrl Pts',(-51.5208862126315,-49.6189509577452,
0.));
#138543=CARTESIAN_POINT('Ctrl Pts',(-51.4999651347523,-49.6091889656866,
0.));
#138544=CARTESIAN_POINT('Ctrl Pts',(-51.4790941716888,-49.5994250204031,
0.));
#138545=CARTESIAN_POINT('Ctrl Pts',(-51.4582734149583,-49.5896592380654,
0.));
#138546=CARTESIAN_POINT('Ctrl Pts',(-51.4375029564197,-49.5798917354366,
0.));
#138547=CARTESIAN_POINT('Ctrl Pts',(-51.4167828882756,-49.5701226298769,
0.));
#138548=CARTESIAN_POINT('Ctrl Pts',(-51.396113303067,-49.5603520393496,
0.));
#138549=CARTESIAN_POINT('Ctrl Pts',(-51.3754942936778,-49.550580082425,
0.));
#138550=CARTESIAN_POINT('Ctrl Pts',(-51.3549259533458,-49.5408068782859,
0.));
#138551=CARTESIAN_POINT('Ctrl Pts',(-51.3344083756657,-49.5310325467332,
0.));
#138552=CARTESIAN_POINT('Ctrl Pts',(-51.313941654591,-49.5212572081908,
0.));
#138553=CARTESIAN_POINT('Ctrl Pts',(-51.2935258844289,-49.5114809837122,
0.));
#138554=CARTESIAN_POINT('Ctrl Pts',(-51.2731611598475,-49.5017039949852,
0.));
#138555=CARTESIAN_POINT('Ctrl Pts',(-51.2528475758846,-49.4919263643362,
0.));
#138556=CARTESIAN_POINT('Ctrl Pts',(-51.2325852279506,-49.4821482147356,
0.));
#138557=CARTESIAN_POINT('Ctrl Pts',(-51.2123742118287,-49.4723696698021,
0.));
#138558=CARTESIAN_POINT('Ctrl Pts',(-51.1922146236686,-49.4625908538074,
0.));
#138559=CARTESIAN_POINT('Ctrl Pts',(-51.1721065599973,-49.4528118916832,
0.));
#138560=CARTESIAN_POINT('Ctrl Pts',(-51.1520501177291,-49.4430329090287,
0.));
#138561=CARTESIAN_POINT('Ctrl Pts',(-51.1320453941702,-49.4332540321178,
0.));
#138562=CARTESIAN_POINT('Ctrl Pts',(-51.1120924870195,-49.423475387907,
0.));
#138563=CARTESIAN_POINT('Ctrl Pts',(-51.0921914943662,-49.4136971040428,
0.));
#138564=CARTESIAN_POINT('Ctrl Pts',(-51.0723425146985,-49.4039193088634,
0.));
#138565=CARTESIAN_POINT('Ctrl Pts',(-51.052545646907,-49.3941421314013,
0.));
#138566=CARTESIAN_POINT('Ctrl Pts',(-51.0328009902858,-49.3843657013852,
0.));
#138567=CARTESIAN_POINT('Ctrl Pts',(-51.0131086445272,-49.3745901492432,
0.));
#138568=CARTESIAN_POINT('Ctrl Pts',(-50.9934687097188,-49.3648156061058,
0.));
#138569=CARTESIAN_POINT('Ctrl Pts',(-50.9738812863646,-49.355042203823,
0.));
#138570=CARTESIAN_POINT('Ctrl Pts',(-50.9543464753981,-49.345270074981,
0.));
#138571=CARTESIAN_POINT('Ctrl Pts',(-50.9348643781924,-49.3354993529159,
0.));
#138572=CARTESIAN_POINT('Ctrl Pts',(-50.9154350965666,-49.3257301717335,
0.));
#138573=CARTESIAN_POINT('Ctrl Pts',(-50.8960587327848,-49.3159626663109,
0.));
#138574=CARTESIAN_POINT('Ctrl Pts',(-50.8767353895492,-49.3061969722781,
0.));
#138575=CARTESIAN_POINT('Ctrl Pts',(-50.8574651699873,-49.2964332260039,
0.));
#138576=CARTESIAN_POINT('Ctrl Pts',(-50.8382481776403,-49.2866715645838,
0.));
#138577=CARTESIAN_POINT('Ctrl Pts',(-50.819084516434,-49.2769121258164,
0.));
#138578=CARTESIAN_POINT('Ctrl Pts',(-50.7999742907131,-49.2671550482435,
0.));
#138579=CARTESIAN_POINT('Ctrl Pts',(-50.7809176052966,-49.2574004712134,
0.));
#138580=CARTESIAN_POINT('Ctrl Pts',(-50.7619145655207,-49.2476485349373,
0.));
#138581=CARTESIAN_POINT('Ctrl Pts',(-50.7429652772805,-49.2378993805471,
0.));
#138582=CARTESIAN_POINT('Ctrl Pts',(-50.7240698470679,-49.228153150155,
0.));
#138583=CARTESIAN_POINT('Ctrl Pts',(-50.7052283818922,-49.2184099867461,
0.));
#138584=CARTESIAN_POINT('Ctrl Pts',(-50.6864409891895,-49.2086700340614,
0.));
#138585=CARTESIAN_POINT('Ctrl Pts',(-50.6677077767432,-49.1989334364996,
0.));
#138586=CARTESIAN_POINT('Ctrl Pts',(-50.6490288525656,-49.189200338976,
0.));
#138587=CARTESIAN_POINT('Ctrl Pts',(-50.6304043248821,-49.1794708869099,
0.));
#138588=CARTESIAN_POINT('Ctrl Pts',(-50.6118343023958,-49.1697452265494,
0.));
#138589=CARTESIAN_POINT('Ctrl Pts',(-50.5933188945168,-49.1600235052621,
0.));
#138590=CARTESIAN_POINT('Ctrl Pts',(-50.5748582115565,-49.1503058717821,
0.));
#138591=CARTESIAN_POINT('Ctrl Pts',(-50.556452365038,-49.1405924766144,
0.));
#138592=CARTESIAN_POINT('Ctrl Pts',(-50.5381014674791,-49.1308834717615,
0.));
#138593=CARTESIAN_POINT('Ctrl Pts',(-50.5198056318089,-49.1211790099795,
0.));
#138594=CARTESIAN_POINT('Ctrl Pts',(-50.501564970874,-49.1114792441571,
0.));
#138595=CARTESIAN_POINT('Ctrl Pts',(-50.4833795969318,-49.1017843266803,
0.));
#138596=CARTESIAN_POINT('Ctrl Pts',(-50.4652496210607,-49.0920944087008,
0.));
#138597=CARTESIAN_POINT('Ctrl Pts',(-50.4471751542751,-49.0824096415371,
0.));
#138598=CARTESIAN_POINT('Ctrl Pts',(-50.4291563088547,-49.0727301783494,
0.));
#138599=CARTESIAN_POINT('Ctrl Pts',(-50.4111931994257,-49.0630561755075,
0.));
#138600=CARTESIAN_POINT('Ctrl Pts',(-50.3932859445252,-49.0533877945744,
0.));
#138601=CARTESIAN_POINT('Ctrl Pts',(-50.3754346667353,-49.0437252024832,
0.));
#138602=CARTESIAN_POINT('Ctrl Pts',(-50.3576394894108,-49.0340685673982,
0.));
#138603=CARTESIAN_POINT('Ctrl Pts',(-50.3399005337958,-49.024418055075,
0.));
#138604=CARTESIAN_POINT('Ctrl Pts',(-50.3222179165119,-49.0147738256942,
0.));
#138605=CARTESIAN_POINT('Ctrl Pts',(-50.3045917455424,-49.0051360288044,
0.));
#138606=CARTESIAN_POINT('Ctrl Pts',(-50.2870221241054,-48.9955048082081,
0.));
#138607=CARTESIAN_POINT('Ctrl Pts',(-50.2695091583511,-48.9858803116689,
0.));
#138608=CARTESIAN_POINT('Ctrl Pts',(-50.252052963548,-48.9762626987227,
0.));
#138609=CARTESIAN_POINT('Ctrl Pts',(-50.234653671541,-48.9666521500911,
0.));
#138610=CARTESIAN_POINT('Ctrl Pts',(-50.2173114358325,-48.9570488741167,
0.));
#138611=CARTESIAN_POINT('Ctrl Pts',(-50.2000264157797,-48.9474530868733,
0.));
#138612=CARTESIAN_POINT('Ctrl Pts',(-50.1827987615602,-48.9378649933055,
0.));
#138613=CARTESIAN_POINT('Ctrl Pts',(-50.1656286003997,-48.9282847698294,
0.));
#138614=CARTESIAN_POINT('Ctrl Pts',(-50.1485160184657,-48.9187125418099,
0.));
#138615=CARTESIAN_POINT('Ctrl Pts',(-50.1314610602569,-48.90914838181,0.));
#138616=CARTESIAN_POINT('Ctrl Pts',(-50.1178632067084,-48.9015035372055,
0.));
#138617=CARTESIAN_POINT('Ctrl Pts',(-50.1076907555471,-48.895773555686,
0.));
#138618=CARTESIAN_POINT('Ctrl Pts',(-50.1009206494272,-48.8919551910366,
0.));
#138619=CARTESIAN_POINT('Ctrl Pts',(-50.0975384783635,-48.8900464144686,
0.));
#138620=CARTESIAN_POINT('Ctrl Pts',(-58.722407829904,-45.8467972562798,
0.));
#138621=CARTESIAN_POINT('Ctrl Pts',(-58.722407829904,-45.8467972562798,
12.));
#138622=CARTESIAN_POINT('Ctrl Pts',(-58.7169606500268,-45.8455162977427,
0.));
#138623=CARTESIAN_POINT('Ctrl Pts',(-58.7169606500268,-45.8455162977427,
12.));
#138624=CARTESIAN_POINT('Ctrl Pts',(-58.7060702401686,-45.8429527488786,
0.));
#138625=CARTESIAN_POINT('Ctrl Pts',(-58.7060702401686,-45.8429527488786,
12.));
#138626=CARTESIAN_POINT('Ctrl Pts',(-58.68974647507,-45.8391025302132,0.));
#138627=CARTESIAN_POINT('Ctrl Pts',(-58.68974647507,-45.8391025302132,12.));
#138628=CARTESIAN_POINT('Ctrl Pts',(-58.6680051552762,-45.8339591141834,
0.));
#138629=CARTESIAN_POINT('Ctrl Pts',(-58.6680051552762,-45.8339591141834,
12.));
#138630=CARTESIAN_POINT('Ctrl Pts',(-58.6408680154016,-45.8275135264249,
0.));
#138631=CARTESIAN_POINT('Ctrl Pts',(-58.6408680154016,-45.8275135264249,
12.));
#138632=CARTESIAN_POINT('Ctrl Pts',(-58.6137704035871,-45.8210516273781,
0.));
#138633=CARTESIAN_POINT('Ctrl Pts',(-58.6137704035871,-45.8210516273781,
12.));
#138634=CARTESIAN_POINT('Ctrl Pts',(-58.5867123491018,-45.814573433072,
0.));
#138635=CARTESIAN_POINT('Ctrl Pts',(-58.5867123491018,-45.814573433072,
12.));
#138636=CARTESIAN_POINT('Ctrl Pts',(-58.5596938940195,-45.8080789725084,
0.));
#138637=CARTESIAN_POINT('Ctrl Pts',(-58.5596938940195,-45.8080789725084,
12.));
#138638=CARTESIAN_POINT('Ctrl Pts',(-58.5327150960661,-45.8015682926024,
0.));
#138639=CARTESIAN_POINT('Ctrl Pts',(-58.5327150960661,-45.8015682926024,
12.));
#138640=CARTESIAN_POINT('Ctrl Pts',(-58.5057760270184,-45.7950414569268,
0.));
#138641=CARTESIAN_POINT('Ctrl Pts',(-58.5057760270184,-45.7950414569268,
12.));
#138642=CARTESIAN_POINT('Ctrl Pts',(-58.4788767676949,-45.7884985397018,
0.));
#138643=CARTESIAN_POINT('Ctrl Pts',(-58.4788767676949,-45.7884985397018,
12.));
#138644=CARTESIAN_POINT('Ctrl Pts',(-58.4520174038764,-45.7819396211009,
0.));
#138645=CARTESIAN_POINT('Ctrl Pts',(-58.4520174038764,-45.7819396211009,
12.));
#138646=CARTESIAN_POINT('Ctrl Pts',(-58.425198021955,-45.7753647821513,
0.));
#138647=CARTESIAN_POINT('Ctrl Pts',(-58.425198021955,-45.7753647821513,
12.));
#138648=CARTESIAN_POINT('Ctrl Pts',(-58.3984187044245,-45.7687740994956,
0.));
#138649=CARTESIAN_POINT('Ctrl Pts',(-58.3984187044245,-45.7687740994956,
12.));
#138650=CARTESIAN_POINT('Ctrl Pts',(-58.3716795262353,-45.7621676411434,
0.));
#138651=CARTESIAN_POINT('Ctrl Pts',(-58.3716795262353,-45.7621676411434,
12.));
#138652=CARTESIAN_POINT('Ctrl Pts',(-58.3449805573423,-45.755545469402,
0.));
#138653=CARTESIAN_POINT('Ctrl Pts',(-58.3449805573423,-45.755545469402,
12.));
#138654=CARTESIAN_POINT('Ctrl Pts',(-58.3183218645317,-45.7489076429763,
0.));
#138655=CARTESIAN_POINT('Ctrl Pts',(-58.3183218645317,-45.7489076429763,
12.));
#138656=CARTESIAN_POINT('Ctrl Pts',(-58.291703513584,-45.742254219463,0.));
#138657=CARTESIAN_POINT('Ctrl Pts',(-58.291703513584,-45.742254219463,12.));
#138658=CARTESIAN_POINT('Ctrl Pts',(-58.2651255711453,-45.7355852575106,
0.));
#138659=CARTESIAN_POINT('Ctrl Pts',(-58.2651255711453,-45.7355852575106,
12.));
#138660=CARTESIAN_POINT('Ctrl Pts',(-58.2385881070913,-45.7289008195578,
0.));
#138661=CARTESIAN_POINT('Ctrl Pts',(-58.2385881070913,-45.7289008195578,
12.));
#138662=CARTESIAN_POINT('Ctrl Pts',(-58.2120911942772,-45.7222009715397,
0.));
#138663=CARTESIAN_POINT('Ctrl Pts',(-58.2120911942772,-45.7222009715397,
12.));
#138664=CARTESIAN_POINT('Ctrl Pts',(-58.185634907469,-45.7154857816483,
0.));
#138665=CARTESIAN_POINT('Ctrl Pts',(-58.185634907469,-45.7154857816483,
12.));
#138666=CARTESIAN_POINT('Ctrl Pts',(-58.1592193225137,-45.7087553193771,
0.));
#138667=CARTESIAN_POINT('Ctrl Pts',(-58.1592193225137,-45.7087553193771,
12.));
#138668=CARTESIAN_POINT('Ctrl Pts',(-58.1328445154676,-45.702009654518,
0.));
#138669=CARTESIAN_POINT('Ctrl Pts',(-58.1328445154676,-45.702009654518,
12.));
#138670=CARTESIAN_POINT('Ctrl Pts',(-58.1065105615907,-45.695248856015,
0.));
#138671=CARTESIAN_POINT('Ctrl Pts',(-58.1065105615907,-45.695248856015,
12.));
#138672=CARTESIAN_POINT('Ctrl Pts',(-58.0802175348966,-45.6884729914485,
0.));
#138673=CARTESIAN_POINT('Ctrl Pts',(-58.0802175348966,-45.6884729914485,
12.));
#138674=CARTESIAN_POINT('Ctrl Pts',(-58.0539655087117,-45.6816821276678,
0.));
#138675=CARTESIAN_POINT('Ctrl Pts',(-58.0539655087117,-45.6816821276678,
12.));
#138676=CARTESIAN_POINT('Ctrl Pts',(-58.0277545560012,-45.6748763311643,
0.));
#138677=CARTESIAN_POINT('Ctrl Pts',(-58.0277545560012,-45.6748763311643,
12.));
#138678=CARTESIAN_POINT('Ctrl Pts',(-58.0015847497837,-45.6680556685493,
0.));
#138679=CARTESIAN_POINT('Ctrl Pts',(-58.0015847497837,-45.6680556685493,
12.));
#138680=CARTESIAN_POINT('Ctrl Pts',(-57.9754561635061,-45.661220206992,
0.));
#138681=CARTESIAN_POINT('Ctrl Pts',(-57.9754561635061,-45.661220206992,
12.));
#138682=CARTESIAN_POINT('Ctrl Pts',(-57.9493688714237,-45.6543700146679,
0.));
#138683=CARTESIAN_POINT('Ctrl Pts',(-57.9493688714237,-45.6543700146679,
12.));
#138684=CARTESIAN_POINT('Ctrl Pts',(-57.9233229484311,-45.6475051605535,
0.));
#138685=CARTESIAN_POINT('Ctrl Pts',(-57.9233229484311,-45.6475051605535,
12.));
#138686=CARTESIAN_POINT('Ctrl Pts',(-57.8973184699034,-45.6406257142381,
0.));
#138687=CARTESIAN_POINT('Ctrl Pts',(-57.8973184699034,-45.6406257142381,
12.));
#138688=CARTESIAN_POINT('Ctrl Pts',(-57.8713555115232,-45.6337317457252,
0.));
#138689=CARTESIAN_POINT('Ctrl Pts',(-57.8713555115232,-45.6337317457252,
12.));
#138690=CARTESIAN_POINT('Ctrl Pts',(-57.8454341491238,-45.6268233252544,
0.));
#138691=CARTESIAN_POINT('Ctrl Pts',(-57.8454341491238,-45.6268233252544,
12.));
#138692=CARTESIAN_POINT('Ctrl Pts',(-57.8195544584845,-45.6199005230783,
0.));
#138693=CARTESIAN_POINT('Ctrl Pts',(-57.8195544584845,-45.6199005230783,
12.));
#138694=CARTESIAN_POINT('Ctrl Pts',(-57.7937165153387,-45.6129634094683,
0.));
#138695=CARTESIAN_POINT('Ctrl Pts',(-57.7937165153387,-45.6129634094683,
12.));
#138696=CARTESIAN_POINT('Ctrl Pts',(-57.7679203954742,-45.6060120548205,
0.));
#138697=CARTESIAN_POINT('Ctrl Pts',(-57.7679203954742,-45.6060120548205,
12.));
#138698=CARTESIAN_POINT('Ctrl Pts',(-57.7421661748026,-45.5990465297343,
0.));
#138699=CARTESIAN_POINT('Ctrl Pts',(-57.7421661748026,-45.5990465297343,
12.));
#138700=CARTESIAN_POINT('Ctrl Pts',(-57.7164539294314,-45.5920669050986,
0.));
#138701=CARTESIAN_POINT('Ctrl Pts',(-57.7164539294314,-45.5920669050986,
12.));
#138702=CARTESIAN_POINT('Ctrl Pts',(-57.6907837357418,-45.5850732521895,
0.));
#138703=CARTESIAN_POINT('Ctrl Pts',(-57.6907837357418,-45.5850732521895,
12.));
#138704=CARTESIAN_POINT('Ctrl Pts',(-57.6651556704237,-45.5780656427163,
0.));
#138705=CARTESIAN_POINT('Ctrl Pts',(-57.6651556704237,-45.5780656427163,
12.));
#138706=CARTESIAN_POINT('Ctrl Pts',(-57.6395698104404,-45.5710441487674,
0.));
#138707=CARTESIAN_POINT('Ctrl Pts',(-57.6395698104404,-45.5710441487674,
12.));
#138708=CARTESIAN_POINT('Ctrl Pts',(-57.614026233004,-45.5640088427813,
0.));
#138709=CARTESIAN_POINT('Ctrl Pts',(-57.614026233004,-45.5640088427813,
12.));
#138710=CARTESIAN_POINT('Ctrl Pts',(-57.5885250155433,-45.5569597975096,
0.));
#138711=CARTESIAN_POINT('Ctrl Pts',(-57.5885250155433,-45.5569597975096,
12.));
#138712=CARTESIAN_POINT('Ctrl Pts',(-57.563066235668,-45.5498970859834,
0.));
#138713=CARTESIAN_POINT('Ctrl Pts',(-57.563066235668,-45.5498970859834,
12.));
#138714=CARTESIAN_POINT('Ctrl Pts',(-57.537649971135,-45.542820781484,0.));
#138715=CARTESIAN_POINT('Ctrl Pts',(-57.537649971135,-45.542820781484,12.));
#138716=CARTESIAN_POINT('Ctrl Pts',(-57.5122762998745,-45.5357309575611,
0.));
#138717=CARTESIAN_POINT('Ctrl Pts',(-57.5122762998745,-45.5357309575611,
12.));
#138718=CARTESIAN_POINT('Ctrl Pts',(-57.4869453000063,-45.5286276880484,
0.));
#138719=CARTESIAN_POINT('Ctrl Pts',(-57.4869453000063,-45.5286276880484,
12.));
#138720=CARTESIAN_POINT('Ctrl Pts',(-57.4616570498568,-45.5215110470825,
0.));
#138721=CARTESIAN_POINT('Ctrl Pts',(-57.4616570498568,-45.5215110470825,
12.));
#138722=CARTESIAN_POINT('Ctrl Pts',(-57.4364116279702,-45.5143811091205,
0.));
#138723=CARTESIAN_POINT('Ctrl Pts',(-57.4364116279702,-45.5143811091205,
12.));
#138724=CARTESIAN_POINT('Ctrl Pts',(-57.4112091131183,-45.5072379489631,
0.));
#138725=CARTESIAN_POINT('Ctrl Pts',(-57.4112091131183,-45.5072379489631,
12.));
#138726=CARTESIAN_POINT('Ctrl Pts',(-57.3860495843033,-45.5000816417509,
0.));
#138727=CARTESIAN_POINT('Ctrl Pts',(-57.3860495843033,-45.5000816417509,
12.));
#138728=CARTESIAN_POINT('Ctrl Pts',(-57.3609331207574,-45.4929122629572,
0.));
#138729=CARTESIAN_POINT('Ctrl Pts',(-57.3609331207574,-45.4929122629572,
12.));
#138730=CARTESIAN_POINT('Ctrl Pts',(-57.3358598019389,-45.4857298883824,
0.));
#138731=CARTESIAN_POINT('Ctrl Pts',(-57.3358598019389,-45.4857298883824,
12.));
#138732=CARTESIAN_POINT('Ctrl Pts',(-57.3108297075265,-45.4785345941507,
0.));
#138733=CARTESIAN_POINT('Ctrl Pts',(-57.3108297075265,-45.4785345941507,
12.));
#138734=CARTESIAN_POINT('Ctrl Pts',(-57.2858429174062,-45.4713264567063,
0.));
#138735=CARTESIAN_POINT('Ctrl Pts',(-57.2858429174062,-45.4713264567063,
12.));
#138736=CARTESIAN_POINT('Ctrl Pts',(-57.2608995116733,-45.4641055528141,
0.));
#138737=CARTESIAN_POINT('Ctrl Pts',(-57.2608995116733,-45.4641055528141,
12.));
#138738=CARTESIAN_POINT('Ctrl Pts',(-57.2359995706447,-45.4568719595641,
0.));
#138739=CARTESIAN_POINT('Ctrl Pts',(-57.2359995706447,-45.4568719595641,
12.));
#138740=CARTESIAN_POINT('Ctrl Pts',(-57.2111431748631,-45.4496257543759,
0.));
#138741=CARTESIAN_POINT('Ctrl Pts',(-57.2111431748631,-45.4496257543759,
12.));
#138742=CARTESIAN_POINT('Ctrl Pts',(-57.186330405101,-45.4423670150034,
0.));
#138743=CARTESIAN_POINT('Ctrl Pts',(-57.186330405101,-45.4423670150034,
12.));
#138744=CARTESIAN_POINT('Ctrl Pts',(-57.1615613423584,-45.4350958195433,
0.));
#138745=CARTESIAN_POINT('Ctrl Pts',(-57.1615613423584,-45.4350958195433,
12.));
#138746=CARTESIAN_POINT('Ctrl Pts',(-57.136836067863,-45.4278122464389,
0.));
#138747=CARTESIAN_POINT('Ctrl Pts',(-57.136836067863,-45.4278122464389,
12.));
#138748=CARTESIAN_POINT('Ctrl Pts',(-57.112154663078,-45.4205163744781,
0.));
#138749=CARTESIAN_POINT('Ctrl Pts',(-57.112154663078,-45.4205163744781,
12.));
#138750=CARTESIAN_POINT('Ctrl Pts',(-57.0875172097051,-45.4132082827948,
0.));
#138751=CARTESIAN_POINT('Ctrl Pts',(-57.0875172097051,-45.4132082827948,
12.));
#138752=CARTESIAN_POINT('Ctrl Pts',(-57.0629237896848,-45.4058880508693,
0.));
#138753=CARTESIAN_POINT('Ctrl Pts',(-57.0629237896848,-45.4058880508693,
12.));
#138754=CARTESIAN_POINT('Ctrl Pts',(-57.0383744851913,-45.3985557585311,
0.));
#138755=CARTESIAN_POINT('Ctrl Pts',(-57.0383744851913,-45.3985557585311,
12.));
#138756=CARTESIAN_POINT('Ctrl Pts',(-57.0138693786278,-45.3912114859616,
0.));
#138757=CARTESIAN_POINT('Ctrl Pts',(-57.0138693786278,-45.3912114859616,
12.));
#138758=CARTESIAN_POINT('Ctrl Pts',(-56.9894085526373,-45.3838553136948,
0.));
#138759=CARTESIAN_POINT('Ctrl Pts',(-56.9894085526373,-45.3838553136948,
12.));
#138760=CARTESIAN_POINT('Ctrl Pts',(-56.9649920901073,-45.3764873226196,
0.));
#138761=CARTESIAN_POINT('Ctrl Pts',(-56.9649920901073,-45.3764873226196,
12.));
#138762=CARTESIAN_POINT('Ctrl Pts',(-56.9406200741714,-45.3691075939826,
0.));
#138763=CARTESIAN_POINT('Ctrl Pts',(-56.9406200741714,-45.3691075939826,
12.));
#138764=CARTESIAN_POINT('Ctrl Pts',(-56.9162925882085,-45.3617162093922,
0.));
#138765=CARTESIAN_POINT('Ctrl Pts',(-56.9162925882085,-45.3617162093922,
12.));
#138766=CARTESIAN_POINT('Ctrl Pts',(-56.8920097158377,-45.3543132508238,
0.));
#138767=CARTESIAN_POINT('Ctrl Pts',(-56.8920097158377,-45.3543132508238,
12.));
#138768=CARTESIAN_POINT('Ctrl Pts',(-56.8677715409268,-45.3468988006203,
0.));
#138769=CARTESIAN_POINT('Ctrl Pts',(-56.8677715409268,-45.3468988006203,
12.));
#138770=CARTESIAN_POINT('Ctrl Pts',(-56.8435781475981,-45.3394729414931,
0.));
#138771=CARTESIAN_POINT('Ctrl Pts',(-56.8435781475981,-45.3394729414931,
12.));
#138772=CARTESIAN_POINT('Ctrl Pts',(-56.8194296202291,-45.332035756524,
0.));
#138773=CARTESIAN_POINT('Ctrl Pts',(-56.8194296202291,-45.332035756524,
12.));
#138774=CARTESIAN_POINT('Ctrl Pts',(-56.7953260434524,-45.3245873291684,
0.));
#138775=CARTESIAN_POINT('Ctrl Pts',(-56.7953260434524,-45.3245873291684,
12.));
#138776=CARTESIAN_POINT('Ctrl Pts',(-56.7712675021491,-45.31712774326,0.));
#138777=CARTESIAN_POINT('Ctrl Pts',(-56.7712675021491,-45.31712774326,12.));
#138778=CARTESIAN_POINT('Ctrl Pts',(-56.7472540814554,-45.3096570830117,
0.));
#138779=CARTESIAN_POINT('Ctrl Pts',(-56.7472540814554,-45.3096570830117,
12.));
#138780=CARTESIAN_POINT('Ctrl Pts',(-56.7232858667709,-45.3021754330178,
0.));
#138781=CARTESIAN_POINT('Ctrl Pts',(-56.7232858667709,-45.3021754330178,
12.));
#138782=CARTESIAN_POINT('Ctrl Pts',(-56.69936294376,-45.2946828782559,0.));
#138783=CARTESIAN_POINT('Ctrl Pts',(-56.69936294376,-45.2946828782559,12.));
#138784=CARTESIAN_POINT('Ctrl Pts',(-56.6754853983528,-45.2871795040906,
0.));
#138785=CARTESIAN_POINT('Ctrl Pts',(-56.6754853983528,-45.2871795040906,
12.));
#138786=CARTESIAN_POINT('Ctrl Pts',(-56.6516533167384,-45.2796653962785,
0.));
#138787=CARTESIAN_POINT('Ctrl Pts',(-56.6516533167384,-45.2796653962785,
12.));
#138788=CARTESIAN_POINT('Ctrl Pts',(-56.6278667853702,-45.2721406409695,
0.));
#138789=CARTESIAN_POINT('Ctrl Pts',(-56.6278667853702,-45.2721406409695,
12.));
#138790=CARTESIAN_POINT('Ctrl Pts',(-56.6041258909741,-45.2646053247087,
0.));
#138791=CARTESIAN_POINT('Ctrl Pts',(-56.6041258909741,-45.2646053247087,
12.));
#138792=CARTESIAN_POINT('Ctrl Pts',(-56.5804307205505,-45.257059534438,
0.));
#138793=CARTESIAN_POINT('Ctrl Pts',(-56.5804307205505,-45.257059534438,
12.));
#138794=CARTESIAN_POINT('Ctrl Pts',(-56.5567813613756,-45.2495033575,0.));
#138795=CARTESIAN_POINT('Ctrl Pts',(-56.5567813613756,-45.2495033575,12.));
#138796=CARTESIAN_POINT('Ctrl Pts',(-56.5331779009958,-45.2419368816428,
0.));
#138797=CARTESIAN_POINT('Ctrl Pts',(-56.5331779009958,-45.2419368816428,
12.));
#138798=CARTESIAN_POINT('Ctrl Pts',(-56.5096204272306,-45.2343601950227,
0.));
#138799=CARTESIAN_POINT('Ctrl Pts',(-56.5096204272306,-45.2343601950227,
12.));
#138800=CARTESIAN_POINT('Ctrl Pts',(-56.4861090281823,-45.2267733862049,
0.));
#138801=CARTESIAN_POINT('Ctrl Pts',(-56.4861090281823,-45.2267733862049,
12.));
#138802=CARTESIAN_POINT('Ctrl Pts',(-56.4626437922386,-45.2191765441666,
0.));
#138803=CARTESIAN_POINT('Ctrl Pts',(-56.4626437922386,-45.2191765441666,
12.));
#138804=CARTESIAN_POINT('Ctrl Pts',(-56.4392248080732,-45.2115697583,0.));
#138805=CARTESIAN_POINT('Ctrl Pts',(-56.4392248080732,-45.2115697583,12.));
#138806=CARTESIAN_POINT('Ctrl Pts',(-56.4158521646411,-45.2039531184171,
0.));
#138807=CARTESIAN_POINT('Ctrl Pts',(-56.4158521646411,-45.2039531184171,
12.));
#138808=CARTESIAN_POINT('Ctrl Pts',(-56.3925259511806,-45.1963267147529,
0.));
#138809=CARTESIAN_POINT('Ctrl Pts',(-56.3925259511806,-45.1963267147529,
12.));
#138810=CARTESIAN_POINT('Ctrl Pts',(-56.3692462572231,-45.1886906379667,
0.));
#138811=CARTESIAN_POINT('Ctrl Pts',(-56.3692462572231,-45.1886906379667,
12.));
#138812=CARTESIAN_POINT('Ctrl Pts',(-56.3460131725964,-45.1810449791453,
0.));
#138813=CARTESIAN_POINT('Ctrl Pts',(-56.3460131725964,-45.1810449791453,
12.));
#138814=CARTESIAN_POINT('Ctrl Pts',(-56.3228267874264,-45.173389829806,
0.));
#138815=CARTESIAN_POINT('Ctrl Pts',(-56.3228267874264,-45.173389829806,
12.));
#138816=CARTESIAN_POINT('Ctrl Pts',(-56.2996871921316,-45.1657252819013,
0.));
#138817=CARTESIAN_POINT('Ctrl Pts',(-56.2996871921316,-45.1657252819013,
12.));
#138818=CARTESIAN_POINT('Ctrl Pts',(-56.2765944774245,-45.1580514278223,
0.));
#138819=CARTESIAN_POINT('Ctrl Pts',(-56.2765944774245,-45.1580514278223,
12.));
#138820=CARTESIAN_POINT('Ctrl Pts',(-56.2535487343221,-45.1503683604005,
0.));
#138821=CARTESIAN_POINT('Ctrl Pts',(-56.2535487343221,-45.1503683604005,
12.));
#138822=CARTESIAN_POINT('Ctrl Pts',(-56.230550054149,-45.1426761729105,
0.));
#138823=CARTESIAN_POINT('Ctrl Pts',(-56.230550054149,-45.1426761729105,
12.));
#138824=CARTESIAN_POINT('Ctrl Pts',(-56.2075985285393,-45.1349749590737,
0.));
#138825=CARTESIAN_POINT('Ctrl Pts',(-56.2075985285393,-45.1349749590737,
12.));
#138826=CARTESIAN_POINT('Ctrl Pts',(-56.1846942494325,-45.127264813063,
0.));
#138827=CARTESIAN_POINT('Ctrl Pts',(-56.1846942494325,-45.127264813063,
12.));
#138828=CARTESIAN_POINT('Ctrl Pts',(-56.1618373090732,-45.1195458295062,
0.));
#138829=CARTESIAN_POINT('Ctrl Pts',(-56.1618373090732,-45.1195458295062,
12.));
#138830=CARTESIAN_POINT('Ctrl Pts',(-56.1390278000226,-45.1118181034888,
0.));
#138831=CARTESIAN_POINT('Ctrl Pts',(-56.1390278000226,-45.1118181034888,
12.));
#138832=CARTESIAN_POINT('Ctrl Pts',(-56.116265815162,-45.1040817305561,
0.));
#138833=CARTESIAN_POINT('Ctrl Pts',(-56.116265815162,-45.1040817305561,
12.));
#138834=CARTESIAN_POINT('Ctrl Pts',(-56.0935514476945,-45.0963368067177,
0.));
#138835=CARTESIAN_POINT('Ctrl Pts',(-56.0935514476945,-45.0963368067177,
12.));
#138836=CARTESIAN_POINT('Ctrl Pts',(-56.0708847911416,-45.0885834284517,
0.));
#138837=CARTESIAN_POINT('Ctrl Pts',(-56.0708847911416,-45.0885834284517,
12.));
#138838=CARTESIAN_POINT('Ctrl Pts',(-56.048265939342,-45.0808216927089,
0.));
#138839=CARTESIAN_POINT('Ctrl Pts',(-56.048265939342,-45.0808216927089,
12.));
#138840=CARTESIAN_POINT('Ctrl Pts',(-56.0256949864639,-45.0730516969148,
0.));
#138841=CARTESIAN_POINT('Ctrl Pts',(-56.0256949864639,-45.0730516969148,
12.));
#138842=CARTESIAN_POINT('Ctrl Pts',(-56.003172027008,-45.0652735389733,
0.));
#138843=CARTESIAN_POINT('Ctrl Pts',(-56.003172027008,-45.0652735389733,
12.));
#138844=CARTESIAN_POINT('Ctrl Pts',(-55.9806971558097,-45.0574873172694,
0.));
#138845=CARTESIAN_POINT('Ctrl Pts',(-55.9806971558097,-45.0574873172694,
12.));
#138846=CARTESIAN_POINT('Ctrl Pts',(-55.9582704680356,-45.0496931306755,
0.));
#138847=CARTESIAN_POINT('Ctrl Pts',(-55.9582704680356,-45.0496931306755,
12.));
#138848=CARTESIAN_POINT('Ctrl Pts',(-55.9358920591837,-45.041891078555,
0.));
#138849=CARTESIAN_POINT('Ctrl Pts',(-55.9358920591837,-45.041891078555,
12.));
#138850=CARTESIAN_POINT('Ctrl Pts',(-55.9135620250954,-45.0340812607657,
0.));
#138851=CARTESIAN_POINT('Ctrl Pts',(-55.9135620250954,-45.0340812607657,
12.));
#138852=CARTESIAN_POINT('Ctrl Pts',(-55.8912804619577,-45.0262637776614,
0.));
#138853=CARTESIAN_POINT('Ctrl Pts',(-55.8912804619577,-45.0262637776614,
12.));
#138854=CARTESIAN_POINT('Ctrl Pts',(-55.8690474663065,-45.0184387300973,
0.));
#138855=CARTESIAN_POINT('Ctrl Pts',(-55.8690474663065,-45.0184387300973,
12.));
#138856=CARTESIAN_POINT('Ctrl Pts',(-55.8468631350218,-45.0106062194342,
0.));
#138857=CARTESIAN_POINT('Ctrl Pts',(-55.8468631350218,-45.0106062194342,
12.));
#138858=CARTESIAN_POINT('Ctrl Pts',(-55.8247275653289,-45.0027663475433,
0.));
#138859=CARTESIAN_POINT('Ctrl Pts',(-55.8247275653289,-45.0027663475433,
12.));
#138860=CARTESIAN_POINT('Ctrl Pts',(-55.8026408548105,-44.9949192168093,
0.));
#138861=CARTESIAN_POINT('Ctrl Pts',(-55.8026408548105,-44.9949192168093,
12.));
#138862=CARTESIAN_POINT('Ctrl Pts',(-55.7806031014106,-44.9870649301342,
0.));
#138863=CARTESIAN_POINT('Ctrl Pts',(-55.7806031014106,-44.9870649301342,
12.));
#138864=CARTESIAN_POINT('Ctrl Pts',(-55.7586144034367,-44.9792035909413,
0.));
#138865=CARTESIAN_POINT('Ctrl Pts',(-55.7586144034367,-44.9792035909413,
12.));
#138866=CARTESIAN_POINT('Ctrl Pts',(-55.7366748595552,-44.9713353031804,
0.));
#138867=CARTESIAN_POINT('Ctrl Pts',(-55.7366748595552,-44.9713353031804,
12.));
#138868=CARTESIAN_POINT('Ctrl Pts',(-55.714784568793,-44.9634601713321,
0.));
#138869=CARTESIAN_POINT('Ctrl Pts',(-55.714784568793,-44.9634601713321,
12.));
#138870=CARTESIAN_POINT('Ctrl Pts',(-55.6929436305489,-44.9555783004106,
0.));
#138871=CARTESIAN_POINT('Ctrl Pts',(-55.6929436305489,-44.9555783004106,
12.));
#138872=CARTESIAN_POINT('Ctrl Pts',(-55.6711521445979,-44.9476897959684,
0.));
#138873=CARTESIAN_POINT('Ctrl Pts',(-55.6711521445979,-44.9476897959684,
12.));
#138874=CARTESIAN_POINT('Ctrl Pts',(-55.6494102110935,-44.9397947641006,
0.));
#138875=CARTESIAN_POINT('Ctrl Pts',(-55.6494102110935,-44.9397947641006,
12.));
#138876=CARTESIAN_POINT('Ctrl Pts',(-55.6277179305633,-44.9318933114506,
0.));
#138877=CARTESIAN_POINT('Ctrl Pts',(-55.6277179305633,-44.9318933114506,
12.));
#138878=CARTESIAN_POINT('Ctrl Pts',(-55.6060754039121,-44.9239855452144,
0.));
#138879=CARTESIAN_POINT('Ctrl Pts',(-55.6060754039121,-44.9239855452144,
12.));
#138880=CARTESIAN_POINT('Ctrl Pts',(-55.5844827324338,-44.9160715731443,
0.));
#138881=CARTESIAN_POINT('Ctrl Pts',(-55.5844827324338,-44.9160715731443,
12.));
#138882=CARTESIAN_POINT('Ctrl Pts',(-55.5629400178142,-44.908151503553,
0.));
#138883=CARTESIAN_POINT('Ctrl Pts',(-55.5629400178142,-44.908151503553,
12.));
#138884=CARTESIAN_POINT('Ctrl Pts',(-55.541447362134,-44.9002254453183,
0.));
#138885=CARTESIAN_POINT('Ctrl Pts',(-55.541447362134,-44.9002254453183,
12.));
#138886=CARTESIAN_POINT('Ctrl Pts',(-55.5200048678629,-44.8922935078889,
0.));
#138887=CARTESIAN_POINT('Ctrl Pts',(-55.5200048678629,-44.8922935078889,
12.));
#138888=CARTESIAN_POINT('Ctrl Pts',(-55.4986126378656,-44.8843558012886,
0.));
#138889=CARTESIAN_POINT('Ctrl Pts',(-55.4986126378656,-44.8843558012886,
12.));
#138890=CARTESIAN_POINT('Ctrl Pts',(-55.4772707754126,-44.8764124361206,
0.));
#138891=CARTESIAN_POINT('Ctrl Pts',(-55.4772707754126,-44.8764124361206,
12.));
#138892=CARTESIAN_POINT('Ctrl Pts',(-55.4559793841836,-44.8684635235725,
0.));
#138893=CARTESIAN_POINT('Ctrl Pts',(-55.4559793841836,-44.8684635235725,
12.));
#138894=CARTESIAN_POINT('Ctrl Pts',(-55.4347385682704,-44.8605091754214,
0.));
#138895=CARTESIAN_POINT('Ctrl Pts',(-55.4347385682704,-44.8605091754214,
12.));
#138896=CARTESIAN_POINT('Ctrl Pts',(-55.4135484321718,-44.8525495040408,
0.));
#138897=CARTESIAN_POINT('Ctrl Pts',(-55.4135484321718,-44.8525495040408,
12.));
#138898=CARTESIAN_POINT('Ctrl Pts',(-55.3924090808014,-44.8445846224044,
0.));
#138899=CARTESIAN_POINT('Ctrl Pts',(-55.3924090808014,-44.8445846224044,
12.));
#138900=CARTESIAN_POINT('Ctrl Pts',(-55.3713206194967,-44.8366146440901,
0.));
#138901=CARTESIAN_POINT('Ctrl Pts',(-55.3713206194967,-44.8366146440901,
12.));
#138902=CARTESIAN_POINT('Ctrl Pts',(-55.3502831540228,-44.8286396832847,
0.));
#138903=CARTESIAN_POINT('Ctrl Pts',(-55.3502831540228,-44.8286396832847,
12.));
#138904=CARTESIAN_POINT('Ctrl Pts',(-55.3292967905725,-44.8206598547887,
0.));
#138905=CARTESIAN_POINT('Ctrl Pts',(-55.3292967905725,-44.8206598547887,
12.));
#138906=CARTESIAN_POINT('Ctrl Pts',(-55.3083616357605,-44.8126752740208,
0.));
#138907=CARTESIAN_POINT('Ctrl Pts',(-55.3083616357605,-44.8126752740208,
12.));
#138908=CARTESIAN_POINT('Ctrl Pts',(-55.287477796635,-44.8046860570244,
0.));
#138909=CARTESIAN_POINT('Ctrl Pts',(-55.287477796635,-44.8046860570244,
12.));
#138910=CARTESIAN_POINT('Ctrl Pts',(-55.2666453806883,-44.796692320474,
0.));
#138911=CARTESIAN_POINT('Ctrl Pts',(-55.2666453806883,-44.796692320474,
12.));
#138912=CARTESIAN_POINT('Ctrl Pts',(-55.2458644958617,-44.7886941816823,
0.));
#138913=CARTESIAN_POINT('Ctrl Pts',(-55.2458644958617,-44.7886941816823,
12.));
#138914=CARTESIAN_POINT('Ctrl Pts',(-55.2251352505474,-44.7806917586077,
0.));
#138915=CARTESIAN_POINT('Ctrl Pts',(-55.2251352505474,-44.7806917586077,
12.));
#138916=CARTESIAN_POINT('Ctrl Pts',(-55.2044577535865,-44.7726851698618,
0.));
#138917=CARTESIAN_POINT('Ctrl Pts',(-55.2044577535865,-44.7726851698618,
12.));
#138918=CARTESIAN_POINT('Ctrl Pts',(-55.1838321142777,-44.7646745347108,
0.));
#138919=CARTESIAN_POINT('Ctrl Pts',(-55.1838321142777,-44.7646745347108,
12.));
#138920=CARTESIAN_POINT('Ctrl Pts',(-55.1632584423813,-44.7566599730771,
0.));
#138921=CARTESIAN_POINT('Ctrl Pts',(-55.1632584423813,-44.7566599730771,
12.));
#138922=CARTESIAN_POINT('Ctrl Pts',(-55.1427368481201,-44.7486416055419,
0.));
#138923=CARTESIAN_POINT('Ctrl Pts',(-55.1427368481201,-44.7486416055419,
12.));
#138924=CARTESIAN_POINT('Ctrl Pts',(-55.1222674421747,-44.7406195533482,
0.));
#138925=CARTESIAN_POINT('Ctrl Pts',(-55.1222674421747,-44.7406195533482,
12.));
#138926=CARTESIAN_POINT('Ctrl Pts',(-55.1018503356806,-44.7325939384042,
0.));
#138927=CARTESIAN_POINT('Ctrl Pts',(-55.1018503356806,-44.7325939384042,
12.));
#138928=CARTESIAN_POINT('Ctrl Pts',(-55.0814856402507,-44.7245648832988,
0.));
#138929=CARTESIAN_POINT('Ctrl Pts',(-55.0814856402507,-44.7245648832988,
12.));
#138930=CARTESIAN_POINT('Ctrl Pts',(-55.0611734679902,-44.7165325113165,
0.));
#138931=CARTESIAN_POINT('Ctrl Pts',(-55.0611734679902,-44.7165325113165,
12.));
#138932=CARTESIAN_POINT('Ctrl Pts',(-55.0409139315074,-44.7084969464509,
0.));
#138933=CARTESIAN_POINT('Ctrl Pts',(-55.0409139315074,-44.7084969464509,
12.));
#138934=CARTESIAN_POINT('Ctrl Pts',(-55.020707143922,-44.7004583134235,
0.));
#138935=CARTESIAN_POINT('Ctrl Pts',(-55.020707143922,-44.7004583134235,
12.));
#138936=CARTESIAN_POINT('Ctrl Pts',(-55.0005532188644,-44.6924167376851,
0.));
#138937=CARTESIAN_POINT('Ctrl Pts',(-55.0005532188644,-44.6924167376851,
12.));
#138938=CARTESIAN_POINT('Ctrl Pts',(-54.9804522704668,-44.6843723453985,
0.));
#138939=CARTESIAN_POINT('Ctrl Pts',(-54.9804522704668,-44.6843723453985,
12.));
#138940=CARTESIAN_POINT('Ctrl Pts',(-54.9604044133497,-44.6763252634255,
0.));
#138941=CARTESIAN_POINT('Ctrl Pts',(-54.9604044133497,-44.6763252634255,
12.));
#138942=CARTESIAN_POINT('Ctrl Pts',(-54.9404097626088,-44.6682756193155,
0.));
#138943=CARTESIAN_POINT('Ctrl Pts',(-54.9404097626088,-44.6682756193155,
12.));
#138944=CARTESIAN_POINT('Ctrl Pts',(-54.9204684337845,-44.6602235412853,
0.));
#138945=CARTESIAN_POINT('Ctrl Pts',(-54.9204684337845,-44.6602235412853,
12.));
#138946=CARTESIAN_POINT('Ctrl Pts',(-54.9005805428991,-44.6521691582551,
0.));
#138947=CARTESIAN_POINT('Ctrl Pts',(-54.9005805428991,-44.6521691582551,
12.));
#138948=CARTESIAN_POINT('Ctrl Pts',(-54.8807462065177,-44.6441125999074,
0.));
#138949=CARTESIAN_POINT('Ctrl Pts',(-54.8807462065177,-44.6441125999074,
12.));
#138950=CARTESIAN_POINT('Ctrl Pts',(-54.860965541796,-44.6360539967392,
0.));
#138951=CARTESIAN_POINT('Ctrl Pts',(-54.860965541796,-44.6360539967392,
12.));
#138952=CARTESIAN_POINT('Ctrl Pts',(-54.8412386665264,-44.6279934801159,
0.));
#138953=CARTESIAN_POINT('Ctrl Pts',(-54.8412386665264,-44.6279934801159,
12.));
#138954=CARTESIAN_POINT('Ctrl Pts',(-54.8215656991817,-44.6199311823276,
0.));
#138955=CARTESIAN_POINT('Ctrl Pts',(-54.8215656991817,-44.6199311823276,
12.));
#138956=CARTESIAN_POINT('Ctrl Pts',(-54.8019467588258,-44.6118672364889,
0.));
#138957=CARTESIAN_POINT('Ctrl Pts',(-54.8019467588258,-44.6118672364889,
12.));
#138958=CARTESIAN_POINT('Ctrl Pts',(-54.7823819650137,-44.60380177643,0.));
#138959=CARTESIAN_POINT('Ctrl Pts',(-54.7823819650137,-44.60380177643,12.));
#138960=CARTESIAN_POINT('Ctrl Pts',(-54.7628714377042,-44.5957349366062,
0.));
#138961=CARTESIAN_POINT('Ctrl Pts',(-54.7628714377042,-44.5957349366062,
12.));
#138962=CARTESIAN_POINT('Ctrl Pts',(-54.7434152971285,-44.5876668519676,
0.));
#138963=CARTESIAN_POINT('Ctrl Pts',(-54.7434152971285,-44.5876668519676,
12.));
#138964=CARTESIAN_POINT('Ctrl Pts',(-54.7240136637744,-44.5795976579476,
0.));
#138965=CARTESIAN_POINT('Ctrl Pts',(-54.7240136637744,-44.5795976579476,
12.));
#138966=CARTESIAN_POINT('Ctrl Pts',(-54.7046666586777,-44.5715274907637,
0.));
#138967=CARTESIAN_POINT('Ctrl Pts',(-54.7046666586777,-44.5715274907637,
12.));
#138968=CARTESIAN_POINT('Ctrl Pts',(-54.685374403676,-44.5634564876869,
0.));
#138969=CARTESIAN_POINT('Ctrl Pts',(-54.685374403676,-44.5634564876869,
12.));
#138970=CARTESIAN_POINT('Ctrl Pts',(-54.6661370216242,-44.5553847872712,
0.));
#138971=CARTESIAN_POINT('Ctrl Pts',(-54.6661370216242,-44.5553847872712,
12.));
#138972=CARTESIAN_POINT('Ctrl Pts',(-54.6469546367381,-44.5473125297289,
0.));
#138973=CARTESIAN_POINT('Ctrl Pts',(-54.6469546367381,-44.5473125297289,
12.));
#138974=CARTESIAN_POINT('Ctrl Pts',(-54.6278273743554,-44.5392398566775,
0.));
#138975=CARTESIAN_POINT('Ctrl Pts',(-54.6278273743554,-44.5392398566775,
12.));
#138976=CARTESIAN_POINT('Ctrl Pts',(-54.6087553602889,-44.5311669104494,
0.));
#138977=CARTESIAN_POINT('Ctrl Pts',(-54.6087553602889,-44.5311669104494,
12.));
#138978=CARTESIAN_POINT('Ctrl Pts',(-54.5897387202812,-44.5230938335165,
0.));
#138979=CARTESIAN_POINT('Ctrl Pts',(-54.5897387202812,-44.5230938335165,
12.));
#138980=CARTESIAN_POINT('Ctrl Pts',(-54.5707775794436,-44.5150207679007,
0.));
#138981=CARTESIAN_POINT('Ctrl Pts',(-54.5707775794436,-44.5150207679007,
12.));
#138982=CARTESIAN_POINT('Ctrl Pts',(-54.5518720616056,-44.5069478544977,
0.));
#138983=CARTESIAN_POINT('Ctrl Pts',(-54.5518720616056,-44.5069478544977,
12.));
#138984=CARTESIAN_POINT('Ctrl Pts',(-54.5330222905475,-44.4988752343744,
0.));
#138985=CARTESIAN_POINT('Ctrl Pts',(-54.5330222905475,-44.4988752343744,
12.));
#138986=CARTESIAN_POINT('Ctrl Pts',(-54.5142283914704,-44.4908030503225,
0.));
#138987=CARTESIAN_POINT('Ctrl Pts',(-54.5142283914704,-44.4908030503225,
12.));
#138988=CARTESIAN_POINT('Ctrl Pts',(-54.495490492193,-44.4827314481264,
0.));
#138989=CARTESIAN_POINT('Ctrl Pts',(-54.495490492193,-44.4827314481264,
12.));
#138990=CARTESIAN_POINT('Ctrl Pts',(-54.4768087248824,-44.4746605784031,
0.));
#138991=CARTESIAN_POINT('Ctrl Pts',(-54.4768087248824,-44.4746605784031,
12.));
#138992=CARTESIAN_POINT('Ctrl Pts',(-54.4581832262033,-44.4665905967668,
0.));
#138993=CARTESIAN_POINT('Ctrl Pts',(-54.4581832262033,-44.4665905967668,
12.));
#138994=CARTESIAN_POINT('Ctrl Pts',(-54.4396141336978,-44.4585216599907,
0.));
#138995=CARTESIAN_POINT('Ctrl Pts',(-54.4396141336978,-44.4585216599907,
12.));
#138996=CARTESIAN_POINT('Ctrl Pts',(-54.421101582595,-44.4504539226327,
0.));
#138997=CARTESIAN_POINT('Ctrl Pts',(-54.421101582595,-44.4504539226327,
12.));
#138998=CARTESIAN_POINT('Ctrl Pts',(-54.4026457030335,-44.4423875340995,
0.));
#138999=CARTESIAN_POINT('Ctrl Pts',(-54.4026457030335,-44.4423875340995,
12.));
#139000=CARTESIAN_POINT('Ctrl Pts',(-54.3842466156196,-44.4343226339592,
0.));
#139001=CARTESIAN_POINT('Ctrl Pts',(-54.3842466156196,-44.4343226339592,
12.));
#139002=CARTESIAN_POINT('Ctrl Pts',(-54.3659044357119,-44.4262593564712,
0.));
#139003=CARTESIAN_POINT('Ctrl Pts',(-54.3659044357119,-44.4262593564712,
12.));
#139004=CARTESIAN_POINT('Ctrl Pts',(-54.3476192819352,-44.4181978395851,
0.));
#139005=CARTESIAN_POINT('Ctrl Pts',(-54.3476192819352,-44.4181978395851,
12.));
#139006=CARTESIAN_POINT('Ctrl Pts',(-54.3293912830237,-44.4101382321834,
0.));
#139007=CARTESIAN_POINT('Ctrl Pts',(-54.3293912830237,-44.4101382321834,
12.));
#139008=CARTESIAN_POINT('Ctrl Pts',(-54.3112205860716,-44.402080702809,
0.));
#139009=CARTESIAN_POINT('Ctrl Pts',(-54.3112205860716,-44.402080702809,
12.));
#139010=CARTESIAN_POINT('Ctrl Pts',(-54.2931073621553,-44.3940254456331,
0.));
#139011=CARTESIAN_POINT('Ctrl Pts',(-54.2931073621553,-44.3940254456331,
12.));
#139012=CARTESIAN_POINT('Ctrl Pts',(-54.2750517888579,-44.3859726620183,
0.));
#139013=CARTESIAN_POINT('Ctrl Pts',(-54.2750517888579,-44.3859726620183,
12.));
#139014=CARTESIAN_POINT('Ctrl Pts',(-54.2570540336475,-44.3779225430405,
0.));
#139015=CARTESIAN_POINT('Ctrl Pts',(-54.2570540336475,-44.3779225430405,
12.));
#139016=CARTESIAN_POINT('Ctrl Pts',(-54.2391142386412,-44.3698752533561,
0.));
#139017=CARTESIAN_POINT('Ctrl Pts',(-54.2391142386412,-44.3698752533561,
12.));
#139018=CARTESIAN_POINT('Ctrl Pts',(-54.2212325006052,-44.361830910343,
0.));
#139019=CARTESIAN_POINT('Ctrl Pts',(-54.2212325006052,-44.361830910343,
12.));
#139020=CARTESIAN_POINT('Ctrl Pts',(-54.2034088701928,-44.3537895824096,
0.));
#139021=CARTESIAN_POINT('Ctrl Pts',(-54.2034088701928,-44.3537895824096,
12.));
#139022=CARTESIAN_POINT('Ctrl Pts',(-54.1891964684727,-44.3473589597726,
0.));
#139023=CARTESIAN_POINT('Ctrl Pts',(-54.1891964684727,-44.3473589597726,
12.));
#139024=CARTESIAN_POINT('Ctrl Pts',(-54.1785633257639,-44.3425373700993,
0.));
#139025=CARTESIAN_POINT('Ctrl Pts',(-54.1785633257639,-44.3425373700993,
12.));
#139026=CARTESIAN_POINT('Ctrl Pts',(-54.1714861895346,-44.3393235891075,
0.));
#139027=CARTESIAN_POINT('Ctrl Pts',(-54.1714861895346,-44.3393235891075,
12.));
#139028=CARTESIAN_POINT('Ctrl Pts',(-54.1679505278134,-44.3377168516418,
0.));
#139029=CARTESIAN_POINT('Ctrl Pts',(-54.1679505278134,-44.3377168516418,
12.));
#139030=CARTESIAN_POINT('',(-54.1679505278134,-44.3377168516418,12.));
#139031=CARTESIAN_POINT('Ctrl Pts',(-54.1679505278134,-44.3377168516418,
12.));
#139032=CARTESIAN_POINT('Ctrl Pts',(-54.1714861895346,-44.3393235891075,
12.));
#139033=CARTESIAN_POINT('Ctrl Pts',(-54.1785633257639,-44.3425373700993,
12.));
#139034=CARTESIAN_POINT('Ctrl Pts',(-54.1891964684727,-44.3473589597726,
12.));
#139035=CARTESIAN_POINT('Ctrl Pts',(-54.2034088701928,-44.3537895824096,
12.));
#139036=CARTESIAN_POINT('Ctrl Pts',(-54.2212325006052,-44.361830910343,
12.));
#139037=CARTESIAN_POINT('Ctrl Pts',(-54.2391142386412,-44.3698752533561,
12.));
#139038=CARTESIAN_POINT('Ctrl Pts',(-54.2570540336475,-44.3779225430405,
12.));
#139039=CARTESIAN_POINT('Ctrl Pts',(-54.2750517888579,-44.3859726620183,
12.));
#139040=CARTESIAN_POINT('Ctrl Pts',(-54.2931073621553,-44.3940254456331,
12.));
#139041=CARTESIAN_POINT('Ctrl Pts',(-54.3112205860716,-44.402080702809,
12.));
#139042=CARTESIAN_POINT('Ctrl Pts',(-54.3293912830237,-44.4101382321834,
12.));
#139043=CARTESIAN_POINT('Ctrl Pts',(-54.3476192819352,-44.4181978395851,
12.));
#139044=CARTESIAN_POINT('Ctrl Pts',(-54.3659044357119,-44.4262593564712,
12.));
#139045=CARTESIAN_POINT('Ctrl Pts',(-54.3842466156196,-44.4343226339592,
12.));
#139046=CARTESIAN_POINT('Ctrl Pts',(-54.4026457030335,-44.4423875340995,
12.));
#139047=CARTESIAN_POINT('Ctrl Pts',(-54.421101582595,-44.4504539226327,
12.));
#139048=CARTESIAN_POINT('Ctrl Pts',(-54.4396141336978,-44.4585216599907,
12.));
#139049=CARTESIAN_POINT('Ctrl Pts',(-54.4581832262033,-44.4665905967668,
12.));
#139050=CARTESIAN_POINT('Ctrl Pts',(-54.4768087248824,-44.4746605784031,
12.));
#139051=CARTESIAN_POINT('Ctrl Pts',(-54.495490492193,-44.4827314481264,
12.));
#139052=CARTESIAN_POINT('Ctrl Pts',(-54.5142283914704,-44.4908030503225,
12.));
#139053=CARTESIAN_POINT('Ctrl Pts',(-54.5330222905475,-44.4988752343744,
12.));
#139054=CARTESIAN_POINT('Ctrl Pts',(-54.5518720616056,-44.5069478544977,
12.));
#139055=CARTESIAN_POINT('Ctrl Pts',(-54.5707775794436,-44.5150207679007,
12.));
#139056=CARTESIAN_POINT('Ctrl Pts',(-54.5897387202812,-44.5230938335165,
12.));
#139057=CARTESIAN_POINT('Ctrl Pts',(-54.6087553602889,-44.5311669104494,
12.));
#139058=CARTESIAN_POINT('Ctrl Pts',(-54.6278273743554,-44.5392398566775,
12.));
#139059=CARTESIAN_POINT('Ctrl Pts',(-54.6469546367381,-44.5473125297289,
12.));
#139060=CARTESIAN_POINT('Ctrl Pts',(-54.6661370216242,-44.5553847872712,
12.));
#139061=CARTESIAN_POINT('Ctrl Pts',(-54.685374403676,-44.5634564876869,
12.));
#139062=CARTESIAN_POINT('Ctrl Pts',(-54.7046666586777,-44.5715274907637,
12.));
#139063=CARTESIAN_POINT('Ctrl Pts',(-54.7240136637744,-44.5795976579476,
12.));
#139064=CARTESIAN_POINT('Ctrl Pts',(-54.7434152971285,-44.5876668519676,
12.));
#139065=CARTESIAN_POINT('Ctrl Pts',(-54.7628714377042,-44.5957349366062,
12.));
#139066=CARTESIAN_POINT('Ctrl Pts',(-54.7823819650137,-44.60380177643,12.));
#139067=CARTESIAN_POINT('Ctrl Pts',(-54.8019467588258,-44.6118672364889,
12.));
#139068=CARTESIAN_POINT('Ctrl Pts',(-54.8215656991817,-44.6199311823276,
12.));
#139069=CARTESIAN_POINT('Ctrl Pts',(-54.8412386665264,-44.6279934801159,
12.));
#139070=CARTESIAN_POINT('Ctrl Pts',(-54.860965541796,-44.6360539967392,
12.));
#139071=CARTESIAN_POINT('Ctrl Pts',(-54.8807462065177,-44.6441125999074,
12.));
#139072=CARTESIAN_POINT('Ctrl Pts',(-54.9005805428991,-44.6521691582551,
12.));
#139073=CARTESIAN_POINT('Ctrl Pts',(-54.9204684337845,-44.6602235412853,
12.));
#139074=CARTESIAN_POINT('Ctrl Pts',(-54.9404097626088,-44.6682756193155,
12.));
#139075=CARTESIAN_POINT('Ctrl Pts',(-54.9604044133497,-44.6763252634255,
12.));
#139076=CARTESIAN_POINT('Ctrl Pts',(-54.9804522704668,-44.6843723453985,
12.));
#139077=CARTESIAN_POINT('Ctrl Pts',(-55.0005532188644,-44.6924167376851,
12.));
#139078=CARTESIAN_POINT('Ctrl Pts',(-55.020707143922,-44.7004583134235,
12.));
#139079=CARTESIAN_POINT('Ctrl Pts',(-55.0409139315074,-44.7084969464509,
12.));
#139080=CARTESIAN_POINT('Ctrl Pts',(-55.0611734679902,-44.7165325113165,
12.));
#139081=CARTESIAN_POINT('Ctrl Pts',(-55.0814856402507,-44.7245648832988,
12.));
#139082=CARTESIAN_POINT('Ctrl Pts',(-55.1018503356806,-44.7325939384042,
12.));
#139083=CARTESIAN_POINT('Ctrl Pts',(-55.1222674421747,-44.7406195533482,
12.));
#139084=CARTESIAN_POINT('Ctrl Pts',(-55.1427368481201,-44.7486416055419,
12.));
#139085=CARTESIAN_POINT('Ctrl Pts',(-55.1632584423813,-44.7566599730771,
12.));
#139086=CARTESIAN_POINT('Ctrl Pts',(-55.1838321142777,-44.7646745347108,
12.));
#139087=CARTESIAN_POINT('Ctrl Pts',(-55.2044577535865,-44.7726851698618,
12.));
#139088=CARTESIAN_POINT('Ctrl Pts',(-55.2251352505474,-44.7806917586077,
12.));
#139089=CARTESIAN_POINT('Ctrl Pts',(-55.2458644958617,-44.7886941816823,
12.));
#139090=CARTESIAN_POINT('Ctrl Pts',(-55.2666453806883,-44.796692320474,
12.));
#139091=CARTESIAN_POINT('Ctrl Pts',(-55.287477796635,-44.8046860570244,
12.));
#139092=CARTESIAN_POINT('Ctrl Pts',(-55.3083616357605,-44.8126752740208,
12.));
#139093=CARTESIAN_POINT('Ctrl Pts',(-55.3292967905725,-44.8206598547887,
12.));
#139094=CARTESIAN_POINT('Ctrl Pts',(-55.3502831540228,-44.8286396832847,
12.));
#139095=CARTESIAN_POINT('Ctrl Pts',(-55.3713206194967,-44.8366146440901,
12.));
#139096=CARTESIAN_POINT('Ctrl Pts',(-55.3924090808014,-44.8445846224044,
12.));
#139097=CARTESIAN_POINT('Ctrl Pts',(-55.4135484321718,-44.8525495040408,
12.));
#139098=CARTESIAN_POINT('Ctrl Pts',(-55.4347385682704,-44.8605091754214,
12.));
#139099=CARTESIAN_POINT('Ctrl Pts',(-55.4559793841836,-44.8684635235725,
12.));
#139100=CARTESIAN_POINT('Ctrl Pts',(-55.4772707754126,-44.8764124361206,
12.));
#139101=CARTESIAN_POINT('Ctrl Pts',(-55.4986126378656,-44.8843558012886,
12.));
#139102=CARTESIAN_POINT('Ctrl Pts',(-55.5200048678629,-44.8922935078889,
12.));
#139103=CARTESIAN_POINT('Ctrl Pts',(-55.541447362134,-44.9002254453183,
12.));
#139104=CARTESIAN_POINT('Ctrl Pts',(-55.5629400178142,-44.908151503553,
12.));
#139105=CARTESIAN_POINT('Ctrl Pts',(-55.5844827324338,-44.9160715731443,
12.));
#139106=CARTESIAN_POINT('Ctrl Pts',(-55.6060754039121,-44.9239855452144,
12.));
#139107=CARTESIAN_POINT('Ctrl Pts',(-55.6277179305633,-44.9318933114506,
12.));
#139108=CARTESIAN_POINT('Ctrl Pts',(-55.6494102110935,-44.9397947641006,
12.));
#139109=CARTESIAN_POINT('Ctrl Pts',(-55.6711521445979,-44.9476897959684,
12.));
#139110=CARTESIAN_POINT('Ctrl Pts',(-55.6929436305489,-44.9555783004106,
12.));
#139111=CARTESIAN_POINT('Ctrl Pts',(-55.714784568793,-44.9634601713321,
12.));
#139112=CARTESIAN_POINT('Ctrl Pts',(-55.7366748595552,-44.9713353031804,
12.));
#139113=CARTESIAN_POINT('Ctrl Pts',(-55.7586144034367,-44.9792035909413,
12.));
#139114=CARTESIAN_POINT('Ctrl Pts',(-55.7806031014106,-44.9870649301342,
12.));
#139115=CARTESIAN_POINT('Ctrl Pts',(-55.8026408548105,-44.9949192168093,
12.));
#139116=CARTESIAN_POINT('Ctrl Pts',(-55.8247275653289,-45.0027663475433,
12.));
#139117=CARTESIAN_POINT('Ctrl Pts',(-55.8468631350218,-45.0106062194342,
12.));
#139118=CARTESIAN_POINT('Ctrl Pts',(-55.8690474663065,-45.0184387300973,
12.));
#139119=CARTESIAN_POINT('Ctrl Pts',(-55.8912804619577,-45.0262637776614,
12.));
#139120=CARTESIAN_POINT('Ctrl Pts',(-55.9135620250954,-45.0340812607657,
12.));
#139121=CARTESIAN_POINT('Ctrl Pts',(-55.9358920591837,-45.041891078555,
12.));
#139122=CARTESIAN_POINT('Ctrl Pts',(-55.9582704680356,-45.0496931306755,
12.));
#139123=CARTESIAN_POINT('Ctrl Pts',(-55.9806971558097,-45.0574873172694,
12.));
#139124=CARTESIAN_POINT('Ctrl Pts',(-56.003172027008,-45.0652735389733,
12.));
#139125=CARTESIAN_POINT('Ctrl Pts',(-56.0256949864639,-45.0730516969148,
12.));
#139126=CARTESIAN_POINT('Ctrl Pts',(-56.048265939342,-45.0808216927089,
12.));
#139127=CARTESIAN_POINT('Ctrl Pts',(-56.0708847911416,-45.0885834284517,
12.));
#139128=CARTESIAN_POINT('Ctrl Pts',(-56.0935514476945,-45.0963368067177,
12.));
#139129=CARTESIAN_POINT('Ctrl Pts',(-56.116265815162,-45.1040817305561,
12.));
#139130=CARTESIAN_POINT('Ctrl Pts',(-56.1390278000226,-45.1118181034888,
12.));
#139131=CARTESIAN_POINT('Ctrl Pts',(-56.1618373090732,-45.1195458295062,
12.));
#139132=CARTESIAN_POINT('Ctrl Pts',(-56.1846942494325,-45.127264813063,
12.));
#139133=CARTESIAN_POINT('Ctrl Pts',(-56.2075985285393,-45.1349749590737,
12.));
#139134=CARTESIAN_POINT('Ctrl Pts',(-56.230550054149,-45.1426761729105,
12.));
#139135=CARTESIAN_POINT('Ctrl Pts',(-56.2535487343221,-45.1503683604005,
12.));
#139136=CARTESIAN_POINT('Ctrl Pts',(-56.2765944774245,-45.1580514278223,
12.));
#139137=CARTESIAN_POINT('Ctrl Pts',(-56.2996871921316,-45.1657252819013,
12.));
#139138=CARTESIAN_POINT('Ctrl Pts',(-56.3228267874264,-45.173389829806,
12.));
#139139=CARTESIAN_POINT('Ctrl Pts',(-56.3460131725964,-45.1810449791453,
12.));
#139140=CARTESIAN_POINT('Ctrl Pts',(-56.3692462572231,-45.1886906379667,
12.));
#139141=CARTESIAN_POINT('Ctrl Pts',(-56.3925259511806,-45.1963267147529,
12.));
#139142=CARTESIAN_POINT('Ctrl Pts',(-56.4158521646411,-45.2039531184171,
12.));
#139143=CARTESIAN_POINT('Ctrl Pts',(-56.4392248080732,-45.2115697583,12.));
#139144=CARTESIAN_POINT('Ctrl Pts',(-56.4626437922386,-45.2191765441666,
12.));
#139145=CARTESIAN_POINT('Ctrl Pts',(-56.4861090281823,-45.2267733862049,
12.));
#139146=CARTESIAN_POINT('Ctrl Pts',(-56.5096204272306,-45.2343601950227,
12.));
#139147=CARTESIAN_POINT('Ctrl Pts',(-56.5331779009958,-45.2419368816428,
12.));
#139148=CARTESIAN_POINT('Ctrl Pts',(-56.5567813613756,-45.2495033575,12.));
#139149=CARTESIAN_POINT('Ctrl Pts',(-56.5804307205505,-45.257059534438,
12.));
#139150=CARTESIAN_POINT('Ctrl Pts',(-56.6041258909741,-45.2646053247087,
12.));
#139151=CARTESIAN_POINT('Ctrl Pts',(-56.6278667853702,-45.2721406409695,
12.));
#139152=CARTESIAN_POINT('Ctrl Pts',(-56.6516533167384,-45.2796653962785,
12.));
#139153=CARTESIAN_POINT('Ctrl Pts',(-56.6754853983528,-45.2871795040906,
12.));
#139154=CARTESIAN_POINT('Ctrl Pts',(-56.69936294376,-45.2946828782559,12.));
#139155=CARTESIAN_POINT('Ctrl Pts',(-56.7232858667709,-45.3021754330178,
12.));
#139156=CARTESIAN_POINT('Ctrl Pts',(-56.7472540814554,-45.3096570830117,
12.));
#139157=CARTESIAN_POINT('Ctrl Pts',(-56.7712675021491,-45.31712774326,12.));
#139158=CARTESIAN_POINT('Ctrl Pts',(-56.7953260434524,-45.3245873291684,
12.));
#139159=CARTESIAN_POINT('Ctrl Pts',(-56.8194296202291,-45.332035756524,
12.));
#139160=CARTESIAN_POINT('Ctrl Pts',(-56.8435781475981,-45.3394729414931,
12.));
#139161=CARTESIAN_POINT('Ctrl Pts',(-56.8677715409268,-45.3468988006203,
12.));
#139162=CARTESIAN_POINT('Ctrl Pts',(-56.8920097158377,-45.3543132508238,
12.));
#139163=CARTESIAN_POINT('Ctrl Pts',(-56.9162925882085,-45.3617162093922,
12.));
#139164=CARTESIAN_POINT('Ctrl Pts',(-56.9406200741714,-45.3691075939826,
12.));
#139165=CARTESIAN_POINT('Ctrl Pts',(-56.9649920901073,-45.3764873226196,
12.));
#139166=CARTESIAN_POINT('Ctrl Pts',(-56.9894085526373,-45.3838553136948,
12.));
#139167=CARTESIAN_POINT('Ctrl Pts',(-57.0138693786278,-45.3912114859616,
12.));
#139168=CARTESIAN_POINT('Ctrl Pts',(-57.0383744851913,-45.3985557585311,
12.));
#139169=CARTESIAN_POINT('Ctrl Pts',(-57.0629237896848,-45.4058880508693,
12.));
#139170=CARTESIAN_POINT('Ctrl Pts',(-57.0875172097051,-45.4132082827948,
12.));
#139171=CARTESIAN_POINT('Ctrl Pts',(-57.112154663078,-45.4205163744781,
12.));
#139172=CARTESIAN_POINT('Ctrl Pts',(-57.136836067863,-45.4278122464389,
12.));
#139173=CARTESIAN_POINT('Ctrl Pts',(-57.1615613423584,-45.4350958195433,
12.));
#139174=CARTESIAN_POINT('Ctrl Pts',(-57.186330405101,-45.4423670150034,
12.));
#139175=CARTESIAN_POINT('Ctrl Pts',(-57.2111431748631,-45.4496257543759,
12.));
#139176=CARTESIAN_POINT('Ctrl Pts',(-57.2359995706447,-45.4568719595641,
12.));
#139177=CARTESIAN_POINT('Ctrl Pts',(-57.2608995116733,-45.4641055528141,
12.));
#139178=CARTESIAN_POINT('Ctrl Pts',(-57.2858429174062,-45.4713264567063,
12.));
#139179=CARTESIAN_POINT('Ctrl Pts',(-57.3108297075265,-45.4785345941507,
12.));
#139180=CARTESIAN_POINT('Ctrl Pts',(-57.3358598019389,-45.4857298883824,
12.));
#139181=CARTESIAN_POINT('Ctrl Pts',(-57.3609331207574,-45.4929122629572,
12.));
#139182=CARTESIAN_POINT('Ctrl Pts',(-57.3860495843033,-45.5000816417509,
12.));
#139183=CARTESIAN_POINT('Ctrl Pts',(-57.4112091131183,-45.5072379489631,
12.));
#139184=CARTESIAN_POINT('Ctrl Pts',(-57.4364116279702,-45.5143811091205,
12.));
#139185=CARTESIAN_POINT('Ctrl Pts',(-57.4616570498568,-45.5215110470825,
12.));
#139186=CARTESIAN_POINT('Ctrl Pts',(-57.4869453000063,-45.5286276880484,
12.));
#139187=CARTESIAN_POINT('Ctrl Pts',(-57.5122762998745,-45.5357309575611,
12.));
#139188=CARTESIAN_POINT('Ctrl Pts',(-57.537649971135,-45.542820781484,12.));
#139189=CARTESIAN_POINT('Ctrl Pts',(-57.563066235668,-45.5498970859834,
12.));
#139190=CARTESIAN_POINT('Ctrl Pts',(-57.5885250155433,-45.5569597975096,
12.));
#139191=CARTESIAN_POINT('Ctrl Pts',(-57.614026233004,-45.5640088427813,
12.));
#139192=CARTESIAN_POINT('Ctrl Pts',(-57.6395698104404,-45.5710441487674,
12.));
#139193=CARTESIAN_POINT('Ctrl Pts',(-57.6651556704237,-45.5780656427163,
12.));
#139194=CARTESIAN_POINT('Ctrl Pts',(-57.6907837357418,-45.5850732521895,
12.));
#139195=CARTESIAN_POINT('Ctrl Pts',(-57.7164539294314,-45.5920669050986,
12.));
#139196=CARTESIAN_POINT('Ctrl Pts',(-57.7421661748026,-45.5990465297343,
12.));
#139197=CARTESIAN_POINT('Ctrl Pts',(-57.7679203954742,-45.6060120548205,
12.));
#139198=CARTESIAN_POINT('Ctrl Pts',(-57.7937165153387,-45.6129634094683,
12.));
#139199=CARTESIAN_POINT('Ctrl Pts',(-57.8195544584845,-45.6199005230783,
12.));
#139200=CARTESIAN_POINT('Ctrl Pts',(-57.8454341491238,-45.6268233252544,
12.));
#139201=CARTESIAN_POINT('Ctrl Pts',(-57.8713555115232,-45.6337317457252,
12.));
#139202=CARTESIAN_POINT('Ctrl Pts',(-57.8973184699034,-45.6406257142381,
12.));
#139203=CARTESIAN_POINT('Ctrl Pts',(-57.9233229484311,-45.6475051605535,
12.));
#139204=CARTESIAN_POINT('Ctrl Pts',(-57.9493688714237,-45.6543700146679,
12.));
#139205=CARTESIAN_POINT('Ctrl Pts',(-57.9754561635061,-45.661220206992,
12.));
#139206=CARTESIAN_POINT('Ctrl Pts',(-58.0015847497837,-45.6680556685493,
12.));
#139207=CARTESIAN_POINT('Ctrl Pts',(-58.0277545560012,-45.6748763311643,
12.));
#139208=CARTESIAN_POINT('Ctrl Pts',(-58.0539655087117,-45.6816821276678,
12.));
#139209=CARTESIAN_POINT('Ctrl Pts',(-58.0802175348966,-45.6884729914485,
12.));
#139210=CARTESIAN_POINT('Ctrl Pts',(-58.1065105615907,-45.695248856015,
12.));
#139211=CARTESIAN_POINT('Ctrl Pts',(-58.1328445154676,-45.702009654518,
12.));
#139212=CARTESIAN_POINT('Ctrl Pts',(-58.1592193225137,-45.7087553193771,
12.));
#139213=CARTESIAN_POINT('Ctrl Pts',(-58.185634907469,-45.7154857816483,
12.));
#139214=CARTESIAN_POINT('Ctrl Pts',(-58.2120911942772,-45.7222009715397,
12.));
#139215=CARTESIAN_POINT('Ctrl Pts',(-58.2385881070913,-45.7289008195578,
12.));
#139216=CARTESIAN_POINT('Ctrl Pts',(-58.2651255711453,-45.7355852575106,
12.));
#139217=CARTESIAN_POINT('Ctrl Pts',(-58.291703513584,-45.742254219463,12.));
#139218=CARTESIAN_POINT('Ctrl Pts',(-58.3183218645317,-45.7489076429763,
12.));
#139219=CARTESIAN_POINT('Ctrl Pts',(-58.3449805573423,-45.755545469402,
12.));
#139220=CARTESIAN_POINT('Ctrl Pts',(-58.3678667473438,-45.7612219538124,
12.));
#139221=CARTESIAN_POINT('Ctrl Pts',(-58.3854348517444,-45.7655655205367,
12.));
#139222=CARTESIAN_POINT('Ctrl Pts',(-58.397667048107,-45.7685831165565,
12.));
#139223=CARTESIAN_POINT('Ctrl Pts',(-58.4045515723357,-45.7702793558177,
12.));
#139224=CARTESIAN_POINT('Ctrl Pts',(-58.4060826907797,-45.7706564944896,
12.));
#139225=CARTESIAN_POINT('',(-54.1679505278134,-44.3377168516418,0.));
#139226=CARTESIAN_POINT('',(-54.1679505278134,-44.3377168516418,0.));
#139227=CARTESIAN_POINT('Ctrl Pts',(-58.4060826907797,-45.7706564944896,
0.));
#139228=CARTESIAN_POINT('Ctrl Pts',(-58.4045515723357,-45.7702793558177,
0.));
#139229=CARTESIAN_POINT('Ctrl Pts',(-58.397667048107,-45.7685831165565,
0.));
#139230=CARTESIAN_POINT('Ctrl Pts',(-58.3854348517444,-45.7655655205367,
0.));
#139231=CARTESIAN_POINT('Ctrl Pts',(-58.3678667473437,-45.7612219538124,
0.));
#139232=CARTESIAN_POINT('Ctrl Pts',(-58.3449805573423,-45.755545469402,
0.));
#139233=CARTESIAN_POINT('Ctrl Pts',(-58.3183218645317,-45.7489076429763,
0.));
#139234=CARTESIAN_POINT('Ctrl Pts',(-58.291703513584,-45.742254219463,0.));
#139235=CARTESIAN_POINT('Ctrl Pts',(-58.2651255711453,-45.7355852575106,
0.));
#139236=CARTESIAN_POINT('Ctrl Pts',(-58.2385881070913,-45.7289008195578,
0.));
#139237=CARTESIAN_POINT('Ctrl Pts',(-58.2120911942772,-45.7222009715397,
0.));
#139238=CARTESIAN_POINT('Ctrl Pts',(-58.185634907469,-45.7154857816483,
0.));
#139239=CARTESIAN_POINT('Ctrl Pts',(-58.1592193225137,-45.7087553193771,
0.));
#139240=CARTESIAN_POINT('Ctrl Pts',(-58.1328445154676,-45.702009654518,
0.));
#139241=CARTESIAN_POINT('Ctrl Pts',(-58.1065105615907,-45.695248856015,
0.));
#139242=CARTESIAN_POINT('Ctrl Pts',(-58.0802175348966,-45.6884729914485,
0.));
#139243=CARTESIAN_POINT('Ctrl Pts',(-58.0539655087117,-45.6816821276678,
0.));
#139244=CARTESIAN_POINT('Ctrl Pts',(-58.0277545560012,-45.6748763311643,
0.));
#139245=CARTESIAN_POINT('Ctrl Pts',(-58.0015847497837,-45.6680556685493,
0.));
#139246=CARTESIAN_POINT('Ctrl Pts',(-57.9754561635061,-45.661220206992,
0.));
#139247=CARTESIAN_POINT('Ctrl Pts',(-57.9493688714237,-45.6543700146679,
0.));
#139248=CARTESIAN_POINT('Ctrl Pts',(-57.9233229484311,-45.6475051605535,
0.));
#139249=CARTESIAN_POINT('Ctrl Pts',(-57.8973184699034,-45.6406257142381,
0.));
#139250=CARTESIAN_POINT('Ctrl Pts',(-57.8713555115232,-45.6337317457252,
0.));
#139251=CARTESIAN_POINT('Ctrl Pts',(-57.8454341491238,-45.6268233252544,
0.));
#139252=CARTESIAN_POINT('Ctrl Pts',(-57.8195544584845,-45.6199005230783,
0.));
#139253=CARTESIAN_POINT('Ctrl Pts',(-57.7937165153387,-45.6129634094683,
0.));
#139254=CARTESIAN_POINT('Ctrl Pts',(-57.7679203954742,-45.6060120548205,
0.));
#139255=CARTESIAN_POINT('Ctrl Pts',(-57.7421661748026,-45.5990465297343,
0.));
#139256=CARTESIAN_POINT('Ctrl Pts',(-57.7164539294314,-45.5920669050986,
0.));
#139257=CARTESIAN_POINT('Ctrl Pts',(-57.6907837357418,-45.5850732521895,
0.));
#139258=CARTESIAN_POINT('Ctrl Pts',(-57.6651556704237,-45.5780656427163,
0.));
#139259=CARTESIAN_POINT('Ctrl Pts',(-57.6395698104404,-45.5710441487674,
0.));
#139260=CARTESIAN_POINT('Ctrl Pts',(-57.614026233004,-45.5640088427813,
0.));
#139261=CARTESIAN_POINT('Ctrl Pts',(-57.5885250155433,-45.5569597975096,
0.));
#139262=CARTESIAN_POINT('Ctrl Pts',(-57.563066235668,-45.5498970859834,
0.));
#139263=CARTESIAN_POINT('Ctrl Pts',(-57.537649971135,-45.542820781484,0.));
#139264=CARTESIAN_POINT('Ctrl Pts',(-57.5122762998745,-45.5357309575611,
0.));
#139265=CARTESIAN_POINT('Ctrl Pts',(-57.4869453000063,-45.5286276880484,
0.));
#139266=CARTESIAN_POINT('Ctrl Pts',(-57.4616570498568,-45.5215110470825,
0.));
#139267=CARTESIAN_POINT('Ctrl Pts',(-57.4364116279702,-45.5143811091205,
0.));
#139268=CARTESIAN_POINT('Ctrl Pts',(-57.4112091131183,-45.5072379489631,
0.));
#139269=CARTESIAN_POINT('Ctrl Pts',(-57.3860495843033,-45.5000816417509,
0.));
#139270=CARTESIAN_POINT('Ctrl Pts',(-57.3609331207574,-45.4929122629572,
0.));
#139271=CARTESIAN_POINT('Ctrl Pts',(-57.3358598019389,-45.4857298883824,
0.));
#139272=CARTESIAN_POINT('Ctrl Pts',(-57.3108297075265,-45.4785345941507,
0.));
#139273=CARTESIAN_POINT('Ctrl Pts',(-57.2858429174062,-45.4713264567063,
0.));
#139274=CARTESIAN_POINT('Ctrl Pts',(-57.2608995116733,-45.4641055528141,
0.));
#139275=CARTESIAN_POINT('Ctrl Pts',(-57.2359995706447,-45.4568719595641,
0.));
#139276=CARTESIAN_POINT('Ctrl Pts',(-57.2111431748631,-45.4496257543759,
0.));
#139277=CARTESIAN_POINT('Ctrl Pts',(-57.186330405101,-45.4423670150034,
0.));
#139278=CARTESIAN_POINT('Ctrl Pts',(-57.1615613423584,-45.4350958195433,
0.));
#139279=CARTESIAN_POINT('Ctrl Pts',(-57.136836067863,-45.4278122464389,
0.));
#139280=CARTESIAN_POINT('Ctrl Pts',(-57.112154663078,-45.4205163744781,
0.));
#139281=CARTESIAN_POINT('Ctrl Pts',(-57.0875172097051,-45.4132082827948,
0.));
#139282=CARTESIAN_POINT('Ctrl Pts',(-57.0629237896848,-45.4058880508693,
0.));
#139283=CARTESIAN_POINT('Ctrl Pts',(-57.0383744851913,-45.3985557585311,
0.));
#139284=CARTESIAN_POINT('Ctrl Pts',(-57.0138693786278,-45.3912114859616,
0.));
#139285=CARTESIAN_POINT('Ctrl Pts',(-56.9894085526373,-45.3838553136948,
0.));
#139286=CARTESIAN_POINT('Ctrl Pts',(-56.9649920901073,-45.3764873226196,
0.));
#139287=CARTESIAN_POINT('Ctrl Pts',(-56.9406200741714,-45.3691075939826,
0.));
#139288=CARTESIAN_POINT('Ctrl Pts',(-56.9162925882085,-45.3617162093922,
0.));
#139289=CARTESIAN_POINT('Ctrl Pts',(-56.8920097158377,-45.3543132508238,
0.));
#139290=CARTESIAN_POINT('Ctrl Pts',(-56.8677715409268,-45.3468988006203,
0.));
#139291=CARTESIAN_POINT('Ctrl Pts',(-56.8435781475981,-45.3394729414931,
0.));
#139292=CARTESIAN_POINT('Ctrl Pts',(-56.8194296202291,-45.332035756524,
0.));
#139293=CARTESIAN_POINT('Ctrl Pts',(-56.7953260434524,-45.3245873291684,
0.));
#139294=CARTESIAN_POINT('Ctrl Pts',(-56.7712675021491,-45.31712774326,0.));
#139295=CARTESIAN_POINT('Ctrl Pts',(-56.7472540814554,-45.3096570830117,
0.));
#139296=CARTESIAN_POINT('Ctrl Pts',(-56.7232858667709,-45.3021754330178,
0.));
#139297=CARTESIAN_POINT('Ctrl Pts',(-56.69936294376,-45.2946828782559,0.));
#139298=CARTESIAN_POINT('Ctrl Pts',(-56.6754853983528,-45.2871795040906,
0.));
#139299=CARTESIAN_POINT('Ctrl Pts',(-56.6516533167384,-45.2796653962785,
0.));
#139300=CARTESIAN_POINT('Ctrl Pts',(-56.6278667853702,-45.2721406409695,
0.));
#139301=CARTESIAN_POINT('Ctrl Pts',(-56.6041258909741,-45.2646053247087,
0.));
#139302=CARTESIAN_POINT('Ctrl Pts',(-56.5804307205505,-45.257059534438,
0.));
#139303=CARTESIAN_POINT('Ctrl Pts',(-56.5567813613756,-45.2495033575,0.));
#139304=CARTESIAN_POINT('Ctrl Pts',(-56.5331779009958,-45.2419368816428,
0.));
#139305=CARTESIAN_POINT('Ctrl Pts',(-56.5096204272306,-45.2343601950227,
0.));
#139306=CARTESIAN_POINT('Ctrl Pts',(-56.4861090281823,-45.2267733862049,
0.));
#139307=CARTESIAN_POINT('Ctrl Pts',(-56.4626437922386,-45.2191765441666,
0.));
#139308=CARTESIAN_POINT('Ctrl Pts',(-56.4392248080732,-45.2115697583,0.));
#139309=CARTESIAN_POINT('Ctrl Pts',(-56.4158521646411,-45.2039531184171,
0.));
#139310=CARTESIAN_POINT('Ctrl Pts',(-56.3925259511806,-45.1963267147529,
0.));
#139311=CARTESIAN_POINT('Ctrl Pts',(-56.3692462572231,-45.1886906379667,
0.));
#139312=CARTESIAN_POINT('Ctrl Pts',(-56.3460131725964,-45.1810449791453,
0.));
#139313=CARTESIAN_POINT('Ctrl Pts',(-56.3228267874264,-45.173389829806,
0.));
#139314=CARTESIAN_POINT('Ctrl Pts',(-56.2996871921316,-45.1657252819013,
0.));
#139315=CARTESIAN_POINT('Ctrl Pts',(-56.2765944774245,-45.1580514278223,
0.));
#139316=CARTESIAN_POINT('Ctrl Pts',(-56.2535487343221,-45.1503683604005,
0.));
#139317=CARTESIAN_POINT('Ctrl Pts',(-56.230550054149,-45.1426761729105,
0.));
#139318=CARTESIAN_POINT('Ctrl Pts',(-56.2075985285393,-45.1349749590737,
0.));
#139319=CARTESIAN_POINT('Ctrl Pts',(-56.1846942494325,-45.127264813063,
0.));
#139320=CARTESIAN_POINT('Ctrl Pts',(-56.1618373090732,-45.1195458295062,
0.));
#139321=CARTESIAN_POINT('Ctrl Pts',(-56.1390278000226,-45.1118181034888,
0.));
#139322=CARTESIAN_POINT('Ctrl Pts',(-56.116265815162,-45.1040817305561,
0.));
#139323=CARTESIAN_POINT('Ctrl Pts',(-56.0935514476945,-45.0963368067177,
0.));
#139324=CARTESIAN_POINT('Ctrl Pts',(-56.0708847911416,-45.0885834284517,
0.));
#139325=CARTESIAN_POINT('Ctrl Pts',(-56.048265939342,-45.0808216927089,
0.));
#139326=CARTESIAN_POINT('Ctrl Pts',(-56.0256949864639,-45.0730516969148,
0.));
#139327=CARTESIAN_POINT('Ctrl Pts',(-56.003172027008,-45.0652735389733,
0.));
#139328=CARTESIAN_POINT('Ctrl Pts',(-55.9806971558097,-45.0574873172694,
0.));
#139329=CARTESIAN_POINT('Ctrl Pts',(-55.9582704680356,-45.0496931306755,
0.));
#139330=CARTESIAN_POINT('Ctrl Pts',(-55.9358920591837,-45.041891078555,
0.));
#139331=CARTESIAN_POINT('Ctrl Pts',(-55.9135620250954,-45.0340812607657,
0.));
#139332=CARTESIAN_POINT('Ctrl Pts',(-55.8912804619577,-45.0262637776614,
0.));
#139333=CARTESIAN_POINT('Ctrl Pts',(-55.8690474663065,-45.0184387300973,
0.));
#139334=CARTESIAN_POINT('Ctrl Pts',(-55.8468631350218,-45.0106062194342,
0.));
#139335=CARTESIAN_POINT('Ctrl Pts',(-55.8247275653289,-45.0027663475433,
0.));
#139336=CARTESIAN_POINT('Ctrl Pts',(-55.8026408548105,-44.9949192168093,
0.));
#139337=CARTESIAN_POINT('Ctrl Pts',(-55.7806031014106,-44.9870649301342,
0.));
#139338=CARTESIAN_POINT('Ctrl Pts',(-55.7586144034367,-44.9792035909413,
0.));
#139339=CARTESIAN_POINT('Ctrl Pts',(-55.7366748595552,-44.9713353031804,
0.));
#139340=CARTESIAN_POINT('Ctrl Pts',(-55.714784568793,-44.9634601713321,
0.));
#139341=CARTESIAN_POINT('Ctrl Pts',(-55.6929436305489,-44.9555783004106,
0.));
#139342=CARTESIAN_POINT('Ctrl Pts',(-55.6711521445979,-44.9476897959684,
0.));
#139343=CARTESIAN_POINT('Ctrl Pts',(-55.6494102110935,-44.9397947641006,
0.));
#139344=CARTESIAN_POINT('Ctrl Pts',(-55.6277179305633,-44.9318933114506,
0.));
#139345=CARTESIAN_POINT('Ctrl Pts',(-55.6060754039121,-44.9239855452144,
0.));
#139346=CARTESIAN_POINT('Ctrl Pts',(-55.5844827324338,-44.9160715731443,
0.));
#139347=CARTESIAN_POINT('Ctrl Pts',(-55.5629400178142,-44.908151503553,
0.));
#139348=CARTESIAN_POINT('Ctrl Pts',(-55.541447362134,-44.9002254453183,
0.));
#139349=CARTESIAN_POINT('Ctrl Pts',(-55.5200048678629,-44.8922935078889,
0.));
#139350=CARTESIAN_POINT('Ctrl Pts',(-55.4986126378656,-44.8843558012886,
0.));
#139351=CARTESIAN_POINT('Ctrl Pts',(-55.4772707754126,-44.8764124361206,
0.));
#139352=CARTESIAN_POINT('Ctrl Pts',(-55.4559793841836,-44.8684635235725,
0.));
#139353=CARTESIAN_POINT('Ctrl Pts',(-55.4347385682704,-44.8605091754214,
0.));
#139354=CARTESIAN_POINT('Ctrl Pts',(-55.4135484321718,-44.8525495040408,
0.));
#139355=CARTESIAN_POINT('Ctrl Pts',(-55.3924090808014,-44.8445846224044,
0.));
#139356=CARTESIAN_POINT('Ctrl Pts',(-55.3713206194967,-44.8366146440901,
0.));
#139357=CARTESIAN_POINT('Ctrl Pts',(-55.3502831540228,-44.8286396832847,
0.));
#139358=CARTESIAN_POINT('Ctrl Pts',(-55.3292967905725,-44.8206598547887,
0.));
#139359=CARTESIAN_POINT('Ctrl Pts',(-55.3083616357605,-44.8126752740208,
0.));
#139360=CARTESIAN_POINT('Ctrl Pts',(-55.287477796635,-44.8046860570244,
0.));
#139361=CARTESIAN_POINT('Ctrl Pts',(-55.2666453806883,-44.796692320474,
0.));
#139362=CARTESIAN_POINT('Ctrl Pts',(-55.2458644958617,-44.7886941816823,
0.));
#139363=CARTESIAN_POINT('Ctrl Pts',(-55.2251352505474,-44.7806917586077,
0.));
#139364=CARTESIAN_POINT('Ctrl Pts',(-55.2044577535865,-44.7726851698618,
0.));
#139365=CARTESIAN_POINT('Ctrl Pts',(-55.1838321142777,-44.7646745347108,
0.));
#139366=CARTESIAN_POINT('Ctrl Pts',(-55.1632584423813,-44.7566599730771,
0.));
#139367=CARTESIAN_POINT('Ctrl Pts',(-55.1427368481201,-44.7486416055419,
0.));
#139368=CARTESIAN_POINT('Ctrl Pts',(-55.1222674421747,-44.7406195533482,
0.));
#139369=CARTESIAN_POINT('Ctrl Pts',(-55.1018503356806,-44.7325939384042,
0.));
#139370=CARTESIAN_POINT('Ctrl Pts',(-55.0814856402507,-44.7245648832988,
0.));
#139371=CARTESIAN_POINT('Ctrl Pts',(-55.0611734679902,-44.7165325113165,
0.));
#139372=CARTESIAN_POINT('Ctrl Pts',(-55.0409139315074,-44.7084969464509,
0.));
#139373=CARTESIAN_POINT('Ctrl Pts',(-55.020707143922,-44.7004583134235,
0.));
#139374=CARTESIAN_POINT('Ctrl Pts',(-55.0005532188644,-44.6924167376851,
0.));
#139375=CARTESIAN_POINT('Ctrl Pts',(-54.9804522704668,-44.6843723453985,
0.));
#139376=CARTESIAN_POINT('Ctrl Pts',(-54.9604044133497,-44.6763252634255,
0.));
#139377=CARTESIAN_POINT('Ctrl Pts',(-54.9404097626088,-44.6682756193155,
0.));
#139378=CARTESIAN_POINT('Ctrl Pts',(-54.9204684337845,-44.6602235412853,
0.));
#139379=CARTESIAN_POINT('Ctrl Pts',(-54.9005805428991,-44.6521691582551,
0.));
#139380=CARTESIAN_POINT('Ctrl Pts',(-54.8807462065177,-44.6441125999074,
0.));
#139381=CARTESIAN_POINT('Ctrl Pts',(-54.860965541796,-44.6360539967392,
0.));
#139382=CARTESIAN_POINT('Ctrl Pts',(-54.8412386665264,-44.6279934801159,
0.));
#139383=CARTESIAN_POINT('Ctrl Pts',(-54.8215656991817,-44.6199311823276,
0.));
#139384=CARTESIAN_POINT('Ctrl Pts',(-54.8019467588258,-44.6118672364889,
0.));
#139385=CARTESIAN_POINT('Ctrl Pts',(-54.7823819650137,-44.60380177643,0.));
#139386=CARTESIAN_POINT('Ctrl Pts',(-54.7628714377042,-44.5957349366062,
0.));
#139387=CARTESIAN_POINT('Ctrl Pts',(-54.7434152971285,-44.5876668519676,
0.));
#139388=CARTESIAN_POINT('Ctrl Pts',(-54.7240136637744,-44.5795976579476,
0.));
#139389=CARTESIAN_POINT('Ctrl Pts',(-54.7046666586777,-44.5715274907637,
0.));
#139390=CARTESIAN_POINT('Ctrl Pts',(-54.685374403676,-44.5634564876869,
0.));
#139391=CARTESIAN_POINT('Ctrl Pts',(-54.6661370216242,-44.5553847872712,
0.));
#139392=CARTESIAN_POINT('Ctrl Pts',(-54.6469546367381,-44.5473125297289,
0.));
#139393=CARTESIAN_POINT('Ctrl Pts',(-54.6278273743554,-44.5392398566775,
0.));
#139394=CARTESIAN_POINT('Ctrl Pts',(-54.6087553602889,-44.5311669104494,
0.));
#139395=CARTESIAN_POINT('Ctrl Pts',(-54.5897387202812,-44.5230938335165,
0.));
#139396=CARTESIAN_POINT('Ctrl Pts',(-54.5707775794436,-44.5150207679007,
0.));
#139397=CARTESIAN_POINT('Ctrl Pts',(-54.5518720616056,-44.5069478544977,
0.));
#139398=CARTESIAN_POINT('Ctrl Pts',(-54.5330222905475,-44.4988752343744,
0.));
#139399=CARTESIAN_POINT('Ctrl Pts',(-54.5142283914704,-44.4908030503225,
0.));
#139400=CARTESIAN_POINT('Ctrl Pts',(-54.495490492193,-44.4827314481264,
0.));
#139401=CARTESIAN_POINT('Ctrl Pts',(-54.4768087248824,-44.4746605784031,
0.));
#139402=CARTESIAN_POINT('Ctrl Pts',(-54.4581832262033,-44.4665905967668,
0.));
#139403=CARTESIAN_POINT('Ctrl Pts',(-54.4396141336978,-44.4585216599907,
0.));
#139404=CARTESIAN_POINT('Ctrl Pts',(-54.421101582595,-44.4504539226327,
0.));
#139405=CARTESIAN_POINT('Ctrl Pts',(-54.4026457030335,-44.4423875340995,
0.));
#139406=CARTESIAN_POINT('Ctrl Pts',(-54.3842466156196,-44.4343226339592,
0.));
#139407=CARTESIAN_POINT('Ctrl Pts',(-54.3659044357119,-44.4262593564712,
0.));
#139408=CARTESIAN_POINT('Ctrl Pts',(-54.3476192819352,-44.4181978395851,
0.));
#139409=CARTESIAN_POINT('Ctrl Pts',(-54.3293912830237,-44.4101382321834,
0.));
#139410=CARTESIAN_POINT('Ctrl Pts',(-54.3112205860716,-44.402080702809,
0.));
#139411=CARTESIAN_POINT('Ctrl Pts',(-54.2931073621553,-44.3940254456331,
0.));
#139412=CARTESIAN_POINT('Ctrl Pts',(-54.2750517888579,-44.3859726620183,
0.));
#139413=CARTESIAN_POINT('Ctrl Pts',(-54.2570540336475,-44.3779225430405,
0.));
#139414=CARTESIAN_POINT('Ctrl Pts',(-54.2391142386412,-44.3698752533561,
0.));
#139415=CARTESIAN_POINT('Ctrl Pts',(-54.2212325006052,-44.361830910343,
0.));
#139416=CARTESIAN_POINT('Ctrl Pts',(-54.2034088701928,-44.3537895824096,
0.));
#139417=CARTESIAN_POINT('Ctrl Pts',(-54.1891964684727,-44.3473589597726,
0.));
#139418=CARTESIAN_POINT('Ctrl Pts',(-54.1785633257639,-44.3425373700993,
0.));
#139419=CARTESIAN_POINT('Ctrl Pts',(-54.1714861895346,-44.3393235891075,
0.));
#139420=CARTESIAN_POINT('Ctrl Pts',(-54.1679505278134,-44.3377168516418,
0.));
#139421=CARTESIAN_POINT('Ctrl Pts',(-62.494763006804,-40.5543412808469,
0.));
#139422=CARTESIAN_POINT('Ctrl Pts',(-62.494763006804,-40.5543412808469,
12.));
#139423=CARTESIAN_POINT('Ctrl Pts',(-62.489224912198,-40.5535399497519,
0.));
#139424=CARTESIAN_POINT('Ctrl Pts',(-62.489224912198,-40.5535399497519,
12.));
#139425=CARTESIAN_POINT('Ctrl Pts',(-62.4781525156318,-40.5519353177252,
0.));
#139426=CARTESIAN_POINT('Ctrl Pts',(-62.4781525156318,-40.5519353177252,
12.));
#139427=CARTESIAN_POINT('Ctrl Pts',(-62.4615552987202,-40.5495224601758,
0.));
#139428=CARTESIAN_POINT('Ctrl Pts',(-62.4615552987202,-40.5495224601758,
12.));
#139429=CARTESIAN_POINT('Ctrl Pts',(-62.4394484329678,-40.5462934972718,
0.));
#139430=CARTESIAN_POINT('Ctrl Pts',(-62.4394484329678,-40.5462934972718,
12.));
#139431=CARTESIAN_POINT('Ctrl Pts',(-62.4118527881148,-40.5422375945026,
0.));
#139432=CARTESIAN_POINT('Ctrl Pts',(-62.4118527881148,-40.5422375945026,
12.));
#139433=CARTESIAN_POINT('Ctrl Pts',(-62.3842950992833,-40.5381619974169,
0.));
#139434=CARTESIAN_POINT('Ctrl Pts',(-62.3842950992833,-40.5381619974169,
12.));
#139435=CARTESIAN_POINT('Ctrl Pts',(-62.3567753970279,-40.5340667194319,
0.));
#139436=CARTESIAN_POINT('Ctrl Pts',(-62.3567753970279,-40.5340667194319,
12.));
#139437=CARTESIAN_POINT('Ctrl Pts',(-62.3292937257902,-40.5299517857721,
0.));
#139438=CARTESIAN_POINT('Ctrl Pts',(-62.3292937257902,-40.5299517857721,
12.));
#139439=CARTESIAN_POINT('Ctrl Pts',(-62.301850147165,-40.5258172381428,
0.));
#139440=CARTESIAN_POINT('Ctrl Pts',(-62.301850147165,-40.5258172381428,
12.));
#139441=CARTESIAN_POINT('Ctrl Pts',(-62.2744447381971,-40.5216631336193,
0.));
#139442=CARTESIAN_POINT('Ctrl Pts',(-62.2744447381971,-40.5216631336193,
12.));
#139443=CARTESIAN_POINT('Ctrl Pts',(-62.247077585866,-40.5174895390954,
0.));
#139444=CARTESIAN_POINT('Ctrl Pts',(-62.247077585866,-40.5174895390954,
12.));
#139445=CARTESIAN_POINT('Ctrl Pts',(-62.2197487826136,-40.5132965269633,
0.));
#139446=CARTESIAN_POINT('Ctrl Pts',(-62.2197487826136,-40.5132965269633,
12.));
#139447=CARTESIAN_POINT('Ctrl Pts',(-62.1924584215653,-40.5090841704122,
0.));
#139448=CARTESIAN_POINT('Ctrl Pts',(-62.1924584215653,-40.5090841704122,
12.));
#139449=CARTESIAN_POINT('Ctrl Pts',(-62.1652065915808,-40.5048525386035,
0.));
#139450=CARTESIAN_POINT('Ctrl Pts',(-62.1652065915808,-40.5048525386035,
12.));
#139451=CARTESIAN_POINT('Ctrl Pts',(-62.1379933732528,-40.5006016927554,
0.));
#139452=CARTESIAN_POINT('Ctrl Pts',(-62.1379933732528,-40.5006016927554,
12.));
#139453=CARTESIAN_POINT('Ctrl Pts',(-62.1108188417004,-40.4963316888412,
0.));
#139454=CARTESIAN_POINT('Ctrl Pts',(-62.1108188417004,-40.4963316888412,
12.));
#139455=CARTESIAN_POINT('Ctrl Pts',(-62.083683068572,-40.4920425795216,
0.));
#139456=CARTESIAN_POINT('Ctrl Pts',(-62.083683068572,-40.4920425795216,
12.));
#139457=CARTESIAN_POINT('Ctrl Pts',(-62.0565861244179,-40.4877344164411,
0.));
#139458=CARTESIAN_POINT('Ctrl Pts',(-62.0565861244179,-40.4877344164411,
12.));
#139459=CARTESIAN_POINT('Ctrl Pts',(-62.029528080742,-40.4834072522164,
0.));
#139460=CARTESIAN_POINT('Ctrl Pts',(-62.029528080742,-40.4834072522164,
12.));
#139461=CARTESIAN_POINT('Ctrl Pts',(-62.0025090125959,-40.4790611429583,
0.));
#139462=CARTESIAN_POINT('Ctrl Pts',(-62.0025090125959,-40.4790611429583,
12.));
#139463=CARTESIAN_POINT('Ctrl Pts',(-61.9755289983044,-40.4746961480015,
0.));
#139464=CARTESIAN_POINT('Ctrl Pts',(-61.9755289983044,-40.4746961480015,
12.));
#139465=CARTESIAN_POINT('Ctrl Pts',(-61.9485881182921,-40.470312328762,
0.));
#139466=CARTESIAN_POINT('Ctrl Pts',(-61.9485881182921,-40.470312328762,
12.));
#139467=CARTESIAN_POINT('Ctrl Pts',(-61.9216864541744,-40.4659097478587,
0.));
#139468=CARTESIAN_POINT('Ctrl Pts',(-61.9216864541744,-40.4659097478587,
12.));
#139469=CARTESIAN_POINT('Ctrl Pts',(-61.8948240878008,-40.4614884681889,
0.));
#139470=CARTESIAN_POINT('Ctrl Pts',(-61.8948240878008,-40.4614884681889,
12.));
#139471=CARTESIAN_POINT('Ctrl Pts',(-61.8680011001537,-40.4570485518749,
0.));
#139472=CARTESIAN_POINT('Ctrl Pts',(-61.8680011001537,-40.4570485518749,
12.));
#139473=CARTESIAN_POINT('Ctrl Pts',(-61.8412175708553,-40.4525900597894,
0.));
#139474=CARTESIAN_POINT('Ctrl Pts',(-61.8412175708553,-40.4525900597894,
12.));
#139475=CARTESIAN_POINT('Ctrl Pts',(-61.814473578779,-40.4481130521364,
0.));
#139476=CARTESIAN_POINT('Ctrl Pts',(-61.814473578779,-40.4481130521364,
12.));
#139477=CARTESIAN_POINT('Ctrl Pts',(-61.7877692024076,-40.4436175887949,
0.));
#139478=CARTESIAN_POINT('Ctrl Pts',(-61.7877692024076,-40.4436175887949,
12.));
#139479=CARTESIAN_POINT('Ctrl Pts',(-61.7611045202874,-40.4391037297588,
0.));
#139480=CARTESIAN_POINT('Ctrl Pts',(-61.7611045202874,-40.4391037297588,
12.));
#139481=CARTESIAN_POINT('Ctrl Pts',(-61.7344796114399,-40.4345715355404,
0.));
#139482=CARTESIAN_POINT('Ctrl Pts',(-61.7344796114399,-40.4345715355404,
12.));
#139483=CARTESIAN_POINT('Ctrl Pts',(-61.7078945557799,-40.430021067584,
0.));
#139484=CARTESIAN_POINT('Ctrl Pts',(-61.7078945557799,-40.430021067584,
12.));
#139485=CARTESIAN_POINT('Ctrl Pts',(-61.6813494339286,-40.425452388076,
0.));
#139486=CARTESIAN_POINT('Ctrl Pts',(-61.6813494339286,-40.425452388076,
12.));
#139487=CARTESIAN_POINT('Ctrl Pts',(-61.6548443270394,-40.4208655597717,
0.));
#139488=CARTESIAN_POINT('Ctrl Pts',(-61.6548443270394,-40.4208655597717,
12.));
#139489=CARTESIAN_POINT('Ctrl Pts',(-61.628379316608,-40.4162606458118,
0.));
#139490=CARTESIAN_POINT('Ctrl Pts',(-61.628379316608,-40.4162606458118,
12.));
#139491=CARTESIAN_POINT('Ctrl Pts',(-61.6019544843011,-40.4116377095596,
0.));
#139492=CARTESIAN_POINT('Ctrl Pts',(-61.6019544843011,-40.4116377095596,
12.));
#139493=CARTESIAN_POINT('Ctrl Pts',(-61.5755699117324,-40.4069968143956,
0.));
#139494=CARTESIAN_POINT('Ctrl Pts',(-61.5755699117324,-40.4069968143956,
12.));
#139495=CARTESIAN_POINT('Ctrl Pts',(-61.5492256804717,-40.4023380237232,
0.));
#139496=CARTESIAN_POINT('Ctrl Pts',(-61.5492256804717,-40.4023380237232,
12.));
#139497=CARTESIAN_POINT('Ctrl Pts',(-61.522921872154,-40.3976614010652,
0.));
#139498=CARTESIAN_POINT('Ctrl Pts',(-61.522921872154,-40.3976614010652,
12.));
#139499=CARTESIAN_POINT('Ctrl Pts',(-61.4966585685549,-40.3929670101365,
0.));
#139500=CARTESIAN_POINT('Ctrl Pts',(-61.4966585685549,-40.3929670101365,
12.));
#139501=CARTESIAN_POINT('Ctrl Pts',(-61.4704358516709,-40.3882549149227,
0.));
#139502=CARTESIAN_POINT('Ctrl Pts',(-61.4704358516709,-40.3882549149227,
12.));
#139503=CARTESIAN_POINT('Ctrl Pts',(-61.4442538038044,-40.383525179772,
0.));
#139504=CARTESIAN_POINT('Ctrl Pts',(-61.4442538038044,-40.383525179772,
12.));
#139505=CARTESIAN_POINT('Ctrl Pts',(-61.4181125076037,-40.3787778694364,
0.));
#139506=CARTESIAN_POINT('Ctrl Pts',(-61.4181125076037,-40.3787778694364,
12.));
#139507=CARTESIAN_POINT('Ctrl Pts',(-61.3920120460219,-40.3740130490225,
0.));
#139508=CARTESIAN_POINT('Ctrl Pts',(-61.3920120460219,-40.3740130490225,
12.));
#139509=CARTESIAN_POINT('Ctrl Pts',(-61.3659525022908,-40.3692307839636,
0.));
#139510=CARTESIAN_POINT('Ctrl Pts',(-61.3659525022908,-40.3692307839636,
12.));
#139511=CARTESIAN_POINT('Ctrl Pts',(-61.3399339598853,-40.3644311399861,
0.));
#139512=CARTESIAN_POINT('Ctrl Pts',(-61.3399339598853,-40.3644311399861,
12.));
#139513=CARTESIAN_POINT('Ctrl Pts',(-61.3139565024847,-40.3596141830791,
0.));
#139514=CARTESIAN_POINT('Ctrl Pts',(-61.3139565024847,-40.3596141830791,
12.));
#139515=CARTESIAN_POINT('Ctrl Pts',(-61.2880202139371,-40.3547799794679,
0.));
#139516=CARTESIAN_POINT('Ctrl Pts',(-61.2880202139371,-40.3547799794679,
12.));
#139517=CARTESIAN_POINT('Ctrl Pts',(-61.2621251782863,-40.3499285956304,
0.));
#139518=CARTESIAN_POINT('Ctrl Pts',(-61.2621251782863,-40.3499285956304,
12.));
#139519=CARTESIAN_POINT('Ctrl Pts',(-61.23627147979,-40.3450600983109,0.));
#139520=CARTESIAN_POINT('Ctrl Pts',(-61.23627147979,-40.3450600983109,12.));
#139521=CARTESIAN_POINT('Ctrl Pts',(-61.2104592029377,-40.340174554537,
0.));
#139522=CARTESIAN_POINT('Ctrl Pts',(-61.2104592029377,-40.340174554537,
12.));
#139523=CARTESIAN_POINT('Ctrl Pts',(-61.1846884324644,-40.335272031637,
0.));
#139524=CARTESIAN_POINT('Ctrl Pts',(-61.1846884324644,-40.335272031637,
12.));
#139525=CARTESIAN_POINT('Ctrl Pts',(-61.1589592533613,-40.3303525972615,
0.));
#139526=CARTESIAN_POINT('Ctrl Pts',(-61.1589592533613,-40.3303525972615,
12.));
#139527=CARTESIAN_POINT('Ctrl Pts',(-61.1332717508789,-40.32541631938,0.));
#139528=CARTESIAN_POINT('Ctrl Pts',(-61.1332717508789,-40.32541631938,12.));
#139529=CARTESIAN_POINT('Ctrl Pts',(-61.1076260105258,-40.3204632662725,
0.));
#139530=CARTESIAN_POINT('Ctrl Pts',(-61.1076260105258,-40.3204632662725,
12.));
#139531=CARTESIAN_POINT('Ctrl Pts',(-61.0820221180645,-40.3154935065262,
0.));
#139532=CARTESIAN_POINT('Ctrl Pts',(-61.0820221180645,-40.3154935065262,
12.));
#139533=CARTESIAN_POINT('Ctrl Pts',(-61.056460159505,-40.3105071090309,
0.));
#139534=CARTESIAN_POINT('Ctrl Pts',(-61.056460159505,-40.3105071090309,
12.));
#139535=CARTESIAN_POINT('Ctrl Pts',(-61.0309402210921,-40.3055041429775,
0.));
#139536=CARTESIAN_POINT('Ctrl Pts',(-61.0309402210921,-40.3055041429775,
12.));
#139537=CARTESIAN_POINT('Ctrl Pts',(-61.0054623893066,-40.300484677858,
0.));
#139538=CARTESIAN_POINT('Ctrl Pts',(-61.0054623893066,-40.300484677858,
12.));
#139539=CARTESIAN_POINT('Ctrl Pts',(-60.9800267508787,-40.295448783469,
0.));
#139540=CARTESIAN_POINT('Ctrl Pts',(-60.9800267508787,-40.295448783469,
12.));
#139541=CARTESIAN_POINT('Ctrl Pts',(-60.9546333927921,-40.2903965299155,
0.));
#139542=CARTESIAN_POINT('Ctrl Pts',(-60.9546333927921,-40.2903965299155,
12.));
#139543=CARTESIAN_POINT('Ctrl Pts',(-60.9292824022887,-40.2853279876161,
0.));
#139544=CARTESIAN_POINT('Ctrl Pts',(-60.9292824022887,-40.2853279876161,
12.));
#139545=CARTESIAN_POINT('Ctrl Pts',(-60.9039738668669,-40.2802432273104,
0.));
#139546=CARTESIAN_POINT('Ctrl Pts',(-60.9039738668669,-40.2802432273104,
12.));
#139547=CARTESIAN_POINT('Ctrl Pts',(-60.8787078742818,-40.2751423200639,
0.));
#139548=CARTESIAN_POINT('Ctrl Pts',(-60.8787078742818,-40.2751423200639,
12.));
#139549=CARTESIAN_POINT('Ctrl Pts',(-60.8534845125538,-40.2700253372647,
0.));
#139550=CARTESIAN_POINT('Ctrl Pts',(-60.8534845125538,-40.2700253372647,
12.));
#139551=CARTESIAN_POINT('Ctrl Pts',(-60.8283038699706,-40.2648923506248,
0.));
#139552=CARTESIAN_POINT('Ctrl Pts',(-60.8283038699706,-40.2648923506248,
12.));
#139553=CARTESIAN_POINT('Ctrl Pts',(-60.8031660350879,-40.2597434321803,
0.));
#139554=CARTESIAN_POINT('Ctrl Pts',(-60.8031660350879,-40.2597434321803,
12.));
#139555=CARTESIAN_POINT('Ctrl Pts',(-60.7780710967248,-40.2545786542953,
0.));
#139556=CARTESIAN_POINT('Ctrl Pts',(-60.7780710967248,-40.2545786542953,
12.));
#139557=CARTESIAN_POINT('Ctrl Pts',(-60.7530191439593,-40.2493980896638,
0.));
#139558=CARTESIAN_POINT('Ctrl Pts',(-60.7530191439593,-40.2493980896638,
12.));
#139559=CARTESIAN_POINT('Ctrl Pts',(-60.728010266139,-40.2442018113108,
0.));
#139560=CARTESIAN_POINT('Ctrl Pts',(-60.728010266139,-40.2442018113108,
12.));
#139561=CARTESIAN_POINT('Ctrl Pts',(-60.7030445528857,-40.2389898925932,
0.));
#139562=CARTESIAN_POINT('Ctrl Pts',(-60.7030445528857,-40.2389898925932,
12.));
#139563=CARTESIAN_POINT('Ctrl Pts',(-60.678122094098,-40.2337624072028,
0.));
#139564=CARTESIAN_POINT('Ctrl Pts',(-60.678122094098,-40.2337624072028,
12.));
#139565=CARTESIAN_POINT('Ctrl Pts',(-60.6532429799499,-40.2285194291706,
0.));
#139566=CARTESIAN_POINT('Ctrl Pts',(-60.6532429799499,-40.2285194291706,
12.));
#139567=CARTESIAN_POINT('Ctrl Pts',(-60.6284073008871,-40.2232610328721,
0.));
#139568=CARTESIAN_POINT('Ctrl Pts',(-60.6284073008871,-40.2232610328721,
12.));
#139569=CARTESIAN_POINT('Ctrl Pts',(-60.6036151476349,-40.2179872930273,
0.));
#139570=CARTESIAN_POINT('Ctrl Pts',(-60.6036151476349,-40.2179872930273,
12.));
#139571=CARTESIAN_POINT('Ctrl Pts',(-60.5788666112042,-40.2126982847011,
0.));
#139572=CARTESIAN_POINT('Ctrl Pts',(-60.5788666112042,-40.2126982847011,
12.));
#139573=CARTESIAN_POINT('Ctrl Pts',(-60.5541617828925,-40.2073940833052,
0.));
#139574=CARTESIAN_POINT('Ctrl Pts',(-60.5541617828925,-40.2073940833052,
12.));
#139575=CARTESIAN_POINT('Ctrl Pts',(-60.5295007542841,-40.2020747646014,
0.));
#139576=CARTESIAN_POINT('Ctrl Pts',(-60.5295007542841,-40.2020747646014,
12.));
#139577=CARTESIAN_POINT('Ctrl Pts',(-60.5048836172435,-40.1967404047062,
0.));
#139578=CARTESIAN_POINT('Ctrl Pts',(-60.5048836172435,-40.1967404047062,
12.));
#139579=CARTESIAN_POINT('Ctrl Pts',(-60.4803104639226,-40.1913910800921,
0.));
#139580=CARTESIAN_POINT('Ctrl Pts',(-60.4803104639226,-40.1913910800921,
12.));
#139581=CARTESIAN_POINT('Ctrl Pts',(-60.455781386769,-40.1860268675883,
0.));
#139582=CARTESIAN_POINT('Ctrl Pts',(-60.455781386769,-40.1860268675883,
12.));
#139583=CARTESIAN_POINT('Ctrl Pts',(-60.4312964785273,-40.180647844383,
0.));
#139584=CARTESIAN_POINT('Ctrl Pts',(-60.4312964785273,-40.180647844383,
12.));
#139585=CARTESIAN_POINT('Ctrl Pts',(-60.4068558322407,-40.1752540880268,
0.));
#139586=CARTESIAN_POINT('Ctrl Pts',(-60.4068558322407,-40.1752540880268,
12.));
#139587=CARTESIAN_POINT('Ctrl Pts',(-60.3824595412446,-40.1698456764377,
0.));
#139588=CARTESIAN_POINT('Ctrl Pts',(-60.3824595412446,-40.1698456764377,
12.));
#139589=CARTESIAN_POINT('Ctrl Pts',(-60.3581076991716,-40.1644226879033,
0.));
#139590=CARTESIAN_POINT('Ctrl Pts',(-60.3581076991716,-40.1644226879033,
12.));
#139591=CARTESIAN_POINT('Ctrl Pts',(-60.3338003999607,-40.1589852010804,
0.));
#139592=CARTESIAN_POINT('Ctrl Pts',(-60.3338003999607,-40.1589852010804,
12.));
#139593=CARTESIAN_POINT('Ctrl Pts',(-60.3095377378586,-40.1535332949976,
0.));
#139594=CARTESIAN_POINT('Ctrl Pts',(-60.3095377378586,-40.1535332949976,
12.));
#139595=CARTESIAN_POINT('Ctrl Pts',(-60.285319807422,-40.1480670490585,
0.));
#139596=CARTESIAN_POINT('Ctrl Pts',(-60.285319807422,-40.1480670490585,
12.));
#139597=CARTESIAN_POINT('Ctrl Pts',(-60.2611467035117,-40.1425865430472,
0.));
#139598=CARTESIAN_POINT('Ctrl Pts',(-60.2611467035117,-40.1425865430472,
12.));
#139599=CARTESIAN_POINT('Ctrl Pts',(-60.2370185212965,-40.1370918571304,
0.));
#139600=CARTESIAN_POINT('Ctrl Pts',(-60.2370185212965,-40.1370918571304,
12.));
#139601=CARTESIAN_POINT('Ctrl Pts',(-60.2129353562622,-40.1315830718577,
0.));
#139602=CARTESIAN_POINT('Ctrl Pts',(-60.2129353562622,-40.1315830718577,
12.));
#139603=CARTESIAN_POINT('Ctrl Pts',(-60.1888973042152,-40.1260602681644,
0.));
#139604=CARTESIAN_POINT('Ctrl Pts',(-60.1888973042152,-40.1260602681644,
12.));
#139605=CARTESIAN_POINT('Ctrl Pts',(-60.1649044612828,-40.1205235273739,
0.));
#139606=CARTESIAN_POINT('Ctrl Pts',(-60.1649044612828,-40.1205235273739,
12.));
#139607=CARTESIAN_POINT('Ctrl Pts',(-60.1409569239092,-40.1149729312036,
0.));
#139608=CARTESIAN_POINT('Ctrl Pts',(-60.1409569239092,-40.1149729312036,
12.));
#139609=CARTESIAN_POINT('Ctrl Pts',(-60.1170547888574,-40.1094085617674,
0.));
#139610=CARTESIAN_POINT('Ctrl Pts',(-60.1170547888574,-40.1094085617674,
12.));
#139611=CARTESIAN_POINT('Ctrl Pts',(-60.0931981532198,-40.1038305015766,
0.));
#139612=CARTESIAN_POINT('Ctrl Pts',(-60.0931981532198,-40.1038305015766,
12.));
#139613=CARTESIAN_POINT('Ctrl Pts',(-60.069387114421,-40.0982388335423,
0.));
#139614=CARTESIAN_POINT('Ctrl Pts',(-60.069387114421,-40.0982388335423,
12.));
#139615=CARTESIAN_POINT('Ctrl Pts',(-60.0456217702202,-40.0926336409785,
0.));
#139616=CARTESIAN_POINT('Ctrl Pts',(-60.0456217702202,-40.0926336409785,
12.));
#139617=CARTESIAN_POINT('Ctrl Pts',(-60.021902218706,-40.0870150076073,
0.));
#139618=CARTESIAN_POINT('Ctrl Pts',(-60.021902218706,-40.0870150076073,
12.));
#139619=CARTESIAN_POINT('Ctrl Pts',(-59.9982285582983,-40.0813830175623,
0.));
#139620=CARTESIAN_POINT('Ctrl Pts',(-59.9982285582983,-40.0813830175623,
12.));
#139621=CARTESIAN_POINT('Ctrl Pts',(-59.9746008877584,-40.0757377553888,
0.));
#139622=CARTESIAN_POINT('Ctrl Pts',(-59.9746008877584,-40.0757377553888,
12.));
#139623=CARTESIAN_POINT('Ctrl Pts',(-59.9510193061927,-40.0700793060473,
0.));
#139624=CARTESIAN_POINT('Ctrl Pts',(-59.9510193061927,-40.0700793060473,
12.));
#139625=CARTESIAN_POINT('Ctrl Pts',(-59.9274839130553,-40.0644077549159,
0.));
#139626=CARTESIAN_POINT('Ctrl Pts',(-59.9274839130553,-40.0644077549159,
12.));
#139627=CARTESIAN_POINT('Ctrl Pts',(-59.9039948081432,-40.0587231877961,
0.));
#139628=CARTESIAN_POINT('Ctrl Pts',(-59.9039948081432,-40.0587231877961,
12.));
#139629=CARTESIAN_POINT('Ctrl Pts',(-59.8805520915975,-40.0530256909162,
0.));
#139630=CARTESIAN_POINT('Ctrl Pts',(-59.8805520915975,-40.0530256909162,
12.));
#139631=CARTESIAN_POINT('Ctrl Pts',(-59.8571558639145,-40.0473153509323,
0.));
#139632=CARTESIAN_POINT('Ctrl Pts',(-59.8571558639145,-40.0473153509323,
12.));
#139633=CARTESIAN_POINT('Ctrl Pts',(-59.8338062259491,-40.0415922549313,
0.));
#139634=CARTESIAN_POINT('Ctrl Pts',(-59.8338062259491,-40.0415922549313,
12.));
#139635=CARTESIAN_POINT('Ctrl Pts',(-59.8105032789179,-40.035856490434,
0.));
#139636=CARTESIAN_POINT('Ctrl Pts',(-59.8105032789179,-40.035856490434,
12.));
#139637=CARTESIAN_POINT('Ctrl Pts',(-59.7872471243948,-40.0301081454006,
0.));
#139638=CARTESIAN_POINT('Ctrl Pts',(-59.7872471243948,-40.0301081454006,
12.));
#139639=CARTESIAN_POINT('Ctrl Pts',(-59.7640378643115,-40.0243473082343,
0.));
#139640=CARTESIAN_POINT('Ctrl Pts',(-59.7640378643115,-40.0243473082343,
12.));
#139641=CARTESIAN_POINT('Ctrl Pts',(-59.7408756009688,-40.0185740677827,
0.));
#139642=CARTESIAN_POINT('Ctrl Pts',(-59.7408756009688,-40.0185740677827,
12.));
#139643=CARTESIAN_POINT('Ctrl Pts',(-59.7177604370409,-40.0127885133407,
0.));
#139644=CARTESIAN_POINT('Ctrl Pts',(-59.7177604370409,-40.0127885133407,
12.));
#139645=CARTESIAN_POINT('Ctrl Pts',(-59.6946924755771,-40.0069907346536,
0.));
#139646=CARTESIAN_POINT('Ctrl Pts',(-59.6946924755771,-40.0069907346536,
12.));
#139647=CARTESIAN_POINT('Ctrl Pts',(-59.671671819999,-40.001180821923,0.));
#139648=CARTESIAN_POINT('Ctrl Pts',(-59.671671819999,-40.001180821923,12.));
#139649=CARTESIAN_POINT('Ctrl Pts',(-59.6486985741015,-39.9953588658114,
0.));
#139650=CARTESIAN_POINT('Ctrl Pts',(-59.6486985741015,-39.9953588658114,
12.));
#139651=CARTESIAN_POINT('Ctrl Pts',(-59.6257728420644,-39.9895249574432,
0.));
#139652=CARTESIAN_POINT('Ctrl Pts',(-59.6257728420644,-39.9895249574432,
12.));
#139653=CARTESIAN_POINT('Ctrl Pts',(-59.6028947284551,-39.9836791884071,
0.));
#139654=CARTESIAN_POINT('Ctrl Pts',(-59.6028947284551,-39.9836791884071,
12.));
#139655=CARTESIAN_POINT('Ctrl Pts',(-59.5800643382322,-39.9778216507609,
0.));
#139656=CARTESIAN_POINT('Ctrl Pts',(-59.5800643382322,-39.9778216507609,
12.));
#139657=CARTESIAN_POINT('Ctrl Pts',(-59.5572817767412,-39.971952437036,
0.));
#139658=CARTESIAN_POINT('Ctrl Pts',(-59.5572817767412,-39.971952437036,
12.));
#139659=CARTESIAN_POINT('Ctrl Pts',(-59.5345471497162,-39.9660716402423,
0.));
#139660=CARTESIAN_POINT('Ctrl Pts',(-59.5345471497162,-39.9660716402423,
12.));
#139661=CARTESIAN_POINT('Ctrl Pts',(-59.511860563292,-39.96017935387,0.));
#139662=CARTESIAN_POINT('Ctrl Pts',(-59.511860563292,-39.96017935387,12.));
#139663=CARTESIAN_POINT('Ctrl Pts',(-59.4892221240082,-39.954275671893,
0.));
#139664=CARTESIAN_POINT('Ctrl Pts',(-59.4892221240082,-39.954275671893,
12.));
#139665=CARTESIAN_POINT('Ctrl Pts',(-59.4666319388123,-39.9483606887731,
0.));
#139666=CARTESIAN_POINT('Ctrl Pts',(-59.4666319388123,-39.9483606887731,
12.));
#139667=CARTESIAN_POINT('Ctrl Pts',(-59.444090115055,-39.9424344994652,
0.));
#139668=CARTESIAN_POINT('Ctrl Pts',(-59.444090115055,-39.9424344994652,
12.));
#139669=CARTESIAN_POINT('Ctrl Pts',(-59.4215967604925,-39.9364971994215,
0.));
#139670=CARTESIAN_POINT('Ctrl Pts',(-59.4215967604925,-39.9364971994215,
12.));
#139671=CARTESIAN_POINT('Ctrl Pts',(-59.3991519832981,-39.9305488845934,
0.));
#139672=CARTESIAN_POINT('Ctrl Pts',(-59.3991519832981,-39.9305488845934,
12.));
#139673=CARTESIAN_POINT('Ctrl Pts',(-59.3767558920663,-39.9245896514359,
0.));
#139674=CARTESIAN_POINT('Ctrl Pts',(-59.3767558920663,-39.9245896514359,
12.));
#139675=CARTESIAN_POINT('Ctrl Pts',(-59.3544085958165,-39.9186195969113,
0.));
#139676=CARTESIAN_POINT('Ctrl Pts',(-59.3544085958165,-39.9186195969113,
12.));
#139677=CARTESIAN_POINT('Ctrl Pts',(-59.3321102039883,-39.9126388184956,
0.));
#139678=CARTESIAN_POINT('Ctrl Pts',(-59.3321102039883,-39.9126388184956,
12.));
#139679=CARTESIAN_POINT('Ctrl Pts',(-59.3098608264452,-39.9066474141826,
0.));
#139680=CARTESIAN_POINT('Ctrl Pts',(-59.3098608264452,-39.9066474141826,
12.));
#139681=CARTESIAN_POINT('Ctrl Pts',(-59.2876605734871,-39.9006454824861,
0.));
#139682=CARTESIAN_POINT('Ctrl Pts',(-59.2876605734871,-39.9006454824861,
12.));
#139683=CARTESIAN_POINT('Ctrl Pts',(-59.2655095558527,-39.8946331224442,
0.));
#139684=CARTESIAN_POINT('Ctrl Pts',(-59.2655095558527,-39.8946331224442,
12.));
#139685=CARTESIAN_POINT('Ctrl Pts',(-59.2434078847236,-39.8886104336234,
0.));
#139686=CARTESIAN_POINT('Ctrl Pts',(-59.2434078847236,-39.8886104336234,
12.));
#139687=CARTESIAN_POINT('Ctrl Pts',(-59.2213556717189,-39.8825775161252,
0.));
#139688=CARTESIAN_POINT('Ctrl Pts',(-59.2213556717189,-39.8825775161252,
12.));
#139689=CARTESIAN_POINT('Ctrl Pts',(-59.1993530289008,-39.8765344705894,
0.));
#139690=CARTESIAN_POINT('Ctrl Pts',(-59.1993530289008,-39.8765344705894,
12.));
#139691=CARTESIAN_POINT('Ctrl Pts',(-59.1774000687865,-39.8704813981978,
0.));
#139692=CARTESIAN_POINT('Ctrl Pts',(-59.1774000687865,-39.8704813981978,
12.));
#139693=CARTESIAN_POINT('Ctrl Pts',(-59.155496904352,-39.8644184006785,
0.));
#139694=CARTESIAN_POINT('Ctrl Pts',(-59.155496904352,-39.8644184006785,
12.));
#139695=CARTESIAN_POINT('Ctrl Pts',(-59.133643649035,-39.8583455803111,
0.));
#139696=CARTESIAN_POINT('Ctrl Pts',(-59.133643649035,-39.8583455803111,
12.));
#139697=CARTESIAN_POINT('Ctrl Pts',(-59.1118404167304,-39.8522630399337,
0.));
#139698=CARTESIAN_POINT('Ctrl Pts',(-59.1118404167304,-39.8522630399337,
12.));
#139699=CARTESIAN_POINT('Ctrl Pts',(-59.0900873217993,-39.8461708829465,
0.));
#139700=CARTESIAN_POINT('Ctrl Pts',(-59.0900873217993,-39.8461708829465,
12.));
#139701=CARTESIAN_POINT('Ctrl Pts',(-59.068384479077,-39.8400692133143,
0.));
#139702=CARTESIAN_POINT('Ctrl Pts',(-59.068384479077,-39.8400692133143,
12.));
#139703=CARTESIAN_POINT('Ctrl Pts',(-59.0467320038783,-39.8339581355714,
0.));
#139704=CARTESIAN_POINT('Ctrl Pts',(-59.0467320038783,-39.8339581355714,
12.));
#139705=CARTESIAN_POINT('Ctrl Pts',(-59.0251300119973,-39.8278377548261,
0.));
#139706=CARTESIAN_POINT('Ctrl Pts',(-59.0251300119973,-39.8278377548261,
12.));
#139707=CARTESIAN_POINT('Ctrl Pts',(-59.0035786197024,-39.8217081767658,
0.));
#139708=CARTESIAN_POINT('Ctrl Pts',(-59.0035786197024,-39.8217081767658,
12.));
#139709=CARTESIAN_POINT('Ctrl Pts',(-58.9820779437485,-39.8155695076624,
0.));
#139710=CARTESIAN_POINT('Ctrl Pts',(-58.9820779437485,-39.8155695076624,
12.));
#139711=CARTESIAN_POINT('Ctrl Pts',(-58.9606281013876,-39.8094218543781,
0.));
#139712=CARTESIAN_POINT('Ctrl Pts',(-58.9606281013876,-39.8094218543781,
12.));
#139713=CARTESIAN_POINT('Ctrl Pts',(-58.9392292103747,-39.8032653243712,
0.));
#139714=CARTESIAN_POINT('Ctrl Pts',(-58.9392292103747,-39.8032653243712,
12.));
#139715=CARTESIAN_POINT('Ctrl Pts',(-58.9178813889703,-39.7971000257044,
0.));
#139716=CARTESIAN_POINT('Ctrl Pts',(-58.9178813889703,-39.7971000257044,
12.));
#139717=CARTESIAN_POINT('Ctrl Pts',(-58.896584755939,-39.7909260670517,
0.));
#139718=CARTESIAN_POINT('Ctrl Pts',(-58.896584755939,-39.7909260670517,
12.));
#139719=CARTESIAN_POINT('Ctrl Pts',(-58.8753394305583,-39.7847435576995,
0.));
#139720=CARTESIAN_POINT('Ctrl Pts',(-58.8753394305583,-39.7847435576995,
12.));
#139721=CARTESIAN_POINT('Ctrl Pts',(-58.8541455326229,-39.7785526075477,
0.));
#139722=CARTESIAN_POINT('Ctrl Pts',(-58.8541455326229,-39.7785526075477,
12.));
#139723=CARTESIAN_POINT('Ctrl Pts',(-58.8330031824453,-39.772353327112,
0.));
#139724=CARTESIAN_POINT('Ctrl Pts',(-58.8330031824453,-39.772353327112,
12.));
#139725=CARTESIAN_POINT('Ctrl Pts',(-58.8119125008521,-39.7661458275276,
0.));
#139726=CARTESIAN_POINT('Ctrl Pts',(-58.8119125008521,-39.7661458275276,
12.));
#139727=CARTESIAN_POINT('Ctrl Pts',(-58.7908736091808,-39.7599302205527,
0.));
#139728=CARTESIAN_POINT('Ctrl Pts',(-58.7908736091808,-39.7599302205527,
12.));
#139729=CARTESIAN_POINT('Ctrl Pts',(-58.7698866293041,-39.753706618582,
0.));
#139730=CARTESIAN_POINT('Ctrl Pts',(-58.7698866293041,-39.753706618582,
12.));
#139731=CARTESIAN_POINT('Ctrl Pts',(-58.7489516836453,-39.7474751346603,
0.));
#139732=CARTESIAN_POINT('Ctrl Pts',(-58.7489516836453,-39.7474751346603,
12.));
#139733=CARTESIAN_POINT('Ctrl Pts',(-58.7280688951911,-39.7412358824949,
0.));
#139734=CARTESIAN_POINT('Ctrl Pts',(-58.7280688951911,-39.7412358824949,
12.));
#139735=CARTESIAN_POINT('Ctrl Pts',(-58.7072383875009,-39.7349889764737,
0.));
#139736=CARTESIAN_POINT('Ctrl Pts',(-58.7072383875009,-39.7349889764737,
12.));
#139737=CARTESIAN_POINT('Ctrl Pts',(-58.6864602847065,-39.7287345316664,
0.));
#139738=CARTESIAN_POINT('Ctrl Pts',(-58.6864602847065,-39.7287345316664,
12.));
#139739=CARTESIAN_POINT('Ctrl Pts',(-58.6657347115015,-39.7224726638087,
0.));
#139740=CARTESIAN_POINT('Ctrl Pts',(-58.6657347115015,-39.7224726638087,
12.));
#139741=CARTESIAN_POINT('Ctrl Pts',(-58.6450617931269,-39.7162034892896,
0.));
#139742=CARTESIAN_POINT('Ctrl Pts',(-58.6450617931269,-39.7162034892896,
12.));
#139743=CARTESIAN_POINT('Ctrl Pts',(-58.6244416553574,-39.7099271251421,
0.));
#139744=CARTESIAN_POINT('Ctrl Pts',(-58.6244416553574,-39.7099271251421,
12.));
#139745=CARTESIAN_POINT('Ctrl Pts',(-58.6038744244683,-39.7036436890248,
0.));
#139746=CARTESIAN_POINT('Ctrl Pts',(-58.6038744244683,-39.7036436890248,
12.));
#139747=CARTESIAN_POINT('Ctrl Pts',(-58.5833602272767,-39.6973532992555,
0.));
#139748=CARTESIAN_POINT('Ctrl Pts',(-58.5833602272767,-39.6973532992555,
12.));
#139749=CARTESIAN_POINT('Ctrl Pts',(-58.5628991912067,-39.6910560748639,
0.));
#139750=CARTESIAN_POINT('Ctrl Pts',(-58.5628991912067,-39.6910560748639,
12.));
#139751=CARTESIAN_POINT('Ctrl Pts',(-58.5424914443415,-39.6847521356395,
0.));
#139752=CARTESIAN_POINT('Ctrl Pts',(-58.5424914443415,-39.6847521356395,
12.));
#139753=CARTESIAN_POINT('Ctrl Pts',(-58.5221371154748,-39.6784416021817,
0.));
#139754=CARTESIAN_POINT('Ctrl Pts',(-58.5221371154748,-39.6784416021817,
12.));
#139755=CARTESIAN_POINT('Ctrl Pts',(-58.5018363341582,-39.6721245959516,
0.));
#139756=CARTESIAN_POINT('Ctrl Pts',(-58.5018363341582,-39.6721245959516,
12.));
#139757=CARTESIAN_POINT('Ctrl Pts',(-58.4815892306044,-39.66580123918,0.));
#139758=CARTESIAN_POINT('Ctrl Pts',(-58.4815892306044,-39.66580123918,12.));
#139759=CARTESIAN_POINT('Ctrl Pts',(-58.4613959355776,-39.659471654768,
0.));
#139760=CARTESIAN_POINT('Ctrl Pts',(-58.4613959355776,-39.659471654768,
12.));
#139761=CARTESIAN_POINT('Ctrl Pts',(-58.4412565802984,-39.6531359662043,
0.));
#139762=CARTESIAN_POINT('Ctrl Pts',(-58.4412565802984,-39.6531359662043,
12.));
#139763=CARTESIAN_POINT('Ctrl Pts',(-58.4211712963024,-39.6467942974464,
0.));
#139764=CARTESIAN_POINT('Ctrl Pts',(-58.4211712963024,-39.6467942974464,
12.));
#139765=CARTESIAN_POINT('Ctrl Pts',(-58.4011402154225,-39.6404467729113,
0.));
#139766=CARTESIAN_POINT('Ctrl Pts',(-58.4011402154225,-39.6404467729113,
12.));
#139767=CARTESIAN_POINT('Ctrl Pts',(-58.3811634701061,-39.6340935177492,
0.));
#139768=CARTESIAN_POINT('Ctrl Pts',(-58.3811634701061,-39.6340935177492,
12.));
#139769=CARTESIAN_POINT('Ctrl Pts',(-58.3612411936914,-39.6277346580898,
0.));
#139770=CARTESIAN_POINT('Ctrl Pts',(-58.3612411936914,-39.6277346580898,
12.));
#139771=CARTESIAN_POINT('Ctrl Pts',(-58.3413735206412,-39.6213703212522,
0.));
#139772=CARTESIAN_POINT('Ctrl Pts',(-58.3413735206412,-39.6213703212522,
12.));
#139773=CARTESIAN_POINT('Ctrl Pts',(-58.3215605869192,-39.6150006360894,
0.));
#139774=CARTESIAN_POINT('Ctrl Pts',(-58.3215605869192,-39.6150006360894,
12.));
#139775=CARTESIAN_POINT('Ctrl Pts',(-58.3018025297288,-39.6086257327559,
0.));
#139776=CARTESIAN_POINT('Ctrl Pts',(-58.3018025297288,-39.6086257327559,
12.));
#139777=CARTESIAN_POINT('Ctrl Pts',(-58.2820994868092,-39.6022457420772,
0.));
#139778=CARTESIAN_POINT('Ctrl Pts',(-58.2820994868092,-39.6022457420772,
12.));
#139779=CARTESIAN_POINT('Ctrl Pts',(-58.2624515958416,-39.5958607950237,
0.));
#139780=CARTESIAN_POINT('Ctrl Pts',(-58.2624515958416,-39.5958607950237,
12.));
#139781=CARTESIAN_POINT('Ctrl Pts',(-58.2428589938395,-39.5894710221729,
0.));
#139782=CARTESIAN_POINT('Ctrl Pts',(-58.2428589938395,-39.5894710221729,
12.));
#139783=CARTESIAN_POINT('Ctrl Pts',(-58.2233218164408,-39.5830765530919,
0.));
#139784=CARTESIAN_POINT('Ctrl Pts',(-58.2233218164408,-39.5830765530919,
12.));
#139785=CARTESIAN_POINT('Ctrl Pts',(-58.2038401992496,-39.5766775175226,
0.));
#139786=CARTESIAN_POINT('Ctrl Pts',(-58.2038401992496,-39.5766775175226,
12.));
#139787=CARTESIAN_POINT('Ctrl Pts',(-58.1844142794359,-39.5702740468013,
0.));
#139788=CARTESIAN_POINT('Ctrl Pts',(-58.1844142794359,-39.5702740468013,
12.));
#139789=CARTESIAN_POINT('Ctrl Pts',(-58.1650441970379,-39.5638662750174,
0.));
#139790=CARTESIAN_POINT('Ctrl Pts',(-58.1650441970379,-39.5638662750174,
12.));
#139791=CARTESIAN_POINT('Ctrl Pts',(-58.1457300968467,-39.5574543406959,
0.));
#139792=CARTESIAN_POINT('Ctrl Pts',(-58.1457300968467,-39.5574543406959,
12.));
#139793=CARTESIAN_POINT('Ctrl Pts',(-58.1264721285698,-39.5510383869476,
0.));
#139794=CARTESIAN_POINT('Ctrl Pts',(-58.1264721285698,-39.5510383869476,
12.));
#139795=CARTESIAN_POINT('Ctrl Pts',(-58.1072704428895,-39.5446185579615,
0.));
#139796=CARTESIAN_POINT('Ctrl Pts',(-58.1072704428895,-39.5446185579615,
12.));
#139797=CARTESIAN_POINT('Ctrl Pts',(-58.0881251879911,-39.5381949959214,
0.));
#139798=CARTESIAN_POINT('Ctrl Pts',(-58.0881251879911,-39.5381949959214,
12.));
#139799=CARTESIAN_POINT('Ctrl Pts',(-58.0690365065393,-39.5317678383231,
0.));
#139800=CARTESIAN_POINT('Ctrl Pts',(-58.0690365065393,-39.5317678383231,
12.));
#139801=CARTESIAN_POINT('Ctrl Pts',(-58.050004530846,-39.5253372136921,
0.));
#139802=CARTESIAN_POINT('Ctrl Pts',(-58.050004530846,-39.5253372136921,
12.));
#139803=CARTESIAN_POINT('Ctrl Pts',(-58.0310293875321,-39.5189032457227,
0.));
#139804=CARTESIAN_POINT('Ctrl Pts',(-58.0310293875321,-39.5189032457227,
12.));
#139805=CARTESIAN_POINT('Ctrl Pts',(-58.012111206794,-39.5124660615009,
0.));
#139806=CARTESIAN_POINT('Ctrl Pts',(-58.012111206794,-39.5124660615009,
12.));
#139807=CARTESIAN_POINT('Ctrl Pts',(-57.9932501298522,-39.5060257981225,
0.));
#139808=CARTESIAN_POINT('Ctrl Pts',(-57.9932501298522,-39.5060257981225,
12.));
#139809=CARTESIAN_POINT('Ctrl Pts',(-57.9744463179305,-39.4995826106691,
0.));
#139810=CARTESIAN_POINT('Ctrl Pts',(-57.9744463179305,-39.4995826106691,
12.));
#139811=CARTESIAN_POINT('Ctrl Pts',(-57.9556999583777,-39.4931366776627,
0.));
#139812=CARTESIAN_POINT('Ctrl Pts',(-57.9556999583777,-39.4931366776627,
12.));
#139813=CARTESIAN_POINT('Ctrl Pts',(-57.9370112456506,-39.4866881842223,
0.));
#139814=CARTESIAN_POINT('Ctrl Pts',(-57.9370112456506,-39.4866881842223,
12.));
#139815=CARTESIAN_POINT('Ctrl Pts',(-57.9183803632337,-39.4802373061008,
0.));
#139816=CARTESIAN_POINT('Ctrl Pts',(-57.9183803632337,-39.4802373061008,
12.));
#139817=CARTESIAN_POINT('Ctrl Pts',(-57.8998074670541,-39.4737841949417,
0.));
#139818=CARTESIAN_POINT('Ctrl Pts',(-57.8998074670541,-39.4737841949417,
12.));
#139819=CARTESIAN_POINT('Ctrl Pts',(-57.8812926637397,-39.4673289592425,
0.));
#139820=CARTESIAN_POINT('Ctrl Pts',(-57.8812926637397,-39.4673289592425,
12.));
#139821=CARTESIAN_POINT('Ctrl Pts',(-57.8628360097134,-39.4608716627367,
0.));
#139822=CARTESIAN_POINT('Ctrl Pts',(-57.8628360097134,-39.4608716627367,
12.));
#139823=CARTESIAN_POINT('Ctrl Pts',(-57.8481172247805,-39.4557042029884,
0.));
#139824=CARTESIAN_POINT('Ctrl Pts',(-57.8481172247805,-39.4557042029884,
12.));
#139825=CARTESIAN_POINT('Ctrl Pts',(-57.8371043151607,-39.45182770037,0.));
#139826=CARTESIAN_POINT('Ctrl Pts',(-57.8371043151607,-39.45182770037,12.));
#139827=CARTESIAN_POINT('Ctrl Pts',(-57.829774010102,-39.4492429618498,
0.));
#139828=CARTESIAN_POINT('Ctrl Pts',(-57.829774010102,-39.4492429618498,
12.));
#139829=CARTESIAN_POINT('Ctrl Pts',(-57.8261117662439,-39.4479504917286,
0.));
#139830=CARTESIAN_POINT('Ctrl Pts',(-57.8261117662439,-39.4479504917286,
12.));
#139831=CARTESIAN_POINT('',(-57.8261117662439,-39.4479504917286,12.));
#139832=CARTESIAN_POINT('Ctrl Pts',(-57.8261117662439,-39.4479504917286,
12.));
#139833=CARTESIAN_POINT('Ctrl Pts',(-57.829774010102,-39.4492429618498,
12.));
#139834=CARTESIAN_POINT('Ctrl Pts',(-57.8371043151607,-39.45182770037,12.));
#139835=CARTESIAN_POINT('Ctrl Pts',(-57.8481172247805,-39.4557042029884,
12.));
#139836=CARTESIAN_POINT('Ctrl Pts',(-57.8628360097134,-39.4608716627367,
12.));
#139837=CARTESIAN_POINT('Ctrl Pts',(-57.8812926637397,-39.4673289592425,
12.));
#139838=CARTESIAN_POINT('Ctrl Pts',(-57.8998074670541,-39.4737841949417,
12.));
#139839=CARTESIAN_POINT('Ctrl Pts',(-57.9183803632337,-39.4802373061008,
12.));
#139840=CARTESIAN_POINT('Ctrl Pts',(-57.9370112456506,-39.4866881842223,
12.));
#139841=CARTESIAN_POINT('Ctrl Pts',(-57.9556999583777,-39.4931366776627,
12.));
#139842=CARTESIAN_POINT('Ctrl Pts',(-57.9744463179305,-39.4995826106691,
12.));
#139843=CARTESIAN_POINT('Ctrl Pts',(-57.9932501298522,-39.5060257981225,
12.));
#139844=CARTESIAN_POINT('Ctrl Pts',(-58.012111206794,-39.5124660615009,
12.));
#139845=CARTESIAN_POINT('Ctrl Pts',(-58.0310293875321,-39.5189032457227,
12.));
#139846=CARTESIAN_POINT('Ctrl Pts',(-58.050004530846,-39.5253372136921,
12.));
#139847=CARTESIAN_POINT('Ctrl Pts',(-58.0690365065393,-39.5317678383231,
12.));
#139848=CARTESIAN_POINT('Ctrl Pts',(-58.0881251879911,-39.5381949959214,
12.));
#139849=CARTESIAN_POINT('Ctrl Pts',(-58.1072704428895,-39.5446185579615,
12.));
#139850=CARTESIAN_POINT('Ctrl Pts',(-58.1264721285698,-39.5510383869476,
12.));
#139851=CARTESIAN_POINT('Ctrl Pts',(-58.1457300968467,-39.5574543406959,
12.));
#139852=CARTESIAN_POINT('Ctrl Pts',(-58.1650441970379,-39.5638662750174,
12.));
#139853=CARTESIAN_POINT('Ctrl Pts',(-58.1844142794359,-39.5702740468013,
12.));
#139854=CARTESIAN_POINT('Ctrl Pts',(-58.2038401992496,-39.5766775175226,
12.));
#139855=CARTESIAN_POINT('Ctrl Pts',(-58.2233218164408,-39.5830765530919,
12.));
#139856=CARTESIAN_POINT('Ctrl Pts',(-58.2428589938395,-39.5894710221729,
12.));
#139857=CARTESIAN_POINT('Ctrl Pts',(-58.2624515958416,-39.5958607950237,
12.));
#139858=CARTESIAN_POINT('Ctrl Pts',(-58.2820994868092,-39.6022457420772,
12.));
#139859=CARTESIAN_POINT('Ctrl Pts',(-58.3018025297288,-39.6086257327559,
12.));
#139860=CARTESIAN_POINT('Ctrl Pts',(-58.3215605869192,-39.6150006360894,
12.));
#139861=CARTESIAN_POINT('Ctrl Pts',(-58.3413735206412,-39.6213703212522,
12.));
#139862=CARTESIAN_POINT('Ctrl Pts',(-58.3612411936914,-39.6277346580898,
12.));
#139863=CARTESIAN_POINT('Ctrl Pts',(-58.3811634701061,-39.6340935177492,
12.));
#139864=CARTESIAN_POINT('Ctrl Pts',(-58.4011402154225,-39.6404467729113,
12.));
#139865=CARTESIAN_POINT('Ctrl Pts',(-58.4211712963024,-39.6467942974464,
12.));
#139866=CARTESIAN_POINT('Ctrl Pts',(-58.4412565802984,-39.6531359662043,
12.));
#139867=CARTESIAN_POINT('Ctrl Pts',(-58.4613959355776,-39.659471654768,
12.));
#139868=CARTESIAN_POINT('Ctrl Pts',(-58.4815892306044,-39.66580123918,12.));
#139869=CARTESIAN_POINT('Ctrl Pts',(-58.5018363341582,-39.6721245959516,
12.));
#139870=CARTESIAN_POINT('Ctrl Pts',(-58.5221371154748,-39.6784416021817,
12.));
#139871=CARTESIAN_POINT('Ctrl Pts',(-58.5424914443415,-39.6847521356395,
12.));
#139872=CARTESIAN_POINT('Ctrl Pts',(-58.5628991912067,-39.6910560748639,
12.));
#139873=CARTESIAN_POINT('Ctrl Pts',(-58.5833602272767,-39.6973532992555,
12.));
#139874=CARTESIAN_POINT('Ctrl Pts',(-58.6038744244683,-39.7036436890248,
12.));
#139875=CARTESIAN_POINT('Ctrl Pts',(-58.6244416553574,-39.7099271251421,
12.));
#139876=CARTESIAN_POINT('Ctrl Pts',(-58.6450617931269,-39.7162034892896,
12.));
#139877=CARTESIAN_POINT('Ctrl Pts',(-58.6657347115015,-39.7224726638087,
12.));
#139878=CARTESIAN_POINT('Ctrl Pts',(-58.6864602847065,-39.7287345316664,
12.));
#139879=CARTESIAN_POINT('Ctrl Pts',(-58.7072383875009,-39.7349889764737,
12.));
#139880=CARTESIAN_POINT('Ctrl Pts',(-58.7280688951911,-39.7412358824949,
12.));
#139881=CARTESIAN_POINT('Ctrl Pts',(-58.7489516836453,-39.7474751346603,
12.));
#139882=CARTESIAN_POINT('Ctrl Pts',(-58.7698866293041,-39.753706618582,
12.));
#139883=CARTESIAN_POINT('Ctrl Pts',(-58.7908736091808,-39.7599302205527,
12.));
#139884=CARTESIAN_POINT('Ctrl Pts',(-58.8119125008521,-39.7661458275276,
12.));
#139885=CARTESIAN_POINT('Ctrl Pts',(-58.8330031824453,-39.772353327112,
12.));
#139886=CARTESIAN_POINT('Ctrl Pts',(-58.8541455326229,-39.7785526075477,
12.));
#139887=CARTESIAN_POINT('Ctrl Pts',(-58.8753394305583,-39.7847435576995,
12.));
#139888=CARTESIAN_POINT('Ctrl Pts',(-58.896584755939,-39.7909260670517,
12.));
#139889=CARTESIAN_POINT('Ctrl Pts',(-58.9178813889703,-39.7971000257044,
12.));
#139890=CARTESIAN_POINT('Ctrl Pts',(-58.9392292103747,-39.8032653243712,
12.));
#139891=CARTESIAN_POINT('Ctrl Pts',(-58.9606281013876,-39.8094218543781,
12.));
#139892=CARTESIAN_POINT('Ctrl Pts',(-58.9820779437485,-39.8155695076624,
12.));
#139893=CARTESIAN_POINT('Ctrl Pts',(-59.0035786197024,-39.8217081767658,
12.));
#139894=CARTESIAN_POINT('Ctrl Pts',(-59.0251300119973,-39.8278377548261,
12.));
#139895=CARTESIAN_POINT('Ctrl Pts',(-59.0467320038783,-39.8339581355714,
12.));
#139896=CARTESIAN_POINT('Ctrl Pts',(-59.068384479077,-39.8400692133143,
12.));
#139897=CARTESIAN_POINT('Ctrl Pts',(-59.0900873217993,-39.8461708829465,
12.));
#139898=CARTESIAN_POINT('Ctrl Pts',(-59.1118404167304,-39.8522630399337,
12.));
#139899=CARTESIAN_POINT('Ctrl Pts',(-59.133643649035,-39.8583455803111,
12.));
#139900=CARTESIAN_POINT('Ctrl Pts',(-59.155496904352,-39.8644184006785,
12.));
#139901=CARTESIAN_POINT('Ctrl Pts',(-59.1774000687865,-39.8704813981978,
12.));
#139902=CARTESIAN_POINT('Ctrl Pts',(-59.1993530289008,-39.8765344705894,
12.));
#139903=CARTESIAN_POINT('Ctrl Pts',(-59.2213556717189,-39.8825775161252,
12.));
#139904=CARTESIAN_POINT('Ctrl Pts',(-59.2434078847236,-39.8886104336234,
12.));
#139905=CARTESIAN_POINT('Ctrl Pts',(-59.2655095558527,-39.8946331224442,
12.));
#139906=CARTESIAN_POINT('Ctrl Pts',(-59.2876605734871,-39.9006454824861,
12.));
#139907=CARTESIAN_POINT('Ctrl Pts',(-59.3098608264452,-39.9066474141826,
12.));
#139908=CARTESIAN_POINT('Ctrl Pts',(-59.3321102039883,-39.9126388184956,
12.));
#139909=CARTESIAN_POINT('Ctrl Pts',(-59.3544085958165,-39.9186195969113,
12.));
#139910=CARTESIAN_POINT('Ctrl Pts',(-59.3767558920663,-39.9245896514359,
12.));
#139911=CARTESIAN_POINT('Ctrl Pts',(-59.3991519832981,-39.9305488845934,
12.));
#139912=CARTESIAN_POINT('Ctrl Pts',(-59.4215967604925,-39.9364971994215,
12.));
#139913=CARTESIAN_POINT('Ctrl Pts',(-59.444090115055,-39.9424344994652,
12.));
#139914=CARTESIAN_POINT('Ctrl Pts',(-59.4666319388123,-39.9483606887731,
12.));
#139915=CARTESIAN_POINT('Ctrl Pts',(-59.4892221240082,-39.954275671893,
12.));
#139916=CARTESIAN_POINT('Ctrl Pts',(-59.511860563292,-39.96017935387,12.));
#139917=CARTESIAN_POINT('Ctrl Pts',(-59.5345471497162,-39.9660716402423,
12.));
#139918=CARTESIAN_POINT('Ctrl Pts',(-59.5572817767412,-39.971952437036,
12.));
#139919=CARTESIAN_POINT('Ctrl Pts',(-59.5800643382322,-39.9778216507609,
12.));
#139920=CARTESIAN_POINT('Ctrl Pts',(-59.6028947284551,-39.9836791884071,
12.));
#139921=CARTESIAN_POINT('Ctrl Pts',(-59.6257728420644,-39.9895249574432,
12.));
#139922=CARTESIAN_POINT('Ctrl Pts',(-59.6486985741015,-39.9953588658114,
12.));
#139923=CARTESIAN_POINT('Ctrl Pts',(-59.671671819999,-40.001180821923,12.));
#139924=CARTESIAN_POINT('Ctrl Pts',(-59.6946924755771,-40.0069907346536,
12.));
#139925=CARTESIAN_POINT('Ctrl Pts',(-59.7177604370409,-40.0127885133407,
12.));
#139926=CARTESIAN_POINT('Ctrl Pts',(-59.7408756009688,-40.0185740677827,
12.));
#139927=CARTESIAN_POINT('Ctrl Pts',(-59.7640378643115,-40.0243473082343,
12.));
#139928=CARTESIAN_POINT('Ctrl Pts',(-59.7872471243948,-40.0301081454006,
12.));
#139929=CARTESIAN_POINT('Ctrl Pts',(-59.8105032789179,-40.035856490434,
12.));
#139930=CARTESIAN_POINT('Ctrl Pts',(-59.8338062259491,-40.0415922549313,
12.));
#139931=CARTESIAN_POINT('Ctrl Pts',(-59.8571558639145,-40.0473153509323,
12.));
#139932=CARTESIAN_POINT('Ctrl Pts',(-59.8805520915975,-40.0530256909162,
12.));
#139933=CARTESIAN_POINT('Ctrl Pts',(-59.9039948081432,-40.0587231877961,
12.));
#139934=CARTESIAN_POINT('Ctrl Pts',(-59.9274839130553,-40.0644077549159,
12.));
#139935=CARTESIAN_POINT('Ctrl Pts',(-59.9510193061927,-40.0700793060473,
12.));
#139936=CARTESIAN_POINT('Ctrl Pts',(-59.9746008877584,-40.0757377553888,
12.));
#139937=CARTESIAN_POINT('Ctrl Pts',(-59.9982285582983,-40.0813830175623,
12.));
#139938=CARTESIAN_POINT('Ctrl Pts',(-60.021902218706,-40.0870150076073,
12.));
#139939=CARTESIAN_POINT('Ctrl Pts',(-60.0456217702202,-40.0926336409785,
12.));
#139940=CARTESIAN_POINT('Ctrl Pts',(-60.069387114421,-40.0982388335423,
12.));
#139941=CARTESIAN_POINT('Ctrl Pts',(-60.0931981532198,-40.1038305015766,
12.));
#139942=CARTESIAN_POINT('Ctrl Pts',(-60.1170547888574,-40.1094085617674,
12.));
#139943=CARTESIAN_POINT('Ctrl Pts',(-60.1409569239092,-40.1149729312036,
12.));
#139944=CARTESIAN_POINT('Ctrl Pts',(-60.1649044612828,-40.1205235273739,
12.));
#139945=CARTESIAN_POINT('Ctrl Pts',(-60.1888973042152,-40.1260602681644,
12.));
#139946=CARTESIAN_POINT('Ctrl Pts',(-60.2129353562622,-40.1315830718577,
12.));
#139947=CARTESIAN_POINT('Ctrl Pts',(-60.2370185212965,-40.1370918571304,
12.));
#139948=CARTESIAN_POINT('Ctrl Pts',(-60.2611467035117,-40.1425865430472,
12.));
#139949=CARTESIAN_POINT('Ctrl Pts',(-60.285319807422,-40.1480670490585,
12.));
#139950=CARTESIAN_POINT('Ctrl Pts',(-60.3095377378586,-40.1535332949976,
12.));
#139951=CARTESIAN_POINT('Ctrl Pts',(-60.3338003999607,-40.1589852010804,
12.));
#139952=CARTESIAN_POINT('Ctrl Pts',(-60.3581076991716,-40.1644226879033,
12.));
#139953=CARTESIAN_POINT('Ctrl Pts',(-60.3824595412446,-40.1698456764377,
12.));
#139954=CARTESIAN_POINT('Ctrl Pts',(-60.4068558322407,-40.1752540880268,
12.));
#139955=CARTESIAN_POINT('Ctrl Pts',(-60.4312964785273,-40.180647844383,
12.));
#139956=CARTESIAN_POINT('Ctrl Pts',(-60.455781386769,-40.1860268675883,
12.));
#139957=CARTESIAN_POINT('Ctrl Pts',(-60.4803104639226,-40.1913910800921,
12.));
#139958=CARTESIAN_POINT('Ctrl Pts',(-60.5048836172435,-40.1967404047062,
12.));
#139959=CARTESIAN_POINT('Ctrl Pts',(-60.5295007542841,-40.2020747646014,
12.));
#139960=CARTESIAN_POINT('Ctrl Pts',(-60.5541617828925,-40.2073940833052,
12.));
#139961=CARTESIAN_POINT('Ctrl Pts',(-60.5788666112042,-40.2126982847011,
12.));
#139962=CARTESIAN_POINT('Ctrl Pts',(-60.6036151476349,-40.2179872930273,
12.));
#139963=CARTESIAN_POINT('Ctrl Pts',(-60.6284073008871,-40.2232610328721,
12.));
#139964=CARTESIAN_POINT('Ctrl Pts',(-60.6532429799499,-40.2285194291706,
12.));
#139965=CARTESIAN_POINT('Ctrl Pts',(-60.678122094098,-40.2337624072028,
12.));
#139966=CARTESIAN_POINT('Ctrl Pts',(-60.7030445528857,-40.2389898925932,
12.));
#139967=CARTESIAN_POINT('Ctrl Pts',(-60.728010266139,-40.2442018113108,
12.));
#139968=CARTESIAN_POINT('Ctrl Pts',(-60.7530191439593,-40.2493980896638,
12.));
#139969=CARTESIAN_POINT('Ctrl Pts',(-60.7780710967248,-40.2545786542953,
12.));
#139970=CARTESIAN_POINT('Ctrl Pts',(-60.8031660350879,-40.2597434321803,
12.));
#139971=CARTESIAN_POINT('Ctrl Pts',(-60.8283038699706,-40.2648923506248,
12.));
#139972=CARTESIAN_POINT('Ctrl Pts',(-60.8534845125538,-40.2700253372647,
12.));
#139973=CARTESIAN_POINT('Ctrl Pts',(-60.8787078742818,-40.2751423200639,
12.));
#139974=CARTESIAN_POINT('Ctrl Pts',(-60.9039738668669,-40.2802432273104,
12.));
#139975=CARTESIAN_POINT('Ctrl Pts',(-60.9292824022887,-40.2853279876161,
12.));
#139976=CARTESIAN_POINT('Ctrl Pts',(-60.9546333927921,-40.2903965299155,
12.));
#139977=CARTESIAN_POINT('Ctrl Pts',(-60.9800267508787,-40.295448783469,
12.));
#139978=CARTESIAN_POINT('Ctrl Pts',(-61.0054623893066,-40.300484677858,
12.));
#139979=CARTESIAN_POINT('Ctrl Pts',(-61.0309402210921,-40.3055041429775,
12.));
#139980=CARTESIAN_POINT('Ctrl Pts',(-61.056460159505,-40.3105071090309,
12.));
#139981=CARTESIAN_POINT('Ctrl Pts',(-61.0820221180645,-40.3154935065262,
12.));
#139982=CARTESIAN_POINT('Ctrl Pts',(-61.1076260105258,-40.3204632662725,
12.));
#139983=CARTESIAN_POINT('Ctrl Pts',(-61.1332717508789,-40.32541631938,12.));
#139984=CARTESIAN_POINT('Ctrl Pts',(-61.1589592533613,-40.3303525972615,
12.));
#139985=CARTESIAN_POINT('Ctrl Pts',(-61.1846884324644,-40.335272031637,
12.));
#139986=CARTESIAN_POINT('Ctrl Pts',(-61.2104592029377,-40.340174554537,
12.));
#139987=CARTESIAN_POINT('Ctrl Pts',(-61.23627147979,-40.3450600983109,12.));
#139988=CARTESIAN_POINT('Ctrl Pts',(-61.2621251782863,-40.3499285956304,
12.));
#139989=CARTESIAN_POINT('Ctrl Pts',(-61.2880202139371,-40.3547799794679,
12.));
#139990=CARTESIAN_POINT('Ctrl Pts',(-61.3139565024847,-40.3596141830791,
12.));
#139991=CARTESIAN_POINT('Ctrl Pts',(-61.3399339598853,-40.3644311399861,
12.));
#139992=CARTESIAN_POINT('Ctrl Pts',(-61.3659525022908,-40.3692307839636,
12.));
#139993=CARTESIAN_POINT('Ctrl Pts',(-61.3920120460219,-40.3740130490225,
12.));
#139994=CARTESIAN_POINT('Ctrl Pts',(-61.4181125076037,-40.3787778694364,
12.));
#139995=CARTESIAN_POINT('Ctrl Pts',(-61.4442538038044,-40.383525179772,
12.));
#139996=CARTESIAN_POINT('Ctrl Pts',(-61.4704358516709,-40.3882549149227,
12.));
#139997=CARTESIAN_POINT('Ctrl Pts',(-61.4966585685549,-40.3929670101365,
12.));
#139998=CARTESIAN_POINT('Ctrl Pts',(-61.522921872154,-40.3976614010652,
12.));
#139999=CARTESIAN_POINT('Ctrl Pts',(-61.5492256804717,-40.4023380237232,
12.));
#140000=CARTESIAN_POINT('Ctrl Pts',(-61.5755699117324,-40.4069968143956,
12.));
#140001=CARTESIAN_POINT('Ctrl Pts',(-61.6019544843011,-40.4116377095596,
12.));
#140002=CARTESIAN_POINT('Ctrl Pts',(-61.628379316608,-40.4162606458118,
12.));
#140003=CARTESIAN_POINT('Ctrl Pts',(-61.6548443270394,-40.4208655597717,
12.));
#140004=CARTESIAN_POINT('Ctrl Pts',(-61.6813494339286,-40.425452388076,
12.));
#140005=CARTESIAN_POINT('Ctrl Pts',(-61.7078945557799,-40.430021067584,
12.));
#140006=CARTESIAN_POINT('Ctrl Pts',(-61.7344796114399,-40.4345715355404,
12.));
#140007=CARTESIAN_POINT('Ctrl Pts',(-61.7611045202874,-40.4391037297588,
12.));
#140008=CARTESIAN_POINT('Ctrl Pts',(-61.7877692024076,-40.4436175887949,
12.));
#140009=CARTESIAN_POINT('Ctrl Pts',(-61.814473578779,-40.4481130521364,
12.));
#140010=CARTESIAN_POINT('Ctrl Pts',(-61.8412175708553,-40.4525900597894,
12.));
#140011=CARTESIAN_POINT('Ctrl Pts',(-61.8680011001537,-40.4570485518749,
12.));
#140012=CARTESIAN_POINT('Ctrl Pts',(-61.8948240878008,-40.4614884681889,
12.));
#140013=CARTESIAN_POINT('Ctrl Pts',(-61.9216864541744,-40.4659097478587,
12.));
#140014=CARTESIAN_POINT('Ctrl Pts',(-61.9485881182921,-40.470312328762,
12.));
#140015=CARTESIAN_POINT('Ctrl Pts',(-61.9755289983044,-40.4746961480015,
12.));
#140016=CARTESIAN_POINT('Ctrl Pts',(-62.0025090125959,-40.4790611429583,
12.));
#140017=CARTESIAN_POINT('Ctrl Pts',(-62.029528080742,-40.4834072522164,
12.));
#140018=CARTESIAN_POINT('Ctrl Pts',(-62.0565861244179,-40.4877344164411,
12.));
#140019=CARTESIAN_POINT('Ctrl Pts',(-62.083683068572,-40.4920425795216,
12.));
#140020=CARTESIAN_POINT('Ctrl Pts',(-62.1108188417004,-40.4963316888412,
12.));
#140021=CARTESIAN_POINT('Ctrl Pts',(-62.1341126810543,-40.4999919096264,
12.));
#140022=CARTESIAN_POINT('Ctrl Pts',(-62.1519925002978,-40.5027877865803,
12.));
#140023=CARTESIAN_POINT('Ctrl Pts',(-62.1644411502826,-40.5047277935767,
12.));
#140024=CARTESIAN_POINT('Ctrl Pts',(-62.1714473138108,-40.5058175523128,
12.));
#140025=CARTESIAN_POINT('Ctrl Pts',(-62.1730054756879,-40.506059810093,
12.));
#140026=CARTESIAN_POINT('',(-57.8261117662439,-39.4479504917286,0.));
#140027=CARTESIAN_POINT('',(-57.8261117662439,-39.4479504917286,0.));
#140028=CARTESIAN_POINT('Ctrl Pts',(-62.1730054756878,-40.506059810093,
0.));
#140029=CARTESIAN_POINT('Ctrl Pts',(-62.1714473138107,-40.5058175523128,
0.));
#140030=CARTESIAN_POINT('Ctrl Pts',(-62.1644411502825,-40.5047277935767,
0.));
#140031=CARTESIAN_POINT('Ctrl Pts',(-62.1519925002977,-40.5027877865803,
0.));
#140032=CARTESIAN_POINT('Ctrl Pts',(-62.1341126810543,-40.4999919096264,
0.));
#140033=CARTESIAN_POINT('Ctrl Pts',(-62.1108188417004,-40.4963316888412,
0.));
#140034=CARTESIAN_POINT('Ctrl Pts',(-62.083683068572,-40.4920425795216,
0.));
#140035=CARTESIAN_POINT('Ctrl Pts',(-62.0565861244179,-40.4877344164411,
0.));
#140036=CARTESIAN_POINT('Ctrl Pts',(-62.029528080742,-40.4834072522164,
0.));
#140037=CARTESIAN_POINT('Ctrl Pts',(-62.0025090125959,-40.4790611429583,
0.));
#140038=CARTESIAN_POINT('Ctrl Pts',(-61.9755289983044,-40.4746961480015,
0.));
#140039=CARTESIAN_POINT('Ctrl Pts',(-61.9485881182921,-40.470312328762,
0.));
#140040=CARTESIAN_POINT('Ctrl Pts',(-61.9216864541744,-40.4659097478587,
0.));
#140041=CARTESIAN_POINT('Ctrl Pts',(-61.8948240878008,-40.4614884681889,
0.));
#140042=CARTESIAN_POINT('Ctrl Pts',(-61.8680011001537,-40.4570485518749,
0.));
#140043=CARTESIAN_POINT('Ctrl Pts',(-61.8412175708553,-40.4525900597894,
0.));
#140044=CARTESIAN_POINT('Ctrl Pts',(-61.814473578779,-40.4481130521364,
0.));
#140045=CARTESIAN_POINT('Ctrl Pts',(-61.7877692024076,-40.4436175887949,
0.));
#140046=CARTESIAN_POINT('Ctrl Pts',(-61.7611045202874,-40.4391037297588,
0.));
#140047=CARTESIAN_POINT('Ctrl Pts',(-61.7344796114399,-40.4345715355404,
0.));
#140048=CARTESIAN_POINT('Ctrl Pts',(-61.7078945557799,-40.430021067584,
0.));
#140049=CARTESIAN_POINT('Ctrl Pts',(-61.6813494339286,-40.425452388076,
0.));
#140050=CARTESIAN_POINT('Ctrl Pts',(-61.6548443270394,-40.4208655597717,
0.));
#140051=CARTESIAN_POINT('Ctrl Pts',(-61.628379316608,-40.4162606458118,
0.));
#140052=CARTESIAN_POINT('Ctrl Pts',(-61.6019544843011,-40.4116377095596,
0.));
#140053=CARTESIAN_POINT('Ctrl Pts',(-61.5755699117324,-40.4069968143956,
0.));
#140054=CARTESIAN_POINT('Ctrl Pts',(-61.5492256804717,-40.4023380237232,
0.));
#140055=CARTESIAN_POINT('Ctrl Pts',(-61.522921872154,-40.3976614010652,
0.));
#140056=CARTESIAN_POINT('Ctrl Pts',(-61.4966585685549,-40.3929670101365,
0.));
#140057=CARTESIAN_POINT('Ctrl Pts',(-61.4704358516709,-40.3882549149227,
0.));
#140058=CARTESIAN_POINT('Ctrl Pts',(-61.4442538038044,-40.383525179772,
0.));
#140059=CARTESIAN_POINT('Ctrl Pts',(-61.4181125076037,-40.3787778694364,
0.));
#140060=CARTESIAN_POINT('Ctrl Pts',(-61.3920120460219,-40.3740130490225,
0.));
#140061=CARTESIAN_POINT('Ctrl Pts',(-61.3659525022908,-40.3692307839636,
0.));
#140062=CARTESIAN_POINT('Ctrl Pts',(-61.3399339598853,-40.3644311399861,
0.));
#140063=CARTESIAN_POINT('Ctrl Pts',(-61.3139565024847,-40.3596141830791,
0.));
#140064=CARTESIAN_POINT('Ctrl Pts',(-61.2880202139371,-40.3547799794679,
0.));
#140065=CARTESIAN_POINT('Ctrl Pts',(-61.2621251782863,-40.3499285956304,
0.));
#140066=CARTESIAN_POINT('Ctrl Pts',(-61.23627147979,-40.3450600983109,0.));
#140067=CARTESIAN_POINT('Ctrl Pts',(-61.2104592029377,-40.340174554537,
0.));
#140068=CARTESIAN_POINT('Ctrl Pts',(-61.1846884324644,-40.335272031637,
0.));
#140069=CARTESIAN_POINT('Ctrl Pts',(-61.1589592533613,-40.3303525972615,
0.));
#140070=CARTESIAN_POINT('Ctrl Pts',(-61.1332717508789,-40.32541631938,0.));
#140071=CARTESIAN_POINT('Ctrl Pts',(-61.1076260105258,-40.3204632662725,
0.));
#140072=CARTESIAN_POINT('Ctrl Pts',(-61.0820221180645,-40.3154935065262,
0.));
#140073=CARTESIAN_POINT('Ctrl Pts',(-61.056460159505,-40.3105071090309,
0.));
#140074=CARTESIAN_POINT('Ctrl Pts',(-61.0309402210921,-40.3055041429775,
0.));
#140075=CARTESIAN_POINT('Ctrl Pts',(-61.0054623893066,-40.300484677858,
0.));
#140076=CARTESIAN_POINT('Ctrl Pts',(-60.9800267508787,-40.295448783469,
0.));
#140077=CARTESIAN_POINT('Ctrl Pts',(-60.9546333927921,-40.2903965299155,
0.));
#140078=CARTESIAN_POINT('Ctrl Pts',(-60.9292824022887,-40.2853279876161,
0.));
#140079=CARTESIAN_POINT('Ctrl Pts',(-60.9039738668669,-40.2802432273104,
0.));
#140080=CARTESIAN_POINT('Ctrl Pts',(-60.8787078742818,-40.2751423200639,
0.));
#140081=CARTESIAN_POINT('Ctrl Pts',(-60.8534845125538,-40.2700253372647,
0.));
#140082=CARTESIAN_POINT('Ctrl Pts',(-60.8283038699706,-40.2648923506248,
0.));
#140083=CARTESIAN_POINT('Ctrl Pts',(-60.8031660350879,-40.2597434321803,
0.));
#140084=CARTESIAN_POINT('Ctrl Pts',(-60.7780710967248,-40.2545786542953,
0.));
#140085=CARTESIAN_POINT('Ctrl Pts',(-60.7530191439593,-40.2493980896638,
0.));
#140086=CARTESIAN_POINT('Ctrl Pts',(-60.728010266139,-40.2442018113108,
0.));
#140087=CARTESIAN_POINT('Ctrl Pts',(-60.7030445528857,-40.2389898925932,
0.));
#140088=CARTESIAN_POINT('Ctrl Pts',(-60.678122094098,-40.2337624072028,
0.));
#140089=CARTESIAN_POINT('Ctrl Pts',(-60.6532429799499,-40.2285194291706,
0.));
#140090=CARTESIAN_POINT('Ctrl Pts',(-60.6284073008871,-40.2232610328721,
0.));
#140091=CARTESIAN_POINT('Ctrl Pts',(-60.6036151476349,-40.2179872930273,
0.));
#140092=CARTESIAN_POINT('Ctrl Pts',(-60.5788666112042,-40.2126982847011,
0.));
#140093=CARTESIAN_POINT('Ctrl Pts',(-60.5541617828925,-40.2073940833052,
0.));
#140094=CARTESIAN_POINT('Ctrl Pts',(-60.5295007542841,-40.2020747646014,
0.));
#140095=CARTESIAN_POINT('Ctrl Pts',(-60.5048836172435,-40.1967404047062,
0.));
#140096=CARTESIAN_POINT('Ctrl Pts',(-60.4803104639226,-40.1913910800921,
0.));
#140097=CARTESIAN_POINT('Ctrl Pts',(-60.455781386769,-40.1860268675883,
0.));
#140098=CARTESIAN_POINT('Ctrl Pts',(-60.4312964785273,-40.180647844383,
0.));
#140099=CARTESIAN_POINT('Ctrl Pts',(-60.4068558322407,-40.1752540880268,
0.));
#140100=CARTESIAN_POINT('Ctrl Pts',(-60.3824595412446,-40.1698456764377,
0.));
#140101=CARTESIAN_POINT('Ctrl Pts',(-60.3581076991716,-40.1644226879033,
0.));
#140102=CARTESIAN_POINT('Ctrl Pts',(-60.3338003999607,-40.1589852010804,
0.));
#140103=CARTESIAN_POINT('Ctrl Pts',(-60.3095377378586,-40.1535332949976,
0.));
#140104=CARTESIAN_POINT('Ctrl Pts',(-60.285319807422,-40.1480670490585,
0.));
#140105=CARTESIAN_POINT('Ctrl Pts',(-60.2611467035117,-40.1425865430472,
0.));
#140106=CARTESIAN_POINT('Ctrl Pts',(-60.2370185212965,-40.1370918571304,
0.));
#140107=CARTESIAN_POINT('Ctrl Pts',(-60.2129353562622,-40.1315830718577,
0.));
#140108=CARTESIAN_POINT('Ctrl Pts',(-60.1888973042152,-40.1260602681644,
0.));
#140109=CARTESIAN_POINT('Ctrl Pts',(-60.1649044612828,-40.1205235273739,
0.));
#140110=CARTESIAN_POINT('Ctrl Pts',(-60.1409569239092,-40.1149729312036,
0.));
#140111=CARTESIAN_POINT('Ctrl Pts',(-60.1170547888574,-40.1094085617674,
0.));
#140112=CARTESIAN_POINT('Ctrl Pts',(-60.0931981532198,-40.1038305015766,
0.));
#140113=CARTESIAN_POINT('Ctrl Pts',(-60.069387114421,-40.0982388335423,
0.));
#140114=CARTESIAN_POINT('Ctrl Pts',(-60.0456217702202,-40.0926336409785,
0.));
#140115=CARTESIAN_POINT('Ctrl Pts',(-60.021902218706,-40.0870150076073,
0.));
#140116=CARTESIAN_POINT('Ctrl Pts',(-59.9982285582983,-40.0813830175623,
0.));
#140117=CARTESIAN_POINT('Ctrl Pts',(-59.9746008877584,-40.0757377553888,
0.));
#140118=CARTESIAN_POINT('Ctrl Pts',(-59.9510193061927,-40.0700793060473,
0.));
#140119=CARTESIAN_POINT('Ctrl Pts',(-59.9274839130553,-40.0644077549159,
0.));
#140120=CARTESIAN_POINT('Ctrl Pts',(-59.9039948081432,-40.0587231877961,
0.));
#140121=CARTESIAN_POINT('Ctrl Pts',(-59.8805520915975,-40.0530256909162,
0.));
#140122=CARTESIAN_POINT('Ctrl Pts',(-59.8571558639145,-40.0473153509323,
0.));
#140123=CARTESIAN_POINT('Ctrl Pts',(-59.8338062259491,-40.0415922549313,
0.));
#140124=CARTESIAN_POINT('Ctrl Pts',(-59.8105032789179,-40.035856490434,
0.));
#140125=CARTESIAN_POINT('Ctrl Pts',(-59.7872471243948,-40.0301081454006,
0.));
#140126=CARTESIAN_POINT('Ctrl Pts',(-59.7640378643115,-40.0243473082343,
0.));
#140127=CARTESIAN_POINT('Ctrl Pts',(-59.7408756009688,-40.0185740677827,
0.));
#140128=CARTESIAN_POINT('Ctrl Pts',(-59.7177604370409,-40.0127885133407,
0.));
#140129=CARTESIAN_POINT('Ctrl Pts',(-59.6946924755771,-40.0069907346536,
0.));
#140130=CARTESIAN_POINT('Ctrl Pts',(-59.671671819999,-40.001180821923,0.));
#140131=CARTESIAN_POINT('Ctrl Pts',(-59.6486985741015,-39.9953588658114,
0.));
#140132=CARTESIAN_POINT('Ctrl Pts',(-59.6257728420644,-39.9895249574432,
0.));
#140133=CARTESIAN_POINT('Ctrl Pts',(-59.6028947284551,-39.9836791884071,
0.));
#140134=CARTESIAN_POINT('Ctrl Pts',(-59.5800643382322,-39.9778216507609,
0.));
#140135=CARTESIAN_POINT('Ctrl Pts',(-59.5572817767412,-39.971952437036,
0.));
#140136=CARTESIAN_POINT('Ctrl Pts',(-59.5345471497162,-39.9660716402423,
0.));
#140137=CARTESIAN_POINT('Ctrl Pts',(-59.511860563292,-39.96017935387,0.));
#140138=CARTESIAN_POINT('Ctrl Pts',(-59.4892221240082,-39.954275671893,
0.));
#140139=CARTESIAN_POINT('Ctrl Pts',(-59.4666319388123,-39.9483606887731,
0.));
#140140=CARTESIAN_POINT('Ctrl Pts',(-59.444090115055,-39.9424344994652,
0.));
#140141=CARTESIAN_POINT('Ctrl Pts',(-59.4215967604925,-39.9364971994215,
0.));
#140142=CARTESIAN_POINT('Ctrl Pts',(-59.3991519832981,-39.9305488845934,
0.));
#140143=CARTESIAN_POINT('Ctrl Pts',(-59.3767558920663,-39.9245896514359,
0.));
#140144=CARTESIAN_POINT('Ctrl Pts',(-59.3544085958165,-39.9186195969113,
0.));
#140145=CARTESIAN_POINT('Ctrl Pts',(-59.3321102039883,-39.9126388184956,
0.));
#140146=CARTESIAN_POINT('Ctrl Pts',(-59.3098608264452,-39.9066474141826,
0.));
#140147=CARTESIAN_POINT('Ctrl Pts',(-59.2876605734871,-39.9006454824861,
0.));
#140148=CARTESIAN_POINT('Ctrl Pts',(-59.2655095558527,-39.8946331224442,
0.));
#140149=CARTESIAN_POINT('Ctrl Pts',(-59.2434078847236,-39.8886104336234,
0.));
#140150=CARTESIAN_POINT('Ctrl Pts',(-59.2213556717189,-39.8825775161252,
0.));
#140151=CARTESIAN_POINT('Ctrl Pts',(-59.1993530289008,-39.8765344705894,
0.));
#140152=CARTESIAN_POINT('Ctrl Pts',(-59.1774000687865,-39.8704813981978,
0.));
#140153=CARTESIAN_POINT('Ctrl Pts',(-59.155496904352,-39.8644184006785,
0.));
#140154=CARTESIAN_POINT('Ctrl Pts',(-59.133643649035,-39.8583455803111,
0.));
#140155=CARTESIAN_POINT('Ctrl Pts',(-59.1118404167304,-39.8522630399337,
0.));
#140156=CARTESIAN_POINT('Ctrl Pts',(-59.0900873217993,-39.8461708829465,
0.));
#140157=CARTESIAN_POINT('Ctrl Pts',(-59.068384479077,-39.8400692133143,
0.));
#140158=CARTESIAN_POINT('Ctrl Pts',(-59.0467320038783,-39.8339581355714,
0.));
#140159=CARTESIAN_POINT('Ctrl Pts',(-59.0251300119973,-39.8278377548261,
0.));
#140160=CARTESIAN_POINT('Ctrl Pts',(-59.0035786197024,-39.8217081767658,
0.));
#140161=CARTESIAN_POINT('Ctrl Pts',(-58.9820779437485,-39.8155695076624,
0.));
#140162=CARTESIAN_POINT('Ctrl Pts',(-58.9606281013876,-39.8094218543781,
0.));
#140163=CARTESIAN_POINT('Ctrl Pts',(-58.9392292103747,-39.8032653243712,
0.));
#140164=CARTESIAN_POINT('Ctrl Pts',(-58.9178813889703,-39.7971000257044,
0.));
#140165=CARTESIAN_POINT('Ctrl Pts',(-58.896584755939,-39.7909260670517,
0.));
#140166=CARTESIAN_POINT('Ctrl Pts',(-58.8753394305583,-39.7847435576995,
0.));
#140167=CARTESIAN_POINT('Ctrl Pts',(-58.8541455326229,-39.7785526075477,
0.));
#140168=CARTESIAN_POINT('Ctrl Pts',(-58.8330031824453,-39.772353327112,
0.));
#140169=CARTESIAN_POINT('Ctrl Pts',(-58.8119125008521,-39.7661458275276,
0.));
#140170=CARTESIAN_POINT('Ctrl Pts',(-58.7908736091808,-39.7599302205527,
0.));
#140171=CARTESIAN_POINT('Ctrl Pts',(-58.7698866293041,-39.753706618582,
0.));
#140172=CARTESIAN_POINT('Ctrl Pts',(-58.7489516836453,-39.7474751346603,
0.));
#140173=CARTESIAN_POINT('Ctrl Pts',(-58.7280688951911,-39.7412358824949,
0.));
#140174=CARTESIAN_POINT('Ctrl Pts',(-58.7072383875009,-39.7349889764737,
0.));
#140175=CARTESIAN_POINT('Ctrl Pts',(-58.6864602847065,-39.7287345316664,
0.));
#140176=CARTESIAN_POINT('Ctrl Pts',(-58.6657347115015,-39.7224726638087,
0.));
#140177=CARTESIAN_POINT('Ctrl Pts',(-58.6450617931269,-39.7162034892896,
0.));
#140178=CARTESIAN_POINT('Ctrl Pts',(-58.6244416553574,-39.7099271251421,
0.));
#140179=CARTESIAN_POINT('Ctrl Pts',(-58.6038744244683,-39.7036436890248,
0.));
#140180=CARTESIAN_POINT('Ctrl Pts',(-58.5833602272767,-39.6973532992555,
0.));
#140181=CARTESIAN_POINT('Ctrl Pts',(-58.5628991912067,-39.6910560748639,
0.));
#140182=CARTESIAN_POINT('Ctrl Pts',(-58.5424914443415,-39.6847521356395,
0.));
#140183=CARTESIAN_POINT('Ctrl Pts',(-58.5221371154748,-39.6784416021817,
0.));
#140184=CARTESIAN_POINT('Ctrl Pts',(-58.5018363341582,-39.6721245959516,
0.));
#140185=CARTESIAN_POINT('Ctrl Pts',(-58.4815892306044,-39.66580123918,0.));
#140186=CARTESIAN_POINT('Ctrl Pts',(-58.4613959355776,-39.659471654768,
0.));
#140187=CARTESIAN_POINT('Ctrl Pts',(-58.4412565802984,-39.6531359662043,
0.));
#140188=CARTESIAN_POINT('Ctrl Pts',(-58.4211712963024,-39.6467942974464,
0.));
#140189=CARTESIAN_POINT('Ctrl Pts',(-58.4011402154225,-39.6404467729113,
0.));
#140190=CARTESIAN_POINT('Ctrl Pts',(-58.3811634701061,-39.6340935177492,
0.));
#140191=CARTESIAN_POINT('Ctrl Pts',(-58.3612411936914,-39.6277346580898,
0.));
#140192=CARTESIAN_POINT('Ctrl Pts',(-58.3413735206412,-39.6213703212522,
0.));
#140193=CARTESIAN_POINT('Ctrl Pts',(-58.3215605869192,-39.6150006360894,
0.));
#140194=CARTESIAN_POINT('Ctrl Pts',(-58.3018025297288,-39.6086257327559,
0.));
#140195=CARTESIAN_POINT('Ctrl Pts',(-58.2820994868092,-39.6022457420772,
0.));
#140196=CARTESIAN_POINT('Ctrl Pts',(-58.2624515958416,-39.5958607950237,
0.));
#140197=CARTESIAN_POINT('Ctrl Pts',(-58.2428589938395,-39.5894710221729,
0.));
#140198=CARTESIAN_POINT('Ctrl Pts',(-58.2233218164408,-39.5830765530919,
0.));
#140199=CARTESIAN_POINT('Ctrl Pts',(-58.2038401992496,-39.5766775175226,
0.));
#140200=CARTESIAN_POINT('Ctrl Pts',(-58.1844142794359,-39.5702740468013,
0.));
#140201=CARTESIAN_POINT('Ctrl Pts',(-58.1650441970379,-39.5638662750174,
0.));
#140202=CARTESIAN_POINT('Ctrl Pts',(-58.1457300968467,-39.5574543406959,
0.));
#140203=CARTESIAN_POINT('Ctrl Pts',(-58.1264721285698,-39.5510383869476,
0.));
#140204=CARTESIAN_POINT('Ctrl Pts',(-58.1072704428895,-39.5446185579615,
0.));
#140205=CARTESIAN_POINT('Ctrl Pts',(-58.0881251879911,-39.5381949959214,
0.));
#140206=CARTESIAN_POINT('Ctrl Pts',(-58.0690365065393,-39.5317678383231,
0.));
#140207=CARTESIAN_POINT('Ctrl Pts',(-58.050004530846,-39.5253372136921,
0.));
#140208=CARTESIAN_POINT('Ctrl Pts',(-58.0310293875321,-39.5189032457227,
0.));
#140209=CARTESIAN_POINT('Ctrl Pts',(-58.012111206794,-39.5124660615009,
0.));
#140210=CARTESIAN_POINT('Ctrl Pts',(-57.9932501298522,-39.5060257981225,
0.));
#140211=CARTESIAN_POINT('Ctrl Pts',(-57.9744463179305,-39.4995826106691,
0.));
#140212=CARTESIAN_POINT('Ctrl Pts',(-57.9556999583777,-39.4931366776627,
0.));
#140213=CARTESIAN_POINT('Ctrl Pts',(-57.9370112456506,-39.4866881842223,
0.));
#140214=CARTESIAN_POINT('Ctrl Pts',(-57.9183803632337,-39.4802373061008,
0.));
#140215=CARTESIAN_POINT('Ctrl Pts',(-57.8998074670541,-39.4737841949417,
0.));
#140216=CARTESIAN_POINT('Ctrl Pts',(-57.8812926637397,-39.4673289592425,
0.));
#140217=CARTESIAN_POINT('Ctrl Pts',(-57.8628360097134,-39.4608716627367,
0.));
#140218=CARTESIAN_POINT('Ctrl Pts',(-57.8481172247805,-39.4557042029884,
0.));
#140219=CARTESIAN_POINT('Ctrl Pts',(-57.8371043151607,-39.45182770037,0.));
#140220=CARTESIAN_POINT('Ctrl Pts',(-57.829774010102,-39.4492429618498,
0.));
#140221=CARTESIAN_POINT('Ctrl Pts',(-57.8261117662439,-39.4479504917286,
0.));
#140222=CARTESIAN_POINT('Ctrl Pts',(-65.7914953018525,-34.9532422808861,
0.));
#140223=CARTESIAN_POINT('Ctrl Pts',(-65.7914953018525,-34.9532422808861,
12.));
#140224=CARTESIAN_POINT('Ctrl Pts',(-65.7859084407617,-34.9529266758465,
0.));
#140225=CARTESIAN_POINT('Ctrl Pts',(-65.7859084407617,-34.9529266758465,
12.));
#140226=CARTESIAN_POINT('Ctrl Pts',(-65.7747383251112,-34.9522931728759,
0.));
#140227=CARTESIAN_POINT('Ctrl Pts',(-65.7747383251112,-34.9522931728759,
12.));
#140228=CARTESIAN_POINT('Ctrl Pts',(-65.7579939712289,-34.9513360397454,
0.));
#140229=CARTESIAN_POINT('Ctrl Pts',(-65.7579939712289,-34.9513360397454,
12.));
#140230=CARTESIAN_POINT('Ctrl Pts',(-65.7356898061147,-34.9500461043246,
0.));
#140231=CARTESIAN_POINT('Ctrl Pts',(-65.7356898061147,-34.9500461043246,
12.));
#140232=CARTESIAN_POINT('Ctrl Pts',(-65.7078456758034,-34.9484107544137,
0.));
#140233=CARTESIAN_POINT('Ctrl Pts',(-65.7078456758034,-34.9484107544137,
12.));
#140234=CARTESIAN_POINT('Ctrl Pts',(-65.6800376406066,-34.9467524770438,
0.));
#140235=CARTESIAN_POINT('Ctrl Pts',(-65.6800376406066,-34.9467524770438,
12.));
#140236=CARTESIAN_POINT('Ctrl Pts',(-65.6522657321322,-34.9450712829182,
0.));
#140237=CARTESIAN_POINT('Ctrl Pts',(-65.6522657321322,-34.9450712829182,
12.));
#140238=CARTESIAN_POINT('Ctrl Pts',(-65.624529996851,-34.943367193292,0.));
#140239=CARTESIAN_POINT('Ctrl Pts',(-65.624529996851,-34.943367193292,12.));
#140240=CARTESIAN_POINT('Ctrl Pts',(-65.5968304997584,-34.9416402443435,
0.));
#140241=CARTESIAN_POINT('Ctrl Pts',(-65.5968304997584,-34.9416402443435,
12.));
#140242=CARTESIAN_POINT('Ctrl Pts',(-65.5691673225803,-34.9398904862157,
0.));
#140243=CARTESIAN_POINT('Ctrl Pts',(-65.5691673225803,-34.9398904862157,
12.));
#140244=CARTESIAN_POINT('Ctrl Pts',(-65.5415405577955,-34.9381179779673,
0.));
#140245=CARTESIAN_POINT('Ctrl Pts',(-65.5415405577955,-34.9381179779673,
12.));
#140246=CARTESIAN_POINT('Ctrl Pts',(-65.5139503038036,-34.9363227836582,
0.));
#140247=CARTESIAN_POINT('Ctrl Pts',(-65.5139503038036,-34.9363227836582,
12.));
#140248=CARTESIAN_POINT('Ctrl Pts',(-65.4863966597544,-34.9345049680825,
0.));
#140249=CARTESIAN_POINT('Ctrl Pts',(-65.4863966597544,-34.9345049680825,
12.));
#140250=CARTESIAN_POINT('Ctrl Pts',(-65.4588797201972,-34.932664592394,
0.));
#140251=CARTESIAN_POINT('Ctrl Pts',(-65.4588797201972,-34.932664592394,
12.));
#140252=CARTESIAN_POINT('Ctrl Pts',(-65.4313995707536,-34.9308017105536,
0.));
#140253=CARTESIAN_POINT('Ctrl Pts',(-65.4313995707536,-34.9308017105536,
12.));
#140254=CARTESIAN_POINT('Ctrl Pts',(-65.4039562911352,-34.9289163717747,
0.));
#140255=CARTESIAN_POINT('Ctrl Pts',(-65.4039562911352,-34.9289163717747,
12.));
#140256=CARTESIAN_POINT('Ctrl Pts',(-65.3765499573077,-34.9270086222731,
0.));
#140257=CARTESIAN_POINT('Ctrl Pts',(-65.3765499573077,-34.9270086222731,
12.));
#140258=CARTESIAN_POINT('Ctrl Pts',(-65.3491806440537,-34.9250785073477,
0.));
#140259=CARTESIAN_POINT('Ctrl Pts',(-65.3491806440537,-34.9250785073477,
12.));
#140260=CARTESIAN_POINT('Ctrl Pts',(-65.321848427191,-34.9231260731831,
0.));
#140261=CARTESIAN_POINT('Ctrl Pts',(-65.321848427191,-34.9231260731831,
12.));
#140262=CARTESIAN_POINT('Ctrl Pts',(-65.2945533863761,-34.9211513691355,
0.));
#140263=CARTESIAN_POINT('Ctrl Pts',(-65.2945533863761,-34.9211513691355,
12.));
#140264=CARTESIAN_POINT('Ctrl Pts',(-65.2672956048069,-34.9191544474872,
0.));
#140265=CARTESIAN_POINT('Ctrl Pts',(-65.2672956048069,-34.9191544474872,
12.));
#140266=CARTESIAN_POINT('Ctrl Pts',(-65.2400751679549,-34.9171353624113,
0.));
#140267=CARTESIAN_POINT('Ctrl Pts',(-65.2400751679549,-34.9171353624113,
12.));
#140268=CARTESIAN_POINT('Ctrl Pts',(-65.2128921625823,-34.9150941691747,
0.));
#140269=CARTESIAN_POINT('Ctrl Pts',(-65.2128921625823,-34.9150941691747,
12.));
#140270=CARTESIAN_POINT('Ctrl Pts',(-65.1857466757092,-34.9130309233022,
0.));
#140271=CARTESIAN_POINT('Ctrl Pts',(-65.1857466757092,-34.9130309233022,
12.));
#140272=CARTESIAN_POINT('Ctrl Pts',(-65.1586387934241,-34.9109456796213,
0.));
#140273=CARTESIAN_POINT('Ctrl Pts',(-65.1586387934241,-34.9109456796213,
12.));
#140274=CARTESIAN_POINT('Ctrl Pts',(-65.1315686003516,-34.9088384918336,
0.));
#140275=CARTESIAN_POINT('Ctrl Pts',(-65.1315686003516,-34.9088384918336,
12.));
#140276=CARTESIAN_POINT('Ctrl Pts',(-65.1045361803121,-34.9067094130399,
0.));
#140277=CARTESIAN_POINT('Ctrl Pts',(-65.1045361803121,-34.9067094130399,
12.));
#140278=CARTESIAN_POINT('Ctrl Pts',(-65.0775416167085,-34.9045584960509,
0.));
#140279=CARTESIAN_POINT('Ctrl Pts',(-65.0775416167085,-34.9045584960509,
12.));
#140280=CARTESIAN_POINT('Ctrl Pts',(-65.0505849930171,-34.9023857937865,
0.));
#140281=CARTESIAN_POINT('Ctrl Pts',(-65.0505849930171,-34.9023857937865,
12.));
#140282=CARTESIAN_POINT('Ctrl Pts',(-65.0236663932328,-34.9001913596416,
0.));
#140283=CARTESIAN_POINT('Ctrl Pts',(-65.0236663932328,-34.9001913596416,
12.));
#140284=CARTESIAN_POINT('Ctrl Pts',(-64.9967859023212,-34.8979752478616,
0.));
#140285=CARTESIAN_POINT('Ctrl Pts',(-64.9967859023212,-34.8979752478616,
12.));
#140286=CARTESIAN_POINT('Ctrl Pts',(-64.9699436060169,-34.8957375133697,
0.));
#140287=CARTESIAN_POINT('Ctrl Pts',(-64.9699436060169,-34.8957375133697,
12.));
#140288=CARTESIAN_POINT('Ctrl Pts',(-64.9431395906337,-34.8934782116095,
0.));
#140289=CARTESIAN_POINT('Ctrl Pts',(-64.9431395906337,-34.8934782116095,
12.));
#140290=CARTESIAN_POINT('Ctrl Pts',(-64.9163739428605,-34.8911973983785,
0.));
#140291=CARTESIAN_POINT('Ctrl Pts',(-64.9163739428605,-34.8911973983785,
12.));
#140292=CARTESIAN_POINT('Ctrl Pts',(-64.8896467495757,-34.888895129681,
0.));
#140293=CARTESIAN_POINT('Ctrl Pts',(-64.8896467495757,-34.888895129681,
12.));
#140294=CARTESIAN_POINT('Ctrl Pts',(-64.8629580976063,-34.8865714615436,
0.));
#140295=CARTESIAN_POINT('Ctrl Pts',(-64.8629580976063,-34.8865714615436,
12.));
#140296=CARTESIAN_POINT('Ctrl Pts',(-64.8363080737377,-34.8842264500188,
0.));
#140297=CARTESIAN_POINT('Ctrl Pts',(-64.8363080737377,-34.8842264500188,
12.));
#140298=CARTESIAN_POINT('Ctrl Pts',(-64.8096967648307,-34.881860151273,
0.));
#140299=CARTESIAN_POINT('Ctrl Pts',(-64.8096967648307,-34.881860151273,
12.));
#140300=CARTESIAN_POINT('Ctrl Pts',(-64.7831242579028,-34.8794726216513,
0.));
#140301=CARTESIAN_POINT('Ctrl Pts',(-64.7831242579028,-34.8794726216513,
12.));
#140302=CARTESIAN_POINT('Ctrl Pts',(-64.7565906402151,-34.8770639177493,
0.));
#140303=CARTESIAN_POINT('Ctrl Pts',(-64.7565906402151,-34.8770639177493,
12.));
#140304=CARTESIAN_POINT('Ctrl Pts',(-64.7300959993653,-34.8746340964971,
0.));
#140305=CARTESIAN_POINT('Ctrl Pts',(-64.7300959993653,-34.8746340964971,
12.));
#140306=CARTESIAN_POINT('Ctrl Pts',(-64.7036404233306,-34.8721832151974,
0.));
#140307=CARTESIAN_POINT('Ctrl Pts',(-64.7036404233306,-34.8721832151974,
12.));
#140308=CARTESIAN_POINT('Ctrl Pts',(-64.6772240004228,-34.869711331479,
0.));
#140309=CARTESIAN_POINT('Ctrl Pts',(-64.6772240004228,-34.869711331479,
12.));
#140310=CARTESIAN_POINT('Ctrl Pts',(-64.6508468192599,-34.867218503272,
0.));
#140311=CARTESIAN_POINT('Ctrl Pts',(-64.6508468192599,-34.867218503272,
12.));
#140312=CARTESIAN_POINT('Ctrl Pts',(-64.6245089687277,-34.8647047887774,
0.));
#140313=CARTESIAN_POINT('Ctrl Pts',(-64.6245089687277,-34.8647047887774,
12.));
#140314=CARTESIAN_POINT('Ctrl Pts',(-64.5982105379383,-34.8621702464401,
0.));
#140315=CARTESIAN_POINT('Ctrl Pts',(-64.5982105379383,-34.8621702464401,
12.));
#140316=CARTESIAN_POINT('Ctrl Pts',(-64.5719516161927,-34.8596149349256,
0.));
#140317=CARTESIAN_POINT('Ctrl Pts',(-64.5719516161927,-34.8596149349256,
12.));
#140318=CARTESIAN_POINT('Ctrl Pts',(-64.5457322930088,-34.857038913134,
0.));
#140319=CARTESIAN_POINT('Ctrl Pts',(-64.5457322930088,-34.857038913134,
12.));
#140320=CARTESIAN_POINT('Ctrl Pts',(-64.5195526581407,-34.8544422402118,
0.));
#140321=CARTESIAN_POINT('Ctrl Pts',(-64.5195526581407,-34.8544422402118,
12.));
#140322=CARTESIAN_POINT('Ctrl Pts',(-64.4934128015985,-34.851824975568,
0.));
#140323=CARTESIAN_POINT('Ctrl Pts',(-64.4934128015985,-34.851824975568,
12.));
#140324=CARTESIAN_POINT('Ctrl Pts',(-64.4673128136625,-34.8491871788895,
0.));
#140325=CARTESIAN_POINT('Ctrl Pts',(-64.4673128136625,-34.8491871788895,
12.));
#140326=CARTESIAN_POINT('Ctrl Pts',(-64.4412527848969,-34.8465289101621,
0.));
#140327=CARTESIAN_POINT('Ctrl Pts',(-64.4412527848969,-34.8465289101621,
12.));
#140328=CARTESIAN_POINT('Ctrl Pts',(-64.4152328061515,-34.8438502296664,
0.));
#140329=CARTESIAN_POINT('Ctrl Pts',(-64.4152328061515,-34.8438502296664,
12.));
#140330=CARTESIAN_POINT('Ctrl Pts',(-64.3892529685607,-34.8411511979702,
0.));
#140331=CARTESIAN_POINT('Ctrl Pts',(-64.3892529685607,-34.8411511979702,
12.));
#140332=CARTESIAN_POINT('Ctrl Pts',(-64.3633133635382,-34.8384318759248,
0.));
#140333=CARTESIAN_POINT('Ctrl Pts',(-64.3633133635382,-34.8384318759248,
12.));
#140334=CARTESIAN_POINT('Ctrl Pts',(-64.3374140827711,-34.8356923246618,
0.));
#140335=CARTESIAN_POINT('Ctrl Pts',(-64.3374140827711,-34.8356923246618,
12.));
#140336=CARTESIAN_POINT('Ctrl Pts',(-64.3115552182062,-34.8329326055919,
0.));
#140337=CARTESIAN_POINT('Ctrl Pts',(-64.3115552182062,-34.8329326055919,
12.));
#140338=CARTESIAN_POINT('Ctrl Pts',(-64.285736862052,-34.8301527804054,
0.));
#140339=CARTESIAN_POINT('Ctrl Pts',(-64.285736862052,-34.8301527804054,
12.));
#140340=CARTESIAN_POINT('Ctrl Pts',(-64.2599591067916,-34.8273529110744,
0.));
#140341=CARTESIAN_POINT('Ctrl Pts',(-64.2599591067916,-34.8273529110744,
12.));
#140342=CARTESIAN_POINT('Ctrl Pts',(-64.234222045188,-34.8245330598559,
0.));
#140343=CARTESIAN_POINT('Ctrl Pts',(-64.234222045188,-34.8245330598559,
12.));
#140344=CARTESIAN_POINT('Ctrl Pts',(-64.2085257702884,-34.8216932892968,
0.));
#140345=CARTESIAN_POINT('Ctrl Pts',(-64.2085257702884,-34.8216932892968,
12.));
#140346=CARTESIAN_POINT('Ctrl Pts',(-64.1828703754236,-34.8188336622419,
0.));
#140347=CARTESIAN_POINT('Ctrl Pts',(-64.1828703754236,-34.8188336622419,
12.));
#140348=CARTESIAN_POINT('Ctrl Pts',(-64.1572559542086,-34.8159542418374,
0.));
#140349=CARTESIAN_POINT('Ctrl Pts',(-64.1572559542086,-34.8159542418374,
12.));
#140350=CARTESIAN_POINT('Ctrl Pts',(-64.1316826005506,-34.8130550915287,
0.));
#140351=CARTESIAN_POINT('Ctrl Pts',(-64.1316826005506,-34.8130550915287,
12.));
#140352=CARTESIAN_POINT('Ctrl Pts',(-64.1061504086515,-34.8101362750597,
0.));
#140353=CARTESIAN_POINT('Ctrl Pts',(-64.1061504086515,-34.8101362750597,
12.));
#140354=CARTESIAN_POINT('Ctrl Pts',(-64.0806594730085,-34.8071978564747,
0.));
#140355=CARTESIAN_POINT('Ctrl Pts',(-64.0806594730085,-34.8071978564747,
12.));
#140356=CARTESIAN_POINT('Ctrl Pts',(-64.0552098884095,-34.8042399001211,
0.));
#140357=CARTESIAN_POINT('Ctrl Pts',(-64.0552098884095,-34.8042399001211,
12.));
#140358=CARTESIAN_POINT('Ctrl Pts',(-64.0298017499294,-34.8012624706526,
0.));
#140359=CARTESIAN_POINT('Ctrl Pts',(-64.0298017499294,-34.8012624706526,
12.));
#140360=CARTESIAN_POINT('Ctrl Pts',(-64.0044351529402,-34.7982656330293,
0.));
#140361=CARTESIAN_POINT('Ctrl Pts',(-64.0044351529402,-34.7982656330293,
12.));
#140362=CARTESIAN_POINT('Ctrl Pts',(-63.9791101931162,-34.7952494525177,
0.));
#140363=CARTESIAN_POINT('Ctrl Pts',(-63.9791101931162,-34.7952494525177,
12.));
#140364=CARTESIAN_POINT('Ctrl Pts',(-63.9538269664366,-34.7922139946943,
0.));
#140365=CARTESIAN_POINT('Ctrl Pts',(-63.9538269664366,-34.7922139946943,
12.));
#140366=CARTESIAN_POINT('Ctrl Pts',(-63.9285855691845,-34.7891593254488,
0.));
#140367=CARTESIAN_POINT('Ctrl Pts',(-63.9285855691845,-34.7891593254488,
12.));
#140368=CARTESIAN_POINT('Ctrl Pts',(-63.9033860979435,-34.7860855109911,
0.));
#140369=CARTESIAN_POINT('Ctrl Pts',(-63.9033860979435,-34.7860855109911,
12.));
#140370=CARTESIAN_POINT('Ctrl Pts',(-63.8782286496062,-34.7829926178496,
0.));
#140371=CARTESIAN_POINT('Ctrl Pts',(-63.8782286496062,-34.7829926178496,
12.));
#140372=CARTESIAN_POINT('Ctrl Pts',(-63.8531133213793,-34.7798807128715,
0.));
#140373=CARTESIAN_POINT('Ctrl Pts',(-63.8531133213793,-34.7798807128715,
12.));
#140374=CARTESIAN_POINT('Ctrl Pts',(-63.8280402107856,-34.7767498632243,
0.));
#140375=CARTESIAN_POINT('Ctrl Pts',(-63.8280402107856,-34.7767498632243,
12.));
#140376=CARTESIAN_POINT('Ctrl Pts',(-63.8030094156639,-34.7736001363993,
0.));
#140377=CARTESIAN_POINT('Ctrl Pts',(-63.8030094156639,-34.7736001363993,
12.));
#140378=CARTESIAN_POINT('Ctrl Pts',(-63.778021034163,-34.7704316002171,
0.));
#140379=CARTESIAN_POINT('Ctrl Pts',(-63.778021034163,-34.7704316002171,
12.));
#140380=CARTESIAN_POINT('Ctrl Pts',(-63.7530751647494,-34.7672443228275,
0.));
#140381=CARTESIAN_POINT('Ctrl Pts',(-63.7530751647494,-34.7672443228275,
12.));
#140382=CARTESIAN_POINT('Ctrl Pts',(-63.7281719062149,-34.76403837271,0.));
#140383=CARTESIAN_POINT('Ctrl Pts',(-63.7281719062149,-34.76403837271,12.));
#140384=CARTESIAN_POINT('Ctrl Pts',(-63.7033113576785,-34.7608138186759,
0.));
#140385=CARTESIAN_POINT('Ctrl Pts',(-63.7033113576785,-34.7608138186759,
12.));
#140386=CARTESIAN_POINT('Ctrl Pts',(-63.6784936185885,-34.7575707298713,
0.));
#140387=CARTESIAN_POINT('Ctrl Pts',(-63.6784936185885,-34.7575707298713,
12.));
#140388=CARTESIAN_POINT('Ctrl Pts',(-63.6537187887159,-34.7543091757833,
0.));
#140389=CARTESIAN_POINT('Ctrl Pts',(-63.6537187887159,-34.7543091757833,
12.));
#140390=CARTESIAN_POINT('Ctrl Pts',(-63.6289869681604,-34.7510292262406,
0.));
#140391=CARTESIAN_POINT('Ctrl Pts',(-63.6289869681604,-34.7510292262406,
12.));
#140392=CARTESIAN_POINT('Ctrl Pts',(-63.6042982573588,-34.7477309514136,
0.));
#140393=CARTESIAN_POINT('Ctrl Pts',(-63.6042982573588,-34.7477309514136,
12.));
#140394=CARTESIAN_POINT('Ctrl Pts',(-63.5796527570871,-34.744414421816,
0.));
#140395=CARTESIAN_POINT('Ctrl Pts',(-63.5796527570871,-34.744414421816,
12.));
#140396=CARTESIAN_POINT('Ctrl Pts',(-63.5550505684626,-34.7410797083081,
0.));
#140397=CARTESIAN_POINT('Ctrl Pts',(-63.5550505684626,-34.7410797083081,
12.));
#140398=CARTESIAN_POINT('Ctrl Pts',(-63.5304917929386,-34.7377268821025,
0.));
#140399=CARTESIAN_POINT('Ctrl Pts',(-63.5304917929386,-34.7377268821025,
12.));
#140400=CARTESIAN_POINT('Ctrl Pts',(-63.505976532309,-34.7343560147667,
0.));
#140401=CARTESIAN_POINT('Ctrl Pts',(-63.505976532309,-34.7343560147667,
12.));
#140402=CARTESIAN_POINT('Ctrl Pts',(-63.4815048887165,-34.7309671782214,
0.));
#140403=CARTESIAN_POINT('Ctrl Pts',(-63.4815048887165,-34.7309671782214,
12.));
#140404=CARTESIAN_POINT('Ctrl Pts',(-63.4570769646569,-34.7275604447438,
0.));
#140405=CARTESIAN_POINT('Ctrl Pts',(-63.4570769646569,-34.7275604447438,
12.));
#140406=CARTESIAN_POINT('Ctrl Pts',(-63.4326928629795,-34.7241358869701,
0.));
#140407=CARTESIAN_POINT('Ctrl Pts',(-63.4326928629795,-34.7241358869701,
12.));
#140408=CARTESIAN_POINT('Ctrl Pts',(-63.4083526868836,-34.7206935779007,
0.));
#140409=CARTESIAN_POINT('Ctrl Pts',(-63.4083526868836,-34.7206935779007,
12.));
#140410=CARTESIAN_POINT('Ctrl Pts',(-63.3840565399208,-34.7172335909038,
0.));
#140411=CARTESIAN_POINT('Ctrl Pts',(-63.3840565399208,-34.7172335909038,
12.));
#140412=CARTESIAN_POINT('Ctrl Pts',(-63.3598045260053,-34.7137559997146,
0.));
#140413=CARTESIAN_POINT('Ctrl Pts',(-63.3598045260053,-34.7137559997146,
12.));
#140414=CARTESIAN_POINT('Ctrl Pts',(-63.3355967494171,-34.7102608784374,
0.));
#140415=CARTESIAN_POINT('Ctrl Pts',(-63.3355967494171,-34.7102608784374,
12.));
#140416=CARTESIAN_POINT('Ctrl Pts',(-63.3114333148048,-34.7067483015491,
0.));
#140417=CARTESIAN_POINT('Ctrl Pts',(-63.3114333148048,-34.7067483015491,
12.));
#140418=CARTESIAN_POINT('Ctrl Pts',(-63.2873143271807,-34.703218343904,
0.));
#140419=CARTESIAN_POINT('Ctrl Pts',(-63.2873143271807,-34.703218343904,
12.));
#140420=CARTESIAN_POINT('Ctrl Pts',(-63.2632398919225,-34.6996710807378,
0.));
#140421=CARTESIAN_POINT('Ctrl Pts',(-63.2632398919225,-34.6996710807378,
12.));
#140422=CARTESIAN_POINT('Ctrl Pts',(-63.2392101147847,-34.6961065876666,
0.));
#140423=CARTESIAN_POINT('Ctrl Pts',(-63.2392101147847,-34.6961065876666,
12.));
#140424=CARTESIAN_POINT('Ctrl Pts',(-63.2152251019012,-34.6925249406897,
0.));
#140425=CARTESIAN_POINT('Ctrl Pts',(-63.2152251019012,-34.6925249406897,
12.));
#140426=CARTESIAN_POINT('Ctrl Pts',(-63.1912849597887,-34.6889262161924,
0.));
#140427=CARTESIAN_POINT('Ctrl Pts',(-63.1912849597887,-34.6889262161924,
12.));
#140428=CARTESIAN_POINT('Ctrl Pts',(-63.1673897953429,-34.6853104909518,
0.));
#140429=CARTESIAN_POINT('Ctrl Pts',(-63.1673897953429,-34.6853104909518,
12.));
#140430=CARTESIAN_POINT('Ctrl Pts',(-63.1435397158388,-34.6816778421402,
0.));
#140431=CARTESIAN_POINT('Ctrl Pts',(-63.1435397158388,-34.6816778421402,
12.));
#140432=CARTESIAN_POINT('Ctrl Pts',(-63.119734828943,-34.6780283473252,
0.));
#140433=CARTESIAN_POINT('Ctrl Pts',(-63.119734828943,-34.6780283473252,
12.));
#140434=CARTESIAN_POINT('Ctrl Pts',(-63.0959752427168,-34.674362084472,
0.));
#140435=CARTESIAN_POINT('Ctrl Pts',(-63.0959752427168,-34.674362084472,
12.));
#140436=CARTESIAN_POINT('Ctrl Pts',(-63.0722610656194,-34.670679131947,
0.));
#140437=CARTESIAN_POINT('Ctrl Pts',(-63.0722610656194,-34.670679131947,
12.));
#140438=CARTESIAN_POINT('Ctrl Pts',(-63.0485924065045,-34.6669795685228,
0.));
#140439=CARTESIAN_POINT('Ctrl Pts',(-63.0485924065045,-34.6669795685228,
12.));
#140440=CARTESIAN_POINT('Ctrl Pts',(-63.0249693746208,-34.6632634733824,
0.));
#140441=CARTESIAN_POINT('Ctrl Pts',(-63.0249693746208,-34.6632634733824,
12.));
#140442=CARTESIAN_POINT('Ctrl Pts',(-63.0013920796235,-34.6595309261191,
0.));
#140443=CARTESIAN_POINT('Ctrl Pts',(-63.0013920796235,-34.6595309261191,
12.));
#140444=CARTESIAN_POINT('Ctrl Pts',(-62.9778606315783,-34.6557820067393,
0.));
#140445=CARTESIAN_POINT('Ctrl Pts',(-62.9778606315783,-34.6557820067393,
12.));
#140446=CARTESIAN_POINT('Ctrl Pts',(-62.9543751409646,-34.6520167956655,
0.));
#140447=CARTESIAN_POINT('Ctrl Pts',(-62.9543751409646,-34.6520167956655,
12.));
#140448=CARTESIAN_POINT('Ctrl Pts',(-62.9309357186717,-34.6482353737424,
0.));
#140449=CARTESIAN_POINT('Ctrl Pts',(-62.9309357186717,-34.6482353737424,
12.));
#140450=CARTESIAN_POINT('Ctrl Pts',(-62.9075424760015,-34.644437822241,
0.));
#140451=CARTESIAN_POINT('Ctrl Pts',(-62.9075424760015,-34.644437822241,
12.));
#140452=CARTESIAN_POINT('Ctrl Pts',(-62.8841955246794,-34.6406242228592,
0.));
#140453=CARTESIAN_POINT('Ctrl Pts',(-62.8841955246794,-34.6406242228592,
12.));
#140454=CARTESIAN_POINT('Ctrl Pts',(-62.8608949768571,-34.6367946577235,
0.));
#140455=CARTESIAN_POINT('Ctrl Pts',(-62.8608949768571,-34.6367946577235,
12.));
#140456=CARTESIAN_POINT('Ctrl Pts',(-62.8376409451175,-34.6329492093935,
0.));
#140457=CARTESIAN_POINT('Ctrl Pts',(-62.8376409451175,-34.6329492093935,
12.));
#140458=CARTESIAN_POINT('Ctrl Pts',(-62.8144335424697,-34.6290879608673,
0.));
#140459=CARTESIAN_POINT('Ctrl Pts',(-62.8144335424697,-34.6290879608673,
12.));
#140460=CARTESIAN_POINT('Ctrl Pts',(-62.7912728823518,-34.6252109955853,
0.));
#140461=CARTESIAN_POINT('Ctrl Pts',(-62.7912728823518,-34.6252109955853,
12.));
#140462=CARTESIAN_POINT('Ctrl Pts',(-62.7681590786429,-34.6213183974317,
0.));
#140463=CARTESIAN_POINT('Ctrl Pts',(-62.7681590786429,-34.6213183974317,
12.));
#140464=CARTESIAN_POINT('Ctrl Pts',(-62.7450922456676,-34.6174102507375,
0.));
#140465=CARTESIAN_POINT('Ctrl Pts',(-62.7450922456676,-34.6174102507375,
12.));
#140466=CARTESIAN_POINT('Ctrl Pts',(-62.7220724981994,-34.6134866402837,
0.));
#140467=CARTESIAN_POINT('Ctrl Pts',(-62.7220724981994,-34.6134866402837,
12.));
#140468=CARTESIAN_POINT('Ctrl Pts',(-62.6990999514563,-34.6095476513077,
0.));
#140469=CARTESIAN_POINT('Ctrl Pts',(-62.6990999514563,-34.6095476513077,
12.));
#140470=CARTESIAN_POINT('Ctrl Pts',(-62.6761747211037,-34.6055933695069,
0.));
#140471=CARTESIAN_POINT('Ctrl Pts',(-62.6761747211037,-34.6055933695069,
12.));
#140472=CARTESIAN_POINT('Ctrl Pts',(-62.6532969232657,-34.6016238810398,
0.));
#140473=CARTESIAN_POINT('Ctrl Pts',(-62.6532969232657,-34.6016238810398,
12.));
#140474=CARTESIAN_POINT('Ctrl Pts',(-62.6304666745306,-34.5976392725296,
0.));
#140475=CARTESIAN_POINT('Ctrl Pts',(-62.6304666745306,-34.5976392725296,
12.));
#140476=CARTESIAN_POINT('Ctrl Pts',(-62.6076840919536,-34.5936396310679,
0.));
#140477=CARTESIAN_POINT('Ctrl Pts',(-62.6076840919536,-34.5936396310679,
12.));
#140478=CARTESIAN_POINT('Ctrl Pts',(-62.5849492930533,-34.5896250442216,
0.));
#140479=CARTESIAN_POINT('Ctrl Pts',(-62.5849492930533,-34.5896250442216,
12.));
#140480=CARTESIAN_POINT('Ctrl Pts',(-62.562262395816,-34.5855956000363,
0.));
#140481=CARTESIAN_POINT('Ctrl Pts',(-62.562262395816,-34.5855956000363,
12.));
#140482=CARTESIAN_POINT('Ctrl Pts',(-62.5396235187079,-34.5815513870377,
0.));
#140483=CARTESIAN_POINT('Ctrl Pts',(-62.5396235187079,-34.5815513870377,
12.));
#140484=CARTESIAN_POINT('Ctrl Pts',(-62.5170327806781,-34.5774924942355,
0.));
#140485=CARTESIAN_POINT('Ctrl Pts',(-62.5170327806781,-34.5774924942355,
12.));
#140486=CARTESIAN_POINT('Ctrl Pts',(-62.4944903011628,-34.5734190111272,
0.));
#140487=CARTESIAN_POINT('Ctrl Pts',(-62.4944903011628,-34.5734190111272,
12.));
#140488=CARTESIAN_POINT('Ctrl Pts',(-62.4719962000808,-34.5693310277051,
0.));
#140489=CARTESIAN_POINT('Ctrl Pts',(-62.4719962000808,-34.5693310277051,
12.));
#140490=CARTESIAN_POINT('Ctrl Pts',(-62.4495505978393,-34.5652286344593,
0.));
#140491=CARTESIAN_POINT('Ctrl Pts',(-62.4495505978393,-34.5652286344593,
12.));
#140492=CARTESIAN_POINT('Ctrl Pts',(-62.4271536153459,-34.5611119223798,
0.));
#140493=CARTESIAN_POINT('Ctrl Pts',(-62.4271536153459,-34.5611119223798,
12.));
#140494=CARTESIAN_POINT('Ctrl Pts',(-62.4048053740127,-34.5569809829613,
0.));
#140495=CARTESIAN_POINT('Ctrl Pts',(-62.4048053740127,-34.5569809829613,
12.));
#140496=CARTESIAN_POINT('Ctrl Pts',(-62.3825059957601,-34.5528359082075,
0.));
#140497=CARTESIAN_POINT('Ctrl Pts',(-62.3825059957601,-34.5528359082075,
12.));
#140498=CARTESIAN_POINT('Ctrl Pts',(-62.3602556030127,-34.5486767906384,
0.));
#140499=CARTESIAN_POINT('Ctrl Pts',(-62.3602556030127,-34.5486767906384,
12.));
#140500=CARTESIAN_POINT('Ctrl Pts',(-62.338054318708,-34.5445037232936,
0.));
#140501=CARTESIAN_POINT('Ctrl Pts',(-62.338054318708,-34.5445037232936,
12.));
#140502=CARTESIAN_POINT('Ctrl Pts',(-62.3159022663058,-34.5403167997337,
0.));
#140503=CARTESIAN_POINT('Ctrl Pts',(-62.3159022663058,-34.5403167997337,
12.));
#140504=CARTESIAN_POINT('Ctrl Pts',(-62.2937995697925,-34.5361161140449,
0.));
#140505=CARTESIAN_POINT('Ctrl Pts',(-62.2937995697925,-34.5361161140449,
12.));
#140506=CARTESIAN_POINT('Ctrl Pts',(-62.2717463536827,-34.5319017608433,
0.));
#140507=CARTESIAN_POINT('Ctrl Pts',(-62.2717463536827,-34.5319017608433,
12.));
#140508=CARTESIAN_POINT('Ctrl Pts',(-62.2497427430135,-34.5276738352808,
0.));
#140509=CARTESIAN_POINT('Ctrl Pts',(-62.2497427430135,-34.5276738352808,
12.));
#140510=CARTESIAN_POINT('Ctrl Pts',(-62.2277888633576,-34.523432433049,
0.));
#140511=CARTESIAN_POINT('Ctrl Pts',(-62.2277888633576,-34.523432433049,
12.));
#140512=CARTESIAN_POINT('Ctrl Pts',(-62.2058848408347,-34.5191776503842,
0.));
#140513=CARTESIAN_POINT('Ctrl Pts',(-62.2058848408347,-34.5191776503842,
12.));
#140514=CARTESIAN_POINT('Ctrl Pts',(-62.1840308021171,-34.5149095840729,
0.));
#140515=CARTESIAN_POINT('Ctrl Pts',(-62.1840308021171,-34.5149095840729,
12.));
#140516=CARTESIAN_POINT('Ctrl Pts',(-62.1622268744336,-34.5106283314594,
0.));
#140517=CARTESIAN_POINT('Ctrl Pts',(-62.1622268744336,-34.5106283314594,
12.));
#140518=CARTESIAN_POINT('Ctrl Pts',(-62.1404731855686,-34.5063339904533,
0.));
#140519=CARTESIAN_POINT('Ctrl Pts',(-62.1404731855686,-34.5063339904533,
12.));
#140520=CARTESIAN_POINT('Ctrl Pts',(-62.1187698638705,-34.5020266595292,
0.));
#140521=CARTESIAN_POINT('Ctrl Pts',(-62.1187698638705,-34.5020266595292,
12.));
#140522=CARTESIAN_POINT('Ctrl Pts',(-62.0971170382565,-34.4977064377281,
0.));
#140523=CARTESIAN_POINT('Ctrl Pts',(-62.0971170382565,-34.4977064377281,
12.));
#140524=CARTESIAN_POINT('Ctrl Pts',(-62.0755148382136,-34.4933734246592,
0.));
#140525=CARTESIAN_POINT('Ctrl Pts',(-62.0755148382136,-34.4933734246592,
12.));
#140526=CARTESIAN_POINT('Ctrl Pts',(-62.0539633937944,-34.4890277205041,
0.));
#140527=CARTESIAN_POINT('Ctrl Pts',(-62.0539633937944,-34.4890277205041,
12.));
#140528=CARTESIAN_POINT('Ctrl Pts',(-62.0324628356152,-34.4846694260205,
0.));
#140529=CARTESIAN_POINT('Ctrl Pts',(-62.0324628356152,-34.4846694260205,
12.));
#140530=CARTESIAN_POINT('Ctrl Pts',(-62.0110132948807,-34.4802986425535,
0.));
#140531=CARTESIAN_POINT('Ctrl Pts',(-62.0110132948807,-34.4802986425535,
12.));
#140532=CARTESIAN_POINT('Ctrl Pts',(-61.9896149034009,-34.4759154720477,
0.));
#140533=CARTESIAN_POINT('Ctrl Pts',(-61.9896149034009,-34.4759154720477,
12.));
#140534=CARTESIAN_POINT('Ctrl Pts',(-61.9682677936048,-34.4715200170589,
0.));
#140535=CARTESIAN_POINT('Ctrl Pts',(-61.9682677936048,-34.4715200170589,
12.));
#140536=CARTESIAN_POINT('Ctrl Pts',(-61.9469720985512,-34.4671123807706,
0.));
#140537=CARTESIAN_POINT('Ctrl Pts',(-61.9469720985512,-34.4671123807706,
12.));
#140538=CARTESIAN_POINT('Ctrl Pts',(-61.9257279519283,-34.462692666996,
0.));
#140539=CARTESIAN_POINT('Ctrl Pts',(-61.9257279519283,-34.462692666996,
12.));
#140540=CARTESIAN_POINT('Ctrl Pts',(-61.9045354880424,-34.4582609801625,
0.));
#140541=CARTESIAN_POINT('Ctrl Pts',(-61.9045354880424,-34.4582609801625,
12.));
#140542=CARTESIAN_POINT('Ctrl Pts',(-61.883394841802,-34.4538174253009,
0.));
#140543=CARTESIAN_POINT('Ctrl Pts',(-61.883394841802,-34.4538174253009,
12.));
#140544=CARTESIAN_POINT('Ctrl Pts',(-61.862306148703,-34.4493621080367,
0.));
#140545=CARTESIAN_POINT('Ctrl Pts',(-61.862306148703,-34.4493621080367,
12.));
#140546=CARTESIAN_POINT('Ctrl Pts',(-61.8412695447951,-34.4448951345753,
0.));
#140547=CARTESIAN_POINT('Ctrl Pts',(-61.8412695447951,-34.4448951345753,
12.));
#140548=CARTESIAN_POINT('Ctrl Pts',(-61.8202851667247,-34.4404166117313,
0.));
#140549=CARTESIAN_POINT('Ctrl Pts',(-61.8202851667247,-34.4404166117313,
12.));
#140550=CARTESIAN_POINT('Ctrl Pts',(-61.7993531518052,-34.4359266469757,
0.));
#140551=CARTESIAN_POINT('Ctrl Pts',(-61.7993531518052,-34.4359266469757,
12.));
#140552=CARTESIAN_POINT('Ctrl Pts',(-61.7784736380727,-34.4314253484791,
0.));
#140553=CARTESIAN_POINT('Ctrl Pts',(-61.7784736380727,-34.4314253484791,
12.));
#140554=CARTESIAN_POINT('Ctrl Pts',(-61.7576467643419,-34.4269128251569,
0.));
#140555=CARTESIAN_POINT('Ctrl Pts',(-61.7576467643419,-34.4269128251569,
12.));
#140556=CARTESIAN_POINT('Ctrl Pts',(-61.7368726702573,-34.4223891867166,
0.));
#140557=CARTESIAN_POINT('Ctrl Pts',(-61.7368726702573,-34.4223891867166,
12.));
#140558=CARTESIAN_POINT('Ctrl Pts',(-61.7161514961892,-34.4178545435753,
0.));
#140559=CARTESIAN_POINT('Ctrl Pts',(-61.7161514961892,-34.4178545435753,
12.));
#140560=CARTESIAN_POINT('Ctrl Pts',(-61.6954833831157,-34.4133090067696,
0.));
#140561=CARTESIAN_POINT('Ctrl Pts',(-61.6954833831157,-34.4133090067696,
12.));
#140562=CARTESIAN_POINT('Ctrl Pts',(-61.674868472521,-34.4087526878815,
0.));
#140563=CARTESIAN_POINT('Ctrl Pts',(-61.674868472521,-34.4087526878815,
12.));
#140564=CARTESIAN_POINT('Ctrl Pts',(-61.6543069062436,-34.4041856989328,
0.));
#140565=CARTESIAN_POINT('Ctrl Pts',(-61.6543069062436,-34.4041856989328,
12.));
#140566=CARTESIAN_POINT('Ctrl Pts',(-61.6337988264586,-34.399608152377,
0.));
#140567=CARTESIAN_POINT('Ctrl Pts',(-61.6337988264586,-34.399608152377,
12.));
#140568=CARTESIAN_POINT('Ctrl Pts',(-61.6133443760168,-34.3950201613446,
0.));
#140569=CARTESIAN_POINT('Ctrl Pts',(-61.6133443760168,-34.3950201613446,
12.));
#140570=CARTESIAN_POINT('Ctrl Pts',(-61.5929436987419,-34.3904218398642,
0.));
#140571=CARTESIAN_POINT('Ctrl Pts',(-61.5929436987419,-34.3904218398642,
12.));
#140572=CARTESIAN_POINT('Ctrl Pts',(-61.5725969396817,-34.3858133030511,
0.));
#140573=CARTESIAN_POINT('Ctrl Pts',(-61.5725969396817,-34.3858133030511,
12.));
#140574=CARTESIAN_POINT('Ctrl Pts',(-61.5523042455127,-34.3811946674179,
0.));
#140575=CARTESIAN_POINT('Ctrl Pts',(-61.5523042455127,-34.3811946674179,
12.));
#140576=CARTESIAN_POINT('Ctrl Pts',(-61.5320657642601,-34.3765660506659,
0.));
#140577=CARTESIAN_POINT('Ctrl Pts',(-61.5320657642601,-34.3765660506659,
12.));
#140578=CARTESIAN_POINT('Ctrl Pts',(-61.511881644541,-34.3719275711179,
0.));
#140579=CARTESIAN_POINT('Ctrl Pts',(-61.511881644541,-34.3719275711179,
12.));
#140580=CARTESIAN_POINT('Ctrl Pts',(-61.4917520349276,-34.3672793472463,
0.));
#140581=CARTESIAN_POINT('Ctrl Pts',(-61.4917520349276,-34.3672793472463,
12.));
#140582=CARTESIAN_POINT('Ctrl Pts',(-61.4716770832924,-34.3626214971903,
0.));
#140583=CARTESIAN_POINT('Ctrl Pts',(-61.4716770832924,-34.3626214971903,
12.));
#140584=CARTESIAN_POINT('Ctrl Pts',(-61.4516569360499,-34.357954138202,
0.));
#140585=CARTESIAN_POINT('Ctrl Pts',(-61.4516569360499,-34.357954138202,
12.));
#140586=CARTESIAN_POINT('Ctrl Pts',(-61.4316917395959,-34.3532773877112,
0.));
#140587=CARTESIAN_POINT('Ctrl Pts',(-61.4316917395959,-34.3532773877112,
12.));
#140588=CARTESIAN_POINT('Ctrl Pts',(-61.4117816420251,-34.3485913645991,
0.));
#140589=CARTESIAN_POINT('Ctrl Pts',(-61.4117816420251,-34.3485913645991,
12.));
#140590=CARTESIAN_POINT('Ctrl Pts',(-61.3919267945293,-34.34389619024,0.));
#140591=CARTESIAN_POINT('Ctrl Pts',(-61.3919267945293,-34.34389619024,12.));
#140592=CARTESIAN_POINT('Ctrl Pts',(-61.3721273534222,-34.339191990012,
0.));
#140593=CARTESIAN_POINT('Ctrl Pts',(-61.3721273534222,-34.339191990012,
12.));
#140594=CARTESIAN_POINT('Ctrl Pts',(-61.3523834803144,-34.3344788934337,
0.));
#140595=CARTESIAN_POINT('Ctrl Pts',(-61.3523834803144,-34.3344788934337,
12.));
#140596=CARTESIAN_POINT('Ctrl Pts',(-61.3326953378817,-34.3297570310126,
0.));
#140597=CARTESIAN_POINT('Ctrl Pts',(-61.3326953378817,-34.3297570310126,
12.));
#140598=CARTESIAN_POINT('Ctrl Pts',(-61.3130630861375,-34.3250265314761,
0.));
#140599=CARTESIAN_POINT('Ctrl Pts',(-61.3130630861375,-34.3250265314761,
12.));
#140600=CARTESIAN_POINT('Ctrl Pts',(-61.2934868791875,-34.3202875193629,
0.));
#140601=CARTESIAN_POINT('Ctrl Pts',(-61.2934868791875,-34.3202875193629,
12.));
#140602=CARTESIAN_POINT('Ctrl Pts',(-61.2739668600415,-34.3155401111776,
0.));
#140603=CARTESIAN_POINT('Ctrl Pts',(-61.2739668600415,-34.3155401111776,
12.));
#140604=CARTESIAN_POINT('Ctrl Pts',(-61.2545031656196,-34.3107844191081,
0.));
#140605=CARTESIAN_POINT('Ctrl Pts',(-61.2545031656196,-34.3107844191081,
12.));
#140606=CARTESIAN_POINT('Ctrl Pts',(-61.2350959366987,-34.3060205584093,
0.));
#140607=CARTESIAN_POINT('Ctrl Pts',(-61.2350959366987,-34.3060205584093,
12.));
#140608=CARTESIAN_POINT('Ctrl Pts',(-61.2157453259107,-34.3012486533474,
0.));
#140609=CARTESIAN_POINT('Ctrl Pts',(-61.2157453259107,-34.3012486533474,
12.));
#140610=CARTESIAN_POINT('Ctrl Pts',(-61.1964515073823,-34.296468844362,
0.));
#140611=CARTESIAN_POINT('Ctrl Pts',(-61.1964515073823,-34.296468844362,
12.));
#140612=CARTESIAN_POINT('Ctrl Pts',(-61.1772146833083,-34.2916812929675,
0.));
#140613=CARTESIAN_POINT('Ctrl Pts',(-61.1772146833083,-34.2916812929675,
12.));
#140614=CARTESIAN_POINT('Ctrl Pts',(-61.15803506354,-34.2868861666301,0.));
#140615=CARTESIAN_POINT('Ctrl Pts',(-61.15803506354,-34.2868861666301,12.));
#140616=CARTESIAN_POINT('Ctrl Pts',(-61.1389128461815,-34.2820836244425,
0.));
#140617=CARTESIAN_POINT('Ctrl Pts',(-61.1389128461815,-34.2820836244425,
12.));
#140618=CARTESIAN_POINT('Ctrl Pts',(-61.119848199783,-34.2772738038811,
0.));
#140619=CARTESIAN_POINT('Ctrl Pts',(-61.119848199783,-34.2772738038811,
12.));
#140620=CARTESIAN_POINT('Ctrl Pts',(-61.100841240023,-34.2724568037374,
0.));
#140621=CARTESIAN_POINT('Ctrl Pts',(-61.100841240023,-34.2724568037374,
12.));
#140622=CARTESIAN_POINT('Ctrl Pts',(-61.0818920286644,-34.2676326825846,
0.));
#140623=CARTESIAN_POINT('Ctrl Pts',(-61.0818920286644,-34.2676326825846,
12.));
#140624=CARTESIAN_POINT('Ctrl Pts',(-61.0667788793594,-34.2637677132139,
0.));
#140625=CARTESIAN_POINT('Ctrl Pts',(-61.0667788793594,-34.2637677132139,
12.));
#140626=CARTESIAN_POINT('Ctrl Pts',(-61.0554700177206,-34.2608658001761,
0.));
#140627=CARTESIAN_POINT('Ctrl Pts',(-61.0554700177206,-34.2608658001761,
12.));
#140628=CARTESIAN_POINT('Ctrl Pts',(-61.0479423318803,-34.2589297755482,
0.));
#140629=CARTESIAN_POINT('Ctrl Pts',(-61.0479423318803,-34.2589297755482,
12.));
#140630=CARTESIAN_POINT('Ctrl Pts',(-61.0441813777723,-34.2579614092497,
0.));
#140631=CARTESIAN_POINT('Ctrl Pts',(-61.0441813777723,-34.2579614092497,
12.));
#140632=CARTESIAN_POINT('',(-61.0441813777723,-34.2579614092497,12.));
#140633=CARTESIAN_POINT('Ctrl Pts',(-61.0441813777723,-34.2579614092497,
12.));
#140634=CARTESIAN_POINT('Ctrl Pts',(-61.0479423318803,-34.2589297755482,
12.));
#140635=CARTESIAN_POINT('Ctrl Pts',(-61.0554700177206,-34.2608658001761,
12.));
#140636=CARTESIAN_POINT('Ctrl Pts',(-61.0667788793594,-34.2637677132139,
12.));
#140637=CARTESIAN_POINT('Ctrl Pts',(-61.0818920286644,-34.2676326825846,
12.));
#140638=CARTESIAN_POINT('Ctrl Pts',(-61.100841240023,-34.2724568037374,
12.));
#140639=CARTESIAN_POINT('Ctrl Pts',(-61.119848199783,-34.2772738038811,
12.));
#140640=CARTESIAN_POINT('Ctrl Pts',(-61.1389128461815,-34.2820836244425,
12.));
#140641=CARTESIAN_POINT('Ctrl Pts',(-61.15803506354,-34.2868861666301,12.));
#140642=CARTESIAN_POINT('Ctrl Pts',(-61.1772146833083,-34.2916812929675,
12.));
#140643=CARTESIAN_POINT('Ctrl Pts',(-61.1964515073823,-34.296468844362,
12.));
#140644=CARTESIAN_POINT('Ctrl Pts',(-61.2157453259107,-34.3012486533474,
12.));
#140645=CARTESIAN_POINT('Ctrl Pts',(-61.2350959366987,-34.3060205584093,
12.));
#140646=CARTESIAN_POINT('Ctrl Pts',(-61.2545031656196,-34.3107844191081,
12.));
#140647=CARTESIAN_POINT('Ctrl Pts',(-61.2739668600415,-34.3155401111776,
12.));
#140648=CARTESIAN_POINT('Ctrl Pts',(-61.2934868791875,-34.3202875193629,
12.));
#140649=CARTESIAN_POINT('Ctrl Pts',(-61.3130630861375,-34.3250265314761,
12.));
#140650=CARTESIAN_POINT('Ctrl Pts',(-61.3326953378817,-34.3297570310126,
12.));
#140651=CARTESIAN_POINT('Ctrl Pts',(-61.3523834803144,-34.3344788934337,
12.));
#140652=CARTESIAN_POINT('Ctrl Pts',(-61.3721273534222,-34.339191990012,
12.));
#140653=CARTESIAN_POINT('Ctrl Pts',(-61.3919267945293,-34.34389619024,12.));
#140654=CARTESIAN_POINT('Ctrl Pts',(-61.4117816420251,-34.3485913645991,
12.));
#140655=CARTESIAN_POINT('Ctrl Pts',(-61.4316917395959,-34.3532773877112,
12.));
#140656=CARTESIAN_POINT('Ctrl Pts',(-61.4516569360499,-34.357954138202,
12.));
#140657=CARTESIAN_POINT('Ctrl Pts',(-61.4716770832924,-34.3626214971903,
12.));
#140658=CARTESIAN_POINT('Ctrl Pts',(-61.4917520349276,-34.3672793472463,
12.));
#140659=CARTESIAN_POINT('Ctrl Pts',(-61.511881644541,-34.3719275711179,
12.));
#140660=CARTESIAN_POINT('Ctrl Pts',(-61.5320657642601,-34.3765660506659,
12.));
#140661=CARTESIAN_POINT('Ctrl Pts',(-61.5523042455127,-34.3811946674179,
12.));
#140662=CARTESIAN_POINT('Ctrl Pts',(-61.5725969396817,-34.3858133030511,
12.));
#140663=CARTESIAN_POINT('Ctrl Pts',(-61.5929436987419,-34.3904218398642,
12.));
#140664=CARTESIAN_POINT('Ctrl Pts',(-61.6133443760168,-34.3950201613446,
12.));
#140665=CARTESIAN_POINT('Ctrl Pts',(-61.6337988264586,-34.399608152377,
12.));
#140666=CARTESIAN_POINT('Ctrl Pts',(-61.6543069062436,-34.4041856989328,
12.));
#140667=CARTESIAN_POINT('Ctrl Pts',(-61.674868472521,-34.4087526878815,
12.));
#140668=CARTESIAN_POINT('Ctrl Pts',(-61.6954833831157,-34.4133090067696,
12.));
#140669=CARTESIAN_POINT('Ctrl Pts',(-61.7161514961892,-34.4178545435753,
12.));
#140670=CARTESIAN_POINT('Ctrl Pts',(-61.7368726702573,-34.4223891867166,
12.));
#140671=CARTESIAN_POINT('Ctrl Pts',(-61.7576467643419,-34.4269128251569,
12.));
#140672=CARTESIAN_POINT('Ctrl Pts',(-61.7784736380727,-34.4314253484791,
12.));
#140673=CARTESIAN_POINT('Ctrl Pts',(-61.7993531518052,-34.4359266469757,
12.));
#140674=CARTESIAN_POINT('Ctrl Pts',(-61.8202851667247,-34.4404166117313,
12.));
#140675=CARTESIAN_POINT('Ctrl Pts',(-61.8412695447951,-34.4448951345753,
12.));
#140676=CARTESIAN_POINT('Ctrl Pts',(-61.862306148703,-34.4493621080367,
12.));
#140677=CARTESIAN_POINT('Ctrl Pts',(-61.883394841802,-34.4538174253009,
12.));
#140678=CARTESIAN_POINT('Ctrl Pts',(-61.9045354880424,-34.4582609801625,
12.));
#140679=CARTESIAN_POINT('Ctrl Pts',(-61.9257279519283,-34.462692666996,
12.));
#140680=CARTESIAN_POINT('Ctrl Pts',(-61.9469720985512,-34.4671123807706,
12.));
#140681=CARTESIAN_POINT('Ctrl Pts',(-61.9682677936048,-34.4715200170589,
12.));
#140682=CARTESIAN_POINT('Ctrl Pts',(-61.9896149034009,-34.4759154720477,
12.));
#140683=CARTESIAN_POINT('Ctrl Pts',(-62.0110132948807,-34.4802986425535,
12.));
#140684=CARTESIAN_POINT('Ctrl Pts',(-62.0324628356152,-34.4846694260205,
12.));
#140685=CARTESIAN_POINT('Ctrl Pts',(-62.0539633937944,-34.4890277205041,
12.));
#140686=CARTESIAN_POINT('Ctrl Pts',(-62.0755148382136,-34.4933734246592,
12.));
#140687=CARTESIAN_POINT('Ctrl Pts',(-62.0971170382565,-34.4977064377281,
12.));
#140688=CARTESIAN_POINT('Ctrl Pts',(-62.1187698638705,-34.5020266595292,
12.));
#140689=CARTESIAN_POINT('Ctrl Pts',(-62.1404731855686,-34.5063339904533,
12.));
#140690=CARTESIAN_POINT('Ctrl Pts',(-62.1622268744336,-34.5106283314594,
12.));
#140691=CARTESIAN_POINT('Ctrl Pts',(-62.1840308021171,-34.5149095840729,
12.));
#140692=CARTESIAN_POINT('Ctrl Pts',(-62.2058848408347,-34.5191776503842,
12.));
#140693=CARTESIAN_POINT('Ctrl Pts',(-62.2277888633576,-34.523432433049,
12.));
#140694=CARTESIAN_POINT('Ctrl Pts',(-62.2497427430135,-34.5276738352808,
12.));
#140695=CARTESIAN_POINT('Ctrl Pts',(-62.2717463536827,-34.5319017608433,
12.));
#140696=CARTESIAN_POINT('Ctrl Pts',(-62.2937995697925,-34.5361161140449,
12.));
#140697=CARTESIAN_POINT('Ctrl Pts',(-62.3159022663058,-34.5403167997337,
12.));
#140698=CARTESIAN_POINT('Ctrl Pts',(-62.338054318708,-34.5445037232936,
12.));
#140699=CARTESIAN_POINT('Ctrl Pts',(-62.3602556030127,-34.5486767906384,
12.));
#140700=CARTESIAN_POINT('Ctrl Pts',(-62.3825059957601,-34.5528359082075,
12.));
#140701=CARTESIAN_POINT('Ctrl Pts',(-62.4048053740127,-34.5569809829613,
12.));
#140702=CARTESIAN_POINT('Ctrl Pts',(-62.4271536153459,-34.5611119223798,
12.));
#140703=CARTESIAN_POINT('Ctrl Pts',(-62.4495505978393,-34.5652286344593,
12.));
#140704=CARTESIAN_POINT('Ctrl Pts',(-62.4719962000808,-34.5693310277051,
12.));
#140705=CARTESIAN_POINT('Ctrl Pts',(-62.4944903011628,-34.5734190111272,
12.));
#140706=CARTESIAN_POINT('Ctrl Pts',(-62.5170327806781,-34.5774924942355,
12.));
#140707=CARTESIAN_POINT('Ctrl Pts',(-62.5396235187079,-34.5815513870377,
12.));
#140708=CARTESIAN_POINT('Ctrl Pts',(-62.562262395816,-34.5855956000363,
12.));
#140709=CARTESIAN_POINT('Ctrl Pts',(-62.5849492930533,-34.5896250442216,
12.));
#140710=CARTESIAN_POINT('Ctrl Pts',(-62.6076840919536,-34.5936396310679,
12.));
#140711=CARTESIAN_POINT('Ctrl Pts',(-62.6304666745306,-34.5976392725296,
12.));
#140712=CARTESIAN_POINT('Ctrl Pts',(-62.6532969232657,-34.6016238810398,
12.));
#140713=CARTESIAN_POINT('Ctrl Pts',(-62.6761747211037,-34.6055933695069,
12.));
#140714=CARTESIAN_POINT('Ctrl Pts',(-62.6990999514563,-34.6095476513077,
12.));
#140715=CARTESIAN_POINT('Ctrl Pts',(-62.7220724981994,-34.6134866402837,
12.));
#140716=CARTESIAN_POINT('Ctrl Pts',(-62.7450922456676,-34.6174102507375,
12.));
#140717=CARTESIAN_POINT('Ctrl Pts',(-62.7681590786429,-34.6213183974317,
12.));
#140718=CARTESIAN_POINT('Ctrl Pts',(-62.7912728823518,-34.6252109955853,
12.));
#140719=CARTESIAN_POINT('Ctrl Pts',(-62.8144335424697,-34.6290879608673,
12.));
#140720=CARTESIAN_POINT('Ctrl Pts',(-62.8376409451175,-34.6329492093935,
12.));
#140721=CARTESIAN_POINT('Ctrl Pts',(-62.8608949768571,-34.6367946577235,
12.));
#140722=CARTESIAN_POINT('Ctrl Pts',(-62.8841955246794,-34.6406242228592,
12.));
#140723=CARTESIAN_POINT('Ctrl Pts',(-62.9075424760015,-34.644437822241,
12.));
#140724=CARTESIAN_POINT('Ctrl Pts',(-62.9309357186717,-34.6482353737424,
12.));
#140725=CARTESIAN_POINT('Ctrl Pts',(-62.9543751409646,-34.6520167956655,
12.));
#140726=CARTESIAN_POINT('Ctrl Pts',(-62.9778606315783,-34.6557820067393,
12.));
#140727=CARTESIAN_POINT('Ctrl Pts',(-63.0013920796235,-34.6595309261191,
12.));
#140728=CARTESIAN_POINT('Ctrl Pts',(-63.0249693746208,-34.6632634733824,
12.));
#140729=CARTESIAN_POINT('Ctrl Pts',(-63.0485924065045,-34.6669795685228,
12.));
#140730=CARTESIAN_POINT('Ctrl Pts',(-63.0722610656194,-34.670679131947,
12.));
#140731=CARTESIAN_POINT('Ctrl Pts',(-63.0959752427168,-34.674362084472,
12.));
#140732=CARTESIAN_POINT('Ctrl Pts',(-63.119734828943,-34.6780283473252,
12.));
#140733=CARTESIAN_POINT('Ctrl Pts',(-63.1435397158388,-34.6816778421402,
12.));
#140734=CARTESIAN_POINT('Ctrl Pts',(-63.1673897953429,-34.6853104909518,
12.));
#140735=CARTESIAN_POINT('Ctrl Pts',(-63.1912849597887,-34.6889262161924,
12.));
#140736=CARTESIAN_POINT('Ctrl Pts',(-63.2152251019012,-34.6925249406897,
12.));
#140737=CARTESIAN_POINT('Ctrl Pts',(-63.2392101147847,-34.6961065876666,
12.));
#140738=CARTESIAN_POINT('Ctrl Pts',(-63.2632398919225,-34.6996710807378,
12.));
#140739=CARTESIAN_POINT('Ctrl Pts',(-63.2873143271807,-34.703218343904,
12.));
#140740=CARTESIAN_POINT('Ctrl Pts',(-63.3114333148048,-34.7067483015491,
12.));
#140741=CARTESIAN_POINT('Ctrl Pts',(-63.3355967494171,-34.7102608784374,
12.));
#140742=CARTESIAN_POINT('Ctrl Pts',(-63.3598045260053,-34.7137559997146,
12.));
#140743=CARTESIAN_POINT('Ctrl Pts',(-63.3840565399208,-34.7172335909038,
12.));
#140744=CARTESIAN_POINT('Ctrl Pts',(-63.4083526868836,-34.7206935779007,
12.));
#140745=CARTESIAN_POINT('Ctrl Pts',(-63.4326928629795,-34.7241358869701,
12.));
#140746=CARTESIAN_POINT('Ctrl Pts',(-63.4570769646569,-34.7275604447438,
12.));
#140747=CARTESIAN_POINT('Ctrl Pts',(-63.4815048887165,-34.7309671782214,
12.));
#140748=CARTESIAN_POINT('Ctrl Pts',(-63.505976532309,-34.7343560147667,
12.));
#140749=CARTESIAN_POINT('Ctrl Pts',(-63.5304917929386,-34.7377268821025,
12.));
#140750=CARTESIAN_POINT('Ctrl Pts',(-63.5550505684626,-34.7410797083081,
12.));
#140751=CARTESIAN_POINT('Ctrl Pts',(-63.5796527570871,-34.744414421816,
12.));
#140752=CARTESIAN_POINT('Ctrl Pts',(-63.6042982573588,-34.7477309514136,
12.));
#140753=CARTESIAN_POINT('Ctrl Pts',(-63.6289869681604,-34.7510292262406,
12.));
#140754=CARTESIAN_POINT('Ctrl Pts',(-63.6537187887159,-34.7543091757833,
12.));
#140755=CARTESIAN_POINT('Ctrl Pts',(-63.6784936185885,-34.7575707298713,
12.));
#140756=CARTESIAN_POINT('Ctrl Pts',(-63.7033113576785,-34.7608138186759,
12.));
#140757=CARTESIAN_POINT('Ctrl Pts',(-63.7281719062149,-34.76403837271,12.));
#140758=CARTESIAN_POINT('Ctrl Pts',(-63.7530751647494,-34.7672443228275,
12.));
#140759=CARTESIAN_POINT('Ctrl Pts',(-63.778021034163,-34.7704316002171,
12.));
#140760=CARTESIAN_POINT('Ctrl Pts',(-63.8030094156639,-34.7736001363993,
12.));
#140761=CARTESIAN_POINT('Ctrl Pts',(-63.8280402107856,-34.7767498632243,
12.));
#140762=CARTESIAN_POINT('Ctrl Pts',(-63.8531133213793,-34.7798807128715,
12.));
#140763=CARTESIAN_POINT('Ctrl Pts',(-63.8782286496062,-34.7829926178496,
12.));
#140764=CARTESIAN_POINT('Ctrl Pts',(-63.9033860979435,-34.7860855109911,
12.));
#140765=CARTESIAN_POINT('Ctrl Pts',(-63.9285855691845,-34.7891593254488,
12.));
#140766=CARTESIAN_POINT('Ctrl Pts',(-63.9538269664366,-34.7922139946943,
12.));
#140767=CARTESIAN_POINT('Ctrl Pts',(-63.9791101931162,-34.7952494525177,
12.));
#140768=CARTESIAN_POINT('Ctrl Pts',(-64.0044351529402,-34.7982656330293,
12.));
#140769=CARTESIAN_POINT('Ctrl Pts',(-64.0298017499294,-34.8012624706526,
12.));
#140770=CARTESIAN_POINT('Ctrl Pts',(-64.0552098884095,-34.8042399001211,
12.));
#140771=CARTESIAN_POINT('Ctrl Pts',(-64.0806594730085,-34.8071978564747,
12.));
#140772=CARTESIAN_POINT('Ctrl Pts',(-64.1061504086515,-34.8101362750597,
12.));
#140773=CARTESIAN_POINT('Ctrl Pts',(-64.1316826005506,-34.8130550915287,
12.));
#140774=CARTESIAN_POINT('Ctrl Pts',(-64.1572559542086,-34.8159542418374,
12.));
#140775=CARTESIAN_POINT('Ctrl Pts',(-64.1828703754236,-34.8188336622419,
12.));
#140776=CARTESIAN_POINT('Ctrl Pts',(-64.2085257702884,-34.8216932892968,
12.));
#140777=CARTESIAN_POINT('Ctrl Pts',(-64.234222045188,-34.8245330598559,
12.));
#140778=CARTESIAN_POINT('Ctrl Pts',(-64.2599591067916,-34.8273529110744,
12.));
#140779=CARTESIAN_POINT('Ctrl Pts',(-64.285736862052,-34.8301527804054,
12.));
#140780=CARTESIAN_POINT('Ctrl Pts',(-64.3115552182062,-34.8329326055919,
12.));
#140781=CARTESIAN_POINT('Ctrl Pts',(-64.3374140827711,-34.8356923246618,
12.));
#140782=CARTESIAN_POINT('Ctrl Pts',(-64.3633133635382,-34.8384318759248,
12.));
#140783=CARTESIAN_POINT('Ctrl Pts',(-64.3892529685607,-34.8411511979702,
12.));
#140784=CARTESIAN_POINT('Ctrl Pts',(-64.4152328061515,-34.8438502296664,
12.));
#140785=CARTESIAN_POINT('Ctrl Pts',(-64.4412527848969,-34.8465289101621,
12.));
#140786=CARTESIAN_POINT('Ctrl Pts',(-64.4673128136625,-34.8491871788895,
12.));
#140787=CARTESIAN_POINT('Ctrl Pts',(-64.4934128015985,-34.851824975568,
12.));
#140788=CARTESIAN_POINT('Ctrl Pts',(-64.5195526581407,-34.8544422402118,
12.));
#140789=CARTESIAN_POINT('Ctrl Pts',(-64.5457322930088,-34.857038913134,
12.));
#140790=CARTESIAN_POINT('Ctrl Pts',(-64.5719516161927,-34.8596149349256,
12.));
#140791=CARTESIAN_POINT('Ctrl Pts',(-64.5982105379383,-34.8621702464401,
12.));
#140792=CARTESIAN_POINT('Ctrl Pts',(-64.6245089687277,-34.8647047887774,
12.));
#140793=CARTESIAN_POINT('Ctrl Pts',(-64.6508468192599,-34.867218503272,
12.));
#140794=CARTESIAN_POINT('Ctrl Pts',(-64.6772240004228,-34.869711331479,
12.));
#140795=CARTESIAN_POINT('Ctrl Pts',(-64.7036404233306,-34.8721832151974,
12.));
#140796=CARTESIAN_POINT('Ctrl Pts',(-64.7300959993653,-34.8746340964971,
12.));
#140797=CARTESIAN_POINT('Ctrl Pts',(-64.7565906402151,-34.8770639177493,
12.));
#140798=CARTESIAN_POINT('Ctrl Pts',(-64.7831242579028,-34.8794726216513,
12.));
#140799=CARTESIAN_POINT('Ctrl Pts',(-64.8096967648307,-34.881860151273,
12.));
#140800=CARTESIAN_POINT('Ctrl Pts',(-64.8363080737377,-34.8842264500188,
12.));
#140801=CARTESIAN_POINT('Ctrl Pts',(-64.8629580976063,-34.8865714615436,
12.));
#140802=CARTESIAN_POINT('Ctrl Pts',(-64.8896467495757,-34.888895129681,
12.));
#140803=CARTESIAN_POINT('Ctrl Pts',(-64.9163739428605,-34.8911973983785,
12.));
#140804=CARTESIAN_POINT('Ctrl Pts',(-64.9431395906337,-34.8934782116095,
12.));
#140805=CARTESIAN_POINT('Ctrl Pts',(-64.9699436060169,-34.8957375133697,
12.));
#140806=CARTESIAN_POINT('Ctrl Pts',(-64.9967859023212,-34.8979752478616,
12.));
#140807=CARTESIAN_POINT('Ctrl Pts',(-65.0236663932328,-34.9001913596416,
12.));
#140808=CARTESIAN_POINT('Ctrl Pts',(-65.0505849930171,-34.9023857937865,
12.));
#140809=CARTESIAN_POINT('Ctrl Pts',(-65.0775416167085,-34.9045584960509,
12.));
#140810=CARTESIAN_POINT('Ctrl Pts',(-65.1045361803121,-34.9067094130399,
12.));
#140811=CARTESIAN_POINT('Ctrl Pts',(-65.1315686003516,-34.9088384918336,
12.));
#140812=CARTESIAN_POINT('Ctrl Pts',(-65.1586387934241,-34.9109456796213,
12.));
#140813=CARTESIAN_POINT('Ctrl Pts',(-65.1857466757092,-34.9130309233022,
12.));
#140814=CARTESIAN_POINT('Ctrl Pts',(-65.2128921625823,-34.9150941691747,
12.));
#140815=CARTESIAN_POINT('Ctrl Pts',(-65.2400751679549,-34.9171353624113,
12.));
#140816=CARTESIAN_POINT('Ctrl Pts',(-65.2672956048069,-34.9191544474872,
12.));
#140817=CARTESIAN_POINT('Ctrl Pts',(-65.2945533863761,-34.9211513691355,
12.));
#140818=CARTESIAN_POINT('Ctrl Pts',(-65.321848427191,-34.9231260731831,
12.));
#140819=CARTESIAN_POINT('Ctrl Pts',(-65.3491806440537,-34.9250785073477,
12.));
#140820=CARTESIAN_POINT('Ctrl Pts',(-65.3765499573077,-34.9270086222731,
12.));
#140821=CARTESIAN_POINT('Ctrl Pts',(-65.4039562911352,-34.9289163717747,
12.));
#140822=CARTESIAN_POINT('Ctrl Pts',(-65.4274804996589,-34.9305324724445,
12.));
#140823=CARTESIAN_POINT('Ctrl Pts',(-65.4455359575245,-34.931759381316,
12.));
#140824=CARTESIAN_POINT('Ctrl Pts',(-65.4581063193883,-34.9326070346645,
12.));
#140825=CARTESIAN_POINT('Ctrl Pts',(-65.4651808010811,-34.9330820191535,
12.));
#140826=CARTESIAN_POINT('Ctrl Pts',(-65.4667541478385,-34.933187552314,
12.));
#140827=CARTESIAN_POINT('',(-61.0441813777723,-34.2579614092497,0.));
#140828=CARTESIAN_POINT('',(-61.0441813777723,-34.2579614092497,0.));
#140829=CARTESIAN_POINT('Ctrl Pts',(-65.4667541478385,-34.933187552314,
0.));
#140830=CARTESIAN_POINT('Ctrl Pts',(-65.465180801081,-34.9330820191535,
0.));
#140831=CARTESIAN_POINT('Ctrl Pts',(-65.4581063193883,-34.9326070346645,
0.));
#140832=CARTESIAN_POINT('Ctrl Pts',(-65.4455359575245,-34.931759381316,
0.));
#140833=CARTESIAN_POINT('Ctrl Pts',(-65.4274804996589,-34.9305324724445,
0.));
#140834=CARTESIAN_POINT('Ctrl Pts',(-65.4039562911352,-34.9289163717747,
0.));
#140835=CARTESIAN_POINT('Ctrl Pts',(-65.3765499573077,-34.9270086222731,
0.));
#140836=CARTESIAN_POINT('Ctrl Pts',(-65.3491806440537,-34.9250785073477,
0.));
#140837=CARTESIAN_POINT('Ctrl Pts',(-65.321848427191,-34.9231260731831,
0.));
#140838=CARTESIAN_POINT('Ctrl Pts',(-65.2945533863761,-34.9211513691355,
0.));
#140839=CARTESIAN_POINT('Ctrl Pts',(-65.2672956048069,-34.9191544474872,
0.));
#140840=CARTESIAN_POINT('Ctrl Pts',(-65.2400751679549,-34.9171353624113,
0.));
#140841=CARTESIAN_POINT('Ctrl Pts',(-65.2128921625823,-34.9150941691747,
0.));
#140842=CARTESIAN_POINT('Ctrl Pts',(-65.1857466757092,-34.9130309233022,
0.));
#140843=CARTESIAN_POINT('Ctrl Pts',(-65.1586387934241,-34.9109456796213,
0.));
#140844=CARTESIAN_POINT('Ctrl Pts',(-65.1315686003516,-34.9088384918336,
0.));
#140845=CARTESIAN_POINT('Ctrl Pts',(-65.1045361803121,-34.9067094130399,
0.));
#140846=CARTESIAN_POINT('Ctrl Pts',(-65.0775416167085,-34.9045584960509,
0.));
#140847=CARTESIAN_POINT('Ctrl Pts',(-65.0505849930171,-34.9023857937865,
0.));
#140848=CARTESIAN_POINT('Ctrl Pts',(-65.0236663932328,-34.9001913596416,
0.));
#140849=CARTESIAN_POINT('Ctrl Pts',(-64.9967859023212,-34.8979752478616,
0.));
#140850=CARTESIAN_POINT('Ctrl Pts',(-64.9699436060169,-34.8957375133697,
0.));
#140851=CARTESIAN_POINT('Ctrl Pts',(-64.9431395906337,-34.8934782116095,
0.));
#140852=CARTESIAN_POINT('Ctrl Pts',(-64.9163739428605,-34.8911973983785,
0.));
#140853=CARTESIAN_POINT('Ctrl Pts',(-64.8896467495757,-34.888895129681,
0.));
#140854=CARTESIAN_POINT('Ctrl Pts',(-64.8629580976063,-34.8865714615436,
0.));
#140855=CARTESIAN_POINT('Ctrl Pts',(-64.8363080737377,-34.8842264500188,
0.));
#140856=CARTESIAN_POINT('Ctrl Pts',(-64.8096967648307,-34.881860151273,
0.));
#140857=CARTESIAN_POINT('Ctrl Pts',(-64.7831242579028,-34.8794726216513,
0.));
#140858=CARTESIAN_POINT('Ctrl Pts',(-64.7565906402151,-34.8770639177493,
0.));
#140859=CARTESIAN_POINT('Ctrl Pts',(-64.7300959993653,-34.8746340964971,
0.));
#140860=CARTESIAN_POINT('Ctrl Pts',(-64.7036404233306,-34.8721832151974,
0.));
#140861=CARTESIAN_POINT('Ctrl Pts',(-64.6772240004228,-34.869711331479,
0.));
#140862=CARTESIAN_POINT('Ctrl Pts',(-64.6508468192599,-34.867218503272,
0.));
#140863=CARTESIAN_POINT('Ctrl Pts',(-64.6245089687277,-34.8647047887774,
0.));
#140864=CARTESIAN_POINT('Ctrl Pts',(-64.5982105379383,-34.8621702464401,
0.));
#140865=CARTESIAN_POINT('Ctrl Pts',(-64.5719516161927,-34.8596149349256,
0.));
#140866=CARTESIAN_POINT('Ctrl Pts',(-64.5457322930088,-34.857038913134,
0.));
#140867=CARTESIAN_POINT('Ctrl Pts',(-64.5195526581407,-34.8544422402118,
0.));
#140868=CARTESIAN_POINT('Ctrl Pts',(-64.4934128015985,-34.851824975568,
0.));
#140869=CARTESIAN_POINT('Ctrl Pts',(-64.4673128136625,-34.8491871788895,
0.));
#140870=CARTESIAN_POINT('Ctrl Pts',(-64.4412527848969,-34.8465289101621,
0.));
#140871=CARTESIAN_POINT('Ctrl Pts',(-64.4152328061515,-34.8438502296664,
0.));
#140872=CARTESIAN_POINT('Ctrl Pts',(-64.3892529685607,-34.8411511979702,
0.));
#140873=CARTESIAN_POINT('Ctrl Pts',(-64.3633133635382,-34.8384318759248,
0.));
#140874=CARTESIAN_POINT('Ctrl Pts',(-64.3374140827711,-34.8356923246618,
0.));
#140875=CARTESIAN_POINT('Ctrl Pts',(-64.3115552182062,-34.8329326055919,
0.));
#140876=CARTESIAN_POINT('Ctrl Pts',(-64.285736862052,-34.8301527804054,
0.));
#140877=CARTESIAN_POINT('Ctrl Pts',(-64.2599591067916,-34.8273529110744,
0.));
#140878=CARTESIAN_POINT('Ctrl Pts',(-64.234222045188,-34.8245330598559,
0.));
#140879=CARTESIAN_POINT('Ctrl Pts',(-64.2085257702884,-34.8216932892968,
0.));
#140880=CARTESIAN_POINT('Ctrl Pts',(-64.1828703754236,-34.8188336622419,
0.));
#140881=CARTESIAN_POINT('Ctrl Pts',(-64.1572559542086,-34.8159542418374,
0.));
#140882=CARTESIAN_POINT('Ctrl Pts',(-64.1316826005506,-34.8130550915287,
0.));
#140883=CARTESIAN_POINT('Ctrl Pts',(-64.1061504086515,-34.8101362750597,
0.));
#140884=CARTESIAN_POINT('Ctrl Pts',(-64.0806594730085,-34.8071978564747,
0.));
#140885=CARTESIAN_POINT('Ctrl Pts',(-64.0552098884095,-34.8042399001211,
0.));
#140886=CARTESIAN_POINT('Ctrl Pts',(-64.0298017499294,-34.8012624706526,
0.));
#140887=CARTESIAN_POINT('Ctrl Pts',(-64.0044351529402,-34.7982656330293,
0.));
#140888=CARTESIAN_POINT('Ctrl Pts',(-63.9791101931162,-34.7952494525177,
0.));
#140889=CARTESIAN_POINT('Ctrl Pts',(-63.9538269664366,-34.7922139946943,
0.));
#140890=CARTESIAN_POINT('Ctrl Pts',(-63.9285855691845,-34.7891593254488,
0.));
#140891=CARTESIAN_POINT('Ctrl Pts',(-63.9033860979435,-34.7860855109911,
0.));
#140892=CARTESIAN_POINT('Ctrl Pts',(-63.8782286496062,-34.7829926178496,
0.));
#140893=CARTESIAN_POINT('Ctrl Pts',(-63.8531133213793,-34.7798807128715,
0.));
#140894=CARTESIAN_POINT('Ctrl Pts',(-63.8280402107856,-34.7767498632243,
0.));
#140895=CARTESIAN_POINT('Ctrl Pts',(-63.8030094156639,-34.7736001363993,
0.));
#140896=CARTESIAN_POINT('Ctrl Pts',(-63.778021034163,-34.7704316002171,
0.));
#140897=CARTESIAN_POINT('Ctrl Pts',(-63.7530751647494,-34.7672443228275,
0.));
#140898=CARTESIAN_POINT('Ctrl Pts',(-63.7281719062149,-34.76403837271,0.));
#140899=CARTESIAN_POINT('Ctrl Pts',(-63.7033113576785,-34.7608138186759,
0.));
#140900=CARTESIAN_POINT('Ctrl Pts',(-63.6784936185885,-34.7575707298713,
0.));
#140901=CARTESIAN_POINT('Ctrl Pts',(-63.6537187887159,-34.7543091757833,
0.));
#140902=CARTESIAN_POINT('Ctrl Pts',(-63.6289869681604,-34.7510292262406,
0.));
#140903=CARTESIAN_POINT('Ctrl Pts',(-63.6042982573588,-34.7477309514136,
0.));
#140904=CARTESIAN_POINT('Ctrl Pts',(-63.5796527570871,-34.744414421816,
0.));
#140905=CARTESIAN_POINT('Ctrl Pts',(-63.5550505684626,-34.7410797083081,
0.));
#140906=CARTESIAN_POINT('Ctrl Pts',(-63.5304917929386,-34.7377268821025,
0.));
#140907=CARTESIAN_POINT('Ctrl Pts',(-63.505976532309,-34.7343560147667,
0.));
#140908=CARTESIAN_POINT('Ctrl Pts',(-63.4815048887165,-34.7309671782214,
0.));
#140909=CARTESIAN_POINT('Ctrl Pts',(-63.4570769646569,-34.7275604447438,
0.));
#140910=CARTESIAN_POINT('Ctrl Pts',(-63.4326928629795,-34.7241358869701,
0.));
#140911=CARTESIAN_POINT('Ctrl Pts',(-63.4083526868836,-34.7206935779007,
0.));
#140912=CARTESIAN_POINT('Ctrl Pts',(-63.3840565399208,-34.7172335909038,
0.));
#140913=CARTESIAN_POINT('Ctrl Pts',(-63.3598045260053,-34.7137559997146,
0.));
#140914=CARTESIAN_POINT('Ctrl Pts',(-63.3355967494171,-34.7102608784374,
0.));
#140915=CARTESIAN_POINT('Ctrl Pts',(-63.3114333148048,-34.7067483015491,
0.));
#140916=CARTESIAN_POINT('Ctrl Pts',(-63.2873143271807,-34.703218343904,
0.));
#140917=CARTESIAN_POINT('Ctrl Pts',(-63.2632398919225,-34.6996710807378,
0.));
#140918=CARTESIAN_POINT('Ctrl Pts',(-63.2392101147847,-34.6961065876666,
0.));
#140919=CARTESIAN_POINT('Ctrl Pts',(-63.2152251019012,-34.6925249406897,
0.));
#140920=CARTESIAN_POINT('Ctrl Pts',(-63.1912849597887,-34.6889262161924,
0.));
#140921=CARTESIAN_POINT('Ctrl Pts',(-63.1673897953429,-34.6853104909518,
0.));
#140922=CARTESIAN_POINT('Ctrl Pts',(-63.1435397158388,-34.6816778421402,
0.));
#140923=CARTESIAN_POINT('Ctrl Pts',(-63.119734828943,-34.6780283473252,
0.));
#140924=CARTESIAN_POINT('Ctrl Pts',(-63.0959752427168,-34.674362084472,
0.));
#140925=CARTESIAN_POINT('Ctrl Pts',(-63.0722610656194,-34.670679131947,
0.));
#140926=CARTESIAN_POINT('Ctrl Pts',(-63.0485924065045,-34.6669795685228,
0.));
#140927=CARTESIAN_POINT('Ctrl Pts',(-63.0249693746208,-34.6632634733824,
0.));
#140928=CARTESIAN_POINT('Ctrl Pts',(-63.0013920796235,-34.6595309261191,
0.));
#140929=CARTESIAN_POINT('Ctrl Pts',(-62.9778606315783,-34.6557820067393,
0.));
#140930=CARTESIAN_POINT('Ctrl Pts',(-62.9543751409646,-34.6520167956655,
0.));
#140931=CARTESIAN_POINT('Ctrl Pts',(-62.9309357186717,-34.6482353737424,
0.));
#140932=CARTESIAN_POINT('Ctrl Pts',(-62.9075424760015,-34.644437822241,
0.));
#140933=CARTESIAN_POINT('Ctrl Pts',(-62.8841955246794,-34.6406242228592,
0.));
#140934=CARTESIAN_POINT('Ctrl Pts',(-62.8608949768571,-34.6367946577235,
0.));
#140935=CARTESIAN_POINT('Ctrl Pts',(-62.8376409451175,-34.6329492093935,
0.));
#140936=CARTESIAN_POINT('Ctrl Pts',(-62.8144335424697,-34.6290879608673,
0.));
#140937=CARTESIAN_POINT('Ctrl Pts',(-62.7912728823518,-34.6252109955853,
0.));
#140938=CARTESIAN_POINT('Ctrl Pts',(-62.7681590786429,-34.6213183974317,
0.));
#140939=CARTESIAN_POINT('Ctrl Pts',(-62.7450922456676,-34.6174102507375,
0.));
#140940=CARTESIAN_POINT('Ctrl Pts',(-62.7220724981994,-34.6134866402837,
0.));
#140941=CARTESIAN_POINT('Ctrl Pts',(-62.6990999514563,-34.6095476513077,
0.));
#140942=CARTESIAN_POINT('Ctrl Pts',(-62.6761747211037,-34.6055933695069,
0.));
#140943=CARTESIAN_POINT('Ctrl Pts',(-62.6532969232657,-34.6016238810398,
0.));
#140944=CARTESIAN_POINT('Ctrl Pts',(-62.6304666745306,-34.5976392725296,
0.));
#140945=CARTESIAN_POINT('Ctrl Pts',(-62.6076840919536,-34.5936396310679,
0.));
#140946=CARTESIAN_POINT('Ctrl Pts',(-62.5849492930533,-34.5896250442216,
0.));
#140947=CARTESIAN_POINT('Ctrl Pts',(-62.562262395816,-34.5855956000363,
0.));
#140948=CARTESIAN_POINT('Ctrl Pts',(-62.5396235187079,-34.5815513870377,
0.));
#140949=CARTESIAN_POINT('Ctrl Pts',(-62.5170327806781,-34.5774924942355,
0.));
#140950=CARTESIAN_POINT('Ctrl Pts',(-62.4944903011628,-34.5734190111272,
0.));
#140951=CARTESIAN_POINT('Ctrl Pts',(-62.4719962000808,-34.5693310277051,
0.));
#140952=CARTESIAN_POINT('Ctrl Pts',(-62.4495505978393,-34.5652286344593,
0.));
#140953=CARTESIAN_POINT('Ctrl Pts',(-62.4271536153459,-34.5611119223798,
0.));
#140954=CARTESIAN_POINT('Ctrl Pts',(-62.4048053740127,-34.5569809829613,
0.));
#140955=CARTESIAN_POINT('Ctrl Pts',(-62.3825059957601,-34.5528359082075,
0.));
#140956=CARTESIAN_POINT('Ctrl Pts',(-62.3602556030127,-34.5486767906384,
0.));
#140957=CARTESIAN_POINT('Ctrl Pts',(-62.338054318708,-34.5445037232936,
0.));
#140958=CARTESIAN_POINT('Ctrl Pts',(-62.3159022663058,-34.5403167997337,
0.));
#140959=CARTESIAN_POINT('Ctrl Pts',(-62.2937995697925,-34.5361161140449,
0.));
#140960=CARTESIAN_POINT('Ctrl Pts',(-62.2717463536827,-34.5319017608433,
0.));
#140961=CARTESIAN_POINT('Ctrl Pts',(-62.2497427430135,-34.5276738352808,
0.));
#140962=CARTESIAN_POINT('Ctrl Pts',(-62.2277888633576,-34.523432433049,
0.));
#140963=CARTESIAN_POINT('Ctrl Pts',(-62.2058848408347,-34.5191776503842,
0.));
#140964=CARTESIAN_POINT('Ctrl Pts',(-62.1840308021171,-34.5149095840729,
0.));
#140965=CARTESIAN_POINT('Ctrl Pts',(-62.1622268744336,-34.5106283314594,
0.));
#140966=CARTESIAN_POINT('Ctrl Pts',(-62.1404731855686,-34.5063339904533,
0.));
#140967=CARTESIAN_POINT('Ctrl Pts',(-62.1187698638705,-34.5020266595292,
0.));
#140968=CARTESIAN_POINT('Ctrl Pts',(-62.0971170382565,-34.4977064377281,
0.));
#140969=CARTESIAN_POINT('Ctrl Pts',(-62.0755148382136,-34.4933734246592,
0.));
#140970=CARTESIAN_POINT('Ctrl Pts',(-62.0539633937944,-34.4890277205041,
0.));
#140971=CARTESIAN_POINT('Ctrl Pts',(-62.0324628356152,-34.4846694260205,
0.));
#140972=CARTESIAN_POINT('Ctrl Pts',(-62.0110132948807,-34.4802986425535,
0.));
#140973=CARTESIAN_POINT('Ctrl Pts',(-61.9896149034009,-34.4759154720477,
0.));
#140974=CARTESIAN_POINT('Ctrl Pts',(-61.9682677936048,-34.4715200170589,
0.));
#140975=CARTESIAN_POINT('Ctrl Pts',(-61.9469720985512,-34.4671123807706,
0.));
#140976=CARTESIAN_POINT('Ctrl Pts',(-61.9257279519283,-34.462692666996,
0.));
#140977=CARTESIAN_POINT('Ctrl Pts',(-61.9045354880424,-34.4582609801625,
0.));
#140978=CARTESIAN_POINT('Ctrl Pts',(-61.883394841802,-34.4538174253009,
0.));
#140979=CARTESIAN_POINT('Ctrl Pts',(-61.862306148703,-34.4493621080367,
0.));
#140980=CARTESIAN_POINT('Ctrl Pts',(-61.8412695447951,-34.4448951345753,
0.));
#140981=CARTESIAN_POINT('Ctrl Pts',(-61.8202851667247,-34.4404166117313,
0.));
#140982=CARTESIAN_POINT('Ctrl Pts',(-61.7993531518052,-34.4359266469757,
0.));
#140983=CARTESIAN_POINT('Ctrl Pts',(-61.7784736380727,-34.4314253484791,
0.));
#140984=CARTESIAN_POINT('Ctrl Pts',(-61.7576467643419,-34.4269128251569,
0.));
#140985=CARTESIAN_POINT('Ctrl Pts',(-61.7368726702573,-34.4223891867166,
0.));
#140986=CARTESIAN_POINT('Ctrl Pts',(-61.7161514961892,-34.4178545435753,
0.));
#140987=CARTESIAN_POINT('Ctrl Pts',(-61.6954833831157,-34.4133090067696,
0.));
#140988=CARTESIAN_POINT('Ctrl Pts',(-61.674868472521,-34.4087526878815,
0.));
#140989=CARTESIAN_POINT('Ctrl Pts',(-61.6543069062436,-34.4041856989328,
0.));
#140990=CARTESIAN_POINT('Ctrl Pts',(-61.6337988264586,-34.399608152377,
0.));
#140991=CARTESIAN_POINT('Ctrl Pts',(-61.6133443760168,-34.3950201613446,
0.));
#140992=CARTESIAN_POINT('Ctrl Pts',(-61.5929436987419,-34.3904218398642,
0.));
#140993=CARTESIAN_POINT('Ctrl Pts',(-61.5725969396817,-34.3858133030511,
0.));
#140994=CARTESIAN_POINT('Ctrl Pts',(-61.5523042455127,-34.3811946674179,
0.));
#140995=CARTESIAN_POINT('Ctrl Pts',(-61.5320657642601,-34.3765660506659,
0.));
#140996=CARTESIAN_POINT('Ctrl Pts',(-61.511881644541,-34.3719275711179,
0.));
#140997=CARTESIAN_POINT('Ctrl Pts',(-61.4917520349276,-34.3672793472463,
0.));
#140998=CARTESIAN_POINT('Ctrl Pts',(-61.4716770832924,-34.3626214971903,
0.));
#140999=CARTESIAN_POINT('Ctrl Pts',(-61.4516569360499,-34.357954138202,
0.));
#141000=CARTESIAN_POINT('Ctrl Pts',(-61.4316917395959,-34.3532773877112,
0.));
#141001=CARTESIAN_POINT('Ctrl Pts',(-61.4117816420251,-34.3485913645991,
0.));
#141002=CARTESIAN_POINT('Ctrl Pts',(-61.3919267945293,-34.34389619024,0.));
#141003=CARTESIAN_POINT('Ctrl Pts',(-61.3721273534222,-34.339191990012,
0.));
#141004=CARTESIAN_POINT('Ctrl Pts',(-61.3523834803144,-34.3344788934337,
0.));
#141005=CARTESIAN_POINT('Ctrl Pts',(-61.3326953378817,-34.3297570310126,
0.));
#141006=CARTESIAN_POINT('Ctrl Pts',(-61.3130630861375,-34.3250265314761,
0.));
#141007=CARTESIAN_POINT('Ctrl Pts',(-61.2934868791875,-34.3202875193629,
0.));
#141008=CARTESIAN_POINT('Ctrl Pts',(-61.2739668600415,-34.3155401111776,
0.));
#141009=CARTESIAN_POINT('Ctrl Pts',(-61.2545031656196,-34.3107844191081,
0.));
#141010=CARTESIAN_POINT('Ctrl Pts',(-61.2350959366987,-34.3060205584093,
0.));
#141011=CARTESIAN_POINT('Ctrl Pts',(-61.2157453259107,-34.3012486533474,
0.));
#141012=CARTESIAN_POINT('Ctrl Pts',(-61.1964515073823,-34.296468844362,
0.));
#141013=CARTESIAN_POINT('Ctrl Pts',(-61.1772146833083,-34.2916812929675,
0.));
#141014=CARTESIAN_POINT('Ctrl Pts',(-61.15803506354,-34.2868861666301,0.));
#141015=CARTESIAN_POINT('Ctrl Pts',(-61.1389128461815,-34.2820836244425,
0.));
#141016=CARTESIAN_POINT('Ctrl Pts',(-61.119848199783,-34.2772738038811,
0.));
#141017=CARTESIAN_POINT('Ctrl Pts',(-61.100841240023,-34.2724568037374,
0.));
#141018=CARTESIAN_POINT('Ctrl Pts',(-61.0818920286644,-34.2676326825846,
0.));
#141019=CARTESIAN_POINT('Ctrl Pts',(-61.0667788793594,-34.2637677132139,
0.));
#141020=CARTESIAN_POINT('Ctrl Pts',(-61.0554700177206,-34.2608658001761,
0.));
#141021=CARTESIAN_POINT('Ctrl Pts',(-61.0479423318803,-34.2589297755482,
0.));
#141022=CARTESIAN_POINT('Ctrl Pts',(-61.0441813777723,-34.2579614092497,
0.));
#141023=CARTESIAN_POINT('Ctrl Pts',(-68.5875145916629,-29.0861280018229,
0.));
#141024=CARTESIAN_POINT('Ctrl Pts',(-68.5875145916629,-29.0861280018229,
12.));
#141025=CARTESIAN_POINT('Ctrl Pts',(-68.5819214834737,-29.0863005247839,
0.));
#141026=CARTESIAN_POINT('Ctrl Pts',(-68.5819214834737,-29.0863005247839,
12.));
#141027=CARTESIAN_POINT('Ctrl Pts',(-68.5707386600636,-29.0866429722093,
0.));
#141028=CARTESIAN_POINT('Ctrl Pts',(-68.5707386600636,-29.0866429722093,
12.));
#141029=CARTESIAN_POINT('Ctrl Pts',(-68.5539746038542,-29.0871488478588,
0.));
#141030=CARTESIAN_POINT('Ctrl Pts',(-68.5539746038542,-29.0871488478588,
12.));
#141031=CARTESIAN_POINT('Ctrl Pts',(-68.5316428875424,-29.0878077571086,
0.));
#141032=CARTESIAN_POINT('Ctrl Pts',(-68.5316428875424,-29.0878077571086,
12.));
#141033=CARTESIAN_POINT('Ctrl Pts',(-68.5037621824171,-29.0886054060563,
0.));
#141034=CARTESIAN_POINT('Ctrl Pts',(-68.5037621824171,-29.0886054060563,
12.));
#141035=CARTESIAN_POINT('Ctrl Pts',(-68.4759154367939,-29.0893770688944,
0.));
#141036=CARTESIAN_POINT('Ctrl Pts',(-68.4759154367939,-29.0893770688944,
12.));
#141037=CARTESIAN_POINT('Ctrl Pts',(-68.4481026830931,-29.0901227535307,
0.));
#141038=CARTESIAN_POINT('Ctrl Pts',(-68.4481026830931,-29.0901227535307,
12.));
#141039=CARTESIAN_POINT('Ctrl Pts',(-68.4203239694612,-29.090842477089,
0.));
#141040=CARTESIAN_POINT('Ctrl Pts',(-68.4203239694612,-29.090842477089,
12.));
#141041=CARTESIAN_POINT('Ctrl Pts',(-68.3925793637995,-29.0915362699455,
0.));
#141042=CARTESIAN_POINT('Ctrl Pts',(-68.3925793637995,-29.0915362699455,
12.));
#141043=CARTESIAN_POINT('Ctrl Pts',(-68.364868951893,-29.0922041749294,
0.));
#141044=CARTESIAN_POINT('Ctrl Pts',(-68.364868951893,-29.0922041749294,
12.));
#141045=CARTESIAN_POINT('Ctrl Pts',(-68.3371928310161,-29.0928462428145,
0.));
#141046=CARTESIAN_POINT('Ctrl Pts',(-68.3371928310161,-29.0928462428145,
12.));
#141047=CARTESIAN_POINT('Ctrl Pts',(-68.3095511047769,-29.0934625288409,
0.));
#141048=CARTESIAN_POINT('Ctrl Pts',(-68.3095511047769,-29.0934625288409,
12.));
#141049=CARTESIAN_POINT('Ctrl Pts',(-68.2819438775953,-29.0940530889149,
0.));
#141050=CARTESIAN_POINT('Ctrl Pts',(-68.2819438775953,-29.0940530889149,
12.));
#141051=CARTESIAN_POINT('Ctrl Pts',(-68.2543712489906,-29.0946179757167,
0.));
#141052=CARTESIAN_POINT('Ctrl Pts',(-68.2543712489906,-29.0946179757167,
12.));
#141053=CARTESIAN_POINT('Ctrl Pts',(-68.2268333089617,-29.0951572355397,
0.));
#141054=CARTESIAN_POINT('Ctrl Pts',(-68.2268333089617,-29.0951572355397,
12.));
#141055=CARTESIAN_POINT('Ctrl Pts',(-68.1993301412061,-29.0956709104627,
0.));
#141056=CARTESIAN_POINT('Ctrl Pts',(-68.1993301412061,-29.0956709104627,
12.));
#141057=CARTESIAN_POINT('Ctrl Pts',(-68.1718618254281,-29.0961590399046,
0.));
#141058=CARTESIAN_POINT('Ctrl Pts',(-68.1718618254281,-29.0961590399046,
12.));
#141059=CARTESIAN_POINT('Ctrl Pts',(-68.1444284400742,-29.0966216624743,
0.));
#141060=CARTESIAN_POINT('Ctrl Pts',(-68.1444284400742,-29.0966216624743,
12.));
#141061=CARTESIAN_POINT('Ctrl Pts',(-68.1170300646987,-29.0970588175728,
0.));
#141062=CARTESIAN_POINT('Ctrl Pts',(-68.1170300646987,-29.0970588175728,
12.));
#141063=CARTESIAN_POINT('Ctrl Pts',(-68.0896667829567,-29.0974705474259,
0.));
#141064=CARTESIAN_POINT('Ctrl Pts',(-68.0896667829567,-29.0974705474259,
12.));
#141065=CARTESIAN_POINT('Ctrl Pts',(-68.0623386822863,-29.0978568968657,
0.));
#141066=CARTESIAN_POINT('Ctrl Pts',(-68.0623386822863,-29.0978568968657,
12.));
#141067=CARTESIAN_POINT('Ctrl Pts',(-68.0350458525551,-29.0982179124097,
0.));
#141068=CARTESIAN_POINT('Ctrl Pts',(-68.0350458525551,-29.0982179124097,
12.));
#141069=CARTESIAN_POINT('Ctrl Pts',(-68.0077883850121,-29.0985536415531,
0.));
#141070=CARTESIAN_POINT('Ctrl Pts',(-68.0077883850121,-29.0985536415531,
12.));
#141071=CARTESIAN_POINT('Ctrl Pts',(-67.9805663711855,-29.0988641320247,
0.));
#141072=CARTESIAN_POINT('Ctrl Pts',(-67.9805663711855,-29.0988641320247,
12.));
#141073=CARTESIAN_POINT('Ctrl Pts',(-67.9533799016148,-29.0991494309404,
0.));
#141074=CARTESIAN_POINT('Ctrl Pts',(-67.9533799016148,-29.0991494309404,
12.));
#141075=CARTESIAN_POINT('Ctrl Pts',(-67.9262290652829,-29.099409584422,
0.));
#141076=CARTESIAN_POINT('Ctrl Pts',(-67.9262290652829,-29.099409584422,
12.));
#141077=CARTESIAN_POINT('Ctrl Pts',(-67.8991139503193,-29.0996446380626,
0.));
#141078=CARTESIAN_POINT('Ctrl Pts',(-67.8991139503193,-29.0996446380626,
12.));
#141079=CARTESIAN_POINT('Ctrl Pts',(-67.8720346444124,-29.0998546372032,
0.));
#141080=CARTESIAN_POINT('Ctrl Pts',(-67.8720346444124,-29.0998546372032,
12.));
#141081=CARTESIAN_POINT('Ctrl Pts',(-67.8449912353329,-29.1000396272867,
0.));
#141082=CARTESIAN_POINT('Ctrl Pts',(-67.8449912353329,-29.1000396272867,
12.));
#141083=CARTESIAN_POINT('Ctrl Pts',(-67.8179838114099,-29.1001996541842,
0.));
#141084=CARTESIAN_POINT('Ctrl Pts',(-67.8179838114099,-29.1001996541842,
12.));
#141085=CARTESIAN_POINT('Ctrl Pts',(-67.7910124620135,-29.1003347645294,
0.));
#141086=CARTESIAN_POINT('Ctrl Pts',(-67.7910124620135,-29.1003347645294,
12.));
#141087=CARTESIAN_POINT('Ctrl Pts',(-67.7640772773388,-29.1004450055643,
0.));
#141088=CARTESIAN_POINT('Ctrl Pts',(-67.7640772773388,-29.1004450055643,
12.));
#141089=CARTESIAN_POINT('Ctrl Pts',(-67.7371783482035,-29.1005304249987,
0.));
#141090=CARTESIAN_POINT('Ctrl Pts',(-67.7371783482035,-29.1005304249987,
12.));
#141091=CARTESIAN_POINT('Ctrl Pts',(-67.7103157658296,-29.1005910708624,
0.));
#141092=CARTESIAN_POINT('Ctrl Pts',(-67.7103157658296,-29.1005910708624,
12.));
#141093=CARTESIAN_POINT('Ctrl Pts',(-67.6834896216461,-29.1006269913747,
0.));
#141094=CARTESIAN_POINT('Ctrl Pts',(-67.6834896216461,-29.1006269913747,
12.));
#141095=CARTESIAN_POINT('Ctrl Pts',(-67.6567000070326,-29.1006382347814,
0.));
#141096=CARTESIAN_POINT('Ctrl Pts',(-67.6567000070326,-29.1006382347814,
12.));
#141097=CARTESIAN_POINT('Ctrl Pts',(-67.6299470133295,-29.100624849358,
0.));
#141098=CARTESIAN_POINT('Ctrl Pts',(-67.6299470133295,-29.100624849358,
12.));
#141099=CARTESIAN_POINT('Ctrl Pts',(-67.6032307319623,-29.1005868834866,
0.));
#141100=CARTESIAN_POINT('Ctrl Pts',(-67.6032307319623,-29.1005868834866,
12.));
#141101=CARTESIAN_POINT('Ctrl Pts',(-67.5765512545281,-29.1005243857139,
0.));
#141102=CARTESIAN_POINT('Ctrl Pts',(-67.5765512545281,-29.1005243857139,
12.));
#141103=CARTESIAN_POINT('Ctrl Pts',(-67.5499086728888,-29.1004374048148,
0.));
#141104=CARTESIAN_POINT('Ctrl Pts',(-67.5499086728888,-29.1004374048148,
12.));
#141105=CARTESIAN_POINT('Ctrl Pts',(-67.5233030792704,-29.1003259898682,
0.));
#141106=CARTESIAN_POINT('Ctrl Pts',(-67.5233030792704,-29.1003259898682,
12.));
#141107=CARTESIAN_POINT('Ctrl Pts',(-67.4967345663096,-29.1001901902909,
0.));
#141108=CARTESIAN_POINT('Ctrl Pts',(-67.4967345663096,-29.1001901902909,
12.));
#141109=CARTESIAN_POINT('Ctrl Pts',(-67.4702032270048,-29.1000300557955,
0.));
#141110=CARTESIAN_POINT('Ctrl Pts',(-67.4702032270048,-29.1000300557955,
12.));
#141111=CARTESIAN_POINT('Ctrl Pts',(-67.4437091546859,-29.0998456363683,
0.));
#141112=CARTESIAN_POINT('Ctrl Pts',(-67.4437091546859,-29.0998456363683,
12.));
#141113=CARTESIAN_POINT('Ctrl Pts',(-67.4172524429727,-29.0996369822418,
0.));
#141114=CARTESIAN_POINT('Ctrl Pts',(-67.4172524429727,-29.0996369822418,
12.));
#141115=CARTESIAN_POINT('Ctrl Pts',(-67.3908331857323,-29.0994041438719,
0.));
#141116=CARTESIAN_POINT('Ctrl Pts',(-67.3908331857323,-29.0994041438719,
12.));
#141117=CARTESIAN_POINT('Ctrl Pts',(-67.3644514770387,-29.0991471719176,
0.));
#141118=CARTESIAN_POINT('Ctrl Pts',(-67.3644514770387,-29.0991471719176,
12.));
#141119=CARTESIAN_POINT('Ctrl Pts',(-67.3381074112027,-29.0988661172531,
0.));
#141120=CARTESIAN_POINT('Ctrl Pts',(-67.3381074112027,-29.0988661172531,
12.));
#141121=CARTESIAN_POINT('Ctrl Pts',(-67.311801082792,-29.0985610309771,
0.));
#141122=CARTESIAN_POINT('Ctrl Pts',(-67.311801082792,-29.0985610309771,
12.));
#141123=CARTESIAN_POINT('Ctrl Pts',(-67.2855325866517,-29.0982319644277,
0.));
#141124=CARTESIAN_POINT('Ctrl Pts',(-67.2855325866517,-29.0982319644277,
12.));
#141125=CARTESIAN_POINT('Ctrl Pts',(-67.2593020179209,-29.0978789691962,
0.));
#141126=CARTESIAN_POINT('Ctrl Pts',(-67.2593020179209,-29.0978789691962,
12.));
#141127=CARTESIAN_POINT('Ctrl Pts',(-67.2331094720471,-29.097502097147,
0.));
#141128=CARTESIAN_POINT('Ctrl Pts',(-67.2331094720471,-29.097502097147,
12.));
#141129=CARTESIAN_POINT('Ctrl Pts',(-67.2069550447883,-29.0971014004131,
0.));
#141130=CARTESIAN_POINT('Ctrl Pts',(-67.2069550447883,-29.0971014004131,
12.));
#141131=CARTESIAN_POINT('Ctrl Pts',(-67.1808388322109,-29.096676931389,
0.));
#141132=CARTESIAN_POINT('Ctrl Pts',(-67.1808388322109,-29.096676931389,
12.));
#141133=CARTESIAN_POINT('Ctrl Pts',(-67.1547609306843,-29.0962287427273,
0.));
#141134=CARTESIAN_POINT('Ctrl Pts',(-67.1547609306843,-29.0962287427273,
12.));
#141135=CARTESIAN_POINT('Ctrl Pts',(-67.1287214368746,-29.0957568873358,
0.));
#141136=CARTESIAN_POINT('Ctrl Pts',(-67.1287214368746,-29.0957568873358,
12.));
#141137=CARTESIAN_POINT('Ctrl Pts',(-67.1027204477311,-29.0952614183779,
0.));
#141138=CARTESIAN_POINT('Ctrl Pts',(-67.1027204477311,-29.0952614183779,
12.));
#141139=CARTESIAN_POINT('Ctrl Pts',(-67.0767580604879,-29.0947423892727,
0.));
#141140=CARTESIAN_POINT('Ctrl Pts',(-67.0767580604879,-29.0947423892727,
12.));
#141141=CARTESIAN_POINT('Ctrl Pts',(-67.0508343726776,-29.0941998536959,
0.));
#141142=CARTESIAN_POINT('Ctrl Pts',(-67.0508343726776,-29.0941998536959,
12.));
#141143=CARTESIAN_POINT('Ctrl Pts',(-67.0249494821363,-29.0936338655828,
0.));
#141144=CARTESIAN_POINT('Ctrl Pts',(-67.0249494821363,-29.0936338655828,
12.));
#141145=CARTESIAN_POINT('Ctrl Pts',(-66.9991034870083,-29.0930444791328,
0.));
#141146=CARTESIAN_POINT('Ctrl Pts',(-66.9991034870083,-29.0930444791328,
12.));
#141147=CARTESIAN_POINT('Ctrl Pts',(-66.9732964857466,-29.092431748817,
0.));
#141148=CARTESIAN_POINT('Ctrl Pts',(-66.9732964857466,-29.092431748817,
12.));
#141149=CARTESIAN_POINT('Ctrl Pts',(-66.9475285771135,-29.0917957293826,
0.));
#141150=CARTESIAN_POINT('Ctrl Pts',(-66.9475285771135,-29.0917957293826,
12.));
#141151=CARTESIAN_POINT('Ctrl Pts',(-66.9217998601885,-29.0911364758487,
0.));
#141152=CARTESIAN_POINT('Ctrl Pts',(-66.9217998601885,-29.0911364758487,
12.));
#141153=CARTESIAN_POINT('Ctrl Pts',(-66.8961104343707,-29.0904540435065,
0.));
#141154=CARTESIAN_POINT('Ctrl Pts',(-66.8961104343707,-29.0904540435065,
12.));
#141155=CARTESIAN_POINT('Ctrl Pts',(-66.8704603993794,-29.0897484879207,
0.));
#141156=CARTESIAN_POINT('Ctrl Pts',(-66.8704603993794,-29.0897484879207,
12.));
#141157=CARTESIAN_POINT('Ctrl Pts',(-66.8448498552503,-29.0890198649323,
0.));
#141158=CARTESIAN_POINT('Ctrl Pts',(-66.8448498552503,-29.0890198649323,
12.));
#141159=CARTESIAN_POINT('Ctrl Pts',(-66.8192789023312,-29.088268230663,
0.));
#141160=CARTESIAN_POINT('Ctrl Pts',(-66.8192789023312,-29.088268230663,
12.));
#141161=CARTESIAN_POINT('Ctrl Pts',(-66.793747641293,-29.0874936415132,
0.));
#141162=CARTESIAN_POINT('Ctrl Pts',(-66.793747641293,-29.0874936415132,
12.));
#141163=CARTESIAN_POINT('Ctrl Pts',(-66.7682561731341,-29.0866961541626,
0.));
#141164=CARTESIAN_POINT('Ctrl Pts',(-66.7682561731341,-29.0866961541626,
12.));
#141165=CARTESIAN_POINT('Ctrl Pts',(-66.7428045991841,-29.0858758255729,
0.));
#141166=CARTESIAN_POINT('Ctrl Pts',(-66.7428045991841,-29.0858758255729,
12.));
#141167=CARTESIAN_POINT('Ctrl Pts',(-66.7173930211022,-29.0850327129916,
0.));
#141168=CARTESIAN_POINT('Ctrl Pts',(-66.7173930211022,-29.0850327129916,
12.));
#141169=CARTESIAN_POINT('Ctrl Pts',(-66.6920215408751,-29.0841668739588,
0.));
#141170=CARTESIAN_POINT('Ctrl Pts',(-66.6920215408751,-29.0841668739588,
12.));
#141171=CARTESIAN_POINT('Ctrl Pts',(-66.6666902608249,-29.0832783663049,
0.));
#141172=CARTESIAN_POINT('Ctrl Pts',(-66.6666902608249,-29.0832783663049,
12.));
#141173=CARTESIAN_POINT('Ctrl Pts',(-66.6413992836147,-29.0823672481507,
0.));
#141174=CARTESIAN_POINT('Ctrl Pts',(-66.6413992836147,-29.0823672481507,
12.));
#141175=CARTESIAN_POINT('Ctrl Pts',(-66.6161487122502,-29.0814335779084,
0.));
#141176=CARTESIAN_POINT('Ctrl Pts',(-66.6161487122502,-29.0814335779084,
12.));
#141177=CARTESIAN_POINT('Ctrl Pts',(-66.59093865008,-29.0804774142854,0.));
#141178=CARTESIAN_POINT('Ctrl Pts',(-66.59093865008,-29.0804774142854,12.));
#141179=CARTESIAN_POINT('Ctrl Pts',(-66.5657692007906,-29.0794988162897,
0.));
#141180=CARTESIAN_POINT('Ctrl Pts',(-66.5657692007906,-29.0794988162897,
12.));
#141181=CARTESIAN_POINT('Ctrl Pts',(-66.5406404684132,-29.0784978432301,
0.));
#141182=CARTESIAN_POINT('Ctrl Pts',(-66.5406404684132,-29.0784978432301,
12.));
#141183=CARTESIAN_POINT('Ctrl Pts',(-66.5155525573323,-29.0774745547151,
0.));
#141184=CARTESIAN_POINT('Ctrl Pts',(-66.5155525573323,-29.0774745547151,
12.));
#141185=CARTESIAN_POINT('Ctrl Pts',(-66.4905055722868,-29.0764290106554,
0.));
#141186=CARTESIAN_POINT('Ctrl Pts',(-66.4905055722868,-29.0764290106554,
12.));
#141187=CARTESIAN_POINT('Ctrl Pts',(-66.4654996183731,-29.0753612712666,
0.));
#141188=CARTESIAN_POINT('Ctrl Pts',(-66.4654996183731,-29.0753612712666,
12.));
#141189=CARTESIAN_POINT('Ctrl Pts',(-66.4405348010388,-29.0742713970755,
0.));
#141190=CARTESIAN_POINT('Ctrl Pts',(-66.4405348010388,-29.0742713970755,
12.));
#141191=CARTESIAN_POINT('Ctrl Pts',(-66.4156112260887,-29.0731594489211,
0.));
#141192=CARTESIAN_POINT('Ctrl Pts',(-66.4156112260887,-29.0731594489211,
12.));
#141193=CARTESIAN_POINT('Ctrl Pts',(-66.3907289996932,-29.072025487953,
0.));
#141194=CARTESIAN_POINT('Ctrl Pts',(-66.3907289996932,-29.072025487953,
12.));
#141195=CARTESIAN_POINT('Ctrl Pts',(-66.3658882283903,-29.0708695756334,
0.));
#141196=CARTESIAN_POINT('Ctrl Pts',(-66.3658882283903,-29.0708695756334,
12.));
#141197=CARTESIAN_POINT('Ctrl Pts',(-66.3410890190884,-29.0696917737399,
0.));
#141198=CARTESIAN_POINT('Ctrl Pts',(-66.3410890190884,-29.0696917737399,
12.));
#141199=CARTESIAN_POINT('Ctrl Pts',(-66.3163314790615,-29.0684921443721,
0.));
#141200=CARTESIAN_POINT('Ctrl Pts',(-66.3163314790615,-29.0684921443721,
12.));
#141201=CARTESIAN_POINT('Ctrl Pts',(-66.2916157159536,-29.067270749953,
0.));
#141202=CARTESIAN_POINT('Ctrl Pts',(-66.2916157159536,-29.067270749953,
12.));
#141203=CARTESIAN_POINT('Ctrl Pts',(-66.2669418377871,-29.0660276532274,
0.));
#141204=CARTESIAN_POINT('Ctrl Pts',(-66.2669418377871,-29.0660276532274,
12.));
#141205=CARTESIAN_POINT('Ctrl Pts',(-66.2423099529669,-29.0647629172645,
0.));
#141206=CARTESIAN_POINT('Ctrl Pts',(-66.2423099529669,-29.0647629172645,
12.));
#141207=CARTESIAN_POINT('Ctrl Pts',(-66.2177201702818,-29.0634766054598,
0.));
#141208=CARTESIAN_POINT('Ctrl Pts',(-66.2177201702818,-29.0634766054598,
12.));
#141209=CARTESIAN_POINT('Ctrl Pts',(-66.1931725989008,-29.062168781542,
0.));
#141210=CARTESIAN_POINT('Ctrl Pts',(-66.1931725989008,-29.062168781542,
12.));
#141211=CARTESIAN_POINT('Ctrl Pts',(-66.1686673483757,-29.0608395095747,
0.));
#141212=CARTESIAN_POINT('Ctrl Pts',(-66.1686673483757,-29.0608395095747,
12.));
#141213=CARTESIAN_POINT('Ctrl Pts',(-66.144204528652,-29.0594888539558,
0.));
#141214=CARTESIAN_POINT('Ctrl Pts',(-66.144204528652,-29.0594888539558,
12.));
#141215=CARTESIAN_POINT('Ctrl Pts',(-66.1197842500714,-29.0581168794191,
0.));
#141216=CARTESIAN_POINT('Ctrl Pts',(-66.1197842500714,-29.0581168794191,
12.));
#141217=CARTESIAN_POINT('Ctrl Pts',(-66.0954066233752,-29.0567236510372,
0.));
#141218=CARTESIAN_POINT('Ctrl Pts',(-66.0954066233752,-29.0567236510372,
12.));
#141219=CARTESIAN_POINT('Ctrl Pts',(-66.0710717597003,-29.0553092342275,
0.));
#141220=CARTESIAN_POINT('Ctrl Pts',(-66.0710717597003,-29.0553092342275,
12.));
#141221=CARTESIAN_POINT('Ctrl Pts',(-66.0467797705806,-29.0538736947547,
0.));
#141222=CARTESIAN_POINT('Ctrl Pts',(-66.0467797705806,-29.0538736947547,
12.));
#141223=CARTESIAN_POINT('Ctrl Pts',(-66.0225307679584,-29.0524170987303,
0.));
#141224=CARTESIAN_POINT('Ctrl Pts',(-66.0225307679584,-29.0524170987303,
12.));
#141225=CARTESIAN_POINT('Ctrl Pts',(-65.9983248641877,-29.0509395126141,
0.));
#141226=CARTESIAN_POINT('Ctrl Pts',(-65.9983248641877,-29.0509395126141,
12.));
#141227=CARTESIAN_POINT('Ctrl Pts',(-65.9741621720372,-29.0494410032173,
0.));
#141228=CARTESIAN_POINT('Ctrl Pts',(-65.9741621720372,-29.0494410032173,
12.));
#141229=CARTESIAN_POINT('Ctrl Pts',(-65.9500428046873,-29.0479216377082,
0.));
#141230=CARTESIAN_POINT('Ctrl Pts',(-65.9500428046873,-29.0479216377082,
12.));
#141231=CARTESIAN_POINT('Ctrl Pts',(-65.9259668757309,-29.0463814836158,
0.));
#141232=CARTESIAN_POINT('Ctrl Pts',(-65.9259668757309,-29.0463814836158,
12.));
#141233=CARTESIAN_POINT('Ctrl Pts',(-65.9019344991854,-29.0448206088288,
0.));
#141234=CARTESIAN_POINT('Ctrl Pts',(-65.9019344991854,-29.0448206088288,
12.));
#141235=CARTESIAN_POINT('Ctrl Pts',(-65.8779457894959,-29.0432390815977,
0.));
#141236=CARTESIAN_POINT('Ctrl Pts',(-65.8779457894959,-29.0432390815977,
12.));
#141237=CARTESIAN_POINT('Ctrl Pts',(-65.854000861539,-29.0416369705375,
0.));
#141238=CARTESIAN_POINT('Ctrl Pts',(-65.854000861539,-29.0416369705375,
12.));
#141239=CARTESIAN_POINT('Ctrl Pts',(-65.8300998306198,-29.0400143446341,
0.));
#141240=CARTESIAN_POINT('Ctrl Pts',(-65.8300998306198,-29.0400143446341,
12.));
#141241=CARTESIAN_POINT('Ctrl Pts',(-65.8062428124723,-29.0383712732473,
0.));
#141242=CARTESIAN_POINT('Ctrl Pts',(-65.8062428124723,-29.0383712732473,
12.));
#141243=CARTESIAN_POINT('Ctrl Pts',(-65.7824299232715,-29.0367078261107,
0.));
#141244=CARTESIAN_POINT('Ctrl Pts',(-65.7824299232715,-29.0367078261107,
12.));
#141245=CARTESIAN_POINT('Ctrl Pts',(-65.7586612796375,-29.0350240733333,
0.));
#141246=CARTESIAN_POINT('Ctrl Pts',(-65.7586612796375,-29.0350240733333,
12.));
#141247=CARTESIAN_POINT('Ctrl Pts',(-65.7349369986382,-29.0333200854026,
0.));
#141248=CARTESIAN_POINT('Ctrl Pts',(-65.7349369986382,-29.0333200854026,
12.));
#141249=CARTESIAN_POINT('Ctrl Pts',(-65.7112571977874,-29.0315959331911,
0.));
#141250=CARTESIAN_POINT('Ctrl Pts',(-65.7112571977874,-29.0315959331911,
12.));
#141251=CARTESIAN_POINT('Ctrl Pts',(-65.6876219950465,-29.0298516879599,
0.));
#141252=CARTESIAN_POINT('Ctrl Pts',(-65.6876219950465,-29.0298516879599,
12.));
#141253=CARTESIAN_POINT('Ctrl Pts',(-65.664031508836,-29.0280874213584,
0.));
#141254=CARTESIAN_POINT('Ctrl Pts',(-65.664031508836,-29.0280874213584,
12.));
#141255=CARTESIAN_POINT('Ctrl Pts',(-65.6404858580391,-29.0263032054261,
0.));
#141256=CARTESIAN_POINT('Ctrl Pts',(-65.6404858580391,-29.0263032054261,
12.));
#141257=CARTESIAN_POINT('Ctrl Pts',(-65.6169851620054,-29.0244991125962,
0.));
#141258=CARTESIAN_POINT('Ctrl Pts',(-65.6169851620054,-29.0244991125962,
12.));
#141259=CARTESIAN_POINT('Ctrl Pts',(-65.593529540548,-29.0226752157013,
0.));
#141260=CARTESIAN_POINT('Ctrl Pts',(-65.593529540548,-29.0226752157013,
12.));
#141261=CARTESIAN_POINT('Ctrl Pts',(-65.5701191139455,-29.0208315879778,
0.));
#141262=CARTESIAN_POINT('Ctrl Pts',(-65.5701191139455,-29.0208315879778,
12.));
#141263=CARTESIAN_POINT('Ctrl Pts',(-65.5467540029546,-29.0189683030654,
0.));
#141264=CARTESIAN_POINT('Ctrl Pts',(-65.5467540029546,-29.0189683030654,
12.));
#141265=CARTESIAN_POINT('Ctrl Pts',(-65.523434328815,-29.01708543501,0.));
#141266=CARTESIAN_POINT('Ctrl Pts',(-65.523434328815,-29.01708543501,12.));
#141267=CARTESIAN_POINT('Ctrl Pts',(-65.5001602132524,-29.015183058267,
0.));
#141268=CARTESIAN_POINT('Ctrl Pts',(-65.5001602132524,-29.015183058267,
12.));
#141269=CARTESIAN_POINT('Ctrl Pts',(-65.4769317784754,-29.0132612477075,
0.));
#141270=CARTESIAN_POINT('Ctrl Pts',(-65.4769317784754,-29.0132612477075,
12.));
#141271=CARTESIAN_POINT('Ctrl Pts',(-65.4537491471782,-29.0113200786219,
0.));
#141272=CARTESIAN_POINT('Ctrl Pts',(-65.4537491471782,-29.0113200786219,
12.));
#141273=CARTESIAN_POINT('Ctrl Pts',(-65.4306124425524,-29.0093596267198,
0.));
#141274=CARTESIAN_POINT('Ctrl Pts',(-65.4306124425524,-29.0093596267198,
12.));
#141275=CARTESIAN_POINT('Ctrl Pts',(-65.4075217882921,-29.0073799681336,
0.));
#141276=CARTESIAN_POINT('Ctrl Pts',(-65.4075217882921,-29.0073799681336,
12.));
#141277=CARTESIAN_POINT('Ctrl Pts',(-65.3844773085976,-29.0053811794214,
0.));
#141278=CARTESIAN_POINT('Ctrl Pts',(-65.3844773085976,-29.0053811794214,
12.));
#141279=CARTESIAN_POINT('Ctrl Pts',(-65.3614791281726,-29.0033633375745,
0.));
#141280=CARTESIAN_POINT('Ctrl Pts',(-65.3614791281726,-29.0033633375745,
12.));
#141281=CARTESIAN_POINT('Ctrl Pts',(-65.3385273722278,-29.0013265200201,
0.));
#141282=CARTESIAN_POINT('Ctrl Pts',(-65.3385273722278,-29.0013265200201,
12.));
#141283=CARTESIAN_POINT('Ctrl Pts',(-65.3156221664942,-28.9992708046223,
0.));
#141284=CARTESIAN_POINT('Ctrl Pts',(-65.3156221664942,-28.9992708046223,
12.));
#141285=CARTESIAN_POINT('Ctrl Pts',(-65.2927636372261,-28.9971962696848,
0.));
#141286=CARTESIAN_POINT('Ctrl Pts',(-65.2927636372261,-28.9971962696848,
12.));
#141287=CARTESIAN_POINT('Ctrl Pts',(-65.2699519112052,-28.9951029939551,
0.));
#141288=CARTESIAN_POINT('Ctrl Pts',(-65.2699519112052,-28.9951029939551,
12.));
#141289=CARTESIAN_POINT('Ctrl Pts',(-65.2471871157375,-28.9929910566314,
0.));
#141290=CARTESIAN_POINT('Ctrl Pts',(-65.2471871157375,-28.9929910566314,
12.));
#141291=CARTESIAN_POINT('Ctrl Pts',(-65.2244693786586,-28.9908605373652,
0.));
#141292=CARTESIAN_POINT('Ctrl Pts',(-65.2244693786586,-28.9908605373652,
12.));
#141293=CARTESIAN_POINT('Ctrl Pts',(-65.2017988283465,-28.9887115162626,
0.));
#141294=CARTESIAN_POINT('Ctrl Pts',(-65.2017988283465,-28.9887115162626,
12.));
#141295=CARTESIAN_POINT('Ctrl Pts',(-65.1791755937254,-28.9865440738882,
0.));
#141296=CARTESIAN_POINT('Ctrl Pts',(-65.1791755937254,-28.9865440738882,
12.));
#141297=CARTESIAN_POINT('Ctrl Pts',(-65.1565998042705,-28.9843582912697,
0.));
#141298=CARTESIAN_POINT('Ctrl Pts',(-65.1565998042705,-28.9843582912697,
12.));
#141299=CARTESIAN_POINT('Ctrl Pts',(-65.1340715900042,-28.9821542499049,
0.));
#141300=CARTESIAN_POINT('Ctrl Pts',(-65.1340715900042,-28.9821542499049,
12.));
#141301=CARTESIAN_POINT('Ctrl Pts',(-65.111591081505,-28.9799320317648,
0.));
#141302=CARTESIAN_POINT('Ctrl Pts',(-65.111591081505,-28.9799320317648,
12.));
#141303=CARTESIAN_POINT('Ctrl Pts',(-65.0891584099174,-28.9776917192936,
0.));
#141304=CARTESIAN_POINT('Ctrl Pts',(-65.0891584099174,-28.9776917192936,
12.));
#141305=CARTESIAN_POINT('Ctrl Pts',(-65.0667737069562,-28.9754333954134,
0.));
#141306=CARTESIAN_POINT('Ctrl Pts',(-65.0667737069562,-28.9754333954134,
12.));
#141307=CARTESIAN_POINT('Ctrl Pts',(-65.0444371049082,-28.9731571435281,
0.));
#141308=CARTESIAN_POINT('Ctrl Pts',(-65.0444371049082,-28.9731571435281,
12.));
#141309=CARTESIAN_POINT('Ctrl Pts',(-65.0221487366279,-28.9708630475298,
0.));
#141310=CARTESIAN_POINT('Ctrl Pts',(-65.0221487366279,-28.9708630475298,
12.));
#141311=CARTESIAN_POINT('Ctrl Pts',(-64.9999087355504,-28.9685511918017,
0.));
#141312=CARTESIAN_POINT('Ctrl Pts',(-64.9999087355504,-28.9685511918017,
12.));
#141313=CARTESIAN_POINT('Ctrl Pts',(-64.9777172357028,-28.9662216612216,
0.));
#141314=CARTESIAN_POINT('Ctrl Pts',(-64.9777172357028,-28.9662216612216,
12.));
#141315=CARTESIAN_POINT('Ctrl Pts',(-64.955574371711,-28.9638745411677,
0.));
#141316=CARTESIAN_POINT('Ctrl Pts',(-64.955574371711,-28.9638745411677,
12.));
#141317=CARTESIAN_POINT('Ctrl Pts',(-64.9334802788037,-28.961509917525,
0.));
#141318=CARTESIAN_POINT('Ctrl Pts',(-64.9334802788037,-28.961509917525,
12.));
#141319=CARTESIAN_POINT('Ctrl Pts',(-64.9114350928124,-28.9591278766934,
0.));
#141320=CARTESIAN_POINT('Ctrl Pts',(-64.9114350928124,-28.9591278766934,
12.));
#141321=CARTESIAN_POINT('Ctrl Pts',(-64.8894389501799,-28.9567285055866,
0.));
#141322=CARTESIAN_POINT('Ctrl Pts',(-64.8894389501799,-28.9567285055866,
12.));
#141323=CARTESIAN_POINT('Ctrl Pts',(-64.8674919879646,-28.9543118916327,
0.));
#141324=CARTESIAN_POINT('Ctrl Pts',(-64.8674919879646,-28.9543118916327,
12.));
#141325=CARTESIAN_POINT('Ctrl Pts',(-64.8455943438423,-28.9518781227765,
0.));
#141326=CARTESIAN_POINT('Ctrl Pts',(-64.8455943438423,-28.9518781227765,
12.));
#141327=CARTESIAN_POINT('Ctrl Pts',(-64.8237461561024,-28.9494272874833,
0.));
#141328=CARTESIAN_POINT('Ctrl Pts',(-64.8237461561024,-28.9494272874833,
12.));
#141329=CARTESIAN_POINT('Ctrl Pts',(-64.8019475636454,-28.9469594747436,
0.));
#141330=CARTESIAN_POINT('Ctrl Pts',(-64.8019475636454,-28.9469594747436,
12.));
#141331=CARTESIAN_POINT('Ctrl Pts',(-64.7801987060097,-28.9444747740815,
0.));
#141332=CARTESIAN_POINT('Ctrl Pts',(-64.7801987060097,-28.9444747740815,
12.));
#141333=CARTESIAN_POINT('Ctrl Pts',(-64.7584997233889,-28.9419732755659,
0.));
#141334=CARTESIAN_POINT('Ctrl Pts',(-64.7584997233889,-28.9419732755659,
12.));
#141335=CARTESIAN_POINT('Ctrl Pts',(-64.7368507566461,-28.9394550698201,
0.));
#141336=CARTESIAN_POINT('Ctrl Pts',(-64.7368507566461,-28.9394550698201,
12.));
#141337=CARTESIAN_POINT('Ctrl Pts',(-64.715251947327,-28.9369202480383,
0.));
#141338=CARTESIAN_POINT('Ctrl Pts',(-64.715251947327,-28.9369202480383,
12.));
#141339=CARTESIAN_POINT('Ctrl Pts',(-64.6937034376591,-28.934368901987,
0.));
#141340=CARTESIAN_POINT('Ctrl Pts',(-64.6937034376591,-28.934368901987,
12.));
#141341=CARTESIAN_POINT('Ctrl Pts',(-64.6722053705389,-28.9318011239905,
0.));
#141342=CARTESIAN_POINT('Ctrl Pts',(-64.6722053705389,-28.9318011239905,
12.));
#141343=CARTESIAN_POINT('Ctrl Pts',(-64.6507578895155,-28.9292170069219,
0.));
#141344=CARTESIAN_POINT('Ctrl Pts',(-64.6507578895155,-28.9292170069219,
12.));
#141345=CARTESIAN_POINT('Ctrl Pts',(-64.6293611387753,-28.9266166441956,
0.));
#141346=CARTESIAN_POINT('Ctrl Pts',(-64.6293611387753,-28.9266166441956,
12.));
#141347=CARTESIAN_POINT('Ctrl Pts',(-64.6080152631065,-28.9240001297553,
0.));
#141348=CARTESIAN_POINT('Ctrl Pts',(-64.6080152631065,-28.9240001297553,
12.));
#141349=CARTESIAN_POINT('Ctrl Pts',(-64.5867204079452,-28.9213675580996,
0.));
#141350=CARTESIAN_POINT('Ctrl Pts',(-64.5867204079452,-28.9213675580996,
12.));
#141351=CARTESIAN_POINT('Ctrl Pts',(-64.5654767194487,-28.9187190243231,
0.));
#141352=CARTESIAN_POINT('Ctrl Pts',(-64.5654767194487,-28.9187190243231,
12.));
#141353=CARTESIAN_POINT('Ctrl Pts',(-64.544284344556,-28.9160546241538,
0.));
#141354=CARTESIAN_POINT('Ctrl Pts',(-64.544284344556,-28.9160546241538,
12.));
#141355=CARTESIAN_POINT('Ctrl Pts',(-64.5231434310457,-28.9133744539943,
0.));
#141356=CARTESIAN_POINT('Ctrl Pts',(-64.5231434310457,-28.9133744539943,
12.));
#141357=CARTESIAN_POINT('Ctrl Pts',(-64.5020541275927,-28.9106786109639,
0.));
#141358=CARTESIAN_POINT('Ctrl Pts',(-64.5020541275927,-28.9106786109639,
12.));
#141359=CARTESIAN_POINT('Ctrl Pts',(-64.4810165836568,-28.9079671928253,
0.));
#141360=CARTESIAN_POINT('Ctrl Pts',(-64.4810165836568,-28.9079671928253,
12.));
#141361=CARTESIAN_POINT('Ctrl Pts',(-64.460030949357,-28.9052402979055,
0.));
#141362=CARTESIAN_POINT('Ctrl Pts',(-64.460030949357,-28.9052402979055,
12.));
#141363=CARTESIAN_POINT('Ctrl Pts',(-64.439097375364,-28.9024980250309,
0.));
#141364=CARTESIAN_POINT('Ctrl Pts',(-64.439097375364,-28.9024980250309,
12.));
#141365=CARTESIAN_POINT('Ctrl Pts',(-64.4182160127401,-28.899740473435,
0.));
#141366=CARTESIAN_POINT('Ctrl Pts',(-64.4182160127401,-28.899740473435,
12.));
#141367=CARTESIAN_POINT('Ctrl Pts',(-64.3973870129201,-28.8969677427519,
0.));
#141368=CARTESIAN_POINT('Ctrl Pts',(-64.3973870129201,-28.8969677427519,
12.));
#141369=CARTESIAN_POINT('Ctrl Pts',(-64.3766105280715,-28.8941799332312,
0.));
#141370=CARTESIAN_POINT('Ctrl Pts',(-64.3766105280715,-28.8941799332312,
12.));
#141371=CARTESIAN_POINT('Ctrl Pts',(-64.3558867114087,-28.8913771459327,
0.));
#141372=CARTESIAN_POINT('Ctrl Pts',(-64.3558867114087,-28.8913771459327,
12.));
#141373=CARTESIAN_POINT('Ctrl Pts',(-64.3352157174606,-28.888559482892,
0.));
#141374=CARTESIAN_POINT('Ctrl Pts',(-64.3352157174606,-28.888559482892,
12.));
#141375=CARTESIAN_POINT('Ctrl Pts',(-64.3145977025005,-28.8857270473944,
0.));
#141376=CARTESIAN_POINT('Ctrl Pts',(-64.3145977025005,-28.8857270473944,
12.));
#141377=CARTESIAN_POINT('Ctrl Pts',(-64.2940328242482,-28.8828799437922,
0.));
#141378=CARTESIAN_POINT('Ctrl Pts',(-64.2940328242482,-28.8828799437922,
12.));
#141379=CARTESIAN_POINT('Ctrl Pts',(-64.2735212410682,-28.8800182770052,
0.));
#141380=CARTESIAN_POINT('Ctrl Pts',(-64.2735212410682,-28.8800182770052,
12.));
#141381=CARTESIAN_POINT('Ctrl Pts',(-64.2530631112926,-28.8771421521058,
0.));
#141382=CARTESIAN_POINT('Ctrl Pts',(-64.2530631112926,-28.8771421521058,
12.));
#141383=CARTESIAN_POINT('Ctrl Pts',(-64.232658592528,-28.8742516738959,
0.));
#141384=CARTESIAN_POINT('Ctrl Pts',(-64.232658592528,-28.8742516738959,
12.));
#141385=CARTESIAN_POINT('Ctrl Pts',(-64.2123078408507,-28.8713469464205,
0.));
#141386=CARTESIAN_POINT('Ctrl Pts',(-64.2123078408507,-28.8713469464205,
12.));
#141387=CARTESIAN_POINT('Ctrl Pts',(-64.1920110123342,-28.8684280739033,
0.));
#141388=CARTESIAN_POINT('Ctrl Pts',(-64.1920110123342,-28.8684280739033,
12.));
#141389=CARTESIAN_POINT('Ctrl Pts',(-64.1717682648708,-28.8654951618659,
0.));
#141390=CARTESIAN_POINT('Ctrl Pts',(-64.1717682648708,-28.8654951618659,
12.));
#141391=CARTESIAN_POINT('Ctrl Pts',(-64.1515797596555,-28.8625483180433,
0.));
#141392=CARTESIAN_POINT('Ctrl Pts',(-64.1515797596555,-28.8625483180433,
12.));
#141393=CARTESIAN_POINT('Ctrl Pts',(-64.1314456633345,-28.8595876537132,
0.));
#141394=CARTESIAN_POINT('Ctrl Pts',(-64.1314456633345,-28.8595876537132,
12.));
#141395=CARTESIAN_POINT('Ctrl Pts',(-64.1113661481918,-28.8566132838157,
0.));
#141396=CARTESIAN_POINT('Ctrl Pts',(-64.1113661481918,-28.8566132838157,
12.));
#141397=CARTESIAN_POINT('Ctrl Pts',(-64.0913413876586,-28.8536253241837,
0.));
#141398=CARTESIAN_POINT('Ctrl Pts',(-64.0913413876586,-28.8536253241837,
12.));
#141399=CARTESIAN_POINT('Ctrl Pts',(-64.0713715523588,-28.8506238891087,
0.));
#141400=CARTESIAN_POINT('Ctrl Pts',(-64.0713715523588,-28.8506238891087,
12.));
#141401=CARTESIAN_POINT('Ctrl Pts',(-64.0514568066659,-28.8476090892242,
0.));
#141402=CARTESIAN_POINT('Ctrl Pts',(-64.0514568066659,-28.8476090892242,
12.));
#141403=CARTESIAN_POINT('Ctrl Pts',(-64.0315973031994,-28.8445810281275,
0.));
#141404=CARTESIAN_POINT('Ctrl Pts',(-64.0315973031994,-28.8445810281275,
12.));
#141405=CARTESIAN_POINT('Ctrl Pts',(-64.0117931881364,-28.841539805646,
0.));
#141406=CARTESIAN_POINT('Ctrl Pts',(-64.0117931881364,-28.841539805646,
12.));
#141407=CARTESIAN_POINT('Ctrl Pts',(-63.9920446117632,-28.8384855243267,
0.));
#141408=CARTESIAN_POINT('Ctrl Pts',(-63.9920446117632,-28.8384855243267,
12.));
#141409=CARTESIAN_POINT('Ctrl Pts',(-63.9723517369614,-28.8354182946601,
0.));
#141410=CARTESIAN_POINT('Ctrl Pts',(-63.9723517369614,-28.8354182946601,
12.));
#141411=CARTESIAN_POINT('Ctrl Pts',(-63.9527147494351,-28.8323382413752,
0.));
#141412=CARTESIAN_POINT('Ctrl Pts',(-63.9527147494351,-28.8323382413752,
12.));
#141413=CARTESIAN_POINT('Ctrl Pts',(-63.9331338646868,-28.8292455077494,
0.));
#141414=CARTESIAN_POINT('Ctrl Pts',(-63.9331338646868,-28.8292455077494,
12.));
#141415=CARTESIAN_POINT('Ctrl Pts',(-63.9136093063647,-28.826140242322,
0.));
#141416=CARTESIAN_POINT('Ctrl Pts',(-63.9136093063647,-28.826140242322,
12.));
#141417=CARTESIAN_POINT('Ctrl Pts',(-63.894141285685,-28.8230225863142,
0.));
#141418=CARTESIAN_POINT('Ctrl Pts',(-63.894141285685,-28.8230225863142,
12.));
#141419=CARTESIAN_POINT('Ctrl Pts',(-63.8747299825383,-28.8198926619893,
0.));
#141420=CARTESIAN_POINT('Ctrl Pts',(-63.8747299825383,-28.8198926619893,
12.));
#141421=CARTESIAN_POINT('Ctrl Pts',(-63.8553755207732,-28.8167505576806,
0.));
#141422=CARTESIAN_POINT('Ctrl Pts',(-63.8553755207732,-28.8167505576806,
12.));
#141423=CARTESIAN_POINT('Ctrl Pts',(-63.8360779670226,-28.8135963263557,
0.));
#141424=CARTESIAN_POINT('Ctrl Pts',(-63.8360779670226,-28.8135963263557,
12.));
#141425=CARTESIAN_POINT('Ctrl Pts',(-63.8206854735372,-28.8110632621133,
0.));
#141426=CARTESIAN_POINT('Ctrl Pts',(-63.8206854735372,-28.8110632621133,
12.));
#141427=CARTESIAN_POINT('Ctrl Pts',(-63.809166727145,-28.8091580239664,
0.));
#141428=CARTESIAN_POINT('Ctrl Pts',(-63.809166727145,-28.8091580239664,
12.));
#141429=CARTESIAN_POINT('Ctrl Pts',(-63.8014989507575,-28.8078854475473,
0.));
#141430=CARTESIAN_POINT('Ctrl Pts',(-63.8014989507575,-28.8078854475473,
12.));
#141431=CARTESIAN_POINT('Ctrl Pts',(-63.7976679095314,-28.8072485549236,
0.));
#141432=CARTESIAN_POINT('Ctrl Pts',(-63.7976679095314,-28.8072485549236,
12.));
#141433=CARTESIAN_POINT('',(-63.7976679095314,-28.8072485549236,12.));
#141434=CARTESIAN_POINT('Ctrl Pts',(-63.7976679095314,-28.8072485549236,
12.));
#141435=CARTESIAN_POINT('Ctrl Pts',(-63.8014989507575,-28.8078854475473,
12.));
#141436=CARTESIAN_POINT('Ctrl Pts',(-63.809166727145,-28.8091580239664,
12.));
#141437=CARTESIAN_POINT('Ctrl Pts',(-63.8206854735372,-28.8110632621133,
12.));
#141438=CARTESIAN_POINT('Ctrl Pts',(-63.8360779670226,-28.8135963263557,
12.));
#141439=CARTESIAN_POINT('Ctrl Pts',(-63.8553755207732,-28.8167505576806,
12.));
#141440=CARTESIAN_POINT('Ctrl Pts',(-63.8747299825383,-28.8198926619893,
12.));
#141441=CARTESIAN_POINT('Ctrl Pts',(-63.894141285685,-28.8230225863142,
12.));
#141442=CARTESIAN_POINT('Ctrl Pts',(-63.9136093063647,-28.826140242322,
12.));
#141443=CARTESIAN_POINT('Ctrl Pts',(-63.9331338646868,-28.8292455077494,
12.));
#141444=CARTESIAN_POINT('Ctrl Pts',(-63.9527147494351,-28.8323382413752,
12.));
#141445=CARTESIAN_POINT('Ctrl Pts',(-63.9723517369614,-28.8354182946601,
12.));
#141446=CARTESIAN_POINT('Ctrl Pts',(-63.9920446117632,-28.8384855243267,
12.));
#141447=CARTESIAN_POINT('Ctrl Pts',(-64.0117931881364,-28.841539805646,
12.));
#141448=CARTESIAN_POINT('Ctrl Pts',(-64.0315973031994,-28.8445810281275,
12.));
#141449=CARTESIAN_POINT('Ctrl Pts',(-64.0514568066659,-28.8476090892242,
12.));
#141450=CARTESIAN_POINT('Ctrl Pts',(-64.0713715523588,-28.8506238891087,
12.));
#141451=CARTESIAN_POINT('Ctrl Pts',(-64.0913413876586,-28.8536253241837,
12.));
#141452=CARTESIAN_POINT('Ctrl Pts',(-64.1113661481918,-28.8566132838157,
12.));
#141453=CARTESIAN_POINT('Ctrl Pts',(-64.1314456633345,-28.8595876537132,
12.));
#141454=CARTESIAN_POINT('Ctrl Pts',(-64.1515797596555,-28.8625483180433,
12.));
#141455=CARTESIAN_POINT('Ctrl Pts',(-64.1717682648708,-28.8654951618659,
12.));
#141456=CARTESIAN_POINT('Ctrl Pts',(-64.1920110123342,-28.8684280739033,
12.));
#141457=CARTESIAN_POINT('Ctrl Pts',(-64.2123078408507,-28.8713469464205,
12.));
#141458=CARTESIAN_POINT('Ctrl Pts',(-64.232658592528,-28.8742516738959,
12.));
#141459=CARTESIAN_POINT('Ctrl Pts',(-64.2530631112926,-28.8771421521058,
12.));
#141460=CARTESIAN_POINT('Ctrl Pts',(-64.2735212410682,-28.8800182770052,
12.));
#141461=CARTESIAN_POINT('Ctrl Pts',(-64.2940328242482,-28.8828799437922,
12.));
#141462=CARTESIAN_POINT('Ctrl Pts',(-64.3145977025005,-28.8857270473944,
12.));
#141463=CARTESIAN_POINT('Ctrl Pts',(-64.3352157174606,-28.888559482892,
12.));
#141464=CARTESIAN_POINT('Ctrl Pts',(-64.3558867114087,-28.8913771459327,
12.));
#141465=CARTESIAN_POINT('Ctrl Pts',(-64.3766105280715,-28.8941799332312,
12.));
#141466=CARTESIAN_POINT('Ctrl Pts',(-64.3973870129201,-28.8969677427519,
12.));
#141467=CARTESIAN_POINT('Ctrl Pts',(-64.4182160127401,-28.899740473435,
12.));
#141468=CARTESIAN_POINT('Ctrl Pts',(-64.439097375364,-28.9024980250309,
12.));
#141469=CARTESIAN_POINT('Ctrl Pts',(-64.460030949357,-28.9052402979055,
12.));
#141470=CARTESIAN_POINT('Ctrl Pts',(-64.4810165836568,-28.9079671928253,
12.));
#141471=CARTESIAN_POINT('Ctrl Pts',(-64.5020541275927,-28.9106786109639,
12.));
#141472=CARTESIAN_POINT('Ctrl Pts',(-64.5231434310457,-28.9133744539943,
12.));
#141473=CARTESIAN_POINT('Ctrl Pts',(-64.544284344556,-28.9160546241538,
12.));
#141474=CARTESIAN_POINT('Ctrl Pts',(-64.5654767194487,-28.9187190243231,
12.));
#141475=CARTESIAN_POINT('Ctrl Pts',(-64.5867204079452,-28.9213675580996,
12.));
#141476=CARTESIAN_POINT('Ctrl Pts',(-64.6080152631065,-28.9240001297553,
12.));
#141477=CARTESIAN_POINT('Ctrl Pts',(-64.6293611387753,-28.9266166441956,
12.));
#141478=CARTESIAN_POINT('Ctrl Pts',(-64.6507578895155,-28.9292170069219,
12.));
#141479=CARTESIAN_POINT('Ctrl Pts',(-64.6722053705389,-28.9318011239905,
12.));
#141480=CARTESIAN_POINT('Ctrl Pts',(-64.6937034376591,-28.934368901987,
12.));
#141481=CARTESIAN_POINT('Ctrl Pts',(-64.715251947327,-28.9369202480383,
12.));
#141482=CARTESIAN_POINT('Ctrl Pts',(-64.7368507566461,-28.9394550698201,
12.));
#141483=CARTESIAN_POINT('Ctrl Pts',(-64.7584997233889,-28.9419732755659,
12.));
#141484=CARTESIAN_POINT('Ctrl Pts',(-64.7801987060097,-28.9444747740815,
12.));
#141485=CARTESIAN_POINT('Ctrl Pts',(-64.8019475636454,-28.9469594747436,
12.));
#141486=CARTESIAN_POINT('Ctrl Pts',(-64.8237461561024,-28.9494272874833,
12.));
#141487=CARTESIAN_POINT('Ctrl Pts',(-64.8455943438423,-28.9518781227765,
12.));
#141488=CARTESIAN_POINT('Ctrl Pts',(-64.8674919879646,-28.9543118916327,
12.));
#141489=CARTESIAN_POINT('Ctrl Pts',(-64.8894389501799,-28.9567285055866,
12.));
#141490=CARTESIAN_POINT('Ctrl Pts',(-64.9114350928124,-28.9591278766934,
12.));
#141491=CARTESIAN_POINT('Ctrl Pts',(-64.9334802788037,-28.961509917525,
12.));
#141492=CARTESIAN_POINT('Ctrl Pts',(-64.955574371711,-28.9638745411677,
12.));
#141493=CARTESIAN_POINT('Ctrl Pts',(-64.9777172357028,-28.9662216612216,
12.));
#141494=CARTESIAN_POINT('Ctrl Pts',(-64.9999087355504,-28.9685511918017,
12.));
#141495=CARTESIAN_POINT('Ctrl Pts',(-65.0221487366279,-28.9708630475298,
12.));
#141496=CARTESIAN_POINT('Ctrl Pts',(-65.0444371049082,-28.9731571435281,
12.));
#141497=CARTESIAN_POINT('Ctrl Pts',(-65.0667737069562,-28.9754333954134,
12.));
#141498=CARTESIAN_POINT('Ctrl Pts',(-65.0891584099174,-28.9776917192936,
12.));
#141499=CARTESIAN_POINT('Ctrl Pts',(-65.111591081505,-28.9799320317648,
12.));
#141500=CARTESIAN_POINT('Ctrl Pts',(-65.1340715900042,-28.9821542499049,
12.));
#141501=CARTESIAN_POINT('Ctrl Pts',(-65.1565998042705,-28.9843582912697,
12.));
#141502=CARTESIAN_POINT('Ctrl Pts',(-65.1791755937254,-28.9865440738882,
12.));
#141503=CARTESIAN_POINT('Ctrl Pts',(-65.2017988283465,-28.9887115162626,
12.));
#141504=CARTESIAN_POINT('Ctrl Pts',(-65.2244693786586,-28.9908605373652,
12.));
#141505=CARTESIAN_POINT('Ctrl Pts',(-65.2471871157375,-28.9929910566314,
12.));
#141506=CARTESIAN_POINT('Ctrl Pts',(-65.2699519112052,-28.9951029939551,
12.));
#141507=CARTESIAN_POINT('Ctrl Pts',(-65.2927636372261,-28.9971962696848,
12.));
#141508=CARTESIAN_POINT('Ctrl Pts',(-65.3156221664942,-28.9992708046223,
12.));
#141509=CARTESIAN_POINT('Ctrl Pts',(-65.3385273722278,-29.0013265200201,
12.));
#141510=CARTESIAN_POINT('Ctrl Pts',(-65.3614791281726,-29.0033633375745,
12.));
#141511=CARTESIAN_POINT('Ctrl Pts',(-65.3844773085976,-29.0053811794214,
12.));
#141512=CARTESIAN_POINT('Ctrl Pts',(-65.4075217882921,-29.0073799681336,
12.));
#141513=CARTESIAN_POINT('Ctrl Pts',(-65.4306124425524,-29.0093596267198,
12.));
#141514=CARTESIAN_POINT('Ctrl Pts',(-65.4537491471782,-29.0113200786219,
12.));
#141515=CARTESIAN_POINT('Ctrl Pts',(-65.4769317784754,-29.0132612477075,
12.));
#141516=CARTESIAN_POINT('Ctrl Pts',(-65.5001602132524,-29.015183058267,
12.));
#141517=CARTESIAN_POINT('Ctrl Pts',(-65.523434328815,-29.01708543501,12.));
#141518=CARTESIAN_POINT('Ctrl Pts',(-65.5467540029546,-29.0189683030654,
12.));
#141519=CARTESIAN_POINT('Ctrl Pts',(-65.5701191139455,-29.0208315879778,
12.));
#141520=CARTESIAN_POINT('Ctrl Pts',(-65.593529540548,-29.0226752157013,
12.));
#141521=CARTESIAN_POINT('Ctrl Pts',(-65.6169851620054,-29.0244991125962,
12.));
#141522=CARTESIAN_POINT('Ctrl Pts',(-65.6404858580391,-29.0263032054261,
12.));
#141523=CARTESIAN_POINT('Ctrl Pts',(-65.664031508836,-29.0280874213584,
12.));
#141524=CARTESIAN_POINT('Ctrl Pts',(-65.6876219950465,-29.0298516879599,
12.));
#141525=CARTESIAN_POINT('Ctrl Pts',(-65.7112571977874,-29.0315959331911,
12.));
#141526=CARTESIAN_POINT('Ctrl Pts',(-65.7349369986382,-29.0333200854026,
12.));
#141527=CARTESIAN_POINT('Ctrl Pts',(-65.7586612796375,-29.0350240733333,
12.));
#141528=CARTESIAN_POINT('Ctrl Pts',(-65.7824299232715,-29.0367078261107,
12.));
#141529=CARTESIAN_POINT('Ctrl Pts',(-65.8062428124723,-29.0383712732473,
12.));
#141530=CARTESIAN_POINT('Ctrl Pts',(-65.8300998306198,-29.0400143446341,
12.));
#141531=CARTESIAN_POINT('Ctrl Pts',(-65.854000861539,-29.0416369705375,
12.));
#141532=CARTESIAN_POINT('Ctrl Pts',(-65.8779457894959,-29.0432390815977,
12.));
#141533=CARTESIAN_POINT('Ctrl Pts',(-65.9019344991854,-29.0448206088288,
12.));
#141534=CARTESIAN_POINT('Ctrl Pts',(-65.9259668757309,-29.0463814836158,
12.));
#141535=CARTESIAN_POINT('Ctrl Pts',(-65.9500428046873,-29.0479216377082,
12.));
#141536=CARTESIAN_POINT('Ctrl Pts',(-65.9741621720372,-29.0494410032173,
12.));
#141537=CARTESIAN_POINT('Ctrl Pts',(-65.9983248641877,-29.0509395126141,
12.));
#141538=CARTESIAN_POINT('Ctrl Pts',(-66.0225307679584,-29.0524170987303,
12.));
#141539=CARTESIAN_POINT('Ctrl Pts',(-66.0467797705806,-29.0538736947547,
12.));
#141540=CARTESIAN_POINT('Ctrl Pts',(-66.0710717597003,-29.0553092342275,
12.));
#141541=CARTESIAN_POINT('Ctrl Pts',(-66.0954066233752,-29.0567236510372,
12.));
#141542=CARTESIAN_POINT('Ctrl Pts',(-66.1197842500714,-29.0581168794191,
12.));
#141543=CARTESIAN_POINT('Ctrl Pts',(-66.144204528652,-29.0594888539558,
12.));
#141544=CARTESIAN_POINT('Ctrl Pts',(-66.1686673483757,-29.0608395095747,
12.));
#141545=CARTESIAN_POINT('Ctrl Pts',(-66.1931725989008,-29.062168781542,
12.));
#141546=CARTESIAN_POINT('Ctrl Pts',(-66.2177201702818,-29.0634766054598,
12.));
#141547=CARTESIAN_POINT('Ctrl Pts',(-66.2423099529669,-29.0647629172645,
12.));
#141548=CARTESIAN_POINT('Ctrl Pts',(-66.2669418377871,-29.0660276532274,
12.));
#141549=CARTESIAN_POINT('Ctrl Pts',(-66.2916157159536,-29.067270749953,
12.));
#141550=CARTESIAN_POINT('Ctrl Pts',(-66.3163314790615,-29.0684921443721,
12.));
#141551=CARTESIAN_POINT('Ctrl Pts',(-66.3410890190884,-29.0696917737399,
12.));
#141552=CARTESIAN_POINT('Ctrl Pts',(-66.3658882283903,-29.0708695756334,
12.));
#141553=CARTESIAN_POINT('Ctrl Pts',(-66.3907289996932,-29.072025487953,
12.));
#141554=CARTESIAN_POINT('Ctrl Pts',(-66.4156112260887,-29.0731594489211,
12.));
#141555=CARTESIAN_POINT('Ctrl Pts',(-66.4405348010388,-29.0742713970755,
12.));
#141556=CARTESIAN_POINT('Ctrl Pts',(-66.4654996183731,-29.0753612712666,
12.));
#141557=CARTESIAN_POINT('Ctrl Pts',(-66.4905055722868,-29.0764290106554,
12.));
#141558=CARTESIAN_POINT('Ctrl Pts',(-66.5155525573323,-29.0774745547151,
12.));
#141559=CARTESIAN_POINT('Ctrl Pts',(-66.5406404684132,-29.0784978432301,
12.));
#141560=CARTESIAN_POINT('Ctrl Pts',(-66.5657692007906,-29.0794988162897,
12.));
#141561=CARTESIAN_POINT('Ctrl Pts',(-66.59093865008,-29.0804774142854,12.));
#141562=CARTESIAN_POINT('Ctrl Pts',(-66.6161487122502,-29.0814335779084,
12.));
#141563=CARTESIAN_POINT('Ctrl Pts',(-66.6413992836147,-29.0823672481507,
12.));
#141564=CARTESIAN_POINT('Ctrl Pts',(-66.6666902608249,-29.0832783663049,
12.));
#141565=CARTESIAN_POINT('Ctrl Pts',(-66.6920215408751,-29.0841668739588,
12.));
#141566=CARTESIAN_POINT('Ctrl Pts',(-66.7173930211022,-29.0850327129916,
12.));
#141567=CARTESIAN_POINT('Ctrl Pts',(-66.7428045991841,-29.0858758255729,
12.));
#141568=CARTESIAN_POINT('Ctrl Pts',(-66.7682561731341,-29.0866961541626,
12.));
#141569=CARTESIAN_POINT('Ctrl Pts',(-66.793747641293,-29.0874936415132,
12.));
#141570=CARTESIAN_POINT('Ctrl Pts',(-66.8192789023312,-29.088268230663,
12.));
#141571=CARTESIAN_POINT('Ctrl Pts',(-66.8448498552503,-29.0890198649323,
12.));
#141572=CARTESIAN_POINT('Ctrl Pts',(-66.8704603993794,-29.0897484879207,
12.));
#141573=CARTESIAN_POINT('Ctrl Pts',(-66.8961104343707,-29.0904540435065,
12.));
#141574=CARTESIAN_POINT('Ctrl Pts',(-66.9217998601885,-29.0911364758487,
12.));
#141575=CARTESIAN_POINT('Ctrl Pts',(-66.9475285771135,-29.0917957293826,
12.));
#141576=CARTESIAN_POINT('Ctrl Pts',(-66.9732964857466,-29.092431748817,
12.));
#141577=CARTESIAN_POINT('Ctrl Pts',(-66.9991034870083,-29.0930444791328,
12.));
#141578=CARTESIAN_POINT('Ctrl Pts',(-67.0249494821363,-29.0936338655828,
12.));
#141579=CARTESIAN_POINT('Ctrl Pts',(-67.0508343726776,-29.0941998536959,
12.));
#141580=CARTESIAN_POINT('Ctrl Pts',(-67.0767580604879,-29.0947423892727,
12.));
#141581=CARTESIAN_POINT('Ctrl Pts',(-67.1027204477311,-29.0952614183779,
12.));
#141582=CARTESIAN_POINT('Ctrl Pts',(-67.1287214368746,-29.0957568873358,
12.));
#141583=CARTESIAN_POINT('Ctrl Pts',(-67.1547609306843,-29.0962287427273,
12.));
#141584=CARTESIAN_POINT('Ctrl Pts',(-67.1808388322109,-29.096676931389,
12.));
#141585=CARTESIAN_POINT('Ctrl Pts',(-67.2069550447883,-29.0971014004131,
12.));
#141586=CARTESIAN_POINT('Ctrl Pts',(-67.2331094720471,-29.097502097147,
12.));
#141587=CARTESIAN_POINT('Ctrl Pts',(-67.2593020179209,-29.0978789691962,
12.));
#141588=CARTESIAN_POINT('Ctrl Pts',(-67.2855325866517,-29.0982319644277,
12.));
#141589=CARTESIAN_POINT('Ctrl Pts',(-67.311801082792,-29.0985610309771,
12.));
#141590=CARTESIAN_POINT('Ctrl Pts',(-67.3381074112027,-29.0988661172531,
12.));
#141591=CARTESIAN_POINT('Ctrl Pts',(-67.3644514770387,-29.0991471719176,
12.));
#141592=CARTESIAN_POINT('Ctrl Pts',(-67.3908331857323,-29.0994041438719,
12.));
#141593=CARTESIAN_POINT('Ctrl Pts',(-67.4172524429727,-29.0996369822418,
12.));
#141594=CARTESIAN_POINT('Ctrl Pts',(-67.4437091546859,-29.0998456363683,
12.));
#141595=CARTESIAN_POINT('Ctrl Pts',(-67.4702032270048,-29.1000300557955,
12.));
#141596=CARTESIAN_POINT('Ctrl Pts',(-67.4967345663096,-29.1001901902909,
12.));
#141597=CARTESIAN_POINT('Ctrl Pts',(-67.5233030792704,-29.1003259898682,
12.));
#141598=CARTESIAN_POINT('Ctrl Pts',(-67.5499086728888,-29.1004374048148,
12.));
#141599=CARTESIAN_POINT('Ctrl Pts',(-67.5765512545281,-29.1005243857139,
12.));
#141600=CARTESIAN_POINT('Ctrl Pts',(-67.6032307319623,-29.1005868834866,
12.));
#141601=CARTESIAN_POINT('Ctrl Pts',(-67.6299470133295,-29.100624849358,
12.));
#141602=CARTESIAN_POINT('Ctrl Pts',(-67.6567000070326,-29.1006382347814,
12.));
#141603=CARTESIAN_POINT('Ctrl Pts',(-67.6834896216461,-29.1006269913747,
12.));
#141604=CARTESIAN_POINT('Ctrl Pts',(-67.7103157658296,-29.1005910708624,
12.));
#141605=CARTESIAN_POINT('Ctrl Pts',(-67.7371783482035,-29.1005304249987,
12.));
#141606=CARTESIAN_POINT('Ctrl Pts',(-67.7640772773388,-29.1004450055643,
12.));
#141607=CARTESIAN_POINT('Ctrl Pts',(-67.7910124620135,-29.1003347645294,
12.));
#141608=CARTESIAN_POINT('Ctrl Pts',(-67.8179838114099,-29.1001996541842,
12.));
#141609=CARTESIAN_POINT('Ctrl Pts',(-67.8449912353329,-29.1000396272867,
12.));
#141610=CARTESIAN_POINT('Ctrl Pts',(-67.8720346444124,-29.0998546372032,
12.));
#141611=CARTESIAN_POINT('Ctrl Pts',(-67.8991139503193,-29.0996446380626,
12.));
#141612=CARTESIAN_POINT('Ctrl Pts',(-67.9262290652829,-29.099409584422,
12.));
#141613=CARTESIAN_POINT('Ctrl Pts',(-67.9533799016148,-29.0991494309404,
12.));
#141614=CARTESIAN_POINT('Ctrl Pts',(-67.9805663711855,-29.0988641320247,
12.));
#141615=CARTESIAN_POINT('Ctrl Pts',(-68.0077883850121,-29.0985536415531,
12.));
#141616=CARTESIAN_POINT('Ctrl Pts',(-68.0350458525551,-29.0982179124097,
12.));
#141617=CARTESIAN_POINT('Ctrl Pts',(-68.0623386822863,-29.0978568968657,
12.));
#141618=CARTESIAN_POINT('Ctrl Pts',(-68.0896667829567,-29.0974705474259,
12.));
#141619=CARTESIAN_POINT('Ctrl Pts',(-68.1170300646987,-29.0970588175728,
12.));
#141620=CARTESIAN_POINT('Ctrl Pts',(-68.1444284400742,-29.0966216624743,
12.));
#141621=CARTESIAN_POINT('Ctrl Pts',(-68.1718618254281,-29.0961590399046,
12.));
#141622=CARTESIAN_POINT('Ctrl Pts',(-68.1993301412061,-29.0956709104627,
12.));
#141623=CARTESIAN_POINT('Ctrl Pts',(-68.2229056854683,-29.095230591515,
12.));
#141624=CARTESIAN_POINT('Ctrl Pts',(-68.2409993690196,-29.094879194787,
12.));
#141625=CARTESIAN_POINT('Ctrl Pts',(-68.2535957747187,-29.0946280433337,
12.));
#141626=CARTESIAN_POINT('Ctrl Pts',(-68.2606847334987,-29.0944846386568,
12.));
#141627=CARTESIAN_POINT('Ctrl Pts',(-68.2622612910177,-29.0944526440266,
12.));
#141628=CARTESIAN_POINT('',(-63.7976679095314,-28.8072485549236,0.));
#141629=CARTESIAN_POINT('',(-63.7976679095314,-28.8072485549236,0.));
#141630=CARTESIAN_POINT('Ctrl Pts',(-68.2622612910177,-29.0944526440266,
0.));
#141631=CARTESIAN_POINT('Ctrl Pts',(-68.2606847334987,-29.0944846386568,
0.));
#141632=CARTESIAN_POINT('Ctrl Pts',(-68.2535957747187,-29.0946280433337,
0.));
#141633=CARTESIAN_POINT('Ctrl Pts',(-68.2409993690197,-29.094879194787,
0.));
#141634=CARTESIAN_POINT('Ctrl Pts',(-68.2229056854683,-29.095230591515,
0.));
#141635=CARTESIAN_POINT('Ctrl Pts',(-68.1993301412061,-29.0956709104627,
0.));
#141636=CARTESIAN_POINT('Ctrl Pts',(-68.1718618254281,-29.0961590399046,
0.));
#141637=CARTESIAN_POINT('Ctrl Pts',(-68.1444284400742,-29.0966216624743,
0.));
#141638=CARTESIAN_POINT('Ctrl Pts',(-68.1170300646987,-29.0970588175728,
0.));
#141639=CARTESIAN_POINT('Ctrl Pts',(-68.0896667829567,-29.0974705474259,
0.));
#141640=CARTESIAN_POINT('Ctrl Pts',(-68.0623386822863,-29.0978568968657,
0.));
#141641=CARTESIAN_POINT('Ctrl Pts',(-68.0350458525551,-29.0982179124097,
0.));
#141642=CARTESIAN_POINT('Ctrl Pts',(-68.0077883850121,-29.0985536415531,
0.));
#141643=CARTESIAN_POINT('Ctrl Pts',(-67.9805663711855,-29.0988641320247,
0.));
#141644=CARTESIAN_POINT('Ctrl Pts',(-67.9533799016148,-29.0991494309404,
0.));
#141645=CARTESIAN_POINT('Ctrl Pts',(-67.9262290652829,-29.099409584422,
0.));
#141646=CARTESIAN_POINT('Ctrl Pts',(-67.8991139503193,-29.0996446380626,
0.));
#141647=CARTESIAN_POINT('Ctrl Pts',(-67.8720346444124,-29.0998546372032,
0.));
#141648=CARTESIAN_POINT('Ctrl Pts',(-67.8449912353329,-29.1000396272867,
0.));
#141649=CARTESIAN_POINT('Ctrl Pts',(-67.8179838114099,-29.1001996541842,
0.));
#141650=CARTESIAN_POINT('Ctrl Pts',(-67.7910124620135,-29.1003347645294,
0.));
#141651=CARTESIAN_POINT('Ctrl Pts',(-67.7640772773388,-29.1004450055643,
0.));
#141652=CARTESIAN_POINT('Ctrl Pts',(-67.7371783482035,-29.1005304249987,
0.));
#141653=CARTESIAN_POINT('Ctrl Pts',(-67.7103157658296,-29.1005910708624,
0.));
#141654=CARTESIAN_POINT('Ctrl Pts',(-67.6834896216461,-29.1006269913747,
0.));
#141655=CARTESIAN_POINT('Ctrl Pts',(-67.6567000070326,-29.1006382347814,
0.));
#141656=CARTESIAN_POINT('Ctrl Pts',(-67.6299470133295,-29.100624849358,
0.));
#141657=CARTESIAN_POINT('Ctrl Pts',(-67.6032307319623,-29.1005868834866,
0.));
#141658=CARTESIAN_POINT('Ctrl Pts',(-67.5765512545281,-29.1005243857139,
0.));
#141659=CARTESIAN_POINT('Ctrl Pts',(-67.5499086728888,-29.1004374048148,
0.));
#141660=CARTESIAN_POINT('Ctrl Pts',(-67.5233030792704,-29.1003259898682,
0.));
#141661=CARTESIAN_POINT('Ctrl Pts',(-67.4967345663096,-29.1001901902909,
0.));
#141662=CARTESIAN_POINT('Ctrl Pts',(-67.4702032270048,-29.1000300557955,
0.));
#141663=CARTESIAN_POINT('Ctrl Pts',(-67.4437091546859,-29.0998456363683,
0.));
#141664=CARTESIAN_POINT('Ctrl Pts',(-67.4172524429727,-29.0996369822418,
0.));
#141665=CARTESIAN_POINT('Ctrl Pts',(-67.3908331857323,-29.0994041438719,
0.));
#141666=CARTESIAN_POINT('Ctrl Pts',(-67.3644514770387,-29.0991471719176,
0.));
#141667=CARTESIAN_POINT('Ctrl Pts',(-67.3381074112027,-29.0988661172531,
0.));
#141668=CARTESIAN_POINT('Ctrl Pts',(-67.311801082792,-29.0985610309771,
0.));
#141669=CARTESIAN_POINT('Ctrl Pts',(-67.2855325866517,-29.0982319644277,
0.));
#141670=CARTESIAN_POINT('Ctrl Pts',(-67.2593020179209,-29.0978789691962,
0.));
#141671=CARTESIAN_POINT('Ctrl Pts',(-67.2331094720471,-29.097502097147,
0.));
#141672=CARTESIAN_POINT('Ctrl Pts',(-67.2069550447883,-29.0971014004131,
0.));
#141673=CARTESIAN_POINT('Ctrl Pts',(-67.1808388322109,-29.096676931389,
0.));
#141674=CARTESIAN_POINT('Ctrl Pts',(-67.1547609306843,-29.0962287427273,
0.));
#141675=CARTESIAN_POINT('Ctrl Pts',(-67.1287214368746,-29.0957568873358,
0.));
#141676=CARTESIAN_POINT('Ctrl Pts',(-67.1027204477311,-29.0952614183779,
0.));
#141677=CARTESIAN_POINT('Ctrl Pts',(-67.0767580604879,-29.0947423892727,
0.));
#141678=CARTESIAN_POINT('Ctrl Pts',(-67.0508343726776,-29.0941998536959,
0.));
#141679=CARTESIAN_POINT('Ctrl Pts',(-67.0249494821363,-29.0936338655828,
0.));
#141680=CARTESIAN_POINT('Ctrl Pts',(-66.9991034870083,-29.0930444791328,
0.));
#141681=CARTESIAN_POINT('Ctrl Pts',(-66.9732964857466,-29.092431748817,
0.));
#141682=CARTESIAN_POINT('Ctrl Pts',(-66.9475285771135,-29.0917957293826,
0.));
#141683=CARTESIAN_POINT('Ctrl Pts',(-66.9217998601885,-29.0911364758487,
0.));
#141684=CARTESIAN_POINT('Ctrl Pts',(-66.8961104343707,-29.0904540435065,
0.));
#141685=CARTESIAN_POINT('Ctrl Pts',(-66.8704603993794,-29.0897484879207,
0.));
#141686=CARTESIAN_POINT('Ctrl Pts',(-66.8448498552503,-29.0890198649323,
0.));
#141687=CARTESIAN_POINT('Ctrl Pts',(-66.8192789023312,-29.088268230663,
0.));
#141688=CARTESIAN_POINT('Ctrl Pts',(-66.793747641293,-29.0874936415132,
0.));
#141689=CARTESIAN_POINT('Ctrl Pts',(-66.7682561731341,-29.0866961541626,
0.));
#141690=CARTESIAN_POINT('Ctrl Pts',(-66.7428045991841,-29.0858758255729,
0.));
#141691=CARTESIAN_POINT('Ctrl Pts',(-66.7173930211022,-29.0850327129916,
0.));
#141692=CARTESIAN_POINT('Ctrl Pts',(-66.6920215408751,-29.0841668739588,
0.));
#141693=CARTESIAN_POINT('Ctrl Pts',(-66.6666902608249,-29.0832783663049,
0.));
#141694=CARTESIAN_POINT('Ctrl Pts',(-66.6413992836147,-29.0823672481507,
0.));
#141695=CARTESIAN_POINT('Ctrl Pts',(-66.6161487122502,-29.0814335779084,
0.));
#141696=CARTESIAN_POINT('Ctrl Pts',(-66.59093865008,-29.0804774142854,0.));
#141697=CARTESIAN_POINT('Ctrl Pts',(-66.5657692007906,-29.0794988162897,
0.));
#141698=CARTESIAN_POINT('Ctrl Pts',(-66.5406404684132,-29.0784978432301,
0.));
#141699=CARTESIAN_POINT('Ctrl Pts',(-66.5155525573323,-29.0774745547151,
0.));
#141700=CARTESIAN_POINT('Ctrl Pts',(-66.4905055722868,-29.0764290106554,
0.));
#141701=CARTESIAN_POINT('Ctrl Pts',(-66.4654996183731,-29.0753612712666,
0.));
#141702=CARTESIAN_POINT('Ctrl Pts',(-66.4405348010388,-29.0742713970755,
0.));
#141703=CARTESIAN_POINT('Ctrl Pts',(-66.4156112260887,-29.0731594489211,
0.));
#141704=CARTESIAN_POINT('Ctrl Pts',(-66.3907289996932,-29.072025487953,
0.));
#141705=CARTESIAN_POINT('Ctrl Pts',(-66.3658882283903,-29.0708695756334,
0.));
#141706=CARTESIAN_POINT('Ctrl Pts',(-66.3410890190884,-29.0696917737399,
0.));
#141707=CARTESIAN_POINT('Ctrl Pts',(-66.3163314790615,-29.0684921443721,
0.));
#141708=CARTESIAN_POINT('Ctrl Pts',(-66.2916157159536,-29.067270749953,
0.));
#141709=CARTESIAN_POINT('Ctrl Pts',(-66.2669418377871,-29.0660276532274,
0.));
#141710=CARTESIAN_POINT('Ctrl Pts',(-66.2423099529669,-29.0647629172645,
0.));
#141711=CARTESIAN_POINT('Ctrl Pts',(-66.2177201702818,-29.0634766054598,
0.));
#141712=CARTESIAN_POINT('Ctrl Pts',(-66.1931725989008,-29.062168781542,
0.));
#141713=CARTESIAN_POINT('Ctrl Pts',(-66.1686673483757,-29.0608395095747,
0.));
#141714=CARTESIAN_POINT('Ctrl Pts',(-66.144204528652,-29.0594888539558,
0.));
#141715=CARTESIAN_POINT('Ctrl Pts',(-66.1197842500714,-29.0581168794191,
0.));
#141716=CARTESIAN_POINT('Ctrl Pts',(-66.0954066233752,-29.0567236510372,
0.));
#141717=CARTESIAN_POINT('Ctrl Pts',(-66.0710717597003,-29.0553092342275,
0.));
#141718=CARTESIAN_POINT('Ctrl Pts',(-66.0467797705806,-29.0538736947547,
0.));
#141719=CARTESIAN_POINT('Ctrl Pts',(-66.0225307679584,-29.0524170987303,
0.));
#141720=CARTESIAN_POINT('Ctrl Pts',(-65.9983248641877,-29.0509395126141,
0.));
#141721=CARTESIAN_POINT('Ctrl Pts',(-65.9741621720372,-29.0494410032173,
0.));
#141722=CARTESIAN_POINT('Ctrl Pts',(-65.9500428046873,-29.0479216377082,
0.));
#141723=CARTESIAN_POINT('Ctrl Pts',(-65.9259668757309,-29.0463814836158,
0.));
#141724=CARTESIAN_POINT('Ctrl Pts',(-65.9019344991854,-29.0448206088288,
0.));
#141725=CARTESIAN_POINT('Ctrl Pts',(-65.8779457894959,-29.0432390815977,
0.));
#141726=CARTESIAN_POINT('Ctrl Pts',(-65.854000861539,-29.0416369705375,
0.));
#141727=CARTESIAN_POINT('Ctrl Pts',(-65.8300998306198,-29.0400143446341,
0.));
#141728=CARTESIAN_POINT('Ctrl Pts',(-65.8062428124723,-29.0383712732473,
0.));
#141729=CARTESIAN_POINT('Ctrl Pts',(-65.7824299232715,-29.0367078261107,
0.));
#141730=CARTESIAN_POINT('Ctrl Pts',(-65.7586612796375,-29.0350240733333,
0.));
#141731=CARTESIAN_POINT('Ctrl Pts',(-65.7349369986382,-29.0333200854026,
0.));
#141732=CARTESIAN_POINT('Ctrl Pts',(-65.7112571977874,-29.0315959331911,
0.));
#141733=CARTESIAN_POINT('Ctrl Pts',(-65.6876219950465,-29.0298516879599,
0.));
#141734=CARTESIAN_POINT('Ctrl Pts',(-65.664031508836,-29.0280874213584,
0.));
#141735=CARTESIAN_POINT('Ctrl Pts',(-65.6404858580391,-29.0263032054261,
0.));
#141736=CARTESIAN_POINT('Ctrl Pts',(-65.6169851620054,-29.0244991125962,
0.));
#141737=CARTESIAN_POINT('Ctrl Pts',(-65.593529540548,-29.0226752157013,
0.));
#141738=CARTESIAN_POINT('Ctrl Pts',(-65.5701191139455,-29.0208315879778,
0.));
#141739=CARTESIAN_POINT('Ctrl Pts',(-65.5467540029546,-29.0189683030654,
0.));
#141740=CARTESIAN_POINT('Ctrl Pts',(-65.523434328815,-29.01708543501,0.));
#141741=CARTESIAN_POINT('Ctrl Pts',(-65.5001602132524,-29.015183058267,
0.));
#141742=CARTESIAN_POINT('Ctrl Pts',(-65.4769317784754,-29.0132612477075,
0.));
#141743=CARTESIAN_POINT('Ctrl Pts',(-65.4537491471782,-29.0113200786219,
0.));
#141744=CARTESIAN_POINT('Ctrl Pts',(-65.4306124425524,-29.0093596267198,
0.));
#141745=CARTESIAN_POINT('Ctrl Pts',(-65.4075217882921,-29.0073799681336,
0.));
#141746=CARTESIAN_POINT('Ctrl Pts',(-65.3844773085976,-29.0053811794214,
0.));
#141747=CARTESIAN_POINT('Ctrl Pts',(-65.3614791281726,-29.0033633375745,
0.));
#141748=CARTESIAN_POINT('Ctrl Pts',(-65.3385273722278,-29.0013265200201,
0.));
#141749=CARTESIAN_POINT('Ctrl Pts',(-65.3156221664942,-28.9992708046223,
0.));
#141750=CARTESIAN_POINT('Ctrl Pts',(-65.2927636372261,-28.9971962696848,
0.));
#141751=CARTESIAN_POINT('Ctrl Pts',(-65.2699519112052,-28.9951029939551,
0.));
#141752=CARTESIAN_POINT('Ctrl Pts',(-65.2471871157375,-28.9929910566314,
0.));
#141753=CARTESIAN_POINT('Ctrl Pts',(-65.2244693786586,-28.9908605373652,
0.));
#141754=CARTESIAN_POINT('Ctrl Pts',(-65.2017988283465,-28.9887115162626,
0.));
#141755=CARTESIAN_POINT('Ctrl Pts',(-65.1791755937254,-28.9865440738882,
0.));
#141756=CARTESIAN_POINT('Ctrl Pts',(-65.1565998042705,-28.9843582912697,
0.));
#141757=CARTESIAN_POINT('Ctrl Pts',(-65.1340715900042,-28.9821542499049,
0.));
#141758=CARTESIAN_POINT('Ctrl Pts',(-65.111591081505,-28.9799320317648,
0.));
#141759=CARTESIAN_POINT('Ctrl Pts',(-65.0891584099174,-28.9776917192936,
0.));
#141760=CARTESIAN_POINT('Ctrl Pts',(-65.0667737069562,-28.9754333954134,
0.));
#141761=CARTESIAN_POINT('Ctrl Pts',(-65.0444371049082,-28.9731571435281,
0.));
#141762=CARTESIAN_POINT('Ctrl Pts',(-65.0221487366279,-28.9708630475298,
0.));
#141763=CARTESIAN_POINT('Ctrl Pts',(-64.9999087355504,-28.9685511918017,
0.));
#141764=CARTESIAN_POINT('Ctrl Pts',(-64.9777172357028,-28.9662216612216,
0.));
#141765=CARTESIAN_POINT('Ctrl Pts',(-64.955574371711,-28.9638745411677,
0.));
#141766=CARTESIAN_POINT('Ctrl Pts',(-64.9334802788037,-28.961509917525,
0.));
#141767=CARTESIAN_POINT('Ctrl Pts',(-64.9114350928124,-28.9591278766934,
0.));
#141768=CARTESIAN_POINT('Ctrl Pts',(-64.8894389501799,-28.9567285055866,
0.));
#141769=CARTESIAN_POINT('Ctrl Pts',(-64.8674919879646,-28.9543118916327,
0.));
#141770=CARTESIAN_POINT('Ctrl Pts',(-64.8455943438423,-28.9518781227765,
0.));
#141771=CARTESIAN_POINT('Ctrl Pts',(-64.8237461561024,-28.9494272874833,
0.));
#141772=CARTESIAN_POINT('Ctrl Pts',(-64.8019475636454,-28.9469594747436,
0.));
#141773=CARTESIAN_POINT('Ctrl Pts',(-64.7801987060097,-28.9444747740815,
0.));
#141774=CARTESIAN_POINT('Ctrl Pts',(-64.7584997233889,-28.9419732755659,
0.));
#141775=CARTESIAN_POINT('Ctrl Pts',(-64.7368507566461,-28.9394550698201,
0.));
#141776=CARTESIAN_POINT('Ctrl Pts',(-64.715251947327,-28.9369202480383,
0.));
#141777=CARTESIAN_POINT('Ctrl Pts',(-64.6937034376591,-28.934368901987,
0.));
#141778=CARTESIAN_POINT('Ctrl Pts',(-64.6722053705389,-28.9318011239905,
0.));
#141779=CARTESIAN_POINT('Ctrl Pts',(-64.6507578895155,-28.9292170069219,
0.));
#141780=CARTESIAN_POINT('Ctrl Pts',(-64.6293611387753,-28.9266166441956,
0.));
#141781=CARTESIAN_POINT('Ctrl Pts',(-64.6080152631065,-28.9240001297553,
0.));
#141782=CARTESIAN_POINT('Ctrl Pts',(-64.5867204079452,-28.9213675580996,
0.));
#141783=CARTESIAN_POINT('Ctrl Pts',(-64.5654767194487,-28.9187190243231,
0.));
#141784=CARTESIAN_POINT('Ctrl Pts',(-64.544284344556,-28.9160546241538,
0.));
#141785=CARTESIAN_POINT('Ctrl Pts',(-64.5231434310457,-28.9133744539943,
0.));
#141786=CARTESIAN_POINT('Ctrl Pts',(-64.5020541275927,-28.9106786109639,
0.));
#141787=CARTESIAN_POINT('Ctrl Pts',(-64.4810165836568,-28.9079671928253,
0.));
#141788=CARTESIAN_POINT('Ctrl Pts',(-64.460030949357,-28.9052402979055,
0.));
#141789=CARTESIAN_POINT('Ctrl Pts',(-64.439097375364,-28.9024980250309,
0.));
#141790=CARTESIAN_POINT('Ctrl Pts',(-64.4182160127401,-28.899740473435,
0.));
#141791=CARTESIAN_POINT('Ctrl Pts',(-64.3973870129201,-28.8969677427519,
0.));
#141792=CARTESIAN_POINT('Ctrl Pts',(-64.3766105280715,-28.8941799332312,
0.));
#141793=CARTESIAN_POINT('Ctrl Pts',(-64.3558867114087,-28.8913771459327,
0.));
#141794=CARTESIAN_POINT('Ctrl Pts',(-64.3352157174606,-28.888559482892,
0.));
#141795=CARTESIAN_POINT('Ctrl Pts',(-64.3145977025005,-28.8857270473944,
0.));
#141796=CARTESIAN_POINT('Ctrl Pts',(-64.2940328242482,-28.8828799437922,
0.));
#141797=CARTESIAN_POINT('Ctrl Pts',(-64.2735212410682,-28.8800182770052,
0.));
#141798=CARTESIAN_POINT('Ctrl Pts',(-64.2530631112926,-28.8771421521058,
0.));
#141799=CARTESIAN_POINT('Ctrl Pts',(-64.232658592528,-28.8742516738959,
0.));
#141800=CARTESIAN_POINT('Ctrl Pts',(-64.2123078408507,-28.8713469464205,
0.));
#141801=CARTESIAN_POINT('Ctrl Pts',(-64.1920110123342,-28.8684280739033,
0.));
#141802=CARTESIAN_POINT('Ctrl Pts',(-64.1717682648708,-28.8654951618659,
0.));
#141803=CARTESIAN_POINT('Ctrl Pts',(-64.1515797596555,-28.8625483180433,
0.));
#141804=CARTESIAN_POINT('Ctrl Pts',(-64.1314456633345,-28.8595876537132,
0.));
#141805=CARTESIAN_POINT('Ctrl Pts',(-64.1113661481918,-28.8566132838157,
0.));
#141806=CARTESIAN_POINT('Ctrl Pts',(-64.0913413876586,-28.8536253241837,
0.));
#141807=CARTESIAN_POINT('Ctrl Pts',(-64.0713715523588,-28.8506238891087,
0.));
#141808=CARTESIAN_POINT('Ctrl Pts',(-64.0514568066659,-28.8476090892242,
0.));
#141809=CARTESIAN_POINT('Ctrl Pts',(-64.0315973031994,-28.8445810281275,
0.));
#141810=CARTESIAN_POINT('Ctrl Pts',(-64.0117931881364,-28.841539805646,
0.));
#141811=CARTESIAN_POINT('Ctrl Pts',(-63.9920446117632,-28.8384855243267,
0.));
#141812=CARTESIAN_POINT('Ctrl Pts',(-63.9723517369614,-28.8354182946601,
0.));
#141813=CARTESIAN_POINT('Ctrl Pts',(-63.9527147494351,-28.8323382413752,
0.));
#141814=CARTESIAN_POINT('Ctrl Pts',(-63.9331338646868,-28.8292455077494,
0.));
#141815=CARTESIAN_POINT('Ctrl Pts',(-63.9136093063647,-28.826140242322,
0.));
#141816=CARTESIAN_POINT('Ctrl Pts',(-63.894141285685,-28.8230225863142,
0.));
#141817=CARTESIAN_POINT('Ctrl Pts',(-63.8747299825383,-28.8198926619893,
0.));
#141818=CARTESIAN_POINT('Ctrl Pts',(-63.8553755207732,-28.8167505576806,
0.));
#141819=CARTESIAN_POINT('Ctrl Pts',(-63.8360779670226,-28.8135963263557,
0.));
#141820=CARTESIAN_POINT('Ctrl Pts',(-63.8206854735372,-28.8110632621133,
0.));
#141821=CARTESIAN_POINT('Ctrl Pts',(-63.809166727145,-28.8091580239664,
0.));
#141822=CARTESIAN_POINT('Ctrl Pts',(-63.8014989507575,-28.8078854475473,
0.));
#141823=CARTESIAN_POINT('Ctrl Pts',(-63.7976679095314,-28.8072485549236,
0.));
#141824=CARTESIAN_POINT('Ctrl Pts',(-70.8615414811571,-22.9976507259816,
0.));
#141825=CARTESIAN_POINT('Ctrl Pts',(-70.8615414811571,-22.9976507259816,
12.));
#141826=CARTESIAN_POINT('Ctrl Pts',(-70.8559846928,-22.9983100639391,0.));
#141827=CARTESIAN_POINT('Ctrl Pts',(-70.8559846928,-22.9983100639391,12.));
#141828=CARTESIAN_POINT('Ctrl Pts',(-70.8448742696689,-22.9996258555291,
0.));
#141829=CARTESIAN_POINT('Ctrl Pts',(-70.8448742696689,-22.9996258555291,
12.));
#141830=CARTESIAN_POINT('Ctrl Pts',(-70.8282180957225,-23.0015908899394,
0.));
#141831=CARTESIAN_POINT('Ctrl Pts',(-70.8282180957225,-23.0015908899394,
12.));
#141832=CARTESIAN_POINT('Ctrl Pts',(-70.8060287860585,-23.0041936291626,
0.));
#141833=CARTESIAN_POINT('Ctrl Pts',(-70.8060287860585,-23.0041936291626,
12.));
#141834=CARTESIAN_POINT('Ctrl Pts',(-70.7783236951202,-23.0074182063787,
0.));
#141835=CARTESIAN_POINT('Ctrl Pts',(-70.7783236951202,-23.0074182063787,
12.));
#141836=CARTESIAN_POINT('Ctrl Pts',(-70.750650169619,-23.0106139366046,
0.));
#141837=CARTESIAN_POINT('Ctrl Pts',(-70.750650169619,-23.0106139366046,
12.));
#141838=CARTESIAN_POINT('Ctrl Pts',(-70.7230082425412,-23.0137808248924,
0.));
#141839=CARTESIAN_POINT('Ctrl Pts',(-70.7230082425412,-23.0137808248924,
12.));
#141840=CARTESIAN_POINT('Ctrl Pts',(-70.6953979633426,-23.0169188841045,
0.));
#141841=CARTESIAN_POINT('Ctrl Pts',(-70.6953979633426,-23.0169188841045,
12.));
#141842=CARTESIAN_POINT('Ctrl Pts',(-70.6678194023135,-23.0200281385833,
0.));
#141843=CARTESIAN_POINT('Ctrl Pts',(-70.6678194023135,-23.0200281385833,
12.));
#141844=CARTESIAN_POINT('Ctrl Pts',(-70.6402726486453,-23.0231086235186,
0.));
#141845=CARTESIAN_POINT('Ctrl Pts',(-70.6402726486453,-23.0231086235186,
12.));
#141846=CARTESIAN_POINT('Ctrl Pts',(-70.6127578036673,-23.026160381013,
0.));
#141847=CARTESIAN_POINT('Ctrl Pts',(-70.6127578036673,-23.026160381013,
12.));
#141848=CARTESIAN_POINT('Ctrl Pts',(-70.5852749754082,-23.0291834570663,
0.));
#141849=CARTESIAN_POINT('Ctrl Pts',(-70.5852749754082,-23.0291834570663,
12.));
#141850=CARTESIAN_POINT('Ctrl Pts',(-70.5578242727627,-23.0321778982711,
0.));
#141851=CARTESIAN_POINT('Ctrl Pts',(-70.5578242727627,-23.0321778982711,
12.));
#141852=CARTESIAN_POINT('Ctrl Pts',(-70.5304057994631,-23.0351437484336,
0.));
#141853=CARTESIAN_POINT('Ctrl Pts',(-70.5304057994631,-23.0351437484336,
12.));
#141854=CARTESIAN_POINT('Ctrl Pts',(-70.5030196492003,-23.0380810458271,
0.));
#141855=CARTESIAN_POINT('Ctrl Pts',(-70.5030196492003,-23.0380810458271,
12.));
#141856=CARTESIAN_POINT('Ctrl Pts',(-70.4756659090209,-23.0409898250756,
0.));
#141857=CARTESIAN_POINT('Ctrl Pts',(-70.4756659090209,-23.0409898250756,
12.));
#141858=CARTESIAN_POINT('Ctrl Pts',(-70.4483446617614,-23.0438701185013,
0.));
#141859=CARTESIAN_POINT('Ctrl Pts',(-70.4483446617614,-23.0438701185013,
12.));
#141860=CARTESIAN_POINT('Ctrl Pts',(-70.4210559889348,-23.0467219577291,
0.));
#141861=CARTESIAN_POINT('Ctrl Pts',(-70.4210559889348,-23.0467219577291,
12.));
#141862=CARTESIAN_POINT('Ctrl Pts',(-70.3937999732267,-23.0495453750763,
0.));
#141863=CARTESIAN_POINT('Ctrl Pts',(-70.3937999732267,-23.0495453750763,
12.));
#141864=CARTESIAN_POINT('Ctrl Pts',(-70.3665767016542,-23.0523404053172,
0.));
#141865=CARTESIAN_POINT('Ctrl Pts',(-70.3665767016542,-23.0523404053172,
12.));
#141866=CARTESIAN_POINT('Ctrl Pts',(-70.3393862652297,-23.0551070854926,
0.));
#141867=CARTESIAN_POINT('Ctrl Pts',(-70.3393862652297,-23.0551070854926,
12.));
#141868=CARTESIAN_POINT('Ctrl Pts',(-70.3122287575335,-23.0578454541104,
0.));
#141869=CARTESIAN_POINT('Ctrl Pts',(-70.3122287575335,-23.0578454541104,
12.));
#141870=CARTESIAN_POINT('Ctrl Pts',(-70.2851042736066,-23.0605555505321,
0.));
#141871=CARTESIAN_POINT('Ctrl Pts',(-70.2851042736066,-23.0605555505321,
12.));
#141872=CARTESIAN_POINT('Ctrl Pts',(-70.2580129087888,-23.0632374143279,
0.));
#141873=CARTESIAN_POINT('Ctrl Pts',(-70.2580129087888,-23.0632374143279,
12.));
#141874=CARTESIAN_POINT('Ctrl Pts',(-70.2309547573815,-23.0658910845433,
0.));
#141875=CARTESIAN_POINT('Ctrl Pts',(-70.2309547573815,-23.0658910845433,
12.));
#141876=CARTESIAN_POINT('Ctrl Pts',(-70.2039299120488,-23.0685165993691,
0.));
#141877=CARTESIAN_POINT('Ctrl Pts',(-70.2039299120488,-23.0685165993691,
12.));
#141878=CARTESIAN_POINT('Ctrl Pts',(-70.1769384645586,-23.071113996544,
0.));
#141879=CARTESIAN_POINT('Ctrl Pts',(-70.1769384645586,-23.071113996544,
12.));
#141880=CARTESIAN_POINT('Ctrl Pts',(-70.1499805062172,-23.0736833135938,
0.));
#141881=CARTESIAN_POINT('Ctrl Pts',(-70.1499805062172,-23.0736833135938,
12.));
#141882=CARTESIAN_POINT('Ctrl Pts',(-70.123056128422,-23.0762245881389,
0.));
#141883=CARTESIAN_POINT('Ctrl Pts',(-70.123056128422,-23.0762245881389,
12.));
#141884=CARTESIAN_POINT('Ctrl Pts',(-70.0961654231639,-23.0787378581774,
0.));
#141885=CARTESIAN_POINT('Ctrl Pts',(-70.0961654231639,-23.0787378581774,
12.));
#141886=CARTESIAN_POINT('Ctrl Pts',(-70.0693084835373,-23.0812231623765,
0.));
#141887=CARTESIAN_POINT('Ctrl Pts',(-70.0693084835373,-23.0812231623765,
12.));
#141888=CARTESIAN_POINT('Ctrl Pts',(-70.0424854035115,-23.0836805399374,
0.));
#141889=CARTESIAN_POINT('Ctrl Pts',(-70.0424854035115,-23.0836805399374,
12.));
#141890=CARTESIAN_POINT('Ctrl Pts',(-70.0156962777169,-23.0861100304729,
0.));
#141891=CARTESIAN_POINT('Ctrl Pts',(-70.0156962777169,-23.0861100304729,
12.));
#141892=CARTESIAN_POINT('Ctrl Pts',(-69.9889412012143,-23.0885116738798,
0.));
#141893=CARTESIAN_POINT('Ctrl Pts',(-69.9889412012143,-23.0885116738798,
12.));
#141894=CARTESIAN_POINT('Ctrl Pts',(-69.9622202692873,-23.0908855102251,
0.));
#141895=CARTESIAN_POINT('Ctrl Pts',(-69.9622202692873,-23.0908855102251,
12.));
#141896=CARTESIAN_POINT('Ctrl Pts',(-69.9355335771729,-23.0932315796068,
0.));
#141897=CARTESIAN_POINT('Ctrl Pts',(-69.9355335771729,-23.0932315796068,
12.));
#141898=CARTESIAN_POINT('Ctrl Pts',(-69.9088812200713,-23.0955499221558,
0.));
#141899=CARTESIAN_POINT('Ctrl Pts',(-69.9088812200713,-23.0955499221558,
12.));
#141900=CARTESIAN_POINT('Ctrl Pts',(-69.8822632932768,-23.0978405781021,
0.));
#141901=CARTESIAN_POINT('Ctrl Pts',(-69.8822632932768,-23.0978405781021,
12.));
#141902=CARTESIAN_POINT('Ctrl Pts',(-69.8556798922693,-23.1001035878241,
0.));
#141903=CARTESIAN_POINT('Ctrl Pts',(-69.8556798922693,-23.1001035878241,
12.));
#141904=CARTESIAN_POINT('Ctrl Pts',(-69.8291311128118,-23.1023389919051,
0.));
#141905=CARTESIAN_POINT('Ctrl Pts',(-69.8291311128118,-23.1023389919051,
12.));
#141906=CARTESIAN_POINT('Ctrl Pts',(-69.8026170510572,-23.1045468311991,
0.));
#141907=CARTESIAN_POINT('Ctrl Pts',(-69.8026170510572,-23.1045468311991,
12.));
#141908=CARTESIAN_POINT('Ctrl Pts',(-69.7761378035964,-23.106727146861,
0.));
#141909=CARTESIAN_POINT('Ctrl Pts',(-69.7761378035964,-23.106727146861,
12.));
#141910=CARTESIAN_POINT('Ctrl Pts',(-69.7496934674069,-23.1088799803089,
0.));
#141911=CARTESIAN_POINT('Ctrl Pts',(-69.7496934674069,-23.1088799803089,
12.));
#141912=CARTESIAN_POINT('Ctrl Pts',(-69.7232841398197,-23.1110053732046,
0.));
#141913=CARTESIAN_POINT('Ctrl Pts',(-69.7232841398197,-23.1110053732046,
12.));
#141914=CARTESIAN_POINT('Ctrl Pts',(-69.6969099184767,-23.1131033674301,
0.));
#141915=CARTESIAN_POINT('Ctrl Pts',(-69.6969099184767,-23.1131033674301,
12.));
#141916=CARTESIAN_POINT('Ctrl Pts',(-69.6705709012852,-23.1151740050681,
0.));
#141917=CARTESIAN_POINT('Ctrl Pts',(-69.6705709012852,-23.1151740050681,
12.));
#141918=CARTESIAN_POINT('Ctrl Pts',(-69.6442671863765,-23.1172173283859,
0.));
#141919=CARTESIAN_POINT('Ctrl Pts',(-69.6442671863765,-23.1172173283859,
12.));
#141920=CARTESIAN_POINT('Ctrl Pts',(-69.6179988721365,-23.1192333798441,
0.));
#141921=CARTESIAN_POINT('Ctrl Pts',(-69.6179988721365,-23.1192333798441,
12.));
#141922=CARTESIAN_POINT('Ctrl Pts',(-69.5917660572265,-23.1212222021051,
0.));
#141923=CARTESIAN_POINT('Ctrl Pts',(-69.5917660572265,-23.1212222021051,
12.));
#141924=CARTESIAN_POINT('Ctrl Pts',(-69.5655688406052,-23.1231838380452,
0.));
#141925=CARTESIAN_POINT('Ctrl Pts',(-69.5655688406052,-23.1231838380452,
12.));
#141926=CARTESIAN_POINT('Ctrl Pts',(-69.539407321546,-23.1251183307676,
0.));
#141927=CARTESIAN_POINT('Ctrl Pts',(-69.539407321546,-23.1251183307676,
12.));
#141928=CARTESIAN_POINT('Ctrl Pts',(-69.5132815996537,-23.1270257236204,
0.));
#141929=CARTESIAN_POINT('Ctrl Pts',(-69.5132815996537,-23.1270257236204,
12.));
#141930=CARTESIAN_POINT('Ctrl Pts',(-69.4871917748654,-23.1289060601924,
0.));
#141931=CARTESIAN_POINT('Ctrl Pts',(-69.4871917748654,-23.1289060601924,
12.));
#141932=CARTESIAN_POINT('Ctrl Pts',(-69.4611379474484,-23.1307593843061,
0.));
#141933=CARTESIAN_POINT('Ctrl Pts',(-69.4611379474484,-23.1307593843061,
12.));
#141934=CARTESIAN_POINT('Ctrl Pts',(-69.4351202179946,-23.1325857400144,
0.));
#141935=CARTESIAN_POINT('Ctrl Pts',(-69.4351202179946,-23.1325857400144,
12.));
#141936=CARTESIAN_POINT('Ctrl Pts',(-69.4091386874132,-23.1343851715989,
0.));
#141937=CARTESIAN_POINT('Ctrl Pts',(-69.4091386874132,-23.1343851715989,
12.));
#141938=CARTESIAN_POINT('Ctrl Pts',(-69.3831934569182,-23.1361577235709,
0.));
#141939=CARTESIAN_POINT('Ctrl Pts',(-69.3831934569182,-23.1361577235709,
12.));
#141940=CARTESIAN_POINT('Ctrl Pts',(-69.3572846280296,-23.1379034406718,
0.));
#141941=CARTESIAN_POINT('Ctrl Pts',(-69.3572846280296,-23.1379034406718,
12.));
#141942=CARTESIAN_POINT('Ctrl Pts',(-69.3314123025869,-23.1396223678725,
0.));
#141943=CARTESIAN_POINT('Ctrl Pts',(-69.3314123025869,-23.1396223678725,
12.));
#141944=CARTESIAN_POINT('Ctrl Pts',(-69.3055765827546,-23.1413145503762,
0.));
#141945=CARTESIAN_POINT('Ctrl Pts',(-69.3055765827546,-23.1413145503762,
12.));
#141946=CARTESIAN_POINT('Ctrl Pts',(-69.2797775710273,-23.142980033622,
0.));
#141947=CARTESIAN_POINT('Ctrl Pts',(-69.2797775710273,-23.142980033622,
12.));
#141948=CARTESIAN_POINT('Ctrl Pts',(-69.254015370231,-23.1446188632931,
0.));
#141949=CARTESIAN_POINT('Ctrl Pts',(-69.254015370231,-23.1446188632931,
12.));
#141950=CARTESIAN_POINT('Ctrl Pts',(-69.2282900835235,-23.1462310853206,
0.));
#141951=CARTESIAN_POINT('Ctrl Pts',(-69.2282900835235,-23.1462310853206,
12.));
#141952=CARTESIAN_POINT('Ctrl Pts',(-69.2026018144028,-23.147816745879,
0.));
#141953=CARTESIAN_POINT('Ctrl Pts',(-69.2026018144028,-23.147816745879,
12.));
#141954=CARTESIAN_POINT('Ctrl Pts',(-69.1769506667084,-23.1493758913859,
0.));
#141955=CARTESIAN_POINT('Ctrl Pts',(-69.1769506667084,-23.1493758913859,
12.));
#141956=CARTESIAN_POINT('Ctrl Pts',(-69.1513367446231,-23.1509085685032,
0.));
#141957=CARTESIAN_POINT('Ctrl Pts',(-69.1513367446231,-23.1509085685032,
12.));
#141958=CARTESIAN_POINT('Ctrl Pts',(-69.1257601526687,-23.152414824141,
0.));
#141959=CARTESIAN_POINT('Ctrl Pts',(-69.1257601526687,-23.152414824141,
12.));
#141960=CARTESIAN_POINT('Ctrl Pts',(-69.1002209957025,-23.1538947054615,
0.));
#141961=CARTESIAN_POINT('Ctrl Pts',(-69.1002209957025,-23.1538947054615,
12.));
#141962=CARTESIAN_POINT('Ctrl Pts',(-69.074719378928,-23.1553482598762,
0.));
#141963=CARTESIAN_POINT('Ctrl Pts',(-69.074719378928,-23.1553482598762,
12.));
#141964=CARTESIAN_POINT('Ctrl Pts',(-69.0492554078992,-23.1567755350469,
0.));
#141965=CARTESIAN_POINT('Ctrl Pts',(-69.0492554078992,-23.1567755350469,
12.));
#141966=CARTESIAN_POINT('Ctrl Pts',(-69.0238291885245,-23.1581765788869,
0.));
#141967=CARTESIAN_POINT('Ctrl Pts',(-69.0238291885245,-23.1581765788869,
12.));
#141968=CARTESIAN_POINT('Ctrl Pts',(-68.9984408270659,-23.1595514395656,
0.));
#141969=CARTESIAN_POINT('Ctrl Pts',(-68.9984408270659,-23.1595514395656,
12.));
#141970=CARTESIAN_POINT('Ctrl Pts',(-68.9730904301369,-23.1609001655156,
0.));
#141971=CARTESIAN_POINT('Ctrl Pts',(-68.9730904301369,-23.1609001655156,
12.));
#141972=CARTESIAN_POINT('Ctrl Pts',(-68.9477781047106,-23.1622228054291,
0.));
#141973=CARTESIAN_POINT('Ctrl Pts',(-68.9477781047106,-23.1622228054291,
12.));
#141974=CARTESIAN_POINT('Ctrl Pts',(-68.9225039581248,-23.1635194082581,
0.));
#141975=CARTESIAN_POINT('Ctrl Pts',(-68.9225039581248,-23.1635194082581,
12.));
#141976=CARTESIAN_POINT('Ctrl Pts',(-68.8972680980842,-23.164790023215,
0.));
#141977=CARTESIAN_POINT('Ctrl Pts',(-68.8972680980842,-23.164790023215,
12.));
#141978=CARTESIAN_POINT('Ctrl Pts',(-68.8720706326609,-23.1660346997764,
0.));
#141979=CARTESIAN_POINT('Ctrl Pts',(-68.8720706326609,-23.1660346997764,
12.));
#141980=CARTESIAN_POINT('Ctrl Pts',(-68.8469116702898,-23.1672534876889,
0.));
#141981=CARTESIAN_POINT('Ctrl Pts',(-68.8469116702898,-23.1672534876889,
12.));
#141982=CARTESIAN_POINT('Ctrl Pts',(-68.8217913197752,-23.1684464369686,
0.));
#141983=CARTESIAN_POINT('Ctrl Pts',(-68.8217913197752,-23.1684464369686,
12.));
#141984=CARTESIAN_POINT('Ctrl Pts',(-68.7967096902996,-23.1696135978997,
0.));
#141985=CARTESIAN_POINT('Ctrl Pts',(-68.7967096902996,-23.1696135978997,
12.));
#141986=CARTESIAN_POINT('Ctrl Pts',(-68.771666891425,-23.170755021036,0.));
#141987=CARTESIAN_POINT('Ctrl Pts',(-68.771666891425,-23.170755021036,12.));
#141988=CARTESIAN_POINT('Ctrl Pts',(-68.746663033096,-23.1718707572043,
0.));
#141989=CARTESIAN_POINT('Ctrl Pts',(-68.746663033096,-23.1718707572043,
12.));
#141990=CARTESIAN_POINT('Ctrl Pts',(-68.7216982256341,-23.172960857511,
0.));
#141991=CARTESIAN_POINT('Ctrl Pts',(-68.7216982256341,-23.172960857511,
12.));
#141992=CARTESIAN_POINT('Ctrl Pts',(-68.696772579744,-23.1740253733417,
0.));
#141993=CARTESIAN_POINT('Ctrl Pts',(-68.696772579744,-23.1740253733417,
12.));
#141994=CARTESIAN_POINT('Ctrl Pts',(-68.6718862065216,-23.1750643563602,
0.));
#141995=CARTESIAN_POINT('Ctrl Pts',(-68.6718862065216,-23.1750643563602,
12.));
#141996=CARTESIAN_POINT('Ctrl Pts',(-68.6470392174564,-23.1760778585092,
0.));
#141997=CARTESIAN_POINT('Ctrl Pts',(-68.6470392174564,-23.1760778585092,
12.));
#141998=CARTESIAN_POINT('Ctrl Pts',(-68.6222317244341,-23.1770659320138,
0.));
#141999=CARTESIAN_POINT('Ctrl Pts',(-68.6222317244341,-23.1770659320138,
12.));
#142000=CARTESIAN_POINT('Ctrl Pts',(-68.597463839733,-23.1780286293875,
0.));
#142001=CARTESIAN_POINT('Ctrl Pts',(-68.597463839733,-23.1780286293875,
12.));
#142002=CARTESIAN_POINT('Ctrl Pts',(-68.5727356760278,-23.1789660034342,
0.));
#142003=CARTESIAN_POINT('Ctrl Pts',(-68.5727356760278,-23.1789660034342,
12.));
#142004=CARTESIAN_POINT('Ctrl Pts',(-68.5480473463985,-23.179878107245,
0.));
#142005=CARTESIAN_POINT('Ctrl Pts',(-68.5480473463985,-23.179878107245,
12.));
#142006=CARTESIAN_POINT('Ctrl Pts',(-68.5233989643345,-23.180764994201,
0.));
#142007=CARTESIAN_POINT('Ctrl Pts',(-68.5233989643345,-23.180764994201,
12.));
#142008=CARTESIAN_POINT('Ctrl Pts',(-68.4987906437356,-23.1816267179751,
0.));
#142009=CARTESIAN_POINT('Ctrl Pts',(-68.4987906437356,-23.1816267179751,
12.));
#142010=CARTESIAN_POINT('Ctrl Pts',(-68.4742224989098,-23.1824633325385,
0.));
#142011=CARTESIAN_POINT('Ctrl Pts',(-68.4742224989098,-23.1824633325385,
12.));
#142012=CARTESIAN_POINT('Ctrl Pts',(-68.4496946445758,-23.183274892163,
0.));
#142013=CARTESIAN_POINT('Ctrl Pts',(-68.4496946445758,-23.183274892163,
12.));
#142014=CARTESIAN_POINT('Ctrl Pts',(-68.4252071958729,-23.1840614514192,
0.));
#142015=CARTESIAN_POINT('Ctrl Pts',(-68.4252071958729,-23.1840614514192,
12.));
#142016=CARTESIAN_POINT('Ctrl Pts',(-68.4007602683652,-23.1848230651777,
0.));
#142017=CARTESIAN_POINT('Ctrl Pts',(-68.4007602683652,-23.1848230651777,
12.));
#142018=CARTESIAN_POINT('Ctrl Pts',(-68.376353978044,-23.1855597886116,
0.));
#142019=CARTESIAN_POINT('Ctrl Pts',(-68.376353978044,-23.1855597886116,
12.));
#142020=CARTESIAN_POINT('Ctrl Pts',(-68.3519884413246,-23.1862716772031,
0.));
#142021=CARTESIAN_POINT('Ctrl Pts',(-68.3519884413246,-23.1862716772031,
12.));
#142022=CARTESIAN_POINT('Ctrl Pts',(-68.3276637750485,-23.1869587867459,
0.));
#142023=CARTESIAN_POINT('Ctrl Pts',(-68.3276637750485,-23.1869587867459,
12.));
#142024=CARTESIAN_POINT('Ctrl Pts',(-68.3033800964939,-23.1876211733436,
0.));
#142025=CARTESIAN_POINT('Ctrl Pts',(-68.3033800964939,-23.1876211733436,
12.));
#142026=CARTESIAN_POINT('Ctrl Pts',(-68.2791375233795,-23.1882588934107,
0.));
#142027=CARTESIAN_POINT('Ctrl Pts',(-68.2791375233795,-23.1882588934107,
12.));
#142028=CARTESIAN_POINT('Ctrl Pts',(-68.2549361738681,-23.1888720036757,
0.));
#142029=CARTESIAN_POINT('Ctrl Pts',(-68.2549361738681,-23.1888720036757,
12.));
#142030=CARTESIAN_POINT('Ctrl Pts',(-68.2307761665633,-23.1894605611871,
0.));
#142031=CARTESIAN_POINT('Ctrl Pts',(-68.2307761665633,-23.1894605611871,
12.));
#142032=CARTESIAN_POINT('Ctrl Pts',(-68.2066576205116,-23.1900246233165,
0.));
#142033=CARTESIAN_POINT('Ctrl Pts',(-68.2066576205116,-23.1900246233165,
12.));
#142034=CARTESIAN_POINT('Ctrl Pts',(-68.1825806552129,-23.1905642477571,
0.));
#142035=CARTESIAN_POINT('Ctrl Pts',(-68.1825806552129,-23.1905642477571,
12.));
#142036=CARTESIAN_POINT('Ctrl Pts',(-68.1585453906257,-23.1910794925251,
0.));
#142037=CARTESIAN_POINT('Ctrl Pts',(-68.1585453906257,-23.1910794925251,
12.));
#142038=CARTESIAN_POINT('Ctrl Pts',(-68.1345519471695,-23.1915704159623,
0.));
#142039=CARTESIAN_POINT('Ctrl Pts',(-68.1345519471695,-23.1915704159623,
12.));
#142040=CARTESIAN_POINT('Ctrl Pts',(-68.110600445723,-23.1920370767426,
0.));
#142041=CARTESIAN_POINT('Ctrl Pts',(-68.110600445723,-23.1920370767426,
12.));
#142042=CARTESIAN_POINT('Ctrl Pts',(-68.0866910076251,-23.1924795338749,
0.));
#142043=CARTESIAN_POINT('Ctrl Pts',(-68.0866910076251,-23.1924795338749,
12.));
#142044=CARTESIAN_POINT('Ctrl Pts',(-68.0628237546863,-23.1928978467021,
0.));
#142045=CARTESIAN_POINT('Ctrl Pts',(-68.0628237546863,-23.1928978467021,
12.));
#142046=CARTESIAN_POINT('Ctrl Pts',(-68.0389988091933,-23.1932920749023,
0.));
#142047=CARTESIAN_POINT('Ctrl Pts',(-68.0389988091933,-23.1932920749023,
12.));
#142048=CARTESIAN_POINT('Ctrl Pts',(-68.0152162939121,-23.1936622784919,
0.));
#142049=CARTESIAN_POINT('Ctrl Pts',(-68.0152162939121,-23.1936622784919,
12.));
#142050=CARTESIAN_POINT('Ctrl Pts',(-67.991476332086,-23.1940085178313,
0.));
#142051=CARTESIAN_POINT('Ctrl Pts',(-67.991476332086,-23.1940085178313,
12.));
#142052=CARTESIAN_POINT('Ctrl Pts',(-67.9677790474385,-23.1943308536297,
0.));
#142053=CARTESIAN_POINT('Ctrl Pts',(-67.9677790474385,-23.1943308536297,
12.));
#142054=CARTESIAN_POINT('Ctrl Pts',(-67.9441245641842,-23.1946293469427,
0.));
#142055=CARTESIAN_POINT('Ctrl Pts',(-67.9441245641842,-23.1946293469427,
12.));
#142056=CARTESIAN_POINT('Ctrl Pts',(-67.9205130070324,-23.1949040591744,
0.));
#142057=CARTESIAN_POINT('Ctrl Pts',(-67.9205130070324,-23.1949040591744,
12.));
#142058=CARTESIAN_POINT('Ctrl Pts',(-67.8969445011916,-23.1951550520802,
0.));
#142059=CARTESIAN_POINT('Ctrl Pts',(-67.8969445011916,-23.1951550520802,
12.));
#142060=CARTESIAN_POINT('Ctrl Pts',(-67.8734191723667,-23.1953823877734,
0.));
#142061=CARTESIAN_POINT('Ctrl Pts',(-67.8734191723667,-23.1953823877734,
12.));
#142062=CARTESIAN_POINT('Ctrl Pts',(-67.8499371467616,-23.1955861287286,
0.));
#142063=CARTESIAN_POINT('Ctrl Pts',(-67.8499371467616,-23.1955861287286,
12.));
#142064=CARTESIAN_POINT('Ctrl Pts',(-67.8264985510917,-23.1957663377807,
0.));
#142065=CARTESIAN_POINT('Ctrl Pts',(-67.8264985510917,-23.1957663377807,
12.));
#142066=CARTESIAN_POINT('Ctrl Pts',(-67.8031035125887,-23.1959230781269,
0.));
#142067=CARTESIAN_POINT('Ctrl Pts',(-67.8031035125887,-23.1959230781269,
12.));
#142068=CARTESIAN_POINT('Ctrl Pts',(-67.7797521590045,-23.1960564133304,
0.));
#142069=CARTESIAN_POINT('Ctrl Pts',(-67.7797521590045,-23.1960564133304,
12.));
#142070=CARTESIAN_POINT('Ctrl Pts',(-67.7564446186079,-23.1961664073262,
0.));
#142071=CARTESIAN_POINT('Ctrl Pts',(-67.7564446186079,-23.1961664073262,
12.));
#142072=CARTESIAN_POINT('Ctrl Pts',(-67.7331810201883,-23.1962531244245,
0.));
#142073=CARTESIAN_POINT('Ctrl Pts',(-67.7331810201883,-23.1962531244245,
12.));
#142074=CARTESIAN_POINT('Ctrl Pts',(-67.7099614930671,-23.1963166293102,
0.));
#142075=CARTESIAN_POINT('Ctrl Pts',(-67.7099614930671,-23.1963166293102,
12.));
#142076=CARTESIAN_POINT('Ctrl Pts',(-67.6867861671031,-23.1963569870451,
0.));
#142077=CARTESIAN_POINT('Ctrl Pts',(-67.6867861671031,-23.1963569870451,
12.));
#142078=CARTESIAN_POINT('Ctrl Pts',(-67.6636551726964,-23.1963742630715,
0.));
#142079=CARTESIAN_POINT('Ctrl Pts',(-67.6636551726964,-23.1963742630715,
12.));
#142080=CARTESIAN_POINT('Ctrl Pts',(-67.6405686407863,-23.1963685232188,
0.));
#142081=CARTESIAN_POINT('Ctrl Pts',(-67.6405686407863,-23.1963685232188,
12.));
#142082=CARTESIAN_POINT('Ctrl Pts',(-67.6175267028555,-23.1963398337069,
0.));
#142083=CARTESIAN_POINT('Ctrl Pts',(-67.6175267028555,-23.1963398337069,
12.));
#142084=CARTESIAN_POINT('Ctrl Pts',(-67.5945294909426,-23.1962882611453,
0.));
#142085=CARTESIAN_POINT('Ctrl Pts',(-67.5945294909426,-23.1962882611453,
12.));
#142086=CARTESIAN_POINT('Ctrl Pts',(-67.5715771376461,-23.196213872536,
0.));
#142087=CARTESIAN_POINT('Ctrl Pts',(-67.5715771376461,-23.196213872536,
12.));
#142088=CARTESIAN_POINT('Ctrl Pts',(-67.5486697761288,-23.1961167352772,
0.));
#142089=CARTESIAN_POINT('Ctrl Pts',(-67.5486697761288,-23.1961167352772,
12.));
#142090=CARTESIAN_POINT('Ctrl Pts',(-67.5258075401146,-23.1959969171701,
0.));
#142091=CARTESIAN_POINT('Ctrl Pts',(-67.5258075401146,-23.1959969171701,
12.));
#142092=CARTESIAN_POINT('Ctrl Pts',(-67.5029905638949,-23.1958544864215,
0.));
#142093=CARTESIAN_POINT('Ctrl Pts',(-67.5029905638949,-23.1958544864215,
12.));
#142094=CARTESIAN_POINT('Ctrl Pts',(-67.4802189823408,-23.195689511644,
0.));
#142095=CARTESIAN_POINT('Ctrl Pts',(-67.4802189823408,-23.195689511644,
12.));
#142096=CARTESIAN_POINT('Ctrl Pts',(-67.4574929309076,-23.195502061859,
0.));
#142097=CARTESIAN_POINT('Ctrl Pts',(-67.4574929309076,-23.195502061859,
12.));
#142098=CARTESIAN_POINT('Ctrl Pts',(-67.4348125456398,-23.1952922065012,
0.));
#142099=CARTESIAN_POINT('Ctrl Pts',(-67.4348125456398,-23.1952922065012,
12.));
#142100=CARTESIAN_POINT('Ctrl Pts',(-67.412177963168,-23.1950600154265,
0.));
#142101=CARTESIAN_POINT('Ctrl Pts',(-67.412177963168,-23.1950600154265,
12.));
#142102=CARTESIAN_POINT('Ctrl Pts',(-67.3895893207182,-23.1948055589129,
0.));
#142103=CARTESIAN_POINT('Ctrl Pts',(-67.3895893207182,-23.1948055589129,
12.));
#142104=CARTESIAN_POINT('Ctrl Pts',(-67.3670467561212,-23.194528907661,
0.));
#142105=CARTESIAN_POINT('Ctrl Pts',(-67.3670467561212,-23.194528907661,
12.));
#142106=CARTESIAN_POINT('Ctrl Pts',(-67.3445504078176,-23.1942301327978,
0.));
#142107=CARTESIAN_POINT('Ctrl Pts',(-67.3445504078176,-23.1942301327978,
12.));
#142108=CARTESIAN_POINT('Ctrl Pts',(-67.3221004148603,-23.1939093058801,
0.));
#142109=CARTESIAN_POINT('Ctrl Pts',(-67.3221004148603,-23.1939093058801,
12.));
#142110=CARTESIAN_POINT('Ctrl Pts',(-67.2996969169098,-23.1935664989018,
0.));
#142111=CARTESIAN_POINT('Ctrl Pts',(-67.2996969169098,-23.1935664989018,
12.));
#142112=CARTESIAN_POINT('Ctrl Pts',(-67.2773400542477,-23.1932017842953,
0.));
#142113=CARTESIAN_POINT('Ctrl Pts',(-67.2773400542477,-23.1932017842953,
12.));
#142114=CARTESIAN_POINT('Ctrl Pts',(-67.2550299677888,-23.1928152349343,
0.));
#142115=CARTESIAN_POINT('Ctrl Pts',(-67.2550299677888,-23.1928152349343,
12.));
#142116=CARTESIAN_POINT('Ctrl Pts',(-67.232766799088,-23.1924069241385,
0.));
#142117=CARTESIAN_POINT('Ctrl Pts',(-67.232766799088,-23.1924069241385,
12.));
#142118=CARTESIAN_POINT('Ctrl Pts',(-67.2105506903447,-23.1919769256803,
0.));
#142119=CARTESIAN_POINT('Ctrl Pts',(-67.2105506903447,-23.1919769256803,
12.));
#142120=CARTESIAN_POINT('Ctrl Pts',(-67.1883817844038,-23.1915253137924,
0.));
#142121=CARTESIAN_POINT('Ctrl Pts',(-67.1883817844038,-23.1915253137924,
12.));
#142122=CARTESIAN_POINT('Ctrl Pts',(-67.1662602247639,-23.1910521631657,
0.));
#142123=CARTESIAN_POINT('Ctrl Pts',(-67.1662602247639,-23.1910521631657,
12.));
#142124=CARTESIAN_POINT('Ctrl Pts',(-67.1441861555817,-23.1905575489505,
0.));
#142125=CARTESIAN_POINT('Ctrl Pts',(-67.1441861555817,-23.1905575489505,
12.));
#142126=CARTESIAN_POINT('Ctrl Pts',(-67.1221597216741,-23.1900415467574,
0.));
#142127=CARTESIAN_POINT('Ctrl Pts',(-67.1221597216741,-23.1900415467574,
12.));
#142128=CARTESIAN_POINT('Ctrl Pts',(-67.1001810685143,-23.1895042326627,
0.));
#142129=CARTESIAN_POINT('Ctrl Pts',(-67.1001810685143,-23.1895042326627,
12.));
#142130=CARTESIAN_POINT('Ctrl Pts',(-67.0782503422305,-23.1889456832119,
0.));
#142131=CARTESIAN_POINT('Ctrl Pts',(-67.0782503422305,-23.1889456832119,
12.));
#142132=CARTESIAN_POINT('Ctrl Pts',(-67.0563676896325,-23.1883659754271,
0.));
#142133=CARTESIAN_POINT('Ctrl Pts',(-67.0563676896325,-23.1883659754271,
12.));
#142134=CARTESIAN_POINT('Ctrl Pts',(-67.0345332582306,-23.1877651868158,
0.));
#142135=CARTESIAN_POINT('Ctrl Pts',(-67.0345332582306,-23.1877651868158,
12.));
#142136=CARTESIAN_POINT('Ctrl Pts',(-67.0127471962501,-23.1871433953793,
0.));
#142137=CARTESIAN_POINT('Ctrl Pts',(-67.0127471962501,-23.1871433953793,
12.));
#142138=CARTESIAN_POINT('Ctrl Pts',(-66.9910096526462,-23.1865006796284,
0.));
#142139=CARTESIAN_POINT('Ctrl Pts',(-66.9910096526462,-23.1865006796284,
12.));
#142140=CARTESIAN_POINT('Ctrl Pts',(-66.9693207771031,-23.1858371185842,
0.));
#142141=CARTESIAN_POINT('Ctrl Pts',(-66.9693207771031,-23.1858371185842,
12.));
#142142=CARTESIAN_POINT('Ctrl Pts',(-66.9476807200203,-23.1851527917657,
0.));
#142143=CARTESIAN_POINT('Ctrl Pts',(-66.9476807200203,-23.1851527917657,
12.));
#142144=CARTESIAN_POINT('Ctrl Pts',(-66.9260896324949,-23.1844477791814,
0.));
#142145=CARTESIAN_POINT('Ctrl Pts',(-66.9260896324949,-23.1844477791814,
12.));
#142146=CARTESIAN_POINT('Ctrl Pts',(-66.9045476663063,-23.1837221613235,
0.));
#142147=CARTESIAN_POINT('Ctrl Pts',(-66.9045476663063,-23.1837221613235,
12.));
#142148=CARTESIAN_POINT('Ctrl Pts',(-66.8830549738795,-23.1829760191591,
0.));
#142149=CARTESIAN_POINT('Ctrl Pts',(-66.8830549738795,-23.1829760191591,
12.));
#142150=CARTESIAN_POINT('Ctrl Pts',(-66.8616117083331,-23.1822094341517,
0.));
#142151=CARTESIAN_POINT('Ctrl Pts',(-66.8616117083331,-23.1822094341517,
12.));
#142152=CARTESIAN_POINT('Ctrl Pts',(-66.8402180235566,-23.1814224882954,
0.));
#142153=CARTESIAN_POINT('Ctrl Pts',(-66.8402180235566,-23.1814224882954,
12.));
#142154=CARTESIAN_POINT('Ctrl Pts',(-66.8188740742727,-23.1806152641475,
0.));
#142155=CARTESIAN_POINT('Ctrl Pts',(-66.8188740742727,-23.1806152641475,
12.));
#142156=CARTESIAN_POINT('Ctrl Pts',(-66.7975800161,-23.1797878448639,0.));
#142157=CARTESIAN_POINT('Ctrl Pts',(-66.7975800161,-23.1797878448639,12.));
#142158=CARTESIAN_POINT('Ctrl Pts',(-66.776336005612,-23.1789403142366,
0.));
#142159=CARTESIAN_POINT('Ctrl Pts',(-66.776336005612,-23.1789403142366,
12.));
#142160=CARTESIAN_POINT('Ctrl Pts',(-66.7551422002204,-23.17807275663,0.));
#142161=CARTESIAN_POINT('Ctrl Pts',(-66.7551422002204,-23.17807275663,12.));
#142162=CARTESIAN_POINT('Ctrl Pts',(-66.7339987580427,-23.1771852569131,
0.));
#142163=CARTESIAN_POINT('Ctrl Pts',(-66.7339987580427,-23.1771852569131,
12.));
#142164=CARTESIAN_POINT('Ctrl Pts',(-66.7129058377896,-23.1762779004044,
0.));
#142165=CARTESIAN_POINT('Ctrl Pts',(-66.7129058377896,-23.1762779004044,
12.));
#142166=CARTESIAN_POINT('Ctrl Pts',(-66.6918635985972,-23.1753507727939,
0.));
#142167=CARTESIAN_POINT('Ctrl Pts',(-66.6918635985972,-23.1753507727939,
12.));
#142168=CARTESIAN_POINT('Ctrl Pts',(-66.6708722000079,-23.1744039601382,
0.));
#142169=CARTESIAN_POINT('Ctrl Pts',(-66.6708722000079,-23.1744039601382,
12.));
#142170=CARTESIAN_POINT('Ctrl Pts',(-66.6499318023473,-23.1734375490431,
0.));
#142171=CARTESIAN_POINT('Ctrl Pts',(-66.6499318023473,-23.1734375490431,
12.));
#142172=CARTESIAN_POINT('Ctrl Pts',(-66.6290425670548,-23.1724516268302,
0.));
#142173=CARTESIAN_POINT('Ctrl Pts',(-66.6290425670548,-23.1724516268302,
12.));
#142174=CARTESIAN_POINT('Ctrl Pts',(-66.6082046569644,-23.1714462816789,
0.));
#142175=CARTESIAN_POINT('Ctrl Pts',(-66.6082046569644,-23.1714462816789,
12.));
#142176=CARTESIAN_POINT('Ctrl Pts',(-66.5874182367563,-23.1704216028614,
0.));
#142177=CARTESIAN_POINT('Ctrl Pts',(-66.5874182367563,-23.1704216028614,
12.));
#142178=CARTESIAN_POINT('Ctrl Pts',(-66.5666834726454,-23.1693776805866,
0.));
#142179=CARTESIAN_POINT('Ctrl Pts',(-66.5666834726454,-23.1693776805866,
12.));
#142180=CARTESIAN_POINT('Ctrl Pts',(-66.5460005315376,-23.1683146055726,
0.));
#142181=CARTESIAN_POINT('Ctrl Pts',(-66.5460005315376,-23.1683146055726,
12.));
#142182=CARTESIAN_POINT('Ctrl Pts',(-66.5253695803205,-23.1672324686926,
0.));
#142183=CARTESIAN_POINT('Ctrl Pts',(-66.5253695803205,-23.1672324686926,
12.));
#142184=CARTESIAN_POINT('Ctrl Pts',(-66.5047907851348,-23.1661313606132,
0.));
#142185=CARTESIAN_POINT('Ctrl Pts',(-66.5047907851348,-23.1661313606132,
12.));
#142186=CARTESIAN_POINT('Ctrl Pts',(-66.4842643105311,-23.1650113713808,
0.));
#142187=CARTESIAN_POINT('Ctrl Pts',(-66.4842643105311,-23.1650113713808,
12.));
#142188=CARTESIAN_POINT('Ctrl Pts',(-66.4637903210727,-23.1638725912195,
0.));
#142189=CARTESIAN_POINT('Ctrl Pts',(-66.4637903210727,-23.1638725912195,
12.));
#142190=CARTESIAN_POINT('Ctrl Pts',(-66.4433689832478,-23.1627151114883,
0.));
#142191=CARTESIAN_POINT('Ctrl Pts',(-66.4433689832478,-23.1627151114883,
12.));
#142192=CARTESIAN_POINT('Ctrl Pts',(-66.4230004670278,-23.1615390254632,
0.));
#142193=CARTESIAN_POINT('Ctrl Pts',(-66.4230004670278,-23.1615390254632,
12.));
#142194=CARTESIAN_POINT('Ctrl Pts',(-66.4026849481232,-23.160344429474,
0.));
#142195=CARTESIAN_POINT('Ctrl Pts',(-66.4026849481232,-23.160344429474,
12.));
#142196=CARTESIAN_POINT('Ctrl Pts',(-66.3824226081801,-23.1591314230083,
0.));
#142197=CARTESIAN_POINT('Ctrl Pts',(-66.3824226081801,-23.1591314230083,
12.));
#142198=CARTESIAN_POINT('Ctrl Pts',(-66.3622136300654,-23.1579001063424,
0.));
#142199=CARTESIAN_POINT('Ctrl Pts',(-66.3622136300654,-23.1579001063424,
12.));
#142200=CARTESIAN_POINT('Ctrl Pts',(-66.3420581937147,-23.1566505784621,
0.));
#142201=CARTESIAN_POINT('Ctrl Pts',(-66.3420581937147,-23.1566505784621,
12.));
#142202=CARTESIAN_POINT('Ctrl Pts',(-66.3219564725184,-23.1553829352539,
0.));
#142203=CARTESIAN_POINT('Ctrl Pts',(-66.3219564725184,-23.1553829352539,
12.));
#142204=CARTESIAN_POINT('Ctrl Pts',(-66.3019086275444,-23.1540972666191,
0.));
#142205=CARTESIAN_POINT('Ctrl Pts',(-66.3019086275444,-23.1540972666191,
12.));
#142206=CARTESIAN_POINT('Ctrl Pts',(-66.281914813114,-23.1527936592651,
0.));
#142207=CARTESIAN_POINT('Ctrl Pts',(-66.281914813114,-23.1527936592651,
12.));
#142208=CARTESIAN_POINT('Ctrl Pts',(-66.2619751878793,-23.1514722022503,
0.));
#142209=CARTESIAN_POINT('Ctrl Pts',(-66.2619751878793,-23.1514722022503,
12.));
#142210=CARTESIAN_POINT('Ctrl Pts',(-66.2420899237318,-23.1501329914488,
0.));
#142211=CARTESIAN_POINT('Ctrl Pts',(-66.2420899237318,-23.1501329914488,
12.));
#142212=CARTESIAN_POINT('Ctrl Pts',(-66.2222592165398,-23.1487761349298,
0.));
#142213=CARTESIAN_POINT('Ctrl Pts',(-66.2222592165398,-23.1487761349298,
12.));
#142214=CARTESIAN_POINT('Ctrl Pts',(-66.2024832934733,-23.147401756643,
0.));
#142215=CARTESIAN_POINT('Ctrl Pts',(-66.2024832934733,-23.147401756643,
12.));
#142216=CARTESIAN_POINT('Ctrl Pts',(-66.1827623902755,-23.1460099850704,
0.));
#142217=CARTESIAN_POINT('Ctrl Pts',(-66.1827623902755,-23.1460099850704,
12.));
#142218=CARTESIAN_POINT('Ctrl Pts',(-66.163096729667,-23.1446009424872,
0.));
#142219=CARTESIAN_POINT('Ctrl Pts',(-66.163096729667,-23.1446009424872,
12.));
#142220=CARTESIAN_POINT('Ctrl Pts',(-66.14348650151,-23.1431747350127,0.));
#142221=CARTESIAN_POINT('Ctrl Pts',(-66.14348650151,-23.1431747350127,12.));
#142222=CARTESIAN_POINT('Ctrl Pts',(-66.1239318368803,-23.1417314398501,
0.));
#142223=CARTESIAN_POINT('Ctrl Pts',(-66.1239318368803,-23.1417314398501,
12.));
#142224=CARTESIAN_POINT('Ctrl Pts',(-66.1044328067739,-23.140271103958,
0.));
#142225=CARTESIAN_POINT('Ctrl Pts',(-66.1044328067739,-23.140271103958,
12.));
#142226=CARTESIAN_POINT('Ctrl Pts',(-66.0888781152779,-23.1390892229923,
0.));
#142227=CARTESIAN_POINT('Ctrl Pts',(-66.0888781152779,-23.1390892229923,
12.));
#142228=CARTESIAN_POINT('Ctrl Pts',(-66.0772371487475,-23.1381951597491,
0.));
#142229=CARTESIAN_POINT('Ctrl Pts',(-66.0772371487475,-23.1381951597491,
12.));
#142230=CARTESIAN_POINT('Ctrl Pts',(-66.0694876382212,-23.1375957166138,
0.));
#142231=CARTESIAN_POINT('Ctrl Pts',(-66.0694876382212,-23.1375957166138,
12.));
#142232=CARTESIAN_POINT('Ctrl Pts',(-66.0656156664138,-23.1372951448024,
0.));
#142233=CARTESIAN_POINT('Ctrl Pts',(-66.0656156664138,-23.1372951448024,
12.));
#142234=CARTESIAN_POINT('',(-66.0656156664138,-23.1372951448024,12.));
#142235=CARTESIAN_POINT('Ctrl Pts',(-66.0656156664138,-23.1372951448024,
12.));
#142236=CARTESIAN_POINT('Ctrl Pts',(-66.0694876382212,-23.1375957166138,
12.));
#142237=CARTESIAN_POINT('Ctrl Pts',(-66.0772371487475,-23.1381951597491,
12.));
#142238=CARTESIAN_POINT('Ctrl Pts',(-66.0888781152779,-23.1390892229923,
12.));
#142239=CARTESIAN_POINT('Ctrl Pts',(-66.1044328067739,-23.140271103958,
12.));
#142240=CARTESIAN_POINT('Ctrl Pts',(-66.1239318368803,-23.1417314398501,
12.));
#142241=CARTESIAN_POINT('Ctrl Pts',(-66.14348650151,-23.1431747350127,12.));
#142242=CARTESIAN_POINT('Ctrl Pts',(-66.163096729667,-23.1446009424872,
12.));
#142243=CARTESIAN_POINT('Ctrl Pts',(-66.1827623902755,-23.1460099850704,
12.));
#142244=CARTESIAN_POINT('Ctrl Pts',(-66.2024832934733,-23.147401756643,
12.));
#142245=CARTESIAN_POINT('Ctrl Pts',(-66.2222592165398,-23.1487761349298,
12.));
#142246=CARTESIAN_POINT('Ctrl Pts',(-66.2420899237318,-23.1501329914488,
12.));
#142247=CARTESIAN_POINT('Ctrl Pts',(-66.2619751878793,-23.1514722022503,
12.));
#142248=CARTESIAN_POINT('Ctrl Pts',(-66.281914813114,-23.1527936592651,
12.));
#142249=CARTESIAN_POINT('Ctrl Pts',(-66.3019086275444,-23.1540972666191,
12.));
#142250=CARTESIAN_POINT('Ctrl Pts',(-66.3219564725184,-23.1553829352539,
12.));
#142251=CARTESIAN_POINT('Ctrl Pts',(-66.3420581937147,-23.1566505784621,
12.));
#142252=CARTESIAN_POINT('Ctrl Pts',(-66.3622136300654,-23.1579001063424,
12.));
#142253=CARTESIAN_POINT('Ctrl Pts',(-66.3824226081801,-23.1591314230083,
12.));
#142254=CARTESIAN_POINT('Ctrl Pts',(-66.4026849481232,-23.160344429474,
12.));
#142255=CARTESIAN_POINT('Ctrl Pts',(-66.4230004670278,-23.1615390254632,
12.));
#142256=CARTESIAN_POINT('Ctrl Pts',(-66.4433689832478,-23.1627151114883,
12.));
#142257=CARTESIAN_POINT('Ctrl Pts',(-66.4637903210727,-23.1638725912195,
12.));
#142258=CARTESIAN_POINT('Ctrl Pts',(-66.4842643105311,-23.1650113713808,
12.));
#142259=CARTESIAN_POINT('Ctrl Pts',(-66.5047907851348,-23.1661313606132,
12.));
#142260=CARTESIAN_POINT('Ctrl Pts',(-66.5253695803205,-23.1672324686926,
12.));
#142261=CARTESIAN_POINT('Ctrl Pts',(-66.5460005315376,-23.1683146055726,
12.));
#142262=CARTESIAN_POINT('Ctrl Pts',(-66.5666834726454,-23.1693776805866,
12.));
#142263=CARTESIAN_POINT('Ctrl Pts',(-66.5874182367563,-23.1704216028614,
12.));
#142264=CARTESIAN_POINT('Ctrl Pts',(-66.6082046569644,-23.1714462816789,
12.));
#142265=CARTESIAN_POINT('Ctrl Pts',(-66.6290425670548,-23.1724516268302,
12.));
#142266=CARTESIAN_POINT('Ctrl Pts',(-66.6499318023473,-23.1734375490431,
12.));
#142267=CARTESIAN_POINT('Ctrl Pts',(-66.6708722000079,-23.1744039601382,
12.));
#142268=CARTESIAN_POINT('Ctrl Pts',(-66.6918635985972,-23.1753507727939,
12.));
#142269=CARTESIAN_POINT('Ctrl Pts',(-66.7129058377896,-23.1762779004044,
12.));
#142270=CARTESIAN_POINT('Ctrl Pts',(-66.7339987580427,-23.1771852569131,
12.));
#142271=CARTESIAN_POINT('Ctrl Pts',(-66.7551422002204,-23.17807275663,12.));
#142272=CARTESIAN_POINT('Ctrl Pts',(-66.776336005612,-23.1789403142366,
12.));
#142273=CARTESIAN_POINT('Ctrl Pts',(-66.7975800161,-23.1797878448639,12.));
#142274=CARTESIAN_POINT('Ctrl Pts',(-66.8188740742727,-23.1806152641475,
12.));
#142275=CARTESIAN_POINT('Ctrl Pts',(-66.8402180235566,-23.1814224882954,
12.));
#142276=CARTESIAN_POINT('Ctrl Pts',(-66.8616117083331,-23.1822094341517,
12.));
#142277=CARTESIAN_POINT('Ctrl Pts',(-66.8830549738795,-23.1829760191591,
12.));
#142278=CARTESIAN_POINT('Ctrl Pts',(-66.9045476663063,-23.1837221613235,
12.));
#142279=CARTESIAN_POINT('Ctrl Pts',(-66.9260896324949,-23.1844477791814,
12.));
#142280=CARTESIAN_POINT('Ctrl Pts',(-66.9476807200203,-23.1851527917657,
12.));
#142281=CARTESIAN_POINT('Ctrl Pts',(-66.9693207771031,-23.1858371185842,
12.));
#142282=CARTESIAN_POINT('Ctrl Pts',(-66.9910096526462,-23.1865006796284,
12.));
#142283=CARTESIAN_POINT('Ctrl Pts',(-67.0127471962501,-23.1871433953793,
12.));
#142284=CARTESIAN_POINT('Ctrl Pts',(-67.0345332582306,-23.1877651868158,
12.));
#142285=CARTESIAN_POINT('Ctrl Pts',(-67.0563676896325,-23.1883659754271,
12.));
#142286=CARTESIAN_POINT('Ctrl Pts',(-67.0782503422305,-23.1889456832119,
12.));
#142287=CARTESIAN_POINT('Ctrl Pts',(-67.1001810685143,-23.1895042326627,
12.));
#142288=CARTESIAN_POINT('Ctrl Pts',(-67.1221597216741,-23.1900415467574,
12.));
#142289=CARTESIAN_POINT('Ctrl Pts',(-67.1441861555817,-23.1905575489505,
12.));
#142290=CARTESIAN_POINT('Ctrl Pts',(-67.1662602247639,-23.1910521631657,
12.));
#142291=CARTESIAN_POINT('Ctrl Pts',(-67.1883817844038,-23.1915253137924,
12.));
#142292=CARTESIAN_POINT('Ctrl Pts',(-67.2105506903447,-23.1919769256803,
12.));
#142293=CARTESIAN_POINT('Ctrl Pts',(-67.232766799088,-23.1924069241385,
12.));
#142294=CARTESIAN_POINT('Ctrl Pts',(-67.2550299677888,-23.1928152349343,
12.));
#142295=CARTESIAN_POINT('Ctrl Pts',(-67.2773400542477,-23.1932017842953,
12.));
#142296=CARTESIAN_POINT('Ctrl Pts',(-67.2996969169098,-23.1935664989018,
12.));
#142297=CARTESIAN_POINT('Ctrl Pts',(-67.3221004148603,-23.1939093058801,
12.));
#142298=CARTESIAN_POINT('Ctrl Pts',(-67.3445504078176,-23.1942301327978,
12.));
#142299=CARTESIAN_POINT('Ctrl Pts',(-67.3670467561212,-23.194528907661,
12.));
#142300=CARTESIAN_POINT('Ctrl Pts',(-67.3895893207182,-23.1948055589129,
12.));
#142301=CARTESIAN_POINT('Ctrl Pts',(-67.412177963168,-23.1950600154265,
12.));
#142302=CARTESIAN_POINT('Ctrl Pts',(-67.4348125456398,-23.1952922065012,
12.));
#142303=CARTESIAN_POINT('Ctrl Pts',(-67.4574929309076,-23.195502061859,
12.));
#142304=CARTESIAN_POINT('Ctrl Pts',(-67.4802189823408,-23.195689511644,
12.));
#142305=CARTESIAN_POINT('Ctrl Pts',(-67.5029905638949,-23.1958544864215,
12.));
#142306=CARTESIAN_POINT('Ctrl Pts',(-67.5258075401146,-23.1959969171701,
12.));
#142307=CARTESIAN_POINT('Ctrl Pts',(-67.5486697761288,-23.1961167352772,
12.));
#142308=CARTESIAN_POINT('Ctrl Pts',(-67.5715771376461,-23.196213872536,
12.));
#142309=CARTESIAN_POINT('Ctrl Pts',(-67.5945294909426,-23.1962882611453,
12.));
#142310=CARTESIAN_POINT('Ctrl Pts',(-67.6175267028555,-23.1963398337069,
12.));
#142311=CARTESIAN_POINT('Ctrl Pts',(-67.6405686407863,-23.1963685232188,
12.));
#142312=CARTESIAN_POINT('Ctrl Pts',(-67.6636551726964,-23.1963742630715,
12.));
#142313=CARTESIAN_POINT('Ctrl Pts',(-67.6867861671031,-23.1963569870451,
12.));
#142314=CARTESIAN_POINT('Ctrl Pts',(-67.7099614930671,-23.1963166293102,
12.));
#142315=CARTESIAN_POINT('Ctrl Pts',(-67.7331810201883,-23.1962531244245,
12.));
#142316=CARTESIAN_POINT('Ctrl Pts',(-67.7564446186079,-23.1961664073262,
12.));
#142317=CARTESIAN_POINT('Ctrl Pts',(-67.7797521590045,-23.1960564133304,
12.));
#142318=CARTESIAN_POINT('Ctrl Pts',(-67.8031035125887,-23.1959230781269,
12.));
#142319=CARTESIAN_POINT('Ctrl Pts',(-67.8264985510917,-23.1957663377807,
12.));
#142320=CARTESIAN_POINT('Ctrl Pts',(-67.8499371467616,-23.1955861287286,
12.));
#142321=CARTESIAN_POINT('Ctrl Pts',(-67.8734191723667,-23.1953823877734,
12.));
#142322=CARTESIAN_POINT('Ctrl Pts',(-67.8969445011916,-23.1951550520802,
12.));
#142323=CARTESIAN_POINT('Ctrl Pts',(-67.9205130070324,-23.1949040591744,
12.));
#142324=CARTESIAN_POINT('Ctrl Pts',(-67.9441245641842,-23.1946293469427,
12.));
#142325=CARTESIAN_POINT('Ctrl Pts',(-67.9677790474385,-23.1943308536297,
12.));
#142326=CARTESIAN_POINT('Ctrl Pts',(-67.991476332086,-23.1940085178313,
12.));
#142327=CARTESIAN_POINT('Ctrl Pts',(-68.0152162939121,-23.1936622784919,
12.));
#142328=CARTESIAN_POINT('Ctrl Pts',(-68.0389988091933,-23.1932920749023,
12.));
#142329=CARTESIAN_POINT('Ctrl Pts',(-68.0628237546863,-23.1928978467021,
12.));
#142330=CARTESIAN_POINT('Ctrl Pts',(-68.0866910076251,-23.1924795338749,
12.));
#142331=CARTESIAN_POINT('Ctrl Pts',(-68.110600445723,-23.1920370767426,
12.));
#142332=CARTESIAN_POINT('Ctrl Pts',(-68.1345519471695,-23.1915704159623,
12.));
#142333=CARTESIAN_POINT('Ctrl Pts',(-68.1585453906257,-23.1910794925251,
12.));
#142334=CARTESIAN_POINT('Ctrl Pts',(-68.1825806552129,-23.1905642477571,
12.));
#142335=CARTESIAN_POINT('Ctrl Pts',(-68.2066576205116,-23.1900246233165,
12.));
#142336=CARTESIAN_POINT('Ctrl Pts',(-68.2307761665633,-23.1894605611871,
12.));
#142337=CARTESIAN_POINT('Ctrl Pts',(-68.2549361738681,-23.1888720036757,
12.));
#142338=CARTESIAN_POINT('Ctrl Pts',(-68.2791375233795,-23.1882588934107,
12.));
#142339=CARTESIAN_POINT('Ctrl Pts',(-68.3033800964939,-23.1876211733436,
12.));
#142340=CARTESIAN_POINT('Ctrl Pts',(-68.3276637750485,-23.1869587867459,
12.));
#142341=CARTESIAN_POINT('Ctrl Pts',(-68.3519884413246,-23.1862716772031,
12.));
#142342=CARTESIAN_POINT('Ctrl Pts',(-68.376353978044,-23.1855597886116,
12.));
#142343=CARTESIAN_POINT('Ctrl Pts',(-68.4007602683652,-23.1848230651777,
12.));
#142344=CARTESIAN_POINT('Ctrl Pts',(-68.4252071958729,-23.1840614514192,
12.));
#142345=CARTESIAN_POINT('Ctrl Pts',(-68.4496946445758,-23.183274892163,
12.));
#142346=CARTESIAN_POINT('Ctrl Pts',(-68.4742224989098,-23.1824633325385,
12.));
#142347=CARTESIAN_POINT('Ctrl Pts',(-68.4987906437356,-23.1816267179751,
12.));
#142348=CARTESIAN_POINT('Ctrl Pts',(-68.5233989643345,-23.180764994201,
12.));
#142349=CARTESIAN_POINT('Ctrl Pts',(-68.5480473463985,-23.179878107245,
12.));
#142350=CARTESIAN_POINT('Ctrl Pts',(-68.5727356760278,-23.1789660034342,
12.));
#142351=CARTESIAN_POINT('Ctrl Pts',(-68.597463839733,-23.1780286293875,
12.));
#142352=CARTESIAN_POINT('Ctrl Pts',(-68.6222317244341,-23.1770659320138,
12.));
#142353=CARTESIAN_POINT('Ctrl Pts',(-68.6470392174564,-23.1760778585092,
12.));
#142354=CARTESIAN_POINT('Ctrl Pts',(-68.6718862065216,-23.1750643563602,
12.));
#142355=CARTESIAN_POINT('Ctrl Pts',(-68.696772579744,-23.1740253733417,
12.));
#142356=CARTESIAN_POINT('Ctrl Pts',(-68.7216982256341,-23.172960857511,
12.));
#142357=CARTESIAN_POINT('Ctrl Pts',(-68.746663033096,-23.1718707572043,
12.));
#142358=CARTESIAN_POINT('Ctrl Pts',(-68.771666891425,-23.170755021036,12.));
#142359=CARTESIAN_POINT('Ctrl Pts',(-68.7967096902996,-23.1696135978997,
12.));
#142360=CARTESIAN_POINT('Ctrl Pts',(-68.8217913197752,-23.1684464369686,
12.));
#142361=CARTESIAN_POINT('Ctrl Pts',(-68.8469116702898,-23.1672534876889,
12.));
#142362=CARTESIAN_POINT('Ctrl Pts',(-68.8720706326609,-23.1660346997764,
12.));
#142363=CARTESIAN_POINT('Ctrl Pts',(-68.8972680980842,-23.164790023215,
12.));
#142364=CARTESIAN_POINT('Ctrl Pts',(-68.9225039581248,-23.1635194082581,
12.));
#142365=CARTESIAN_POINT('Ctrl Pts',(-68.9477781047106,-23.1622228054291,
12.));
#142366=CARTESIAN_POINT('Ctrl Pts',(-68.9730904301369,-23.1609001655156,
12.));
#142367=CARTESIAN_POINT('Ctrl Pts',(-68.9984408270659,-23.1595514395656,
12.));
#142368=CARTESIAN_POINT('Ctrl Pts',(-69.0238291885245,-23.1581765788869,
12.));
#142369=CARTESIAN_POINT('Ctrl Pts',(-69.0492554078992,-23.1567755350469,
12.));
#142370=CARTESIAN_POINT('Ctrl Pts',(-69.074719378928,-23.1553482598762,
12.));
#142371=CARTESIAN_POINT('Ctrl Pts',(-69.1002209957025,-23.1538947054615,
12.));
#142372=CARTESIAN_POINT('Ctrl Pts',(-69.1257601526687,-23.152414824141,
12.));
#142373=CARTESIAN_POINT('Ctrl Pts',(-69.1513367446231,-23.1509085685032,
12.));
#142374=CARTESIAN_POINT('Ctrl Pts',(-69.1769506667084,-23.1493758913859,
12.));
#142375=CARTESIAN_POINT('Ctrl Pts',(-69.2026018144028,-23.147816745879,
12.));
#142376=CARTESIAN_POINT('Ctrl Pts',(-69.2282900835235,-23.1462310853206,
12.));
#142377=CARTESIAN_POINT('Ctrl Pts',(-69.254015370231,-23.1446188632931,
12.));
#142378=CARTESIAN_POINT('Ctrl Pts',(-69.2797775710273,-23.142980033622,
12.));
#142379=CARTESIAN_POINT('Ctrl Pts',(-69.3055765827546,-23.1413145503762,
12.));
#142380=CARTESIAN_POINT('Ctrl Pts',(-69.3314123025869,-23.1396223678725,
12.));
#142381=CARTESIAN_POINT('Ctrl Pts',(-69.3572846280296,-23.1379034406718,
12.));
#142382=CARTESIAN_POINT('Ctrl Pts',(-69.3831934569182,-23.1361577235709,
12.));
#142383=CARTESIAN_POINT('Ctrl Pts',(-69.4091386874132,-23.1343851715989,
12.));
#142384=CARTESIAN_POINT('Ctrl Pts',(-69.4351202179946,-23.1325857400144,
12.));
#142385=CARTESIAN_POINT('Ctrl Pts',(-69.4611379474484,-23.1307593843061,
12.));
#142386=CARTESIAN_POINT('Ctrl Pts',(-69.4871917748654,-23.1289060601924,
12.));
#142387=CARTESIAN_POINT('Ctrl Pts',(-69.5132815996537,-23.1270257236204,
12.));
#142388=CARTESIAN_POINT('Ctrl Pts',(-69.539407321546,-23.1251183307676,
12.));
#142389=CARTESIAN_POINT('Ctrl Pts',(-69.5655688406052,-23.1231838380452,
12.));
#142390=CARTESIAN_POINT('Ctrl Pts',(-69.5917660572265,-23.1212222021051,
12.));
#142391=CARTESIAN_POINT('Ctrl Pts',(-69.6179988721365,-23.1192333798441,
12.));
#142392=CARTESIAN_POINT('Ctrl Pts',(-69.6442671863765,-23.1172173283859,
12.));
#142393=CARTESIAN_POINT('Ctrl Pts',(-69.6705709012852,-23.1151740050681,
12.));
#142394=CARTESIAN_POINT('Ctrl Pts',(-69.6969099184767,-23.1131033674301,
12.));
#142395=CARTESIAN_POINT('Ctrl Pts',(-69.7232841398197,-23.1110053732046,
12.));
#142396=CARTESIAN_POINT('Ctrl Pts',(-69.7496934674069,-23.1088799803089,
12.));
#142397=CARTESIAN_POINT('Ctrl Pts',(-69.7761378035964,-23.106727146861,
12.));
#142398=CARTESIAN_POINT('Ctrl Pts',(-69.8026170510572,-23.1045468311991,
12.));
#142399=CARTESIAN_POINT('Ctrl Pts',(-69.8291311128118,-23.1023389919051,
12.));
#142400=CARTESIAN_POINT('Ctrl Pts',(-69.8556798922693,-23.1001035878241,
12.));
#142401=CARTESIAN_POINT('Ctrl Pts',(-69.8822632932768,-23.0978405781021,
12.));
#142402=CARTESIAN_POINT('Ctrl Pts',(-69.9088812200713,-23.0955499221558,
12.));
#142403=CARTESIAN_POINT('Ctrl Pts',(-69.9355335771729,-23.0932315796068,
12.));
#142404=CARTESIAN_POINT('Ctrl Pts',(-69.9622202692873,-23.0908855102251,
12.));
#142405=CARTESIAN_POINT('Ctrl Pts',(-69.9889412012143,-23.0885116738798,
12.));
#142406=CARTESIAN_POINT('Ctrl Pts',(-70.0156962777169,-23.0861100304729,
12.));
#142407=CARTESIAN_POINT('Ctrl Pts',(-70.0424854035115,-23.0836805399374,
12.));
#142408=CARTESIAN_POINT('Ctrl Pts',(-70.0693084835373,-23.0812231623765,
12.));
#142409=CARTESIAN_POINT('Ctrl Pts',(-70.0961654231639,-23.0787378581774,
12.));
#142410=CARTESIAN_POINT('Ctrl Pts',(-70.123056128422,-23.0762245881389,
12.));
#142411=CARTESIAN_POINT('Ctrl Pts',(-70.1499805062172,-23.0736833135938,
12.));
#142412=CARTESIAN_POINT('Ctrl Pts',(-70.1769384645586,-23.071113996544,
12.));
#142413=CARTESIAN_POINT('Ctrl Pts',(-70.2039299120488,-23.0685165993691,
12.));
#142414=CARTESIAN_POINT('Ctrl Pts',(-70.2309547573815,-23.0658910845433,
12.));
#142415=CARTESIAN_POINT('Ctrl Pts',(-70.2580129087888,-23.0632374143279,
12.));
#142416=CARTESIAN_POINT('Ctrl Pts',(-70.2851042736066,-23.0605555505321,
12.));
#142417=CARTESIAN_POINT('Ctrl Pts',(-70.3122287575335,-23.0578454541104,
12.));
#142418=CARTESIAN_POINT('Ctrl Pts',(-70.3393862652297,-23.0551070854926,
12.));
#142419=CARTESIAN_POINT('Ctrl Pts',(-70.3665767016542,-23.0523404053172,
12.));
#142420=CARTESIAN_POINT('Ctrl Pts',(-70.3937999732267,-23.0495453750763,
12.));
#142421=CARTESIAN_POINT('Ctrl Pts',(-70.4210559889348,-23.0467219577291,
12.));
#142422=CARTESIAN_POINT('Ctrl Pts',(-70.4483446617614,-23.0438701185013,
12.));
#142423=CARTESIAN_POINT('Ctrl Pts',(-70.4756659090209,-23.0409898250756,
12.));
#142424=CARTESIAN_POINT('Ctrl Pts',(-70.4991133648947,-23.0384964376036,
12.));
#142425=CARTESIAN_POINT('Ctrl Pts',(-70.5171075702746,-23.0365694096173,
12.));
#142426=CARTESIAN_POINT('Ctrl Pts',(-70.5296341535556,-23.0352213647765,
12.));
#142427=CARTESIAN_POINT('Ctrl Pts',(-70.5366836381661,-23.0344606623299,
12.));
#142428=CARTESIAN_POINT('Ctrl Pts',(-70.538251407892,-23.0342913834073,
12.));
#142429=CARTESIAN_POINT('',(-66.0656156664138,-23.1372951448024,0.));
#142430=CARTESIAN_POINT('',(-66.0656156664138,-23.1372951448024,0.));
#142431=CARTESIAN_POINT('Ctrl Pts',(-70.538251407892,-23.0342913834073,
0.));
#142432=CARTESIAN_POINT('Ctrl Pts',(-70.5366836381661,-23.0344606623299,
0.));
#142433=CARTESIAN_POINT('Ctrl Pts',(-70.5296341535556,-23.0352213647765,
0.));
#142434=CARTESIAN_POINT('Ctrl Pts',(-70.5171075702746,-23.0365694096173,
0.));
#142435=CARTESIAN_POINT('Ctrl Pts',(-70.4991133648947,-23.0384964376036,
0.));
#142436=CARTESIAN_POINT('Ctrl Pts',(-70.4756659090209,-23.0409898250756,
0.));
#142437=CARTESIAN_POINT('Ctrl Pts',(-70.4483446617614,-23.0438701185013,
0.));
#142438=CARTESIAN_POINT('Ctrl Pts',(-70.4210559889348,-23.0467219577291,
0.));
#142439=CARTESIAN_POINT('Ctrl Pts',(-70.3937999732267,-23.0495453750763,
0.));
#142440=CARTESIAN_POINT('Ctrl Pts',(-70.3665767016542,-23.0523404053172,
0.));
#142441=CARTESIAN_POINT('Ctrl Pts',(-70.3393862652297,-23.0551070854926,
0.));
#142442=CARTESIAN_POINT('Ctrl Pts',(-70.3122287575335,-23.0578454541104,
0.));
#142443=CARTESIAN_POINT('Ctrl Pts',(-70.2851042736066,-23.0605555505321,
0.));
#142444=CARTESIAN_POINT('Ctrl Pts',(-70.2580129087888,-23.0632374143279,
0.));
#142445=CARTESIAN_POINT('Ctrl Pts',(-70.2309547573815,-23.0658910845433,
0.));
#142446=CARTESIAN_POINT('Ctrl Pts',(-70.2039299120488,-23.0685165993691,
0.));
#142447=CARTESIAN_POINT('Ctrl Pts',(-70.1769384645586,-23.071113996544,
0.));
#142448=CARTESIAN_POINT('Ctrl Pts',(-70.1499805062172,-23.0736833135938,
0.));
#142449=CARTESIAN_POINT('Ctrl Pts',(-70.123056128422,-23.0762245881389,
0.));
#142450=CARTESIAN_POINT('Ctrl Pts',(-70.0961654231639,-23.0787378581774,
0.));
#142451=CARTESIAN_POINT('Ctrl Pts',(-70.0693084835373,-23.0812231623765,
0.));
#142452=CARTESIAN_POINT('Ctrl Pts',(-70.0424854035115,-23.0836805399374,
0.));
#142453=CARTESIAN_POINT('Ctrl Pts',(-70.0156962777169,-23.0861100304729,
0.));
#142454=CARTESIAN_POINT('Ctrl Pts',(-69.9889412012143,-23.0885116738798,
0.));
#142455=CARTESIAN_POINT('Ctrl Pts',(-69.9622202692873,-23.0908855102251,
0.));
#142456=CARTESIAN_POINT('Ctrl Pts',(-69.9355335771729,-23.0932315796068,
0.));
#142457=CARTESIAN_POINT('Ctrl Pts',(-69.9088812200713,-23.0955499221558,
0.));
#142458=CARTESIAN_POINT('Ctrl Pts',(-69.8822632932768,-23.0978405781021,
0.));
#142459=CARTESIAN_POINT('Ctrl Pts',(-69.8556798922693,-23.1001035878241,
0.));
#142460=CARTESIAN_POINT('Ctrl Pts',(-69.8291311128118,-23.1023389919051,
0.));
#142461=CARTESIAN_POINT('Ctrl Pts',(-69.8026170510572,-23.1045468311991,
0.));
#142462=CARTESIAN_POINT('Ctrl Pts',(-69.7761378035964,-23.106727146861,
0.));
#142463=CARTESIAN_POINT('Ctrl Pts',(-69.7496934674069,-23.1088799803089,
0.));
#142464=CARTESIAN_POINT('Ctrl Pts',(-69.7232841398197,-23.1110053732046,
0.));
#142465=CARTESIAN_POINT('Ctrl Pts',(-69.6969099184767,-23.1131033674301,
0.));
#142466=CARTESIAN_POINT('Ctrl Pts',(-69.6705709012852,-23.1151740050681,
0.));
#142467=CARTESIAN_POINT('Ctrl Pts',(-69.6442671863765,-23.1172173283859,
0.));
#142468=CARTESIAN_POINT('Ctrl Pts',(-69.6179988721365,-23.1192333798441,
0.));
#142469=CARTESIAN_POINT('Ctrl Pts',(-69.5917660572265,-23.1212222021051,
0.));
#142470=CARTESIAN_POINT('Ctrl Pts',(-69.5655688406052,-23.1231838380452,
0.));
#142471=CARTESIAN_POINT('Ctrl Pts',(-69.539407321546,-23.1251183307676,
0.));
#142472=CARTESIAN_POINT('Ctrl Pts',(-69.5132815996537,-23.1270257236204,
0.));
#142473=CARTESIAN_POINT('Ctrl Pts',(-69.4871917748654,-23.1289060601924,
0.));
#142474=CARTESIAN_POINT('Ctrl Pts',(-69.4611379474484,-23.1307593843061,
0.));
#142475=CARTESIAN_POINT('Ctrl Pts',(-69.4351202179946,-23.1325857400144,
0.));
#142476=CARTESIAN_POINT('Ctrl Pts',(-69.4091386874132,-23.1343851715989,
0.));
#142477=CARTESIAN_POINT('Ctrl Pts',(-69.3831934569182,-23.1361577235709,
0.));
#142478=CARTESIAN_POINT('Ctrl Pts',(-69.3572846280296,-23.1379034406718,
0.));
#142479=CARTESIAN_POINT('Ctrl Pts',(-69.3314123025869,-23.1396223678725,
0.));
#142480=CARTESIAN_POINT('Ctrl Pts',(-69.3055765827546,-23.1413145503762,
0.));
#142481=CARTESIAN_POINT('Ctrl Pts',(-69.2797775710273,-23.142980033622,
0.));
#142482=CARTESIAN_POINT('Ctrl Pts',(-69.254015370231,-23.1446188632931,
0.));
#142483=CARTESIAN_POINT('Ctrl Pts',(-69.2282900835235,-23.1462310853206,
0.));
#142484=CARTESIAN_POINT('Ctrl Pts',(-69.2026018144028,-23.147816745879,
0.));
#142485=CARTESIAN_POINT('Ctrl Pts',(-69.1769506667084,-23.1493758913859,
0.));
#142486=CARTESIAN_POINT('Ctrl Pts',(-69.1513367446231,-23.1509085685032,
0.));
#142487=CARTESIAN_POINT('Ctrl Pts',(-69.1257601526687,-23.152414824141,
0.));
#142488=CARTESIAN_POINT('Ctrl Pts',(-69.1002209957025,-23.1538947054615,
0.));
#142489=CARTESIAN_POINT('Ctrl Pts',(-69.074719378928,-23.1553482598762,
0.));
#142490=CARTESIAN_POINT('Ctrl Pts',(-69.0492554078992,-23.1567755350469,
0.));
#142491=CARTESIAN_POINT('Ctrl Pts',(-69.0238291885245,-23.1581765788869,
0.));
#142492=CARTESIAN_POINT('Ctrl Pts',(-68.9984408270659,-23.1595514395656,
0.));
#142493=CARTESIAN_POINT('Ctrl Pts',(-68.9730904301369,-23.1609001655156,
0.));
#142494=CARTESIAN_POINT('Ctrl Pts',(-68.9477781047106,-23.1622228054291,
0.));
#142495=CARTESIAN_POINT('Ctrl Pts',(-68.9225039581248,-23.1635194082581,
0.));
#142496=CARTESIAN_POINT('Ctrl Pts',(-68.8972680980842,-23.164790023215,
0.));
#142497=CARTESIAN_POINT('Ctrl Pts',(-68.8720706326609,-23.1660346997764,
0.));
#142498=CARTESIAN_POINT('Ctrl Pts',(-68.8469116702898,-23.1672534876889,
0.));
#142499=CARTESIAN_POINT('Ctrl Pts',(-68.8217913197752,-23.1684464369686,
0.));
#142500=CARTESIAN_POINT('Ctrl Pts',(-68.7967096902996,-23.1696135978997,
0.));
#142501=CARTESIAN_POINT('Ctrl Pts',(-68.771666891425,-23.170755021036,0.));
#142502=CARTESIAN_POINT('Ctrl Pts',(-68.746663033096,-23.1718707572043,
0.));
#142503=CARTESIAN_POINT('Ctrl Pts',(-68.7216982256341,-23.172960857511,
0.));
#142504=CARTESIAN_POINT('Ctrl Pts',(-68.696772579744,-23.1740253733417,
0.));
#142505=CARTESIAN_POINT('Ctrl Pts',(-68.6718862065216,-23.1750643563602,
0.));
#142506=CARTESIAN_POINT('Ctrl Pts',(-68.6470392174564,-23.1760778585092,
0.));
#142507=CARTESIAN_POINT('Ctrl Pts',(-68.6222317244341,-23.1770659320138,
0.));
#142508=CARTESIAN_POINT('Ctrl Pts',(-68.597463839733,-23.1780286293875,
0.));
#142509=CARTESIAN_POINT('Ctrl Pts',(-68.5727356760278,-23.1789660034342,
0.));
#142510=CARTESIAN_POINT('Ctrl Pts',(-68.5480473463985,-23.179878107245,
0.));
#142511=CARTESIAN_POINT('Ctrl Pts',(-68.5233989643345,-23.180764994201,
0.));
#142512=CARTESIAN_POINT('Ctrl Pts',(-68.4987906437356,-23.1816267179751,
0.));
#142513=CARTESIAN_POINT('Ctrl Pts',(-68.4742224989098,-23.1824633325385,
0.));
#142514=CARTESIAN_POINT('Ctrl Pts',(-68.4496946445758,-23.183274892163,
0.));
#142515=CARTESIAN_POINT('Ctrl Pts',(-68.4252071958729,-23.1840614514192,
0.));
#142516=CARTESIAN_POINT('Ctrl Pts',(-68.4007602683652,-23.1848230651777,
0.));
#142517=CARTESIAN_POINT('Ctrl Pts',(-68.376353978044,-23.1855597886116,
0.));
#142518=CARTESIAN_POINT('Ctrl Pts',(-68.3519884413246,-23.1862716772031,
0.));
#142519=CARTESIAN_POINT('Ctrl Pts',(-68.3276637750485,-23.1869587867459,
0.));
#142520=CARTESIAN_POINT('Ctrl Pts',(-68.3033800964939,-23.1876211733436,
0.));
#142521=CARTESIAN_POINT('Ctrl Pts',(-68.2791375233795,-23.1882588934107,
0.));
#142522=CARTESIAN_POINT('Ctrl Pts',(-68.2549361738681,-23.1888720036757,
0.));
#142523=CARTESIAN_POINT('Ctrl Pts',(-68.2307761665633,-23.1894605611871,
0.));
#142524=CARTESIAN_POINT('Ctrl Pts',(-68.2066576205116,-23.1900246233165,
0.));
#142525=CARTESIAN_POINT('Ctrl Pts',(-68.1825806552129,-23.1905642477571,
0.));
#142526=CARTESIAN_POINT('Ctrl Pts',(-68.1585453906257,-23.1910794925251,
0.));
#142527=CARTESIAN_POINT('Ctrl Pts',(-68.1345519471695,-23.1915704159623,
0.));
#142528=CARTESIAN_POINT('Ctrl Pts',(-68.110600445723,-23.1920370767426,
0.));
#142529=CARTESIAN_POINT('Ctrl Pts',(-68.0866910076251,-23.1924795338749,
0.));
#142530=CARTESIAN_POINT('Ctrl Pts',(-68.0628237546863,-23.1928978467021,
0.));
#142531=CARTESIAN_POINT('Ctrl Pts',(-68.0389988091933,-23.1932920749023,
0.));
#142532=CARTESIAN_POINT('Ctrl Pts',(-68.0152162939121,-23.1936622784919,
0.));
#142533=CARTESIAN_POINT('Ctrl Pts',(-67.991476332086,-23.1940085178313,
0.));
#142534=CARTESIAN_POINT('Ctrl Pts',(-67.9677790474385,-23.1943308536297,
0.));
#142535=CARTESIAN_POINT('Ctrl Pts',(-67.9441245641842,-23.1946293469427,
0.));
#142536=CARTESIAN_POINT('Ctrl Pts',(-67.9205130070324,-23.1949040591744,
0.));
#142537=CARTESIAN_POINT('Ctrl Pts',(-67.8969445011916,-23.1951550520802,
0.));
#142538=CARTESIAN_POINT('Ctrl Pts',(-67.8734191723667,-23.1953823877734,
0.));
#142539=CARTESIAN_POINT('Ctrl Pts',(-67.8499371467616,-23.1955861287286,
0.));
#142540=CARTESIAN_POINT('Ctrl Pts',(-67.8264985510917,-23.1957663377807,
0.));
#142541=CARTESIAN_POINT('Ctrl Pts',(-67.8031035125887,-23.1959230781269,
0.));
#142542=CARTESIAN_POINT('Ctrl Pts',(-67.7797521590045,-23.1960564133304,
0.));
#142543=CARTESIAN_POINT('Ctrl Pts',(-67.7564446186079,-23.1961664073262,
0.));
#142544=CARTESIAN_POINT('Ctrl Pts',(-67.7331810201883,-23.1962531244245,
0.));
#142545=CARTESIAN_POINT('Ctrl Pts',(-67.7099614930671,-23.1963166293102,
0.));
#142546=CARTESIAN_POINT('Ctrl Pts',(-67.6867861671031,-23.1963569870451,
0.));
#142547=CARTESIAN_POINT('Ctrl Pts',(-67.6636551726964,-23.1963742630715,
0.));
#142548=CARTESIAN_POINT('Ctrl Pts',(-67.6405686407863,-23.1963685232188,
0.));
#142549=CARTESIAN_POINT('Ctrl Pts',(-67.6175267028555,-23.1963398337069,
0.));
#142550=CARTESIAN_POINT('Ctrl Pts',(-67.5945294909426,-23.1962882611453,
0.));
#142551=CARTESIAN_POINT('Ctrl Pts',(-67.5715771376461,-23.196213872536,
0.));
#142552=CARTESIAN_POINT('Ctrl Pts',(-67.5486697761288,-23.1961167352772,
0.));
#142553=CARTESIAN_POINT('Ctrl Pts',(-67.5258075401146,-23.1959969171701,
0.));
#142554=CARTESIAN_POINT('Ctrl Pts',(-67.5029905638949,-23.1958544864215,
0.));
#142555=CARTESIAN_POINT('Ctrl Pts',(-67.4802189823408,-23.195689511644,
0.));
#142556=CARTESIAN_POINT('Ctrl Pts',(-67.4574929309076,-23.195502061859,
0.));
#142557=CARTESIAN_POINT('Ctrl Pts',(-67.4348125456398,-23.1952922065012,
0.));
#142558=CARTESIAN_POINT('Ctrl Pts',(-67.412177963168,-23.1950600154265,
0.));
#142559=CARTESIAN_POINT('Ctrl Pts',(-67.3895893207182,-23.1948055589129,
0.));
#142560=CARTESIAN_POINT('Ctrl Pts',(-67.3670467561212,-23.194528907661,
0.));
#142561=CARTESIAN_POINT('Ctrl Pts',(-67.3445504078176,-23.1942301327978,
0.));
#142562=CARTESIAN_POINT('Ctrl Pts',(-67.3221004148603,-23.1939093058801,
0.));
#142563=CARTESIAN_POINT('Ctrl Pts',(-67.2996969169098,-23.1935664989018,
0.));
#142564=CARTESIAN_POINT('Ctrl Pts',(-67.2773400542477,-23.1932017842953,
0.));
#142565=CARTESIAN_POINT('Ctrl Pts',(-67.2550299677888,-23.1928152349343,
0.));
#142566=CARTESIAN_POINT('Ctrl Pts',(-67.232766799088,-23.1924069241385,
0.));
#142567=CARTESIAN_POINT('Ctrl Pts',(-67.2105506903447,-23.1919769256803,
0.));
#142568=CARTESIAN_POINT('Ctrl Pts',(-67.1883817844038,-23.1915253137924,
0.));
#142569=CARTESIAN_POINT('Ctrl Pts',(-67.1662602247639,-23.1910521631657,
0.));
#142570=CARTESIAN_POINT('Ctrl Pts',(-67.1441861555817,-23.1905575489505,
0.));
#142571=CARTESIAN_POINT('Ctrl Pts',(-67.1221597216741,-23.1900415467574,
0.));
#142572=CARTESIAN_POINT('Ctrl Pts',(-67.1001810685143,-23.1895042326627,
0.));
#142573=CARTESIAN_POINT('Ctrl Pts',(-67.0782503422305,-23.1889456832119,
0.));
#142574=CARTESIAN_POINT('Ctrl Pts',(-67.0563676896325,-23.1883659754271,
0.));
#142575=CARTESIAN_POINT('Ctrl Pts',(-67.0345332582306,-23.1877651868158,
0.));
#142576=CARTESIAN_POINT('Ctrl Pts',(-67.0127471962501,-23.1871433953793,
0.));
#142577=CARTESIAN_POINT('Ctrl Pts',(-66.9910096526462,-23.1865006796284,
0.));
#142578=CARTESIAN_POINT('Ctrl Pts',(-66.9693207771031,-23.1858371185842,
0.));
#142579=CARTESIAN_POINT('Ctrl Pts',(-66.9476807200203,-23.1851527917657,
0.));
#142580=CARTESIAN_POINT('Ctrl Pts',(-66.9260896324949,-23.1844477791814,
0.));
#142581=CARTESIAN_POINT('Ctrl Pts',(-66.9045476663063,-23.1837221613235,
0.));
#142582=CARTESIAN_POINT('Ctrl Pts',(-66.8830549738795,-23.1829760191591,
0.));
#142583=CARTESIAN_POINT('Ctrl Pts',(-66.8616117083331,-23.1822094341517,
0.));
#142584=CARTESIAN_POINT('Ctrl Pts',(-66.8402180235566,-23.1814224882954,
0.));
#142585=CARTESIAN_POINT('Ctrl Pts',(-66.8188740742727,-23.1806152641475,
0.));
#142586=CARTESIAN_POINT('Ctrl Pts',(-66.7975800161,-23.1797878448639,0.));
#142587=CARTESIAN_POINT('Ctrl Pts',(-66.776336005612,-23.1789403142366,
0.));
#142588=CARTESIAN_POINT('Ctrl Pts',(-66.7551422002204,-23.17807275663,0.));
#142589=CARTESIAN_POINT('Ctrl Pts',(-66.7339987580427,-23.1771852569131,
0.));
#142590=CARTESIAN_POINT('Ctrl Pts',(-66.7129058377896,-23.1762779004044,
0.));
#142591=CARTESIAN_POINT('Ctrl Pts',(-66.6918635985972,-23.1753507727939,
0.));
#142592=CARTESIAN_POINT('Ctrl Pts',(-66.6708722000079,-23.1744039601382,
0.));
#142593=CARTESIAN_POINT('Ctrl Pts',(-66.6499318023473,-23.1734375490431,
0.));
#142594=CARTESIAN_POINT('Ctrl Pts',(-66.6290425670548,-23.1724516268302,
0.));
#142595=CARTESIAN_POINT('Ctrl Pts',(-66.6082046569644,-23.1714462816789,
0.));
#142596=CARTESIAN_POINT('Ctrl Pts',(-66.5874182367563,-23.1704216028614,
0.));
#142597=CARTESIAN_POINT('Ctrl Pts',(-66.5666834726454,-23.1693776805866,
0.));
#142598=CARTESIAN_POINT('Ctrl Pts',(-66.5460005315376,-23.1683146055726,
0.));
#142599=CARTESIAN_POINT('Ctrl Pts',(-66.5253695803205,-23.1672324686926,
0.));
#142600=CARTESIAN_POINT('Ctrl Pts',(-66.5047907851348,-23.1661313606132,
0.));
#142601=CARTESIAN_POINT('Ctrl Pts',(-66.4842643105311,-23.1650113713808,
0.));
#142602=CARTESIAN_POINT('Ctrl Pts',(-66.4637903210727,-23.1638725912195,
0.));
#142603=CARTESIAN_POINT('Ctrl Pts',(-66.4433689832478,-23.1627151114883,
0.));
#142604=CARTESIAN_POINT('Ctrl Pts',(-66.4230004670278,-23.1615390254632,
0.));
#142605=CARTESIAN_POINT('Ctrl Pts',(-66.4026849481232,-23.160344429474,
0.));
#142606=CARTESIAN_POINT('Ctrl Pts',(-66.3824226081801,-23.1591314230083,
0.));
#142607=CARTESIAN_POINT('Ctrl Pts',(-66.3622136300654,-23.1579001063424,
0.));
#142608=CARTESIAN_POINT('Ctrl Pts',(-66.3420581937147,-23.1566505784621,
0.));
#142609=CARTESIAN_POINT('Ctrl Pts',(-66.3219564725184,-23.1553829352539,
0.));
#142610=CARTESIAN_POINT('Ctrl Pts',(-66.3019086275444,-23.1540972666191,
0.));
#142611=CARTESIAN_POINT('Ctrl Pts',(-66.281914813114,-23.1527936592651,
0.));
#142612=CARTESIAN_POINT('Ctrl Pts',(-66.2619751878793,-23.1514722022503,
0.));
#142613=CARTESIAN_POINT('Ctrl Pts',(-66.2420899237318,-23.1501329914488,
0.));
#142614=CARTESIAN_POINT('Ctrl Pts',(-66.2222592165398,-23.1487761349298,
0.));
#142615=CARTESIAN_POINT('Ctrl Pts',(-66.2024832934733,-23.147401756643,
0.));
#142616=CARTESIAN_POINT('Ctrl Pts',(-66.1827623902755,-23.1460099850704,
0.));
#142617=CARTESIAN_POINT('Ctrl Pts',(-66.163096729667,-23.1446009424872,
0.));
#142618=CARTESIAN_POINT('Ctrl Pts',(-66.14348650151,-23.1431747350127,0.));
#142619=CARTESIAN_POINT('Ctrl Pts',(-66.1239318368803,-23.1417314398501,
0.));
#142620=CARTESIAN_POINT('Ctrl Pts',(-66.1044328067739,-23.140271103958,
0.));
#142621=CARTESIAN_POINT('Ctrl Pts',(-66.0888781152779,-23.1390892229923,
0.));
#142622=CARTESIAN_POINT('Ctrl Pts',(-66.0772371487475,-23.1381951597491,
0.));
#142623=CARTESIAN_POINT('Ctrl Pts',(-66.0694876382212,-23.1375957166138,
0.));
#142624=CARTESIAN_POINT('Ctrl Pts',(-66.0656156664138,-23.1372951448024,
0.));
#142625=CARTESIAN_POINT('Ctrl Pts',(-72.5962692526112,-16.7341474417544,
0.));
#142626=CARTESIAN_POINT('Ctrl Pts',(-72.5962692526112,-16.7341474417544,
12.));
#142627=CARTESIAN_POINT('Ctrl Pts',(-72.5907910746008,-16.7352885767485,
0.));
#142628=CARTESIAN_POINT('Ctrl Pts',(-72.5907910746008,-16.7352885767485,
12.));
#142629=CARTESIAN_POINT('Ctrl Pts',(-72.5798376087774,-16.7375676985344,
0.));
#142630=CARTESIAN_POINT('Ctrl Pts',(-72.5798376087774,-16.7375676985344,
12.));
#142631=CARTESIAN_POINT('Ctrl Pts',(-72.5634160806351,-16.7409769366072,
0.));
#142632=CARTESIAN_POINT('Ctrl Pts',(-72.5634160806351,-16.7409769366072,
12.));
#142633=CARTESIAN_POINT('Ctrl Pts',(-72.5415380516636,-16.7455036973866,
0.));
#142634=CARTESIAN_POINT('Ctrl Pts',(-72.5415380516636,-16.7455036973866,
12.));
#142635=CARTESIAN_POINT('Ctrl Pts',(-72.514219427383,-16.7511306618915,
0.));
#142636=CARTESIAN_POINT('Ctrl Pts',(-72.514219427383,-16.7511306618915,
12.));
#142637=CARTESIAN_POINT('Ctrl Pts',(-72.4869297342427,-16.7567261380687,
0.));
#142638=CARTESIAN_POINT('Ctrl Pts',(-72.4869297342427,-16.7567261380687,
12.));
#142639=CARTESIAN_POINT('Ctrl Pts',(-72.4596690055437,-16.7622901280758,
0.));
#142640=CARTESIAN_POINT('Ctrl Pts',(-72.4596690055437,-16.7622901280758,
12.));
#142641=CARTESIAN_POINT('Ctrl Pts',(-72.4324372916746,-16.7678226404162,
0.));
#142642=CARTESIAN_POINT('Ctrl Pts',(-72.4324372916746,-16.7678226404162,
12.));
#142643=CARTESIAN_POINT('Ctrl Pts',(-72.4052346647799,-16.7733236932135,
0.));
#142644=CARTESIAN_POINT('Ctrl Pts',(-72.4052346647799,-16.7733236932135,
12.));
#142645=CARTESIAN_POINT('Ctrl Pts',(-72.3780612167786,-16.7787933137498,
0.));
#142646=CARTESIAN_POINT('Ctrl Pts',(-72.3780612167786,-16.7787933137498,
12.));
#142647=CARTESIAN_POINT('Ctrl Pts',(-72.3509170522838,-16.7842315351362,
0.));
#142648=CARTESIAN_POINT('Ctrl Pts',(-72.3509170522838,-16.7842315351362,
12.));
#142649=CARTESIAN_POINT('Ctrl Pts',(-72.3238022829223,-16.7896383937822,
0.));
#142650=CARTESIAN_POINT('Ctrl Pts',(-72.3238022829223,-16.7896383937822,
12.));
#142651=CARTESIAN_POINT('Ctrl Pts',(-72.2967170212353,-16.7950139266121,
0.));
#142652=CARTESIAN_POINT('Ctrl Pts',(-72.2967170212353,-16.7950139266121,
12.));
#142653=CARTESIAN_POINT('Ctrl Pts',(-72.2696613743782,-16.8003581682248,
0.));
#142654=CARTESIAN_POINT('Ctrl Pts',(-72.2696613743782,-16.8003581682248,
12.));
#142655=CARTESIAN_POINT('Ctrl Pts',(-72.2426354390213,-16.8056711485821,
0.));
#142656=CARTESIAN_POINT('Ctrl Pts',(-72.2426354390213,-16.8056711485821,
12.));
#142657=CARTESIAN_POINT('Ctrl Pts',(-72.2156393048975,-16.8109528945896,
0.));
#142658=CARTESIAN_POINT('Ctrl Pts',(-72.2156393048975,-16.8109528945896,
12.));
#142659=CARTESIAN_POINT('Ctrl Pts',(-72.1886730573452,-16.8162034312269,
0.));
#142660=CARTESIAN_POINT('Ctrl Pts',(-72.1886730573452,-16.8162034312269,
12.));
#142661=CARTESIAN_POINT('Ctrl Pts',(-72.1617367803235,-16.8214227828942,
0.));
#142662=CARTESIAN_POINT('Ctrl Pts',(-72.1617367803235,-16.8214227828942,
12.));
#142663=CARTESIAN_POINT('Ctrl Pts',(-72.13483055902,-16.8266109745795,0.));
#142664=CARTESIAN_POINT('Ctrl Pts',(-72.13483055902,-16.8266109745795,12.));
#142665=CARTESIAN_POINT('Ctrl Pts',(-72.1079544831513,-16.8317680333404,
0.));
#142666=CARTESIAN_POINT('Ctrl Pts',(-72.1079544831513,-16.8317680333404,
12.));
#142667=CARTESIAN_POINT('Ctrl Pts',(-72.0811086466121,-16.8368939881446,
0.));
#142668=CARTESIAN_POINT('Ctrl Pts',(-72.0811086466121,-16.8368939881446,
12.));
#142669=CARTESIAN_POINT('Ctrl Pts',(-72.0542931459825,-16.8419888691976,
0.));
#142670=CARTESIAN_POINT('Ctrl Pts',(-72.0542931459825,-16.8419888691976,
12.));
#142671=CARTESIAN_POINT('Ctrl Pts',(-72.0275080793727,-16.8470527074275,
0.));
#142672=CARTESIAN_POINT('Ctrl Pts',(-72.0275080793727,-16.8470527074275,
12.));
#142673=CARTESIAN_POINT('Ctrl Pts',(-72.0007535452081,-16.8520855339446,
0.));
#142674=CARTESIAN_POINT('Ctrl Pts',(-72.0007535452081,-16.8520855339446,
12.));
#142675=CARTESIAN_POINT('Ctrl Pts',(-71.9740296408347,-16.8570873794269,
0.));
#142676=CARTESIAN_POINT('Ctrl Pts',(-71.9740296408347,-16.8570873794269,
12.));
#142677=CARTESIAN_POINT('Ctrl Pts',(-71.9473364618922,-16.8620582738437,
0.));
#142678=CARTESIAN_POINT('Ctrl Pts',(-71.9473364618922,-16.8620582738437,
12.));
#142679=CARTESIAN_POINT('Ctrl Pts',(-71.9206741030887,-16.866998246792,
0.));
#142680=CARTESIAN_POINT('Ctrl Pts',(-71.9206741030887,-16.866998246792,
12.));
#142681=CARTESIAN_POINT('Ctrl Pts',(-71.8940426586534,-16.871907327697,
0.));
#142682=CARTESIAN_POINT('Ctrl Pts',(-71.8940426586534,-16.871907327697,
12.));
#142683=CARTESIAN_POINT('Ctrl Pts',(-71.8674422229149,-16.87678554607,0.));
#142684=CARTESIAN_POINT('Ctrl Pts',(-71.8674422229149,-16.87678554607,12.));
#142685=CARTESIAN_POINT('Ctrl Pts',(-71.8408728908258,-16.881632931747,
0.));
#142686=CARTESIAN_POINT('Ctrl Pts',(-71.8408728908258,-16.881632931747,
12.));
#142687=CARTESIAN_POINT('Ctrl Pts',(-71.8143347584962,-16.8864495151344,
0.));
#142688=CARTESIAN_POINT('Ctrl Pts',(-71.8143347584962,-16.8864495151344,
12.));
#142689=CARTESIAN_POINT('Ctrl Pts',(-71.7878279229546,-16.8912353270942,
0.));
#142690=CARTESIAN_POINT('Ctrl Pts',(-71.7878279229546,-16.8912353270942,
12.));
#142691=CARTESIAN_POINT('Ctrl Pts',(-71.7613524819235,-16.8959903988409,
0.));
#142692=CARTESIAN_POINT('Ctrl Pts',(-71.7613524819235,-16.8959903988409,
12.));
#142693=CARTESIAN_POINT('Ctrl Pts',(-71.7349085335796,-16.9007147618344,
0.));
#142694=CARTESIAN_POINT('Ctrl Pts',(-71.7349085335796,-16.9007147618344,
12.));
#142695=CARTESIAN_POINT('Ctrl Pts',(-71.7084961763357,-16.9054084476847,
0.));
#142696=CARTESIAN_POINT('Ctrl Pts',(-71.7084961763357,-16.9054084476847,
12.));
#142697=CARTESIAN_POINT('Ctrl Pts',(-71.6821155085612,-16.9100714880368,
0.));
#142698=CARTESIAN_POINT('Ctrl Pts',(-71.6821155085612,-16.9100714880368,
12.));
#142699=CARTESIAN_POINT('Ctrl Pts',(-71.6557666285917,-16.9147039145717,
0.));
#142700=CARTESIAN_POINT('Ctrl Pts',(-71.6557666285917,-16.9147039145717,
12.));
#142701=CARTESIAN_POINT('Ctrl Pts',(-71.6294496348652,-16.9193057590607,
0.));
#142702=CARTESIAN_POINT('Ctrl Pts',(-71.6294496348652,-16.9193057590607,
12.));
#142703=CARTESIAN_POINT('Ctrl Pts',(-71.6031646260174,-16.9238770534071,
0.));
#142704=CARTESIAN_POINT('Ctrl Pts',(-71.6031646260174,-16.9238770534071,
12.));
#142705=CARTESIAN_POINT('Ctrl Pts',(-71.5769117009842,-16.9284178296933,
0.));
#142706=CARTESIAN_POINT('Ctrl Pts',(-71.5769117009842,-16.9284178296933,
12.));
#142707=CARTESIAN_POINT('Ctrl Pts',(-71.5506909591128,-16.9329281202377,
0.));
#142708=CARTESIAN_POINT('Ctrl Pts',(-71.5506909591128,-16.9329281202377,
12.));
#142709=CARTESIAN_POINT('Ctrl Pts',(-71.5245025002139,-16.9374079576201,
0.));
#142710=CARTESIAN_POINT('Ctrl Pts',(-71.5245025002139,-16.9374079576201,
12.));
#142711=CARTESIAN_POINT('Ctrl Pts',(-71.4983464245055,-16.9418573746488,
0.));
#142712=CARTESIAN_POINT('Ctrl Pts',(-71.4983464245055,-16.9418573746488,
12.));
#142713=CARTESIAN_POINT('Ctrl Pts',(-71.4722228325794,-16.9462764043443,
0.));
#142714=CARTESIAN_POINT('Ctrl Pts',(-71.4722228325794,-16.9462764043443,
12.));
#142715=CARTESIAN_POINT('Ctrl Pts',(-71.4461318253563,-16.9506650799189,
0.));
#142716=CARTESIAN_POINT('Ctrl Pts',(-71.4461318253563,-16.9506650799189,
12.));
#142717=CARTESIAN_POINT('Ctrl Pts',(-71.4200735040384,-16.955023434762,
0.));
#142718=CARTESIAN_POINT('Ctrl Pts',(-71.4200735040384,-16.955023434762,
12.));
#142719=CARTESIAN_POINT('Ctrl Pts',(-71.3940479700677,-16.9593515024276,
0.));
#142720=CARTESIAN_POINT('Ctrl Pts',(-71.3940479700677,-16.9593515024276,
12.));
#142721=CARTESIAN_POINT('Ctrl Pts',(-71.3680553251562,-16.9636493166397,
0.));
#142722=CARTESIAN_POINT('Ctrl Pts',(-71.3680553251562,-16.9636493166397,
12.));
#142723=CARTESIAN_POINT('Ctrl Pts',(-71.3420956713082,-16.9679169112994,
0.));
#142724=CARTESIAN_POINT('Ctrl Pts',(-71.3420956713082,-16.9679169112994,
12.));
#142725=CARTESIAN_POINT('Ctrl Pts',(-71.3161691108427,-16.9721543204951,
0.));
#142726=CARTESIAN_POINT('Ctrl Pts',(-71.3161691108427,-16.9721543204951,
12.));
#142727=CARTESIAN_POINT('Ctrl Pts',(-71.290275746412,-16.9763615785136,
0.));
#142728=CARTESIAN_POINT('Ctrl Pts',(-71.290275746412,-16.9763615785136,
12.));
#142729=CARTESIAN_POINT('Ctrl Pts',(-71.2644156810198,-16.9805387198571,
0.));
#142730=CARTESIAN_POINT('Ctrl Pts',(-71.2644156810198,-16.9805387198571,
12.));
#142731=CARTESIAN_POINT('Ctrl Pts',(-71.2385890180221,-16.9846857792383,
0.));
#142732=CARTESIAN_POINT('Ctrl Pts',(-71.2385890180221,-16.9846857792383,
12.));
#142733=CARTESIAN_POINT('Ctrl Pts',(-71.212795861124,-16.9888027915742,
0.));
#142734=CARTESIAN_POINT('Ctrl Pts',(-71.212795861124,-16.9888027915742,
12.));
#142735=CARTESIAN_POINT('Ctrl Pts',(-71.187036314374,-16.9928897919828,
0.));
#142736=CARTESIAN_POINT('Ctrl Pts',(-71.187036314374,-16.9928897919828,
12.));
#142737=CARTESIAN_POINT('Ctrl Pts',(-71.1613104821568,-16.9969468157824,
0.));
#142738=CARTESIAN_POINT('Ctrl Pts',(-71.1613104821568,-16.9969468157824,
12.));
#142739=CARTESIAN_POINT('Ctrl Pts',(-71.1356184691806,-17.0009738984935,
0.));
#142740=CARTESIAN_POINT('Ctrl Pts',(-71.1356184691806,-17.0009738984935,
12.));
#142741=CARTESIAN_POINT('Ctrl Pts',(-71.1099603804786,-17.0049710758393,
0.));
#142742=CARTESIAN_POINT('Ctrl Pts',(-71.1099603804786,-17.0049710758393,
12.));
#142743=CARTESIAN_POINT('Ctrl Pts',(-71.0843363214221,-17.0089383837437,
0.));
#142744=CARTESIAN_POINT('Ctrl Pts',(-71.0843363214221,-17.0089383837437,
12.));
#142745=CARTESIAN_POINT('Ctrl Pts',(-71.0587463977268,-17.0128758583334,
0.));
#142746=CARTESIAN_POINT('Ctrl Pts',(-71.0587463977268,-17.0128758583334,
12.));
#142747=CARTESIAN_POINT('Ctrl Pts',(-71.0331907154574,-17.0167835359419,
0.));
#142748=CARTESIAN_POINT('Ctrl Pts',(-71.0331907154574,-17.0167835359419,
12.));
#142749=CARTESIAN_POINT('Ctrl Pts',(-71.0076693810301,-17.0206614531166,
0.));
#142750=CARTESIAN_POINT('Ctrl Pts',(-71.0076693810301,-17.0206614531166,
12.));
#142751=CARTESIAN_POINT('Ctrl Pts',(-70.9821825012136,-17.0245096466229,
0.));
#142752=CARTESIAN_POINT('Ctrl Pts',(-70.9821825012136,-17.0245096466229,
12.));
#142753=CARTESIAN_POINT('Ctrl Pts',(-70.956730183136,-17.0283281534392,
0.));
#142754=CARTESIAN_POINT('Ctrl Pts',(-70.956730183136,-17.0283281534392,
12.));
#142755=CARTESIAN_POINT('Ctrl Pts',(-70.9313125342876,-17.0321170107564,
0.));
#142756=CARTESIAN_POINT('Ctrl Pts',(-70.9313125342876,-17.0321170107564,
12.));
#142757=CARTESIAN_POINT('Ctrl Pts',(-70.9059296625214,-17.0358762559786,
0.));
#142758=CARTESIAN_POINT('Ctrl Pts',(-70.9059296625214,-17.0358762559786,
12.));
#142759=CARTESIAN_POINT('Ctrl Pts',(-70.8805816760501,-17.0396059267277,
0.));
#142760=CARTESIAN_POINT('Ctrl Pts',(-70.8805816760501,-17.0396059267277,
12.));
#142761=CARTESIAN_POINT('Ctrl Pts',(-70.8552686834423,-17.0433060608474,
0.));
#142762=CARTESIAN_POINT('Ctrl Pts',(-70.8552686834423,-17.0433060608474,
12.));
#142763=CARTESIAN_POINT('Ctrl Pts',(-70.8299907936334,-17.0469766964001,
0.));
#142764=CARTESIAN_POINT('Ctrl Pts',(-70.8299907936334,-17.0469766964001,
12.));
#142765=CARTESIAN_POINT('Ctrl Pts',(-70.8047481159298,-17.0506178716661,
0.));
#142766=CARTESIAN_POINT('Ctrl Pts',(-70.8047481159298,-17.0506178716661,
12.));
#142767=CARTESIAN_POINT('Ctrl Pts',(-70.7795407600127,-17.0542296251462,
0.));
#142768=CARTESIAN_POINT('Ctrl Pts',(-70.7795407600127,-17.0542296251462,
12.));
#142769=CARTESIAN_POINT('Ctrl Pts',(-70.754368835938,-17.0578119955651,
0.));
#142770=CARTESIAN_POINT('Ctrl Pts',(-70.754368835938,-17.0578119955651,
12.));
#142771=CARTESIAN_POINT('Ctrl Pts',(-70.7292324541348,-17.0613650218788,
0.));
#142772=CARTESIAN_POINT('Ctrl Pts',(-70.7292324541348,-17.0613650218788,
12.));
#142773=CARTESIAN_POINT('Ctrl Pts',(-70.7041317254127,-17.0648887432714,
0.));
#142774=CARTESIAN_POINT('Ctrl Pts',(-70.7041317254127,-17.0648887432714,
12.));
#142775=CARTESIAN_POINT('Ctrl Pts',(-70.6790667609678,-17.0683831991532,
0.));
#142776=CARTESIAN_POINT('Ctrl Pts',(-70.6790667609678,-17.0683831991532,
12.));
#142777=CARTESIAN_POINT('Ctrl Pts',(-70.6540376723839,-17.0718484291623,
0.));
#142778=CARTESIAN_POINT('Ctrl Pts',(-70.6540376723839,-17.0718484291623,
12.));
#142779=CARTESIAN_POINT('Ctrl Pts',(-70.6290445716341,-17.0752844731679,
0.));
#142780=CARTESIAN_POINT('Ctrl Pts',(-70.6290445716341,-17.0752844731679,
12.));
#142781=CARTESIAN_POINT('Ctrl Pts',(-70.6040875710762,-17.0786913712766,
0.));
#142782=CARTESIAN_POINT('Ctrl Pts',(-70.6040875710762,-17.0786913712766,
12.));
#142783=CARTESIAN_POINT('Ctrl Pts',(-70.5791667834599,-17.0820691638314,
0.));
#142784=CARTESIAN_POINT('Ctrl Pts',(-70.5791667834599,-17.0820691638314,
12.));
#142785=CARTESIAN_POINT('Ctrl Pts',(-70.5542823219346,-17.085417891409,
0.));
#142786=CARTESIAN_POINT('Ctrl Pts',(-70.5542823219346,-17.085417891409,
12.));
#142787=CARTESIAN_POINT('Ctrl Pts',(-70.5294343000516,-17.0887375948221,
0.));
#142788=CARTESIAN_POINT('Ctrl Pts',(-70.5294343000516,-17.0887375948221,
12.));
#142789=CARTESIAN_POINT('Ctrl Pts',(-70.5046228317669,-17.0920283151217,
0.));
#142790=CARTESIAN_POINT('Ctrl Pts',(-70.5046228317669,-17.0920283151217,
12.));
#142791=CARTESIAN_POINT('Ctrl Pts',(-70.4798480314364,-17.0952900936044,
0.));
#142792=CARTESIAN_POINT('Ctrl Pts',(-70.4798480314364,-17.0952900936044,
12.));
#142793=CARTESIAN_POINT('Ctrl Pts',(-70.4551100138221,-17.098522971812,
0.));
#142794=CARTESIAN_POINT('Ctrl Pts',(-70.4551100138221,-17.098522971812,
12.));
#142795=CARTESIAN_POINT('Ctrl Pts',(-70.4304088940998,-17.1017269915289,
0.));
#142796=CARTESIAN_POINT('Ctrl Pts',(-70.4304088940998,-17.1017269915289,
12.));
#142797=CARTESIAN_POINT('Ctrl Pts',(-70.4057447878621,-17.1049021947833,
0.));
#142798=CARTESIAN_POINT('Ctrl Pts',(-70.4057447878621,-17.1049021947833,
12.));
#142799=CARTESIAN_POINT('Ctrl Pts',(-70.3811178111206,-17.1080486238499,
0.));
#142800=CARTESIAN_POINT('Ctrl Pts',(-70.3811178111206,-17.1080486238499,
12.));
#142801=CARTESIAN_POINT('Ctrl Pts',(-70.356528080303,-17.111166321257,0.));
#142802=CARTESIAN_POINT('Ctrl Pts',(-70.356528080303,-17.111166321257,12.));
#142803=CARTESIAN_POINT('Ctrl Pts',(-70.3319757122576,-17.1142553297869,
0.));
#142804=CARTESIAN_POINT('Ctrl Pts',(-70.3319757122576,-17.1142553297869,
12.));
#142805=CARTESIAN_POINT('Ctrl Pts',(-70.3074608242613,-17.1173156924733,
0.));
#142806=CARTESIAN_POINT('Ctrl Pts',(-70.3074608242613,-17.1173156924733,
12.));
#142807=CARTESIAN_POINT('Ctrl Pts',(-70.2829835340239,-17.1203474526031,
0.));
#142808=CARTESIAN_POINT('Ctrl Pts',(-70.2829835340239,-17.1203474526031,
12.));
#142809=CARTESIAN_POINT('Ctrl Pts',(-70.2585439596899,-17.1233506537176,
0.));
#142810=CARTESIAN_POINT('Ctrl Pts',(-70.2585439596899,-17.1233506537176,
12.));
#142811=CARTESIAN_POINT('Ctrl Pts',(-70.2341422198362,-17.1263253396202,
0.));
#142812=CARTESIAN_POINT('Ctrl Pts',(-70.2341422198362,-17.1263253396202,
12.));
#142813=CARTESIAN_POINT('Ctrl Pts',(-70.2097784334749,-17.1292715543779,
0.));
#142814=CARTESIAN_POINT('Ctrl Pts',(-70.2097784334749,-17.1292715543779,
12.));
#142815=CARTESIAN_POINT('Ctrl Pts',(-70.1854527200636,-17.1321893423183,
0.));
#142816=CARTESIAN_POINT('Ctrl Pts',(-70.1854527200636,-17.1321893423183,
12.));
#142817=CARTESIAN_POINT('Ctrl Pts',(-70.1611651995085,-17.1350787480313,
0.));
#142818=CARTESIAN_POINT('Ctrl Pts',(-70.1611651995085,-17.1350787480313,
12.));
#142819=CARTESIAN_POINT('Ctrl Pts',(-70.1369159921686,-17.1379398163708,
0.));
#142820=CARTESIAN_POINT('Ctrl Pts',(-70.1369159921686,-17.1379398163708,
12.));
#142821=CARTESIAN_POINT('Ctrl Pts',(-70.1127052188515,-17.1407725924615,
0.));
#142822=CARTESIAN_POINT('Ctrl Pts',(-70.1127052188515,-17.1407725924615,
12.));
#142823=CARTESIAN_POINT('Ctrl Pts',(-70.0885330008169,-17.1435771217015,
0.));
#142824=CARTESIAN_POINT('Ctrl Pts',(-70.0885330008169,-17.1435771217015,
12.));
#142825=CARTESIAN_POINT('Ctrl Pts',(-70.0643994597865,-17.1463534497592,
0.));
#142826=CARTESIAN_POINT('Ctrl Pts',(-70.0643994597865,-17.1463534497592,
12.));
#142827=CARTESIAN_POINT('Ctrl Pts',(-70.040304717948,-17.1491016225748,
0.));
#142828=CARTESIAN_POINT('Ctrl Pts',(-70.040304717948,-17.1491016225748,
12.));
#142829=CARTESIAN_POINT('Ctrl Pts',(-70.0162488979586,-17.1518216863624,
0.));
#142830=CARTESIAN_POINT('Ctrl Pts',(-70.0162488979586,-17.1518216863624,
12.));
#142831=CARTESIAN_POINT('Ctrl Pts',(-69.9922321229428,-17.1545136876161,
0.));
#142832=CARTESIAN_POINT('Ctrl Pts',(-69.9922321229428,-17.1545136876161,
12.));
#142833=CARTESIAN_POINT('Ctrl Pts',(-69.9682545164942,-17.157177673114,
0.));
#142834=CARTESIAN_POINT('Ctrl Pts',(-69.9682545164942,-17.157177673114,
12.));
#142835=CARTESIAN_POINT('Ctrl Pts',(-69.9443162026865,-17.1598136899144,
0.));
#142836=CARTESIAN_POINT('Ctrl Pts',(-69.9443162026865,-17.1598136899144,
12.));
#142837=CARTESIAN_POINT('Ctrl Pts',(-69.9204173060779,-17.1624217853577,
0.));
#142838=CARTESIAN_POINT('Ctrl Pts',(-69.9204173060779,-17.1624217853577,
12.));
#142839=CARTESIAN_POINT('Ctrl Pts',(-69.8965579517147,-17.1650020070686,
0.));
#142840=CARTESIAN_POINT('Ctrl Pts',(-69.8965579517147,-17.1650020070686,
12.));
#142841=CARTESIAN_POINT('Ctrl Pts',(-69.8727382651292,-17.1675544029621,
0.));
#142842=CARTESIAN_POINT('Ctrl Pts',(-69.8727382651292,-17.1675544029621,
12.));
#142843=CARTESIAN_POINT('Ctrl Pts',(-69.8489583723417,-17.1700790212476,
0.));
#142844=CARTESIAN_POINT('Ctrl Pts',(-69.8489583723417,-17.1700790212476,
12.));
#142845=CARTESIAN_POINT('Ctrl Pts',(-69.8252183998713,-17.1725759104254,
0.));
#142846=CARTESIAN_POINT('Ctrl Pts',(-69.8252183998713,-17.1725759104254,
12.));
#142847=CARTESIAN_POINT('Ctrl Pts',(-69.8015184747404,-17.1750451192887,
0.));
#142848=CARTESIAN_POINT('Ctrl Pts',(-69.8015184747404,-17.1750451192887,
12.));
#142849=CARTESIAN_POINT('Ctrl Pts',(-69.7778587244788,-17.1774866969256,
0.));
#142850=CARTESIAN_POINT('Ctrl Pts',(-69.7778587244788,-17.1774866969256,
12.));
#142851=CARTESIAN_POINT('Ctrl Pts',(-69.7542392771216,-17.1799006927255,
0.));
#142852=CARTESIAN_POINT('Ctrl Pts',(-69.7542392771216,-17.1799006927255,
12.));
#142853=CARTESIAN_POINT('Ctrl Pts',(-69.7306602612125,-17.1822871563834,
0.));
#142854=CARTESIAN_POINT('Ctrl Pts',(-69.7306602612125,-17.1822871563834,
12.));
#142855=CARTESIAN_POINT('Ctrl Pts',(-69.7071218058149,-17.1846461378966,
0.));
#142856=CARTESIAN_POINT('Ctrl Pts',(-69.7071218058149,-17.1846461378966,
12.));
#142857=CARTESIAN_POINT('Ctrl Pts',(-69.6836240405151,-17.1869776875663,
0.));
#142858=CARTESIAN_POINT('Ctrl Pts',(-69.6836240405151,-17.1869776875663,
12.));
#142859=CARTESIAN_POINT('Ctrl Pts',(-69.6601670954277,-17.1892818560004,
0.));
#142860=CARTESIAN_POINT('Ctrl Pts',(-69.6601670954277,-17.1892818560004,
12.));
#142861=CARTESIAN_POINT('Ctrl Pts',(-69.6367511011927,-17.1915586941198,
0.));
#142862=CARTESIAN_POINT('Ctrl Pts',(-69.6367511011927,-17.1915586941198,
12.));
#142863=CARTESIAN_POINT('Ctrl Pts',(-69.6133761889787,-17.1938082531619,
0.));
#142864=CARTESIAN_POINT('Ctrl Pts',(-69.6133761889787,-17.1938082531619,
12.));
#142865=CARTESIAN_POINT('Ctrl Pts',(-69.5900424904954,-17.1960305846787,
0.));
#142866=CARTESIAN_POINT('Ctrl Pts',(-69.5900424904954,-17.1960305846787,
12.));
#142867=CARTESIAN_POINT('Ctrl Pts',(-69.5667501379984,-17.198225740538,
0.));
#142868=CARTESIAN_POINT('Ctrl Pts',(-69.5667501379984,-17.198225740538,
12.));
#142869=CARTESIAN_POINT('Ctrl Pts',(-69.5434992642932,-17.2003937729266,
0.));
#142870=CARTESIAN_POINT('Ctrl Pts',(-69.5434992642932,-17.2003937729266,
12.));
#142871=CARTESIAN_POINT('Ctrl Pts',(-69.5202900027329,-17.2025347343568,
0.));
#142872=CARTESIAN_POINT('Ctrl Pts',(-69.5202900027329,-17.2025347343568,
12.));
#142873=CARTESIAN_POINT('Ctrl Pts',(-69.497122487222,-17.2046486776697,
0.));
#142874=CARTESIAN_POINT('Ctrl Pts',(-69.497122487222,-17.2046486776697,
12.));
#142875=CARTESIAN_POINT('Ctrl Pts',(-69.4739968522271,-17.2067356560326,
0.));
#142876=CARTESIAN_POINT('Ctrl Pts',(-69.4739968522271,-17.2067356560326,
12.));
#142877=CARTESIAN_POINT('Ctrl Pts',(-69.4509132327836,-17.208795722942,
0.));
#142878=CARTESIAN_POINT('Ctrl Pts',(-69.4509132327836,-17.208795722942,
12.));
#142879=CARTESIAN_POINT('Ctrl Pts',(-69.4278717644989,-17.2108289322258,
0.));
#142880=CARTESIAN_POINT('Ctrl Pts',(-69.4278717644989,-17.2108289322258,
12.));
#142881=CARTESIAN_POINT('Ctrl Pts',(-69.4048725835516,-17.2128353380511,
0.));
#142882=CARTESIAN_POINT('Ctrl Pts',(-69.4048725835516,-17.2128353380511,
12.));
#142883=CARTESIAN_POINT('Ctrl Pts',(-69.3819158266955,-17.2148149949261,
0.));
#142884=CARTESIAN_POINT('Ctrl Pts',(-69.3819158266955,-17.2148149949261,
12.));
#142885=CARTESIAN_POINT('Ctrl Pts',(-69.359001631272,-17.2167679576991,
0.));
#142886=CARTESIAN_POINT('Ctrl Pts',(-69.359001631272,-17.2167679576991,
12.));
#142887=CARTESIAN_POINT('Ctrl Pts',(-69.3361301352149,-17.2186942815603,
0.));
#142888=CARTESIAN_POINT('Ctrl Pts',(-69.3361301352149,-17.2186942815603,
12.));
#142889=CARTESIAN_POINT('Ctrl Pts',(-69.3133014770542,-17.2205940220455,
0.));
#142890=CARTESIAN_POINT('Ctrl Pts',(-69.3133014770542,-17.2205940220455,
12.));
#142891=CARTESIAN_POINT('Ctrl Pts',(-69.2905157959141,-17.2224672350432,
0.));
#142892=CARTESIAN_POINT('Ctrl Pts',(-69.2905157959141,-17.2224672350432,
12.));
#142893=CARTESIAN_POINT('Ctrl Pts',(-69.2677732315199,-17.2243139767963,
0.));
#142894=CARTESIAN_POINT('Ctrl Pts',(-69.2677732315199,-17.2243139767963,
12.));
#142895=CARTESIAN_POINT('Ctrl Pts',(-69.2450739242092,-17.2261343039015,
0.));
#142896=CARTESIAN_POINT('Ctrl Pts',(-69.2450739242092,-17.2261343039015,
12.));
#142897=CARTESIAN_POINT('Ctrl Pts',(-69.2224180149377,-17.2279282733119,
0.));
#142898=CARTESIAN_POINT('Ctrl Pts',(-69.2224180149377,-17.2279282733119,
12.));
#142899=CARTESIAN_POINT('Ctrl Pts',(-69.1998056452837,-17.229695942341,
0.));
#142900=CARTESIAN_POINT('Ctrl Pts',(-69.1998056452837,-17.229695942341,
12.));
#142901=CARTESIAN_POINT('Ctrl Pts',(-69.1772369574462,-17.2314373686705,
0.));
#142902=CARTESIAN_POINT('Ctrl Pts',(-69.1772369574462,-17.2314373686705,
12.));
#142903=CARTESIAN_POINT('Ctrl Pts',(-69.1547120942542,-17.2331526103511,
0.));
#142904=CARTESIAN_POINT('Ctrl Pts',(-69.1547120942542,-17.2331526103511,
12.));
#142905=CARTESIAN_POINT('Ctrl Pts',(-69.1322311991759,-17.2348417258017,
0.));
#142906=CARTESIAN_POINT('Ctrl Pts',(-69.1322311991759,-17.2348417258017,
12.));
#142907=CARTESIAN_POINT('Ctrl Pts',(-69.1097944163244,-17.2365047738125,
0.));
#142908=CARTESIAN_POINT('Ctrl Pts',(-69.1097944163244,-17.2365047738125,
12.));
#142909=CARTESIAN_POINT('Ctrl Pts',(-69.0874018904598,-17.238141813549,
0.));
#142910=CARTESIAN_POINT('Ctrl Pts',(-69.0874018904598,-17.238141813549,
12.));
#142911=CARTESIAN_POINT('Ctrl Pts',(-69.0650537669859,-17.2397529045587,
0.));
#142912=CARTESIAN_POINT('Ctrl Pts',(-69.0650537669859,-17.2397529045587,
12.));
#142913=CARTESIAN_POINT('Ctrl Pts',(-69.0427501919636,-17.2413381067722,
0.));
#142914=CARTESIAN_POINT('Ctrl Pts',(-69.0427501919636,-17.2413381067722,
12.));
#142915=CARTESIAN_POINT('Ctrl Pts',(-69.0204913121226,-17.2428974805043,
0.));
#142916=CARTESIAN_POINT('Ctrl Pts',(-69.0204913121226,-17.2428974805043,
12.));
#142917=CARTESIAN_POINT('Ctrl Pts',(-68.9982772748694,-17.2444310864585,
0.));
#142918=CARTESIAN_POINT('Ctrl Pts',(-68.9982772748694,-17.2444310864585,
12.));
#142919=CARTESIAN_POINT('Ctrl Pts',(-68.9761082282922,-17.2459389857327,
0.));
#142920=CARTESIAN_POINT('Ctrl Pts',(-68.9761082282922,-17.2459389857327,
12.));
#142921=CARTESIAN_POINT('Ctrl Pts',(-68.9539843211618,-17.2474212398275,
0.));
#142922=CARTESIAN_POINT('Ctrl Pts',(-68.9539843211618,-17.2474212398275,
12.));
#142923=CARTESIAN_POINT('Ctrl Pts',(-68.9319057029407,-17.248877910643,
0.));
#142924=CARTESIAN_POINT('Ctrl Pts',(-68.9319057029407,-17.248877910643,
12.));
#142925=CARTESIAN_POINT('Ctrl Pts',(-68.9098725237868,-17.2503090604792,
0.));
#142926=CARTESIAN_POINT('Ctrl Pts',(-68.9098725237868,-17.2503090604792,
12.));
#142927=CARTESIAN_POINT('Ctrl Pts',(-68.8878849345557,-17.2517147520376,
0.));
#142928=CARTESIAN_POINT('Ctrl Pts',(-68.8878849345557,-17.2517147520376,
12.));
#142929=CARTESIAN_POINT('Ctrl Pts',(-68.8659430867977,-17.2530950484259,
0.));
#142930=CARTESIAN_POINT('Ctrl Pts',(-68.8659430867977,-17.2530950484259,
12.));
#142931=CARTESIAN_POINT('Ctrl Pts',(-68.8440471327563,-17.2544500131627,
0.));
#142932=CARTESIAN_POINT('Ctrl Pts',(-68.8440471327563,-17.2544500131627,
12.));
#142933=CARTESIAN_POINT('Ctrl Pts',(-68.8221972253954,-17.2557797101815,
0.));
#142934=CARTESIAN_POINT('Ctrl Pts',(-68.8221972253954,-17.2557797101815,
12.));
#142935=CARTESIAN_POINT('Ctrl Pts',(-68.8003935184193,-17.2570842038385,
0.));
#142936=CARTESIAN_POINT('Ctrl Pts',(-68.8003935184193,-17.2570842038385,
12.));
#142937=CARTESIAN_POINT('Ctrl Pts',(-68.7786361662876,-17.2583635589196,
0.));
#142938=CARTESIAN_POINT('Ctrl Pts',(-68.7786361662876,-17.2583635589196,
12.));
#142939=CARTESIAN_POINT('Ctrl Pts',(-68.7569253242312,-17.2596178406545,
0.));
#142940=CARTESIAN_POINT('Ctrl Pts',(-68.7569253242312,-17.2596178406545,
12.));
#142941=CARTESIAN_POINT('Ctrl Pts',(-68.7352611482519,-17.2608471147178,
0.));
#142942=CARTESIAN_POINT('Ctrl Pts',(-68.7352611482519,-17.2608471147178,
12.));
#142943=CARTESIAN_POINT('Ctrl Pts',(-68.7136437951074,-17.2620514472176,
0.));
#142944=CARTESIAN_POINT('Ctrl Pts',(-68.7136437951074,-17.2620514472176,
12.));
#142945=CARTESIAN_POINT('Ctrl Pts',(-68.6920734222932,-17.263230904689,
0.));
#142946=CARTESIAN_POINT('Ctrl Pts',(-68.6920734222932,-17.263230904689,
12.));
#142947=CARTESIAN_POINT('Ctrl Pts',(-68.6705501880263,-17.2643855540895,
0.));
#142948=CARTESIAN_POINT('Ctrl Pts',(-68.6705501880263,-17.2643855540895,
12.));
#142949=CARTESIAN_POINT('Ctrl Pts',(-68.6490742512085,-17.2655154627935,
0.));
#142950=CARTESIAN_POINT('Ctrl Pts',(-68.6490742512085,-17.2655154627935,
12.));
#142951=CARTESIAN_POINT('Ctrl Pts',(-68.6276457714757,-17.266620698609,
0.));
#142952=CARTESIAN_POINT('Ctrl Pts',(-68.6276457714757,-17.266620698609,
12.));
#142953=CARTESIAN_POINT('Ctrl Pts',(-68.606264909278,-17.2677013298061,
0.));
#142954=CARTESIAN_POINT('Ctrl Pts',(-68.606264909278,-17.2677013298061,
12.));
#142955=CARTESIAN_POINT('Ctrl Pts',(-68.5849318259449,-17.2687574251428,
0.));
#142956=CARTESIAN_POINT('Ctrl Pts',(-68.5849318259449,-17.2687574251428,
12.));
#142957=CARTESIAN_POINT('Ctrl Pts',(-68.5636466837502,-17.2697890538956,
0.));
#142958=CARTESIAN_POINT('Ctrl Pts',(-68.5636466837502,-17.2697890538956,
12.));
#142959=CARTESIAN_POINT('Ctrl Pts',(-68.5424096459746,-17.2707962858912,
0.));
#142960=CARTESIAN_POINT('Ctrl Pts',(-68.5424096459746,-17.2707962858912,
12.));
#142961=CARTESIAN_POINT('Ctrl Pts',(-68.5212208767835,-17.2717791914538,
0.));
#142962=CARTESIAN_POINT('Ctrl Pts',(-68.5212208767835,-17.2717791914538,
12.));
#142963=CARTESIAN_POINT('Ctrl Pts',(-68.5000805410896,-17.2727378413485,
0.));
#142964=CARTESIAN_POINT('Ctrl Pts',(-68.5000805410896,-17.2727378413485,
12.));
#142965=CARTESIAN_POINT('Ctrl Pts',(-68.4789888044357,-17.2736723067366,
0.));
#142966=CARTESIAN_POINT('Ctrl Pts',(-68.4789888044357,-17.2736723067366,
12.));
#142967=CARTESIAN_POINT('Ctrl Pts',(-68.4579458328208,-17.2745826591125,
0.));
#142968=CARTESIAN_POINT('Ctrl Pts',(-68.4579458328208,-17.2745826591125,
12.));
#142969=CARTESIAN_POINT('Ctrl Pts',(-68.4369517926803,-17.2754689703001,
0.));
#142970=CARTESIAN_POINT('Ctrl Pts',(-68.4369517926803,-17.2754689703001,
12.));
#142971=CARTESIAN_POINT('Ctrl Pts',(-68.4160068512781,-17.2763313126025,
0.));
#142972=CARTESIAN_POINT('Ctrl Pts',(-68.4160068512781,-17.2763313126025,
12.));
#142973=CARTESIAN_POINT('Ctrl Pts',(-68.3951111770498,-17.2771697589387,
0.));
#142974=CARTESIAN_POINT('Ctrl Pts',(-68.3951111770498,-17.2771697589387,
12.));
#142975=CARTESIAN_POINT('Ctrl Pts',(-68.374264939895,-17.2779843829605,
0.));
#142976=CARTESIAN_POINT('Ctrl Pts',(-68.374264939895,-17.2779843829605,
12.));
#142977=CARTESIAN_POINT('Ctrl Pts',(-68.353468311648,-17.2787752592475,
0.));
#142978=CARTESIAN_POINT('Ctrl Pts',(-68.353468311648,-17.2787752592475,
12.));
#142979=CARTESIAN_POINT('Ctrl Pts',(-68.3327214657533,-17.2795424631789,
0.));
#142980=CARTESIAN_POINT('Ctrl Pts',(-68.3327214657533,-17.2795424631789,
12.));
#142981=CARTESIAN_POINT('Ctrl Pts',(-68.3120245763884,-17.2802860705807,
0.));
#142982=CARTESIAN_POINT('Ctrl Pts',(-68.3120245763884,-17.2802860705807,
12.));
#142983=CARTESIAN_POINT('Ctrl Pts',(-68.2913778177258,-17.2810061574352,
0.));
#142984=CARTESIAN_POINT('Ctrl Pts',(-68.2913778177258,-17.2810061574352,
12.));
#142985=CARTESIAN_POINT('Ctrl Pts',(-68.2707813631761,-17.2817027995838,
0.));
#142986=CARTESIAN_POINT('Ctrl Pts',(-68.2707813631761,-17.2817027995838,
12.));
#142987=CARTESIAN_POINT('Ctrl Pts',(-68.250235384512,-17.2823760723886,
0.));
#142988=CARTESIAN_POINT('Ctrl Pts',(-68.250235384512,-17.2823760723886,
12.));
#142989=CARTESIAN_POINT('Ctrl Pts',(-68.2297400535339,-17.2830260513878,
0.));
#142990=CARTESIAN_POINT('Ctrl Pts',(-68.2297400535339,-17.2830260513878,
12.));
#142991=CARTESIAN_POINT('Ctrl Pts',(-68.2092955440591,-17.2836528130825,
0.));
#142992=CARTESIAN_POINT('Ctrl Pts',(-68.2092955440591,-17.2836528130825,
12.));
#142993=CARTESIAN_POINT('Ctrl Pts',(-68.1889020335418,-17.2842564355796,
0.));
#142994=CARTESIAN_POINT('Ctrl Pts',(-68.1889020335418,-17.2842564355796,
12.));
#142995=CARTESIAN_POINT('Ctrl Pts',(-68.1685597054193,-17.2848369995283,
0.));
#142996=CARTESIAN_POINT('Ctrl Pts',(-68.1685597054193,-17.2848369995283,
12.));
#142997=CARTESIAN_POINT('Ctrl Pts',(-68.1482687493176,-17.2853945882059,
0.));
#142998=CARTESIAN_POINT('Ctrl Pts',(-68.1482687493176,-17.2853945882059,
12.));
#142999=CARTESIAN_POINT('Ctrl Pts',(-68.1280293561473,-17.2859292855694,
0.));
#143000=CARTESIAN_POINT('Ctrl Pts',(-68.1280293561473,-17.2859292855694,
12.));
#143001=CARTESIAN_POINT('Ctrl Pts',(-68.1078417137865,-17.2864411745455,
0.));
#143002=CARTESIAN_POINT('Ctrl Pts',(-68.1078417137865,-17.2864411745455,
12.));
#143003=CARTESIAN_POINT('Ctrl Pts',(-68.0877060033229,-17.2869303355438,
0.));
#143004=CARTESIAN_POINT('Ctrl Pts',(-68.0877060033229,-17.2869303355438,
12.));
#143005=CARTESIAN_POINT('Ctrl Pts',(-68.0676223930469,-17.2873968440855,
0.));
#143006=CARTESIAN_POINT('Ctrl Pts',(-68.0676223930469,-17.2873968440855,
12.));
#143007=CARTESIAN_POINT('Ctrl Pts',(-68.0475910442494,-17.2878407730981,
0.));
#143008=CARTESIAN_POINT('Ctrl Pts',(-68.0475910442494,-17.2878407730981,
12.));
#143009=CARTESIAN_POINT('Ctrl Pts',(-68.027612122741,-17.2882621974737,
0.));
#143010=CARTESIAN_POINT('Ctrl Pts',(-68.027612122741,-17.2882621974737,
12.));
#143011=CARTESIAN_POINT('Ctrl Pts',(-68.007685808115,-17.28866119774,0.));
#143012=CARTESIAN_POINT('Ctrl Pts',(-68.007685808115,-17.28866119774,12.));
#143013=CARTESIAN_POINT('Ctrl Pts',(-67.9878123049132,-17.2890378644843,
0.));
#143014=CARTESIAN_POINT('Ctrl Pts',(-67.9878123049132,-17.2890378644843,
12.));
#143015=CARTESIAN_POINT('Ctrl Pts',(-67.9679918502441,-17.2893923013852,
0.));
#143016=CARTESIAN_POINT('Ctrl Pts',(-67.9679918502441,-17.2893923013852,
12.));
#143017=CARTESIAN_POINT('Ctrl Pts',(-67.9482246901517,-17.2897246158895,
0.));
#143018=CARTESIAN_POINT('Ctrl Pts',(-67.9482246901517,-17.2897246158895,
12.));
#143019=CARTESIAN_POINT('Ctrl Pts',(-67.9285110571662,-17.2900349103956,
0.));
#143020=CARTESIAN_POINT('Ctrl Pts',(-67.9285110571662,-17.2900349103956,
12.));
#143021=CARTESIAN_POINT('Ctrl Pts',(-67.908851149676,-17.2903232740717,
0.));
#143022=CARTESIAN_POINT('Ctrl Pts',(-67.908851149676,-17.2903232740717,
12.));
#143023=CARTESIAN_POINT('Ctrl Pts',(-67.8892451049871,-17.2905897724029,
0.));
#143024=CARTESIAN_POINT('Ctrl Pts',(-67.8892451049871,-17.2905897724029,
12.));
#143025=CARTESIAN_POINT('Ctrl Pts',(-67.8696929979178,-17.2908344459816,
0.));
#143026=CARTESIAN_POINT('Ctrl Pts',(-67.8696929979178,-17.2908344459816,
12.));
#143027=CARTESIAN_POINT('Ctrl Pts',(-67.8540944890057,-17.2910127431203,
0.));
#143028=CARTESIAN_POINT('Ctrl Pts',(-67.8540944890057,-17.2910127431203,
12.));
#143029=CARTESIAN_POINT('Ctrl Pts',(-67.8424198971214,-17.2911366591419,
0.));
#143030=CARTESIAN_POINT('Ctrl Pts',(-67.8424198971214,-17.2911366591419,
12.));
#143031=CARTESIAN_POINT('Ctrl Pts',(-67.8346476309106,-17.2912149114145,
0.));
#143032=CARTESIAN_POINT('Ctrl Pts',(-67.8346476309106,-17.2912149114145,
12.));
#143033=CARTESIAN_POINT('Ctrl Pts',(-67.8307641965655,-17.2912529479484,
0.));
#143034=CARTESIAN_POINT('Ctrl Pts',(-67.8307641965655,-17.2912529479484,
12.));
#143035=CARTESIAN_POINT('',(-67.8307641965655,-17.2912529479484,12.));
#143036=CARTESIAN_POINT('Ctrl Pts',(-67.8307641965655,-17.2912529479484,
12.));
#143037=CARTESIAN_POINT('Ctrl Pts',(-67.8346476309106,-17.2912149114145,
12.));
#143038=CARTESIAN_POINT('Ctrl Pts',(-67.8424198971214,-17.2911366591419,
12.));
#143039=CARTESIAN_POINT('Ctrl Pts',(-67.8540944890057,-17.2910127431203,
12.));
#143040=CARTESIAN_POINT('Ctrl Pts',(-67.8696929979178,-17.2908344459816,
12.));
#143041=CARTESIAN_POINT('Ctrl Pts',(-67.8892451049871,-17.2905897724029,
12.));
#143042=CARTESIAN_POINT('Ctrl Pts',(-67.908851149676,-17.2903232740717,
12.));
#143043=CARTESIAN_POINT('Ctrl Pts',(-67.9285110571662,-17.2900349103956,
12.));
#143044=CARTESIAN_POINT('Ctrl Pts',(-67.9482246901517,-17.2897246158895,
12.));
#143045=CARTESIAN_POINT('Ctrl Pts',(-67.9679918502441,-17.2893923013852,
12.));
#143046=CARTESIAN_POINT('Ctrl Pts',(-67.9878123049132,-17.2890378644843,
12.));
#143047=CARTESIAN_POINT('Ctrl Pts',(-68.007685808115,-17.28866119774,12.));
#143048=CARTESIAN_POINT('Ctrl Pts',(-68.027612122741,-17.2882621974737,
12.));
#143049=CARTESIAN_POINT('Ctrl Pts',(-68.0475910442494,-17.2878407730981,
12.));
#143050=CARTESIAN_POINT('Ctrl Pts',(-68.0676223930469,-17.2873968440855,
12.));
#143051=CARTESIAN_POINT('Ctrl Pts',(-68.0877060033229,-17.2869303355438,
12.));
#143052=CARTESIAN_POINT('Ctrl Pts',(-68.1078417137865,-17.2864411745455,
12.));
#143053=CARTESIAN_POINT('Ctrl Pts',(-68.1280293561473,-17.2859292855694,
12.));
#143054=CARTESIAN_POINT('Ctrl Pts',(-68.1482687493176,-17.2853945882059,
12.));
#143055=CARTESIAN_POINT('Ctrl Pts',(-68.1685597054193,-17.2848369995283,
12.));
#143056=CARTESIAN_POINT('Ctrl Pts',(-68.1889020335418,-17.2842564355796,
12.));
#143057=CARTESIAN_POINT('Ctrl Pts',(-68.2092955440591,-17.2836528130825,
12.));
#143058=CARTESIAN_POINT('Ctrl Pts',(-68.2297400535339,-17.2830260513878,
12.));
#143059=CARTESIAN_POINT('Ctrl Pts',(-68.250235384512,-17.2823760723886,
12.));
#143060=CARTESIAN_POINT('Ctrl Pts',(-68.2707813631761,-17.2817027995838,
12.));
#143061=CARTESIAN_POINT('Ctrl Pts',(-68.2913778177258,-17.2810061574352,
12.));
#143062=CARTESIAN_POINT('Ctrl Pts',(-68.3120245763884,-17.2802860705807,
12.));
#143063=CARTESIAN_POINT('Ctrl Pts',(-68.3327214657533,-17.2795424631789,
12.));
#143064=CARTESIAN_POINT('Ctrl Pts',(-68.353468311648,-17.2787752592475,
12.));
#143065=CARTESIAN_POINT('Ctrl Pts',(-68.374264939895,-17.2779843829605,
12.));
#143066=CARTESIAN_POINT('Ctrl Pts',(-68.3951111770498,-17.2771697589387,
12.));
#143067=CARTESIAN_POINT('Ctrl Pts',(-68.4160068512781,-17.2763313126025,
12.));
#143068=CARTESIAN_POINT('Ctrl Pts',(-68.4369517926803,-17.2754689703001,
12.));
#143069=CARTESIAN_POINT('Ctrl Pts',(-68.4579458328208,-17.2745826591125,
12.));
#143070=CARTESIAN_POINT('Ctrl Pts',(-68.4789888044357,-17.2736723067366,
12.));
#143071=CARTESIAN_POINT('Ctrl Pts',(-68.5000805410896,-17.2727378413485,
12.));
#143072=CARTESIAN_POINT('Ctrl Pts',(-68.5212208767835,-17.2717791914538,
12.));
#143073=CARTESIAN_POINT('Ctrl Pts',(-68.5424096459746,-17.2707962858912,
12.));
#143074=CARTESIAN_POINT('Ctrl Pts',(-68.5636466837502,-17.2697890538956,
12.));
#143075=CARTESIAN_POINT('Ctrl Pts',(-68.5849318259449,-17.2687574251428,
12.));
#143076=CARTESIAN_POINT('Ctrl Pts',(-68.606264909278,-17.2677013298061,
12.));
#143077=CARTESIAN_POINT('Ctrl Pts',(-68.6276457714757,-17.266620698609,
12.));
#143078=CARTESIAN_POINT('Ctrl Pts',(-68.6490742512085,-17.2655154627935,
12.));
#143079=CARTESIAN_POINT('Ctrl Pts',(-68.6705501880263,-17.2643855540895,
12.));
#143080=CARTESIAN_POINT('Ctrl Pts',(-68.6920734222932,-17.263230904689,
12.));
#143081=CARTESIAN_POINT('Ctrl Pts',(-68.7136437951074,-17.2620514472176,
12.));
#143082=CARTESIAN_POINT('Ctrl Pts',(-68.7352611482519,-17.2608471147178,
12.));
#143083=CARTESIAN_POINT('Ctrl Pts',(-68.7569253242312,-17.2596178406545,
12.));
#143084=CARTESIAN_POINT('Ctrl Pts',(-68.7786361662876,-17.2583635589196,
12.));
#143085=CARTESIAN_POINT('Ctrl Pts',(-68.8003935184193,-17.2570842038385,
12.));
#143086=CARTESIAN_POINT('Ctrl Pts',(-68.8221972253954,-17.2557797101815,
12.));
#143087=CARTESIAN_POINT('Ctrl Pts',(-68.8440471327563,-17.2544500131627,
12.));
#143088=CARTESIAN_POINT('Ctrl Pts',(-68.8659430867977,-17.2530950484259,
12.));
#143089=CARTESIAN_POINT('Ctrl Pts',(-68.8878849345557,-17.2517147520376,
12.));
#143090=CARTESIAN_POINT('Ctrl Pts',(-68.9098725237868,-17.2503090604792,
12.));
#143091=CARTESIAN_POINT('Ctrl Pts',(-68.9319057029407,-17.248877910643,
12.));
#143092=CARTESIAN_POINT('Ctrl Pts',(-68.9539843211618,-17.2474212398275,
12.));
#143093=CARTESIAN_POINT('Ctrl Pts',(-68.9761082282922,-17.2459389857327,
12.));
#143094=CARTESIAN_POINT('Ctrl Pts',(-68.9982772748694,-17.2444310864585,
12.));
#143095=CARTESIAN_POINT('Ctrl Pts',(-69.0204913121226,-17.2428974805043,
12.));
#143096=CARTESIAN_POINT('Ctrl Pts',(-69.0427501919636,-17.2413381067722,
12.));
#143097=CARTESIAN_POINT('Ctrl Pts',(-69.0650537669859,-17.2397529045587,
12.));
#143098=CARTESIAN_POINT('Ctrl Pts',(-69.0874018904598,-17.238141813549,
12.));
#143099=CARTESIAN_POINT('Ctrl Pts',(-69.1097944163244,-17.2365047738125,
12.));
#143100=CARTESIAN_POINT('Ctrl Pts',(-69.1322311991759,-17.2348417258017,
12.));
#143101=CARTESIAN_POINT('Ctrl Pts',(-69.1547120942542,-17.2331526103511,
12.));
#143102=CARTESIAN_POINT('Ctrl Pts',(-69.1772369574462,-17.2314373686705,
12.));
#143103=CARTESIAN_POINT('Ctrl Pts',(-69.1998056452837,-17.229695942341,
12.));
#143104=CARTESIAN_POINT('Ctrl Pts',(-69.2224180149377,-17.2279282733119,
12.));
#143105=CARTESIAN_POINT('Ctrl Pts',(-69.2450739242092,-17.2261343039015,
12.));
#143106=CARTESIAN_POINT('Ctrl Pts',(-69.2677732315199,-17.2243139767963,
12.));
#143107=CARTESIAN_POINT('Ctrl Pts',(-69.2905157959141,-17.2224672350432,
12.));
#143108=CARTESIAN_POINT('Ctrl Pts',(-69.3133014770542,-17.2205940220455,
12.));
#143109=CARTESIAN_POINT('Ctrl Pts',(-69.3361301352149,-17.2186942815603,
12.));
#143110=CARTESIAN_POINT('Ctrl Pts',(-69.359001631272,-17.2167679576991,
12.));
#143111=CARTESIAN_POINT('Ctrl Pts',(-69.3819158266955,-17.2148149949261,
12.));
#143112=CARTESIAN_POINT('Ctrl Pts',(-69.4048725835516,-17.2128353380511,
12.));
#143113=CARTESIAN_POINT('Ctrl Pts',(-69.4278717644989,-17.2108289322258,
12.));
#143114=CARTESIAN_POINT('Ctrl Pts',(-69.4509132327836,-17.208795722942,
12.));
#143115=CARTESIAN_POINT('Ctrl Pts',(-69.4739968522271,-17.2067356560326,
12.));
#143116=CARTESIAN_POINT('Ctrl Pts',(-69.497122487222,-17.2046486776697,
12.));
#143117=CARTESIAN_POINT('Ctrl Pts',(-69.5202900027329,-17.2025347343568,
12.));
#143118=CARTESIAN_POINT('Ctrl Pts',(-69.5434992642932,-17.2003937729266,
12.));
#143119=CARTESIAN_POINT('Ctrl Pts',(-69.5667501379984,-17.198225740538,
12.));
#143120=CARTESIAN_POINT('Ctrl Pts',(-69.5900424904954,-17.1960305846787,
12.));
#143121=CARTESIAN_POINT('Ctrl Pts',(-69.6133761889787,-17.1938082531619,
12.));
#143122=CARTESIAN_POINT('Ctrl Pts',(-69.6367511011927,-17.1915586941198,
12.));
#143123=CARTESIAN_POINT('Ctrl Pts',(-69.6601670954277,-17.1892818560004,
12.));
#143124=CARTESIAN_POINT('Ctrl Pts',(-69.6836240405151,-17.1869776875663,
12.));
#143125=CARTESIAN_POINT('Ctrl Pts',(-69.7071218058149,-17.1846461378966,
12.));
#143126=CARTESIAN_POINT('Ctrl Pts',(-69.7306602612125,-17.1822871563834,
12.));
#143127=CARTESIAN_POINT('Ctrl Pts',(-69.7542392771216,-17.1799006927255,
12.));
#143128=CARTESIAN_POINT('Ctrl Pts',(-69.7778587244788,-17.1774866969256,
12.));
#143129=CARTESIAN_POINT('Ctrl Pts',(-69.8015184747404,-17.1750451192887,
12.));
#143130=CARTESIAN_POINT('Ctrl Pts',(-69.8252183998713,-17.1725759104254,
12.));
#143131=CARTESIAN_POINT('Ctrl Pts',(-69.8489583723417,-17.1700790212476,
12.));
#143132=CARTESIAN_POINT('Ctrl Pts',(-69.8727382651292,-17.1675544029621,
12.));
#143133=CARTESIAN_POINT('Ctrl Pts',(-69.8965579517147,-17.1650020070686,
12.));
#143134=CARTESIAN_POINT('Ctrl Pts',(-69.9204173060779,-17.1624217853577,
12.));
#143135=CARTESIAN_POINT('Ctrl Pts',(-69.9443162026865,-17.1598136899144,
12.));
#143136=CARTESIAN_POINT('Ctrl Pts',(-69.9682545164942,-17.157177673114,
12.));
#143137=CARTESIAN_POINT('Ctrl Pts',(-69.9922321229428,-17.1545136876161,
12.));
#143138=CARTESIAN_POINT('Ctrl Pts',(-70.0162488979586,-17.1518216863624,
12.));
#143139=CARTESIAN_POINT('Ctrl Pts',(-70.040304717948,-17.1491016225748,
12.));
#143140=CARTESIAN_POINT('Ctrl Pts',(-70.0643994597865,-17.1463534497592,
12.));
#143141=CARTESIAN_POINT('Ctrl Pts',(-70.0885330008169,-17.1435771217015,
12.));
#143142=CARTESIAN_POINT('Ctrl Pts',(-70.1127052188515,-17.1407725924615,
12.));
#143143=CARTESIAN_POINT('Ctrl Pts',(-70.1369159921686,-17.1379398163708,
12.));
#143144=CARTESIAN_POINT('Ctrl Pts',(-70.1611651995085,-17.1350787480313,
12.));
#143145=CARTESIAN_POINT('Ctrl Pts',(-70.1854527200636,-17.1321893423183,
12.));
#143146=CARTESIAN_POINT('Ctrl Pts',(-70.2097784334749,-17.1292715543779,
12.));
#143147=CARTESIAN_POINT('Ctrl Pts',(-70.2341422198362,-17.1263253396202,
12.));
#143148=CARTESIAN_POINT('Ctrl Pts',(-70.2585439596899,-17.1233506537176,
12.));
#143149=CARTESIAN_POINT('Ctrl Pts',(-70.2829835340239,-17.1203474526031,
12.));
#143150=CARTESIAN_POINT('Ctrl Pts',(-70.3074608242613,-17.1173156924733,
12.));
#143151=CARTESIAN_POINT('Ctrl Pts',(-70.3319757122576,-17.1142553297869,
12.));
#143152=CARTESIAN_POINT('Ctrl Pts',(-70.356528080303,-17.111166321257,12.));
#143153=CARTESIAN_POINT('Ctrl Pts',(-70.3811178111206,-17.1080486238499,
12.));
#143154=CARTESIAN_POINT('Ctrl Pts',(-70.4057447878621,-17.1049021947833,
12.));
#143155=CARTESIAN_POINT('Ctrl Pts',(-70.4304088940998,-17.1017269915289,
12.));
#143156=CARTESIAN_POINT('Ctrl Pts',(-70.4551100138221,-17.098522971812,
12.));
#143157=CARTESIAN_POINT('Ctrl Pts',(-70.4798480314364,-17.0952900936044,
12.));
#143158=CARTESIAN_POINT('Ctrl Pts',(-70.5046228317669,-17.0920283151217,
12.));
#143159=CARTESIAN_POINT('Ctrl Pts',(-70.5294343000516,-17.0887375948221,
12.));
#143160=CARTESIAN_POINT('Ctrl Pts',(-70.5542823219346,-17.085417891409,
12.));
#143161=CARTESIAN_POINT('Ctrl Pts',(-70.5791667834599,-17.0820691638314,
12.));
#143162=CARTESIAN_POINT('Ctrl Pts',(-70.6040875710762,-17.0786913712766,
12.));
#143163=CARTESIAN_POINT('Ctrl Pts',(-70.6290445716341,-17.0752844731679,
12.));
#143164=CARTESIAN_POINT('Ctrl Pts',(-70.6540376723839,-17.0718484291623,
12.));
#143165=CARTESIAN_POINT('Ctrl Pts',(-70.6790667609678,-17.0683831991532,
12.));
#143166=CARTESIAN_POINT('Ctrl Pts',(-70.7041317254127,-17.0648887432714,
12.));
#143167=CARTESIAN_POINT('Ctrl Pts',(-70.7292324541348,-17.0613650218788,
12.));
#143168=CARTESIAN_POINT('Ctrl Pts',(-70.754368835938,-17.0578119955651,
12.));
#143169=CARTESIAN_POINT('Ctrl Pts',(-70.7795407600127,-17.0542296251462,
12.));
#143170=CARTESIAN_POINT('Ctrl Pts',(-70.8047481159298,-17.0506178716661,
12.));
#143171=CARTESIAN_POINT('Ctrl Pts',(-70.8299907936334,-17.0469766964001,
12.));
#143172=CARTESIAN_POINT('Ctrl Pts',(-70.8552686834423,-17.0433060608474,
12.));
#143173=CARTESIAN_POINT('Ctrl Pts',(-70.8805816760501,-17.0396059267277,
12.));
#143174=CARTESIAN_POINT('Ctrl Pts',(-70.9059296625214,-17.0358762559786,
12.));
#143175=CARTESIAN_POINT('Ctrl Pts',(-70.9313125342876,-17.0321170107564,
12.));
#143176=CARTESIAN_POINT('Ctrl Pts',(-70.956730183136,-17.0283281534392,
12.));
#143177=CARTESIAN_POINT('Ctrl Pts',(-70.9821825012136,-17.0245096466229,
12.));
#143178=CARTESIAN_POINT('Ctrl Pts',(-71.0076693810301,-17.0206614531166,
12.));
#143179=CARTESIAN_POINT('Ctrl Pts',(-71.0331907154574,-17.0167835359419,
12.));
#143180=CARTESIAN_POINT('Ctrl Pts',(-71.0587463977268,-17.0128758583334,
12.));
#143181=CARTESIAN_POINT('Ctrl Pts',(-71.0843363214221,-17.0089383837437,
12.));
#143182=CARTESIAN_POINT('Ctrl Pts',(-71.1099603804786,-17.0049710758393,
12.));
#143183=CARTESIAN_POINT('Ctrl Pts',(-71.1356184691806,-17.0009738984935,
12.));
#143184=CARTESIAN_POINT('Ctrl Pts',(-71.1613104821568,-16.9969468157824,
12.));
#143185=CARTESIAN_POINT('Ctrl Pts',(-71.187036314374,-16.9928897919828,
12.));
#143186=CARTESIAN_POINT('Ctrl Pts',(-71.212795861124,-16.9888027915742,
12.));
#143187=CARTESIAN_POINT('Ctrl Pts',(-71.2385890180221,-16.9846857792383,
12.));
#143188=CARTESIAN_POINT('Ctrl Pts',(-71.2644156810198,-16.9805387198571,
12.));
#143189=CARTESIAN_POINT('Ctrl Pts',(-71.290275746412,-16.9763615785136,
12.));
#143190=CARTESIAN_POINT('Ctrl Pts',(-71.3161691108427,-16.9721543204951,
12.));
#143191=CARTESIAN_POINT('Ctrl Pts',(-71.3420956713082,-16.9679169112994,
12.));
#143192=CARTESIAN_POINT('Ctrl Pts',(-71.3680553251562,-16.9636493166397,
12.));
#143193=CARTESIAN_POINT('Ctrl Pts',(-71.3940479700677,-16.9593515024276,
12.));
#143194=CARTESIAN_POINT('Ctrl Pts',(-71.4200735040384,-16.955023434762,
12.));
#143195=CARTESIAN_POINT('Ctrl Pts',(-71.4461318253563,-16.9506650799189,
12.));
#143196=CARTESIAN_POINT('Ctrl Pts',(-71.4722228325794,-16.9462764043443,
12.));
#143197=CARTESIAN_POINT('Ctrl Pts',(-71.4983464245055,-16.9418573746488,
12.));
#143198=CARTESIAN_POINT('Ctrl Pts',(-71.5245025002139,-16.9374079576201,
12.));
#143199=CARTESIAN_POINT('Ctrl Pts',(-71.5506909591128,-16.9329281202377,
12.));
#143200=CARTESIAN_POINT('Ctrl Pts',(-71.5769117009842,-16.9284178296933,
12.));
#143201=CARTESIAN_POINT('Ctrl Pts',(-71.6031646260174,-16.9238770534071,
12.));
#143202=CARTESIAN_POINT('Ctrl Pts',(-71.6294496348652,-16.9193057590607,
12.));
#143203=CARTESIAN_POINT('Ctrl Pts',(-71.6557666285917,-16.9147039145717,
12.));
#143204=CARTESIAN_POINT('Ctrl Pts',(-71.6821155085612,-16.9100714880368,
12.));
#143205=CARTESIAN_POINT('Ctrl Pts',(-71.7084961763357,-16.9054084476847,
12.));
#143206=CARTESIAN_POINT('Ctrl Pts',(-71.7349085335796,-16.9007147618344,
12.));
#143207=CARTESIAN_POINT('Ctrl Pts',(-71.7613524819235,-16.8959903988409,
12.));
#143208=CARTESIAN_POINT('Ctrl Pts',(-71.7878279229546,-16.8912353270942,
12.));
#143209=CARTESIAN_POINT('Ctrl Pts',(-71.8143347584962,-16.8864495151344,
12.));
#143210=CARTESIAN_POINT('Ctrl Pts',(-71.8408728908258,-16.881632931747,
12.));
#143211=CARTESIAN_POINT('Ctrl Pts',(-71.8674422229149,-16.87678554607,12.));
#143212=CARTESIAN_POINT('Ctrl Pts',(-71.8940426586534,-16.871907327697,
12.));
#143213=CARTESIAN_POINT('Ctrl Pts',(-71.9206741030887,-16.866998246792,
12.));
#143214=CARTESIAN_POINT('Ctrl Pts',(-71.9473364618922,-16.8620582738437,
12.));
#143215=CARTESIAN_POINT('Ctrl Pts',(-71.9740296408347,-16.8570873794269,
12.));
#143216=CARTESIAN_POINT('Ctrl Pts',(-72.0007535452081,-16.8520855339446,
12.));
#143217=CARTESIAN_POINT('Ctrl Pts',(-72.0275080793727,-16.8470527074275,
12.));
#143218=CARTESIAN_POINT('Ctrl Pts',(-72.0542931459825,-16.8419888691976,
12.));
#143219=CARTESIAN_POINT('Ctrl Pts',(-72.0811086466121,-16.8368939881446,
12.));
#143220=CARTESIAN_POINT('Ctrl Pts',(-72.1079544831513,-16.8317680333404,
12.));
#143221=CARTESIAN_POINT('Ctrl Pts',(-72.13483055902,-16.8266109745795,12.));
#143222=CARTESIAN_POINT('Ctrl Pts',(-72.1617367803235,-16.8214227828942,
12.));
#143223=CARTESIAN_POINT('Ctrl Pts',(-72.1886730573452,-16.8162034312269,
12.));
#143224=CARTESIAN_POINT('Ctrl Pts',(-72.2156393048975,-16.8109528945896,
12.));
#143225=CARTESIAN_POINT('Ctrl Pts',(-72.2387802230855,-16.8064254147775,
12.));
#143226=CARTESIAN_POINT('Ctrl Pts',(-72.2565380035259,-16.8029374213794,
12.));
#143227=CARTESIAN_POINT('Ctrl Pts',(-72.2688994295262,-16.8005027425863,
12.));
#143228=CARTESIAN_POINT('Ctrl Pts',(-72.2758557891326,-16.799130531775,
12.));
#143229=CARTESIAN_POINT('Ctrl Pts',(-72.2774028393911,-16.7988252568749,
12.));
#143230=CARTESIAN_POINT('',(-67.8307641965655,-17.2912529479484,0.));
#143231=CARTESIAN_POINT('',(-67.8307641965655,-17.2912529479484,0.));
#143232=CARTESIAN_POINT('Ctrl Pts',(-72.277402839391,-16.7988252568749,
0.));
#143233=CARTESIAN_POINT('Ctrl Pts',(-72.2758557891325,-16.799130531775,
0.));
#143234=CARTESIAN_POINT('Ctrl Pts',(-72.2688994295261,-16.8005027425863,
0.));
#143235=CARTESIAN_POINT('Ctrl Pts',(-72.2565380035259,-16.8029374213794,
0.));
#143236=CARTESIAN_POINT('Ctrl Pts',(-72.2387802230855,-16.8064254147775,
0.));
#143237=CARTESIAN_POINT('Ctrl Pts',(-72.2156393048975,-16.8109528945896,
0.));
#143238=CARTESIAN_POINT('Ctrl Pts',(-72.1886730573452,-16.8162034312269,
0.));
#143239=CARTESIAN_POINT('Ctrl Pts',(-72.1617367803235,-16.8214227828942,
0.));
#143240=CARTESIAN_POINT('Ctrl Pts',(-72.13483055902,-16.8266109745795,0.));
#143241=CARTESIAN_POINT('Ctrl Pts',(-72.1079544831513,-16.8317680333404,
0.));
#143242=CARTESIAN_POINT('Ctrl Pts',(-72.0811086466121,-16.8368939881446,
0.));
#143243=CARTESIAN_POINT('Ctrl Pts',(-72.0542931459825,-16.8419888691976,
0.));
#143244=CARTESIAN_POINT('Ctrl Pts',(-72.0275080793727,-16.8470527074275,
0.));
#143245=CARTESIAN_POINT('Ctrl Pts',(-72.0007535452081,-16.8520855339446,
0.));
#143246=CARTESIAN_POINT('Ctrl Pts',(-71.9740296408347,-16.8570873794269,
0.));
#143247=CARTESIAN_POINT('Ctrl Pts',(-71.9473364618922,-16.8620582738437,
0.));
#143248=CARTESIAN_POINT('Ctrl Pts',(-71.9206741030887,-16.866998246792,
0.));
#143249=CARTESIAN_POINT('Ctrl Pts',(-71.8940426586534,-16.871907327697,
0.));
#143250=CARTESIAN_POINT('Ctrl Pts',(-71.8674422229149,-16.87678554607,0.));
#143251=CARTESIAN_POINT('Ctrl Pts',(-71.8408728908258,-16.881632931747,
0.));
#143252=CARTESIAN_POINT('Ctrl Pts',(-71.8143347584962,-16.8864495151344,
0.));
#143253=CARTESIAN_POINT('Ctrl Pts',(-71.7878279229546,-16.8912353270942,
0.));
#143254=CARTESIAN_POINT('Ctrl Pts',(-71.7613524819235,-16.8959903988409,
0.));
#143255=CARTESIAN_POINT('Ctrl Pts',(-71.7349085335796,-16.9007147618344,
0.));
#143256=CARTESIAN_POINT('Ctrl Pts',(-71.7084961763357,-16.9054084476847,
0.));
#143257=CARTESIAN_POINT('Ctrl Pts',(-71.6821155085612,-16.9100714880368,
0.));
#143258=CARTESIAN_POINT('Ctrl Pts',(-71.6557666285917,-16.9147039145717,
0.));
#143259=CARTESIAN_POINT('Ctrl Pts',(-71.6294496348652,-16.9193057590607,
0.));
#143260=CARTESIAN_POINT('Ctrl Pts',(-71.6031646260174,-16.9238770534071,
0.));
#143261=CARTESIAN_POINT('Ctrl Pts',(-71.5769117009842,-16.9284178296933,
0.));
#143262=CARTESIAN_POINT('Ctrl Pts',(-71.5506909591128,-16.9329281202377,
0.));
#143263=CARTESIAN_POINT('Ctrl Pts',(-71.5245025002139,-16.9374079576201,
0.));
#143264=CARTESIAN_POINT('Ctrl Pts',(-71.4983464245055,-16.9418573746488,
0.));
#143265=CARTESIAN_POINT('Ctrl Pts',(-71.4722228325794,-16.9462764043443,
0.));
#143266=CARTESIAN_POINT('Ctrl Pts',(-71.4461318253563,-16.9506650799189,
0.));
#143267=CARTESIAN_POINT('Ctrl Pts',(-71.4200735040384,-16.955023434762,
0.));
#143268=CARTESIAN_POINT('Ctrl Pts',(-71.3940479700677,-16.9593515024276,
0.));
#143269=CARTESIAN_POINT('Ctrl Pts',(-71.3680553251562,-16.9636493166397,
0.));
#143270=CARTESIAN_POINT('Ctrl Pts',(-71.3420956713082,-16.9679169112994,
0.));
#143271=CARTESIAN_POINT('Ctrl Pts',(-71.3161691108427,-16.9721543204951,
0.));
#143272=CARTESIAN_POINT('Ctrl Pts',(-71.290275746412,-16.9763615785136,
0.));
#143273=CARTESIAN_POINT('Ctrl Pts',(-71.2644156810198,-16.9805387198571,
0.));
#143274=CARTESIAN_POINT('Ctrl Pts',(-71.2385890180221,-16.9846857792383,
0.));
#143275=CARTESIAN_POINT('Ctrl Pts',(-71.212795861124,-16.9888027915742,
0.));
#143276=CARTESIAN_POINT('Ctrl Pts',(-71.187036314374,-16.9928897919828,
0.));
#143277=CARTESIAN_POINT('Ctrl Pts',(-71.1613104821568,-16.9969468157824,
0.));
#143278=CARTESIAN_POINT('Ctrl Pts',(-71.1356184691806,-17.0009738984935,
0.));
#143279=CARTESIAN_POINT('Ctrl Pts',(-71.1099603804786,-17.0049710758393,
0.));
#143280=CARTESIAN_POINT('Ctrl Pts',(-71.0843363214221,-17.0089383837437,
0.));
#143281=CARTESIAN_POINT('Ctrl Pts',(-71.0587463977268,-17.0128758583334,
0.));
#143282=CARTESIAN_POINT('Ctrl Pts',(-71.0331907154574,-17.0167835359419,
0.));
#143283=CARTESIAN_POINT('Ctrl Pts',(-71.0076693810301,-17.0206614531166,
0.));
#143284=CARTESIAN_POINT('Ctrl Pts',(-70.9821825012136,-17.0245096466229,
0.));
#143285=CARTESIAN_POINT('Ctrl Pts',(-70.956730183136,-17.0283281534392,
0.));
#143286=CARTESIAN_POINT('Ctrl Pts',(-70.9313125342876,-17.0321170107564,
0.));
#143287=CARTESIAN_POINT('Ctrl Pts',(-70.9059296625214,-17.0358762559786,
0.));
#143288=CARTESIAN_POINT('Ctrl Pts',(-70.8805816760501,-17.0396059267277,
0.));
#143289=CARTESIAN_POINT('Ctrl Pts',(-70.8552686834423,-17.0433060608474,
0.));
#143290=CARTESIAN_POINT('Ctrl Pts',(-70.8299907936334,-17.0469766964001,
0.));
#143291=CARTESIAN_POINT('Ctrl Pts',(-70.8047481159298,-17.0506178716661,
0.));
#143292=CARTESIAN_POINT('Ctrl Pts',(-70.7795407600127,-17.0542296251462,
0.));
#143293=CARTESIAN_POINT('Ctrl Pts',(-70.754368835938,-17.0578119955651,
0.));
#143294=CARTESIAN_POINT('Ctrl Pts',(-70.7292324541348,-17.0613650218788,
0.));
#143295=CARTESIAN_POINT('Ctrl Pts',(-70.7041317254127,-17.0648887432714,
0.));
#143296=CARTESIAN_POINT('Ctrl Pts',(-70.6790667609678,-17.0683831991532,
0.));
#143297=CARTESIAN_POINT('Ctrl Pts',(-70.6540376723839,-17.0718484291623,
0.));
#143298=CARTESIAN_POINT('Ctrl Pts',(-70.6290445716341,-17.0752844731679,
0.));
#143299=CARTESIAN_POINT('Ctrl Pts',(-70.6040875710762,-17.0786913712766,
0.));
#143300=CARTESIAN_POINT('Ctrl Pts',(-70.5791667834599,-17.0820691638314,
0.));
#143301=CARTESIAN_POINT('Ctrl Pts',(-70.5542823219346,-17.085417891409,
0.));
#143302=CARTESIAN_POINT('Ctrl Pts',(-70.5294343000516,-17.0887375948221,
0.));
#143303=CARTESIAN_POINT('Ctrl Pts',(-70.5046228317669,-17.0920283151217,
0.));
#143304=CARTESIAN_POINT('Ctrl Pts',(-70.4798480314364,-17.0952900936044,
0.));
#143305=CARTESIAN_POINT('Ctrl Pts',(-70.4551100138221,-17.098522971812,
0.));
#143306=CARTESIAN_POINT('Ctrl Pts',(-70.4304088940998,-17.1017269915289,
0.));
#143307=CARTESIAN_POINT('Ctrl Pts',(-70.4057447878621,-17.1049021947833,
0.));
#143308=CARTESIAN_POINT('Ctrl Pts',(-70.3811178111206,-17.1080486238499,
0.));
#143309=CARTESIAN_POINT('Ctrl Pts',(-70.356528080303,-17.111166321257,0.));
#143310=CARTESIAN_POINT('Ctrl Pts',(-70.3319757122576,-17.1142553297869,
0.));
#143311=CARTESIAN_POINT('Ctrl Pts',(-70.3074608242613,-17.1173156924733,
0.));
#143312=CARTESIAN_POINT('Ctrl Pts',(-70.2829835340239,-17.1203474526031,
0.));
#143313=CARTESIAN_POINT('Ctrl Pts',(-70.2585439596899,-17.1233506537176,
0.));
#143314=CARTESIAN_POINT('Ctrl Pts',(-70.2341422198362,-17.1263253396202,
0.));
#143315=CARTESIAN_POINT('Ctrl Pts',(-70.2097784334749,-17.1292715543779,
0.));
#143316=CARTESIAN_POINT('Ctrl Pts',(-70.1854527200636,-17.1321893423183,
0.));
#143317=CARTESIAN_POINT('Ctrl Pts',(-70.1611651995085,-17.1350787480313,
0.));
#143318=CARTESIAN_POINT('Ctrl Pts',(-70.1369159921686,-17.1379398163708,
0.));
#143319=CARTESIAN_POINT('Ctrl Pts',(-70.1127052188515,-17.1407725924615,
0.));
#143320=CARTESIAN_POINT('Ctrl Pts',(-70.0885330008169,-17.1435771217015,
0.));
#143321=CARTESIAN_POINT('Ctrl Pts',(-70.0643994597865,-17.1463534497592,
0.));
#143322=CARTESIAN_POINT('Ctrl Pts',(-70.040304717948,-17.1491016225748,
0.));
#143323=CARTESIAN_POINT('Ctrl Pts',(-70.0162488979586,-17.1518216863624,
0.));
#143324=CARTESIAN_POINT('Ctrl Pts',(-69.9922321229428,-17.1545136876161,
0.));
#143325=CARTESIAN_POINT('Ctrl Pts',(-69.9682545164942,-17.157177673114,
0.));
#143326=CARTESIAN_POINT('Ctrl Pts',(-69.9443162026865,-17.1598136899144,
0.));
#143327=CARTESIAN_POINT('Ctrl Pts',(-69.9204173060779,-17.1624217853577,
0.));
#143328=CARTESIAN_POINT('Ctrl Pts',(-69.8965579517147,-17.1650020070686,
0.));
#143329=CARTESIAN_POINT('Ctrl Pts',(-69.8727382651292,-17.1675544029621,
0.));
#143330=CARTESIAN_POINT('Ctrl Pts',(-69.8489583723417,-17.1700790212476,
0.));
#143331=CARTESIAN_POINT('Ctrl Pts',(-69.8252183998713,-17.1725759104254,
0.));
#143332=CARTESIAN_POINT('Ctrl Pts',(-69.8015184747404,-17.1750451192887,
0.));
#143333=CARTESIAN_POINT('Ctrl Pts',(-69.7778587244788,-17.1774866969256,
0.));
#143334=CARTESIAN_POINT('Ctrl Pts',(-69.7542392771216,-17.1799006927255,
0.));
#143335=CARTESIAN_POINT('Ctrl Pts',(-69.7306602612125,-17.1822871563834,
0.));
#143336=CARTESIAN_POINT('Ctrl Pts',(-69.7071218058149,-17.1846461378966,
0.));
#143337=CARTESIAN_POINT('Ctrl Pts',(-69.6836240405151,-17.1869776875663,
0.));
#143338=CARTESIAN_POINT('Ctrl Pts',(-69.6601670954277,-17.1892818560004,
0.));
#143339=CARTESIAN_POINT('Ctrl Pts',(-69.6367511011927,-17.1915586941198,
0.));
#143340=CARTESIAN_POINT('Ctrl Pts',(-69.6133761889787,-17.1938082531619,
0.));
#143341=CARTESIAN_POINT('Ctrl Pts',(-69.5900424904954,-17.1960305846787,
0.));
#143342=CARTESIAN_POINT('Ctrl Pts',(-69.5667501379984,-17.198225740538,
0.));
#143343=CARTESIAN_POINT('Ctrl Pts',(-69.5434992642932,-17.2003937729266,
0.));
#143344=CARTESIAN_POINT('Ctrl Pts',(-69.5202900027329,-17.2025347343568,
0.));
#143345=CARTESIAN_POINT('Ctrl Pts',(-69.497122487222,-17.2046486776697,
0.));
#143346=CARTESIAN_POINT('Ctrl Pts',(-69.4739968522271,-17.2067356560326,
0.));
#143347=CARTESIAN_POINT('Ctrl Pts',(-69.4509132327836,-17.208795722942,
0.));
#143348=CARTESIAN_POINT('Ctrl Pts',(-69.4278717644989,-17.2108289322258,
0.));
#143349=CARTESIAN_POINT('Ctrl Pts',(-69.4048725835516,-17.2128353380511,
0.));
#143350=CARTESIAN_POINT('Ctrl Pts',(-69.3819158266955,-17.2148149949261,
0.));
#143351=CARTESIAN_POINT('Ctrl Pts',(-69.359001631272,-17.2167679576991,
0.));
#143352=CARTESIAN_POINT('Ctrl Pts',(-69.3361301352149,-17.2186942815603,
0.));
#143353=CARTESIAN_POINT('Ctrl Pts',(-69.3133014770542,-17.2205940220455,
0.));
#143354=CARTESIAN_POINT('Ctrl Pts',(-69.2905157959141,-17.2224672350432,
0.));
#143355=CARTESIAN_POINT('Ctrl Pts',(-69.2677732315199,-17.2243139767963,
0.));
#143356=CARTESIAN_POINT('Ctrl Pts',(-69.2450739242092,-17.2261343039015,
0.));
#143357=CARTESIAN_POINT('Ctrl Pts',(-69.2224180149377,-17.2279282733119,
0.));
#143358=CARTESIAN_POINT('Ctrl Pts',(-69.1998056452837,-17.229695942341,
0.));
#143359=CARTESIAN_POINT('Ctrl Pts',(-69.1772369574462,-17.2314373686705,
0.));
#143360=CARTESIAN_POINT('Ctrl Pts',(-69.1547120942542,-17.2331526103511,
0.));
#143361=CARTESIAN_POINT('Ctrl Pts',(-69.1322311991759,-17.2348417258017,
0.));
#143362=CARTESIAN_POINT('Ctrl Pts',(-69.1097944163244,-17.2365047738125,
0.));
#143363=CARTESIAN_POINT('Ctrl Pts',(-69.0874018904598,-17.238141813549,
0.));
#143364=CARTESIAN_POINT('Ctrl Pts',(-69.0650537669859,-17.2397529045587,
0.));
#143365=CARTESIAN_POINT('Ctrl Pts',(-69.0427501919636,-17.2413381067722,
0.));
#143366=CARTESIAN_POINT('Ctrl Pts',(-69.0204913121226,-17.2428974805043,
0.));
#143367=CARTESIAN_POINT('Ctrl Pts',(-68.9982772748694,-17.2444310864585,
0.));
#143368=CARTESIAN_POINT('Ctrl Pts',(-68.9761082282922,-17.2459389857327,
0.));
#143369=CARTESIAN_POINT('Ctrl Pts',(-68.9539843211618,-17.2474212398275,
0.));
#143370=CARTESIAN_POINT('Ctrl Pts',(-68.9319057029407,-17.248877910643,
0.));
#143371=CARTESIAN_POINT('Ctrl Pts',(-68.9098725237868,-17.2503090604792,
0.));
#143372=CARTESIAN_POINT('Ctrl Pts',(-68.8878849345557,-17.2517147520376,
0.));
#143373=CARTESIAN_POINT('Ctrl Pts',(-68.8659430867977,-17.2530950484259,
0.));
#143374=CARTESIAN_POINT('Ctrl Pts',(-68.8440471327563,-17.2544500131627,
0.));
#143375=CARTESIAN_POINT('Ctrl Pts',(-68.8221972253954,-17.2557797101815,
0.));
#143376=CARTESIAN_POINT('Ctrl Pts',(-68.8003935184193,-17.2570842038385,
0.));
#143377=CARTESIAN_POINT('Ctrl Pts',(-68.7786361662876,-17.2583635589196,
0.));
#143378=CARTESIAN_POINT('Ctrl Pts',(-68.7569253242312,-17.2596178406545,
0.));
#143379=CARTESIAN_POINT('Ctrl Pts',(-68.7352611482519,-17.2608471147178,
0.));
#143380=CARTESIAN_POINT('Ctrl Pts',(-68.7136437951074,-17.2620514472176,
0.));
#143381=CARTESIAN_POINT('Ctrl Pts',(-68.6920734222932,-17.263230904689,
0.));
#143382=CARTESIAN_POINT('Ctrl Pts',(-68.6705501880263,-17.2643855540895,
0.));
#143383=CARTESIAN_POINT('Ctrl Pts',(-68.6490742512085,-17.2655154627935,
0.));
#143384=CARTESIAN_POINT('Ctrl Pts',(-68.6276457714757,-17.266620698609,
0.));
#143385=CARTESIAN_POINT('Ctrl Pts',(-68.606264909278,-17.2677013298061,
0.));
#143386=CARTESIAN_POINT('Ctrl Pts',(-68.5849318259449,-17.2687574251428,
0.));
#143387=CARTESIAN_POINT('Ctrl Pts',(-68.5636466837502,-17.2697890538956,
0.));
#143388=CARTESIAN_POINT('Ctrl Pts',(-68.5424096459746,-17.2707962858912,
0.));
#143389=CARTESIAN_POINT('Ctrl Pts',(-68.5212208767835,-17.2717791914538,
0.));
#143390=CARTESIAN_POINT('Ctrl Pts',(-68.5000805410896,-17.2727378413485,
0.));
#143391=CARTESIAN_POINT('Ctrl Pts',(-68.4789888044357,-17.2736723067366,
0.));
#143392=CARTESIAN_POINT('Ctrl Pts',(-68.4579458328208,-17.2745826591125,
0.));
#143393=CARTESIAN_POINT('Ctrl Pts',(-68.4369517926803,-17.2754689703001,
0.));
#143394=CARTESIAN_POINT('Ctrl Pts',(-68.4160068512781,-17.2763313126025,
0.));
#143395=CARTESIAN_POINT('Ctrl Pts',(-68.3951111770498,-17.2771697589387,
0.));
#143396=CARTESIAN_POINT('Ctrl Pts',(-68.374264939895,-17.2779843829605,
0.));
#143397=CARTESIAN_POINT('Ctrl Pts',(-68.353468311648,-17.2787752592475,
0.));
#143398=CARTESIAN_POINT('Ctrl Pts',(-68.3327214657533,-17.2795424631789,
0.));
#143399=CARTESIAN_POINT('Ctrl Pts',(-68.3120245763884,-17.2802860705807,
0.));
#143400=CARTESIAN_POINT('Ctrl Pts',(-68.2913778177258,-17.2810061574352,
0.));
#143401=CARTESIAN_POINT('Ctrl Pts',(-68.2707813631761,-17.2817027995838,
0.));
#143402=CARTESIAN_POINT('Ctrl Pts',(-68.250235384512,-17.2823760723886,
0.));
#143403=CARTESIAN_POINT('Ctrl Pts',(-68.2297400535339,-17.2830260513878,
0.));
#143404=CARTESIAN_POINT('Ctrl Pts',(-68.2092955440591,-17.2836528130825,
0.));
#143405=CARTESIAN_POINT('Ctrl Pts',(-68.1889020335418,-17.2842564355796,
0.));
#143406=CARTESIAN_POINT('Ctrl Pts',(-68.1685597054193,-17.2848369995283,
0.));
#143407=CARTESIAN_POINT('Ctrl Pts',(-68.1482687493176,-17.2853945882059,
0.));
#143408=CARTESIAN_POINT('Ctrl Pts',(-68.1280293561473,-17.2859292855694,
0.));
#143409=CARTESIAN_POINT('Ctrl Pts',(-68.1078417137865,-17.2864411745455,
0.));
#143410=CARTESIAN_POINT('Ctrl Pts',(-68.0877060033229,-17.2869303355438,
0.));
#143411=CARTESIAN_POINT('Ctrl Pts',(-68.0676223930469,-17.2873968440855,
0.));
#143412=CARTESIAN_POINT('Ctrl Pts',(-68.0475910442494,-17.2878407730981,
0.));
#143413=CARTESIAN_POINT('Ctrl Pts',(-68.027612122741,-17.2882621974737,
0.));
#143414=CARTESIAN_POINT('Ctrl Pts',(-68.007685808115,-17.28866119774,0.));
#143415=CARTESIAN_POINT('Ctrl Pts',(-67.9878123049132,-17.2890378644843,
0.));
#143416=CARTESIAN_POINT('Ctrl Pts',(-67.9679918502441,-17.2893923013852,
0.));
#143417=CARTESIAN_POINT('Ctrl Pts',(-67.9482246901517,-17.2897246158895,
0.));
#143418=CARTESIAN_POINT('Ctrl Pts',(-67.9285110571662,-17.2900349103956,
0.));
#143419=CARTESIAN_POINT('Ctrl Pts',(-67.908851149676,-17.2903232740717,
0.));
#143420=CARTESIAN_POINT('Ctrl Pts',(-67.8892451049871,-17.2905897724029,
0.));
#143421=CARTESIAN_POINT('Ctrl Pts',(-67.8696929979178,-17.2908344459816,
0.));
#143422=CARTESIAN_POINT('Ctrl Pts',(-67.8540944890057,-17.2910127431203,
0.));
#143423=CARTESIAN_POINT('Ctrl Pts',(-67.8424198971214,-17.2911366591419,
0.));
#143424=CARTESIAN_POINT('Ctrl Pts',(-67.8346476309106,-17.2912149114145,
0.));
#143425=CARTESIAN_POINT('Ctrl Pts',(-67.8307641965655,-17.2912529479484,
0.));
#143426=CARTESIAN_POINT('Ctrl Pts',(-73.778495580227,-10.343287191141,0.));
#143427=CARTESIAN_POINT('Ctrl Pts',(-73.778495580227,-10.343287191141,12.));
#143428=CARTESIAN_POINT('Ctrl Pts',(-73.7731377048058,-10.3449014384453,
0.));
#143429=CARTESIAN_POINT('Ctrl Pts',(-73.7731377048058,-10.3449014384453,
12.));
#143430=CARTESIAN_POINT('Ctrl Pts',(-73.7624245587789,-10.3481265449342,
0.));
#143431=CARTESIAN_POINT('Ctrl Pts',(-73.7624245587789,-10.3481265449342,
12.));
#143432=CARTESIAN_POINT('Ctrl Pts',(-73.7463626541854,-10.3529540403092,
0.));
#143433=CARTESIAN_POINT('Ctrl Pts',(-73.7463626541854,-10.3529540403092,
12.));
#143434=CARTESIAN_POINT('Ctrl Pts',(-73.7249624109173,-10.359370371262,
0.));
#143435=CARTESIAN_POINT('Ctrl Pts',(-73.7249624109173,-10.359370371262,
12.));
#143436=CARTESIAN_POINT('Ctrl Pts',(-73.6982381645206,-10.3673568984582,
0.));
#143437=CARTESIAN_POINT('Ctrl Pts',(-73.6982381645206,-10.3673568984582,
12.));
#143438=CARTESIAN_POINT('Ctrl Pts',(-73.6715399947839,-10.3753095356342,
0.));
#143439=CARTESIAN_POINT('Ctrl Pts',(-73.6715399947839,-10.3753095356342,
12.));
#143440=CARTESIAN_POINT('Ctrl Pts',(-73.6448679350696,-10.3832282820371,
0.));
#143441=CARTESIAN_POINT('Ctrl Pts',(-73.6448679350696,-10.3832282820371,
12.));
#143442=CARTESIAN_POINT('Ctrl Pts',(-73.6182220363156,-10.3911131417463,
0.));
#143443=CARTESIAN_POINT('Ctrl Pts',(-73.6182220363156,-10.3911131417463,
12.));
#143444=CARTESIAN_POINT('Ctrl Pts',(-73.5916023719713,-10.3989641265285,
0.));
#143445=CARTESIAN_POINT('Ctrl Pts',(-73.5916023719713,-10.3989641265285,
12.));
#143446=CARTESIAN_POINT('Ctrl Pts',(-73.5650090359839,-10.406781255551,
0.));
#143447=CARTESIAN_POINT('Ctrl Pts',(-73.5650090359839,-10.406781255551,
12.));
#143448=CARTESIAN_POINT('Ctrl Pts',(-73.5384421354543,-10.414564552681,
0.));
#143449=CARTESIAN_POINT('Ctrl Pts',(-73.5384421354543,-10.414564552681,
12.));
#143450=CARTESIAN_POINT('Ctrl Pts',(-73.5119017847575,-10.4223140444605,
0.));
#143451=CARTESIAN_POINT('Ctrl Pts',(-73.5119017847575,-10.4223140444605,
12.));
#143452=CARTESIAN_POINT('Ctrl Pts',(-73.485388099225,-10.430029757865,0.));
#143453=CARTESIAN_POINT('Ctrl Pts',(-73.485388099225,-10.430029757865,12.));
#143454=CARTESIAN_POINT('Ctrl Pts',(-73.4589011886197,-10.4377117180222,
0.));
#143455=CARTESIAN_POINT('Ctrl Pts',(-73.4589011886197,-10.4377117180222,
12.));
#143456=CARTESIAN_POINT('Ctrl Pts',(-73.4324411518554,-10.4453599463547,
0.));
#143457=CARTESIAN_POINT('Ctrl Pts',(-73.4324411518554,-10.4453599463547,
12.));
#143458=CARTESIAN_POINT('Ctrl Pts',(-73.4060080806686,-10.452974461845,
0.));
#143459=CARTESIAN_POINT('Ctrl Pts',(-73.4060080806686,-10.452974461845,
12.));
#143460=CARTESIAN_POINT('Ctrl Pts',(-73.37960206225,-10.4605552819397,0.));
#143461=CARTESIAN_POINT('Ctrl Pts',(-73.37960206225,-10.4605552819397,12.));
#143462=CARTESIAN_POINT('Ctrl Pts',(-73.3532231823659,-10.4681024236289,
0.));
#143463=CARTESIAN_POINT('Ctrl Pts',(-73.3532231823659,-10.4681024236289,
12.));
#143464=CARTESIAN_POINT('Ctrl Pts',(-73.3268715280575,-10.4756159043806,
0.));
#143465=CARTESIAN_POINT('Ctrl Pts',(-73.3268715280575,-10.4756159043806,
12.));
#143466=CARTESIAN_POINT('Ctrl Pts',(-73.3005471910583,-10.4830957433305,
0.));
#143467=CARTESIAN_POINT('Ctrl Pts',(-73.3005471910583,-10.4830957433305,
12.));
#143468=CARTESIAN_POINT('Ctrl Pts',(-73.2742502674304,-10.4905419611523,
0.));
#143469=CARTESIAN_POINT('Ctrl Pts',(-73.2742502674304,-10.4905419611523,
12.));
#143470=CARTESIAN_POINT('Ctrl Pts',(-73.2479808560189,-10.4979545795192,
0.));
#143471=CARTESIAN_POINT('Ctrl Pts',(-73.2479808560189,-10.4979545795192,
12.));
#143472=CARTESIAN_POINT('Ctrl Pts',(-73.2217390572562,-10.5053336206908,
0.));
#143473=CARTESIAN_POINT('Ctrl Pts',(-73.2217390572562,-10.5053336206908,
12.));
#143474=CARTESIAN_POINT('Ctrl Pts',(-73.1955249719048,-10.5126791070805,
0.));
#143475=CARTESIAN_POINT('Ctrl Pts',(-73.1955249719048,-10.5126791070805,
12.));
#143476=CARTESIAN_POINT('Ctrl Pts',(-73.1693386996138,-10.5199910607654,
0.));
#143477=CARTESIAN_POINT('Ctrl Pts',(-73.1693386996138,-10.5199910607654,
12.));
#143478=CARTESIAN_POINT('Ctrl Pts',(-73.1431803382711,-10.5272695032653,
0.));
#143479=CARTESIAN_POINT('Ctrl Pts',(-73.1431803382711,-10.5272695032653,
12.));
#143480=CARTESIAN_POINT('Ctrl Pts',(-73.1170499848039,-10.53451445581,0.));
#143481=CARTESIAN_POINT('Ctrl Pts',(-73.1170499848039,-10.53451445581,12.));
#143482=CARTESIAN_POINT('Ctrl Pts',(-73.0909477356474,-10.5417259395003,
0.));
#143483=CARTESIAN_POINT('Ctrl Pts',(-73.0909477356474,-10.5417259395003,
12.));
#143484=CARTESIAN_POINT('Ctrl Pts',(-73.0648736873434,-10.5489039755138,
0.));
#143485=CARTESIAN_POINT('Ctrl Pts',(-73.0648736873434,-10.5489039755138,
12.));
#143486=CARTESIAN_POINT('Ctrl Pts',(-73.0388279370834,-10.5560485852974,
0.));
#143487=CARTESIAN_POINT('Ctrl Pts',(-73.0388279370834,-10.5560485852974,
12.));
#143488=CARTESIAN_POINT('Ctrl Pts',(-73.0128105832621,-10.5631597907651,
0.));
#143489=CARTESIAN_POINT('Ctrl Pts',(-73.0128105832621,-10.5631597907651,
12.));
#143490=CARTESIAN_POINT('Ctrl Pts',(-72.9868217252283,-10.570237614205,
0.));
#143491=CARTESIAN_POINT('Ctrl Pts',(-72.9868217252283,-10.570237614205,
12.));
#143492=CARTESIAN_POINT('Ctrl Pts',(-72.9608614630534,-10.5772820781958,
0.));
#143493=CARTESIAN_POINT('Ctrl Pts',(-72.9608614630534,-10.5772820781958,
12.));
#143494=CARTESIAN_POINT('Ctrl Pts',(-72.9349298972822,-10.5842932055209,
0.));
#143495=CARTESIAN_POINT('Ctrl Pts',(-72.9349298972822,-10.5842932055209,
12.));
#143496=CARTESIAN_POINT('Ctrl Pts',(-72.9090271287083,-10.5912710190928,
0.));
#143497=CARTESIAN_POINT('Ctrl Pts',(-72.9090271287083,-10.5912710190928,
12.));
#143498=CARTESIAN_POINT('Ctrl Pts',(-72.8831532580845,-10.5982155418626,
0.));
#143499=CARTESIAN_POINT('Ctrl Pts',(-72.8831532580845,-10.5982155418626,
12.));
#143500=CARTESIAN_POINT('Ctrl Pts',(-72.8573083861337,-10.6051267968203,
0.));
#143501=CARTESIAN_POINT('Ctrl Pts',(-72.8573083861337,-10.6051267968203,
12.));
#143502=CARTESIAN_POINT('Ctrl Pts',(-72.8314926136881,-10.6120048070367,
0.));
#143503=CARTESIAN_POINT('Ctrl Pts',(-72.8314926136881,-10.6120048070367,
12.));
#143504=CARTESIAN_POINT('Ctrl Pts',(-72.8057060417887,-10.6188495956973,
0.));
#143505=CARTESIAN_POINT('Ctrl Pts',(-72.8057060417887,-10.6188495956973,
12.));
#143506=CARTESIAN_POINT('Ctrl Pts',(-72.7799487717911,-10.6256611861394,
0.));
#143507=CARTESIAN_POINT('Ctrl Pts',(-72.7799487717911,-10.6256611861394,
12.));
#143508=CARTESIAN_POINT('Ctrl Pts',(-72.7542209054812,-10.6324396018998,
0.));
#143509=CARTESIAN_POINT('Ctrl Pts',(-72.7542209054812,-10.6324396018998,
12.));
#143510=CARTESIAN_POINT('Ctrl Pts',(-72.7285225451293,-10.6391848667352,
0.));
#143511=CARTESIAN_POINT('Ctrl Pts',(-72.7285225451293,-10.6391848667352,
12.));
#143512=CARTESIAN_POINT('Ctrl Pts',(-72.7028537934317,-10.6458970045946,
0.));
#143513=CARTESIAN_POINT('Ctrl Pts',(-72.7028537934317,-10.6458970045946,
12.));
#143514=CARTESIAN_POINT('Ctrl Pts',(-72.6772147534752,-10.6525760396054,
0.));
#143515=CARTESIAN_POINT('Ctrl Pts',(-72.6772147534752,-10.6525760396054,
12.));
#143516=CARTESIAN_POINT('Ctrl Pts',(-72.651605528691,-10.659221996058,0.));
#143517=CARTESIAN_POINT('Ctrl Pts',(-72.651605528691,-10.659221996058,12.));
#143518=CARTESIAN_POINT('Ctrl Pts',(-72.6260262228065,-10.6658348983944,
0.));
#143519=CARTESIAN_POINT('Ctrl Pts',(-72.6260262228065,-10.6658348983944,
12.));
#143520=CARTESIAN_POINT('Ctrl Pts',(-72.6004769398019,-10.6724147711995,
0.));
#143521=CARTESIAN_POINT('Ctrl Pts',(-72.6004769398019,-10.6724147711995,
12.));
#143522=CARTESIAN_POINT('Ctrl Pts',(-72.5749577839415,-10.6789616392042,
0.));
#143523=CARTESIAN_POINT('Ctrl Pts',(-72.5749577839415,-10.6789616392042,
12.));
#143524=CARTESIAN_POINT('Ctrl Pts',(-72.5494688597961,-10.6854755272904,
0.));
#143525=CARTESIAN_POINT('Ctrl Pts',(-72.5494688597961,-10.6854755272904,
12.));
#143526=CARTESIAN_POINT('Ctrl Pts',(-72.5240102722664,-10.691956460499,
0.));
#143527=CARTESIAN_POINT('Ctrl Pts',(-72.5240102722664,-10.691956460499,
12.));
#143528=CARTESIAN_POINT('Ctrl Pts',(-72.4985821266023,-10.6984044640398,
0.));
#143529=CARTESIAN_POINT('Ctrl Pts',(-72.4985821266023,-10.6984044640398,
12.));
#143530=CARTESIAN_POINT('Ctrl Pts',(-72.4731845284227,-10.7048195633061,
0.));
#143531=CARTESIAN_POINT('Ctrl Pts',(-72.4731845284227,-10.7048195633061,
12.));
#143532=CARTESIAN_POINT('Ctrl Pts',(-72.4478175837156,-10.7112017838706,
0.));
#143533=CARTESIAN_POINT('Ctrl Pts',(-72.4478175837156,-10.7112017838706,
12.));
#143534=CARTESIAN_POINT('Ctrl Pts',(-72.4224813988347,-10.7175511514788,
0.));
#143535=CARTESIAN_POINT('Ctrl Pts',(-72.4224813988347,-10.7175511514788,
12.));
#143536=CARTESIAN_POINT('Ctrl Pts',(-72.3971760804933,-10.7238676920469,
0.));
#143537=CARTESIAN_POINT('Ctrl Pts',(-72.3971760804933,-10.7238676920469,
12.));
#143538=CARTESIAN_POINT('Ctrl Pts',(-72.3719017357571,-10.7301514316607,
0.));
#143539=CARTESIAN_POINT('Ctrl Pts',(-72.3719017357571,-10.7301514316607,
12.));
#143540=CARTESIAN_POINT('Ctrl Pts',(-72.3466584720318,-10.73640239658,0.));
#143541=CARTESIAN_POINT('Ctrl Pts',(-72.3466584720318,-10.73640239658,12.));
#143542=CARTESIAN_POINT('Ctrl Pts',(-72.3214463970641,-10.7426206132375,
0.));
#143543=CARTESIAN_POINT('Ctrl Pts',(-72.3214463970641,-10.7426206132375,
12.));
#143544=CARTESIAN_POINT('Ctrl Pts',(-72.2962656189556,-10.7488061082367,
0.));
#143545=CARTESIAN_POINT('Ctrl Pts',(-72.2962656189556,-10.7488061082367,
12.));
#143546=CARTESIAN_POINT('Ctrl Pts',(-72.2711162461681,-10.7549589083535,
0.));
#143547=CARTESIAN_POINT('Ctrl Pts',(-72.2711162461681,-10.7549589083535,
12.));
#143548=CARTESIAN_POINT('Ctrl Pts',(-72.2459983875296,-10.7610790405385,
0.));
#143549=CARTESIAN_POINT('Ctrl Pts',(-72.2459983875296,-10.7610790405385,
12.));
#143550=CARTESIAN_POINT('Ctrl Pts',(-72.2209121522366,-10.7671665319255,
0.));
#143551=CARTESIAN_POINT('Ctrl Pts',(-72.2209121522366,-10.7671665319255,
12.));
#143552=CARTESIAN_POINT('Ctrl Pts',(-72.1958576498558,-10.7732214098344,
0.));
#143553=CARTESIAN_POINT('Ctrl Pts',(-72.1958576498558,-10.7732214098344,
12.));
#143554=CARTESIAN_POINT('Ctrl Pts',(-72.1708349903305,-10.7792437017662,
0.));
#143555=CARTESIAN_POINT('Ctrl Pts',(-72.1708349903305,-10.7792437017662,
12.));
#143556=CARTESIAN_POINT('Ctrl Pts',(-72.1458442839834,-10.7852334354016,
0.));
#143557=CARTESIAN_POINT('Ctrl Pts',(-72.1458442839834,-10.7852334354016,
12.));
#143558=CARTESIAN_POINT('Ctrl Pts',(-72.1208856415171,-10.7911906386027,
0.));
#143559=CARTESIAN_POINT('Ctrl Pts',(-72.1208856415171,-10.7911906386027,
12.));
#143560=CARTESIAN_POINT('Ctrl Pts',(-72.0959591740114,-10.7971153394166,
0.));
#143561=CARTESIAN_POINT('Ctrl Pts',(-72.0959591740114,-10.7971153394166,
12.));
#143562=CARTESIAN_POINT('Ctrl Pts',(-72.0710649929202,-10.8030075660808,
0.));
#143563=CARTESIAN_POINT('Ctrl Pts',(-72.0710649929202,-10.8030075660808,
12.));
#143564=CARTESIAN_POINT('Ctrl Pts',(-72.0462032100815,-10.8088673470184,
0.));
#143565=CARTESIAN_POINT('Ctrl Pts',(-72.0462032100815,-10.8088673470184,
12.));
#143566=CARTESIAN_POINT('Ctrl Pts',(-72.0213739377223,-10.8146947108375,
0.));
#143567=CARTESIAN_POINT('Ctrl Pts',(-72.0213739377223,-10.8146947108375,
12.));
#143568=CARTESIAN_POINT('Ctrl Pts',(-71.9965772884619,-10.8204896863328,
0.));
#143569=CARTESIAN_POINT('Ctrl Pts',(-71.9965772884619,-10.8204896863328,
12.));
#143570=CARTESIAN_POINT('Ctrl Pts',(-71.9718133753127,-10.8262523024898,
0.));
#143571=CARTESIAN_POINT('Ctrl Pts',(-71.9718133753127,-10.8262523024898,
12.));
#143572=CARTESIAN_POINT('Ctrl Pts',(-71.9470823116785,-10.8319825884918,
0.));
#143573=CARTESIAN_POINT('Ctrl Pts',(-71.9470823116785,-10.8319825884918,
12.));
#143574=CARTESIAN_POINT('Ctrl Pts',(-71.9223842113625,-10.8376805737159,
0.));
#143575=CARTESIAN_POINT('Ctrl Pts',(-71.9223842113625,-10.8376805737159,
12.));
#143576=CARTESIAN_POINT('Ctrl Pts',(-71.8977191885725,-10.8433462877311,
0.));
#143577=CARTESIAN_POINT('Ctrl Pts',(-71.8977191885725,-10.8433462877311,
12.));
#143578=CARTESIAN_POINT('Ctrl Pts',(-71.8730873579224,-10.8489797602997,
0.));
#143579=CARTESIAN_POINT('Ctrl Pts',(-71.8730873579224,-10.8489797602997,
12.));
#143580=CARTESIAN_POINT('Ctrl Pts',(-71.8484888344339,-10.8545810213799,
0.));
#143581=CARTESIAN_POINT('Ctrl Pts',(-71.8484888344339,-10.8545810213799,
12.));
#143582=CARTESIAN_POINT('Ctrl Pts',(-71.8239237335331,-10.8601501011332,
0.));
#143583=CARTESIAN_POINT('Ctrl Pts',(-71.8239237335331,-10.8601501011332,
12.));
#143584=CARTESIAN_POINT('Ctrl Pts',(-71.7993921710564,-10.865687029922,
0.));
#143585=CARTESIAN_POINT('Ctrl Pts',(-71.7993921710564,-10.865687029922,
12.));
#143586=CARTESIAN_POINT('Ctrl Pts',(-71.7748942632593,-10.8711918383073,
0.));
#143587=CARTESIAN_POINT('Ctrl Pts',(-71.7748942632593,-10.8711918383073,
12.));
#143588=CARTESIAN_POINT('Ctrl Pts',(-71.7504301268181,-10.8766645570497,
0.));
#143589=CARTESIAN_POINT('Ctrl Pts',(-71.7504301268181,-10.8766645570497,
12.));
#143590=CARTESIAN_POINT('Ctrl Pts',(-71.7259998788328,-10.882105217112,
0.));
#143591=CARTESIAN_POINT('Ctrl Pts',(-71.7259998788328,-10.882105217112,
12.));
#143592=CARTESIAN_POINT('Ctrl Pts',(-71.7016036368236,-10.8875138496671,
0.));
#143593=CARTESIAN_POINT('Ctrl Pts',(-71.7016036368236,-10.8875138496671,
12.));
#143594=CARTESIAN_POINT('Ctrl Pts',(-71.6772415187364,-10.8928904860964,
0.));
#143595=CARTESIAN_POINT('Ctrl Pts',(-71.6772415187364,-10.8928904860964,
12.));
#143596=CARTESIAN_POINT('Ctrl Pts',(-71.6529136429504,-10.8982351579871,
0.));
#143597=CARTESIAN_POINT('Ctrl Pts',(-71.6529136429504,-10.8982351579871,
12.));
#143598=CARTESIAN_POINT('Ctrl Pts',(-71.6286201282812,-10.9035478971328,
0.));
#143599=CARTESIAN_POINT('Ctrl Pts',(-71.6286201282812,-10.9035478971328,
12.));
#143600=CARTESIAN_POINT('Ctrl Pts',(-71.6043610939835,-10.9088287355365,
0.));
#143601=CARTESIAN_POINT('Ctrl Pts',(-71.6043610939835,-10.9088287355365,
12.));
#143602=CARTESIAN_POINT('Ctrl Pts',(-71.5801366597488,-10.914077705417,
0.));
#143603=CARTESIAN_POINT('Ctrl Pts',(-71.5801366597488,-10.914077705417,
12.));
#143604=CARTESIAN_POINT('Ctrl Pts',(-71.5559469457091,-10.91929483921,0.));
#143605=CARTESIAN_POINT('Ctrl Pts',(-71.5559469457091,-10.91929483921,12.));
#143606=CARTESIAN_POINT('Ctrl Pts',(-71.5317920724459,-10.9244801695642,
0.));
#143607=CARTESIAN_POINT('Ctrl Pts',(-71.5317920724459,-10.9244801695642,
12.));
#143608=CARTESIAN_POINT('Ctrl Pts',(-71.5076721609937,-10.9296337293424,
0.));
#143609=CARTESIAN_POINT('Ctrl Pts',(-71.5076721609937,-10.9296337293424,
12.));
#143610=CARTESIAN_POINT('Ctrl Pts',(-71.4835873328423,-10.9347555516235,
0.));
#143611=CARTESIAN_POINT('Ctrl Pts',(-71.4835873328423,-10.9347555516235,
12.));
#143612=CARTESIAN_POINT('Ctrl Pts',(-71.4595377099351,-10.9398456697095,
0.));
#143613=CARTESIAN_POINT('Ctrl Pts',(-71.4595377099351,-10.9398456697095,
12.));
#143614=CARTESIAN_POINT('Ctrl Pts',(-71.435523414672,-10.944904117127,0.));
#143615=CARTESIAN_POINT('Ctrl Pts',(-71.435523414672,-10.944904117127,12.));
#143616=CARTESIAN_POINT('Ctrl Pts',(-71.4115445699194,-10.9499309276236,
0.));
#143617=CARTESIAN_POINT('Ctrl Pts',(-71.4115445699194,-10.9499309276236,
12.));
#143618=CARTESIAN_POINT('Ctrl Pts',(-71.3876012990138,-10.954926135169,
0.));
#143619=CARTESIAN_POINT('Ctrl Pts',(-71.3876012990138,-10.954926135169,
12.));
#143620=CARTESIAN_POINT('Ctrl Pts',(-71.3636937257649,-10.9598897739564,
0.));
#143621=CARTESIAN_POINT('Ctrl Pts',(-71.3636937257649,-10.9598897739564,
12.));
#143622=CARTESIAN_POINT('Ctrl Pts',(-71.339821974454,-10.9648218784098,
0.));
#143623=CARTESIAN_POINT('Ctrl Pts',(-71.339821974454,-10.9648218784098,
12.));
#143624=CARTESIAN_POINT('Ctrl Pts',(-71.3159861698358,-10.969722483186,
0.));
#143625=CARTESIAN_POINT('Ctrl Pts',(-71.3159861698358,-10.969722483186,
12.));
#143626=CARTESIAN_POINT('Ctrl Pts',(-71.2921864371491,-10.9745916231709,
0.));
#143627=CARTESIAN_POINT('Ctrl Pts',(-71.2921864371491,-10.9745916231709,
12.));
#143628=CARTESIAN_POINT('Ctrl Pts',(-71.2684229021207,-10.9794293334805,
0.));
#143629=CARTESIAN_POINT('Ctrl Pts',(-71.2684229021207,-10.9794293334805,
12.));
#143630=CARTESIAN_POINT('Ctrl Pts',(-71.2446956909687,-10.9842356494627,
0.));
#143631=CARTESIAN_POINT('Ctrl Pts',(-71.2446956909687,-10.9842356494627,
12.));
#143632=CARTESIAN_POINT('Ctrl Pts',(-71.2210049304014,-10.9890106067039,
0.));
#143633=CARTESIAN_POINT('Ctrl Pts',(-71.2210049304014,-10.9890106067039,
12.));
#143634=CARTESIAN_POINT('Ctrl Pts',(-71.1973507476191,-10.993754241032,
0.));
#143635=CARTESIAN_POINT('Ctrl Pts',(-71.1973507476191,-10.993754241032,
12.));
#143636=CARTESIAN_POINT('Ctrl Pts',(-71.1737332703248,-10.9984665885127,
0.));
#143637=CARTESIAN_POINT('Ctrl Pts',(-71.1737332703248,-10.9984665885127,
12.));
#143638=CARTESIAN_POINT('Ctrl Pts',(-71.1501526267286,-11.0031476854502,
0.));
#143639=CARTESIAN_POINT('Ctrl Pts',(-71.1501526267286,-11.0031476854502,
12.));
#143640=CARTESIAN_POINT('Ctrl Pts',(-71.1266089455517,-11.0077975683895,
0.));
#143641=CARTESIAN_POINT('Ctrl Pts',(-71.1266089455517,-11.0077975683895,
12.));
#143642=CARTESIAN_POINT('Ctrl Pts',(-71.1031023560249,-11.0124162741224,
0.));
#143643=CARTESIAN_POINT('Ctrl Pts',(-71.1031023560249,-11.0124162741224,
12.));
#143644=CARTESIAN_POINT('Ctrl Pts',(-71.0796329878907,-11.0170038396915,
0.));
#143645=CARTESIAN_POINT('Ctrl Pts',(-71.0796329878907,-11.0170038396915,
12.));
#143646=CARTESIAN_POINT('Ctrl Pts',(-71.0562009714136,-11.0215603023856,
0.));
#143647=CARTESIAN_POINT('Ctrl Pts',(-71.0562009714136,-11.0215603023856,
12.));
#143648=CARTESIAN_POINT('Ctrl Pts',(-71.0328064373856,-11.0260856997415,
0.));
#143649=CARTESIAN_POINT('Ctrl Pts',(-71.0328064373856,-11.0260856997415,
12.));
#143650=CARTESIAN_POINT('Ctrl Pts',(-71.0094495171292,-11.0305800695456,
0.));
#143651=CARTESIAN_POINT('Ctrl Pts',(-71.0094495171292,-11.0305800695456,
12.));
#143652=CARTESIAN_POINT('Ctrl Pts',(-70.986130342497,-11.0350434498405,
0.));
#143653=CARTESIAN_POINT('Ctrl Pts',(-70.986130342497,-11.0350434498405,
12.));
#143654=CARTESIAN_POINT('Ctrl Pts',(-70.9628490458748,-11.0394758789285,
0.));
#143655=CARTESIAN_POINT('Ctrl Pts',(-70.9628490458748,-11.0394758789285,
12.));
#143656=CARTESIAN_POINT('Ctrl Pts',(-70.9396057601924,-11.0438773953681,
0.));
#143657=CARTESIAN_POINT('Ctrl Pts',(-70.9396057601924,-11.0438773953681,
12.));
#143658=CARTESIAN_POINT('Ctrl Pts',(-70.916400618927,-11.048248037975,0.));
#143659=CARTESIAN_POINT('Ctrl Pts',(-70.916400618927,-11.048248037975,12.));
#143660=CARTESIAN_POINT('Ctrl Pts',(-70.8932337561087,-11.0525878458243,
0.));
#143661=CARTESIAN_POINT('Ctrl Pts',(-70.8932337561087,-11.0525878458243,
12.));
#143662=CARTESIAN_POINT('Ctrl Pts',(-70.8701053063186,-11.0568968582569,
0.));
#143663=CARTESIAN_POINT('Ctrl Pts',(-70.8701053063186,-11.0568968582569,
12.));
#143664=CARTESIAN_POINT('Ctrl Pts',(-70.8470154046919,-11.0611751148835,
0.));
#143665=CARTESIAN_POINT('Ctrl Pts',(-70.8470154046919,-11.0611751148835,
12.));
#143666=CARTESIAN_POINT('Ctrl Pts',(-70.8239641869299,-11.0654226555802,
0.));
#143667=CARTESIAN_POINT('Ctrl Pts',(-70.8239641869299,-11.0654226555802,
12.));
#143668=CARTESIAN_POINT('Ctrl Pts',(-70.8009517893057,-11.0696395204909,
0.));
#143669=CARTESIAN_POINT('Ctrl Pts',(-70.8009517893057,-11.0696395204909,
12.));
#143670=CARTESIAN_POINT('Ctrl Pts',(-70.7779783486677,-11.073825750029,
0.));
#143671=CARTESIAN_POINT('Ctrl Pts',(-70.7779783486677,-11.073825750029,
12.));
#143672=CARTESIAN_POINT('Ctrl Pts',(-70.7550440024384,-11.0779813848846,
0.));
#143673=CARTESIAN_POINT('Ctrl Pts',(-70.7550440024384,-11.0779813848846,
12.));
#143674=CARTESIAN_POINT('Ctrl Pts',(-70.732148888618,-11.0821064660269,
0.));
#143675=CARTESIAN_POINT('Ctrl Pts',(-70.732148888618,-11.0821064660269,
12.));
#143676=CARTESIAN_POINT('Ctrl Pts',(-70.7092931457954,-11.0862010347016,
0.));
#143677=CARTESIAN_POINT('Ctrl Pts',(-70.7092931457954,-11.0862010347016,
12.));
#143678=CARTESIAN_POINT('Ctrl Pts',(-70.6864769131546,-11.0902651324323,
0.));
#143679=CARTESIAN_POINT('Ctrl Pts',(-70.6864769131546,-11.0902651324323,
12.));
#143680=CARTESIAN_POINT('Ctrl Pts',(-70.6637003304785,-11.0942988010233,
0.));
#143681=CARTESIAN_POINT('Ctrl Pts',(-70.6637003304785,-11.0942988010233,
12.));
#143682=CARTESIAN_POINT('Ctrl Pts',(-70.6409635381482,-11.0983020825667,
0.));
#143683=CARTESIAN_POINT('Ctrl Pts',(-70.6409635381482,-11.0983020825667,
12.));
#143684=CARTESIAN_POINT('Ctrl Pts',(-70.6182666771481,-11.1022750194445,
0.));
#143685=CARTESIAN_POINT('Ctrl Pts',(-70.6182666771481,-11.1022750194445,
12.));
#143686=CARTESIAN_POINT('Ctrl Pts',(-70.5956098890773,-11.1062176543262,
0.));
#143687=CARTESIAN_POINT('Ctrl Pts',(-70.5956098890773,-11.1062176543262,
12.));
#143688=CARTESIAN_POINT('Ctrl Pts',(-70.5729933161546,-11.1101300301701,
0.));
#143689=CARTESIAN_POINT('Ctrl Pts',(-70.5729933161546,-11.1101300301701,
12.));
#143690=CARTESIAN_POINT('Ctrl Pts',(-70.5504171012234,-11.1140121902271,
0.));
#143691=CARTESIAN_POINT('Ctrl Pts',(-70.5504171012234,-11.1140121902271,
12.));
#143692=CARTESIAN_POINT('Ctrl Pts',(-70.5278813877494,-11.1178641780476,
0.));
#143693=CARTESIAN_POINT('Ctrl Pts',(-70.5278813877494,-11.1178641780476,
12.));
#143694=CARTESIAN_POINT('Ctrl Pts',(-70.505386319828,-11.1216860374826,
0.));
#143695=CARTESIAN_POINT('Ctrl Pts',(-70.505386319828,-11.1216860374826,
12.));
#143696=CARTESIAN_POINT('Ctrl Pts',(-70.4829320421957,-11.1254778126821,
0.));
#143697=CARTESIAN_POINT('Ctrl Pts',(-70.4829320421957,-11.1254778126821,
12.));
#143698=CARTESIAN_POINT('Ctrl Pts',(-70.4605187002354,-11.1292395480974,
0.));
#143699=CARTESIAN_POINT('Ctrl Pts',(-70.4605187002354,-11.1292395480974,
12.));
#143700=CARTESIAN_POINT('Ctrl Pts',(-70.4381464399819,-11.1329712884846,
0.));
#143701=CARTESIAN_POINT('Ctrl Pts',(-70.4381464399819,-11.1329712884846,
12.));
#143702=CARTESIAN_POINT('Ctrl Pts',(-70.4158154081205,-11.1366730789125,
0.));
#143703=CARTESIAN_POINT('Ctrl Pts',(-70.4158154081205,-11.1366730789125,
12.));
#143704=CARTESIAN_POINT('Ctrl Pts',(-70.393525751996,-11.1403449647625,
0.));
#143705=CARTESIAN_POINT('Ctrl Pts',(-70.393525751996,-11.1403449647625,
12.));
#143706=CARTESIAN_POINT('Ctrl Pts',(-70.3712776196223,-11.143986991727,
0.));
#143707=CARTESIAN_POINT('Ctrl Pts',(-70.3712776196223,-11.143986991727,
12.));
#143708=CARTESIAN_POINT('Ctrl Pts',(-70.349071159688,-11.1475992058124,
0.));
#143709=CARTESIAN_POINT('Ctrl Pts',(-70.349071159688,-11.1475992058124,
12.));
#143710=CARTESIAN_POINT('Ctrl Pts',(-70.326906521559,-11.1511816533421,
0.));
#143711=CARTESIAN_POINT('Ctrl Pts',(-70.326906521559,-11.1511816533421,
12.));
#143712=CARTESIAN_POINT('Ctrl Pts',(-70.3047838552756,-11.1547343809646,
0.));
#143713=CARTESIAN_POINT('Ctrl Pts',(-70.3047838552756,-11.1547343809646,
12.));
#143714=CARTESIAN_POINT('Ctrl Pts',(-70.2827033115662,-11.158257435652,
0.));
#143715=CARTESIAN_POINT('Ctrl Pts',(-70.2827033115662,-11.158257435652,
12.));
#143716=CARTESIAN_POINT('Ctrl Pts',(-70.260665041859,-11.1617508647016,
0.));
#143717=CARTESIAN_POINT('Ctrl Pts',(-70.260665041859,-11.1617508647016,
12.));
#143718=CARTESIAN_POINT('Ctrl Pts',(-70.2386691982902,-11.1652147157383,
0.));
#143719=CARTESIAN_POINT('Ctrl Pts',(-70.2386691982902,-11.1652147157383,
12.));
#143720=CARTESIAN_POINT('Ctrl Pts',(-70.2167159337094,-11.168649036721,
0.));
#143721=CARTESIAN_POINT('Ctrl Pts',(-70.2167159337094,-11.168649036721,
12.));
#143722=CARTESIAN_POINT('Ctrl Pts',(-70.1948054016816,-11.1720538759499,
0.));
#143723=CARTESIAN_POINT('Ctrl Pts',(-70.1948054016816,-11.1720538759499,
12.));
#143724=CARTESIAN_POINT('Ctrl Pts',(-70.1729377564954,-11.1754292820631,
0.));
#143725=CARTESIAN_POINT('Ctrl Pts',(-70.1729377564954,-11.1754292820631,
12.));
#143726=CARTESIAN_POINT('Ctrl Pts',(-70.1511131531672,-11.1787753040363,
0.));
#143727=CARTESIAN_POINT('Ctrl Pts',(-70.1511131531672,-11.1787753040363,
12.));
#143728=CARTESIAN_POINT('Ctrl Pts',(-70.1293317474432,-11.1820919911846,
0.));
#143729=CARTESIAN_POINT('Ctrl Pts',(-70.1293317474432,-11.1820919911846,
12.));
#143730=CARTESIAN_POINT('Ctrl Pts',(-70.1075936957973,-11.185379393167,
0.));
#143731=CARTESIAN_POINT('Ctrl Pts',(-70.1075936957973,-11.185379393167,
12.));
#143732=CARTESIAN_POINT('Ctrl Pts',(-70.0858991554295,-11.1886375599916,
0.));
#143733=CARTESIAN_POINT('Ctrl Pts',(-70.0858991554295,-11.1886375599916,
12.));
#143734=CARTESIAN_POINT('Ctrl Pts',(-70.0642482842942,-11.1918665420168,
0.));
#143735=CARTESIAN_POINT('Ctrl Pts',(-70.0642482842942,-11.1918665420168,
12.));
#143736=CARTESIAN_POINT('Ctrl Pts',(-70.0426412411194,-11.1950663899578,
0.));
#143737=CARTESIAN_POINT('Ctrl Pts',(-70.0426412411194,-11.1950663899578,
12.));
#143738=CARTESIAN_POINT('Ctrl Pts',(-70.0210781854236,-11.1982371548918,
0.));
#143739=CARTESIAN_POINT('Ctrl Pts',(-70.0210781854236,-11.1982371548918,
12.));
#143740=CARTESIAN_POINT('Ctrl Pts',(-69.9995592775322,-11.2013788882711,
0.));
#143741=CARTESIAN_POINT('Ctrl Pts',(-69.9995592775322,-11.2013788882711,
12.));
#143742=CARTESIAN_POINT('Ctrl Pts',(-69.9780846785771,-11.2044916419239,
0.));
#143743=CARTESIAN_POINT('Ctrl Pts',(-69.9780846785771,-11.2044916419239,
12.));
#143744=CARTESIAN_POINT('Ctrl Pts',(-69.9566545504813,-11.2075754680445,
0.));
#143745=CARTESIAN_POINT('Ctrl Pts',(-69.9566545504813,-11.2075754680445,
12.));
#143746=CARTESIAN_POINT('Ctrl Pts',(-69.9352690559399,-11.2106304191881,
0.));
#143747=CARTESIAN_POINT('Ctrl Pts',(-69.9352690559399,-11.2106304191881,
12.));
#143748=CARTESIAN_POINT('Ctrl Pts',(-69.9139283584036,-11.2136565482679,
0.));
#143749=CARTESIAN_POINT('Ctrl Pts',(-69.9139283584036,-11.2136565482679,
12.));
#143750=CARTESIAN_POINT('Ctrl Pts',(-69.8926326220414,-11.2166539085527,
0.));
#143751=CARTESIAN_POINT('Ctrl Pts',(-69.8926326220414,-11.2166539085527,
12.));
#143752=CARTESIAN_POINT('Ctrl Pts',(-69.8713820117918,-11.2196225536794,
0.));
#143753=CARTESIAN_POINT('Ctrl Pts',(-69.8713820117918,-11.2196225536794,
12.));
#143754=CARTESIAN_POINT('Ctrl Pts',(-69.8501766934445,-11.2225625376739,
0.));
#143755=CARTESIAN_POINT('Ctrl Pts',(-69.8501766934445,-11.2225625376739,
12.));
#143756=CARTESIAN_POINT('Ctrl Pts',(-69.8290168337076,-11.225473914972,
0.));
#143757=CARTESIAN_POINT('Ctrl Pts',(-69.8290168337076,-11.225473914972,
12.));
#143758=CARTESIAN_POINT('Ctrl Pts',(-69.8079026002753,-11.2283567404434,
0.));
#143759=CARTESIAN_POINT('Ctrl Pts',(-69.8079026002753,-11.2283567404434,
12.));
#143760=CARTESIAN_POINT('Ctrl Pts',(-69.7868341618927,-11.2312110694183,
0.));
#143761=CARTESIAN_POINT('Ctrl Pts',(-69.7868341618927,-11.2312110694183,
12.));
#143762=CARTESIAN_POINT('Ctrl Pts',(-69.7658116882298,-11.2340369576452,
0.));
#143763=CARTESIAN_POINT('Ctrl Pts',(-69.7658116882298,-11.2340369576452,
12.));
#143764=CARTESIAN_POINT('Ctrl Pts',(-69.7448353497394,-11.236834461247,
0.));
#143765=CARTESIAN_POINT('Ctrl Pts',(-69.7448353497394,-11.236834461247,
12.));
#143766=CARTESIAN_POINT('Ctrl Pts',(-69.7239053175362,-11.2396036366861,
0.));
#143767=CARTESIAN_POINT('Ctrl Pts',(-69.7239053175362,-11.2396036366861,
12.));
#143768=CARTESIAN_POINT('Ctrl Pts',(-69.7030217632187,-11.242344540717,
0.));
#143769=CARTESIAN_POINT('Ctrl Pts',(-69.7030217632187,-11.242344540717,
12.));
#143770=CARTESIAN_POINT('Ctrl Pts',(-69.6821848588492,-11.2450572303847,
0.));
#143771=CARTESIAN_POINT('Ctrl Pts',(-69.6821848588492,-11.2450572303847,
12.));
#143772=CARTESIAN_POINT('Ctrl Pts',(-69.6613947773563,-11.247741763139,
0.));
#143773=CARTESIAN_POINT('Ctrl Pts',(-69.6613947773563,-11.247741763139,
12.));
#143774=CARTESIAN_POINT('Ctrl Pts',(-69.6406516928902,-11.2503981969413,
0.));
#143775=CARTESIAN_POINT('Ctrl Pts',(-69.6406516928902,-11.2503981969413,
12.));
#143776=CARTESIAN_POINT('Ctrl Pts',(-69.6199557811231,-11.2530265903555,
0.));
#143777=CARTESIAN_POINT('Ctrl Pts',(-69.6199557811231,-11.2530265903555,
12.));
#143778=CARTESIAN_POINT('Ctrl Pts',(-69.5993072197355,-11.255627002701,
0.));
#143779=CARTESIAN_POINT('Ctrl Pts',(-69.5993072197355,-11.255627002701,
12.));
#143780=CARTESIAN_POINT('Ctrl Pts',(-69.5787061880815,-11.2581994939534,
0.));
#143781=CARTESIAN_POINT('Ctrl Pts',(-69.5787061880815,-11.2581994939534,
12.));
#143782=CARTESIAN_POINT('Ctrl Pts',(-69.5581528662846,-11.2607441244698,
0.));
#143783=CARTESIAN_POINT('Ctrl Pts',(-69.5581528662846,-11.2607441244698,
12.));
#143784=CARTESIAN_POINT('Ctrl Pts',(-69.5376474344768,-11.2632609547629,
0.));
#143785=CARTESIAN_POINT('Ctrl Pts',(-69.5376474344768,-11.2632609547629,
12.));
#143786=CARTESIAN_POINT('Ctrl Pts',(-69.5171900720188,-11.265750045272,
0.));
#143787=CARTESIAN_POINT('Ctrl Pts',(-69.5171900720188,-11.265750045272,
12.));
#143788=CARTESIAN_POINT('Ctrl Pts',(-69.4967809565978,-11.2682114561015,
0.));
#143789=CARTESIAN_POINT('Ctrl Pts',(-69.4967809565978,-11.2682114561015,
12.));
#143790=CARTESIAN_POINT('Ctrl Pts',(-69.4764202659443,-11.2706452475287,
0.));
#143791=CARTESIAN_POINT('Ctrl Pts',(-69.4764202659443,-11.2706452475287,
12.));
#143792=CARTESIAN_POINT('Ctrl Pts',(-69.4561081798815,-11.2730514806143,
0.));
#143793=CARTESIAN_POINT('Ctrl Pts',(-69.4561081798815,-11.2730514806143,
12.));
#143794=CARTESIAN_POINT('Ctrl Pts',(-69.4358448819957,-11.2754302177019,
0.));
#143795=CARTESIAN_POINT('Ctrl Pts',(-69.4358448819957,-11.2754302177019,
12.));
#143796=CARTESIAN_POINT('Ctrl Pts',(-69.4156305620554,-11.2777815231462,
0.));
#143797=CARTESIAN_POINT('Ctrl Pts',(-69.4156305620554,-11.2777815231462,
12.));
#143798=CARTESIAN_POINT('Ctrl Pts',(-69.395465416223,-11.2801054633807,
0.));
#143799=CARTESIAN_POINT('Ctrl Pts',(-69.395465416223,-11.2801054633807,
12.));
#143800=CARTESIAN_POINT('Ctrl Pts',(-69.375349642,-11.2824021054038,0.));
#143801=CARTESIAN_POINT('Ctrl Pts',(-69.375349642,-11.2824021054038,12.));
#143802=CARTESIAN_POINT('Ctrl Pts',(-69.3552834337771,-11.2846715154521,
0.));
#143803=CARTESIAN_POINT('Ctrl Pts',(-69.3552834337771,-11.2846715154521,
12.));
#143804=CARTESIAN_POINT('Ctrl Pts',(-69.3352669789611,-11.2869137578463,
0.));
#143805=CARTESIAN_POINT('Ctrl Pts',(-69.3352669789611,-11.2869137578463,
12.));
#143806=CARTESIAN_POINT('Ctrl Pts',(-69.315300451784,-11.2891288931528,
0.));
#143807=CARTESIAN_POINT('Ctrl Pts',(-69.315300451784,-11.2891288931528,
12.));
#143808=CARTESIAN_POINT('Ctrl Pts',(-69.2953840192792,-11.2913169799642,
0.));
#143809=CARTESIAN_POINT('Ctrl Pts',(-69.2953840192792,-11.2913169799642,
12.));
#143810=CARTESIAN_POINT('Ctrl Pts',(-69.2755178531534,-11.2934780784361,
0.));
#143811=CARTESIAN_POINT('Ctrl Pts',(-69.2755178531534,-11.2934780784361,
12.));
#143812=CARTESIAN_POINT('Ctrl Pts',(-69.255702139335,-11.2956122531375,
0.));
#143813=CARTESIAN_POINT('Ctrl Pts',(-69.255702139335,-11.2956122531375,
12.));
#143814=CARTESIAN_POINT('Ctrl Pts',(-69.2359370894828,-11.2977195764836,
0.));
#143815=CARTESIAN_POINT('Ctrl Pts',(-69.2359370894828,-11.2977195764836,
12.));
#143816=CARTESIAN_POINT('Ctrl Pts',(-69.216222948839,-11.2998001310934,
0.));
#143817=CARTESIAN_POINT('Ctrl Pts',(-69.216222948839,-11.2998001310934,
12.));
#143818=CARTESIAN_POINT('Ctrl Pts',(-69.1965599718761,-11.3018540025605,
0.));
#143819=CARTESIAN_POINT('Ctrl Pts',(-69.1965599718761,-11.3018540025605,
12.));
#143820=CARTESIAN_POINT('Ctrl Pts',(-69.1769483991639,-11.3038812726275,
0.));
#143821=CARTESIAN_POINT('Ctrl Pts',(-69.1769483991639,-11.3038812726275,
12.));
#143822=CARTESIAN_POINT('Ctrl Pts',(-69.1573884361076,-11.3058820128323,
0.));
#143823=CARTESIAN_POINT('Ctrl Pts',(-69.1573884361076,-11.3058820128323,
12.));
#143824=CARTESIAN_POINT('Ctrl Pts',(-69.137880225198,-11.3078562764442,
0.));
#143825=CARTESIAN_POINT('Ctrl Pts',(-69.137880225198,-11.3078562764442,
12.));
#143826=CARTESIAN_POINT('Ctrl Pts',(-69.1184238445065,-11.3098040973799,
0.));
#143827=CARTESIAN_POINT('Ctrl Pts',(-69.1184238445065,-11.3098040973799,
12.));
#143828=CARTESIAN_POINT('Ctrl Pts',(-69.1029002322497,-11.3113412156742,
0.));
#143829=CARTESIAN_POINT('Ctrl Pts',(-69.1029002322497,-11.3113412156742,
12.));
#143830=CARTESIAN_POINT('Ctrl Pts',(-69.0912808657051,-11.3124821678849,
0.));
#143831=CARTESIAN_POINT('Ctrl Pts',(-69.0912808657051,-11.3124821678849,
12.));
#143832=CARTESIAN_POINT('Ctrl Pts',(-69.0835449954486,-11.3132375200184,
0.));
#143833=CARTESIAN_POINT('Ctrl Pts',(-69.0835449954486,-11.3132375200184,
12.));
#143834=CARTESIAN_POINT('Ctrl Pts',(-69.079679653846,-11.3136138754165,
0.));
#143835=CARTESIAN_POINT('Ctrl Pts',(-69.079679653846,-11.3136138754165,
12.));
#143836=CARTESIAN_POINT('',(-69.079679653846,-11.3136138754165,12.));
#143837=CARTESIAN_POINT('Ctrl Pts',(-69.079679653846,-11.3136138754165,
12.));
#143838=CARTESIAN_POINT('Ctrl Pts',(-69.0835449954486,-11.3132375200184,
12.));
#143839=CARTESIAN_POINT('Ctrl Pts',(-69.0912808657051,-11.3124821678849,
12.));
#143840=CARTESIAN_POINT('Ctrl Pts',(-69.1029002322497,-11.3113412156742,
12.));
#143841=CARTESIAN_POINT('Ctrl Pts',(-69.1184238445065,-11.3098040973799,
12.));
#143842=CARTESIAN_POINT('Ctrl Pts',(-69.137880225198,-11.3078562764442,
12.));
#143843=CARTESIAN_POINT('Ctrl Pts',(-69.1573884361076,-11.3058820128323,
12.));
#143844=CARTESIAN_POINT('Ctrl Pts',(-69.1769483991639,-11.3038812726275,
12.));
#143845=CARTESIAN_POINT('Ctrl Pts',(-69.1965599718761,-11.3018540025605,
12.));
#143846=CARTESIAN_POINT('Ctrl Pts',(-69.216222948839,-11.2998001310934,
12.));
#143847=CARTESIAN_POINT('Ctrl Pts',(-69.2359370894828,-11.2977195764836,
12.));
#143848=CARTESIAN_POINT('Ctrl Pts',(-69.255702139335,-11.2956122531375,
12.));
#143849=CARTESIAN_POINT('Ctrl Pts',(-69.2755178531534,-11.2934780784361,
12.));
#143850=CARTESIAN_POINT('Ctrl Pts',(-69.2953840192792,-11.2913169799642,
12.));
#143851=CARTESIAN_POINT('Ctrl Pts',(-69.315300451784,-11.2891288931528,
12.));
#143852=CARTESIAN_POINT('Ctrl Pts',(-69.3352669789611,-11.2869137578463,
12.));
#143853=CARTESIAN_POINT('Ctrl Pts',(-69.3552834337771,-11.2846715154521,
12.));
#143854=CARTESIAN_POINT('Ctrl Pts',(-69.375349642,-11.2824021054038,12.));
#143855=CARTESIAN_POINT('Ctrl Pts',(-69.395465416223,-11.2801054633807,
12.));
#143856=CARTESIAN_POINT('Ctrl Pts',(-69.4156305620554,-11.2777815231462,
12.));
#143857=CARTESIAN_POINT('Ctrl Pts',(-69.4358448819957,-11.2754302177019,
12.));
#143858=CARTESIAN_POINT('Ctrl Pts',(-69.4561081798815,-11.2730514806143,
12.));
#143859=CARTESIAN_POINT('Ctrl Pts',(-69.4764202659443,-11.2706452475287,
12.));
#143860=CARTESIAN_POINT('Ctrl Pts',(-69.4967809565978,-11.2682114561015,
12.));
#143861=CARTESIAN_POINT('Ctrl Pts',(-69.5171900720188,-11.265750045272,
12.));
#143862=CARTESIAN_POINT('Ctrl Pts',(-69.5376474344768,-11.2632609547629,
12.));
#143863=CARTESIAN_POINT('Ctrl Pts',(-69.5581528662846,-11.2607441244698,
12.));
#143864=CARTESIAN_POINT('Ctrl Pts',(-69.5787061880815,-11.2581994939534,
12.));
#143865=CARTESIAN_POINT('Ctrl Pts',(-69.5993072197355,-11.255627002701,
12.));
#143866=CARTESIAN_POINT('Ctrl Pts',(-69.6199557811231,-11.2530265903555,
12.));
#143867=CARTESIAN_POINT('Ctrl Pts',(-69.6406516928902,-11.2503981969413,
12.));
#143868=CARTESIAN_POINT('Ctrl Pts',(-69.6613947773563,-11.247741763139,
12.));
#143869=CARTESIAN_POINT('Ctrl Pts',(-69.6821848588492,-11.2450572303847,
12.));
#143870=CARTESIAN_POINT('Ctrl Pts',(-69.7030217632187,-11.242344540717,
12.));
#143871=CARTESIAN_POINT('Ctrl Pts',(-69.7239053175362,-11.2396036366861,
12.));
#143872=CARTESIAN_POINT('Ctrl Pts',(-69.7448353497394,-11.236834461247,
12.));
#143873=CARTESIAN_POINT('Ctrl Pts',(-69.7658116882298,-11.2340369576452,
12.));
#143874=CARTESIAN_POINT('Ctrl Pts',(-69.7868341618927,-11.2312110694183,
12.));
#143875=CARTESIAN_POINT('Ctrl Pts',(-69.8079026002753,-11.2283567404434,
12.));
#143876=CARTESIAN_POINT('Ctrl Pts',(-69.8290168337076,-11.225473914972,
12.));
#143877=CARTESIAN_POINT('Ctrl Pts',(-69.8501766934445,-11.2225625376739,
12.));
#143878=CARTESIAN_POINT('Ctrl Pts',(-69.8713820117918,-11.2196225536794,
12.));
#143879=CARTESIAN_POINT('Ctrl Pts',(-69.8926326220414,-11.2166539085527,
12.));
#143880=CARTESIAN_POINT('Ctrl Pts',(-69.9139283584036,-11.2136565482679,
12.));
#143881=CARTESIAN_POINT('Ctrl Pts',(-69.9352690559399,-11.2106304191881,
12.));
#143882=CARTESIAN_POINT('Ctrl Pts',(-69.9566545504813,-11.2075754680445,
12.));
#143883=CARTESIAN_POINT('Ctrl Pts',(-69.9780846785771,-11.2044916419239,
12.));
#143884=CARTESIAN_POINT('Ctrl Pts',(-69.9995592775322,-11.2013788882711,
12.));
#143885=CARTESIAN_POINT('Ctrl Pts',(-70.0210781854236,-11.1982371548918,
12.));
#143886=CARTESIAN_POINT('Ctrl Pts',(-70.0426412411194,-11.1950663899578,
12.));
#143887=CARTESIAN_POINT('Ctrl Pts',(-70.0642482842942,-11.1918665420168,
12.));
#143888=CARTESIAN_POINT('Ctrl Pts',(-70.0858991554295,-11.1886375599916,
12.));
#143889=CARTESIAN_POINT('Ctrl Pts',(-70.1075936957973,-11.185379393167,
12.));
#143890=CARTESIAN_POINT('Ctrl Pts',(-70.1293317474432,-11.1820919911846,
12.));
#143891=CARTESIAN_POINT('Ctrl Pts',(-70.1511131531672,-11.1787753040363,
12.));
#143892=CARTESIAN_POINT('Ctrl Pts',(-70.1729377564954,-11.1754292820631,
12.));
#143893=CARTESIAN_POINT('Ctrl Pts',(-70.1948054016816,-11.1720538759499,
12.));
#143894=CARTESIAN_POINT('Ctrl Pts',(-70.2167159337094,-11.168649036721,
12.));
#143895=CARTESIAN_POINT('Ctrl Pts',(-70.2386691982902,-11.1652147157383,
12.));
#143896=CARTESIAN_POINT('Ctrl Pts',(-70.260665041859,-11.1617508647016,
12.));
#143897=CARTESIAN_POINT('Ctrl Pts',(-70.2827033115662,-11.158257435652,
12.));
#143898=CARTESIAN_POINT('Ctrl Pts',(-70.3047838552756,-11.1547343809646,
12.));
#143899=CARTESIAN_POINT('Ctrl Pts',(-70.326906521559,-11.1511816533421,
12.));
#143900=CARTESIAN_POINT('Ctrl Pts',(-70.349071159688,-11.1475992058124,
12.));
#143901=CARTESIAN_POINT('Ctrl Pts',(-70.3712776196223,-11.143986991727,
12.));
#143902=CARTESIAN_POINT('Ctrl Pts',(-70.393525751996,-11.1403449647625,
12.));
#143903=CARTESIAN_POINT('Ctrl Pts',(-70.4158154081205,-11.1366730789125,
12.));
#143904=CARTESIAN_POINT('Ctrl Pts',(-70.4381464399819,-11.1329712884846,
12.));
#143905=CARTESIAN_POINT('Ctrl Pts',(-70.4605187002354,-11.1292395480974,
12.));
#143906=CARTESIAN_POINT('Ctrl Pts',(-70.4829320421957,-11.1254778126821,
12.));
#143907=CARTESIAN_POINT('Ctrl Pts',(-70.505386319828,-11.1216860374826,
12.));
#143908=CARTESIAN_POINT('Ctrl Pts',(-70.5278813877494,-11.1178641780476,
12.));
#143909=CARTESIAN_POINT('Ctrl Pts',(-70.5504171012234,-11.1140121902271,
12.));
#143910=CARTESIAN_POINT('Ctrl Pts',(-70.5729933161546,-11.1101300301701,
12.));
#143911=CARTESIAN_POINT('Ctrl Pts',(-70.5956098890773,-11.1062176543262,
12.));
#143912=CARTESIAN_POINT('Ctrl Pts',(-70.6182666771481,-11.1022750194445,
12.));
#143913=CARTESIAN_POINT('Ctrl Pts',(-70.6409635381482,-11.0983020825667,
12.));
#143914=CARTESIAN_POINT('Ctrl Pts',(-70.6637003304785,-11.0942988010233,
12.));
#143915=CARTESIAN_POINT('Ctrl Pts',(-70.6864769131546,-11.0902651324323,
12.));
#143916=CARTESIAN_POINT('Ctrl Pts',(-70.7092931457954,-11.0862010347016,
12.));
#143917=CARTESIAN_POINT('Ctrl Pts',(-70.732148888618,-11.0821064660269,
12.));
#143918=CARTESIAN_POINT('Ctrl Pts',(-70.7550440024384,-11.0779813848846,
12.));
#143919=CARTESIAN_POINT('Ctrl Pts',(-70.7779783486677,-11.073825750029,
12.));
#143920=CARTESIAN_POINT('Ctrl Pts',(-70.8009517893057,-11.0696395204909,
12.));
#143921=CARTESIAN_POINT('Ctrl Pts',(-70.8239641869299,-11.0654226555802,
12.));
#143922=CARTESIAN_POINT('Ctrl Pts',(-70.8470154046919,-11.0611751148835,
12.));
#143923=CARTESIAN_POINT('Ctrl Pts',(-70.8701053063186,-11.0568968582569,
12.));
#143924=CARTESIAN_POINT('Ctrl Pts',(-70.8932337561087,-11.0525878458243,
12.));
#143925=CARTESIAN_POINT('Ctrl Pts',(-70.916400618927,-11.048248037975,12.));
#143926=CARTESIAN_POINT('Ctrl Pts',(-70.9396057601924,-11.0438773953681,
12.));
#143927=CARTESIAN_POINT('Ctrl Pts',(-70.9628490458748,-11.0394758789285,
12.));
#143928=CARTESIAN_POINT('Ctrl Pts',(-70.986130342497,-11.0350434498405,
12.));
#143929=CARTESIAN_POINT('Ctrl Pts',(-71.0094495171292,-11.0305800695456,
12.));
#143930=CARTESIAN_POINT('Ctrl Pts',(-71.0328064373856,-11.0260856997415,
12.));
#143931=CARTESIAN_POINT('Ctrl Pts',(-71.0562009714136,-11.0215603023856,
12.));
#143932=CARTESIAN_POINT('Ctrl Pts',(-71.0796329878907,-11.0170038396915,
12.));
#143933=CARTESIAN_POINT('Ctrl Pts',(-71.1031023560249,-11.0124162741224,
12.));
#143934=CARTESIAN_POINT('Ctrl Pts',(-71.1266089455517,-11.0077975683895,
12.));
#143935=CARTESIAN_POINT('Ctrl Pts',(-71.1501526267286,-11.0031476854502,
12.));
#143936=CARTESIAN_POINT('Ctrl Pts',(-71.1737332703248,-10.9984665885127,
12.));
#143937=CARTESIAN_POINT('Ctrl Pts',(-71.1973507476191,-10.993754241032,
12.));
#143938=CARTESIAN_POINT('Ctrl Pts',(-71.2210049304014,-10.9890106067039,
12.));
#143939=CARTESIAN_POINT('Ctrl Pts',(-71.2446956909687,-10.9842356494627,
12.));
#143940=CARTESIAN_POINT('Ctrl Pts',(-71.2684229021207,-10.9794293334805,
12.));
#143941=CARTESIAN_POINT('Ctrl Pts',(-71.2921864371491,-10.9745916231709,
12.));
#143942=CARTESIAN_POINT('Ctrl Pts',(-71.3159861698358,-10.969722483186,
12.));
#143943=CARTESIAN_POINT('Ctrl Pts',(-71.339821974454,-10.9648218784098,
12.));
#143944=CARTESIAN_POINT('Ctrl Pts',(-71.3636937257649,-10.9598897739564,
12.));
#143945=CARTESIAN_POINT('Ctrl Pts',(-71.3876012990138,-10.954926135169,
12.));
#143946=CARTESIAN_POINT('Ctrl Pts',(-71.4115445699194,-10.9499309276236,
12.));
#143947=CARTESIAN_POINT('Ctrl Pts',(-71.435523414672,-10.944904117127,12.));
#143948=CARTESIAN_POINT('Ctrl Pts',(-71.4595377099351,-10.9398456697095,
12.));
#143949=CARTESIAN_POINT('Ctrl Pts',(-71.4835873328423,-10.9347555516235,
12.));
#143950=CARTESIAN_POINT('Ctrl Pts',(-71.5076721609937,-10.9296337293424,
12.));
#143951=CARTESIAN_POINT('Ctrl Pts',(-71.5317920724459,-10.9244801695642,
12.));
#143952=CARTESIAN_POINT('Ctrl Pts',(-71.5559469457091,-10.91929483921,12.));
#143953=CARTESIAN_POINT('Ctrl Pts',(-71.5801366597488,-10.914077705417,
12.));
#143954=CARTESIAN_POINT('Ctrl Pts',(-71.6043610939835,-10.9088287355365,
12.));
#143955=CARTESIAN_POINT('Ctrl Pts',(-71.6286201282812,-10.9035478971328,
12.));
#143956=CARTESIAN_POINT('Ctrl Pts',(-71.6529136429504,-10.8982351579871,
12.));
#143957=CARTESIAN_POINT('Ctrl Pts',(-71.6772415187364,-10.8928904860964,
12.));
#143958=CARTESIAN_POINT('Ctrl Pts',(-71.7016036368236,-10.8875138496671,
12.));
#143959=CARTESIAN_POINT('Ctrl Pts',(-71.7259998788328,-10.882105217112,
12.));
#143960=CARTESIAN_POINT('Ctrl Pts',(-71.7504301268181,-10.8766645570497,
12.));
#143961=CARTESIAN_POINT('Ctrl Pts',(-71.7748942632593,-10.8711918383073,
12.));
#143962=CARTESIAN_POINT('Ctrl Pts',(-71.7993921710564,-10.865687029922,
12.));
#143963=CARTESIAN_POINT('Ctrl Pts',(-71.8239237335331,-10.8601501011332,
12.));
#143964=CARTESIAN_POINT('Ctrl Pts',(-71.8484888344339,-10.8545810213799,
12.));
#143965=CARTESIAN_POINT('Ctrl Pts',(-71.8730873579224,-10.8489797602997,
12.));
#143966=CARTESIAN_POINT('Ctrl Pts',(-71.8977191885725,-10.8433462877311,
12.));
#143967=CARTESIAN_POINT('Ctrl Pts',(-71.9223842113625,-10.8376805737159,
12.));
#143968=CARTESIAN_POINT('Ctrl Pts',(-71.9470823116785,-10.8319825884918,
12.));
#143969=CARTESIAN_POINT('Ctrl Pts',(-71.9718133753127,-10.8262523024898,
12.));
#143970=CARTESIAN_POINT('Ctrl Pts',(-71.9965772884619,-10.8204896863328,
12.));
#143971=CARTESIAN_POINT('Ctrl Pts',(-72.0213739377223,-10.8146947108375,
12.));
#143972=CARTESIAN_POINT('Ctrl Pts',(-72.0462032100815,-10.8088673470184,
12.));
#143973=CARTESIAN_POINT('Ctrl Pts',(-72.0710649929202,-10.8030075660808,
12.));
#143974=CARTESIAN_POINT('Ctrl Pts',(-72.0959591740114,-10.7971153394166,
12.));
#143975=CARTESIAN_POINT('Ctrl Pts',(-72.1208856415171,-10.7911906386027,
12.));
#143976=CARTESIAN_POINT('Ctrl Pts',(-72.1458442839834,-10.7852334354016,
12.));
#143977=CARTESIAN_POINT('Ctrl Pts',(-72.1708349903305,-10.7792437017662,
12.));
#143978=CARTESIAN_POINT('Ctrl Pts',(-72.1958576498558,-10.7732214098344,
12.));
#143979=CARTESIAN_POINT('Ctrl Pts',(-72.2209121522366,-10.7671665319255,
12.));
#143980=CARTESIAN_POINT('Ctrl Pts',(-72.2459983875296,-10.7610790405385,
12.));
#143981=CARTESIAN_POINT('Ctrl Pts',(-72.2711162461681,-10.7549589083535,
12.));
#143982=CARTESIAN_POINT('Ctrl Pts',(-72.2962656189556,-10.7488061082367,
12.));
#143983=CARTESIAN_POINT('Ctrl Pts',(-72.3214463970641,-10.7426206132375,
12.));
#143984=CARTESIAN_POINT('Ctrl Pts',(-72.3466584720318,-10.73640239658,12.));
#143985=CARTESIAN_POINT('Ctrl Pts',(-72.3719017357571,-10.7301514316607,
12.));
#143986=CARTESIAN_POINT('Ctrl Pts',(-72.3971760804933,-10.7238676920469,
12.));
#143987=CARTESIAN_POINT('Ctrl Pts',(-72.4224813988347,-10.7175511514788,
12.));
#143988=CARTESIAN_POINT('Ctrl Pts',(-72.4478175837156,-10.7112017838706,
12.));
#143989=CARTESIAN_POINT('Ctrl Pts',(-72.4731845284227,-10.7048195633061,
12.));
#143990=CARTESIAN_POINT('Ctrl Pts',(-72.4985821266023,-10.6984044640398,
12.));
#143991=CARTESIAN_POINT('Ctrl Pts',(-72.5240102722664,-10.691956460499,
12.));
#143992=CARTESIAN_POINT('Ctrl Pts',(-72.5494688597961,-10.6854755272904,
12.));
#143993=CARTESIAN_POINT('Ctrl Pts',(-72.5749577839415,-10.6789616392042,
12.));
#143994=CARTESIAN_POINT('Ctrl Pts',(-72.6004769398019,-10.6724147711995,
12.));
#143995=CARTESIAN_POINT('Ctrl Pts',(-72.6260262228065,-10.6658348983944,
12.));
#143996=CARTESIAN_POINT('Ctrl Pts',(-72.651605528691,-10.659221996058,12.));
#143997=CARTESIAN_POINT('Ctrl Pts',(-72.6772147534752,-10.6525760396054,
12.));
#143998=CARTESIAN_POINT('Ctrl Pts',(-72.7028537934317,-10.6458970045946,
12.));
#143999=CARTESIAN_POINT('Ctrl Pts',(-72.7285225451293,-10.6391848667352,
12.));
#144000=CARTESIAN_POINT('Ctrl Pts',(-72.7542209054812,-10.6324396018998,
12.));
#144001=CARTESIAN_POINT('Ctrl Pts',(-72.7799487717911,-10.6256611861394,
12.));
#144002=CARTESIAN_POINT('Ctrl Pts',(-72.8057060417887,-10.6188495956973,
12.));
#144003=CARTESIAN_POINT('Ctrl Pts',(-72.8314926136881,-10.6120048070367,
12.));
#144004=CARTESIAN_POINT('Ctrl Pts',(-72.8573083861337,-10.6051267968203,
12.));
#144005=CARTESIAN_POINT('Ctrl Pts',(-72.8831532580845,-10.5982155418626,
12.));
#144006=CARTESIAN_POINT('Ctrl Pts',(-72.9090271287083,-10.5912710190928,
12.));
#144007=CARTESIAN_POINT('Ctrl Pts',(-72.9349298972822,-10.5842932055209,
12.));
#144008=CARTESIAN_POINT('Ctrl Pts',(-72.9608614630534,-10.5772820781958,
12.));
#144009=CARTESIAN_POINT('Ctrl Pts',(-72.9868217252283,-10.570237614205,
12.));
#144010=CARTESIAN_POINT('Ctrl Pts',(-73.0128105832621,-10.5631597907651,
12.));
#144011=CARTESIAN_POINT('Ctrl Pts',(-73.0388279370834,-10.5560485852974,
12.));
#144012=CARTESIAN_POINT('Ctrl Pts',(-73.0648736873434,-10.5489039755138,
12.));
#144013=CARTESIAN_POINT('Ctrl Pts',(-73.0909477356474,-10.5417259395003,
12.));
#144014=CARTESIAN_POINT('Ctrl Pts',(-73.1170499848039,-10.53451445581,12.));
#144015=CARTESIAN_POINT('Ctrl Pts',(-73.1431803382711,-10.5272695032653,
12.));
#144016=CARTESIAN_POINT('Ctrl Pts',(-73.1693386996138,-10.5199910607654,
12.));
#144017=CARTESIAN_POINT('Ctrl Pts',(-73.1955249719048,-10.5126791070805,
12.));
#144018=CARTESIAN_POINT('Ctrl Pts',(-73.2217390572562,-10.5053336206908,
12.));
#144019=CARTESIAN_POINT('Ctrl Pts',(-73.2479808560189,-10.4979545795192,
12.));
#144020=CARTESIAN_POINT('Ctrl Pts',(-73.2742502674304,-10.4905419611523,
12.));
#144021=CARTESIAN_POINT('Ctrl Pts',(-73.3005471910583,-10.4830957433305,
12.));
#144022=CARTESIAN_POINT('Ctrl Pts',(-73.3268715280575,-10.4756159043806,
12.));
#144023=CARTESIAN_POINT('Ctrl Pts',(-73.3532231823659,-10.4681024236289,
12.));
#144024=CARTESIAN_POINT('Ctrl Pts',(-73.37960206225,-10.4605552819397,12.));
#144025=CARTESIAN_POINT('Ctrl Pts',(-73.4060080806686,-10.452974461845,
12.));
#144026=CARTESIAN_POINT('Ctrl Pts',(-73.4286663448108,-10.4464473465479,
12.));
#144027=CARTESIAN_POINT('Ctrl Pts',(-73.4460525528801,-10.4414249334738,
12.));
#144028=CARTESIAN_POINT('Ctrl Pts',(-73.458154743684,-10.437922150104,12.));
#144029=CARTESIAN_POINT('Ctrl Pts',(-73.4649650361896,-10.4359488742808,
12.));
#144030=CARTESIAN_POINT('Ctrl Pts',(-73.4664795929942,-10.4355099267295,
12.));
#144031=CARTESIAN_POINT('',(-69.079679653846,-11.3136138754165,0.));
#144032=CARTESIAN_POINT('',(-69.079679653846,-11.3136138754165,0.));
#144033=CARTESIAN_POINT('Ctrl Pts',(-73.4664795929942,-10.4355099267295,
0.));
#144034=CARTESIAN_POINT('Ctrl Pts',(-73.4649650361896,-10.4359488742808,
0.));
#144035=CARTESIAN_POINT('Ctrl Pts',(-73.458154743684,-10.437922150104,0.));
#144036=CARTESIAN_POINT('Ctrl Pts',(-73.4460525528801,-10.4414249334738,
0.));
#144037=CARTESIAN_POINT('Ctrl Pts',(-73.4286663448108,-10.4464473465479,
0.));
#144038=CARTESIAN_POINT('Ctrl Pts',(-73.4060080806686,-10.452974461845,
0.));
#144039=CARTESIAN_POINT('Ctrl Pts',(-73.37960206225,-10.4605552819397,0.));
#144040=CARTESIAN_POINT('Ctrl Pts',(-73.3532231823659,-10.4681024236289,
0.));
#144041=CARTESIAN_POINT('Ctrl Pts',(-73.3268715280575,-10.4756159043806,
0.));
#144042=CARTESIAN_POINT('Ctrl Pts',(-73.3005471910583,-10.4830957433305,
0.));
#144043=CARTESIAN_POINT('Ctrl Pts',(-73.2742502674304,-10.4905419611523,
0.));
#144044=CARTESIAN_POINT('Ctrl Pts',(-73.2479808560189,-10.4979545795192,
0.));
#144045=CARTESIAN_POINT('Ctrl Pts',(-73.2217390572562,-10.5053336206908,
0.));
#144046=CARTESIAN_POINT('Ctrl Pts',(-73.1955249719048,-10.5126791070805,
0.));
#144047=CARTESIAN_POINT('Ctrl Pts',(-73.1693386996138,-10.5199910607654,
0.));
#144048=CARTESIAN_POINT('Ctrl Pts',(-73.1431803382711,-10.5272695032653,
0.));
#144049=CARTESIAN_POINT('Ctrl Pts',(-73.1170499848039,-10.53451445581,0.));
#144050=CARTESIAN_POINT('Ctrl Pts',(-73.0909477356474,-10.5417259395003,
0.));
#144051=CARTESIAN_POINT('Ctrl Pts',(-73.0648736873434,-10.5489039755138,
0.));
#144052=CARTESIAN_POINT('Ctrl Pts',(-73.0388279370834,-10.5560485852974,
0.));
#144053=CARTESIAN_POINT('Ctrl Pts',(-73.0128105832621,-10.5631597907651,
0.));
#144054=CARTESIAN_POINT('Ctrl Pts',(-72.9868217252283,-10.570237614205,
0.));
#144055=CARTESIAN_POINT('Ctrl Pts',(-72.9608614630534,-10.5772820781958,
0.));
#144056=CARTESIAN_POINT('Ctrl Pts',(-72.9349298972822,-10.5842932055209,
0.));
#144057=CARTESIAN_POINT('Ctrl Pts',(-72.9090271287083,-10.5912710190928,
0.));
#144058=CARTESIAN_POINT('Ctrl Pts',(-72.8831532580845,-10.5982155418626,
0.));
#144059=CARTESIAN_POINT('Ctrl Pts',(-72.8573083861337,-10.6051267968203,
0.));
#144060=CARTESIAN_POINT('Ctrl Pts',(-72.8314926136881,-10.6120048070367,
0.));
#144061=CARTESIAN_POINT('Ctrl Pts',(-72.8057060417887,-10.6188495956973,
0.));
#144062=CARTESIAN_POINT('Ctrl Pts',(-72.7799487717911,-10.6256611861394,
0.));
#144063=CARTESIAN_POINT('Ctrl Pts',(-72.7542209054812,-10.6324396018998,
0.));
#144064=CARTESIAN_POINT('Ctrl Pts',(-72.7285225451293,-10.6391848667352,
0.));
#144065=CARTESIAN_POINT('Ctrl Pts',(-72.7028537934317,-10.6458970045946,
0.));
#144066=CARTESIAN_POINT('Ctrl Pts',(-72.6772147534752,-10.6525760396054,
0.));
#144067=CARTESIAN_POINT('Ctrl Pts',(-72.651605528691,-10.659221996058,0.));
#144068=CARTESIAN_POINT('Ctrl Pts',(-72.6260262228065,-10.6658348983944,
0.));
#144069=CARTESIAN_POINT('Ctrl Pts',(-72.6004769398019,-10.6724147711995,
0.));
#144070=CARTESIAN_POINT('Ctrl Pts',(-72.5749577839415,-10.6789616392042,
0.));
#144071=CARTESIAN_POINT('Ctrl Pts',(-72.5494688597961,-10.6854755272904,
0.));
#144072=CARTESIAN_POINT('Ctrl Pts',(-72.5240102722664,-10.691956460499,
0.));
#144073=CARTESIAN_POINT('Ctrl Pts',(-72.4985821266023,-10.6984044640398,
0.));
#144074=CARTESIAN_POINT('Ctrl Pts',(-72.4731845284227,-10.7048195633061,
0.));
#144075=CARTESIAN_POINT('Ctrl Pts',(-72.4478175837156,-10.7112017838706,
0.));
#144076=CARTESIAN_POINT('Ctrl Pts',(-72.4224813988347,-10.7175511514788,
0.));
#144077=CARTESIAN_POINT('Ctrl Pts',(-72.3971760804933,-10.7238676920469,
0.));
#144078=CARTESIAN_POINT('Ctrl Pts',(-72.3719017357571,-10.7301514316607,
0.));
#144079=CARTESIAN_POINT('Ctrl Pts',(-72.3466584720318,-10.73640239658,0.));
#144080=CARTESIAN_POINT('Ctrl Pts',(-72.3214463970641,-10.7426206132375,
0.));
#144081=CARTESIAN_POINT('Ctrl Pts',(-72.2962656189556,-10.7488061082367,
0.));
#144082=CARTESIAN_POINT('Ctrl Pts',(-72.2711162461681,-10.7549589083535,
0.));
#144083=CARTESIAN_POINT('Ctrl Pts',(-72.2459983875296,-10.7610790405385,
0.));
#144084=CARTESIAN_POINT('Ctrl Pts',(-72.2209121522366,-10.7671665319255,
0.));
#144085=CARTESIAN_POINT('Ctrl Pts',(-72.1958576498558,-10.7732214098344,
0.));
#144086=CARTESIAN_POINT('Ctrl Pts',(-72.1708349903305,-10.7792437017662,
0.));
#144087=CARTESIAN_POINT('Ctrl Pts',(-72.1458442839834,-10.7852334354016,
0.));
#144088=CARTESIAN_POINT('Ctrl Pts',(-72.1208856415171,-10.7911906386027,
0.));
#144089=CARTESIAN_POINT('Ctrl Pts',(-72.0959591740114,-10.7971153394166,
0.));
#144090=CARTESIAN_POINT('Ctrl Pts',(-72.0710649929202,-10.8030075660808,
0.));
#144091=CARTESIAN_POINT('Ctrl Pts',(-72.0462032100815,-10.8088673470184,
0.));
#144092=CARTESIAN_POINT('Ctrl Pts',(-72.0213739377223,-10.8146947108375,
0.));
#144093=CARTESIAN_POINT('Ctrl Pts',(-71.9965772884619,-10.8204896863328,
0.));
#144094=CARTESIAN_POINT('Ctrl Pts',(-71.9718133753127,-10.8262523024898,
0.));
#144095=CARTESIAN_POINT('Ctrl Pts',(-71.9470823116785,-10.8319825884918,
0.));
#144096=CARTESIAN_POINT('Ctrl Pts',(-71.9223842113625,-10.8376805737159,
0.));
#144097=CARTESIAN_POINT('Ctrl Pts',(-71.8977191885725,-10.8433462877311,
0.));
#144098=CARTESIAN_POINT('Ctrl Pts',(-71.8730873579224,-10.8489797602997,
0.));
#144099=CARTESIAN_POINT('Ctrl Pts',(-71.8484888344339,-10.8545810213799,
0.));
#144100=CARTESIAN_POINT('Ctrl Pts',(-71.8239237335331,-10.8601501011332,
0.));
#144101=CARTESIAN_POINT('Ctrl Pts',(-71.7993921710564,-10.865687029922,
0.));
#144102=CARTESIAN_POINT('Ctrl Pts',(-71.7748942632593,-10.8711918383073,
0.));
#144103=CARTESIAN_POINT('Ctrl Pts',(-71.7504301268181,-10.8766645570497,
0.));
#144104=CARTESIAN_POINT('Ctrl Pts',(-71.7259998788328,-10.882105217112,
0.));
#144105=CARTESIAN_POINT('Ctrl Pts',(-71.7016036368236,-10.8875138496671,
0.));
#144106=CARTESIAN_POINT('Ctrl Pts',(-71.6772415187364,-10.8928904860964,
0.));
#144107=CARTESIAN_POINT('Ctrl Pts',(-71.6529136429504,-10.8982351579871,
0.));
#144108=CARTESIAN_POINT('Ctrl Pts',(-71.6286201282812,-10.9035478971328,
0.));
#144109=CARTESIAN_POINT('Ctrl Pts',(-71.6043610939835,-10.9088287355365,
0.));
#144110=CARTESIAN_POINT('Ctrl Pts',(-71.5801366597488,-10.914077705417,
0.));
#144111=CARTESIAN_POINT('Ctrl Pts',(-71.5559469457091,-10.91929483921,0.));
#144112=CARTESIAN_POINT('Ctrl Pts',(-71.5317920724459,-10.9244801695642,
0.));
#144113=CARTESIAN_POINT('Ctrl Pts',(-71.5076721609937,-10.9296337293424,
0.));
#144114=CARTESIAN_POINT('Ctrl Pts',(-71.4835873328423,-10.9347555516235,
0.));
#144115=CARTESIAN_POINT('Ctrl Pts',(-71.4595377099351,-10.9398456697095,
0.));
#144116=CARTESIAN_POINT('Ctrl Pts',(-71.435523414672,-10.944904117127,0.));
#144117=CARTESIAN_POINT('Ctrl Pts',(-71.4115445699194,-10.9499309276236,
0.));
#144118=CARTESIAN_POINT('Ctrl Pts',(-71.3876012990138,-10.954926135169,
0.));
#144119=CARTESIAN_POINT('Ctrl Pts',(-71.3636937257649,-10.9598897739564,
0.));
#144120=CARTESIAN_POINT('Ctrl Pts',(-71.339821974454,-10.9648218784098,
0.));
#144121=CARTESIAN_POINT('Ctrl Pts',(-71.3159861698358,-10.969722483186,
0.));
#144122=CARTESIAN_POINT('Ctrl Pts',(-71.2921864371491,-10.9745916231709,
0.));
#144123=CARTESIAN_POINT('Ctrl Pts',(-71.2684229021207,-10.9794293334805,
0.));
#144124=CARTESIAN_POINT('Ctrl Pts',(-71.2446956909687,-10.9842356494627,
0.));
#144125=CARTESIAN_POINT('Ctrl Pts',(-71.2210049304014,-10.9890106067039,
0.));
#144126=CARTESIAN_POINT('Ctrl Pts',(-71.1973507476191,-10.993754241032,
0.));
#144127=CARTESIAN_POINT('Ctrl Pts',(-71.1737332703248,-10.9984665885127,
0.));
#144128=CARTESIAN_POINT('Ctrl Pts',(-71.1501526267286,-11.0031476854502,
0.));
#144129=CARTESIAN_POINT('Ctrl Pts',(-71.1266089455517,-11.0077975683895,
0.));
#144130=CARTESIAN_POINT('Ctrl Pts',(-71.1031023560249,-11.0124162741224,
0.));
#144131=CARTESIAN_POINT('Ctrl Pts',(-71.0796329878907,-11.0170038396915,
0.));
#144132=CARTESIAN_POINT('Ctrl Pts',(-71.0562009714136,-11.0215603023856,
0.));
#144133=CARTESIAN_POINT('Ctrl Pts',(-71.0328064373856,-11.0260856997415,
0.));
#144134=CARTESIAN_POINT('Ctrl Pts',(-71.0094495171292,-11.0305800695456,
0.));
#144135=CARTESIAN_POINT('Ctrl Pts',(-70.986130342497,-11.0350434498405,
0.));
#144136=CARTESIAN_POINT('Ctrl Pts',(-70.9628490458748,-11.0394758789285,
0.));
#144137=CARTESIAN_POINT('Ctrl Pts',(-70.9396057601924,-11.0438773953681,
0.));
#144138=CARTESIAN_POINT('Ctrl Pts',(-70.916400618927,-11.048248037975,0.));
#144139=CARTESIAN_POINT('Ctrl Pts',(-70.8932337561087,-11.0525878458243,
0.));
#144140=CARTESIAN_POINT('Ctrl Pts',(-70.8701053063186,-11.0568968582569,
0.));
#144141=CARTESIAN_POINT('Ctrl Pts',(-70.8470154046919,-11.0611751148835,
0.));
#144142=CARTESIAN_POINT('Ctrl Pts',(-70.8239641869299,-11.0654226555802,
0.));
#144143=CARTESIAN_POINT('Ctrl Pts',(-70.8009517893057,-11.0696395204909,
0.));
#144144=CARTESIAN_POINT('Ctrl Pts',(-70.7779783486677,-11.073825750029,
0.));
#144145=CARTESIAN_POINT('Ctrl Pts',(-70.7550440024384,-11.0779813848846,
0.));
#144146=CARTESIAN_POINT('Ctrl Pts',(-70.732148888618,-11.0821064660269,
0.));
#144147=CARTESIAN_POINT('Ctrl Pts',(-70.7092931457954,-11.0862010347016,
0.));
#144148=CARTESIAN_POINT('Ctrl Pts',(-70.6864769131546,-11.0902651324323,
0.));
#144149=CARTESIAN_POINT('Ctrl Pts',(-70.6637003304785,-11.0942988010233,
0.));
#144150=CARTESIAN_POINT('Ctrl Pts',(-70.6409635381482,-11.0983020825667,
0.));
#144151=CARTESIAN_POINT('Ctrl Pts',(-70.6182666771481,-11.1022750194445,
0.));
#144152=CARTESIAN_POINT('Ctrl Pts',(-70.5956098890773,-11.1062176543262,
0.));
#144153=CARTESIAN_POINT('Ctrl Pts',(-70.5729933161546,-11.1101300301701,
0.));
#144154=CARTESIAN_POINT('Ctrl Pts',(-70.5504171012234,-11.1140121902271,
0.));
#144155=CARTESIAN_POINT('Ctrl Pts',(-70.5278813877494,-11.1178641780476,
0.));
#144156=CARTESIAN_POINT('Ctrl Pts',(-70.505386319828,-11.1216860374826,
0.));
#144157=CARTESIAN_POINT('Ctrl Pts',(-70.4829320421957,-11.1254778126821,
0.));
#144158=CARTESIAN_POINT('Ctrl Pts',(-70.4605187002354,-11.1292395480974,
0.));
#144159=CARTESIAN_POINT('Ctrl Pts',(-70.4381464399819,-11.1329712884846,
0.));
#144160=CARTESIAN_POINT('Ctrl Pts',(-70.4158154081205,-11.1366730789125,
0.));
#144161=CARTESIAN_POINT('Ctrl Pts',(-70.393525751996,-11.1403449647625,
0.));
#144162=CARTESIAN_POINT('Ctrl Pts',(-70.3712776196223,-11.143986991727,
0.));
#144163=CARTESIAN_POINT('Ctrl Pts',(-70.349071159688,-11.1475992058124,
0.));
#144164=CARTESIAN_POINT('Ctrl Pts',(-70.326906521559,-11.1511816533421,
0.));
#144165=CARTESIAN_POINT('Ctrl Pts',(-70.3047838552756,-11.1547343809646,
0.));
#144166=CARTESIAN_POINT('Ctrl Pts',(-70.2827033115662,-11.158257435652,
0.));
#144167=CARTESIAN_POINT('Ctrl Pts',(-70.260665041859,-11.1617508647016,
0.));
#144168=CARTESIAN_POINT('Ctrl Pts',(-70.2386691982902,-11.1652147157383,
0.));
#144169=CARTESIAN_POINT('Ctrl Pts',(-70.2167159337094,-11.168649036721,
0.));
#144170=CARTESIAN_POINT('Ctrl Pts',(-70.1948054016816,-11.1720538759499,
0.));
#144171=CARTESIAN_POINT('Ctrl Pts',(-70.1729377564954,-11.1754292820631,
0.));
#144172=CARTESIAN_POINT('Ctrl Pts',(-70.1511131531672,-11.1787753040363,
0.));
#144173=CARTESIAN_POINT('Ctrl Pts',(-70.1293317474432,-11.1820919911846,
0.));
#144174=CARTESIAN_POINT('Ctrl Pts',(-70.1075936957973,-11.185379393167,
0.));
#144175=CARTESIAN_POINT('Ctrl Pts',(-70.0858991554295,-11.1886375599916,
0.));
#144176=CARTESIAN_POINT('Ctrl Pts',(-70.0642482842942,-11.1918665420168,
0.));
#144177=CARTESIAN_POINT('Ctrl Pts',(-70.0426412411194,-11.1950663899578,
0.));
#144178=CARTESIAN_POINT('Ctrl Pts',(-70.0210781854236,-11.1982371548918,
0.));
#144179=CARTESIAN_POINT('Ctrl Pts',(-69.9995592775322,-11.2013788882711,
0.));
#144180=CARTESIAN_POINT('Ctrl Pts',(-69.9780846785771,-11.2044916419239,
0.));
#144181=CARTESIAN_POINT('Ctrl Pts',(-69.9566545504813,-11.2075754680445,
0.));
#144182=CARTESIAN_POINT('Ctrl Pts',(-69.9352690559399,-11.2106304191881,
0.));
#144183=CARTESIAN_POINT('Ctrl Pts',(-69.9139283584036,-11.2136565482679,
0.));
#144184=CARTESIAN_POINT('Ctrl Pts',(-69.8926326220414,-11.2166539085527,
0.));
#144185=CARTESIAN_POINT('Ctrl Pts',(-69.8713820117918,-11.2196225536794,
0.));
#144186=CARTESIAN_POINT('Ctrl Pts',(-69.8501766934445,-11.2225625376739,
0.));
#144187=CARTESIAN_POINT('Ctrl Pts',(-69.8290168337076,-11.225473914972,
0.));
#144188=CARTESIAN_POINT('Ctrl Pts',(-69.8079026002753,-11.2283567404434,
0.));
#144189=CARTESIAN_POINT('Ctrl Pts',(-69.7868341618927,-11.2312110694183,
0.));
#144190=CARTESIAN_POINT('Ctrl Pts',(-69.7658116882298,-11.2340369576452,
0.));
#144191=CARTESIAN_POINT('Ctrl Pts',(-69.7448353497394,-11.236834461247,
0.));
#144192=CARTESIAN_POINT('Ctrl Pts',(-69.7239053175362,-11.2396036366861,
0.));
#144193=CARTESIAN_POINT('Ctrl Pts',(-69.7030217632187,-11.242344540717,
0.));
#144194=CARTESIAN_POINT('Ctrl Pts',(-69.6821848588492,-11.2450572303847,
0.));
#144195=CARTESIAN_POINT('Ctrl Pts',(-69.6613947773563,-11.247741763139,
0.));
#144196=CARTESIAN_POINT('Ctrl Pts',(-69.6406516928902,-11.2503981969413,
0.));
#144197=CARTESIAN_POINT('Ctrl Pts',(-69.6199557811231,-11.2530265903555,
0.));
#144198=CARTESIAN_POINT('Ctrl Pts',(-69.5993072197355,-11.255627002701,
0.));
#144199=CARTESIAN_POINT('Ctrl Pts',(-69.5787061880815,-11.2581994939534,
0.));
#144200=CARTESIAN_POINT('Ctrl Pts',(-69.5581528662846,-11.2607441244698,
0.));
#144201=CARTESIAN_POINT('Ctrl Pts',(-69.5376474344768,-11.2632609547629,
0.));
#144202=CARTESIAN_POINT('Ctrl Pts',(-69.5171900720188,-11.265750045272,
0.));
#144203=CARTESIAN_POINT('Ctrl Pts',(-69.4967809565978,-11.2682114561015,
0.));
#144204=CARTESIAN_POINT('Ctrl Pts',(-69.4764202659443,-11.2706452475287,
0.));
#144205=CARTESIAN_POINT('Ctrl Pts',(-69.4561081798815,-11.2730514806143,
0.));
#144206=CARTESIAN_POINT('Ctrl Pts',(-69.4358448819957,-11.2754302177019,
0.));
#144207=CARTESIAN_POINT('Ctrl Pts',(-69.4156305620554,-11.2777815231462,
0.));
#144208=CARTESIAN_POINT('Ctrl Pts',(-69.395465416223,-11.2801054633807,
0.));
#144209=CARTESIAN_POINT('Ctrl Pts',(-69.375349642,-11.2824021054038,0.));
#144210=CARTESIAN_POINT('Ctrl Pts',(-69.3552834337771,-11.2846715154521,
0.));
#144211=CARTESIAN_POINT('Ctrl Pts',(-69.3352669789611,-11.2869137578463,
0.));
#144212=CARTESIAN_POINT('Ctrl Pts',(-69.315300451784,-11.2891288931528,
0.));
#144213=CARTESIAN_POINT('Ctrl Pts',(-69.2953840192792,-11.2913169799642,
0.));
#144214=CARTESIAN_POINT('Ctrl Pts',(-69.2755178531534,-11.2934780784361,
0.));
#144215=CARTESIAN_POINT('Ctrl Pts',(-69.255702139335,-11.2956122531375,
0.));
#144216=CARTESIAN_POINT('Ctrl Pts',(-69.2359370894828,-11.2977195764836,
0.));
#144217=CARTESIAN_POINT('Ctrl Pts',(-69.216222948839,-11.2998001310934,
0.));
#144218=CARTESIAN_POINT('Ctrl Pts',(-69.1965599718761,-11.3018540025605,
0.));
#144219=CARTESIAN_POINT('Ctrl Pts',(-69.1769483991639,-11.3038812726275,
0.));
#144220=CARTESIAN_POINT('Ctrl Pts',(-69.1573884361076,-11.3058820128323,
0.));
#144221=CARTESIAN_POINT('Ctrl Pts',(-69.137880225198,-11.3078562764442,
0.));
#144222=CARTESIAN_POINT('Ctrl Pts',(-69.1184238445065,-11.3098040973799,
0.));
#144223=CARTESIAN_POINT('Ctrl Pts',(-69.1029002322497,-11.3113412156742,
0.));
#144224=CARTESIAN_POINT('Ctrl Pts',(-69.0912808657051,-11.3124821678849,
0.));
#144225=CARTESIAN_POINT('Ctrl Pts',(-69.0835449954486,-11.3132375200184,
0.));
#144226=CARTESIAN_POINT('Ctrl Pts',(-69.079679653846,-11.3136138754165,
0.));
#144227=CARTESIAN_POINT('Ctrl Pts',(-74.3992230078037,-3.87370827955543,
0.));
#144228=CARTESIAN_POINT('Ctrl Pts',(-74.3992230078037,-3.87370827955543,
12.));
#144229=CARTESIAN_POINT('Ctrl Pts',(-74.3940262116388,-3.87578335377325,
0.));
#144230=CARTESIAN_POINT('Ctrl Pts',(-74.3940262116388,-3.87578335377325,
12.));
#144231=CARTESIAN_POINT('Ctrl Pts',(-74.3836349189184,-3.87992989995747,
0.));
#144232=CARTESIAN_POINT('Ctrl Pts',(-74.3836349189184,-3.87992989995747,
12.));
#144233=CARTESIAN_POINT('Ctrl Pts',(-74.3680548786661,-3.88613891247983,
0.));
#144234=CARTESIAN_POINT('Ctrl Pts',(-74.3680548786661,-3.88613891247983,
12.));
#144235=CARTESIAN_POINT('Ctrl Pts',(-74.3472952898745,-3.89439598145328,
0.));
#144236=CARTESIAN_POINT('Ctrl Pts',(-74.3472952898745,-3.89439598145328,
12.));
#144237=CARTESIAN_POINT('Ctrl Pts',(-74.3213688090134,-3.90468128904634,
0.));
#144238=CARTESIAN_POINT('Ctrl Pts',(-74.3213688090134,-3.90468128904634,
12.));
#144239=CARTESIAN_POINT('Ctrl Pts',(-74.2954653518728,-3.9149305628503,
0.));
#144240=CARTESIAN_POINT('Ctrl Pts',(-74.2954653518728,-3.9149305628503,
12.));
#144241=CARTESIAN_POINT('Ctrl Pts',(-74.2695849516226,-3.92514379920743,
0.));
#144242=CARTESIAN_POINT('Ctrl Pts',(-74.2695849516226,-3.92514379920743,
12.));
#144243=CARTESIAN_POINT('Ctrl Pts',(-74.2437276593623,-3.93532099774203,
0.));
#144244=CARTESIAN_POINT('Ctrl Pts',(-74.2437276593623,-3.93532099774203,
12.));
#144245=CARTESIAN_POINT('Ctrl Pts',(-74.2178935492876,-3.94546216377451,
0.));
#144246=CARTESIAN_POINT('Ctrl Pts',(-74.2178935492876,-3.94546216377451,
12.));
#144247=CARTESIAN_POINT('Ctrl Pts',(-74.1920827166585,-3.9555673082111,
0.));
#144248=CARTESIAN_POINT('Ctrl Pts',(-74.1920827166585,-3.9555673082111,
12.));
#144249=CARTESIAN_POINT('Ctrl Pts',(-74.1662952702485,-3.96563644549385,
0.));
#144250=CARTESIAN_POINT('Ctrl Pts',(-74.1662952702485,-3.96563644549385,
12.));
#144251=CARTESIAN_POINT('Ctrl Pts',(-74.1405313263109,-3.97566959209528,
0.));
#144252=CARTESIAN_POINT('Ctrl Pts',(-74.1405313263109,-3.97566959209528,
12.));
#144253=CARTESIAN_POINT('Ctrl Pts',(-74.1147910020891,-3.98566676483641,
0.));
#144254=CARTESIAN_POINT('Ctrl Pts',(-74.1147910020891,-3.98566676483641,
12.));
#144255=CARTESIAN_POINT('Ctrl Pts',(-74.0890744091186,-3.99562797918287,
0.));
#144256=CARTESIAN_POINT('Ctrl Pts',(-74.0890744091186,-3.99562797918287,
12.));
#144257=CARTESIAN_POINT('Ctrl Pts',(-74.0633816478037,-4.0055532478548,
0.));
#144258=CARTESIAN_POINT('Ctrl Pts',(-74.0633816478037,-4.0055532478548,
12.));
#144259=CARTESIAN_POINT('Ctrl Pts',(-74.0377128111863,-4.0154425817671,
0.));
#144260=CARTESIAN_POINT('Ctrl Pts',(-74.0377128111863,-4.0154425817671,
12.));
#144261=CARTESIAN_POINT('Ctrl Pts',(-74.012067987646,-4.02529599070094,
0.));
#144262=CARTESIAN_POINT('Ctrl Pts',(-74.012067987646,-4.02529599070094,
12.));
#144263=CARTESIAN_POINT('Ctrl Pts',(-73.9864472641033,-4.03511348410659,
0.));
#144264=CARTESIAN_POINT('Ctrl Pts',(-73.9864472641033,-4.03511348410659,
12.));
#144265=CARTESIAN_POINT('Ctrl Pts',(-73.9608507287909,-4.04489507179957,
0.));
#144266=CARTESIAN_POINT('Ctrl Pts',(-73.9608507287909,-4.04489507179957,
12.));
#144267=CARTESIAN_POINT('Ctrl Pts',(-73.9352784747608,-4.05464076484752,
0.));
#144268=CARTESIAN_POINT('Ctrl Pts',(-73.9352784747608,-4.05464076484752,
12.));
#144269=CARTESIAN_POINT('Ctrl Pts',(-73.9097305995115,-4.06435057547324,
0.));
#144270=CARTESIAN_POINT('Ctrl Pts',(-73.9097305995115,-4.06435057547324,
12.));
#144271=CARTESIAN_POINT('Ctrl Pts',(-73.8842072034008,-4.07402451665244,
0.));
#144272=CARTESIAN_POINT('Ctrl Pts',(-73.8842072034008,-4.07402451665244,
12.));
#144273=CARTESIAN_POINT('Ctrl Pts',(-73.8587083884191,-4.08366260180674,
0.));
#144274=CARTESIAN_POINT('Ctrl Pts',(-73.8587083884191,-4.08366260180674,
12.));
#144275=CARTESIAN_POINT('Ctrl Pts',(-73.8332342568989,-4.09326484448232,
0.));
#144276=CARTESIAN_POINT('Ctrl Pts',(-73.8332342568989,-4.09326484448232,
12.));
#144277=CARTESIAN_POINT('Ctrl Pts',(-73.8077849100342,-4.10283125798729,
0.));
#144278=CARTESIAN_POINT('Ctrl Pts',(-73.8077849100342,-4.10283125798729,
12.));
#144279=CARTESIAN_POINT('Ctrl Pts',(-73.7823604472159,-4.11236185522787,
0.));
#144280=CARTESIAN_POINT('Ctrl Pts',(-73.7823604472159,-4.11236185522787,
12.));
#144281=CARTESIAN_POINT('Ctrl Pts',(-73.7569609668528,-4.12185664890556,
0.));
#144282=CARTESIAN_POINT('Ctrl Pts',(-73.7569609668528,-4.12185664890556,
12.));
#144283=CARTESIAN_POINT('Ctrl Pts',(-73.7315865668522,-4.13131565163578,
0.));
#144284=CARTESIAN_POINT('Ctrl Pts',(-73.7315865668522,-4.13131565163578,
12.));
#144285=CARTESIAN_POINT('Ctrl Pts',(-73.7062373452342,-4.14073887610153,
0.));
#144286=CARTESIAN_POINT('Ctrl Pts',(-73.7062373452342,-4.14073887610153,
12.));
#144287=CARTESIAN_POINT('Ctrl Pts',(-73.6809134006897,-4.15012633519723,
0.));
#144288=CARTESIAN_POINT('Ctrl Pts',(-73.6809134006897,-4.15012633519723,
12.));
#144289=CARTESIAN_POINT('Ctrl Pts',(-73.6556148331489,-4.15947804217783,
0.));
#144290=CARTESIAN_POINT('Ctrl Pts',(-73.6556148331489,-4.15947804217783,
12.));
#144291=CARTESIAN_POINT('Ctrl Pts',(-73.6303417435251,-4.1687940105878,
0.));
#144292=CARTESIAN_POINT('Ctrl Pts',(-73.6303417435251,-4.1687940105878,
12.));
#144293=CARTESIAN_POINT('Ctrl Pts',(-73.6050942334768,-4.17807425419812,
0.));
#144294=CARTESIAN_POINT('Ctrl Pts',(-73.6050942334768,-4.17807425419812,
12.));
#144295=CARTESIAN_POINT('Ctrl Pts',(-73.5798724051519,-4.18731878694236,
0.));
#144296=CARTESIAN_POINT('Ctrl Pts',(-73.5798724051519,-4.18731878694236,
12.));
#144297=CARTESIAN_POINT('Ctrl Pts',(-73.5546763609572,-4.19652762286126,
0.));
#144298=CARTESIAN_POINT('Ctrl Pts',(-73.5546763609572,-4.19652762286126,
12.));
#144299=CARTESIAN_POINT('Ctrl Pts',(-73.5295062032628,-4.2057007760373,
0.));
#144300=CARTESIAN_POINT('Ctrl Pts',(-73.5295062032628,-4.2057007760373,
12.));
#144301=CARTESIAN_POINT('Ctrl Pts',(-73.5043620344116,-4.21483826059441,
0.));
#144302=CARTESIAN_POINT('Ctrl Pts',(-73.5043620344116,-4.21483826059441,
12.));
#144303=CARTESIAN_POINT('Ctrl Pts',(-73.4792439568633,-4.22394009072756,
0.));
#144304=CARTESIAN_POINT('Ctrl Pts',(-73.4792439568633,-4.22394009072756,
12.));
#144305=CARTESIAN_POINT('Ctrl Pts',(-73.4541520732948,-4.23300628072758,
0.));
#144306=CARTESIAN_POINT('Ctrl Pts',(-73.4541520732948,-4.23300628072758,
12.));
#144307=CARTESIAN_POINT('Ctrl Pts',(-73.4290864867101,-4.24203684500938,
0.));
#144308=CARTESIAN_POINT('Ctrl Pts',(-73.4290864867101,-4.24203684500938,
12.));
#144309=CARTESIAN_POINT('Ctrl Pts',(-73.4040473005592,-4.25103179814886,
0.));
#144310=CARTESIAN_POINT('Ctrl Pts',(-73.4040473005592,-4.25103179814886,
12.));
#144311=CARTESIAN_POINT('Ctrl Pts',(-73.3790346187938,-4.25999115489899,
0.));
#144312=CARTESIAN_POINT('Ctrl Pts',(-73.3790346187938,-4.25999115489899,
12.));
#144313=CARTESIAN_POINT('Ctrl Pts',(-73.3540485458065,-4.26891493016699,
0.));
#144314=CARTESIAN_POINT('Ctrl Pts',(-73.3540485458065,-4.26891493016699,
12.));
#144315=CARTESIAN_POINT('Ctrl Pts',(-73.3290891863949,-4.27780313900389,
0.));
#144316=CARTESIAN_POINT('Ctrl Pts',(-73.3290891863949,-4.27780313900389,
12.));
#144317=CARTESIAN_POINT('Ctrl Pts',(-73.3041566457135,-4.28665579659301,
0.));
#144318=CARTESIAN_POINT('Ctrl Pts',(-73.3041566457135,-4.28665579659301,
12.));
#144319=CARTESIAN_POINT('Ctrl Pts',(-73.2792510292254,-4.29547291824287,
0.));
#144320=CARTESIAN_POINT('Ctrl Pts',(-73.2792510292254,-4.29547291824287,
12.));
#144321=CARTESIAN_POINT('Ctrl Pts',(-73.2543724426577,-4.3042545193823,
0.));
#144322=CARTESIAN_POINT('Ctrl Pts',(-73.2543724426577,-4.3042545193823,
12.));
#144323=CARTESIAN_POINT('Ctrl Pts',(-73.2295209920334,-4.31300061556098,
0.));
#144324=CARTESIAN_POINT('Ctrl Pts',(-73.2295209920334,-4.31300061556098,
12.));
#144325=CARTESIAN_POINT('Ctrl Pts',(-73.204696783694,-4.32171122245214,
0.));
#144326=CARTESIAN_POINT('Ctrl Pts',(-73.204696783694,-4.32171122245214,
12.));
#144327=CARTESIAN_POINT('Ctrl Pts',(-73.1798999243235,-4.33038635585876,
0.));
#144328=CARTESIAN_POINT('Ctrl Pts',(-73.1798999243235,-4.33038635585876,
12.));
#144329=CARTESIAN_POINT('Ctrl Pts',(-73.1551305209685,-4.3390260317214,
0.));
#144330=CARTESIAN_POINT('Ctrl Pts',(-73.1551305209685,-4.3390260317214,
12.));
#144331=CARTESIAN_POINT('Ctrl Pts',(-73.130388681059,-4.34763026613157,
0.));
#144332=CARTESIAN_POINT('Ctrl Pts',(-73.130388681059,-4.34763026613157,
12.));
#144333=CARTESIAN_POINT('Ctrl Pts',(-73.1056745124087,-4.35619907532719,
0.));
#144334=CARTESIAN_POINT('Ctrl Pts',(-73.1056745124087,-4.35619907532719,
12.));
#144335=CARTESIAN_POINT('Ctrl Pts',(-73.0809881232103,-4.36473247568641,
0.));
#144336=CARTESIAN_POINT('Ctrl Pts',(-73.0809881232103,-4.36473247568641,
12.));
#144337=CARTESIAN_POINT('Ctrl Pts',(-73.0563296220299,-4.37323048372607,
0.));
#144338=CARTESIAN_POINT('Ctrl Pts',(-73.0563296220299,-4.37323048372607,
12.));
#144339=CARTESIAN_POINT('Ctrl Pts',(-73.0316991177993,-4.3816931161015,
0.));
#144340=CARTESIAN_POINT('Ctrl Pts',(-73.0316991177993,-4.3816931161015,
12.));
#144341=CARTESIAN_POINT('Ctrl Pts',(-73.007096719804,-4.39012038961139,
0.));
#144342=CARTESIAN_POINT('Ctrl Pts',(-73.007096719804,-4.39012038961139,
12.));
#144343=CARTESIAN_POINT('Ctrl Pts',(-72.9825225376846,-4.39851232119722,
0.));
#144344=CARTESIAN_POINT('Ctrl Pts',(-72.9825225376846,-4.39851232119722,
12.));
#144345=CARTESIAN_POINT('Ctrl Pts',(-72.95797668145,-4.40686892793957,0.));
#144346=CARTESIAN_POINT('Ctrl Pts',(-72.95797668145,-4.40686892793957,12.));
#144347=CARTESIAN_POINT('Ctrl Pts',(-72.9334592614829,-4.41519022705921,
0.));
#144348=CARTESIAN_POINT('Ctrl Pts',(-72.9334592614829,-4.41519022705921,
12.));
#144349=CARTESIAN_POINT('Ctrl Pts',(-72.9089703885462,-4.42347623591941,
0.));
#144350=CARTESIAN_POINT('Ctrl Pts',(-72.9089703885462,-4.42347623591941,
12.));
#144351=CARTESIAN_POINT('Ctrl Pts',(-72.8845101737855,-4.43172697203349,
0.));
#144352=CARTESIAN_POINT('Ctrl Pts',(-72.8845101737855,-4.43172697203349,
12.));
#144353=CARTESIAN_POINT('Ctrl Pts',(-72.8600787287318,-4.43994245306818,
0.));
#144354=CARTESIAN_POINT('Ctrl Pts',(-72.8600787287318,-4.43994245306818,
12.));
#144355=CARTESIAN_POINT('Ctrl Pts',(-72.8356761653069,-4.44812269683737,
0.));
#144356=CARTESIAN_POINT('Ctrl Pts',(-72.8356761653069,-4.44812269683737,
12.));
#144357=CARTESIAN_POINT('Ctrl Pts',(-72.8113025958262,-4.45626772130146,
0.));
#144358=CARTESIAN_POINT('Ctrl Pts',(-72.8113025958262,-4.45626772130146,
12.));
#144359=CARTESIAN_POINT('Ctrl Pts',(-72.7869581329994,-4.46437754456792,
0.));
#144360=CARTESIAN_POINT('Ctrl Pts',(-72.7869581329994,-4.46437754456792,
12.));
#144361=CARTESIAN_POINT('Ctrl Pts',(-72.7626428899281,-4.47245218489609,
0.));
#144362=CARTESIAN_POINT('Ctrl Pts',(-72.7626428899281,-4.47245218489609,
12.));
#144363=CARTESIAN_POINT('Ctrl Pts',(-72.738356980103,-4.48049166070205,
0.));
#144364=CARTESIAN_POINT('Ctrl Pts',(-72.738356980103,-4.48049166070205,
12.));
#144365=CARTESIAN_POINT('Ctrl Pts',(-72.714100517414,-4.48849599055337,
0.));
#144366=CARTESIAN_POINT('Ctrl Pts',(-72.714100517414,-4.48849599055337,
12.));
#144367=CARTESIAN_POINT('Ctrl Pts',(-72.6898736161542,-4.49646519316812,
0.));
#144368=CARTESIAN_POINT('Ctrl Pts',(-72.6898736161542,-4.49646519316812,
12.));
#144369=CARTESIAN_POINT('Ctrl Pts',(-72.6656763910241,-4.50439928741604,
0.));
#144370=CARTESIAN_POINT('Ctrl Pts',(-72.6656763910241,-4.50439928741604,
12.));
#144371=CARTESIAN_POINT('Ctrl Pts',(-72.6415089571321,-4.51229829232264,
0.));
#144372=CARTESIAN_POINT('Ctrl Pts',(-72.6415089571321,-4.51229829232264,
12.));
#144373=CARTESIAN_POINT('Ctrl Pts',(-72.6173714299942,-4.52016222707637,
0.));
#144374=CARTESIAN_POINT('Ctrl Pts',(-72.6173714299942,-4.52016222707637,
12.));
#144375=CARTESIAN_POINT('Ctrl Pts',(-72.5932639255409,-4.52799111102391,
0.));
#144376=CARTESIAN_POINT('Ctrl Pts',(-72.5932639255409,-4.52799111102391,
12.));
#144377=CARTESIAN_POINT('Ctrl Pts',(-72.5691865601223,-4.53578496366799,
0.));
#144378=CARTESIAN_POINT('Ctrl Pts',(-72.5691865601223,-4.53578496366799,
12.));
#144379=CARTESIAN_POINT('Ctrl Pts',(-72.5451394505104,-4.54354380466822,
0.));
#144380=CARTESIAN_POINT('Ctrl Pts',(-72.5451394505104,-4.54354380466822,
12.));
#144381=CARTESIAN_POINT('Ctrl Pts',(-72.5211227139001,-4.55126765384404,
0.));
#144382=CARTESIAN_POINT('Ctrl Pts',(-72.5211227139001,-4.55126765384404,
12.));
#144383=CARTESIAN_POINT('Ctrl Pts',(-72.4971364679068,-4.5589565311822,
0.));
#144384=CARTESIAN_POINT('Ctrl Pts',(-72.4971364679068,-4.5589565311822,
12.));
#144385=CARTESIAN_POINT('Ctrl Pts',(-72.4731808305728,-4.56661045683376,
0.));
#144386=CARTESIAN_POINT('Ctrl Pts',(-72.4731808305728,-4.56661045683376,
12.));
#144387=CARTESIAN_POINT('Ctrl Pts',(-72.4492559203745,-4.57422945111102,
0.));
#144388=CARTESIAN_POINT('Ctrl Pts',(-72.4492559203745,-4.57422945111102,
12.));
#144389=CARTESIAN_POINT('Ctrl Pts',(-72.4253618562252,-4.58181353448851,
0.));
#144390=CARTESIAN_POINT('Ctrl Pts',(-72.4253618562252,-4.58181353448851,
12.));
#144391=CARTESIAN_POINT('Ctrl Pts',(-72.401498757478,-4.58936272760544,
0.));
#144392=CARTESIAN_POINT('Ctrl Pts',(-72.401498757478,-4.58936272760544,
12.));
#144393=CARTESIAN_POINT('Ctrl Pts',(-72.3776667439227,-4.5968770512733,
0.));
#144394=CARTESIAN_POINT('Ctrl Pts',(-72.3776667439227,-4.5968770512733,
12.));
#144395=CARTESIAN_POINT('Ctrl Pts',(-72.3538659357913,-4.60435652647453,
0.));
#144396=CARTESIAN_POINT('Ctrl Pts',(-72.3538659357913,-4.60435652647453,
12.));
#144397=CARTESIAN_POINT('Ctrl Pts',(-72.3300964537658,-4.61180117435862,
0.));
#144398=CARTESIAN_POINT('Ctrl Pts',(-72.3300964537658,-4.61180117435862,
12.));
#144399=CARTESIAN_POINT('Ctrl Pts',(-72.3063584189807,-4.61921101624292,
0.));
#144400=CARTESIAN_POINT('Ctrl Pts',(-72.3063584189807,-4.61921101624292,
12.));
#144401=CARTESIAN_POINT('Ctrl Pts',(-72.2826519530259,-4.62658607361466,
0.));
#144402=CARTESIAN_POINT('Ctrl Pts',(-72.2826519530259,-4.62658607361466,
12.));
#144403=CARTESIAN_POINT('Ctrl Pts',(-72.2589771779456,-4.63392636813843,
0.));
#144404=CARTESIAN_POINT('Ctrl Pts',(-72.2589771779456,-4.63392636813843,
12.));
#144405=CARTESIAN_POINT('Ctrl Pts',(-72.2353342162417,-4.64123192165627,
0.));
#144406=CARTESIAN_POINT('Ctrl Pts',(-72.2353342162417,-4.64123192165627,
12.));
#144407=CARTESIAN_POINT('Ctrl Pts',(-72.2117231908822,-4.64850275618323,
0.));
#144408=CARTESIAN_POINT('Ctrl Pts',(-72.2117231908822,-4.64850275618323,
12.));
#144409=CARTESIAN_POINT('Ctrl Pts',(-72.1881442253053,-4.65573889390822,
0.));
#144410=CARTESIAN_POINT('Ctrl Pts',(-72.1881442253053,-4.65573889390822,
12.));
#144411=CARTESIAN_POINT('Ctrl Pts',(-72.1645974434216,-4.66294035719569,
0.));
#144412=CARTESIAN_POINT('Ctrl Pts',(-72.1645974434216,-4.66294035719569,
12.));
#144413=CARTESIAN_POINT('Ctrl Pts',(-72.1410829696128,-4.67010716859285,
0.));
#144414=CARTESIAN_POINT('Ctrl Pts',(-72.1410829696128,-4.67010716859285,
12.));
#144415=CARTESIAN_POINT('Ctrl Pts',(-72.1176009287351,-4.67723935083094,
0.));
#144416=CARTESIAN_POINT('Ctrl Pts',(-72.1176009287351,-4.67723935083094,
12.));
#144417=CARTESIAN_POINT('Ctrl Pts',(-72.0941514461287,-4.68433692682068,
0.));
#144418=CARTESIAN_POINT('Ctrl Pts',(-72.0941514461287,-4.68433692682068,
12.));
#144419=CARTESIAN_POINT('Ctrl Pts',(-72.0707346476213,-4.69139991965283,
0.));
#144420=CARTESIAN_POINT('Ctrl Pts',(-72.0707346476213,-4.69139991965283,
12.));
#144421=CARTESIAN_POINT('Ctrl Pts',(-72.0473506595318,-4.69842835259992,
0.));
#144422=CARTESIAN_POINT('Ctrl Pts',(-72.0473506595318,-4.69842835259992,
12.));
#144423=CARTESIAN_POINT('Ctrl Pts',(-72.0239996086686,-4.705422249123,0.));
#144424=CARTESIAN_POINT('Ctrl Pts',(-72.0239996086686,-4.705422249123,12.));
#144425=CARTESIAN_POINT('Ctrl Pts',(-72.0006816223325,-4.71238163287396,
0.));
#144426=CARTESIAN_POINT('Ctrl Pts',(-72.0006816223325,-4.71238163287396,
12.));
#144427=CARTESIAN_POINT('Ctrl Pts',(-71.9773968283259,-4.7193065276907,
0.));
#144428=CARTESIAN_POINT('Ctrl Pts',(-71.9773968283259,-4.7193065276907,
12.));
#144429=CARTESIAN_POINT('Ctrl Pts',(-71.9541453549579,-4.72619695759774,
0.));
#144430=CARTESIAN_POINT('Ctrl Pts',(-71.9541453549579,-4.72619695759774,
12.));
#144431=CARTESIAN_POINT('Ctrl Pts',(-71.9309273310471,-4.73305294680785,
0.));
#144432=CARTESIAN_POINT('Ctrl Pts',(-71.9309273310471,-4.73305294680785,
12.));
#144433=CARTESIAN_POINT('Ctrl Pts',(-71.9077428859212,-4.73987451972863,
0.));
#144434=CARTESIAN_POINT('Ctrl Pts',(-71.9077428859212,-4.73987451972863,
12.));
#144435=CARTESIAN_POINT('Ctrl Pts',(-71.8845921494189,-4.74666170096547,
0.));
#144436=CARTESIAN_POINT('Ctrl Pts',(-71.8845921494189,-4.74666170096547,
12.));
#144437=CARTESIAN_POINT('Ctrl Pts',(-71.8614752519008,-4.75341451531669,
0.));
#144438=CARTESIAN_POINT('Ctrl Pts',(-71.8614752519008,-4.75341451531669,
12.));
#144439=CARTESIAN_POINT('Ctrl Pts',(-71.8383923242531,-4.76013298777419,
0.));
#144440=CARTESIAN_POINT('Ctrl Pts',(-71.8383923242531,-4.76013298777419,
12.));
#144441=CARTESIAN_POINT('Ctrl Pts',(-71.8153434978923,-4.76681714352502,
0.));
#144442=CARTESIAN_POINT('Ctrl Pts',(-71.8153434978923,-4.76681714352502,
12.));
#144443=CARTESIAN_POINT('Ctrl Pts',(-71.7923289047643,-4.77346700795792,
0.));
#144444=CARTESIAN_POINT('Ctrl Pts',(-71.7923289047643,-4.77346700795792,
12.));
#144445=CARTESIAN_POINT('Ctrl Pts',(-71.769348677346,-4.7800826066665,0.));
#144446=CARTESIAN_POINT('Ctrl Pts',(-71.769348677346,-4.7800826066665,12.));
#144447=CARTESIAN_POINT('Ctrl Pts',(-71.7464029486563,-4.78666396544458,
0.));
#144448=CARTESIAN_POINT('Ctrl Pts',(-71.7464029486563,-4.78666396544458,
12.));
#144449=CARTESIAN_POINT('Ctrl Pts',(-71.723491852261,-4.79321111028676,
0.));
#144450=CARTESIAN_POINT('Ctrl Pts',(-71.723491852261,-4.79321111028676,
12.));
#144451=CARTESIAN_POINT('Ctrl Pts',(-71.7006155222764,-4.7997240673901,
0.));
#144452=CARTESIAN_POINT('Ctrl Pts',(-71.7006155222764,-4.7997240673901,
12.));
#144453=CARTESIAN_POINT('Ctrl Pts',(-71.6777740933687,-4.80620286316075,
0.));
#144454=CARTESIAN_POINT('Ctrl Pts',(-71.6777740933687,-4.80620286316075,
12.));
#144455=CARTESIAN_POINT('Ctrl Pts',(-71.6549677007582,-4.81264752421713,
0.));
#144456=CARTESIAN_POINT('Ctrl Pts',(-71.6549677007582,-4.81264752421713,
12.));
#144457=CARTESIAN_POINT('Ctrl Pts',(-71.6321964802297,-4.81905807738541,
0.));
#144458=CARTESIAN_POINT('Ctrl Pts',(-71.6321964802297,-4.81905807738541,
12.));
#144459=CARTESIAN_POINT('Ctrl Pts',(-71.6094605681353,-4.8254345497002,
0.));
#144460=CARTESIAN_POINT('Ctrl Pts',(-71.6094605681353,-4.8254345497002,
12.));
#144461=CARTESIAN_POINT('Ctrl Pts',(-71.5867601014008,-4.8317769684064,
0.));
#144462=CARTESIAN_POINT('Ctrl Pts',(-71.5867601014008,-4.8317769684064,
12.));
#144463=CARTESIAN_POINT('Ctrl Pts',(-71.5640952175239,-4.83808536096589,
0.));
#144464=CARTESIAN_POINT('Ctrl Pts',(-71.5640952175239,-4.83808536096589,
12.));
#144465=CARTESIAN_POINT('Ctrl Pts',(-71.5414660545778,-4.84435975506056,
0.));
#144466=CARTESIAN_POINT('Ctrl Pts',(-71.5414660545778,-4.84435975506056,
12.));
#144467=CARTESIAN_POINT('Ctrl Pts',(-71.5188727512231,-4.85060017858786,
0.));
#144468=CARTESIAN_POINT('Ctrl Pts',(-71.5188727512231,-4.85060017858786,
12.));
#144469=CARTESIAN_POINT('Ctrl Pts',(-71.4963154467128,-4.85680665966184,
0.));
#144470=CARTESIAN_POINT('Ctrl Pts',(-71.4963154467128,-4.85680665966184,
12.));
#144471=CARTESIAN_POINT('Ctrl Pts',(-71.4737942808971,-4.86297922661498,
0.));
#144472=CARTESIAN_POINT('Ctrl Pts',(-71.4737942808971,-4.86297922661498,
12.));
#144473=CARTESIAN_POINT('Ctrl Pts',(-71.4513093942216,-4.86911790800533,
0.));
#144474=CARTESIAN_POINT('Ctrl Pts',(-71.4513093942216,-4.86911790800533,
12.));
#144475=CARTESIAN_POINT('Ctrl Pts',(-71.4288609277324,-4.8752227326188,
0.));
#144476=CARTESIAN_POINT('Ctrl Pts',(-71.4288609277324,-4.8752227326188,
12.));
#144477=CARTESIAN_POINT('Ctrl Pts',(-71.4064490230857,-4.88129372946524,
0.));
#144478=CARTESIAN_POINT('Ctrl Pts',(-71.4064490230857,-4.88129372946524,
12.));
#144479=CARTESIAN_POINT('Ctrl Pts',(-71.3840738225548,-4.88733092777964,
0.));
#144480=CARTESIAN_POINT('Ctrl Pts',(-71.3840738225548,-4.88733092777964,
12.));
#144481=CARTESIAN_POINT('Ctrl Pts',(-71.3617354690342,-4.89333435702423,
0.));
#144482=CARTESIAN_POINT('Ctrl Pts',(-71.3617354690342,-4.89333435702423,
12.));
#144483=CARTESIAN_POINT('Ctrl Pts',(-71.3394341060396,-4.89930404689599,
0.));
#144484=CARTESIAN_POINT('Ctrl Pts',(-71.3394341060396,-4.89930404689599,
12.));
#144485=CARTESIAN_POINT('Ctrl Pts',(-71.3171698777124,-4.90524002732806,
0.));
#144486=CARTESIAN_POINT('Ctrl Pts',(-71.3171698777124,-4.90524002732806,
12.));
#144487=CARTESIAN_POINT('Ctrl Pts',(-71.2949429288319,-4.91114232848623,
0.));
#144488=CARTESIAN_POINT('Ctrl Pts',(-71.2949429288319,-4.91114232848623,
12.));
#144489=CARTESIAN_POINT('Ctrl Pts',(-71.27275340482,-4.91701098077041,0.));
#144490=CARTESIAN_POINT('Ctrl Pts',(-71.27275340482,-4.91701098077041,12.));
#144491=CARTESIAN_POINT('Ctrl Pts',(-71.2506014517457,-4.9228460148171,
0.));
#144492=CARTESIAN_POINT('Ctrl Pts',(-71.2506014517457,-4.9228460148171,
12.));
#144493=CARTESIAN_POINT('Ctrl Pts',(-71.2284872163248,-4.92864746150711,
0.));
#144494=CARTESIAN_POINT('Ctrl Pts',(-71.2284872163248,-4.92864746150711,
12.));
#144495=CARTESIAN_POINT('Ctrl Pts',(-71.206410845926,-4.93441535196593,
0.));
#144496=CARTESIAN_POINT('Ctrl Pts',(-71.206410845926,-4.93441535196593,
12.));
#144497=CARTESIAN_POINT('Ctrl Pts',(-71.184372488583,-4.94014971756097,
0.));
#144498=CARTESIAN_POINT('Ctrl Pts',(-71.184372488583,-4.94014971756097,
12.));
#144499=CARTESIAN_POINT('Ctrl Pts',(-71.1623722929998,-4.94585058990336,
0.));
#144500=CARTESIAN_POINT('Ctrl Pts',(-71.1623722929998,-4.94585058990336,
12.));
#144501=CARTESIAN_POINT('Ctrl Pts',(-71.1404104085561,-4.9515180008511,
0.));
#144502=CARTESIAN_POINT('Ctrl Pts',(-71.1404104085561,-4.9515180008511,
12.));
#144503=CARTESIAN_POINT('Ctrl Pts',(-71.1184869853071,-4.95715198251703,
0.));
#144504=CARTESIAN_POINT('Ctrl Pts',(-71.1184869853071,-4.95715198251703,
12.));
#144505=CARTESIAN_POINT('Ctrl Pts',(-71.0966021739922,-4.96275256726786,
0.));
#144506=CARTESIAN_POINT('Ctrl Pts',(-71.0966021739922,-4.96275256726786,
12.));
#144507=CARTESIAN_POINT('Ctrl Pts',(-71.0747561260443,-4.96831978772201,
0.));
#144508=CARTESIAN_POINT('Ctrl Pts',(-71.0747561260443,-4.96831978772201,
12.));
#144509=CARTESIAN_POINT('Ctrl Pts',(-71.0529489935959,-4.97385367675157,
0.));
#144510=CARTESIAN_POINT('Ctrl Pts',(-71.0529489935959,-4.97385367675157,
12.));
#144511=CARTESIAN_POINT('Ctrl Pts',(-71.031180929482,-4.97935426748577,
0.));
#144512=CARTESIAN_POINT('Ctrl Pts',(-71.031180929482,-4.97935426748577,
12.));
#144513=CARTESIAN_POINT('Ctrl Pts',(-71.0094520872375,-4.98482159331851,
0.));
#144514=CARTESIAN_POINT('Ctrl Pts',(-71.0094520872375,-4.98482159331851,
12.));
#144515=CARTESIAN_POINT('Ctrl Pts',(-70.9877626211112,-4.99025568790652,
0.));
#144516=CARTESIAN_POINT('Ctrl Pts',(-70.9877626211112,-4.99025568790652,
12.));
#144517=CARTESIAN_POINT('Ctrl Pts',(-70.9661126860773,-4.99565658516905,
0.));
#144518=CARTESIAN_POINT('Ctrl Pts',(-70.9661126860773,-4.99565658516905,
12.));
#144519=CARTESIAN_POINT('Ctrl Pts',(-70.9445024378439,-5.00102431929039,
0.));
#144520=CARTESIAN_POINT('Ctrl Pts',(-70.9445024378439,-5.00102431929039,
12.));
#144521=CARTESIAN_POINT('Ctrl Pts',(-70.9229320328588,-5.00635892472517,
0.));
#144522=CARTESIAN_POINT('Ctrl Pts',(-70.9229320328588,-5.00635892472517,
12.));
#144523=CARTESIAN_POINT('Ctrl Pts',(-70.9014016283123,-5.01166043620573,
0.));
#144524=CARTESIAN_POINT('Ctrl Pts',(-70.9014016283123,-5.01166043620573,
12.));
#144525=CARTESIAN_POINT('Ctrl Pts',(-70.8799113821449,-5.01692888873793,
0.));
#144526=CARTESIAN_POINT('Ctrl Pts',(-70.8799113821449,-5.01692888873793,
12.));
#144527=CARTESIAN_POINT('Ctrl Pts',(-70.8584614530517,-5.0221643176006,
0.));
#144528=CARTESIAN_POINT('Ctrl Pts',(-70.8584614530517,-5.0221643176006,
12.));
#144529=CARTESIAN_POINT('Ctrl Pts',(-70.8370520004844,-5.02736675834691,
0.));
#144530=CARTESIAN_POINT('Ctrl Pts',(-70.8370520004844,-5.02736675834691,
12.));
#144531=CARTESIAN_POINT('Ctrl Pts',(-70.8156831846494,-5.0325362468094,
0.));
#144532=CARTESIAN_POINT('Ctrl Pts',(-70.8156831846494,-5.0325362468094,
12.));
#144533=CARTESIAN_POINT('Ctrl Pts',(-70.7943551665071,-5.03767281910483,
0.));
#144534=CARTESIAN_POINT('Ctrl Pts',(-70.7943551665071,-5.03767281910483,
12.));
#144535=CARTESIAN_POINT('Ctrl Pts',(-70.7730681077997,-5.04277651163356,
0.));
#144536=CARTESIAN_POINT('Ctrl Pts',(-70.7730681077997,-5.04277651163356,
12.));
#144537=CARTESIAN_POINT('Ctrl Pts',(-70.7518221710715,-5.04784736108351,
0.));
#144538=CARTESIAN_POINT('Ctrl Pts',(-70.7518221710715,-5.04784736108351,
12.));
#144539=CARTESIAN_POINT('Ctrl Pts',(-70.7306175196856,-5.05288540443477,
0.));
#144540=CARTESIAN_POINT('Ctrl Pts',(-70.7306175196856,-5.05288540443477,
12.));
#144541=CARTESIAN_POINT('Ctrl Pts',(-70.7094543178416,-5.05789067897041,
0.));
#144542=CARTESIAN_POINT('Ctrl Pts',(-70.7094543178416,-5.05789067897041,
12.));
#144543=CARTESIAN_POINT('Ctrl Pts',(-70.6883327305755,-5.06286322227796,
0.));
#144544=CARTESIAN_POINT('Ctrl Pts',(-70.6883327305755,-5.06286322227796,
12.));
#144545=CARTESIAN_POINT('Ctrl Pts',(-70.6672529237431,-5.06780307224052,
0.));
#144546=CARTESIAN_POINT('Ctrl Pts',(-70.6672529237431,-5.06780307224052,
12.));
#144547=CARTESIAN_POINT('Ctrl Pts',(-70.6462150640009,-5.0727102670335,
0.));
#144548=CARTESIAN_POINT('Ctrl Pts',(-70.6462150640009,-5.0727102670335,
12.));
#144549=CARTESIAN_POINT('Ctrl Pts',(-70.6252193187892,-5.0775848451231,
0.));
#144550=CARTESIAN_POINT('Ctrl Pts',(-70.6252193187892,-5.0775848451231,
12.));
#144551=CARTESIAN_POINT('Ctrl Pts',(-70.6042658562951,-5.08242684526704,
0.));
#144552=CARTESIAN_POINT('Ctrl Pts',(-70.6042658562951,-5.08242684526704,
12.));
#144553=CARTESIAN_POINT('Ctrl Pts',(-70.5833548455043,-5.0872363065229,
0.));
#144554=CARTESIAN_POINT('Ctrl Pts',(-70.5833548455043,-5.0872363065229,
12.));
#144555=CARTESIAN_POINT('Ctrl Pts',(-70.5624864562841,-5.09201326826146,
0.));
#144556=CARTESIAN_POINT('Ctrl Pts',(-70.5624864562841,-5.09201326826146,
12.));
#144557=CARTESIAN_POINT('Ctrl Pts',(-70.5416608594526,-5.09675777018182,
0.));
#144558=CARTESIAN_POINT('Ctrl Pts',(-70.5416608594526,-5.09675777018182,
12.));
#144559=CARTESIAN_POINT('Ctrl Pts',(-70.5208782268482,-5.10146985232928,
0.));
#144560=CARTESIAN_POINT('Ctrl Pts',(-70.5208782268482,-5.10146985232928,
12.));
#144561=CARTESIAN_POINT('Ctrl Pts',(-70.5001387313963,-5.10614955511643,
0.));
#144562=CARTESIAN_POINT('Ctrl Pts',(-70.5001387313963,-5.10614955511643,
12.));
#144563=CARTESIAN_POINT('Ctrl Pts',(-70.4794425469799,-5.11079691929192,
0.));
#144564=CARTESIAN_POINT('Ctrl Pts',(-70.4794425469799,-5.11079691929192,
12.));
#144565=CARTESIAN_POINT('Ctrl Pts',(-70.4587898482946,-5.1154119859092,
0.));
#144566=CARTESIAN_POINT('Ctrl Pts',(-70.4587898482946,-5.1154119859092,
12.));
#144567=CARTESIAN_POINT('Ctrl Pts',(-70.438180810725,-5.11999479630214,
0.));
#144568=CARTESIAN_POINT('Ctrl Pts',(-70.438180810725,-5.11999479630214,
12.));
#144569=CARTESIAN_POINT('Ctrl Pts',(-70.4176156101633,-5.12454539205346,
0.));
#144570=CARTESIAN_POINT('Ctrl Pts',(-70.4176156101633,-5.12454539205346,
12.));
#144571=CARTESIAN_POINT('Ctrl Pts',(-70.3970944229885,-5.12906381499486,
0.));
#144572=CARTESIAN_POINT('Ctrl Pts',(-70.3970944229885,-5.12906381499486,
12.));
#144573=CARTESIAN_POINT('Ctrl Pts',(-70.3766174264786,-5.1335501072859,
0.));
#144574=CARTESIAN_POINT('Ctrl Pts',(-70.3766174264786,-5.1335501072859,
12.));
#144575=CARTESIAN_POINT('Ctrl Pts',(-70.3561847991725,-5.13800431148911,
0.));
#144576=CARTESIAN_POINT('Ctrl Pts',(-70.3561847991725,-5.13800431148911,
12.));
#144577=CARTESIAN_POINT('Ctrl Pts',(-70.3357967211782,-5.14242647063467,
0.));
#144578=CARTESIAN_POINT('Ctrl Pts',(-70.3357967211782,-5.14242647063467,
12.));
#144579=CARTESIAN_POINT('Ctrl Pts',(-70.31545337467,-5.14681662833053,0.));
#144580=CARTESIAN_POINT('Ctrl Pts',(-70.31545337467,-5.14681662833053,12.));
#144581=CARTESIAN_POINT('Ctrl Pts',(-70.2951549435469,-5.15117482869224,
0.));
#144582=CARTESIAN_POINT('Ctrl Pts',(-70.2951549435469,-5.15117482869224,
12.));
#144583=CARTESIAN_POINT('Ctrl Pts',(-70.2749016125073,-5.15550111614837,
0.));
#144584=CARTESIAN_POINT('Ctrl Pts',(-70.2749016125073,-5.15550111614837,
12.));
#144585=CARTESIAN_POINT('Ctrl Pts',(-70.2546935662719,-5.159795535282,0.));
#144586=CARTESIAN_POINT('Ctrl Pts',(-70.2546935662719,-5.159795535282,12.));
#144587=CARTESIAN_POINT('Ctrl Pts',(-70.2345309887864,-5.16405813066994,
0.));
#144588=CARTESIAN_POINT('Ctrl Pts',(-70.2345309887864,-5.16405813066994,
12.));
#144589=CARTESIAN_POINT('Ctrl Pts',(-70.2144140623004,-5.16828894670139,
0.));
#144590=CARTESIAN_POINT('Ctrl Pts',(-70.2144140623004,-5.16828894670139,
12.));
#144591=CARTESIAN_POINT('Ctrl Pts',(-70.1943429691214,-5.17248802793419,
0.));
#144592=CARTESIAN_POINT('Ctrl Pts',(-70.1943429691214,-5.17248802793419,
12.));
#144593=CARTESIAN_POINT('Ctrl Pts',(-70.1743178937102,-5.17665541952399,
0.));
#144594=CARTESIAN_POINT('Ctrl Pts',(-70.1743178937102,-5.17665541952399,
12.));
#144595=CARTESIAN_POINT('Ctrl Pts',(-70.1543390243882,-5.18079116757658,
0.));
#144596=CARTESIAN_POINT('Ctrl Pts',(-70.1543390243882,-5.18079116757658,
12.));
#144597=CARTESIAN_POINT('Ctrl Pts',(-70.1344065558106,-5.18489531966234,
0.));
#144598=CARTESIAN_POINT('Ctrl Pts',(-70.1344065558106,-5.18489531966234,
12.));
#144599=CARTESIAN_POINT('Ctrl Pts',(-70.1145206891833,-5.18896792486522,
0.));
#144600=CARTESIAN_POINT('Ctrl Pts',(-70.1145206891833,-5.18896792486522,
12.));
#144601=CARTESIAN_POINT('Ctrl Pts',(-70.0946816270957,-5.19300903271544,
0.));
#144602=CARTESIAN_POINT('Ctrl Pts',(-70.0946816270957,-5.19300903271544,
12.));
#144603=CARTESIAN_POINT('Ctrl Pts',(-70.0748895689716,-5.19701869225514,
0.));
#144604=CARTESIAN_POINT('Ctrl Pts',(-70.0748895689716,-5.19701869225514,
12.));
#144605=CARTESIAN_POINT('Ctrl Pts',(-70.0551447071106,-5.20099695122677,
0.));
#144606=CARTESIAN_POINT('Ctrl Pts',(-70.0551447071106,-5.20099695122677,
12.));
#144607=CARTESIAN_POINT('Ctrl Pts',(-70.0354472203604,-5.20494385478083,
0.));
#144608=CARTESIAN_POINT('Ctrl Pts',(-70.0354472203604,-5.20494385478083,
12.));
#144609=CARTESIAN_POINT('Ctrl Pts',(-70.0157972802255,-5.20885944672914,
0.));
#144610=CARTESIAN_POINT('Ctrl Pts',(-70.0157972802255,-5.20885944672914,
12.));
#144611=CARTESIAN_POINT('Ctrl Pts',(-69.996195063002,-5.21274377203321,
0.));
#144612=CARTESIAN_POINT('Ctrl Pts',(-69.996195063002,-5.21274377203321,
12.));
#144613=CARTESIAN_POINT('Ctrl Pts',(-69.9766407595385,-5.21659687881139,
0.));
#144614=CARTESIAN_POINT('Ctrl Pts',(-69.9766407595385,-5.21659687881139,
12.));
#144615=CARTESIAN_POINT('Ctrl Pts',(-69.9571345869996,-5.22041882075626,
0.));
#144616=CARTESIAN_POINT('Ctrl Pts',(-69.9571345869996,-5.22041882075626,
12.));
#144617=CARTESIAN_POINT('Ctrl Pts',(-69.9376767968951,-5.22420965879807,
0.));
#144618=CARTESIAN_POINT('Ctrl Pts',(-69.9376767968951,-5.22420965879807,
12.));
#144619=CARTESIAN_POINT('Ctrl Pts',(-69.9182676501892,-5.22796945602602,
0.));
#144620=CARTESIAN_POINT('Ctrl Pts',(-69.9182676501892,-5.22796945602602,
12.));
#144621=CARTESIAN_POINT('Ctrl Pts',(-69.8989073936606,-5.23169827290451,
0.));
#144622=CARTESIAN_POINT('Ctrl Pts',(-69.8989073936606,-5.23169827290451,
12.));
#144623=CARTESIAN_POINT('Ctrl Pts',(-69.8795962381676,-5.23539616279714,
0.));
#144624=CARTESIAN_POINT('Ctrl Pts',(-69.8795962381676,-5.23539616279714,
12.));
#144625=CARTESIAN_POINT('Ctrl Pts',(-69.8603343303016,-5.2390631663514,
0.));
#144626=CARTESIAN_POINT('Ctrl Pts',(-69.8603343303016,-5.2390631663514,
12.));
#144627=CARTESIAN_POINT('Ctrl Pts',(-69.8411217507931,-5.24269931055075,
0.));
#144628=CARTESIAN_POINT('Ctrl Pts',(-69.8411217507931,-5.24269931055075,
12.));
#144629=CARTESIAN_POINT('Ctrl Pts',(-69.8257911792542,-5.2455835516022,
0.));
#144630=CARTESIAN_POINT('Ctrl Pts',(-69.8257911792542,-5.2455835516022,
12.));
#144631=CARTESIAN_POINT('Ctrl Pts',(-69.8143154684447,-5.24773285666673,
0.));
#144632=CARTESIAN_POINT('Ctrl Pts',(-69.8143154684447,-5.24773285666673,
12.));
#144633=CARTESIAN_POINT('Ctrl Pts',(-69.8066748687863,-5.24915955997536,
0.));
#144634=CARTESIAN_POINT('Ctrl Pts',(-69.8066748687863,-5.24915955997536,
12.));
#144635=CARTESIAN_POINT('Ctrl Pts',(-69.8028570375098,-5.24987136994591,
0.));
#144636=CARTESIAN_POINT('Ctrl Pts',(-69.8028570375098,-5.24987136994591,
12.));
#144637=CARTESIAN_POINT('',(-69.8028570375098,-5.24987136994591,12.));
#144638=CARTESIAN_POINT('Ctrl Pts',(-69.8028570375098,-5.24987136994591,
12.));
#144639=CARTESIAN_POINT('Ctrl Pts',(-69.8066748687863,-5.24915955997536,
12.));
#144640=CARTESIAN_POINT('Ctrl Pts',(-69.8143154684447,-5.24773285666673,
12.));
#144641=CARTESIAN_POINT('Ctrl Pts',(-69.8257911792542,-5.2455835516022,
12.));
#144642=CARTESIAN_POINT('Ctrl Pts',(-69.8411217507931,-5.24269931055075,
12.));
#144643=CARTESIAN_POINT('Ctrl Pts',(-69.8603343303016,-5.2390631663514,
12.));
#144644=CARTESIAN_POINT('Ctrl Pts',(-69.8795962381676,-5.23539616279714,
12.));
#144645=CARTESIAN_POINT('Ctrl Pts',(-69.8989073936606,-5.23169827290451,
12.));
#144646=CARTESIAN_POINT('Ctrl Pts',(-69.9182676501892,-5.22796945602602,
12.));
#144647=CARTESIAN_POINT('Ctrl Pts',(-69.9376767968951,-5.22420965879807,
12.));
#144648=CARTESIAN_POINT('Ctrl Pts',(-69.9571345869996,-5.22041882075626,
12.));
#144649=CARTESIAN_POINT('Ctrl Pts',(-69.9766407595385,-5.21659687881139,
12.));
#144650=CARTESIAN_POINT('Ctrl Pts',(-69.996195063002,-5.21274377203321,
12.));
#144651=CARTESIAN_POINT('Ctrl Pts',(-70.0157972802255,-5.20885944672914,
12.));
#144652=CARTESIAN_POINT('Ctrl Pts',(-70.0354472203604,-5.20494385478083,
12.));
#144653=CARTESIAN_POINT('Ctrl Pts',(-70.0551447071106,-5.20099695122677,
12.));
#144654=CARTESIAN_POINT('Ctrl Pts',(-70.0748895689716,-5.19701869225514,
12.));
#144655=CARTESIAN_POINT('Ctrl Pts',(-70.0946816270957,-5.19300903271544,
12.));
#144656=CARTESIAN_POINT('Ctrl Pts',(-70.1145206891833,-5.18896792486522,
12.));
#144657=CARTESIAN_POINT('Ctrl Pts',(-70.1344065558106,-5.18489531966234,
12.));
#144658=CARTESIAN_POINT('Ctrl Pts',(-70.1543390243882,-5.18079116757658,
12.));
#144659=CARTESIAN_POINT('Ctrl Pts',(-70.1743178937102,-5.17665541952399,
12.));
#144660=CARTESIAN_POINT('Ctrl Pts',(-70.1943429691214,-5.17248802793419,
12.));
#144661=CARTESIAN_POINT('Ctrl Pts',(-70.2144140623004,-5.16828894670139,
12.));
#144662=CARTESIAN_POINT('Ctrl Pts',(-70.2345309887864,-5.16405813066994,
12.));
#144663=CARTESIAN_POINT('Ctrl Pts',(-70.2546935662719,-5.159795535282,12.));
#144664=CARTESIAN_POINT('Ctrl Pts',(-70.2749016125073,-5.15550111614837,
12.));
#144665=CARTESIAN_POINT('Ctrl Pts',(-70.2951549435469,-5.15117482869224,
12.));
#144666=CARTESIAN_POINT('Ctrl Pts',(-70.31545337467,-5.14681662833053,12.));
#144667=CARTESIAN_POINT('Ctrl Pts',(-70.3357967211782,-5.14242647063467,
12.));
#144668=CARTESIAN_POINT('Ctrl Pts',(-70.3561847991725,-5.13800431148911,
12.));
#144669=CARTESIAN_POINT('Ctrl Pts',(-70.3766174264786,-5.1335501072859,
12.));
#144670=CARTESIAN_POINT('Ctrl Pts',(-70.3970944229885,-5.12906381499486,
12.));
#144671=CARTESIAN_POINT('Ctrl Pts',(-70.4176156101633,-5.12454539205346,
12.));
#144672=CARTESIAN_POINT('Ctrl Pts',(-70.438180810725,-5.11999479630214,
12.));
#144673=CARTESIAN_POINT('Ctrl Pts',(-70.4587898482946,-5.1154119859092,
12.));
#144674=CARTESIAN_POINT('Ctrl Pts',(-70.4794425469799,-5.11079691929192,
12.));
#144675=CARTESIAN_POINT('Ctrl Pts',(-70.5001387313963,-5.10614955511643,
12.));
#144676=CARTESIAN_POINT('Ctrl Pts',(-70.5208782268482,-5.10146985232928,
12.));
#144677=CARTESIAN_POINT('Ctrl Pts',(-70.5416608594526,-5.09675777018182,
12.));
#144678=CARTESIAN_POINT('Ctrl Pts',(-70.5624864562841,-5.09201326826146,
12.));
#144679=CARTESIAN_POINT('Ctrl Pts',(-70.5833548455043,-5.0872363065229,
12.));
#144680=CARTESIAN_POINT('Ctrl Pts',(-70.6042658562951,-5.08242684526704,
12.));
#144681=CARTESIAN_POINT('Ctrl Pts',(-70.6252193187892,-5.0775848451231,
12.));
#144682=CARTESIAN_POINT('Ctrl Pts',(-70.6462150640009,-5.0727102670335,
12.));
#144683=CARTESIAN_POINT('Ctrl Pts',(-70.6672529237431,-5.06780307224052,
12.));
#144684=CARTESIAN_POINT('Ctrl Pts',(-70.6883327305755,-5.06286322227796,
12.));
#144685=CARTESIAN_POINT('Ctrl Pts',(-70.7094543178416,-5.05789067897041,
12.));
#144686=CARTESIAN_POINT('Ctrl Pts',(-70.7306175196856,-5.05288540443477,
12.));
#144687=CARTESIAN_POINT('Ctrl Pts',(-70.7518221710715,-5.04784736108351,
12.));
#144688=CARTESIAN_POINT('Ctrl Pts',(-70.7730681077997,-5.04277651163356,
12.));
#144689=CARTESIAN_POINT('Ctrl Pts',(-70.7943551665071,-5.03767281910483,
12.));
#144690=CARTESIAN_POINT('Ctrl Pts',(-70.8156831846494,-5.0325362468094,
12.));
#144691=CARTESIAN_POINT('Ctrl Pts',(-70.8370520004844,-5.02736675834691,
12.));
#144692=CARTESIAN_POINT('Ctrl Pts',(-70.8584614530517,-5.0221643176006,
12.));
#144693=CARTESIAN_POINT('Ctrl Pts',(-70.8799113821449,-5.01692888873793,
12.));
#144694=CARTESIAN_POINT('Ctrl Pts',(-70.9014016283123,-5.01166043620573,
12.));
#144695=CARTESIAN_POINT('Ctrl Pts',(-70.9229320328588,-5.00635892472517,
12.));
#144696=CARTESIAN_POINT('Ctrl Pts',(-70.9445024378439,-5.00102431929039,
12.));
#144697=CARTESIAN_POINT('Ctrl Pts',(-70.9661126860773,-4.99565658516905,
12.));
#144698=CARTESIAN_POINT('Ctrl Pts',(-70.9877626211112,-4.99025568790652,
12.));
#144699=CARTESIAN_POINT('Ctrl Pts',(-71.0094520872375,-4.98482159331851,
12.));
#144700=CARTESIAN_POINT('Ctrl Pts',(-71.031180929482,-4.97935426748577,
12.));
#144701=CARTESIAN_POINT('Ctrl Pts',(-71.0529489935959,-4.97385367675157,
12.));
#144702=CARTESIAN_POINT('Ctrl Pts',(-71.0747561260443,-4.96831978772201,
12.));
#144703=CARTESIAN_POINT('Ctrl Pts',(-71.0966021739922,-4.96275256726786,
12.));
#144704=CARTESIAN_POINT('Ctrl Pts',(-71.1184869853071,-4.95715198251703,
12.));
#144705=CARTESIAN_POINT('Ctrl Pts',(-71.1404104085561,-4.9515180008511,
12.));
#144706=CARTESIAN_POINT('Ctrl Pts',(-71.1623722929998,-4.94585058990336,
12.));
#144707=CARTESIAN_POINT('Ctrl Pts',(-71.184372488583,-4.94014971756097,
12.));
#144708=CARTESIAN_POINT('Ctrl Pts',(-71.206410845926,-4.93441535196593,
12.));
#144709=CARTESIAN_POINT('Ctrl Pts',(-71.2284872163248,-4.92864746150711,
12.));
#144710=CARTESIAN_POINT('Ctrl Pts',(-71.2506014517457,-4.9228460148171,
12.));
#144711=CARTESIAN_POINT('Ctrl Pts',(-71.27275340482,-4.91701098077041,12.));
#144712=CARTESIAN_POINT('Ctrl Pts',(-71.2949429288319,-4.91114232848623,
12.));
#144713=CARTESIAN_POINT('Ctrl Pts',(-71.3171698777124,-4.90524002732806,
12.));
#144714=CARTESIAN_POINT('Ctrl Pts',(-71.3394341060396,-4.89930404689599,
12.));
#144715=CARTESIAN_POINT('Ctrl Pts',(-71.3617354690342,-4.89333435702423,
12.));
#144716=CARTESIAN_POINT('Ctrl Pts',(-71.3840738225548,-4.88733092777964,
12.));
#144717=CARTESIAN_POINT('Ctrl Pts',(-71.4064490230857,-4.88129372946524,
12.));
#144718=CARTESIAN_POINT('Ctrl Pts',(-71.4288609277324,-4.8752227326188,
12.));
#144719=CARTESIAN_POINT('Ctrl Pts',(-71.4513093942216,-4.86911790800533,
12.));
#144720=CARTESIAN_POINT('Ctrl Pts',(-71.4737942808971,-4.86297922661498,
12.));
#144721=CARTESIAN_POINT('Ctrl Pts',(-71.4963154467128,-4.85680665966184,
12.));
#144722=CARTESIAN_POINT('Ctrl Pts',(-71.5188727512231,-4.85060017858786,
12.));
#144723=CARTESIAN_POINT('Ctrl Pts',(-71.5414660545778,-4.84435975506056,
12.));
#144724=CARTESIAN_POINT('Ctrl Pts',(-71.5640952175239,-4.83808536096589,
12.));
#144725=CARTESIAN_POINT('Ctrl Pts',(-71.5867601014008,-4.8317769684064,
12.));
#144726=CARTESIAN_POINT('Ctrl Pts',(-71.6094605681353,-4.8254345497002,
12.));
#144727=CARTESIAN_POINT('Ctrl Pts',(-71.6321964802297,-4.81905807738541,
12.));
#144728=CARTESIAN_POINT('Ctrl Pts',(-71.6549677007582,-4.81264752421713,
12.));
#144729=CARTESIAN_POINT('Ctrl Pts',(-71.6777740933687,-4.80620286316075,
12.));
#144730=CARTESIAN_POINT('Ctrl Pts',(-71.7006155222764,-4.7997240673901,
12.));
#144731=CARTESIAN_POINT('Ctrl Pts',(-71.723491852261,-4.79321111028676,
12.));
#144732=CARTESIAN_POINT('Ctrl Pts',(-71.7464029486563,-4.78666396544458,
12.));
#144733=CARTESIAN_POINT('Ctrl Pts',(-71.769348677346,-4.7800826066665,12.));
#144734=CARTESIAN_POINT('Ctrl Pts',(-71.7923289047643,-4.77346700795792,
12.));
#144735=CARTESIAN_POINT('Ctrl Pts',(-71.8153434978923,-4.76681714352502,
12.));
#144736=CARTESIAN_POINT('Ctrl Pts',(-71.8383923242531,-4.76013298777419,
12.));
#144737=CARTESIAN_POINT('Ctrl Pts',(-71.8614752519008,-4.75341451531669,
12.));
#144738=CARTESIAN_POINT('Ctrl Pts',(-71.8845921494189,-4.74666170096547,
12.));
#144739=CARTESIAN_POINT('Ctrl Pts',(-71.9077428859212,-4.73987451972863,
12.));
#144740=CARTESIAN_POINT('Ctrl Pts',(-71.9309273310471,-4.73305294680785,
12.));
#144741=CARTESIAN_POINT('Ctrl Pts',(-71.9541453549579,-4.72619695759774,
12.));
#144742=CARTESIAN_POINT('Ctrl Pts',(-71.9773968283259,-4.7193065276907,
12.));
#144743=CARTESIAN_POINT('Ctrl Pts',(-72.0006816223325,-4.71238163287396,
12.));
#144744=CARTESIAN_POINT('Ctrl Pts',(-72.0239996086686,-4.705422249123,12.));
#144745=CARTESIAN_POINT('Ctrl Pts',(-72.0473506595318,-4.69842835259992,
12.));
#144746=CARTESIAN_POINT('Ctrl Pts',(-72.0707346476213,-4.69139991965283,
12.));
#144747=CARTESIAN_POINT('Ctrl Pts',(-72.0941514461287,-4.68433692682068,
12.));
#144748=CARTESIAN_POINT('Ctrl Pts',(-72.1176009287351,-4.67723935083094,
12.));
#144749=CARTESIAN_POINT('Ctrl Pts',(-72.1410829696128,-4.67010716859285,
12.));
#144750=CARTESIAN_POINT('Ctrl Pts',(-72.1645974434216,-4.66294035719569,
12.));
#144751=CARTESIAN_POINT('Ctrl Pts',(-72.1881442253053,-4.65573889390822,
12.));
#144752=CARTESIAN_POINT('Ctrl Pts',(-72.2117231908822,-4.64850275618323,
12.));
#144753=CARTESIAN_POINT('Ctrl Pts',(-72.2353342162417,-4.64123192165627,
12.));
#144754=CARTESIAN_POINT('Ctrl Pts',(-72.2589771779456,-4.63392636813843,
12.));
#144755=CARTESIAN_POINT('Ctrl Pts',(-72.2826519530259,-4.62658607361466,
12.));
#144756=CARTESIAN_POINT('Ctrl Pts',(-72.3063584189807,-4.61921101624292,
12.));
#144757=CARTESIAN_POINT('Ctrl Pts',(-72.3300964537658,-4.61180117435862,
12.));
#144758=CARTESIAN_POINT('Ctrl Pts',(-72.3538659357913,-4.60435652647453,
12.));
#144759=CARTESIAN_POINT('Ctrl Pts',(-72.3776667439227,-4.5968770512733,
12.));
#144760=CARTESIAN_POINT('Ctrl Pts',(-72.401498757478,-4.58936272760544,
12.));
#144761=CARTESIAN_POINT('Ctrl Pts',(-72.4253618562252,-4.58181353448851,
12.));
#144762=CARTESIAN_POINT('Ctrl Pts',(-72.4492559203745,-4.57422945111102,
12.));
#144763=CARTESIAN_POINT('Ctrl Pts',(-72.4731808305728,-4.56661045683376,
12.));
#144764=CARTESIAN_POINT('Ctrl Pts',(-72.4971364679068,-4.5589565311822,
12.));
#144765=CARTESIAN_POINT('Ctrl Pts',(-72.5211227139001,-4.55126765384404,
12.));
#144766=CARTESIAN_POINT('Ctrl Pts',(-72.5451394505104,-4.54354380466822,
12.));
#144767=CARTESIAN_POINT('Ctrl Pts',(-72.5691865601223,-4.53578496366799,
12.));
#144768=CARTESIAN_POINT('Ctrl Pts',(-72.5932639255409,-4.52799111102391,
12.));
#144769=CARTESIAN_POINT('Ctrl Pts',(-72.6173714299942,-4.52016222707637,
12.));
#144770=CARTESIAN_POINT('Ctrl Pts',(-72.6415089571321,-4.51229829232264,
12.));
#144771=CARTESIAN_POINT('Ctrl Pts',(-72.6656763910241,-4.50439928741604,
12.));
#144772=CARTESIAN_POINT('Ctrl Pts',(-72.6898736161542,-4.49646519316812,
12.));
#144773=CARTESIAN_POINT('Ctrl Pts',(-72.714100517414,-4.48849599055337,
12.));
#144774=CARTESIAN_POINT('Ctrl Pts',(-72.738356980103,-4.48049166070205,
12.));
#144775=CARTESIAN_POINT('Ctrl Pts',(-72.7626428899281,-4.47245218489609,
12.));
#144776=CARTESIAN_POINT('Ctrl Pts',(-72.7869581329994,-4.46437754456792,
12.));
#144777=CARTESIAN_POINT('Ctrl Pts',(-72.8113025958262,-4.45626772130146,
12.));
#144778=CARTESIAN_POINT('Ctrl Pts',(-72.8356761653069,-4.44812269683737,
12.));
#144779=CARTESIAN_POINT('Ctrl Pts',(-72.8600787287318,-4.43994245306818,
12.));
#144780=CARTESIAN_POINT('Ctrl Pts',(-72.8845101737855,-4.43172697203349,
12.));
#144781=CARTESIAN_POINT('Ctrl Pts',(-72.9089703885462,-4.42347623591941,
12.));
#144782=CARTESIAN_POINT('Ctrl Pts',(-72.9334592614829,-4.41519022705921,
12.));
#144783=CARTESIAN_POINT('Ctrl Pts',(-72.95797668145,-4.40686892793957,12.));
#144784=CARTESIAN_POINT('Ctrl Pts',(-72.9825225376846,-4.39851232119722,
12.));
#144785=CARTESIAN_POINT('Ctrl Pts',(-73.007096719804,-4.39012038961139,
12.));
#144786=CARTESIAN_POINT('Ctrl Pts',(-73.0316991177993,-4.3816931161015,
12.));
#144787=CARTESIAN_POINT('Ctrl Pts',(-73.0563296220299,-4.37323048372607,
12.));
#144788=CARTESIAN_POINT('Ctrl Pts',(-73.0809881232103,-4.36473247568641,
12.));
#144789=CARTESIAN_POINT('Ctrl Pts',(-73.1056745124087,-4.35619907532719,
12.));
#144790=CARTESIAN_POINT('Ctrl Pts',(-73.130388681059,-4.34763026613157,
12.));
#144791=CARTESIAN_POINT('Ctrl Pts',(-73.1551305209685,-4.3390260317214,
12.));
#144792=CARTESIAN_POINT('Ctrl Pts',(-73.1798999243235,-4.33038635585876,
12.));
#144793=CARTESIAN_POINT('Ctrl Pts',(-73.204696783694,-4.32171122245214,
12.));
#144794=CARTESIAN_POINT('Ctrl Pts',(-73.2295209920334,-4.31300061556098,
12.));
#144795=CARTESIAN_POINT('Ctrl Pts',(-73.2543724426577,-4.3042545193823,
12.));
#144796=CARTESIAN_POINT('Ctrl Pts',(-73.2792510292254,-4.29547291824287,
12.));
#144797=CARTESIAN_POINT('Ctrl Pts',(-73.3041566457135,-4.28665579659301,
12.));
#144798=CARTESIAN_POINT('Ctrl Pts',(-73.3290891863949,-4.27780313900389,
12.));
#144799=CARTESIAN_POINT('Ctrl Pts',(-73.3540485458065,-4.26891493016699,
12.));
#144800=CARTESIAN_POINT('Ctrl Pts',(-73.3790346187938,-4.25999115489899,
12.));
#144801=CARTESIAN_POINT('Ctrl Pts',(-73.4040473005592,-4.25103179814886,
12.));
#144802=CARTESIAN_POINT('Ctrl Pts',(-73.4290864867101,-4.24203684500938,
12.));
#144803=CARTESIAN_POINT('Ctrl Pts',(-73.4541520732948,-4.23300628072758,
12.));
#144804=CARTESIAN_POINT('Ctrl Pts',(-73.4792439568633,-4.22394009072756,
12.));
#144805=CARTESIAN_POINT('Ctrl Pts',(-73.5043620344116,-4.21483826059441,
12.));
#144806=CARTESIAN_POINT('Ctrl Pts',(-73.5295062032628,-4.2057007760373,
12.));
#144807=CARTESIAN_POINT('Ctrl Pts',(-73.5546763609572,-4.19652762286126,
12.));
#144808=CARTESIAN_POINT('Ctrl Pts',(-73.5798724051519,-4.18731878694236,
12.));
#144809=CARTESIAN_POINT('Ctrl Pts',(-73.6050942334768,-4.17807425419812,
12.));
#144810=CARTESIAN_POINT('Ctrl Pts',(-73.6303417435251,-4.1687940105878,
12.));
#144811=CARTESIAN_POINT('Ctrl Pts',(-73.6556148331489,-4.15947804217783,
12.));
#144812=CARTESIAN_POINT('Ctrl Pts',(-73.6809134006897,-4.15012633519723,
12.));
#144813=CARTESIAN_POINT('Ctrl Pts',(-73.7062373452342,-4.14073887610153,
12.));
#144814=CARTESIAN_POINT('Ctrl Pts',(-73.7315865668522,-4.13131565163578,
12.));
#144815=CARTESIAN_POINT('Ctrl Pts',(-73.7569609668528,-4.12185664890556,
12.));
#144816=CARTESIAN_POINT('Ctrl Pts',(-73.7823604472159,-4.11236185522787,
12.));
#144817=CARTESIAN_POINT('Ctrl Pts',(-73.8077849100342,-4.10283125798729,
12.));
#144818=CARTESIAN_POINT('Ctrl Pts',(-73.8332342568989,-4.09326484448232,
12.));
#144819=CARTESIAN_POINT('Ctrl Pts',(-73.8587083884191,-4.08366260180674,
12.));
#144820=CARTESIAN_POINT('Ctrl Pts',(-73.8842072034008,-4.07402451665244,
12.));
#144821=CARTESIAN_POINT('Ctrl Pts',(-73.9097305995115,-4.06435057547324,
12.));
#144822=CARTESIAN_POINT('Ctrl Pts',(-73.9352784747608,-4.05464076484752,
12.));
#144823=CARTESIAN_POINT('Ctrl Pts',(-73.9608507287909,-4.04489507179957,
12.));
#144824=CARTESIAN_POINT('Ctrl Pts',(-73.9864472641033,-4.03511348410659,
12.));
#144825=CARTESIAN_POINT('Ctrl Pts',(-74.012067987646,-4.02529599070094,
12.));
#144826=CARTESIAN_POINT('Ctrl Pts',(-74.0377128111863,-4.0154425817671,
12.));
#144827=CARTESIAN_POINT('Ctrl Pts',(-74.059715978211,-4.00696550627363,
12.));
#144828=CARTESIAN_POINT('Ctrl Pts',(-74.0765982943677,-4.0004468971198,
12.));
#144829=CARTESIAN_POINT('Ctrl Pts',(-74.0883491449956,-3.99590266746987,
12.));
#144830=CARTESIAN_POINT('Ctrl Pts',(-74.0949615399621,-3.99334334445522,
12.));
#144831=CARTESIAN_POINT('Ctrl Pts',(-74.0964320766209,-3.99277406490865,
12.));
#144832=CARTESIAN_POINT('',(-69.8028570375098,-5.24987136994591,0.));
#144833=CARTESIAN_POINT('',(-69.8028570375097,-5.24987136994591,0.));
#144834=CARTESIAN_POINT('Ctrl Pts',(-74.0964320766209,-3.99277406490865,
0.));
#144835=CARTESIAN_POINT('Ctrl Pts',(-74.094961539962,-3.99334334445523,
0.));
#144836=CARTESIAN_POINT('Ctrl Pts',(-74.0883491449955,-3.99590266746987,
0.));
#144837=CARTESIAN_POINT('Ctrl Pts',(-74.0765982943677,-4.0004468971198,
0.));
#144838=CARTESIAN_POINT('Ctrl Pts',(-74.059715978211,-4.00696550627363,
0.));
#144839=CARTESIAN_POINT('Ctrl Pts',(-74.0377128111863,-4.0154425817671,
0.));
#144840=CARTESIAN_POINT('Ctrl Pts',(-74.012067987646,-4.02529599070094,
0.));
#144841=CARTESIAN_POINT('Ctrl Pts',(-73.9864472641033,-4.03511348410659,
0.));
#144842=CARTESIAN_POINT('Ctrl Pts',(-73.9608507287909,-4.04489507179957,
0.));
#144843=CARTESIAN_POINT('Ctrl Pts',(-73.9352784747608,-4.05464076484752,
0.));
#144844=CARTESIAN_POINT('Ctrl Pts',(-73.9097305995115,-4.06435057547324,
0.));
#144845=CARTESIAN_POINT('Ctrl Pts',(-73.8842072034008,-4.07402451665244,
0.));
#144846=CARTESIAN_POINT('Ctrl Pts',(-73.8587083884191,-4.08366260180674,
0.));
#144847=CARTESIAN_POINT('Ctrl Pts',(-73.8332342568989,-4.09326484448232,
0.));
#144848=CARTESIAN_POINT('Ctrl Pts',(-73.8077849100342,-4.10283125798729,
0.));
#144849=CARTESIAN_POINT('Ctrl Pts',(-73.7823604472159,-4.11236185522787,
0.));
#144850=CARTESIAN_POINT('Ctrl Pts',(-73.7569609668528,-4.12185664890556,
0.));
#144851=CARTESIAN_POINT('Ctrl Pts',(-73.7315865668522,-4.13131565163578,
0.));
#144852=CARTESIAN_POINT('Ctrl Pts',(-73.7062373452342,-4.14073887610153,
0.));
#144853=CARTESIAN_POINT('Ctrl Pts',(-73.6809134006897,-4.15012633519723,
0.));
#144854=CARTESIAN_POINT('Ctrl Pts',(-73.6556148331489,-4.15947804217783,
0.));
#144855=CARTESIAN_POINT('Ctrl Pts',(-73.6303417435251,-4.1687940105878,
0.));
#144856=CARTESIAN_POINT('Ctrl Pts',(-73.6050942334768,-4.17807425419812,
0.));
#144857=CARTESIAN_POINT('Ctrl Pts',(-73.5798724051519,-4.18731878694236,
0.));
#144858=CARTESIAN_POINT('Ctrl Pts',(-73.5546763609572,-4.19652762286126,
0.));
#144859=CARTESIAN_POINT('Ctrl Pts',(-73.5295062032628,-4.2057007760373,
0.));
#144860=CARTESIAN_POINT('Ctrl Pts',(-73.5043620344116,-4.21483826059441,
0.));
#144861=CARTESIAN_POINT('Ctrl Pts',(-73.4792439568633,-4.22394009072756,
0.));
#144862=CARTESIAN_POINT('Ctrl Pts',(-73.4541520732948,-4.23300628072758,
0.));
#144863=CARTESIAN_POINT('Ctrl Pts',(-73.4290864867101,-4.24203684500938,
0.));
#144864=CARTESIAN_POINT('Ctrl Pts',(-73.4040473005592,-4.25103179814886,
0.));
#144865=CARTESIAN_POINT('Ctrl Pts',(-73.3790346187938,-4.25999115489899,
0.));
#144866=CARTESIAN_POINT('Ctrl Pts',(-73.3540485458065,-4.26891493016699,
0.));
#144867=CARTESIAN_POINT('Ctrl Pts',(-73.3290891863949,-4.27780313900389,
0.));
#144868=CARTESIAN_POINT('Ctrl Pts',(-73.3041566457135,-4.28665579659301,
0.));
#144869=CARTESIAN_POINT('Ctrl Pts',(-73.2792510292254,-4.29547291824287,
0.));
#144870=CARTESIAN_POINT('Ctrl Pts',(-73.2543724426577,-4.3042545193823,
0.));
#144871=CARTESIAN_POINT('Ctrl Pts',(-73.2295209920334,-4.31300061556098,
0.));
#144872=CARTESIAN_POINT('Ctrl Pts',(-73.204696783694,-4.32171122245214,
0.));
#144873=CARTESIAN_POINT('Ctrl Pts',(-73.1798999243235,-4.33038635585876,
0.));
#144874=CARTESIAN_POINT('Ctrl Pts',(-73.1551305209685,-4.3390260317214,
0.));
#144875=CARTESIAN_POINT('Ctrl Pts',(-73.130388681059,-4.34763026613157,
0.));
#144876=CARTESIAN_POINT('Ctrl Pts',(-73.1056745124087,-4.35619907532719,
0.));
#144877=CARTESIAN_POINT('Ctrl Pts',(-73.0809881232103,-4.36473247568641,
0.));
#144878=CARTESIAN_POINT('Ctrl Pts',(-73.0563296220299,-4.37323048372607,
0.));
#144879=CARTESIAN_POINT('Ctrl Pts',(-73.0316991177993,-4.3816931161015,
0.));
#144880=CARTESIAN_POINT('Ctrl Pts',(-73.007096719804,-4.39012038961139,
0.));
#144881=CARTESIAN_POINT('Ctrl Pts',(-72.9825225376846,-4.39851232119722,
0.));
#144882=CARTESIAN_POINT('Ctrl Pts',(-72.95797668145,-4.40686892793957,0.));
#144883=CARTESIAN_POINT('Ctrl Pts',(-72.9334592614829,-4.41519022705921,
0.));
#144884=CARTESIAN_POINT('Ctrl Pts',(-72.9089703885462,-4.42347623591941,
0.));
#144885=CARTESIAN_POINT('Ctrl Pts',(-72.8845101737855,-4.43172697203349,
0.));
#144886=CARTESIAN_POINT('Ctrl Pts',(-72.8600787287318,-4.43994245306818,
0.));
#144887=CARTESIAN_POINT('Ctrl Pts',(-72.8356761653069,-4.44812269683737,
0.));
#144888=CARTESIAN_POINT('Ctrl Pts',(-72.8113025958262,-4.45626772130146,
0.));
#144889=CARTESIAN_POINT('Ctrl Pts',(-72.7869581329994,-4.46437754456792,
0.));
#144890=CARTESIAN_POINT('Ctrl Pts',(-72.7626428899281,-4.47245218489609,
0.));
#144891=CARTESIAN_POINT('Ctrl Pts',(-72.738356980103,-4.48049166070205,
0.));
#144892=CARTESIAN_POINT('Ctrl Pts',(-72.714100517414,-4.48849599055337,
0.));
#144893=CARTESIAN_POINT('Ctrl Pts',(-72.6898736161542,-4.49646519316812,
0.));
#144894=CARTESIAN_POINT('Ctrl Pts',(-72.6656763910241,-4.50439928741604,
0.));
#144895=CARTESIAN_POINT('Ctrl Pts',(-72.6415089571321,-4.51229829232264,
0.));
#144896=CARTESIAN_POINT('Ctrl Pts',(-72.6173714299942,-4.52016222707637,
0.));
#144897=CARTESIAN_POINT('Ctrl Pts',(-72.5932639255409,-4.52799111102391,
0.));
#144898=CARTESIAN_POINT('Ctrl Pts',(-72.5691865601223,-4.53578496366799,
0.));
#144899=CARTESIAN_POINT('Ctrl Pts',(-72.5451394505104,-4.54354380466822,
0.));
#144900=CARTESIAN_POINT('Ctrl Pts',(-72.5211227139001,-4.55126765384404,
0.));
#144901=CARTESIAN_POINT('Ctrl Pts',(-72.4971364679068,-4.5589565311822,
0.));
#144902=CARTESIAN_POINT('Ctrl Pts',(-72.4731808305728,-4.56661045683376,
0.));
#144903=CARTESIAN_POINT('Ctrl Pts',(-72.4492559203745,-4.57422945111102,
0.));
#144904=CARTESIAN_POINT('Ctrl Pts',(-72.4253618562252,-4.58181353448851,
0.));
#144905=CARTESIAN_POINT('Ctrl Pts',(-72.401498757478,-4.58936272760544,
0.));
#144906=CARTESIAN_POINT('Ctrl Pts',(-72.3776667439227,-4.5968770512733,
0.));
#144907=CARTESIAN_POINT('Ctrl Pts',(-72.3538659357913,-4.60435652647453,
0.));
#144908=CARTESIAN_POINT('Ctrl Pts',(-72.3300964537658,-4.61180117435862,
0.));
#144909=CARTESIAN_POINT('Ctrl Pts',(-72.3063584189807,-4.61921101624292,
0.));
#144910=CARTESIAN_POINT('Ctrl Pts',(-72.2826519530259,-4.62658607361466,
0.));
#144911=CARTESIAN_POINT('Ctrl Pts',(-72.2589771779456,-4.63392636813843,
0.));
#144912=CARTESIAN_POINT('Ctrl Pts',(-72.2353342162417,-4.64123192165627,
0.));
#144913=CARTESIAN_POINT('Ctrl Pts',(-72.2117231908822,-4.64850275618323,
0.));
#144914=CARTESIAN_POINT('Ctrl Pts',(-72.1881442253053,-4.65573889390822,
0.));
#144915=CARTESIAN_POINT('Ctrl Pts',(-72.1645974434216,-4.66294035719569,
0.));
#144916=CARTESIAN_POINT('Ctrl Pts',(-72.1410829696128,-4.67010716859285,
0.));
#144917=CARTESIAN_POINT('Ctrl Pts',(-72.1176009287351,-4.67723935083094,
0.));
#144918=CARTESIAN_POINT('Ctrl Pts',(-72.0941514461287,-4.68433692682068,
0.));
#144919=CARTESIAN_POINT('Ctrl Pts',(-72.0707346476213,-4.69139991965283,
0.));
#144920=CARTESIAN_POINT('Ctrl Pts',(-72.0473506595318,-4.69842835259992,
0.));
#144921=CARTESIAN_POINT('Ctrl Pts',(-72.0239996086686,-4.705422249123,0.));
#144922=CARTESIAN_POINT('Ctrl Pts',(-72.0006816223325,-4.71238163287396,
0.));
#144923=CARTESIAN_POINT('Ctrl Pts',(-71.9773968283259,-4.7193065276907,
0.));
#144924=CARTESIAN_POINT('Ctrl Pts',(-71.9541453549579,-4.72619695759774,
0.));
#144925=CARTESIAN_POINT('Ctrl Pts',(-71.9309273310471,-4.73305294680785,
0.));
#144926=CARTESIAN_POINT('Ctrl Pts',(-71.9077428859212,-4.73987451972863,
0.));
#144927=CARTESIAN_POINT('Ctrl Pts',(-71.8845921494189,-4.74666170096547,
0.));
#144928=CARTESIAN_POINT('Ctrl Pts',(-71.8614752519008,-4.75341451531669,
0.));
#144929=CARTESIAN_POINT('Ctrl Pts',(-71.8383923242531,-4.76013298777419,
0.));
#144930=CARTESIAN_POINT('Ctrl Pts',(-71.8153434978923,-4.76681714352502,
0.));
#144931=CARTESIAN_POINT('Ctrl Pts',(-71.7923289047643,-4.77346700795792,
0.));
#144932=CARTESIAN_POINT('Ctrl Pts',(-71.769348677346,-4.7800826066665,0.));
#144933=CARTESIAN_POINT('Ctrl Pts',(-71.7464029486563,-4.78666396544458,
0.));
#144934=CARTESIAN_POINT('Ctrl Pts',(-71.723491852261,-4.79321111028676,
0.));
#144935=CARTESIAN_POINT('Ctrl Pts',(-71.7006155222764,-4.7997240673901,
0.));
#144936=CARTESIAN_POINT('Ctrl Pts',(-71.6777740933687,-4.80620286316075,
0.));
#144937=CARTESIAN_POINT('Ctrl Pts',(-71.6549677007582,-4.81264752421713,
0.));
#144938=CARTESIAN_POINT('Ctrl Pts',(-71.6321964802297,-4.81905807738541,
0.));
#144939=CARTESIAN_POINT('Ctrl Pts',(-71.6094605681353,-4.8254345497002,
0.));
#144940=CARTESIAN_POINT('Ctrl Pts',(-71.5867601014008,-4.8317769684064,
0.));
#144941=CARTESIAN_POINT('Ctrl Pts',(-71.5640952175239,-4.83808536096589,
0.));
#144942=CARTESIAN_POINT('Ctrl Pts',(-71.5414660545778,-4.84435975506056,
0.));
#144943=CARTESIAN_POINT('Ctrl Pts',(-71.5188727512231,-4.85060017858786,
0.));
#144944=CARTESIAN_POINT('Ctrl Pts',(-71.4963154467128,-4.85680665966184,
0.));
#144945=CARTESIAN_POINT('Ctrl Pts',(-71.4737942808971,-4.86297922661498,
0.));
#144946=CARTESIAN_POINT('Ctrl Pts',(-71.4513093942216,-4.86911790800533,
0.));
#144947=CARTESIAN_POINT('Ctrl Pts',(-71.4288609277324,-4.8752227326188,
0.));
#144948=CARTESIAN_POINT('Ctrl Pts',(-71.4064490230857,-4.88129372946524,
0.));
#144949=CARTESIAN_POINT('Ctrl Pts',(-71.3840738225548,-4.88733092777964,
0.));
#144950=CARTESIAN_POINT('Ctrl Pts',(-71.3617354690342,-4.89333435702423,
0.));
#144951=CARTESIAN_POINT('Ctrl Pts',(-71.3394341060396,-4.89930404689599,
0.));
#144952=CARTESIAN_POINT('Ctrl Pts',(-71.3171698777124,-4.90524002732806,
0.));
#144953=CARTESIAN_POINT('Ctrl Pts',(-71.2949429288319,-4.91114232848623,
0.));
#144954=CARTESIAN_POINT('Ctrl Pts',(-71.27275340482,-4.91701098077041,0.));
#144955=CARTESIAN_POINT('Ctrl Pts',(-71.2506014517457,-4.9228460148171,
0.));
#144956=CARTESIAN_POINT('Ctrl Pts',(-71.2284872163248,-4.92864746150711,
0.));
#144957=CARTESIAN_POINT('Ctrl Pts',(-71.206410845926,-4.93441535196593,
0.));
#144958=CARTESIAN_POINT('Ctrl Pts',(-71.184372488583,-4.94014971756097,
0.));
#144959=CARTESIAN_POINT('Ctrl Pts',(-71.1623722929998,-4.94585058990336,
0.));
#144960=CARTESIAN_POINT('Ctrl Pts',(-71.1404104085561,-4.9515180008511,
0.));
#144961=CARTESIAN_POINT('Ctrl Pts',(-71.1184869853071,-4.95715198251703,
0.));
#144962=CARTESIAN_POINT('Ctrl Pts',(-71.0966021739922,-4.96275256726786,
0.));
#144963=CARTESIAN_POINT('Ctrl Pts',(-71.0747561260443,-4.96831978772201,
0.));
#144964=CARTESIAN_POINT('Ctrl Pts',(-71.0529489935959,-4.97385367675157,
0.));
#144965=CARTESIAN_POINT('Ctrl Pts',(-71.031180929482,-4.97935426748577,
0.));
#144966=CARTESIAN_POINT('Ctrl Pts',(-71.0094520872375,-4.98482159331851,
0.));
#144967=CARTESIAN_POINT('Ctrl Pts',(-70.9877626211112,-4.99025568790652,
0.));
#144968=CARTESIAN_POINT('Ctrl Pts',(-70.9661126860773,-4.99565658516905,
0.));
#144969=CARTESIAN_POINT('Ctrl Pts',(-70.9445024378439,-5.00102431929039,
0.));
#144970=CARTESIAN_POINT('Ctrl Pts',(-70.9229320328588,-5.00635892472517,
0.));
#144971=CARTESIAN_POINT('Ctrl Pts',(-70.9014016283123,-5.01166043620573,
0.));
#144972=CARTESIAN_POINT('Ctrl Pts',(-70.8799113821449,-5.01692888873793,
0.));
#144973=CARTESIAN_POINT('Ctrl Pts',(-70.8584614530517,-5.0221643176006,
0.));
#144974=CARTESIAN_POINT('Ctrl Pts',(-70.8370520004844,-5.02736675834691,
0.));
#144975=CARTESIAN_POINT('Ctrl Pts',(-70.8156831846494,-5.0325362468094,
0.));
#144976=CARTESIAN_POINT('Ctrl Pts',(-70.7943551665071,-5.03767281910483,
0.));
#144977=CARTESIAN_POINT('Ctrl Pts',(-70.7730681077997,-5.04277651163356,
0.));
#144978=CARTESIAN_POINT('Ctrl Pts',(-70.7518221710715,-5.04784736108351,
0.));
#144979=CARTESIAN_POINT('Ctrl Pts',(-70.7306175196856,-5.05288540443477,
0.));
#144980=CARTESIAN_POINT('Ctrl Pts',(-70.7094543178416,-5.05789067897041,
0.));
#144981=CARTESIAN_POINT('Ctrl Pts',(-70.6883327305755,-5.06286322227796,
0.));
#144982=CARTESIAN_POINT('Ctrl Pts',(-70.6672529237431,-5.06780307224052,
0.));
#144983=CARTESIAN_POINT('Ctrl Pts',(-70.6462150640009,-5.0727102670335,
0.));
#144984=CARTESIAN_POINT('Ctrl Pts',(-70.6252193187892,-5.0775848451231,
0.));
#144985=CARTESIAN_POINT('Ctrl Pts',(-70.6042658562951,-5.08242684526704,
0.));
#144986=CARTESIAN_POINT('Ctrl Pts',(-70.5833548455043,-5.0872363065229,
0.));
#144987=CARTESIAN_POINT('Ctrl Pts',(-70.5624864562841,-5.09201326826146,
0.));
#144988=CARTESIAN_POINT('Ctrl Pts',(-70.5416608594526,-5.09675777018182,
0.));
#144989=CARTESIAN_POINT('Ctrl Pts',(-70.5208782268482,-5.10146985232928,
0.));
#144990=CARTESIAN_POINT('Ctrl Pts',(-70.5001387313963,-5.10614955511643,
0.));
#144991=CARTESIAN_POINT('Ctrl Pts',(-70.4794425469799,-5.11079691929192,
0.));
#144992=CARTESIAN_POINT('Ctrl Pts',(-70.4587898482946,-5.1154119859092,
0.));
#144993=CARTESIAN_POINT('Ctrl Pts',(-70.438180810725,-5.11999479630214,
0.));
#144994=CARTESIAN_POINT('Ctrl Pts',(-70.4176156101633,-5.12454539205346,
0.));
#144995=CARTESIAN_POINT('Ctrl Pts',(-70.3970944229885,-5.12906381499486,
0.));
#144996=CARTESIAN_POINT('Ctrl Pts',(-70.3766174264786,-5.1335501072859,
0.));
#144997=CARTESIAN_POINT('Ctrl Pts',(-70.3561847991725,-5.13800431148911,
0.));
#144998=CARTESIAN_POINT('Ctrl Pts',(-70.3357967211782,-5.14242647063467,
0.));
#144999=CARTESIAN_POINT('Ctrl Pts',(-70.31545337467,-5.14681662833053,0.));
#145000=CARTESIAN_POINT('Ctrl Pts',(-70.2951549435469,-5.15117482869224,
0.));
#145001=CARTESIAN_POINT('Ctrl Pts',(-70.2749016125073,-5.15550111614837,
0.));
#145002=CARTESIAN_POINT('Ctrl Pts',(-70.2546935662719,-5.159795535282,0.));
#145003=CARTESIAN_POINT('Ctrl Pts',(-70.2345309887864,-5.16405813066994,
0.));
#145004=CARTESIAN_POINT('Ctrl Pts',(-70.2144140623004,-5.16828894670139,
0.));
#145005=CARTESIAN_POINT('Ctrl Pts',(-70.1943429691214,-5.17248802793419,
0.));
#145006=CARTESIAN_POINT('Ctrl Pts',(-70.1743178937102,-5.17665541952399,
0.));
#145007=CARTESIAN_POINT('Ctrl Pts',(-70.1543390243882,-5.18079116757658,
0.));
#145008=CARTESIAN_POINT('Ctrl Pts',(-70.1344065558106,-5.18489531966234,
0.));
#145009=CARTESIAN_POINT('Ctrl Pts',(-70.1145206891833,-5.18896792486522,
0.));
#145010=CARTESIAN_POINT('Ctrl Pts',(-70.0946816270957,-5.19300903271544,
0.));
#145011=CARTESIAN_POINT('Ctrl Pts',(-70.0748895689716,-5.19701869225514,
0.));
#145012=CARTESIAN_POINT('Ctrl Pts',(-70.0551447071106,-5.20099695122677,
0.));
#145013=CARTESIAN_POINT('Ctrl Pts',(-70.0354472203604,-5.20494385478083,
0.));
#145014=CARTESIAN_POINT('Ctrl Pts',(-70.0157972802255,-5.20885944672914,
0.));
#145015=CARTESIAN_POINT('Ctrl Pts',(-69.996195063002,-5.21274377203321,
0.));
#145016=CARTESIAN_POINT('Ctrl Pts',(-69.9766407595385,-5.21659687881139,
0.));
#145017=CARTESIAN_POINT('Ctrl Pts',(-69.9571345869996,-5.22041882075626,
0.));
#145018=CARTESIAN_POINT('Ctrl Pts',(-69.9376767968951,-5.22420965879807,
0.));
#145019=CARTESIAN_POINT('Ctrl Pts',(-69.9182676501892,-5.22796945602602,
0.));
#145020=CARTESIAN_POINT('Ctrl Pts',(-69.8989073936606,-5.23169827290451,
0.));
#145021=CARTESIAN_POINT('Ctrl Pts',(-69.8795962381676,-5.23539616279714,
0.));
#145022=CARTESIAN_POINT('Ctrl Pts',(-69.8603343303016,-5.2390631663514,
0.));
#145023=CARTESIAN_POINT('Ctrl Pts',(-69.8411217507931,-5.24269931055075,
0.));
#145024=CARTESIAN_POINT('Ctrl Pts',(-69.8257911792542,-5.2455835516022,
0.));
#145025=CARTESIAN_POINT('Ctrl Pts',(-69.8143154684447,-5.24773285666673,
0.));
#145026=CARTESIAN_POINT('Ctrl Pts',(-69.8066748687863,-5.24915955997536,
0.));
#145027=CARTESIAN_POINT('Ctrl Pts',(-69.8028570375098,-5.24987136994591,
0.));
#145028=CARTESIAN_POINT('Ctrl Pts',(-74.4537274248118,2.62535189104656,
0.));
#145029=CARTESIAN_POINT('Ctrl Pts',(-74.4537274248118,2.62535189104656,
12.));
#145030=CARTESIAN_POINT('Ctrl Pts',(-74.4487312586601,2.62283178248297,
0.));
#145031=CARTESIAN_POINT('Ctrl Pts',(-74.4487312586601,2.62283178248297,
12.));
#145032=CARTESIAN_POINT('Ctrl Pts',(-74.4387409032582,2.6177953543237,0.));
#145033=CARTESIAN_POINT('Ctrl Pts',(-74.4387409032582,2.6177953543237,12.));
#145034=CARTESIAN_POINT('Ctrl Pts',(-74.4237613008609,2.61025207898831,
0.));
#145035=CARTESIAN_POINT('Ctrl Pts',(-74.4237613008609,2.61025207898831,
12.));
#145036=CARTESIAN_POINT('Ctrl Pts',(-74.4038003595514,2.60021711327491,
0.));
#145037=CARTESIAN_POINT('Ctrl Pts',(-74.4038003595514,2.60021711327491,
12.));
#145038=CARTESIAN_POINT('Ctrl Pts',(-74.3788689604,2.58771130268618,0.));
#145039=CARTESIAN_POINT('Ctrl Pts',(-74.3788689604,2.58771130268618,12.));
#145040=CARTESIAN_POINT('Ctrl Pts',(-74.3539573568054,2.57524339541657,
0.));
#145041=CARTESIAN_POINT('Ctrl Pts',(-74.3539573568054,2.57524339541657,
12.));
#145042=CARTESIAN_POINT('Ctrl Pts',(-74.3290655814922,2.56281339800082,
0.));
#145043=CARTESIAN_POINT('Ctrl Pts',(-74.3290655814922,2.56281339800082,
12.));
#145044=CARTESIAN_POINT('Ctrl Pts',(-74.3041936853329,2.55042131526684,
0.));
#145045=CARTESIAN_POINT('Ctrl Pts',(-74.3041936853329,2.55042131526684,
12.));
#145046=CARTESIAN_POINT('Ctrl Pts',(-74.2793417427044,2.53806714838103,
0.));
#145047=CARTESIAN_POINT('Ctrl Pts',(-74.2793417427044,2.53806714838103,
12.));
#145048=CARTESIAN_POINT('Ctrl Pts',(-74.2545098494549,2.52575089478112,
0.));
#145049=CARTESIAN_POINT('Ctrl Pts',(-74.2545098494549,2.52575089478112,
12.));
#145050=CARTESIAN_POINT('Ctrl Pts',(-74.2296981152027,2.51347254956026,
0.));
#145051=CARTESIAN_POINT('Ctrl Pts',(-74.2296981152027,2.51347254956026,
12.));
#145052=CARTESIAN_POINT('Ctrl Pts',(-74.2049066571942,2.50123210644074,
0.));
#145053=CARTESIAN_POINT('Ctrl Pts',(-74.2049066571942,2.50123210644074,
12.));
#145054=CARTESIAN_POINT('Ctrl Pts',(-74.180135593693,2.48902955888401,0.));
#145055=CARTESIAN_POINT('Ctrl Pts',(-74.180135593693,2.48902955888401,12.));
#145056=CARTESIAN_POINT('Ctrl Pts',(-74.1553850371577,2.47686490120423,
0.));
#145057=CARTESIAN_POINT('Ctrl Pts',(-74.1553850371577,2.47686490120423,
12.));
#145058=CARTESIAN_POINT('Ctrl Pts',(-74.1306550887196,2.46473812948048,
0.));
#145059=CARTESIAN_POINT('Ctrl Pts',(-74.1306550887196,2.46473812948048,
12.));
#145060=CARTESIAN_POINT('Ctrl Pts',(-74.1059458420175,2.45264924094852,
0.));
#145061=CARTESIAN_POINT('Ctrl Pts',(-74.1059458420175,2.45264924094852,
12.));
#145062=CARTESIAN_POINT('Ctrl Pts',(-74.0812573859474,2.44059823356721,
0.));
#145063=CARTESIAN_POINT('Ctrl Pts',(-74.0812573859474,2.44059823356721,
12.));
#145064=CARTESIAN_POINT('Ctrl Pts',(-74.0565898079227,2.42858510549786,
0.));
#145065=CARTESIAN_POINT('Ctrl Pts',(-74.0565898079227,2.42858510549786,
12.));
#145066=CARTESIAN_POINT('Ctrl Pts',(-74.0319431966956,2.41660985465228,
0.));
#145067=CARTESIAN_POINT('Ctrl Pts',(-74.0319431966956,2.41660985465228,
12.));
#145068=CARTESIAN_POINT('Ctrl Pts',(-74.0073176459287,2.40467247811496,
0.));
#145069=CARTESIAN_POINT('Ctrl Pts',(-74.0073176459287,2.40467247811496,
12.));
#145070=CARTESIAN_POINT('Ctrl Pts',(-73.9827132538149,2.39277297220716,
0.));
#145071=CARTESIAN_POINT('Ctrl Pts',(-73.9827132538149,2.39277297220716,
12.));
#145072=CARTESIAN_POINT('Ctrl Pts',(-73.9581301214609,2.38091133274932,
0.));
#145073=CARTESIAN_POINT('Ctrl Pts',(-73.9581301214609,2.38091133274932,
12.));
#145074=CARTESIAN_POINT('Ctrl Pts',(-73.9335683516388,2.36908755525994,
0.));
#145075=CARTESIAN_POINT('Ctrl Pts',(-73.9335683516388,2.36908755525994,
12.));
#145076=CARTESIAN_POINT('Ctrl Pts',(-73.9090280474723,2.35730163516323,
0.));
#145077=CARTESIAN_POINT('Ctrl Pts',(-73.9090280474723,2.35730163516323,
12.));
#145078=CARTESIAN_POINT('Ctrl Pts',(-73.8845093109302,2.34555356802139,
0.));
#145079=CARTESIAN_POINT('Ctrl Pts',(-73.8845093109302,2.34555356802139,
12.));
#145080=CARTESIAN_POINT('Ctrl Pts',(-73.8600122421502,2.3338433496398,0.));
#145081=CARTESIAN_POINT('Ctrl Pts',(-73.8600122421502,2.3338433496398,12.));
#145082=CARTESIAN_POINT('Ctrl Pts',(-73.8355369402733,2.32217097594215,
0.));
#145083=CARTESIAN_POINT('Ctrl Pts',(-73.8355369402733,2.32217097594215,
12.));
#145084=CARTESIAN_POINT('Ctrl Pts',(-73.8110835039341,2.31053644289425,
0.));
#145085=CARTESIAN_POINT('Ctrl Pts',(-73.8110835039341,2.31053644289425,
12.));
#145086=CARTESIAN_POINT('Ctrl Pts',(-73.7866520318849,2.29893974640434,
0.));
#145087=CARTESIAN_POINT('Ctrl Pts',(-73.7866520318849,2.29893974640434,
12.));
#145088=CARTESIAN_POINT('Ctrl Pts',(-73.7622426235648,2.28738088222858,
0.));
#145089=CARTESIAN_POINT('Ctrl Pts',(-73.7622426235648,2.28738088222858,
12.));
#145090=CARTESIAN_POINT('Ctrl Pts',(-73.7378553796792,2.27585984587192,
0.));
#145091=CARTESIAN_POINT('Ctrl Pts',(-73.7378553796792,2.27585984587192,
12.));
#145092=CARTESIAN_POINT('Ctrl Pts',(-73.7134904019378,2.26437663263663,
0.));
#145093=CARTESIAN_POINT('Ctrl Pts',(-73.7134904019378,2.26437663263663,
12.));
#145094=CARTESIAN_POINT('Ctrl Pts',(-73.6891477928124,2.25293123766424,
0.));
#145095=CARTESIAN_POINT('Ctrl Pts',(-73.6891477928124,2.25293123766424,
12.));
#145096=CARTESIAN_POINT('Ctrl Pts',(-73.6648276552766,2.24152365597698,
0.));
#145097=CARTESIAN_POINT('Ctrl Pts',(-73.6648276552766,2.24152365597698,
12.));
#145098=CARTESIAN_POINT('Ctrl Pts',(-73.6405300925714,2.23015388251288,
0.));
#145099=CARTESIAN_POINT('Ctrl Pts',(-73.6405300925714,2.23015388251288,
12.));
#145100=CARTESIAN_POINT('Ctrl Pts',(-73.6162552079044,2.2188219121652,0.));
#145101=CARTESIAN_POINT('Ctrl Pts',(-73.6162552079044,2.2188219121652,12.));
#145102=CARTESIAN_POINT('Ctrl Pts',(-73.5920031044604,2.20752773978352,
0.));
#145103=CARTESIAN_POINT('Ctrl Pts',(-73.5920031044604,2.20752773978352,
12.));
#145104=CARTESIAN_POINT('Ctrl Pts',(-73.5677738855461,2.19627136015682,
0.));
#145105=CARTESIAN_POINT('Ctrl Pts',(-73.5677738855461,2.19627136015682,
12.));
#145106=CARTESIAN_POINT('Ctrl Pts',(-73.5435676546934,2.18505276799756,
0.));
#145107=CARTESIAN_POINT('Ctrl Pts',(-73.5435676546934,2.18505276799756,
12.));
#145108=CARTESIAN_POINT('Ctrl Pts',(-73.5193845157705,2.17387195792305,
0.));
#145109=CARTESIAN_POINT('Ctrl Pts',(-73.5193845157705,2.17387195792305,
12.));
#145110=CARTESIAN_POINT('Ctrl Pts',(-73.4952245731044,2.16272892442915,
0.));
#145111=CARTESIAN_POINT('Ctrl Pts',(-73.4952245731044,2.16272892442915,
12.));
#145112=CARTESIAN_POINT('Ctrl Pts',(-73.4710879315367,2.15162366187898,
0.));
#145113=CARTESIAN_POINT('Ctrl Pts',(-73.4710879315367,2.15162366187898,
12.));
#145114=CARTESIAN_POINT('Ctrl Pts',(-73.4469746963622,2.14055616452048,
0.));
#145115=CARTESIAN_POINT('Ctrl Pts',(-73.4469746963622,2.14055616452048,
12.));
#145116=CARTESIAN_POINT('Ctrl Pts',(-73.4228849732914,2.1295264264936,0.));
#145117=CARTESIAN_POINT('Ctrl Pts',(-73.4228849732914,2.1295264264936,12.));
#145118=CARTESIAN_POINT('Ctrl Pts',(-73.3988188684022,2.11853444183763,
0.));
#145119=CARTESIAN_POINT('Ctrl Pts',(-73.3988188684022,2.11853444183763,
12.));
#145120=CARTESIAN_POINT('Ctrl Pts',(-73.3747764880903,2.107580204494,0.));
#145121=CARTESIAN_POINT('Ctrl Pts',(-73.3747764880903,2.107580204494,12.));
#145122=CARTESIAN_POINT('Ctrl Pts',(-73.3507579390254,2.09666370830733,
0.));
#145123=CARTESIAN_POINT('Ctrl Pts',(-73.3507579390254,2.09666370830733,
12.));
#145124=CARTESIAN_POINT('Ctrl Pts',(-73.3267633281822,2.08578494702761,
0.));
#145125=CARTESIAN_POINT('Ctrl Pts',(-73.3267633281822,2.08578494702761,
12.));
#145126=CARTESIAN_POINT('Ctrl Pts',(-73.3027927628636,2.07494391430953,
0.));
#145127=CARTESIAN_POINT('Ctrl Pts',(-73.3027927628636,2.07494391430953,
12.));
#145128=CARTESIAN_POINT('Ctrl Pts',(-73.2788463507248,2.06414060370837,
0.));
#145129=CARTESIAN_POINT('Ctrl Pts',(-73.2788463507248,2.06414060370837,
12.));
#145130=CARTESIAN_POINT('Ctrl Pts',(-73.2549241997946,2.05337500867395,
0.));
#145131=CARTESIAN_POINT('Ctrl Pts',(-73.2549241997946,2.05337500867395,
12.));
#145132=CARTESIAN_POINT('Ctrl Pts',(-73.2310264184965,2.04264712253915,
0.));
#145133=CARTESIAN_POINT('Ctrl Pts',(-73.2310264184965,2.04264712253915,
12.));
#145134=CARTESIAN_POINT('Ctrl Pts',(-73.2071531156492,2.0319569385244,0.));
#145135=CARTESIAN_POINT('Ctrl Pts',(-73.2071531156492,2.0319569385244,12.));
#145136=CARTESIAN_POINT('Ctrl Pts',(-73.1833044004612,2.02130444974351,
0.));
#145137=CARTESIAN_POINT('Ctrl Pts',(-73.1833044004612,2.02130444974351,
12.));
#145138=CARTESIAN_POINT('Ctrl Pts',(-73.159480382525,2.01068964920464,0.));
#145139=CARTESIAN_POINT('Ctrl Pts',(-73.159480382525,2.01068964920464,12.));
#145140=CARTESIAN_POINT('Ctrl Pts',(-73.1356811718094,2.00011252980987,
0.));
#145141=CARTESIAN_POINT('Ctrl Pts',(-73.1356811718094,2.00011252980987,
12.));
#145142=CARTESIAN_POINT('Ctrl Pts',(-73.1119068786482,1.9895730843493,0.));
#145143=CARTESIAN_POINT('Ctrl Pts',(-73.1119068786482,1.9895730843493,12.));
#145144=CARTESIAN_POINT('Ctrl Pts',(-73.0881576137414,1.97907130550172,
0.));
#145145=CARTESIAN_POINT('Ctrl Pts',(-73.0881576137414,1.97907130550172,
12.));
#145146=CARTESIAN_POINT('Ctrl Pts',(-73.0644334881679,1.96860718583944,
0.));
#145147=CARTESIAN_POINT('Ctrl Pts',(-73.0644334881679,1.96860718583944,
12.));
#145148=CARTESIAN_POINT('Ctrl Pts',(-73.0407346133912,1.95818071782773,
0.));
#145149=CARTESIAN_POINT('Ctrl Pts',(-73.0407346133912,1.95818071782773,
12.));
#145150=CARTESIAN_POINT('Ctrl Pts',(-73.0170611012659,1.947791893823,0.));
#145151=CARTESIAN_POINT('Ctrl Pts',(-73.0170611012659,1.947791893823,12.));
#145152=CARTESIAN_POINT('Ctrl Pts',(-72.9934130640414,1.93744070606557,
0.));
#145153=CARTESIAN_POINT('Ctrl Pts',(-72.9934130640414,1.93744070606557,
12.));
#145154=CARTESIAN_POINT('Ctrl Pts',(-72.9697906143638,1.92712714667648,
0.));
#145155=CARTESIAN_POINT('Ctrl Pts',(-72.9697906143638,1.92712714667648,
12.));
#145156=CARTESIAN_POINT('Ctrl Pts',(-72.9461938652816,1.91685120766427,
0.));
#145157=CARTESIAN_POINT('Ctrl Pts',(-72.9461938652816,1.91685120766427,
12.));
#145158=CARTESIAN_POINT('Ctrl Pts',(-72.9226229302483,1.90661288092582,
0.));
#145159=CARTESIAN_POINT('Ctrl Pts',(-72.9226229302483,1.90661288092582,
12.));
#145160=CARTESIAN_POINT('Ctrl Pts',(-72.8990779231226,1.89641215824584,
0.));
#145161=CARTESIAN_POINT('Ctrl Pts',(-72.8990779231226,1.89641215824584,
12.));
#145162=CARTESIAN_POINT('Ctrl Pts',(-72.8755589581674,1.88624903129195,
0.));
#145163=CARTESIAN_POINT('Ctrl Pts',(-72.8755589581674,1.88624903129195,
12.));
#145164=CARTESIAN_POINT('Ctrl Pts',(-72.8520661500465,1.87612349160952,
0.));
#145165=CARTESIAN_POINT('Ctrl Pts',(-72.8520661500465,1.87612349160952,
12.));
#145166=CARTESIAN_POINT('Ctrl Pts',(-72.8285996138346,1.86603553062776,
0.));
#145167=CARTESIAN_POINT('Ctrl Pts',(-72.8285996138346,1.86603553062776,
12.));
#145168=CARTESIAN_POINT('Ctrl Pts',(-72.8051594650214,1.85598513966115,
0.));
#145169=CARTESIAN_POINT('Ctrl Pts',(-72.8051594650214,1.85598513966115,
12.));
#145170=CARTESIAN_POINT('Ctrl Pts',(-72.7817458195155,1.84597230990858,
0.));
#145171=CARTESIAN_POINT('Ctrl Pts',(-72.7817458195155,1.84597230990858,
12.));
#145172=CARTESIAN_POINT('Ctrl Pts',(-72.7583587936454,1.83599703244926,
0.));
#145173=CARTESIAN_POINT('Ctrl Pts',(-72.7583587936454,1.83599703244926,
12.));
#145174=CARTESIAN_POINT('Ctrl Pts',(-72.73499850416,1.82605929823565,0.));
#145175=CARTESIAN_POINT('Ctrl Pts',(-72.73499850416,1.82605929823565,12.));
#145176=CARTESIAN_POINT('Ctrl Pts',(-72.7116650682347,1.81615909809871,
0.));
#145177=CARTESIAN_POINT('Ctrl Pts',(-72.7116650682347,1.81615909809871,
12.));
#145178=CARTESIAN_POINT('Ctrl Pts',(-72.6883586034768,1.80629642275051,
0.));
#145179=CARTESIAN_POINT('Ctrl Pts',(-72.6883586034768,1.80629642275051,
12.));
#145180=CARTESIAN_POINT('Ctrl Pts',(-72.6650792279271,1.79647126278359,
0.));
#145181=CARTESIAN_POINT('Ctrl Pts',(-72.6650792279271,1.79647126278359,
12.));
#145182=CARTESIAN_POINT('Ctrl Pts',(-72.6418270600623,1.78668360866813,
0.));
#145183=CARTESIAN_POINT('Ctrl Pts',(-72.6418270600623,1.78668360866813,
12.));
#145184=CARTESIAN_POINT('Ctrl Pts',(-72.618602218792,1.7769334507443,0.));
#145185=CARTESIAN_POINT('Ctrl Pts',(-72.618602218792,1.7769334507443,12.));
#145186=CARTESIAN_POINT('Ctrl Pts',(-72.5954048234655,1.76722077922579,
0.));
#145187=CARTESIAN_POINT('Ctrl Pts',(-72.5954048234655,1.76722077922579,
12.));
#145188=CARTESIAN_POINT('Ctrl Pts',(-72.5722349938789,1.75754558420349,
0.));
#145189=CARTESIAN_POINT('Ctrl Pts',(-72.5722349938789,1.75754558420349,
12.));
#145190=CARTESIAN_POINT('Ctrl Pts',(-72.5490928502773,1.74790785564476,
0.));
#145191=CARTESIAN_POINT('Ctrl Pts',(-72.5490928502773,1.74790785564476,
12.));
#145192=CARTESIAN_POINT('Ctrl Pts',(-72.5259785133586,1.73830758339123,
0.));
#145193=CARTESIAN_POINT('Ctrl Pts',(-72.5259785133586,1.73830758339123,
12.));
#145194=CARTESIAN_POINT('Ctrl Pts',(-72.5028921042704,1.72874475715098,
0.));
#145195=CARTESIAN_POINT('Ctrl Pts',(-72.5028921042704,1.72874475715098,
12.));
#145196=CARTESIAN_POINT('Ctrl Pts',(-72.4798337446162,1.71921936650032,
0.));
#145197=CARTESIAN_POINT('Ctrl Pts',(-72.4798337446162,1.71921936650032,
12.));
#145198=CARTESIAN_POINT('Ctrl Pts',(-72.4568035564618,1.70973140088837,
0.));
#145199=CARTESIAN_POINT('Ctrl Pts',(-72.4568035564618,1.70973140088837,
12.));
#145200=CARTESIAN_POINT('Ctrl Pts',(-72.4338016623388,1.70028084963646,
0.));
#145201=CARTESIAN_POINT('Ctrl Pts',(-72.4338016623388,1.70028084963646,
12.));
#145202=CARTESIAN_POINT('Ctrl Pts',(-72.4108281852473,1.6908677019364,0.));
#145203=CARTESIAN_POINT('Ctrl Pts',(-72.4108281852473,1.6908677019364,12.));
#145204=CARTESIAN_POINT('Ctrl Pts',(-72.3878832486549,1.68149194684288,
0.));
#145205=CARTESIAN_POINT('Ctrl Pts',(-72.3878832486549,1.68149194684288,
12.));
#145206=CARTESIAN_POINT('Ctrl Pts',(-72.3649669765013,1.67215357327372,
0.));
#145207=CARTESIAN_POINT('Ctrl Pts',(-72.3649669765013,1.67215357327372,
12.));
#145208=CARTESIAN_POINT('Ctrl Pts',(-72.3420794932052,1.66285257001502,
0.));
#145209=CARTESIAN_POINT('Ctrl Pts',(-72.3420794932052,1.66285257001502,
12.));
#145210=CARTESIAN_POINT('Ctrl Pts',(-72.3192209236691,1.65358892572065,
0.));
#145211=CARTESIAN_POINT('Ctrl Pts',(-72.3192209236691,1.65358892572065,
12.));
#145212=CARTESIAN_POINT('Ctrl Pts',(-72.2963913932811,1.64436262891078,
0.));
#145213=CARTESIAN_POINT('Ctrl Pts',(-72.2963913932811,1.64436262891078,
12.));
#145214=CARTESIAN_POINT('Ctrl Pts',(-72.2735910279149,1.63517366796458,
0.));
#145215=CARTESIAN_POINT('Ctrl Pts',(-72.2735910279149,1.63517366796458,
12.));
#145216=CARTESIAN_POINT('Ctrl Pts',(-72.2508199539325,1.62602203111924,
0.));
#145217=CARTESIAN_POINT('Ctrl Pts',(-72.2508199539325,1.62602203111924,
12.));
#145218=CARTESIAN_POINT('Ctrl Pts',(-72.2280782981941,1.61690770647535,
0.));
#145219=CARTESIAN_POINT('Ctrl Pts',(-72.2280782981941,1.61690770647535,
12.));
#145220=CARTESIAN_POINT('Ctrl Pts',(-72.2053661880611,1.60783068199661,
0.));
#145221=CARTESIAN_POINT('Ctrl Pts',(-72.2053661880611,1.60783068199661,
12.));
#145222=CARTESIAN_POINT('Ctrl Pts',(-72.1826837514,1.59879094550849,0.));
#145223=CARTESIAN_POINT('Ctrl Pts',(-72.1826837514,1.59879094550849,12.));
#145224=CARTESIAN_POINT('Ctrl Pts',(-72.1600311165813,1.58978848469128,
0.));
#145225=CARTESIAN_POINT('Ctrl Pts',(-72.1600311165813,1.58978848469128,
12.));
#145226=CARTESIAN_POINT('Ctrl Pts',(-72.1374084124829,1.58082328707808,
0.));
#145227=CARTESIAN_POINT('Ctrl Pts',(-72.1374084124829,1.58082328707808,
12.));
#145228=CARTESIAN_POINT('Ctrl Pts',(-72.1148157684987,1.57189534006043,
0.));
#145229=CARTESIAN_POINT('Ctrl Pts',(-72.1148157684987,1.57189534006043,
12.));
#145230=CARTESIAN_POINT('Ctrl Pts',(-72.092253314543,1.56300463088811,0.));
#145231=CARTESIAN_POINT('Ctrl Pts',(-72.092253314543,1.56300463088811,12.));
#145232=CARTESIAN_POINT('Ctrl Pts',(-72.0697211810548,1.55415114666774,
0.));
#145233=CARTESIAN_POINT('Ctrl Pts',(-72.0697211810548,1.55415114666774,
12.));
#145234=CARTESIAN_POINT('Ctrl Pts',(-72.0472194989968,1.54533487435626,
0.));
#145235=CARTESIAN_POINT('Ctrl Pts',(-72.0472194989968,1.54533487435626,
12.));
#145236=CARTESIAN_POINT('Ctrl Pts',(-72.0247483998582,1.53655580075813,
0.));
#145237=CARTESIAN_POINT('Ctrl Pts',(-72.0247483998582,1.53655580075813,
12.));
#145238=CARTESIAN_POINT('Ctrl Pts',(-72.0023080156647,1.52781391253103,
0.));
#145239=CARTESIAN_POINT('Ctrl Pts',(-72.0023080156647,1.52781391253103,
12.));
#145240=CARTESIAN_POINT('Ctrl Pts',(-71.9798984789828,1.51910919618566,
0.));
#145241=CARTESIAN_POINT('Ctrl Pts',(-71.9798984789828,1.51910919618566,
12.));
#145242=CARTESIAN_POINT('Ctrl Pts',(-71.9575199229241,1.51044163808454,
0.));
#145243=CARTESIAN_POINT('Ctrl Pts',(-71.9575199229241,1.51044163808454,
12.));
#145244=CARTESIAN_POINT('Ctrl Pts',(-71.935172481145,1.50181122443535,0.));
#145245=CARTESIAN_POINT('Ctrl Pts',(-71.935172481145,1.50181122443535,12.));
#145246=CARTESIAN_POINT('Ctrl Pts',(-71.9128562878491,1.493217941288,0.));
#145247=CARTESIAN_POINT('Ctrl Pts',(-71.9128562878491,1.493217941288,12.));
#145248=CARTESIAN_POINT('Ctrl Pts',(-71.8905714777972,1.48466177454021,
0.));
#145249=CARTESIAN_POINT('Ctrl Pts',(-71.8905714777972,1.48466177454021,
12.));
#145250=CARTESIAN_POINT('Ctrl Pts',(-71.8683181863123,1.4761427099373,0.));
#145251=CARTESIAN_POINT('Ctrl Pts',(-71.8683181863123,1.4761427099373,12.));
#145252=CARTESIAN_POINT('Ctrl Pts',(-71.8460965492836,1.46766073307089,
0.));
#145253=CARTESIAN_POINT('Ctrl Pts',(-71.8460965492836,1.46766073307089,
12.));
#145254=CARTESIAN_POINT('Ctrl Pts',(-71.8239067031664,1.45921582937229,
0.));
#145255=CARTESIAN_POINT('Ctrl Pts',(-71.8239067031664,1.45921582937229,
12.));
#145256=CARTESIAN_POINT('Ctrl Pts',(-71.8017487849865,1.45080798410957,
0.));
#145257=CARTESIAN_POINT('Ctrl Pts',(-71.8017487849865,1.45080798410957,
12.));
#145258=CARTESIAN_POINT('Ctrl Pts',(-71.7796229323496,1.44243718239304,
0.));
#145259=CARTESIAN_POINT('Ctrl Pts',(-71.7796229323496,1.44243718239304,
12.));
#145260=CARTESIAN_POINT('Ctrl Pts',(-71.7575292834456,1.43410340917489,
0.));
#145261=CARTESIAN_POINT('Ctrl Pts',(-71.7575292834456,1.43410340917489,
12.));
#145262=CARTESIAN_POINT('Ctrl Pts',(-71.7354679770537,1.42580664924774,
0.));
#145263=CARTESIAN_POINT('Ctrl Pts',(-71.7354679770537,1.42580664924774,
12.));
#145264=CARTESIAN_POINT('Ctrl Pts',(-71.7134391525417,1.41754688723791,
0.));
#145265=CARTESIAN_POINT('Ctrl Pts',(-71.7134391525417,1.41754688723791,
12.));
#145266=CARTESIAN_POINT('Ctrl Pts',(-71.6914429498702,1.40932410760274,
0.));
#145267=CARTESIAN_POINT('Ctrl Pts',(-71.6914429498702,1.40932410760274,
12.));
#145268=CARTESIAN_POINT('Ctrl Pts',(-71.6694795096034,1.40113829463599,
0.));
#145269=CARTESIAN_POINT('Ctrl Pts',(-71.6694795096034,1.40113829463599,
12.));
#145270=CARTESIAN_POINT('Ctrl Pts',(-71.6475489729149,1.39298943246731,
0.));
#145271=CARTESIAN_POINT('Ctrl Pts',(-71.6475489729149,1.39298943246731,
12.));
#145272=CARTESIAN_POINT('Ctrl Pts',(-71.6256514815918,1.38487750506076,
0.));
#145273=CARTESIAN_POINT('Ctrl Pts',(-71.6256514815918,1.38487750506076,
12.));
#145274=CARTESIAN_POINT('Ctrl Pts',(-71.6037871780347,1.37680249620763,
0.));
#145275=CARTESIAN_POINT('Ctrl Pts',(-71.6037871780347,1.37680249620763,
12.));
#145276=CARTESIAN_POINT('Ctrl Pts',(-71.5819562052613,1.36876438952448,
0.));
#145277=CARTESIAN_POINT('Ctrl Pts',(-71.5819562052613,1.36876438952448,
12.));
#145278=CARTESIAN_POINT('Ctrl Pts',(-71.5601587069175,1.36076316845806,
0.));
#145279=CARTESIAN_POINT('Ctrl Pts',(-71.5601587069175,1.36076316845806,
12.));
#145280=CARTESIAN_POINT('Ctrl Pts',(-71.538394827283,1.35279881628453,0.));
#145281=CARTESIAN_POINT('Ctrl Pts',(-71.538394827283,1.35279881628453,12.));
#145282=CARTESIAN_POINT('Ctrl Pts',(-71.5166647112766,1.34487131610785,
0.));
#145283=CARTESIAN_POINT('Ctrl Pts',(-71.5166647112766,1.34487131610785,
12.));
#145284=CARTESIAN_POINT('Ctrl Pts',(-71.4949685044559,1.33698065085227,
0.));
#145285=CARTESIAN_POINT('Ctrl Pts',(-71.4949685044559,1.33698065085227,
12.));
#145286=CARTESIAN_POINT('Ctrl Pts',(-71.4733063530227,1.32912680326131,
0.));
#145287=CARTESIAN_POINT('Ctrl Pts',(-71.4733063530227,1.32912680326131,
12.));
#145288=CARTESIAN_POINT('Ctrl Pts',(-71.4516784038346,1.32130975590231,
0.));
#145289=CARTESIAN_POINT('Ctrl Pts',(-71.4516784038346,1.32130975590231,
12.));
#145290=CARTESIAN_POINT('Ctrl Pts',(-71.4300848044095,1.31352949116538,
0.));
#145291=CARTESIAN_POINT('Ctrl Pts',(-71.4300848044095,1.31352949116538,
12.));
#145292=CARTESIAN_POINT('Ctrl Pts',(-71.4085257029308,1.30578599126139,
0.));
#145293=CARTESIAN_POINT('Ctrl Pts',(-71.4085257029308,1.30578599126139,
12.));
#145294=CARTESIAN_POINT('Ctrl Pts',(-71.3870012482474,1.29807923821413,
0.));
#145295=CARTESIAN_POINT('Ctrl Pts',(-71.3870012482474,1.29807923821413,
12.));
#145296=CARTESIAN_POINT('Ctrl Pts',(-71.3655115898801,1.2904092138606,0.));
#145297=CARTESIAN_POINT('Ctrl Pts',(-71.3655115898801,1.2904092138606,12.));
#145298=CARTESIAN_POINT('Ctrl Pts',(-71.344056878033,1.28277589985474,0.));
#145299=CARTESIAN_POINT('Ctrl Pts',(-71.344056878033,1.28277589985474,12.));
#145300=CARTESIAN_POINT('Ctrl Pts',(-71.3226372635993,1.2751792776661,0.));
#145301=CARTESIAN_POINT('Ctrl Pts',(-71.3226372635993,1.2751792776661,12.));
#145302=CARTESIAN_POINT('Ctrl Pts',(-71.301252898167,1.26761932857723,0.));
#145303=CARTESIAN_POINT('Ctrl Pts',(-71.301252898167,1.26761932857723,12.));
#145304=CARTESIAN_POINT('Ctrl Pts',(-71.2799039340191,1.26009603367564,
0.));
#145305=CARTESIAN_POINT('Ctrl Pts',(-71.2799039340191,1.26009603367564,
12.));
#145306=CARTESIAN_POINT('Ctrl Pts',(-71.2585905241422,1.2526093738556,0.));
#145307=CARTESIAN_POINT('Ctrl Pts',(-71.2585905241422,1.2526093738556,12.));
#145308=CARTESIAN_POINT('Ctrl Pts',(-71.2373128222359,1.24515932982107,
0.));
#145309=CARTESIAN_POINT('Ctrl Pts',(-71.2373128222359,1.24515932982107,
12.));
#145310=CARTESIAN_POINT('Ctrl Pts',(-71.2160709827189,1.23774588208427,
0.));
#145311=CARTESIAN_POINT('Ctrl Pts',(-71.2160709827189,1.23774588208427,
12.));
#145312=CARTESIAN_POINT('Ctrl Pts',(-71.1948651607319,1.23036901096246,
0.));
#145313=CARTESIAN_POINT('Ctrl Pts',(-71.1948651607319,1.23036901096246,
12.));
#145314=CARTESIAN_POINT('Ctrl Pts',(-71.1736955121361,1.22302869657028,
0.));
#145315=CARTESIAN_POINT('Ctrl Pts',(-71.1736955121361,1.22302869657028,
12.));
#145316=CARTESIAN_POINT('Ctrl Pts',(-71.1525621935266,1.21572491882273,
0.));
#145317=CARTESIAN_POINT('Ctrl Pts',(-71.1525621935266,1.21572491882273,
12.));
#145318=CARTESIAN_POINT('Ctrl Pts',(-71.1314653622442,1.20845765743654,
0.));
#145319=CARTESIAN_POINT('Ctrl Pts',(-71.1314653622442,1.20845765743654,
12.));
#145320=CARTESIAN_POINT('Ctrl Pts',(-71.1104051763839,1.20122689192836,
0.));
#145321=CARTESIAN_POINT('Ctrl Pts',(-71.1104051763839,1.20122689192836,
12.));
#145322=CARTESIAN_POINT('Ctrl Pts',(-71.089381794801,1.19403260160997,0.));
#145323=CARTESIAN_POINT('Ctrl Pts',(-71.089381794801,1.19403260160997,12.));
#145324=CARTESIAN_POINT('Ctrl Pts',(-71.0683953771147,1.18687476558126,
0.));
#145325=CARTESIAN_POINT('Ctrl Pts',(-71.0683953771147,1.18687476558126,
12.));
#145326=CARTESIAN_POINT('Ctrl Pts',(-71.0474460837157,1.17975336273499,
0.));
#145327=CARTESIAN_POINT('Ctrl Pts',(-71.0474460837157,1.17975336273499,
12.));
#145328=CARTESIAN_POINT('Ctrl Pts',(-71.0265340757697,1.17266837175775,
0.));
#145329=CARTESIAN_POINT('Ctrl Pts',(-71.0265340757697,1.17266837175775,
12.));
#145330=CARTESIAN_POINT('Ctrl Pts',(-71.0056595152204,1.16561977112882,
0.));
#145331=CARTESIAN_POINT('Ctrl Pts',(-71.0056595152204,1.16561977112882,
12.));
#145332=CARTESIAN_POINT('Ctrl Pts',(-70.9848225647876,1.15860753911489,
0.));
#145333=CARTESIAN_POINT('Ctrl Pts',(-70.9848225647876,1.15860753911489,
12.));
#145334=CARTESIAN_POINT('Ctrl Pts',(-70.9640233879671,1.1516316537653,0.));
#145335=CARTESIAN_POINT('Ctrl Pts',(-70.9640233879671,1.1516316537653,12.));
#145336=CARTESIAN_POINT('Ctrl Pts',(-70.9432621490579,1.14469209291494,
0.));
#145337=CARTESIAN_POINT('Ctrl Pts',(-70.9432621490579,1.14469209291494,
12.));
#145338=CARTESIAN_POINT('Ctrl Pts',(-70.9225390131835,1.13778883418216,
0.));
#145339=CARTESIAN_POINT('Ctrl Pts',(-70.9225390131835,1.13778883418216,
12.));
#145340=CARTESIAN_POINT('Ctrl Pts',(-70.9018541463083,1.13092185496563,
0.));
#145341=CARTESIAN_POINT('Ctrl Pts',(-70.9018541463083,1.13092185496563,
12.));
#145342=CARTESIAN_POINT('Ctrl Pts',(-70.8812077152564,1.12409113243511,
0.));
#145343=CARTESIAN_POINT('Ctrl Pts',(-70.8812077152564,1.12409113243511,
12.));
#145344=CARTESIAN_POINT('Ctrl Pts',(-70.860599887712,1.1172966435299,0.));
#145345=CARTESIAN_POINT('Ctrl Pts',(-70.860599887712,1.1172966435299,12.));
#145346=CARTESIAN_POINT('Ctrl Pts',(-70.8400308322013,1.11053836496637,
0.));
#145347=CARTESIAN_POINT('Ctrl Pts',(-70.8400308322013,1.11053836496637,
12.));
#145348=CARTESIAN_POINT('Ctrl Pts',(-70.8195007180739,1.10381627323945,
0.));
#145349=CARTESIAN_POINT('Ctrl Pts',(-70.8195007180739,1.10381627323945,
12.));
#145350=CARTESIAN_POINT('Ctrl Pts',(-70.7990097154855,1.09713034462269,
0.));
#145351=CARTESIAN_POINT('Ctrl Pts',(-70.7990097154855,1.09713034462269,
12.));
#145352=CARTESIAN_POINT('Ctrl Pts',(-70.7785579953611,1.09048055516434,
0.));
#145353=CARTESIAN_POINT('Ctrl Pts',(-70.7785579953611,1.09048055516434,
12.));
#145354=CARTESIAN_POINT('Ctrl Pts',(-70.7581457294475,1.08386688068348,
0.));
#145355=CARTESIAN_POINT('Ctrl Pts',(-70.7581457294475,1.08386688068348,
12.));
#145356=CARTESIAN_POINT('Ctrl Pts',(-70.737773090397,1.07728929676412,0.));
#145357=CARTESIAN_POINT('Ctrl Pts',(-70.737773090397,1.07728929676412,12.));
#145358=CARTESIAN_POINT('Ctrl Pts',(-70.7174402518378,1.07074777874596,
0.));
#145359=CARTESIAN_POINT('Ctrl Pts',(-70.7174402518378,1.07074777874596,
12.));
#145360=CARTESIAN_POINT('Ctrl Pts',(-70.6971473884443,1.0642423017128,0.));
#145361=CARTESIAN_POINT('Ctrl Pts',(-70.6971473884443,1.0642423017128,12.));
#145362=CARTESIAN_POINT('Ctrl Pts',(-70.6768946760063,1.05777284047727,
0.));
#145363=CARTESIAN_POINT('Ctrl Pts',(-70.6768946760063,1.05777284047727,
12.));
#145364=CARTESIAN_POINT('Ctrl Pts',(-70.6566822912965,1.05133936960068,
0.));
#145365=CARTESIAN_POINT('Ctrl Pts',(-70.6566822912965,1.05133936960068,
12.));
#145366=CARTESIAN_POINT('Ctrl Pts',(-70.6365104119238,1.04494186341155,
0.));
#145367=CARTESIAN_POINT('Ctrl Pts',(-70.6365104119238,1.04494186341155,
12.));
#145368=CARTESIAN_POINT('Ctrl Pts',(-70.6163792162079,1.03858029601905,
0.));
#145369=CARTESIAN_POINT('Ctrl Pts',(-70.6163792162079,1.03858029601905,
12.));
#145370=CARTESIAN_POINT('Ctrl Pts',(-70.5962888829958,1.03225464132872,
0.));
#145371=CARTESIAN_POINT('Ctrl Pts',(-70.5962888829958,1.03225464132872,
12.));
#145372=CARTESIAN_POINT('Ctrl Pts',(-70.5762395916412,1.02596487304049,
0.));
#145373=CARTESIAN_POINT('Ctrl Pts',(-70.5762395916412,1.02596487304049,
12.));
#145374=CARTESIAN_POINT('Ctrl Pts',(-70.5562315224219,1.01971096460599,
0.));
#145375=CARTESIAN_POINT('Ctrl Pts',(-70.5562315224219,1.01971096460599,
12.));
#145376=CARTESIAN_POINT('Ctrl Pts',(-70.5362648569072,1.01349288918539,
0.));
#145377=CARTESIAN_POINT('Ctrl Pts',(-70.5362648569072,1.01349288918539,
12.));
#145378=CARTESIAN_POINT('Ctrl Pts',(-70.5163397782698,1.00731061960967,
0.));
#145379=CARTESIAN_POINT('Ctrl Pts',(-70.5163397782698,1.00731061960967,
12.));
#145380=CARTESIAN_POINT('Ctrl Pts',(-70.4964564717917,1.00116412831437,
0.));
#145381=CARTESIAN_POINT('Ctrl Pts',(-70.4964564717917,1.00116412831437,
12.));
#145382=CARTESIAN_POINT('Ctrl Pts',(-70.4766151245169,0.995053387379677,
0.));
#145383=CARTESIAN_POINT('Ctrl Pts',(-70.4766151245169,0.995053387379677,
12.));
#145384=CARTESIAN_POINT('Ctrl Pts',(-70.4568159243131,0.988978368643586,
0.));
#145385=CARTESIAN_POINT('Ctrl Pts',(-70.4568159243131,0.988978368643586,
12.));
#145386=CARTESIAN_POINT('Ctrl Pts',(-70.4370590590839,0.982939043792156,
0.));
#145387=CARTESIAN_POINT('Ctrl Pts',(-70.4370590590839,0.982939043792156,
12.));
#145388=CARTESIAN_POINT('Ctrl Pts',(-70.41734471596,0.976935384450124,0.));
#145389=CARTESIAN_POINT('Ctrl Pts',(-70.41734471596,0.976935384450124,12.));
#145390=CARTESIAN_POINT('Ctrl Pts',(-70.3976730803664,0.970967362281299,
0.));
#145391=CARTESIAN_POINT('Ctrl Pts',(-70.3976730803664,0.970967362281299,
12.));
#145392=CARTESIAN_POINT('Ctrl Pts',(-70.3780443378003,0.965034948786555,
0.));
#145393=CARTESIAN_POINT('Ctrl Pts',(-70.3780443378003,0.965034948786555,
12.));
#145394=CARTESIAN_POINT('Ctrl Pts',(-70.3584586759561,0.959138115058882,
0.));
#145395=CARTESIAN_POINT('Ctrl Pts',(-70.3584586759561,0.959138115058882,
12.));
#145396=CARTESIAN_POINT('Ctrl Pts',(-70.338916286457,0.953276831581228,
0.));
#145397=CARTESIAN_POINT('Ctrl Pts',(-70.338916286457,0.953276831581228,
12.));
#145398=CARTESIAN_POINT('Ctrl Pts',(-70.3194173673635,0.94745106792956,
0.));
#145399=CARTESIAN_POINT('Ctrl Pts',(-70.3194173673635,0.94745106792956,
12.));
#145400=CARTESIAN_POINT('Ctrl Pts',(-70.2999621233938,0.941660792742949,
0.));
#145401=CARTESIAN_POINT('Ctrl Pts',(-70.2999621233938,0.941660792742949,
12.));
#145402=CARTESIAN_POINT('Ctrl Pts',(-70.2805507606832,0.935905974336487,
0.));
#145403=CARTESIAN_POINT('Ctrl Pts',(-70.2805507606832,0.935905974336487,
12.));
#145404=CARTESIAN_POINT('Ctrl Pts',(-70.2611834821711,0.930186581235571,
0.));
#145405=CARTESIAN_POINT('Ctrl Pts',(-70.2611834821711,0.930186581235571,
12.));
#145406=CARTESIAN_POINT('Ctrl Pts',(-70.241860483586,0.924502582639448,
0.));
#145407=CARTESIAN_POINT('Ctrl Pts',(-70.241860483586,0.924502582639448,
12.));
#145408=CARTESIAN_POINT('Ctrl Pts',(-70.2225819470306,0.91885394915704,
0.));
#145409=CARTESIAN_POINT('Ctrl Pts',(-70.2225819470306,0.91885394915704,
12.));
#145410=CARTESIAN_POINT('Ctrl Pts',(-70.2033480471749,0.913240652090834,
0.));
#145411=CARTESIAN_POINT('Ctrl Pts',(-70.2033480471749,0.913240652090834,
12.));
#145412=CARTESIAN_POINT('Ctrl Pts',(-70.184158963563,0.907662662015646,
0.));
#145413=CARTESIAN_POINT('Ctrl Pts',(-70.184158963563,0.907662662015646,
12.));
#145414=CARTESIAN_POINT('Ctrl Pts',(-70.1650148905109,0.902119947629768,
0.));
#145415=CARTESIAN_POINT('Ctrl Pts',(-70.1650148905109,0.902119947629768,
12.));
#145416=CARTESIAN_POINT('Ctrl Pts',(-70.1459160490366,0.89661247437208,
0.));
#145417=CARTESIAN_POINT('Ctrl Pts',(-70.1459160490366,0.89661247437208,
12.));
#145418=CARTESIAN_POINT('Ctrl Pts',(-70.1268626950031,0.89114020346472,
0.));
#145419=CARTESIAN_POINT('Ctrl Pts',(-70.1268626950031,0.89114020346472,
12.));
#145420=CARTESIAN_POINT('Ctrl Pts',(-70.1078550938801,0.885703094803082,
0.));
#145421=CARTESIAN_POINT('Ctrl Pts',(-70.1078550938801,0.885703094803082,
12.));
#145422=CARTESIAN_POINT('Ctrl Pts',(-70.0888934967772,0.880301109661035,
0.));
#145423=CARTESIAN_POINT('Ctrl Pts',(-70.0888934967772,0.880301109661035,
12.));
#145424=CARTESIAN_POINT('Ctrl Pts',(-70.0699781184013,0.874934213255568,
0.));
#145425=CARTESIAN_POINT('Ctrl Pts',(-70.0699781184013,0.874934213255568,
12.));
#145426=CARTESIAN_POINT('Ctrl Pts',(-70.0511091083285,0.869602377870135,
0.));
#145427=CARTESIAN_POINT('Ctrl Pts',(-70.0511091083285,0.869602377870135,
12.));
#145428=CARTESIAN_POINT('Ctrl Pts',(-70.0322865493339,0.864305583660085,
0.));
#145429=CARTESIAN_POINT('Ctrl Pts',(-70.0322865493339,0.864305583660085,
12.));
#145430=CARTESIAN_POINT('Ctrl Pts',(-70.0172656934192,0.860096170667396,
0.));
#145431=CARTESIAN_POINT('Ctrl Pts',(-70.0172656934192,0.860096170667396,
12.));
#145432=CARTESIAN_POINT('Ctrl Pts',(-70.0060209754332,0.856954870258366,
0.));
#145433=CARTESIAN_POINT('Ctrl Pts',(-70.0060209754332,0.856954870258366,
12.));
#145434=CARTESIAN_POINT('Ctrl Pts',(-69.9985337959499,0.854867673848289,
0.));
#145435=CARTESIAN_POINT('Ctrl Pts',(-69.9985337959499,0.854867673848289,
12.));
#145436=CARTESIAN_POINT('Ctrl Pts',(-69.9947925310006,0.853825826608988,
0.));
#145437=CARTESIAN_POINT('Ctrl Pts',(-69.9947925310006,0.853825826608988,
12.));
#145438=CARTESIAN_POINT('',(-69.9947925310006,0.853825826608988,12.));
#145439=CARTESIAN_POINT('Ctrl Pts',(-69.9947925310006,0.853825826608988,
12.));
#145440=CARTESIAN_POINT('Ctrl Pts',(-69.9985337959499,0.854867673848289,
12.));
#145441=CARTESIAN_POINT('Ctrl Pts',(-70.0060209754332,0.856954870258366,
12.));
#145442=CARTESIAN_POINT('Ctrl Pts',(-70.0172656934192,0.860096170667396,
12.));
#145443=CARTESIAN_POINT('Ctrl Pts',(-70.0322865493339,0.864305583660085,
12.));
#145444=CARTESIAN_POINT('Ctrl Pts',(-70.0511091083285,0.869602377870135,
12.));
#145445=CARTESIAN_POINT('Ctrl Pts',(-70.0699781184013,0.874934213255568,
12.));
#145446=CARTESIAN_POINT('Ctrl Pts',(-70.0888934967772,0.880301109661035,
12.));
#145447=CARTESIAN_POINT('Ctrl Pts',(-70.1078550938801,0.885703094803082,
12.));
#145448=CARTESIAN_POINT('Ctrl Pts',(-70.1268626950031,0.89114020346472,
12.));
#145449=CARTESIAN_POINT('Ctrl Pts',(-70.1459160490366,0.89661247437208,
12.));
#145450=CARTESIAN_POINT('Ctrl Pts',(-70.1650148905109,0.902119947629768,
12.));
#145451=CARTESIAN_POINT('Ctrl Pts',(-70.184158963563,0.907662662015646,
12.));
#145452=CARTESIAN_POINT('Ctrl Pts',(-70.2033480471749,0.913240652090834,
12.));
#145453=CARTESIAN_POINT('Ctrl Pts',(-70.2225819470306,0.91885394915704,
12.));
#145454=CARTESIAN_POINT('Ctrl Pts',(-70.241860483586,0.924502582639448,
12.));
#145455=CARTESIAN_POINT('Ctrl Pts',(-70.2611834821711,0.930186581235571,
12.));
#145456=CARTESIAN_POINT('Ctrl Pts',(-70.2805507606832,0.935905974336487,
12.));
#145457=CARTESIAN_POINT('Ctrl Pts',(-70.2999621233938,0.941660792742949,
12.));
#145458=CARTESIAN_POINT('Ctrl Pts',(-70.3194173673635,0.94745106792956,
12.));
#145459=CARTESIAN_POINT('Ctrl Pts',(-70.338916286457,0.953276831581228,
12.));
#145460=CARTESIAN_POINT('Ctrl Pts',(-70.3584586759561,0.959138115058882,
12.));
#145461=CARTESIAN_POINT('Ctrl Pts',(-70.3780443378003,0.965034948786555,
12.));
#145462=CARTESIAN_POINT('Ctrl Pts',(-70.3976730803664,0.970967362281299,
12.));
#145463=CARTESIAN_POINT('Ctrl Pts',(-70.41734471596,0.976935384450124,12.));
#145464=CARTESIAN_POINT('Ctrl Pts',(-70.4370590590839,0.982939043792156,
12.));
#145465=CARTESIAN_POINT('Ctrl Pts',(-70.4568159243131,0.988978368643586,
12.));
#145466=CARTESIAN_POINT('Ctrl Pts',(-70.4766151245169,0.995053387379677,
12.));
#145467=CARTESIAN_POINT('Ctrl Pts',(-70.4964564717917,1.00116412831437,
12.));
#145468=CARTESIAN_POINT('Ctrl Pts',(-70.5163397782698,1.00731061960967,
12.));
#145469=CARTESIAN_POINT('Ctrl Pts',(-70.5362648569072,1.01349288918539,
12.));
#145470=CARTESIAN_POINT('Ctrl Pts',(-70.5562315224219,1.01971096460599,
12.));
#145471=CARTESIAN_POINT('Ctrl Pts',(-70.5762395916412,1.02596487304049,
12.));
#145472=CARTESIAN_POINT('Ctrl Pts',(-70.5962888829958,1.03225464132872,
12.));
#145473=CARTESIAN_POINT('Ctrl Pts',(-70.6163792162079,1.03858029601905,
12.));
#145474=CARTESIAN_POINT('Ctrl Pts',(-70.6365104119238,1.04494186341155,
12.));
#145475=CARTESIAN_POINT('Ctrl Pts',(-70.6566822912965,1.05133936960068,
12.));
#145476=CARTESIAN_POINT('Ctrl Pts',(-70.6768946760063,1.05777284047727,
12.));
#145477=CARTESIAN_POINT('Ctrl Pts',(-70.6971473884443,1.0642423017128,12.));
#145478=CARTESIAN_POINT('Ctrl Pts',(-70.7174402518378,1.07074777874596,
12.));
#145479=CARTESIAN_POINT('Ctrl Pts',(-70.737773090397,1.07728929676412,12.));
#145480=CARTESIAN_POINT('Ctrl Pts',(-70.7581457294475,1.08386688068348,
12.));
#145481=CARTESIAN_POINT('Ctrl Pts',(-70.7785579953611,1.09048055516434,
12.));
#145482=CARTESIAN_POINT('Ctrl Pts',(-70.7990097154855,1.09713034462269,
12.));
#145483=CARTESIAN_POINT('Ctrl Pts',(-70.8195007180739,1.10381627323945,
12.));
#145484=CARTESIAN_POINT('Ctrl Pts',(-70.8400308322013,1.11053836496637,
12.));
#145485=CARTESIAN_POINT('Ctrl Pts',(-70.860599887712,1.1172966435299,12.));
#145486=CARTESIAN_POINT('Ctrl Pts',(-70.8812077152564,1.12409113243511,
12.));
#145487=CARTESIAN_POINT('Ctrl Pts',(-70.9018541463083,1.13092185496563,
12.));
#145488=CARTESIAN_POINT('Ctrl Pts',(-70.9225390131835,1.13778883418216,
12.));
#145489=CARTESIAN_POINT('Ctrl Pts',(-70.9432621490579,1.14469209291494,
12.));
#145490=CARTESIAN_POINT('Ctrl Pts',(-70.9640233879671,1.1516316537653,12.));
#145491=CARTESIAN_POINT('Ctrl Pts',(-70.9848225647876,1.15860753911489,
12.));
#145492=CARTESIAN_POINT('Ctrl Pts',(-71.0056595152204,1.16561977112882,
12.));
#145493=CARTESIAN_POINT('Ctrl Pts',(-71.0265340757697,1.17266837175775,
12.));
#145494=CARTESIAN_POINT('Ctrl Pts',(-71.0474460837157,1.17975336273499,
12.));
#145495=CARTESIAN_POINT('Ctrl Pts',(-71.0683953771147,1.18687476558126,
12.));
#145496=CARTESIAN_POINT('Ctrl Pts',(-71.089381794801,1.19403260160997,12.));
#145497=CARTESIAN_POINT('Ctrl Pts',(-71.1104051763839,1.20122689192836,
12.));
#145498=CARTESIAN_POINT('Ctrl Pts',(-71.1314653622442,1.20845765743654,
12.));
#145499=CARTESIAN_POINT('Ctrl Pts',(-71.1525621935266,1.21572491882273,
12.));
#145500=CARTESIAN_POINT('Ctrl Pts',(-71.1736955121361,1.22302869657028,
12.));
#145501=CARTESIAN_POINT('Ctrl Pts',(-71.1948651607319,1.23036901096246,
12.));
#145502=CARTESIAN_POINT('Ctrl Pts',(-71.2160709827189,1.23774588208427,
12.));
#145503=CARTESIAN_POINT('Ctrl Pts',(-71.2373128222359,1.24515932982107,
12.));
#145504=CARTESIAN_POINT('Ctrl Pts',(-71.2585905241422,1.2526093738556,12.));
#145505=CARTESIAN_POINT('Ctrl Pts',(-71.2799039340191,1.26009603367564,
12.));
#145506=CARTESIAN_POINT('Ctrl Pts',(-71.301252898167,1.26761932857723,12.));
#145507=CARTESIAN_POINT('Ctrl Pts',(-71.3226372635993,1.2751792776661,12.));
#145508=CARTESIAN_POINT('Ctrl Pts',(-71.344056878033,1.28277589985474,12.));
#145509=CARTESIAN_POINT('Ctrl Pts',(-71.3655115898801,1.2904092138606,12.));
#145510=CARTESIAN_POINT('Ctrl Pts',(-71.3870012482474,1.29807923821413,
12.));
#145511=CARTESIAN_POINT('Ctrl Pts',(-71.4085257029308,1.30578599126139,
12.));
#145512=CARTESIAN_POINT('Ctrl Pts',(-71.4300848044095,1.31352949116538,
12.));
#145513=CARTESIAN_POINT('Ctrl Pts',(-71.4516784038346,1.32130975590231,
12.));
#145514=CARTESIAN_POINT('Ctrl Pts',(-71.4733063530227,1.32912680326131,
12.));
#145515=CARTESIAN_POINT('Ctrl Pts',(-71.4949685044559,1.33698065085227,
12.));
#145516=CARTESIAN_POINT('Ctrl Pts',(-71.5166647112766,1.34487131610785,
12.));
#145517=CARTESIAN_POINT('Ctrl Pts',(-71.538394827283,1.35279881628453,12.));
#145518=CARTESIAN_POINT('Ctrl Pts',(-71.5601587069175,1.36076316845806,
12.));
#145519=CARTESIAN_POINT('Ctrl Pts',(-71.5819562052613,1.36876438952448,
12.));
#145520=CARTESIAN_POINT('Ctrl Pts',(-71.6037871780347,1.37680249620763,
12.));
#145521=CARTESIAN_POINT('Ctrl Pts',(-71.6256514815918,1.38487750506076,
12.));
#145522=CARTESIAN_POINT('Ctrl Pts',(-71.6475489729149,1.39298943246731,
12.));
#145523=CARTESIAN_POINT('Ctrl Pts',(-71.6694795096034,1.40113829463599,
12.));
#145524=CARTESIAN_POINT('Ctrl Pts',(-71.6914429498702,1.40932410760274,
12.));
#145525=CARTESIAN_POINT('Ctrl Pts',(-71.7134391525417,1.41754688723791,
12.));
#145526=CARTESIAN_POINT('Ctrl Pts',(-71.7354679770537,1.42580664924774,
12.));
#145527=CARTESIAN_POINT('Ctrl Pts',(-71.7575292834456,1.43410340917489,
12.));
#145528=CARTESIAN_POINT('Ctrl Pts',(-71.7796229323496,1.44243718239304,
12.));
#145529=CARTESIAN_POINT('Ctrl Pts',(-71.8017487849865,1.45080798410957,
12.));
#145530=CARTESIAN_POINT('Ctrl Pts',(-71.8239067031664,1.45921582937229,
12.));
#145531=CARTESIAN_POINT('Ctrl Pts',(-71.8460965492836,1.46766073307089,
12.));
#145532=CARTESIAN_POINT('Ctrl Pts',(-71.8683181863123,1.4761427099373,12.));
#145533=CARTESIAN_POINT('Ctrl Pts',(-71.8905714777972,1.48466177454021,
12.));
#145534=CARTESIAN_POINT('Ctrl Pts',(-71.9128562878491,1.493217941288,12.));
#145535=CARTESIAN_POINT('Ctrl Pts',(-71.935172481145,1.50181122443535,12.));
#145536=CARTESIAN_POINT('Ctrl Pts',(-71.9575199229241,1.51044163808454,
12.));
#145537=CARTESIAN_POINT('Ctrl Pts',(-71.9798984789828,1.51910919618566,
12.));
#145538=CARTESIAN_POINT('Ctrl Pts',(-72.0023080156647,1.52781391253103,
12.));
#145539=CARTESIAN_POINT('Ctrl Pts',(-72.0247483998582,1.53655580075813,
12.));
#145540=CARTESIAN_POINT('Ctrl Pts',(-72.0472194989968,1.54533487435626,
12.));
#145541=CARTESIAN_POINT('Ctrl Pts',(-72.0697211810548,1.55415114666774,
12.));
#145542=CARTESIAN_POINT('Ctrl Pts',(-72.092253314543,1.56300463088811,12.));
#145543=CARTESIAN_POINT('Ctrl Pts',(-72.1148157684987,1.57189534006043,
12.));
#145544=CARTESIAN_POINT('Ctrl Pts',(-72.1374084124829,1.58082328707808,
12.));
#145545=CARTESIAN_POINT('Ctrl Pts',(-72.1600311165813,1.58978848469128,
12.));
#145546=CARTESIAN_POINT('Ctrl Pts',(-72.1826837514,1.59879094550849,12.));
#145547=CARTESIAN_POINT('Ctrl Pts',(-72.2053661880611,1.60783068199661,
12.));
#145548=CARTESIAN_POINT('Ctrl Pts',(-72.2280782981941,1.61690770647535,
12.));
#145549=CARTESIAN_POINT('Ctrl Pts',(-72.2508199539325,1.62602203111924,
12.));
#145550=CARTESIAN_POINT('Ctrl Pts',(-72.2735910279149,1.63517366796458,
12.));
#145551=CARTESIAN_POINT('Ctrl Pts',(-72.2963913932811,1.64436262891078,
12.));
#145552=CARTESIAN_POINT('Ctrl Pts',(-72.3192209236691,1.65358892572065,
12.));
#145553=CARTESIAN_POINT('Ctrl Pts',(-72.3420794932052,1.66285257001502,
12.));
#145554=CARTESIAN_POINT('Ctrl Pts',(-72.3649669765013,1.67215357327372,
12.));
#145555=CARTESIAN_POINT('Ctrl Pts',(-72.3878832486549,1.68149194684288,
12.));
#145556=CARTESIAN_POINT('Ctrl Pts',(-72.4108281852473,1.6908677019364,12.));
#145557=CARTESIAN_POINT('Ctrl Pts',(-72.4338016623388,1.70028084963646,
12.));
#145558=CARTESIAN_POINT('Ctrl Pts',(-72.4568035564618,1.70973140088837,
12.));
#145559=CARTESIAN_POINT('Ctrl Pts',(-72.4798337446162,1.71921936650032,
12.));
#145560=CARTESIAN_POINT('Ctrl Pts',(-72.5028921042704,1.72874475715098,
12.));
#145561=CARTESIAN_POINT('Ctrl Pts',(-72.5259785133586,1.73830758339123,
12.));
#145562=CARTESIAN_POINT('Ctrl Pts',(-72.5490928502773,1.74790785564476,
12.));
#145563=CARTESIAN_POINT('Ctrl Pts',(-72.5722349938789,1.75754558420349,
12.));
#145564=CARTESIAN_POINT('Ctrl Pts',(-72.5954048234655,1.76722077922579,
12.));
#145565=CARTESIAN_POINT('Ctrl Pts',(-72.618602218792,1.7769334507443,12.));
#145566=CARTESIAN_POINT('Ctrl Pts',(-72.6418270600623,1.78668360866813,
12.));
#145567=CARTESIAN_POINT('Ctrl Pts',(-72.6650792279271,1.79647126278359,
12.));
#145568=CARTESIAN_POINT('Ctrl Pts',(-72.6883586034768,1.80629642275051,
12.));
#145569=CARTESIAN_POINT('Ctrl Pts',(-72.7116650682347,1.81615909809871,
12.));
#145570=CARTESIAN_POINT('Ctrl Pts',(-72.73499850416,1.82605929823565,12.));
#145571=CARTESIAN_POINT('Ctrl Pts',(-72.7583587936454,1.83599703244926,
12.));
#145572=CARTESIAN_POINT('Ctrl Pts',(-72.7817458195155,1.84597230990858,
12.));
#145573=CARTESIAN_POINT('Ctrl Pts',(-72.8051594650214,1.85598513966115,
12.));
#145574=CARTESIAN_POINT('Ctrl Pts',(-72.8285996138346,1.86603553062776,
12.));
#145575=CARTESIAN_POINT('Ctrl Pts',(-72.8520661500465,1.87612349160952,
12.));
#145576=CARTESIAN_POINT('Ctrl Pts',(-72.8755589581674,1.88624903129195,
12.));
#145577=CARTESIAN_POINT('Ctrl Pts',(-72.8990779231226,1.89641215824584,
12.));
#145578=CARTESIAN_POINT('Ctrl Pts',(-72.9226229302483,1.90661288092582,
12.));
#145579=CARTESIAN_POINT('Ctrl Pts',(-72.9461938652816,1.91685120766427,
12.));
#145580=CARTESIAN_POINT('Ctrl Pts',(-72.9697906143638,1.92712714667648,
12.));
#145581=CARTESIAN_POINT('Ctrl Pts',(-72.9934130640414,1.93744070606557,
12.));
#145582=CARTESIAN_POINT('Ctrl Pts',(-73.0170611012659,1.947791893823,12.));
#145583=CARTESIAN_POINT('Ctrl Pts',(-73.0407346133912,1.95818071782773,
12.));
#145584=CARTESIAN_POINT('Ctrl Pts',(-73.0644334881679,1.96860718583944,
12.));
#145585=CARTESIAN_POINT('Ctrl Pts',(-73.0881576137414,1.97907130550172,
12.));
#145586=CARTESIAN_POINT('Ctrl Pts',(-73.1119068786482,1.9895730843493,12.));
#145587=CARTESIAN_POINT('Ctrl Pts',(-73.1356811718094,2.00011252980987,
12.));
#145588=CARTESIAN_POINT('Ctrl Pts',(-73.159480382525,2.01068964920464,12.));
#145589=CARTESIAN_POINT('Ctrl Pts',(-73.1833044004612,2.02130444974351,
12.));
#145590=CARTESIAN_POINT('Ctrl Pts',(-73.2071531156492,2.0319569385244,12.));
#145591=CARTESIAN_POINT('Ctrl Pts',(-73.2310264184965,2.04264712253915,
12.));
#145592=CARTESIAN_POINT('Ctrl Pts',(-73.2549241997946,2.05337500867395,
12.));
#145593=CARTESIAN_POINT('Ctrl Pts',(-73.2788463507248,2.06414060370837,
12.));
#145594=CARTESIAN_POINT('Ctrl Pts',(-73.3027927628636,2.07494391430953,
12.));
#145595=CARTESIAN_POINT('Ctrl Pts',(-73.3267633281822,2.08578494702761,
12.));
#145596=CARTESIAN_POINT('Ctrl Pts',(-73.3507579390254,2.09666370830733,
12.));
#145597=CARTESIAN_POINT('Ctrl Pts',(-73.3747764880903,2.107580204494,12.));
#145598=CARTESIAN_POINT('Ctrl Pts',(-73.3988188684022,2.11853444183763,
12.));
#145599=CARTESIAN_POINT('Ctrl Pts',(-73.4228849732914,2.1295264264936,12.));
#145600=CARTESIAN_POINT('Ctrl Pts',(-73.4469746963622,2.14055616452048,
12.));
#145601=CARTESIAN_POINT('Ctrl Pts',(-73.4710879315367,2.15162366187898,
12.));
#145602=CARTESIAN_POINT('Ctrl Pts',(-73.4952245731044,2.16272892442915,
12.));
#145603=CARTESIAN_POINT('Ctrl Pts',(-73.5193845157705,2.17387195792305,
12.));
#145604=CARTESIAN_POINT('Ctrl Pts',(-73.5435676546934,2.18505276799756,
12.));
#145605=CARTESIAN_POINT('Ctrl Pts',(-73.5677738855461,2.19627136015682,
12.));
#145606=CARTESIAN_POINT('Ctrl Pts',(-73.5920031044604,2.20752773978352,
12.));
#145607=CARTESIAN_POINT('Ctrl Pts',(-73.6162552079044,2.2188219121652,12.));
#145608=CARTESIAN_POINT('Ctrl Pts',(-73.6405300925714,2.23015388251288,
12.));
#145609=CARTESIAN_POINT('Ctrl Pts',(-73.6648276552766,2.24152365597698,
12.));
#145610=CARTESIAN_POINT('Ctrl Pts',(-73.6891477928124,2.25293123766424,
12.));
#145611=CARTESIAN_POINT('Ctrl Pts',(-73.7134904019378,2.26437663263663,
12.));
#145612=CARTESIAN_POINT('Ctrl Pts',(-73.7378553796792,2.27585984587192,
12.));
#145613=CARTESIAN_POINT('Ctrl Pts',(-73.7622426235648,2.28738088222858,
12.));
#145614=CARTESIAN_POINT('Ctrl Pts',(-73.7866520318849,2.29893974640434,
12.));
#145615=CARTESIAN_POINT('Ctrl Pts',(-73.8110835039341,2.31053644289425,
12.));
#145616=CARTESIAN_POINT('Ctrl Pts',(-73.8355369402733,2.32217097594215,
12.));
#145617=CARTESIAN_POINT('Ctrl Pts',(-73.8600122421502,2.3338433496398,12.));
#145618=CARTESIAN_POINT('Ctrl Pts',(-73.8845093109302,2.34555356802139,
12.));
#145619=CARTESIAN_POINT('Ctrl Pts',(-73.9090280474723,2.35730163516323,
12.));
#145620=CARTESIAN_POINT('Ctrl Pts',(-73.9335683516388,2.36908755525994,
12.));
#145621=CARTESIAN_POINT('Ctrl Pts',(-73.9581301214609,2.38091133274932,
12.));
#145622=CARTESIAN_POINT('Ctrl Pts',(-73.9827132538149,2.39277297220716,
12.));
#145623=CARTESIAN_POINT('Ctrl Pts',(-74.0073176459287,2.40467247811496,
12.));
#145624=CARTESIAN_POINT('Ctrl Pts',(-74.0319431966956,2.41660985465228,
12.));
#145625=CARTESIAN_POINT('Ctrl Pts',(-74.0565898079227,2.42858510549786,
12.));
#145626=CARTESIAN_POINT('Ctrl Pts',(-74.0812573859474,2.44059823356721,
12.));
#145627=CARTESIAN_POINT('Ctrl Pts',(-74.1059458420175,2.45264924094852,
12.));
#145628=CARTESIAN_POINT('Ctrl Pts',(-74.1271264545378,2.46301176097528,
12.));
#145629=CARTESIAN_POINT('Ctrl Pts',(-74.1433763941622,2.47097695565719,
12.));
#145630=CARTESIAN_POINT('Ctrl Pts',(-74.1546864735454,2.47652804725575,
12.));
#145631=CARTESIAN_POINT('Ctrl Pts',(-74.1610506466544,2.47965393946828,
12.));
#145632=CARTESIAN_POINT('Ctrl Pts',(-74.1624659714955,2.48034921844905,
12.));
#145633=CARTESIAN_POINT('',(-69.9947925310006,0.853825826608988,0.));
#145634=CARTESIAN_POINT('',(-69.9947925310006,0.853825826608988,0.));
#145635=CARTESIAN_POINT('Ctrl Pts',(-74.1624659714955,2.48034921844905,
0.));
#145636=CARTESIAN_POINT('Ctrl Pts',(-74.1610506466544,2.47965393946828,
0.));
#145637=CARTESIAN_POINT('Ctrl Pts',(-74.1546864735454,2.47652804725575,
0.));
#145638=CARTESIAN_POINT('Ctrl Pts',(-74.1433763941622,2.47097695565719,
0.));
#145639=CARTESIAN_POINT('Ctrl Pts',(-74.1271264545378,2.46301176097528,
0.));
#145640=CARTESIAN_POINT('Ctrl Pts',(-74.1059458420175,2.45264924094852,
0.));
#145641=CARTESIAN_POINT('Ctrl Pts',(-74.0812573859474,2.44059823356721,
0.));
#145642=CARTESIAN_POINT('Ctrl Pts',(-74.0565898079227,2.42858510549786,
0.));
#145643=CARTESIAN_POINT('Ctrl Pts',(-74.0319431966956,2.41660985465228,
0.));
#145644=CARTESIAN_POINT('Ctrl Pts',(-74.0073176459287,2.40467247811496,
0.));
#145645=CARTESIAN_POINT('Ctrl Pts',(-73.9827132538149,2.39277297220716,
0.));
#145646=CARTESIAN_POINT('Ctrl Pts',(-73.9581301214609,2.38091133274932,
0.));
#145647=CARTESIAN_POINT('Ctrl Pts',(-73.9335683516388,2.36908755525994,
0.));
#145648=CARTESIAN_POINT('Ctrl Pts',(-73.9090280474723,2.35730163516323,
0.));
#145649=CARTESIAN_POINT('Ctrl Pts',(-73.8845093109302,2.34555356802139,
0.));
#145650=CARTESIAN_POINT('Ctrl Pts',(-73.8600122421502,2.3338433496398,0.));
#145651=CARTESIAN_POINT('Ctrl Pts',(-73.8355369402733,2.32217097594215,
0.));
#145652=CARTESIAN_POINT('Ctrl Pts',(-73.8110835039341,2.31053644289425,
0.));
#145653=CARTESIAN_POINT('Ctrl Pts',(-73.7866520318849,2.29893974640434,
0.));
#145654=CARTESIAN_POINT('Ctrl Pts',(-73.7622426235648,2.28738088222858,
0.));
#145655=CARTESIAN_POINT('Ctrl Pts',(-73.7378553796792,2.27585984587192,
0.));
#145656=CARTESIAN_POINT('Ctrl Pts',(-73.7134904019378,2.26437663263663,
0.));
#145657=CARTESIAN_POINT('Ctrl Pts',(-73.6891477928124,2.25293123766424,
0.));
#145658=CARTESIAN_POINT('Ctrl Pts',(-73.6648276552766,2.24152365597698,
0.));
#145659=CARTESIAN_POINT('Ctrl Pts',(-73.6405300925714,2.23015388251288,
0.));
#145660=CARTESIAN_POINT('Ctrl Pts',(-73.6162552079044,2.2188219121652,0.));
#145661=CARTESIAN_POINT('Ctrl Pts',(-73.5920031044604,2.20752773978352,
0.));
#145662=CARTESIAN_POINT('Ctrl Pts',(-73.5677738855461,2.19627136015682,
0.));
#145663=CARTESIAN_POINT('Ctrl Pts',(-73.5435676546934,2.18505276799756,
0.));
#145664=CARTESIAN_POINT('Ctrl Pts',(-73.5193845157705,2.17387195792305,
0.));
#145665=CARTESIAN_POINT('Ctrl Pts',(-73.4952245731044,2.16272892442915,
0.));
#145666=CARTESIAN_POINT('Ctrl Pts',(-73.4710879315367,2.15162366187898,
0.));
#145667=CARTESIAN_POINT('Ctrl Pts',(-73.4469746963622,2.14055616452048,
0.));
#145668=CARTESIAN_POINT('Ctrl Pts',(-73.4228849732914,2.1295264264936,0.));
#145669=CARTESIAN_POINT('Ctrl Pts',(-73.3988188684022,2.11853444183763,
0.));
#145670=CARTESIAN_POINT('Ctrl Pts',(-73.3747764880903,2.107580204494,0.));
#145671=CARTESIAN_POINT('Ctrl Pts',(-73.3507579390254,2.09666370830733,
0.));
#145672=CARTESIAN_POINT('Ctrl Pts',(-73.3267633281822,2.08578494702761,
0.));
#145673=CARTESIAN_POINT('Ctrl Pts',(-73.3027927628636,2.07494391430953,
0.));
#145674=CARTESIAN_POINT('Ctrl Pts',(-73.2788463507248,2.06414060370837,
0.));
#145675=CARTESIAN_POINT('Ctrl Pts',(-73.2549241997946,2.05337500867395,
0.));
#145676=CARTESIAN_POINT('Ctrl Pts',(-73.2310264184965,2.04264712253915,
0.));
#145677=CARTESIAN_POINT('Ctrl Pts',(-73.2071531156492,2.0319569385244,0.));
#145678=CARTESIAN_POINT('Ctrl Pts',(-73.1833044004612,2.02130444974351,
0.));
#145679=CARTESIAN_POINT('Ctrl Pts',(-73.159480382525,2.01068964920464,0.));
#145680=CARTESIAN_POINT('Ctrl Pts',(-73.1356811718094,2.00011252980987,
0.));
#145681=CARTESIAN_POINT('Ctrl Pts',(-73.1119068786482,1.9895730843493,0.));
#145682=CARTESIAN_POINT('Ctrl Pts',(-73.0881576137414,1.97907130550172,
0.));
#145683=CARTESIAN_POINT('Ctrl Pts',(-73.0644334881679,1.96860718583944,
0.));
#145684=CARTESIAN_POINT('Ctrl Pts',(-73.0407346133912,1.95818071782773,
0.));
#145685=CARTESIAN_POINT('Ctrl Pts',(-73.0170611012659,1.947791893823,0.));
#145686=CARTESIAN_POINT('Ctrl Pts',(-72.9934130640414,1.93744070606557,
0.));
#145687=CARTESIAN_POINT('Ctrl Pts',(-72.9697906143638,1.92712714667648,
0.));
#145688=CARTESIAN_POINT('Ctrl Pts',(-72.9461938652816,1.91685120766427,
0.));
#145689=CARTESIAN_POINT('Ctrl Pts',(-72.9226229302483,1.90661288092582,
0.));
#145690=CARTESIAN_POINT('Ctrl Pts',(-72.8990779231226,1.89641215824584,
0.));
#145691=CARTESIAN_POINT('Ctrl Pts',(-72.8755589581674,1.88624903129195,
0.));
#145692=CARTESIAN_POINT('Ctrl Pts',(-72.8520661500465,1.87612349160952,
0.));
#145693=CARTESIAN_POINT('Ctrl Pts',(-72.8285996138346,1.86603553062776,
0.));
#145694=CARTESIAN_POINT('Ctrl Pts',(-72.8051594650214,1.85598513966115,
0.));
#145695=CARTESIAN_POINT('Ctrl Pts',(-72.7817458195155,1.84597230990858,
0.));
#145696=CARTESIAN_POINT('Ctrl Pts',(-72.7583587936454,1.83599703244926,
0.));
#145697=CARTESIAN_POINT('Ctrl Pts',(-72.73499850416,1.82605929823565,0.));
#145698=CARTESIAN_POINT('Ctrl Pts',(-72.7116650682347,1.81615909809871,
0.));
#145699=CARTESIAN_POINT('Ctrl Pts',(-72.6883586034768,1.80629642275051,
0.));
#145700=CARTESIAN_POINT('Ctrl Pts',(-72.6650792279271,1.79647126278359,
0.));
#145701=CARTESIAN_POINT('Ctrl Pts',(-72.6418270600623,1.78668360866813,
0.));
#145702=CARTESIAN_POINT('Ctrl Pts',(-72.618602218792,1.7769334507443,0.));
#145703=CARTESIAN_POINT('Ctrl Pts',(-72.5954048234655,1.76722077922579,
0.));
#145704=CARTESIAN_POINT('Ctrl Pts',(-72.5722349938789,1.75754558420349,
0.));
#145705=CARTESIAN_POINT('Ctrl Pts',(-72.5490928502773,1.74790785564476,
0.));
#145706=CARTESIAN_POINT('Ctrl Pts',(-72.5259785133586,1.73830758339123,
0.));
#145707=CARTESIAN_POINT('Ctrl Pts',(-72.5028921042704,1.72874475715098,
0.));
#145708=CARTESIAN_POINT('Ctrl Pts',(-72.4798337446162,1.71921936650032,
0.));
#145709=CARTESIAN_POINT('Ctrl Pts',(-72.4568035564618,1.70973140088837,
0.));
#145710=CARTESIAN_POINT('Ctrl Pts',(-72.4338016623388,1.70028084963646,
0.));
#145711=CARTESIAN_POINT('Ctrl Pts',(-72.4108281852473,1.6908677019364,0.));
#145712=CARTESIAN_POINT('Ctrl Pts',(-72.3878832486549,1.68149194684288,
0.));
#145713=CARTESIAN_POINT('Ctrl Pts',(-72.3649669765013,1.67215357327372,
0.));
#145714=CARTESIAN_POINT('Ctrl Pts',(-72.3420794932052,1.66285257001502,
0.));
#145715=CARTESIAN_POINT('Ctrl Pts',(-72.3192209236691,1.65358892572065,
0.));
#145716=CARTESIAN_POINT('Ctrl Pts',(-72.2963913932811,1.64436262891078,
0.));
#145717=CARTESIAN_POINT('Ctrl Pts',(-72.2735910279149,1.63517366796458,
0.));
#145718=CARTESIAN_POINT('Ctrl Pts',(-72.2508199539325,1.62602203111924,
0.));
#145719=CARTESIAN_POINT('Ctrl Pts',(-72.2280782981941,1.61690770647535,
0.));
#145720=CARTESIAN_POINT('Ctrl Pts',(-72.2053661880611,1.60783068199661,
0.));
#145721=CARTESIAN_POINT('Ctrl Pts',(-72.1826837514,1.59879094550849,0.));
#145722=CARTESIAN_POINT('Ctrl Pts',(-72.1600311165813,1.58978848469128,
0.));
#145723=CARTESIAN_POINT('Ctrl Pts',(-72.1374084124829,1.58082328707808,
0.));
#145724=CARTESIAN_POINT('Ctrl Pts',(-72.1148157684987,1.57189534006043,
0.));
#145725=CARTESIAN_POINT('Ctrl Pts',(-72.092253314543,1.56300463088811,0.));
#145726=CARTESIAN_POINT('Ctrl Pts',(-72.0697211810548,1.55415114666774,
0.));
#145727=CARTESIAN_POINT('Ctrl Pts',(-72.0472194989968,1.54533487435626,
0.));
#145728=CARTESIAN_POINT('Ctrl Pts',(-72.0247483998582,1.53655580075813,
0.));
#145729=CARTESIAN_POINT('Ctrl Pts',(-72.0023080156647,1.52781391253103,
0.));
#145730=CARTESIAN_POINT('Ctrl Pts',(-71.9798984789828,1.51910919618566,
0.));
#145731=CARTESIAN_POINT('Ctrl Pts',(-71.9575199229241,1.51044163808454,
0.));
#145732=CARTESIAN_POINT('Ctrl Pts',(-71.935172481145,1.50181122443535,0.));
#145733=CARTESIAN_POINT('Ctrl Pts',(-71.9128562878491,1.493217941288,0.));
#145734=CARTESIAN_POINT('Ctrl Pts',(-71.8905714777972,1.48466177454021,
0.));
#145735=CARTESIAN_POINT('Ctrl Pts',(-71.8683181863123,1.4761427099373,0.));
#145736=CARTESIAN_POINT('Ctrl Pts',(-71.8460965492836,1.46766073307089,
0.));
#145737=CARTESIAN_POINT('Ctrl Pts',(-71.8239067031664,1.45921582937229,
0.));
#145738=CARTESIAN_POINT('Ctrl Pts',(-71.8017487849865,1.45080798410957,
0.));
#145739=CARTESIAN_POINT('Ctrl Pts',(-71.7796229323496,1.44243718239304,
0.));
#145740=CARTESIAN_POINT('Ctrl Pts',(-71.7575292834456,1.43410340917489,
0.));
#145741=CARTESIAN_POINT('Ctrl Pts',(-71.7354679770537,1.42580664924774,
0.));
#145742=CARTESIAN_POINT('Ctrl Pts',(-71.7134391525417,1.41754688723791,
0.));
#145743=CARTESIAN_POINT('Ctrl Pts',(-71.6914429498702,1.40932410760274,
0.));
#145744=CARTESIAN_POINT('Ctrl Pts',(-71.6694795096034,1.40113829463599,
0.));
#145745=CARTESIAN_POINT('Ctrl Pts',(-71.6475489729149,1.39298943246731,
0.));
#145746=CARTESIAN_POINT('Ctrl Pts',(-71.6256514815918,1.38487750506076,
0.));
#145747=CARTESIAN_POINT('Ctrl Pts',(-71.6037871780347,1.37680249620763,
0.));
#145748=CARTESIAN_POINT('Ctrl Pts',(-71.5819562052613,1.36876438952448,
0.));
#145749=CARTESIAN_POINT('Ctrl Pts',(-71.5601587069175,1.36076316845806,
0.));
#145750=CARTESIAN_POINT('Ctrl Pts',(-71.538394827283,1.35279881628453,0.));
#145751=CARTESIAN_POINT('Ctrl Pts',(-71.5166647112766,1.34487131610785,
0.));
#145752=CARTESIAN_POINT('Ctrl Pts',(-71.4949685044559,1.33698065085227,
0.));
#145753=CARTESIAN_POINT('Ctrl Pts',(-71.4733063530227,1.32912680326131,
0.));
#145754=CARTESIAN_POINT('Ctrl Pts',(-71.4516784038346,1.32130975590231,
0.));
#145755=CARTESIAN_POINT('Ctrl Pts',(-71.4300848044095,1.31352949116538,
0.));
#145756=CARTESIAN_POINT('Ctrl Pts',(-71.4085257029308,1.30578599126139,
0.));
#145757=CARTESIAN_POINT('Ctrl Pts',(-71.3870012482474,1.29807923821413,
0.));
#145758=CARTESIAN_POINT('Ctrl Pts',(-71.3655115898801,1.2904092138606,0.));
#145759=CARTESIAN_POINT('Ctrl Pts',(-71.344056878033,1.28277589985474,0.));
#145760=CARTESIAN_POINT('Ctrl Pts',(-71.3226372635993,1.2751792776661,0.));
#145761=CARTESIAN_POINT('Ctrl Pts',(-71.301252898167,1.26761932857723,0.));
#145762=CARTESIAN_POINT('Ctrl Pts',(-71.2799039340191,1.26009603367564,
0.));
#145763=CARTESIAN_POINT('Ctrl Pts',(-71.2585905241422,1.2526093738556,0.));
#145764=CARTESIAN_POINT('Ctrl Pts',(-71.2373128222359,1.24515932982107,
0.));
#145765=CARTESIAN_POINT('Ctrl Pts',(-71.2160709827189,1.23774588208427,
0.));
#145766=CARTESIAN_POINT('Ctrl Pts',(-71.1948651607319,1.23036901096246,
0.));
#145767=CARTESIAN_POINT('Ctrl Pts',(-71.1736955121361,1.22302869657028,
0.));
#145768=CARTESIAN_POINT('Ctrl Pts',(-71.1525621935266,1.21572491882273,
0.));
#145769=CARTESIAN_POINT('Ctrl Pts',(-71.1314653622442,1.20845765743654,
0.));
#145770=CARTESIAN_POINT('Ctrl Pts',(-71.1104051763839,1.20122689192836,
0.));
#145771=CARTESIAN_POINT('Ctrl Pts',(-71.089381794801,1.19403260160997,0.));
#145772=CARTESIAN_POINT('Ctrl Pts',(-71.0683953771147,1.18687476558126,
0.));
#145773=CARTESIAN_POINT('Ctrl Pts',(-71.0474460837157,1.17975336273499,
0.));
#145774=CARTESIAN_POINT('Ctrl Pts',(-71.0265340757697,1.17266837175775,
0.));
#145775=CARTESIAN_POINT('Ctrl Pts',(-71.0056595152204,1.16561977112882,
0.));
#145776=CARTESIAN_POINT('Ctrl Pts',(-70.9848225647876,1.15860753911489,
0.));
#145777=CARTESIAN_POINT('Ctrl Pts',(-70.9640233879671,1.1516316537653,0.));
#145778=CARTESIAN_POINT('Ctrl Pts',(-70.9432621490579,1.14469209291494,
0.));
#145779=CARTESIAN_POINT('Ctrl Pts',(-70.9225390131835,1.13778883418216,
0.));
#145780=CARTESIAN_POINT('Ctrl Pts',(-70.9018541463083,1.13092185496563,
0.));
#145781=CARTESIAN_POINT('Ctrl Pts',(-70.8812077152564,1.12409113243511,
0.));
#145782=CARTESIAN_POINT('Ctrl Pts',(-70.860599887712,1.1172966435299,0.));
#145783=CARTESIAN_POINT('Ctrl Pts',(-70.8400308322013,1.11053836496637,
0.));
#145784=CARTESIAN_POINT('Ctrl Pts',(-70.8195007180739,1.10381627323945,
0.));
#145785=CARTESIAN_POINT('Ctrl Pts',(-70.7990097154855,1.09713034462269,
0.));
#145786=CARTESIAN_POINT('Ctrl Pts',(-70.7785579953611,1.09048055516434,
0.));
#145787=CARTESIAN_POINT('Ctrl Pts',(-70.7581457294475,1.08386688068348,
0.));
#145788=CARTESIAN_POINT('Ctrl Pts',(-70.737773090397,1.07728929676412,0.));
#145789=CARTESIAN_POINT('Ctrl Pts',(-70.7174402518378,1.07074777874596,
0.));
#145790=CARTESIAN_POINT('Ctrl Pts',(-70.6971473884443,1.0642423017128,0.));
#145791=CARTESIAN_POINT('Ctrl Pts',(-70.6768946760063,1.05777284047727,
0.));
#145792=CARTESIAN_POINT('Ctrl Pts',(-70.6566822912965,1.05133936960068,
0.));
#145793=CARTESIAN_POINT('Ctrl Pts',(-70.6365104119238,1.04494186341155,
0.));
#145794=CARTESIAN_POINT('Ctrl Pts',(-70.6163792162079,1.03858029601905,
0.));
#145795=CARTESIAN_POINT('Ctrl Pts',(-70.5962888829958,1.03225464132872,
0.));
#145796=CARTESIAN_POINT('Ctrl Pts',(-70.5762395916412,1.02596487304049,
0.));
#145797=CARTESIAN_POINT('Ctrl Pts',(-70.5562315224219,1.01971096460599,
0.));
#145798=CARTESIAN_POINT('Ctrl Pts',(-70.5362648569072,1.01349288918539,
0.));
#145799=CARTESIAN_POINT('Ctrl Pts',(-70.5163397782698,1.00731061960967,
0.));
#145800=CARTESIAN_POINT('Ctrl Pts',(-70.4964564717917,1.00116412831437,
0.));
#145801=CARTESIAN_POINT('Ctrl Pts',(-70.4766151245169,0.995053387379677,
0.));
#145802=CARTESIAN_POINT('Ctrl Pts',(-70.4568159243131,0.988978368643586,
0.));
#145803=CARTESIAN_POINT('Ctrl Pts',(-70.4370590590839,0.982939043792156,
0.));
#145804=CARTESIAN_POINT('Ctrl Pts',(-70.41734471596,0.976935384450124,0.));
#145805=CARTESIAN_POINT('Ctrl Pts',(-70.3976730803664,0.970967362281299,
0.));
#145806=CARTESIAN_POINT('Ctrl Pts',(-70.3780443378003,0.965034948786555,
0.));
#145807=CARTESIAN_POINT('Ctrl Pts',(-70.3584586759561,0.959138115058882,
0.));
#145808=CARTESIAN_POINT('Ctrl Pts',(-70.338916286457,0.953276831581228,
0.));
#145809=CARTESIAN_POINT('Ctrl Pts',(-70.3194173673635,0.94745106792956,
0.));
#145810=CARTESIAN_POINT('Ctrl Pts',(-70.2999621233938,0.941660792742949,
0.));
#145811=CARTESIAN_POINT('Ctrl Pts',(-70.2805507606832,0.935905974336487,
0.));
#145812=CARTESIAN_POINT('Ctrl Pts',(-70.2611834821711,0.930186581235571,
0.));
#145813=CARTESIAN_POINT('Ctrl Pts',(-70.241860483586,0.924502582639448,
0.));
#145814=CARTESIAN_POINT('Ctrl Pts',(-70.2225819470306,0.91885394915704,
0.));
#145815=CARTESIAN_POINT('Ctrl Pts',(-70.2033480471749,0.913240652090834,
0.));
#145816=CARTESIAN_POINT('Ctrl Pts',(-70.184158963563,0.907662662015646,
0.));
#145817=CARTESIAN_POINT('Ctrl Pts',(-70.1650148905109,0.902119947629768,
0.));
#145818=CARTESIAN_POINT('Ctrl Pts',(-70.1459160490366,0.89661247437208,
0.));
#145819=CARTESIAN_POINT('Ctrl Pts',(-70.1268626950031,0.89114020346472,
0.));
#145820=CARTESIAN_POINT('Ctrl Pts',(-70.1078550938801,0.885703094803082,
0.));
#145821=CARTESIAN_POINT('Ctrl Pts',(-70.0888934967772,0.880301109661035,
0.));
#145822=CARTESIAN_POINT('Ctrl Pts',(-70.0699781184013,0.874934213255568,
0.));
#145823=CARTESIAN_POINT('Ctrl Pts',(-70.0511091083285,0.869602377870135,
0.));
#145824=CARTESIAN_POINT('Ctrl Pts',(-70.0322865493339,0.864305583660085,
0.));
#145825=CARTESIAN_POINT('Ctrl Pts',(-70.0172656934192,0.860096170667396,
0.));
#145826=CARTESIAN_POINT('Ctrl Pts',(-70.0060209754332,0.856954870258366,
0.));
#145827=CARTESIAN_POINT('Ctrl Pts',(-69.9985337959499,0.854867673848289,
0.));
#145828=CARTESIAN_POINT('Ctrl Pts',(-69.9947925310006,0.853825826608988,
0.));
#145829=CARTESIAN_POINT('Ctrl Pts',(-73.9415940197274,9.10443154852691,
0.));
#145830=CARTESIAN_POINT('Ctrl Pts',(-73.9415940197274,9.10443154852691,
12.));
#145831=CARTESIAN_POINT('Ctrl Pts',(-73.9368365074299,9.1014855851654,0.));
#145832=CARTESIAN_POINT('Ctrl Pts',(-73.9368365074299,9.1014855851654,12.));
#145833=CARTESIAN_POINT('Ctrl Pts',(-73.9273231219835,9.09559760529044,
0.));
#145834=CARTESIAN_POINT('Ctrl Pts',(-73.9273231219835,9.09559760529044,
12.));
#145835=CARTESIAN_POINT('Ctrl Pts',(-73.9130579612604,9.08677747602208,
0.));
#145836=CARTESIAN_POINT('Ctrl Pts',(-73.9130579612604,9.08677747602208,
12.));
#145837=CARTESIAN_POINT('Ctrl Pts',(-73.8940475822492,9.0750409857171,0.));
#145838=CARTESIAN_POINT('Ctrl Pts',(-73.8940475822492,9.0750409857171,12.));
#145839=CARTESIAN_POINT('Ctrl Pts',(-73.8703010078091,9.06040984890249,
0.));
#145840=CARTESIAN_POINT('Ctrl Pts',(-73.8703010078091,9.06040984890249,
12.));
#145841=CARTESIAN_POINT('Ctrl Pts',(-73.8465708501057,9.04581819646987,
0.));
#145842=CARTESIAN_POINT('Ctrl Pts',(-73.8465708501057,9.04581819646987,
12.));
#145843=CARTESIAN_POINT('Ctrl Pts',(-73.8228571411697,9.03126603778128,
0.));
#145844=CARTESIAN_POINT('Ctrl Pts',(-73.8228571411697,9.03126603778128,
12.));
#145845=CARTESIAN_POINT('Ctrl Pts',(-73.7991599312592,9.01675338208007,
0.));
#145846=CARTESIAN_POINT('Ctrl Pts',(-73.7991599312592,9.01675338208007,
12.));
#145847=CARTESIAN_POINT('Ctrl Pts',(-73.7754792943665,9.00228023701058,
0.));
#145848=CARTESIAN_POINT('Ctrl Pts',(-73.7754792943665,9.00228023701058,
12.));
#145849=CARTESIAN_POINT('Ctrl Pts',(-73.7518153261981,8.987846608374,0.));
#145850=CARTESIAN_POINT('Ctrl Pts',(-73.7518153261981,8.987846608374,12.));
#145851=CARTESIAN_POINT('Ctrl Pts',(-73.728168136383,8.97345250083603,0.));
#145852=CARTESIAN_POINT('Ctrl Pts',(-73.728168136383,8.97345250083603,12.));
#145853=CARTESIAN_POINT('Ctrl Pts',(-73.7045378422686,8.95909791836155,
0.));
#145854=CARTESIAN_POINT('Ctrl Pts',(-73.7045378422686,8.95909791836155,
12.));
#145855=CARTESIAN_POINT('Ctrl Pts',(-73.6809245622383,8.94478286474422,
0.));
#145856=CARTESIAN_POINT('Ctrl Pts',(-73.6809245622383,8.94478286474422,
12.));
#145857=CARTESIAN_POINT('Ctrl Pts',(-73.6573284088184,8.93050734412127,
0.));
#145858=CARTESIAN_POINT('Ctrl Pts',(-73.6573284088184,8.93050734412127,
12.));
#145859=CARTESIAN_POINT('Ctrl Pts',(-73.633749483097,8.91627136140087,0.));
#145860=CARTESIAN_POINT('Ctrl Pts',(-73.633749483097,8.91627136140087,12.));
#145861=CARTESIAN_POINT('Ctrl Pts',(-73.6101878785976,8.90207492199045,
0.));
#145862=CARTESIAN_POINT('Ctrl Pts',(-73.6101878785976,8.90207492199045,
12.));
#145863=CARTESIAN_POINT('Ctrl Pts',(-73.5866436840556,8.88791803160445,
0.));
#145864=CARTESIAN_POINT('Ctrl Pts',(-73.5866436840556,8.88791803160445,
12.));
#145865=CARTESIAN_POINT('Ctrl Pts',(-73.5631169867122,8.87380069602973,
0.));
#145866=CARTESIAN_POINT('Ctrl Pts',(-73.5631169867122,8.87380069602973,
12.));
#145867=CARTESIAN_POINT('Ctrl Pts',(-73.5396078751639,8.85972292092133,
0.));
#145868=CARTESIAN_POINT('Ctrl Pts',(-73.5396078751639,8.85972292092133,
12.));
#145869=CARTESIAN_POINT('Ctrl Pts',(-73.5161164429709,8.84568471153808,
0.));
#145870=CARTESIAN_POINT('Ctrl Pts',(-73.5161164429709,8.84568471153808,
12.));
#145871=CARTESIAN_POINT('Ctrl Pts',(-73.492642788273,8.83168607277327,0.));
#145872=CARTESIAN_POINT('Ctrl Pts',(-73.492642788273,8.83168607277327,12.));
#145873=CARTESIAN_POINT('Ctrl Pts',(-73.4691870121567,8.81772700927533,
0.));
#145874=CARTESIAN_POINT('Ctrl Pts',(-73.4691870121567,8.81772700927533,
12.));
#145875=CARTESIAN_POINT('Ctrl Pts',(-73.4457492173933,8.80380752553694,
0.));
#145876=CARTESIAN_POINT('Ctrl Pts',(-73.4457492173933,8.80380752553694,
12.));
#145877=CARTESIAN_POINT('Ctrl Pts',(-73.422329507113,8.78992762598759,0.));
#145878=CARTESIAN_POINT('Ctrl Pts',(-73.422329507113,8.78992762598759,12.));
#145879=CARTESIAN_POINT('Ctrl Pts',(-73.3989279832835,8.7760873150935,0.));
#145880=CARTESIAN_POINT('Ctrl Pts',(-73.3989279832835,8.7760873150935,12.));
#145881=CARTESIAN_POINT('Ctrl Pts',(-73.3755447460268,8.7622865974036,0.));
#145882=CARTESIAN_POINT('Ctrl Pts',(-73.3755447460268,8.7622865974036,12.));
#145883=CARTESIAN_POINT('Ctrl Pts',(-73.3521798944622,8.74852547749781,
0.));
#145884=CARTESIAN_POINT('Ctrl Pts',(-73.3521798944622,8.74852547749781,
12.));
#145885=CARTESIAN_POINT('Ctrl Pts',(-73.3288335272002,8.73480395995383,
0.));
#145886=CARTESIAN_POINT('Ctrl Pts',(-73.3288335272002,8.73480395995383,
12.));
#145887=CARTESIAN_POINT('Ctrl Pts',(-73.3055057429742,8.72112204930234,
0.));
#145888=CARTESIAN_POINT('Ctrl Pts',(-73.3055057429742,8.72112204930234,
12.));
#145889=CARTESIAN_POINT('Ctrl Pts',(-73.2821966412148,8.70747974998232,
0.));
#145890=CARTESIAN_POINT('Ctrl Pts',(-73.2821966412148,8.70747974998232,
12.));
#145891=CARTESIAN_POINT('Ctrl Pts',(-73.2589063226358,8.69387706629287,
0.));
#145892=CARTESIAN_POINT('Ctrl Pts',(-73.2589063226358,8.69387706629287,
12.));
#145893=CARTESIAN_POINT('Ctrl Pts',(-73.2356348889693,8.68031400241874,
0.));
#145894=CARTESIAN_POINT('Ctrl Pts',(-73.2356348889693,8.68031400241874,
12.));
#145895=CARTESIAN_POINT('Ctrl Pts',(-73.2123824427208,8.66679056245095,
0.));
#145896=CARTESIAN_POINT('Ctrl Pts',(-73.2123824427208,8.66679056245095,
12.));
#145897=CARTESIAN_POINT('Ctrl Pts',(-73.1891490869056,8.65330675040539,
0.));
#145898=CARTESIAN_POINT('Ctrl Pts',(-73.1891490869056,8.65330675040539,
12.));
#145899=CARTESIAN_POINT('Ctrl Pts',(-73.1659349248132,8.63986257023741,
0.));
#145900=CARTESIAN_POINT('Ctrl Pts',(-73.1659349248132,8.63986257023741,
12.));
#145901=CARTESIAN_POINT('Ctrl Pts',(-73.1427400597037,8.62645802585486,
0.));
#145902=CARTESIAN_POINT('Ctrl Pts',(-73.1427400597037,8.62645802585486,
12.));
#145903=CARTESIAN_POINT('Ctrl Pts',(-73.1195645948178,8.61309312112004,
0.));
#145904=CARTESIAN_POINT('Ctrl Pts',(-73.1195645948178,8.61309312112004,
12.));
#145905=CARTESIAN_POINT('Ctrl Pts',(-73.0964086335235,8.59976785984554,
0.));
#145906=CARTESIAN_POINT('Ctrl Pts',(-73.0964086335235,8.59976785984554,
12.));
#145907=CARTESIAN_POINT('Ctrl Pts',(-73.0732722794195,8.58648224578734,
0.));
#145908=CARTESIAN_POINT('Ctrl Pts',(-73.0732722794195,8.58648224578734,
12.));
#145909=CARTESIAN_POINT('Ctrl Pts',(-73.0501556364479,8.57323628263595,
0.));
#145910=CARTESIAN_POINT('Ctrl Pts',(-73.0501556364479,8.57323628263595,
12.));
#145911=CARTESIAN_POINT('Ctrl Pts',(-73.0270588090183,8.56002997400086,
0.));
#145912=CARTESIAN_POINT('Ctrl Pts',(-73.0270588090183,8.56002997400086,
12.));
#145913=CARTESIAN_POINT('Ctrl Pts',(-73.0039819020648,8.5468633234042,0.));
#145914=CARTESIAN_POINT('Ctrl Pts',(-73.0039819020648,8.5468633234042,12.));
#145915=CARTESIAN_POINT('Ctrl Pts',(-72.9809250209828,8.53373633429283,
0.));
#145916=CARTESIAN_POINT('Ctrl Pts',(-72.9809250209828,8.53373633429283,
12.));
#145917=CARTESIAN_POINT('Ctrl Pts',(-72.9578882715912,8.5206490100423,0.));
#145918=CARTESIAN_POINT('Ctrl Pts',(-72.9578882715912,8.5206490100423,12.));
#145919=CARTESIAN_POINT('Ctrl Pts',(-72.9348717600838,8.50760135395986,
0.));
#145920=CARTESIAN_POINT('Ctrl Pts',(-72.9348717600838,8.50760135395986,
12.));
#145921=CARTESIAN_POINT('Ctrl Pts',(-72.9118755929795,8.49459336928298,
0.));
#145922=CARTESIAN_POINT('Ctrl Pts',(-72.9118755929795,8.49459336928298,
12.));
#145923=CARTESIAN_POINT('Ctrl Pts',(-72.8888998770785,8.4816250591766,0.));
#145924=CARTESIAN_POINT('Ctrl Pts',(-72.8888998770785,8.4816250591766,12.));
#145925=CARTESIAN_POINT('Ctrl Pts',(-72.8659447194933,8.46869642673797,
0.));
#145926=CARTESIAN_POINT('Ctrl Pts',(-72.8659447194933,8.46869642673797,
12.));
#145927=CARTESIAN_POINT('Ctrl Pts',(-72.8430102276713,8.45580747499796,
0.));
#145928=CARTESIAN_POINT('Ctrl Pts',(-72.8430102276713,8.45580747499796,
12.));
#145929=CARTESIAN_POINT('Ctrl Pts',(-72.8200965094199,8.44295820691914,
0.));
#145930=CARTESIAN_POINT('Ctrl Pts',(-72.8200965094199,8.44295820691914,
12.));
#145931=CARTESIAN_POINT('Ctrl Pts',(-72.7972036729276,8.4301486253916,0.));
#145932=CARTESIAN_POINT('Ctrl Pts',(-72.7972036729276,8.4301486253916,12.));
#145933=CARTESIAN_POINT('Ctrl Pts',(-72.7743318267865,8.41737873322332,
0.));
#145934=CARTESIAN_POINT('Ctrl Pts',(-72.7743318267865,8.41737873322332,
12.));
#145935=CARTESIAN_POINT('Ctrl Pts',(-72.751481079992,8.40464853314471,0.));
#145936=CARTESIAN_POINT('Ctrl Pts',(-72.751481079992,8.40464853314471,12.));
#145937=CARTESIAN_POINT('Ctrl Pts',(-72.7286515419372,8.39195802781393,
0.));
#145938=CARTESIAN_POINT('Ctrl Pts',(-72.7286515419372,8.39195802781393,
12.));
#145939=CARTESIAN_POINT('Ctrl Pts',(-72.705843322407,8.37930721981733,0.));
#145940=CARTESIAN_POINT('Ctrl Pts',(-72.705843322407,8.37930721981733,12.));
#145941=CARTESIAN_POINT('Ctrl Pts',(-72.6830565315703,8.36669611166845,
0.));
#145942=CARTESIAN_POINT('Ctrl Pts',(-72.6830565315703,8.36669611166845,
12.));
#145943=CARTESIAN_POINT('Ctrl Pts',(-72.6602912799696,8.35412470580104,
0.));
#145944=CARTESIAN_POINT('Ctrl Pts',(-72.6602912799696,8.35412470580104,
12.));
#145945=CARTESIAN_POINT('Ctrl Pts',(-72.6375476785215,8.34159300456989,
0.));
#145946=CARTESIAN_POINT('Ctrl Pts',(-72.6375476785215,8.34159300456989,
12.));
#145947=CARTESIAN_POINT('Ctrl Pts',(-72.6148258385296,8.32910101025673,
0.));
#145948=CARTESIAN_POINT('Ctrl Pts',(-72.6148258385296,8.32910101025673,
12.));
#145949=CARTESIAN_POINT('Ctrl Pts',(-72.5921258716901,8.31664872507019,
0.));
#145950=CARTESIAN_POINT('Ctrl Pts',(-72.5921258716901,8.31664872507019,
12.));
#145951=CARTESIAN_POINT('Ctrl Pts',(-72.5694478900981,8.30423615114455,
0.));
#145952=CARTESIAN_POINT('Ctrl Pts',(-72.5694478900981,8.30423615114455,
12.));
#145953=CARTESIAN_POINT('Ctrl Pts',(-72.5467920062521,8.29186329053282,
0.));
#145954=CARTESIAN_POINT('Ctrl Pts',(-72.5467920062521,8.29186329053282,
12.));
#145955=CARTESIAN_POINT('Ctrl Pts',(-72.5241583330562,8.27953014520378,
0.));
#145956=CARTESIAN_POINT('Ctrl Pts',(-72.5241583330562,8.27953014520378,
12.));
#145957=CARTESIAN_POINT('Ctrl Pts',(-72.5015469838254,8.26723671704922,
0.));
#145958=CARTESIAN_POINT('Ctrl Pts',(-72.5015469838254,8.26723671704922,
12.));
#145959=CARTESIAN_POINT('Ctrl Pts',(-72.4789580722875,8.25498300788496,
0.));
#145960=CARTESIAN_POINT('Ctrl Pts',(-72.4789580722875,8.25498300788496,
12.));
#145961=CARTESIAN_POINT('Ctrl Pts',(-72.4563917125842,8.24276901945042,
0.));
#145962=CARTESIAN_POINT('Ctrl Pts',(-72.4563917125842,8.24276901945042,
12.));
#145963=CARTESIAN_POINT('Ctrl Pts',(-72.4338480192694,8.23059475340359,
0.));
#145964=CARTESIAN_POINT('Ctrl Pts',(-72.4338480192694,8.23059475340359,
12.));
#145965=CARTESIAN_POINT('Ctrl Pts',(-72.4113271073079,8.21846021131563,
0.));
#145966=CARTESIAN_POINT('Ctrl Pts',(-72.4113271073079,8.21846021131563,
12.));
#145967=CARTESIAN_POINT('Ctrl Pts',(-72.3888290920832,8.20636539467778,
0.));
#145968=CARTESIAN_POINT('Ctrl Pts',(-72.3888290920832,8.20636539467778,
12.));
#145969=CARTESIAN_POINT('Ctrl Pts',(-72.3663540894026,8.19431030490317,
0.));
#145970=CARTESIAN_POINT('Ctrl Pts',(-72.3663540894026,8.19431030490317,
12.));
#145971=CARTESIAN_POINT('Ctrl Pts',(-72.3439022155007,8.18229494332626,
0.));
#145972=CARTESIAN_POINT('Ctrl Pts',(-72.3439022155007,8.18229494332626,
12.));
#145973=CARTESIAN_POINT('Ctrl Pts',(-72.3214735870409,8.17031931119893,
0.));
#145974=CARTESIAN_POINT('Ctrl Pts',(-72.3214735870409,8.17031931119893,
12.));
#145975=CARTESIAN_POINT('Ctrl Pts',(-72.2990683211162,8.15838340968338,
0.));
#145976=CARTESIAN_POINT('Ctrl Pts',(-72.2990683211162,8.15838340968338,
12.));
#145977=CARTESIAN_POINT('Ctrl Pts',(-72.2766865352555,8.146487239858,0.));
#145978=CARTESIAN_POINT('Ctrl Pts',(-72.2766865352555,8.146487239858,12.));
#145979=CARTESIAN_POINT('Ctrl Pts',(-72.2543283474278,8.13463080272031,
0.));
#145980=CARTESIAN_POINT('Ctrl Pts',(-72.2543283474278,8.13463080272031,
12.));
#145981=CARTESIAN_POINT('Ctrl Pts',(-72.2319938760449,8.12281409918663,
0.));
#145982=CARTESIAN_POINT('Ctrl Pts',(-72.2319938760449,8.12281409918663,
12.));
#145983=CARTESIAN_POINT('Ctrl Pts',(-72.209683239963,8.11103713008931,0.));
#145984=CARTESIAN_POINT('Ctrl Pts',(-72.209683239963,8.11103713008931,12.));
#145985=CARTESIAN_POINT('Ctrl Pts',(-72.1873965584813,8.09929989616892,
0.));
#145986=CARTESIAN_POINT('Ctrl Pts',(-72.1873965584813,8.09929989616892,
12.));
#145987=CARTESIAN_POINT('Ctrl Pts',(-72.1651339513477,8.08760239807839,
0.));
#145988=CARTESIAN_POINT('Ctrl Pts',(-72.1651339513477,8.08760239807839,
12.));
#145989=CARTESIAN_POINT('Ctrl Pts',(-72.1428955387663,8.07594463638721,
0.));
#145990=CARTESIAN_POINT('Ctrl Pts',(-72.1428955387663,8.07594463638721,
12.));
#145991=CARTESIAN_POINT('Ctrl Pts',(-72.1206814413988,8.06432661158098,
0.));
#145992=CARTESIAN_POINT('Ctrl Pts',(-72.1206814413988,8.06432661158098,
12.));
#145993=CARTESIAN_POINT('Ctrl Pts',(-72.0984917803693,8.05274832405951,
0.));
#145994=CARTESIAN_POINT('Ctrl Pts',(-72.0984917803693,8.05274832405951,
12.));
#145995=CARTESIAN_POINT('Ctrl Pts',(-72.0763266772615,8.04120977412874,
0.));
#145996=CARTESIAN_POINT('Ctrl Pts',(-72.0763266772615,8.04120977412874,
12.));
#145997=CARTESIAN_POINT('Ctrl Pts',(-72.0541862541243,8.0297109620031,0.));
#145998=CARTESIAN_POINT('Ctrl Pts',(-72.0541862541243,8.0297109620031,12.));
#145999=CARTESIAN_POINT('Ctrl Pts',(-72.032070633479,8.01825188781059,0.));
#146000=CARTESIAN_POINT('Ctrl Pts',(-72.032070633479,8.01825188781059,12.));
#146001=CARTESIAN_POINT('Ctrl Pts',(-72.0099799383213,8.0068325515925,0.));
#146002=CARTESIAN_POINT('Ctrl Pts',(-72.0099799383213,8.0068325515925,12.));
#146003=CARTESIAN_POINT('Ctrl Pts',(-71.9879142921254,7.99545295330193,
0.));
#146004=CARTESIAN_POINT('Ctrl Pts',(-71.9879142921254,7.99545295330193,
12.));
#146005=CARTESIAN_POINT('Ctrl Pts',(-71.965873818843,7.98411309279615,0.));
#146006=CARTESIAN_POINT('Ctrl Pts',(-71.965873818843,7.98411309279615,12.));
#146007=CARTESIAN_POINT('Ctrl Pts',(-71.943858642908,7.9728129698372,0.));
#146008=CARTESIAN_POINT('Ctrl Pts',(-71.943858642908,7.9728129698372,12.));
#146009=CARTESIAN_POINT('Ctrl Pts',(-71.9218688892431,7.96155258409766,
0.));
#146010=CARTESIAN_POINT('Ctrl Pts',(-71.9218688892431,7.96155258409766,
12.));
#146011=CARTESIAN_POINT('Ctrl Pts',(-71.8999046832643,7.95033193516053,
0.));
#146012=CARTESIAN_POINT('Ctrl Pts',(-71.8999046832643,7.95033193516053,
12.));
#146013=CARTESIAN_POINT('Ctrl Pts',(-71.8779661508832,7.93915102251797,
0.));
#146014=CARTESIAN_POINT('Ctrl Pts',(-71.8779661508832,7.93915102251797,
12.));
#146015=CARTESIAN_POINT('Ctrl Pts',(-71.8560534185071,7.92800984556398,
0.));
#146016=CARTESIAN_POINT('Ctrl Pts',(-71.8560534185071,7.92800984556398,
12.));
#146017=CARTESIAN_POINT('Ctrl Pts',(-71.8341666130426,7.91690840359369,
0.));
#146018=CARTESIAN_POINT('Ctrl Pts',(-71.8341666130426,7.91690840359369,
12.));
#146019=CARTESIAN_POINT('Ctrl Pts',(-71.8123058619042,7.90584669580958,
0.));
#146020=CARTESIAN_POINT('Ctrl Pts',(-71.8123058619042,7.90584669580958,
12.));
#146021=CARTESIAN_POINT('Ctrl Pts',(-71.7904712930175,7.8948247213214,0.));
#146022=CARTESIAN_POINT('Ctrl Pts',(-71.7904712930175,7.8948247213214,12.));
#146023=CARTESIAN_POINT('Ctrl Pts',(-71.7686630348238,7.88384247914526,
0.));
#146024=CARTESIAN_POINT('Ctrl Pts',(-71.7686630348238,7.88384247914526,
12.));
#146025=CARTESIAN_POINT('Ctrl Pts',(-71.7468812162788,7.87289996819656,
0.));
#146026=CARTESIAN_POINT('Ctrl Pts',(-71.7468812162788,7.87289996819656,
12.));
#146027=CARTESIAN_POINT('Ctrl Pts',(-71.7251259668563,7.86199718728829,
0.));
#146028=CARTESIAN_POINT('Ctrl Pts',(-71.7251259668563,7.86199718728829,
12.));
#146029=CARTESIAN_POINT('Ctrl Pts',(-71.7033974165568,7.85113413513738,
0.));
#146030=CARTESIAN_POINT('Ctrl Pts',(-71.7033974165568,7.85113413513738,
12.));
#146031=CARTESIAN_POINT('Ctrl Pts',(-71.6816956959117,7.84031081036492,
0.));
#146032=CARTESIAN_POINT('Ctrl Pts',(-71.6816956959117,7.84031081036492,
12.));
#146033=CARTESIAN_POINT('Ctrl Pts',(-71.6600209359872,7.8295272114951,0.));
#146034=CARTESIAN_POINT('Ctrl Pts',(-71.6600209359872,7.8295272114951,12.));
#146035=CARTESIAN_POINT('Ctrl Pts',(-71.6383732683844,7.81878333694863,
0.));
#146036=CARTESIAN_POINT('Ctrl Pts',(-71.6383732683844,7.81878333694863,
12.));
#146037=CARTESIAN_POINT('Ctrl Pts',(-71.6167528252423,7.80807918504024,
0.));
#146038=CARTESIAN_POINT('Ctrl Pts',(-71.6167528252423,7.80807918504024,
12.));
#146039=CARTESIAN_POINT('Ctrl Pts',(-71.5951597392471,7.79741475398516,
0.));
#146040=CARTESIAN_POINT('Ctrl Pts',(-71.5951597392471,7.79741475398516,
12.));
#146041=CARTESIAN_POINT('Ctrl Pts',(-71.5735941436364,7.78679004189937,
0.));
#146042=CARTESIAN_POINT('Ctrl Pts',(-71.5735941436364,7.78679004189937,
12.));
#146043=CARTESIAN_POINT('Ctrl Pts',(-71.5520561722039,7.77620504679872,
0.));
#146044=CARTESIAN_POINT('Ctrl Pts',(-71.5520561722039,7.77620504679872,
12.));
#146045=CARTESIAN_POINT('Ctrl Pts',(-71.5305459592994,7.76565976659228,
0.));
#146046=CARTESIAN_POINT('Ctrl Pts',(-71.5305459592994,7.76565976659228,
12.));
#146047=CARTESIAN_POINT('Ctrl Pts',(-71.5090636398318,7.75515419907969,
0.));
#146048=CARTESIAN_POINT('Ctrl Pts',(-71.5090636398318,7.75515419907969,
12.));
#146049=CARTESIAN_POINT('Ctrl Pts',(-71.4876093492781,7.74468834195749,
0.));
#146050=CARTESIAN_POINT('Ctrl Pts',(-71.4876093492781,7.74468834195749,
12.));
#146051=CARTESIAN_POINT('Ctrl Pts',(-71.4661832236888,7.73426219281942,
0.));
#146052=CARTESIAN_POINT('Ctrl Pts',(-71.4661832236888,7.73426219281942,
12.));
#146053=CARTESIAN_POINT('Ctrl Pts',(-71.4447853996916,7.72387574915546,
0.));
#146054=CARTESIAN_POINT('Ctrl Pts',(-71.4447853996916,7.72387574915546,
12.));
#146055=CARTESIAN_POINT('Ctrl Pts',(-71.4234160144925,7.71352900834522,
0.));
#146056=CARTESIAN_POINT('Ctrl Pts',(-71.4234160144925,7.71352900834522,
12.));
#146057=CARTESIAN_POINT('Ctrl Pts',(-71.4020752058796,7.70322196765541,
0.));
#146058=CARTESIAN_POINT('Ctrl Pts',(-71.4020752058796,7.70322196765541,
12.));
#146059=CARTESIAN_POINT('Ctrl Pts',(-71.380763112233,7.69295462424614,0.));
#146060=CARTESIAN_POINT('Ctrl Pts',(-71.380763112233,7.69295462424614,12.));
#146061=CARTESIAN_POINT('Ctrl Pts',(-71.3594798725281,7.68272697517089,
0.));
#146062=CARTESIAN_POINT('Ctrl Pts',(-71.3594798725281,7.68272697517089,
12.));
#146063=CARTESIAN_POINT('Ctrl Pts',(-71.3382256263414,7.67253901737555,
0.));
#146064=CARTESIAN_POINT('Ctrl Pts',(-71.3382256263414,7.67253901737555,
12.));
#146065=CARTESIAN_POINT('Ctrl Pts',(-71.3170005138502,7.66239074769165,
0.));
#146066=CARTESIAN_POINT('Ctrl Pts',(-71.3170005138502,7.66239074769165,
12.));
#146067=CARTESIAN_POINT('Ctrl Pts',(-71.2958046758372,7.65228216283406,
0.));
#146068=CARTESIAN_POINT('Ctrl Pts',(-71.2958046758372,7.65228216283406,
12.));
#146069=CARTESIAN_POINT('Ctrl Pts',(-71.2746382537007,7.64221325940727,
0.));
#146070=CARTESIAN_POINT('Ctrl Pts',(-71.2746382537007,7.64221325940727,
12.));
#146071=CARTESIAN_POINT('Ctrl Pts',(-71.2535013894602,7.6321840339054,0.));
#146072=CARTESIAN_POINT('Ctrl Pts',(-71.2535013894602,7.6321840339054,12.));
#146073=CARTESIAN_POINT('Ctrl Pts',(-71.2323942257609,7.62219448271111,
0.));
#146074=CARTESIAN_POINT('Ctrl Pts',(-71.2323942257609,7.62219448271111,
12.));
#146075=CARTESIAN_POINT('Ctrl Pts',(-71.211316905874,7.6122446020884,0.));
#146076=CARTESIAN_POINT('Ctrl Pts',(-71.211316905874,7.6122446020884,12.));
#146077=CARTESIAN_POINT('Ctrl Pts',(-71.1902695737013,7.60233438818099,
0.));
#146078=CARTESIAN_POINT('Ctrl Pts',(-71.1902695737013,7.60233438818099,
12.));
#146079=CARTESIAN_POINT('Ctrl Pts',(-71.1692523737844,7.59246383701816,
0.));
#146080=CARTESIAN_POINT('Ctrl Pts',(-71.1692523737844,7.59246383701816,
12.));
#146081=CARTESIAN_POINT('Ctrl Pts',(-71.1482654513119,7.58263294451454,
0.));
#146082=CARTESIAN_POINT('Ctrl Pts',(-71.1482654513119,7.58263294451454,
12.));
#146083=CARTESIAN_POINT('Ctrl Pts',(-71.1273089521234,7.57284170646889,
0.));
#146084=CARTESIAN_POINT('Ctrl Pts',(-71.1273089521234,7.57284170646889,
12.));
#146085=CARTESIAN_POINT('Ctrl Pts',(-71.106383022711,7.5630901185566,0.));
#146086=CARTESIAN_POINT('Ctrl Pts',(-71.106383022711,7.5630901185566,12.));
#146087=CARTESIAN_POINT('Ctrl Pts',(-71.0854878102243,7.55337817632919,
0.));
#146088=CARTESIAN_POINT('Ctrl Pts',(-71.0854878102243,7.55337817632919,
12.));
#146089=CARTESIAN_POINT('Ctrl Pts',(-71.0646234624811,7.54370587521982,
0.));
#146090=CARTESIAN_POINT('Ctrl Pts',(-71.0646234624811,7.54370587521982,
12.));
#146091=CARTESIAN_POINT('Ctrl Pts',(-71.043790127973,7.53407321054265,0.));
#146092=CARTESIAN_POINT('Ctrl Pts',(-71.043790127973,7.53407321054265,12.));
#146093=CARTESIAN_POINT('Ctrl Pts',(-71.0229879558699,7.52448017749127,
0.));
#146094=CARTESIAN_POINT('Ctrl Pts',(-71.0229879558699,7.52448017749127,
12.));
#146095=CARTESIAN_POINT('Ctrl Pts',(-71.0022170960211,7.51492677113092,
0.));
#146096=CARTESIAN_POINT('Ctrl Pts',(-71.0022170960211,7.51492677113092,
12.));
#146097=CARTESIAN_POINT('Ctrl Pts',(-70.9814776989612,7.50541298639931,
0.));
#146098=CARTESIAN_POINT('Ctrl Pts',(-70.9814776989612,7.50541298639931,
12.));
#146099=CARTESIAN_POINT('Ctrl Pts',(-70.9607699159218,7.49593881811132,
0.));
#146100=CARTESIAN_POINT('Ctrl Pts',(-70.9607699159218,7.49593881811132,
12.));
#146101=CARTESIAN_POINT('Ctrl Pts',(-70.940093898837,7.48650426095826,0.));
#146102=CARTESIAN_POINT('Ctrl Pts',(-70.940093898837,7.48650426095826,12.));
#146103=CARTESIAN_POINT('Ctrl Pts',(-70.9194498003493,7.47710930950564,
0.));
#146104=CARTESIAN_POINT('Ctrl Pts',(-70.9194498003493,7.47710930950564,
12.));
#146105=CARTESIAN_POINT('Ctrl Pts',(-70.8988377738104,7.46775395818529,
0.));
#146106=CARTESIAN_POINT('Ctrl Pts',(-70.8988377738104,7.46775395818529,
12.));
#146107=CARTESIAN_POINT('Ctrl Pts',(-70.87825797329,7.45843820129784,0.));
#146108=CARTESIAN_POINT('Ctrl Pts',(-70.87825797329,7.45843820129784,12.));
#146109=CARTESIAN_POINT('Ctrl Pts',(-70.8577105535848,7.4491620330165,0.));
#146110=CARTESIAN_POINT('Ctrl Pts',(-70.8577105535848,7.4491620330165,12.));
#146111=CARTESIAN_POINT('Ctrl Pts',(-70.8371956702241,7.43992544738608,
0.));
#146112=CARTESIAN_POINT('Ctrl Pts',(-70.8371956702241,7.43992544738608,
12.));
#146113=CARTESIAN_POINT('Ctrl Pts',(-70.8167134794737,7.43072843832017,
0.));
#146114=CARTESIAN_POINT('Ctrl Pts',(-70.8167134794737,7.43072843832017,
12.));
#146115=CARTESIAN_POINT('Ctrl Pts',(-70.7962641383349,7.42157099959328,
0.));
#146116=CARTESIAN_POINT('Ctrl Pts',(-70.7962641383349,7.42157099959328,
12.));
#146117=CARTESIAN_POINT('Ctrl Pts',(-70.7758478045576,7.412453124845,0.));
#146118=CARTESIAN_POINT('Ctrl Pts',(-70.7758478045576,7.412453124845,12.));
#146119=CARTESIAN_POINT('Ctrl Pts',(-70.7554646366514,7.4033748075824,0.));
#146120=CARTESIAN_POINT('Ctrl Pts',(-70.7554646366514,7.4033748075824,12.));
#146121=CARTESIAN_POINT('Ctrl Pts',(-70.735114793895,7.39433604117894,0.));
#146122=CARTESIAN_POINT('Ctrl Pts',(-70.735114793895,7.39433604117894,12.));
#146123=CARTESIAN_POINT('Ctrl Pts',(-70.7147984363423,7.3853368188703,0.));
#146124=CARTESIAN_POINT('Ctrl Pts',(-70.7147984363423,7.3853368188703,12.));
#146125=CARTESIAN_POINT('Ctrl Pts',(-70.6945157248269,7.37637713374763,
0.));
#146126=CARTESIAN_POINT('Ctrl Pts',(-70.6945157248269,7.37637713374763,
12.));
#146127=CARTESIAN_POINT('Ctrl Pts',(-70.6742668209685,7.36745697876297,
0.));
#146128=CARTESIAN_POINT('Ctrl Pts',(-70.6742668209685,7.36745697876297,
12.));
#146129=CARTESIAN_POINT('Ctrl Pts',(-70.6540518871772,7.35857634673054,
0.));
#146130=CARTESIAN_POINT('Ctrl Pts',(-70.6540518871772,7.35857634673054,
12.));
#146131=CARTESIAN_POINT('Ctrl Pts',(-70.6338710866562,7.34973523032583,
0.));
#146132=CARTESIAN_POINT('Ctrl Pts',(-70.6338710866562,7.34973523032583,
12.));
#146133=CARTESIAN_POINT('Ctrl Pts',(-70.6137245834002,7.3409336220802,0.));
#146134=CARTESIAN_POINT('Ctrl Pts',(-70.6137245834002,7.3409336220802,12.));
#146135=CARTESIAN_POINT('Ctrl Pts',(-70.5936125421958,7.3321715143761,0.));
#146136=CARTESIAN_POINT('Ctrl Pts',(-70.5936125421958,7.3321715143761,12.));
#146137=CARTESIAN_POINT('Ctrl Pts',(-70.573535128649,7.3234488994524,0.));
#146138=CARTESIAN_POINT('Ctrl Pts',(-70.573535128649,7.3234488994524,12.));
#146139=CARTESIAN_POINT('Ctrl Pts',(-70.5534925092052,7.31476576940406,
0.));
#146140=CARTESIAN_POINT('Ctrl Pts',(-70.5534925092052,7.31476576940406,
12.));
#146141=CARTESIAN_POINT('Ctrl Pts',(-70.5334848511675,7.30612211618049,
0.));
#146142=CARTESIAN_POINT('Ctrl Pts',(-70.5334848511675,7.30612211618049,
12.));
#146143=CARTESIAN_POINT('Ctrl Pts',(-70.5135123227147,7.29751793157804,
0.));
#146144=CARTESIAN_POINT('Ctrl Pts',(-70.5135123227147,7.29751793157804,
12.));
#146145=CARTESIAN_POINT('Ctrl Pts',(-70.4935750929029,7.28895320723838,
0.));
#146146=CARTESIAN_POINT('Ctrl Pts',(-70.4935750929029,7.28895320723838,
12.));
#146147=CARTESIAN_POINT('Ctrl Pts',(-70.4736733316463,7.28042793465452,
0.));
#146148=CARTESIAN_POINT('Ctrl Pts',(-70.4736733316463,7.28042793465452,
12.));
#146149=CARTESIAN_POINT('Ctrl Pts',(-70.4538072096986,7.2719421051706,0.));
#146150=CARTESIAN_POINT('Ctrl Pts',(-70.4538072096986,7.2719421051706,12.));
#146151=CARTESIAN_POINT('Ctrl Pts',(-70.433976898636,7.26349570998052,0.));
#146152=CARTESIAN_POINT('Ctrl Pts',(-70.433976898636,7.26349570998052,12.));
#146153=CARTESIAN_POINT('Ctrl Pts',(-70.4141825708207,7.25508874012078,
0.));
#146154=CARTESIAN_POINT('Ctrl Pts',(-70.4141825708207,7.25508874012078,
12.));
#146155=CARTESIAN_POINT('Ctrl Pts',(-70.3944243994532,7.24672118647119,
0.));
#146156=CARTESIAN_POINT('Ctrl Pts',(-70.3944243994532,7.24672118647119,
12.));
#146157=CARTESIAN_POINT('Ctrl Pts',(-70.3747025586569,7.23839303975629,
0.));
#146158=CARTESIAN_POINT('Ctrl Pts',(-70.3747025586569,7.23839303975629,
12.));
#146159=CARTESIAN_POINT('Ctrl Pts',(-70.3550172235486,7.23010429054233,
0.));
#146160=CARTESIAN_POINT('Ctrl Pts',(-70.3550172235486,7.23010429054233,
12.));
#146161=CARTESIAN_POINT('Ctrl Pts',(-70.3353685703097,7.2218549292318,0.));
#146162=CARTESIAN_POINT('Ctrl Pts',(-70.3353685703097,7.2218549292318,12.));
#146163=CARTESIAN_POINT('Ctrl Pts',(-70.3157567762561,7.21364494605427,
0.));
#146164=CARTESIAN_POINT('Ctrl Pts',(-70.3157567762561,7.21364494605427,
12.));
#146165=CARTESIAN_POINT('Ctrl Pts',(-70.2961820197051,7.2054743310746,0.));
#146166=CARTESIAN_POINT('Ctrl Pts',(-70.2961820197051,7.2054743310746,12.));
#146167=CARTESIAN_POINT('Ctrl Pts',(-70.276644479827,7.19734307419863,0.));
#146168=CARTESIAN_POINT('Ctrl Pts',(-70.276644479827,7.19734307419863,12.));
#146169=CARTESIAN_POINT('Ctrl Pts',(-70.2571443365198,7.18925116517565,
0.));
#146170=CARTESIAN_POINT('Ctrl Pts',(-70.2571443365198,7.18925116517565,
12.));
#146171=CARTESIAN_POINT('Ctrl Pts',(-70.2376817702239,7.18119859359803,
0.));
#146172=CARTESIAN_POINT('Ctrl Pts',(-70.2376817702239,7.18119859359803,
12.));
#146173=CARTESIAN_POINT('Ctrl Pts',(-70.2182569619028,7.1731853488975,0.));
#146174=CARTESIAN_POINT('Ctrl Pts',(-70.2182569619028,7.1731853488975,12.));
#146175=CARTESIAN_POINT('Ctrl Pts',(-70.1988700934622,7.16521142033895,
0.));
#146176=CARTESIAN_POINT('Ctrl Pts',(-70.1988700934622,7.16521142033895,
12.));
#146177=CARTESIAN_POINT('Ctrl Pts',(-70.1795213481196,7.15727679700949,
0.));
#146178=CARTESIAN_POINT('Ctrl Pts',(-70.1795213481196,7.15727679700949,
12.));
#146179=CARTESIAN_POINT('Ctrl Pts',(-70.1602109107188,7.14938146780804,
0.));
#146180=CARTESIAN_POINT('Ctrl Pts',(-70.1602109107188,7.14938146780804,
12.));
#146181=CARTESIAN_POINT('Ctrl Pts',(-70.1409389682389,7.14152542142342,
0.));
#146182=CARTESIAN_POINT('Ctrl Pts',(-70.1409389682389,7.14152542142342,
12.));
#146183=CARTESIAN_POINT('Ctrl Pts',(-70.1217057094456,7.13370864634401,
0.));
#146184=CARTESIAN_POINT('Ctrl Pts',(-70.1217057094456,7.13370864634401,
12.));
#146185=CARTESIAN_POINT('Ctrl Pts',(-70.1025113239463,7.12593113088873,
0.));
#146186=CARTESIAN_POINT('Ctrl Pts',(-70.1025113239463,7.12593113088873,
12.));
#146187=CARTESIAN_POINT('Ctrl Pts',(-70.0833560013971,7.11819286322826,
0.));
#146188=CARTESIAN_POINT('Ctrl Pts',(-70.0833560013971,7.11819286322826,
12.));
#146189=CARTESIAN_POINT('Ctrl Pts',(-70.06423993069,7.11049383140484,0.));
#146190=CARTESIAN_POINT('Ctrl Pts',(-70.06423993069,7.11049383140484,12.));
#146191=CARTESIAN_POINT('Ctrl Pts',(-70.0451632990136,7.10283402335094,
0.));
#146192=CARTESIAN_POINT('Ctrl Pts',(-70.0451632990136,7.10283402335094,
12.));
#146193=CARTESIAN_POINT('Ctrl Pts',(-70.0261262936435,7.09521342684304,
0.));
#146194=CARTESIAN_POINT('Ctrl Pts',(-70.0261262936435,7.09521342684304,
12.));
#146195=CARTESIAN_POINT('Ctrl Pts',(-70.0071291040791,7.08763202944276,
0.));
#146196=CARTESIAN_POINT('Ctrl Pts',(-70.0071291040791,7.08763202944276,
12.));
#146197=CARTESIAN_POINT('Ctrl Pts',(-69.988171923787,7.08008981844645,0.));
#146198=CARTESIAN_POINT('Ctrl Pts',(-69.988171923787,7.08008981844645,12.));
#146199=CARTESIAN_POINT('Ctrl Pts',(-69.9692549527256,7.07258678080795,
0.));
#146200=CARTESIAN_POINT('Ctrl Pts',(-69.9692549527256,7.07258678080795,
12.));
#146201=CARTESIAN_POINT('Ctrl Pts',(-69.9503783975676,7.06512290312805,
0.));
#146202=CARTESIAN_POINT('Ctrl Pts',(-69.9503783975676,7.06512290312805,
12.));
#146203=CARTESIAN_POINT('Ctrl Pts',(-69.9315424664252,7.05769817180827,
0.));
#146204=CARTESIAN_POINT('Ctrl Pts',(-69.9315424664252,7.05769817180827,
12.));
#146205=CARTESIAN_POINT('Ctrl Pts',(-69.9127473642086,7.0503125731811,0.));
#146206=CARTESIAN_POINT('Ctrl Pts',(-69.9127473642086,7.0503125731811,12.));
#146207=CARTESIAN_POINT('Ctrl Pts',(-69.8939932885864,7.04296609362189,
0.));
#146208=CARTESIAN_POINT('Ctrl Pts',(-69.8939932885864,7.04296609362189,
12.));
#146209=CARTESIAN_POINT('Ctrl Pts',(-69.8752804235296,7.03565871972267,
0.));
#146210=CARTESIAN_POINT('Ctrl Pts',(-69.8752804235296,7.03565871972267,
12.));
#146211=CARTESIAN_POINT('Ctrl Pts',(-69.8566089455448,7.02839043811865,
0.));
#146212=CARTESIAN_POINT('Ctrl Pts',(-69.8566089455448,7.02839043811865,
12.));
#146213=CARTESIAN_POINT('Ctrl Pts',(-69.8379790360574,7.02116123514489,
0.));
#146214=CARTESIAN_POINT('Ctrl Pts',(-69.8379790360574,7.02116123514489,
12.));
#146215=CARTESIAN_POINT('Ctrl Pts',(-69.8193908913722,7.01397109655458,
0.));
#146216=CARTESIAN_POINT('Ctrl Pts',(-69.8193908913722,7.01397109655458,
12.));
#146217=CARTESIAN_POINT('Ctrl Pts',(-69.8008447346782,7.00682000718107,
0.));
#146218=CARTESIAN_POINT('Ctrl Pts',(-69.8008447346782,7.00682000718107,
12.));
#146219=CARTESIAN_POINT('Ctrl Pts',(-69.7823408242446,6.99970795069402,
0.));
#146220=CARTESIAN_POINT('Ctrl Pts',(-69.7823408242446,6.99970795069402,
12.));
#146221=CARTESIAN_POINT('Ctrl Pts',(-69.7638794280263,6.99263491027862,
0.));
#146222=CARTESIAN_POINT('Ctrl Pts',(-69.7638794280263,6.99263491027862,
12.));
#146223=CARTESIAN_POINT('Ctrl Pts',(-69.7454607995524,6.98560086924175,
0.));
#146224=CARTESIAN_POINT('Ctrl Pts',(-69.7454607995524,6.98560086924175,
12.));
#146225=CARTESIAN_POINT('Ctrl Pts',(-69.7270851557443,6.97860581164571,
0.));
#146226=CARTESIAN_POINT('Ctrl Pts',(-69.7270851557443,6.97860581164571,
12.));
#146227=CARTESIAN_POINT('Ctrl Pts',(-69.7087526480248,6.97164972291584,
0.));
#146228=CARTESIAN_POINT('Ctrl Pts',(-69.7087526480248,6.97164972291584,
12.));
#146229=CARTESIAN_POINT('Ctrl Pts',(-69.6904633605834,6.96473259049732,
0.));
#146230=CARTESIAN_POINT('Ctrl Pts',(-69.6904633605834,6.96473259049732,
12.));
#146231=CARTESIAN_POINT('Ctrl Pts',(-69.6758665380764,6.95923004173798,
0.));
#146232=CARTESIAN_POINT('Ctrl Pts',(-69.6758665380764,6.95923004173798,
12.));
#146233=CARTESIAN_POINT('Ctrl Pts',(-69.6649383920075,6.95512065317733,
0.));
#146234=CARTESIAN_POINT('Ctrl Pts',(-69.6649383920075,6.95512065317733,
12.));
#146235=CARTESIAN_POINT('Ctrl Pts',(-69.6576616146559,6.95238884849078,
0.));
#146236=CARTESIAN_POINT('Ctrl Pts',(-69.6576616146559,6.95238884849078,
12.));
#146237=CARTESIAN_POINT('Ctrl Pts',(-69.6540253893193,6.9510248930693,0.));
#146238=CARTESIAN_POINT('Ctrl Pts',(-69.6540253893193,6.9510248930693,12.));
#146239=CARTESIAN_POINT('',(-69.6540253893193,6.9510248930693,12.));
#146240=CARTESIAN_POINT('Ctrl Pts',(-69.6540253893193,6.9510248930693,12.));
#146241=CARTESIAN_POINT('Ctrl Pts',(-69.6576616146559,6.95238884849078,
12.));
#146242=CARTESIAN_POINT('Ctrl Pts',(-69.6649383920075,6.95512065317733,
12.));
#146243=CARTESIAN_POINT('Ctrl Pts',(-69.6758665380764,6.95923004173798,
12.));
#146244=CARTESIAN_POINT('Ctrl Pts',(-69.6904633605834,6.96473259049732,
12.));
#146245=CARTESIAN_POINT('Ctrl Pts',(-69.7087526480248,6.97164972291584,
12.));
#146246=CARTESIAN_POINT('Ctrl Pts',(-69.7270851557443,6.97860581164571,
12.));
#146247=CARTESIAN_POINT('Ctrl Pts',(-69.7454607995524,6.98560086924175,
12.));
#146248=CARTESIAN_POINT('Ctrl Pts',(-69.7638794280263,6.99263491027862,
12.));
#146249=CARTESIAN_POINT('Ctrl Pts',(-69.7823408242446,6.99970795069402,
12.));
#146250=CARTESIAN_POINT('Ctrl Pts',(-69.8008447346782,7.00682000718107,
12.));
#146251=CARTESIAN_POINT('Ctrl Pts',(-69.8193908913722,7.01397109655458,
12.));
#146252=CARTESIAN_POINT('Ctrl Pts',(-69.8379790360574,7.02116123514489,
12.));
#146253=CARTESIAN_POINT('Ctrl Pts',(-69.8566089455448,7.02839043811865,
12.));
#146254=CARTESIAN_POINT('Ctrl Pts',(-69.8752804235296,7.03565871972267,
12.));
#146255=CARTESIAN_POINT('Ctrl Pts',(-69.8939932885864,7.04296609362189,
12.));
#146256=CARTESIAN_POINT('Ctrl Pts',(-69.9127473642086,7.0503125731811,12.));
#146257=CARTESIAN_POINT('Ctrl Pts',(-69.9315424664252,7.05769817180827,
12.));
#146258=CARTESIAN_POINT('Ctrl Pts',(-69.9503783975676,7.06512290312805,
12.));
#146259=CARTESIAN_POINT('Ctrl Pts',(-69.9692549527256,7.07258678080795,
12.));
#146260=CARTESIAN_POINT('Ctrl Pts',(-69.988171923787,7.08008981844645,12.));
#146261=CARTESIAN_POINT('Ctrl Pts',(-70.0071291040791,7.08763202944276,
12.));
#146262=CARTESIAN_POINT('Ctrl Pts',(-70.0261262936435,7.09521342684304,
12.));
#146263=CARTESIAN_POINT('Ctrl Pts',(-70.0451632990136,7.10283402335094,
12.));
#146264=CARTESIAN_POINT('Ctrl Pts',(-70.06423993069,7.11049383140484,12.));
#146265=CARTESIAN_POINT('Ctrl Pts',(-70.0833560013971,7.11819286322826,
12.));
#146266=CARTESIAN_POINT('Ctrl Pts',(-70.1025113239463,7.12593113088873,
12.));
#146267=CARTESIAN_POINT('Ctrl Pts',(-70.1217057094456,7.13370864634401,
12.));
#146268=CARTESIAN_POINT('Ctrl Pts',(-70.1409389682389,7.14152542142342,
12.));
#146269=CARTESIAN_POINT('Ctrl Pts',(-70.1602109107188,7.14938146780804,
12.));
#146270=CARTESIAN_POINT('Ctrl Pts',(-70.1795213481196,7.15727679700949,
12.));
#146271=CARTESIAN_POINT('Ctrl Pts',(-70.1988700934622,7.16521142033895,
12.));
#146272=CARTESIAN_POINT('Ctrl Pts',(-70.2182569619028,7.1731853488975,12.));
#146273=CARTESIAN_POINT('Ctrl Pts',(-70.2376817702239,7.18119859359803,
12.));
#146274=CARTESIAN_POINT('Ctrl Pts',(-70.2571443365198,7.18925116517565,
12.));
#146275=CARTESIAN_POINT('Ctrl Pts',(-70.276644479827,7.19734307419863,12.));
#146276=CARTESIAN_POINT('Ctrl Pts',(-70.2961820197051,7.2054743310746,12.));
#146277=CARTESIAN_POINT('Ctrl Pts',(-70.3157567762561,7.21364494605427,
12.));
#146278=CARTESIAN_POINT('Ctrl Pts',(-70.3353685703097,7.2218549292318,12.));
#146279=CARTESIAN_POINT('Ctrl Pts',(-70.3550172235486,7.23010429054233,
12.));
#146280=CARTESIAN_POINT('Ctrl Pts',(-70.3747025586569,7.23839303975629,
12.));
#146281=CARTESIAN_POINT('Ctrl Pts',(-70.3944243994532,7.24672118647119,
12.));
#146282=CARTESIAN_POINT('Ctrl Pts',(-70.4141825708207,7.25508874012078,
12.));
#146283=CARTESIAN_POINT('Ctrl Pts',(-70.433976898636,7.26349570998052,12.));
#146284=CARTESIAN_POINT('Ctrl Pts',(-70.4538072096986,7.2719421051706,12.));
#146285=CARTESIAN_POINT('Ctrl Pts',(-70.4736733316463,7.28042793465452,
12.));
#146286=CARTESIAN_POINT('Ctrl Pts',(-70.4935750929029,7.28895320723838,
12.));
#146287=CARTESIAN_POINT('Ctrl Pts',(-70.5135123227147,7.29751793157804,
12.));
#146288=CARTESIAN_POINT('Ctrl Pts',(-70.5334848511675,7.30612211618049,
12.));
#146289=CARTESIAN_POINT('Ctrl Pts',(-70.5534925092052,7.31476576940406,
12.));
#146290=CARTESIAN_POINT('Ctrl Pts',(-70.573535128649,7.3234488994524,12.));
#146291=CARTESIAN_POINT('Ctrl Pts',(-70.5936125421958,7.3321715143761,12.));
#146292=CARTESIAN_POINT('Ctrl Pts',(-70.6137245834002,7.3409336220802,12.));
#146293=CARTESIAN_POINT('Ctrl Pts',(-70.6338710866562,7.34973523032583,
12.));
#146294=CARTESIAN_POINT('Ctrl Pts',(-70.6540518871772,7.35857634673054,
12.));
#146295=CARTESIAN_POINT('Ctrl Pts',(-70.6742668209685,7.36745697876297,
12.));
#146296=CARTESIAN_POINT('Ctrl Pts',(-70.6945157248269,7.37637713374763,
12.));
#146297=CARTESIAN_POINT('Ctrl Pts',(-70.7147984363423,7.3853368188703,12.));
#146298=CARTESIAN_POINT('Ctrl Pts',(-70.735114793895,7.39433604117894,12.));
#146299=CARTESIAN_POINT('Ctrl Pts',(-70.7554646366514,7.4033748075824,12.));
#146300=CARTESIAN_POINT('Ctrl Pts',(-70.7758478045576,7.412453124845,12.));
#146301=CARTESIAN_POINT('Ctrl Pts',(-70.7962641383349,7.42157099959328,
12.));
#146302=CARTESIAN_POINT('Ctrl Pts',(-70.8167134794737,7.43072843832017,
12.));
#146303=CARTESIAN_POINT('Ctrl Pts',(-70.8371956702241,7.43992544738608,
12.));
#146304=CARTESIAN_POINT('Ctrl Pts',(-70.8577105535848,7.4491620330165,12.));
#146305=CARTESIAN_POINT('Ctrl Pts',(-70.87825797329,7.45843820129784,12.));
#146306=CARTESIAN_POINT('Ctrl Pts',(-70.8988377738104,7.46775395818529,
12.));
#146307=CARTESIAN_POINT('Ctrl Pts',(-70.9194498003493,7.47710930950564,
12.));
#146308=CARTESIAN_POINT('Ctrl Pts',(-70.940093898837,7.48650426095826,12.));
#146309=CARTESIAN_POINT('Ctrl Pts',(-70.9607699159218,7.49593881811132,
12.));
#146310=CARTESIAN_POINT('Ctrl Pts',(-70.9814776989612,7.50541298639931,
12.));
#146311=CARTESIAN_POINT('Ctrl Pts',(-71.0022170960211,7.51492677113092,
12.));
#146312=CARTESIAN_POINT('Ctrl Pts',(-71.0229879558699,7.52448017749127,
12.));
#146313=CARTESIAN_POINT('Ctrl Pts',(-71.043790127973,7.53407321054265,12.));
#146314=CARTESIAN_POINT('Ctrl Pts',(-71.0646234624811,7.54370587521982,
12.));
#146315=CARTESIAN_POINT('Ctrl Pts',(-71.0854878102243,7.55337817632919,
12.));
#146316=CARTESIAN_POINT('Ctrl Pts',(-71.106383022711,7.5630901185566,12.));
#146317=CARTESIAN_POINT('Ctrl Pts',(-71.1273089521234,7.57284170646889,
12.));
#146318=CARTESIAN_POINT('Ctrl Pts',(-71.1482654513119,7.58263294451454,
12.));
#146319=CARTESIAN_POINT('Ctrl Pts',(-71.1692523737844,7.59246383701816,
12.));
#146320=CARTESIAN_POINT('Ctrl Pts',(-71.1902695737013,7.60233438818099,
12.));
#146321=CARTESIAN_POINT('Ctrl Pts',(-71.211316905874,7.6122446020884,12.));
#146322=CARTESIAN_POINT('Ctrl Pts',(-71.2323942257609,7.62219448271111,
12.));
#146323=CARTESIAN_POINT('Ctrl Pts',(-71.2535013894602,7.6321840339054,12.));
#146324=CARTESIAN_POINT('Ctrl Pts',(-71.2746382537007,7.64221325940727,
12.));
#146325=CARTESIAN_POINT('Ctrl Pts',(-71.2958046758372,7.65228216283406,
12.));
#146326=CARTESIAN_POINT('Ctrl Pts',(-71.3170005138502,7.66239074769165,
12.));
#146327=CARTESIAN_POINT('Ctrl Pts',(-71.3382256263414,7.67253901737555,
12.));
#146328=CARTESIAN_POINT('Ctrl Pts',(-71.3594798725281,7.68272697517089,
12.));
#146329=CARTESIAN_POINT('Ctrl Pts',(-71.380763112233,7.69295462424614,12.));
#146330=CARTESIAN_POINT('Ctrl Pts',(-71.4020752058796,7.70322196765541,
12.));
#146331=CARTESIAN_POINT('Ctrl Pts',(-71.4234160144925,7.71352900834522,
12.));
#146332=CARTESIAN_POINT('Ctrl Pts',(-71.4447853996916,7.72387574915546,
12.));
#146333=CARTESIAN_POINT('Ctrl Pts',(-71.4661832236888,7.73426219281942,
12.));
#146334=CARTESIAN_POINT('Ctrl Pts',(-71.4876093492781,7.74468834195749,
12.));
#146335=CARTESIAN_POINT('Ctrl Pts',(-71.5090636398318,7.75515419907969,
12.));
#146336=CARTESIAN_POINT('Ctrl Pts',(-71.5305459592994,7.76565976659228,
12.));
#146337=CARTESIAN_POINT('Ctrl Pts',(-71.5520561722039,7.77620504679872,
12.));
#146338=CARTESIAN_POINT('Ctrl Pts',(-71.5735941436364,7.78679004189937,
12.));
#146339=CARTESIAN_POINT('Ctrl Pts',(-71.5951597392471,7.79741475398516,
12.));
#146340=CARTESIAN_POINT('Ctrl Pts',(-71.6167528252423,7.80807918504024,
12.));
#146341=CARTESIAN_POINT('Ctrl Pts',(-71.6383732683844,7.81878333694863,
12.));
#146342=CARTESIAN_POINT('Ctrl Pts',(-71.6600209359872,7.8295272114951,12.));
#146343=CARTESIAN_POINT('Ctrl Pts',(-71.6816956959117,7.84031081036492,
12.));
#146344=CARTESIAN_POINT('Ctrl Pts',(-71.7033974165568,7.85113413513738,
12.));
#146345=CARTESIAN_POINT('Ctrl Pts',(-71.7251259668563,7.86199718728829,
12.));
#146346=CARTESIAN_POINT('Ctrl Pts',(-71.7468812162788,7.87289996819656,
12.));
#146347=CARTESIAN_POINT('Ctrl Pts',(-71.7686630348238,7.88384247914526,
12.));
#146348=CARTESIAN_POINT('Ctrl Pts',(-71.7904712930175,7.8948247213214,12.));
#146349=CARTESIAN_POINT('Ctrl Pts',(-71.8123058619042,7.90584669580958,
12.));
#146350=CARTESIAN_POINT('Ctrl Pts',(-71.8341666130426,7.91690840359369,
12.));
#146351=CARTESIAN_POINT('Ctrl Pts',(-71.8560534185071,7.92800984556398,
12.));
#146352=CARTESIAN_POINT('Ctrl Pts',(-71.8779661508832,7.93915102251797,
12.));
#146353=CARTESIAN_POINT('Ctrl Pts',(-71.8999046832643,7.95033193516053,
12.));
#146354=CARTESIAN_POINT('Ctrl Pts',(-71.9218688892431,7.96155258409766,
12.));
#146355=CARTESIAN_POINT('Ctrl Pts',(-71.943858642908,7.9728129698372,12.));
#146356=CARTESIAN_POINT('Ctrl Pts',(-71.965873818843,7.98411309279615,12.));
#146357=CARTESIAN_POINT('Ctrl Pts',(-71.9879142921254,7.99545295330193,
12.));
#146358=CARTESIAN_POINT('Ctrl Pts',(-72.0099799383213,8.0068325515925,12.));
#146359=CARTESIAN_POINT('Ctrl Pts',(-72.032070633479,8.01825188781059,12.));
#146360=CARTESIAN_POINT('Ctrl Pts',(-72.0541862541243,8.0297109620031,12.));
#146361=CARTESIAN_POINT('Ctrl Pts',(-72.0763266772615,8.04120977412874,
12.));
#146362=CARTESIAN_POINT('Ctrl Pts',(-72.0984917803693,8.05274832405951,
12.));
#146363=CARTESIAN_POINT('Ctrl Pts',(-72.1206814413988,8.06432661158098,
12.));
#146364=CARTESIAN_POINT('Ctrl Pts',(-72.1428955387663,8.07594463638721,
12.));
#146365=CARTESIAN_POINT('Ctrl Pts',(-72.1651339513477,8.08760239807839,
12.));
#146366=CARTESIAN_POINT('Ctrl Pts',(-72.1873965584813,8.09929989616892,
12.));
#146367=CARTESIAN_POINT('Ctrl Pts',(-72.209683239963,8.11103713008931,12.));
#146368=CARTESIAN_POINT('Ctrl Pts',(-72.2319938760449,8.12281409918663,
12.));
#146369=CARTESIAN_POINT('Ctrl Pts',(-72.2543283474278,8.13463080272031,
12.));
#146370=CARTESIAN_POINT('Ctrl Pts',(-72.2766865352555,8.146487239858,12.));
#146371=CARTESIAN_POINT('Ctrl Pts',(-72.2990683211162,8.15838340968338,
12.));
#146372=CARTESIAN_POINT('Ctrl Pts',(-72.3214735870409,8.17031931119893,
12.));
#146373=CARTESIAN_POINT('Ctrl Pts',(-72.3439022155007,8.18229494332626,
12.));
#146374=CARTESIAN_POINT('Ctrl Pts',(-72.3663540894026,8.19431030490317,
12.));
#146375=CARTESIAN_POINT('Ctrl Pts',(-72.3888290920832,8.20636539467778,
12.));
#146376=CARTESIAN_POINT('Ctrl Pts',(-72.4113271073079,8.21846021131563,
12.));
#146377=CARTESIAN_POINT('Ctrl Pts',(-72.4338480192694,8.23059475340359,
12.));
#146378=CARTESIAN_POINT('Ctrl Pts',(-72.4563917125842,8.24276901945042,
12.));
#146379=CARTESIAN_POINT('Ctrl Pts',(-72.4789580722875,8.25498300788496,
12.));
#146380=CARTESIAN_POINT('Ctrl Pts',(-72.5015469838254,8.26723671704922,
12.));
#146381=CARTESIAN_POINT('Ctrl Pts',(-72.5241583330562,8.27953014520378,
12.));
#146382=CARTESIAN_POINT('Ctrl Pts',(-72.5467920062521,8.29186329053282,
12.));
#146383=CARTESIAN_POINT('Ctrl Pts',(-72.5694478900981,8.30423615114455,
12.));
#146384=CARTESIAN_POINT('Ctrl Pts',(-72.5921258716901,8.31664872507019,
12.));
#146385=CARTESIAN_POINT('Ctrl Pts',(-72.6148258385296,8.32910101025673,
12.));
#146386=CARTESIAN_POINT('Ctrl Pts',(-72.6375476785215,8.34159300456989,
12.));
#146387=CARTESIAN_POINT('Ctrl Pts',(-72.6602912799696,8.35412470580104,
12.));
#146388=CARTESIAN_POINT('Ctrl Pts',(-72.6830565315703,8.36669611166845,
12.));
#146389=CARTESIAN_POINT('Ctrl Pts',(-72.705843322407,8.37930721981733,12.));
#146390=CARTESIAN_POINT('Ctrl Pts',(-72.7286515419372,8.39195802781393,
12.));
#146391=CARTESIAN_POINT('Ctrl Pts',(-72.751481079992,8.40464853314471,12.));
#146392=CARTESIAN_POINT('Ctrl Pts',(-72.7743318267865,8.41737873322332,
12.));
#146393=CARTESIAN_POINT('Ctrl Pts',(-72.7972036729276,8.4301486253916,12.));
#146394=CARTESIAN_POINT('Ctrl Pts',(-72.8200965094199,8.44295820691914,
12.));
#146395=CARTESIAN_POINT('Ctrl Pts',(-72.8430102276713,8.45580747499796,
12.));
#146396=CARTESIAN_POINT('Ctrl Pts',(-72.8659447194933,8.46869642673797,
12.));
#146397=CARTESIAN_POINT('Ctrl Pts',(-72.8888998770785,8.4816250591766,12.));
#146398=CARTESIAN_POINT('Ctrl Pts',(-72.9118755929795,8.49459336928298,
12.));
#146399=CARTESIAN_POINT('Ctrl Pts',(-72.9348717600838,8.50760135395986,
12.));
#146400=CARTESIAN_POINT('Ctrl Pts',(-72.9578882715912,8.5206490100423,12.));
#146401=CARTESIAN_POINT('Ctrl Pts',(-72.9809250209828,8.53373633429283,
12.));
#146402=CARTESIAN_POINT('Ctrl Pts',(-73.0039819020648,8.5468633234042,12.));
#146403=CARTESIAN_POINT('Ctrl Pts',(-73.0270588090183,8.56002997400086,
12.));
#146404=CARTESIAN_POINT('Ctrl Pts',(-73.0501556364479,8.57323628263595,
12.));
#146405=CARTESIAN_POINT('Ctrl Pts',(-73.0732722794195,8.58648224578734,
12.));
#146406=CARTESIAN_POINT('Ctrl Pts',(-73.0964086335235,8.59976785984554,
12.));
#146407=CARTESIAN_POINT('Ctrl Pts',(-73.1195645948178,8.61309312112004,
12.));
#146408=CARTESIAN_POINT('Ctrl Pts',(-73.1427400597037,8.62645802585486,
12.));
#146409=CARTESIAN_POINT('Ctrl Pts',(-73.1659349248132,8.63986257023741,
12.));
#146410=CARTESIAN_POINT('Ctrl Pts',(-73.1891490869056,8.65330675040539,
12.));
#146411=CARTESIAN_POINT('Ctrl Pts',(-73.2123824427208,8.66679056245095,
12.));
#146412=CARTESIAN_POINT('Ctrl Pts',(-73.2356348889693,8.68031400241874,
12.));
#146413=CARTESIAN_POINT('Ctrl Pts',(-73.2589063226358,8.69387706629287,
12.));
#146414=CARTESIAN_POINT('Ctrl Pts',(-73.2821966412148,8.70747974998232,
12.));
#146415=CARTESIAN_POINT('Ctrl Pts',(-73.3055057429742,8.72112204930234,
12.));
#146416=CARTESIAN_POINT('Ctrl Pts',(-73.3288335272002,8.73480395995383,
12.));
#146417=CARTESIAN_POINT('Ctrl Pts',(-73.3521798944622,8.74852547749781,
12.));
#146418=CARTESIAN_POINT('Ctrl Pts',(-73.3755447460268,8.7622865974036,12.));
#146419=CARTESIAN_POINT('Ctrl Pts',(-73.3989279832835,8.7760873150935,12.));
#146420=CARTESIAN_POINT('Ctrl Pts',(-73.422329507113,8.78992762598759,12.));
#146421=CARTESIAN_POINT('Ctrl Pts',(-73.4457492173933,8.80380752553694,
12.));
#146422=CARTESIAN_POINT('Ctrl Pts',(-73.4691870121567,8.81772700927533,
12.));
#146423=CARTESIAN_POINT('Ctrl Pts',(-73.492642788273,8.83168607277327,12.));
#146424=CARTESIAN_POINT('Ctrl Pts',(-73.5161164429709,8.84568471153808,
12.));
#146425=CARTESIAN_POINT('Ctrl Pts',(-73.5396078751639,8.85972292092133,
12.));
#146426=CARTESIAN_POINT('Ctrl Pts',(-73.5631169867122,8.87380069602973,
12.));
#146427=CARTESIAN_POINT('Ctrl Pts',(-73.5866436840556,8.88791803160445,
12.));
#146428=CARTESIAN_POINT('Ctrl Pts',(-73.6101878785976,8.90207492199045,
12.));
#146429=CARTESIAN_POINT('Ctrl Pts',(-73.6303847393629,8.914244021516,12.));
#146430=CARTESIAN_POINT('Ctrl Pts',(-73.6458786306023,8.92359518178491,
12.));
#146431=CARTESIAN_POINT('Ctrl Pts',(-73.6566618622073,8.93011088817314,
12.));
#146432=CARTESIAN_POINT('Ctrl Pts',(-73.6627293782587,8.93377955965632,
12.));
#146433=CARTESIAN_POINT('Ctrl Pts',(-73.6640787198055,8.93459554657838,
12.));
#146434=CARTESIAN_POINT('',(-69.6540253893193,6.9510248930693,0.));
#146435=CARTESIAN_POINT('',(-69.6540253893193,6.9510248930693,0.));
#146436=CARTESIAN_POINT('Ctrl Pts',(-73.6640787198055,8.93459554657839,
0.));
#146437=CARTESIAN_POINT('Ctrl Pts',(-73.6627293782587,8.93377955965634,
0.));
#146438=CARTESIAN_POINT('Ctrl Pts',(-73.6566618622074,8.93011088817316,
0.));
#146439=CARTESIAN_POINT('Ctrl Pts',(-73.6458786306023,8.92359518178491,
0.));
#146440=CARTESIAN_POINT('Ctrl Pts',(-73.6303847393629,8.914244021516,0.));
#146441=CARTESIAN_POINT('Ctrl Pts',(-73.6101878785976,8.90207492199045,
0.));
#146442=CARTESIAN_POINT('Ctrl Pts',(-73.5866436840556,8.88791803160445,
0.));
#146443=CARTESIAN_POINT('Ctrl Pts',(-73.5631169867122,8.87380069602973,
0.));
#146444=CARTESIAN_POINT('Ctrl Pts',(-73.5396078751639,8.85972292092133,
0.));
#146445=CARTESIAN_POINT('Ctrl Pts',(-73.5161164429709,8.84568471153808,
0.));
#146446=CARTESIAN_POINT('Ctrl Pts',(-73.492642788273,8.83168607277327,0.));
#146447=CARTESIAN_POINT('Ctrl Pts',(-73.4691870121567,8.81772700927533,
0.));
#146448=CARTESIAN_POINT('Ctrl Pts',(-73.4457492173933,8.80380752553694,
0.));
#146449=CARTESIAN_POINT('Ctrl Pts',(-73.422329507113,8.78992762598759,0.));
#146450=CARTESIAN_POINT('Ctrl Pts',(-73.3989279832835,8.7760873150935,0.));
#146451=CARTESIAN_POINT('Ctrl Pts',(-73.3755447460268,8.7622865974036,0.));
#146452=CARTESIAN_POINT('Ctrl Pts',(-73.3521798944622,8.74852547749781,
0.));
#146453=CARTESIAN_POINT('Ctrl Pts',(-73.3288335272002,8.73480395995383,
0.));
#146454=CARTESIAN_POINT('Ctrl Pts',(-73.3055057429742,8.72112204930234,
0.));
#146455=CARTESIAN_POINT('Ctrl Pts',(-73.2821966412148,8.70747974998232,
0.));
#146456=CARTESIAN_POINT('Ctrl Pts',(-73.2589063226358,8.69387706629287,
0.));
#146457=CARTESIAN_POINT('Ctrl Pts',(-73.2356348889693,8.68031400241874,
0.));
#146458=CARTESIAN_POINT('Ctrl Pts',(-73.2123824427208,8.66679056245095,
0.));
#146459=CARTESIAN_POINT('Ctrl Pts',(-73.1891490869056,8.65330675040539,
0.));
#146460=CARTESIAN_POINT('Ctrl Pts',(-73.1659349248132,8.63986257023741,
0.));
#146461=CARTESIAN_POINT('Ctrl Pts',(-73.1427400597037,8.62645802585486,
0.));
#146462=CARTESIAN_POINT('Ctrl Pts',(-73.1195645948178,8.61309312112004,
0.));
#146463=CARTESIAN_POINT('Ctrl Pts',(-73.0964086335235,8.59976785984554,
0.));
#146464=CARTESIAN_POINT('Ctrl Pts',(-73.0732722794195,8.58648224578734,
0.));
#146465=CARTESIAN_POINT('Ctrl Pts',(-73.0501556364479,8.57323628263595,
0.));
#146466=CARTESIAN_POINT('Ctrl Pts',(-73.0270588090183,8.56002997400086,
0.));
#146467=CARTESIAN_POINT('Ctrl Pts',(-73.0039819020648,8.5468633234042,0.));
#146468=CARTESIAN_POINT('Ctrl Pts',(-72.9809250209828,8.53373633429283,
0.));
#146469=CARTESIAN_POINT('Ctrl Pts',(-72.9578882715912,8.5206490100423,0.));
#146470=CARTESIAN_POINT('Ctrl Pts',(-72.9348717600838,8.50760135395986,
0.));
#146471=CARTESIAN_POINT('Ctrl Pts',(-72.9118755929795,8.49459336928298,
0.));
#146472=CARTESIAN_POINT('Ctrl Pts',(-72.8888998770785,8.4816250591766,0.));
#146473=CARTESIAN_POINT('Ctrl Pts',(-72.8659447194933,8.46869642673797,
0.));
#146474=CARTESIAN_POINT('Ctrl Pts',(-72.8430102276713,8.45580747499796,
0.));
#146475=CARTESIAN_POINT('Ctrl Pts',(-72.8200965094199,8.44295820691914,
0.));
#146476=CARTESIAN_POINT('Ctrl Pts',(-72.7972036729276,8.4301486253916,0.));
#146477=CARTESIAN_POINT('Ctrl Pts',(-72.7743318267865,8.41737873322332,
0.));
#146478=CARTESIAN_POINT('Ctrl Pts',(-72.751481079992,8.40464853314471,0.));
#146479=CARTESIAN_POINT('Ctrl Pts',(-72.7286515419372,8.39195802781393,
0.));
#146480=CARTESIAN_POINT('Ctrl Pts',(-72.705843322407,8.37930721981733,0.));
#146481=CARTESIAN_POINT('Ctrl Pts',(-72.6830565315703,8.36669611166845,
0.));
#146482=CARTESIAN_POINT('Ctrl Pts',(-72.6602912799696,8.35412470580104,
0.));
#146483=CARTESIAN_POINT('Ctrl Pts',(-72.6375476785215,8.34159300456989,
0.));
#146484=CARTESIAN_POINT('Ctrl Pts',(-72.6148258385296,8.32910101025673,
0.));
#146485=CARTESIAN_POINT('Ctrl Pts',(-72.5921258716901,8.31664872507019,
0.));
#146486=CARTESIAN_POINT('Ctrl Pts',(-72.5694478900981,8.30423615114455,
0.));
#146487=CARTESIAN_POINT('Ctrl Pts',(-72.5467920062521,8.29186329053282,
0.));
#146488=CARTESIAN_POINT('Ctrl Pts',(-72.5241583330562,8.27953014520378,
0.));
#146489=CARTESIAN_POINT('Ctrl Pts',(-72.5015469838254,8.26723671704922,
0.));
#146490=CARTESIAN_POINT('Ctrl Pts',(-72.4789580722875,8.25498300788496,
0.));
#146491=CARTESIAN_POINT('Ctrl Pts',(-72.4563917125842,8.24276901945042,
0.));
#146492=CARTESIAN_POINT('Ctrl Pts',(-72.4338480192694,8.23059475340359,
0.));
#146493=CARTESIAN_POINT('Ctrl Pts',(-72.4113271073079,8.21846021131563,
0.));
#146494=CARTESIAN_POINT('Ctrl Pts',(-72.3888290920832,8.20636539467778,
0.));
#146495=CARTESIAN_POINT('Ctrl Pts',(-72.3663540894026,8.19431030490317,
0.));
#146496=CARTESIAN_POINT('Ctrl Pts',(-72.3439022155007,8.18229494332626,
0.));
#146497=CARTESIAN_POINT('Ctrl Pts',(-72.3214735870409,8.17031931119893,
0.));
#146498=CARTESIAN_POINT('Ctrl Pts',(-72.2990683211162,8.15838340968338,
0.));
#146499=CARTESIAN_POINT('Ctrl Pts',(-72.2766865352555,8.146487239858,0.));
#146500=CARTESIAN_POINT('Ctrl Pts',(-72.2543283474278,8.13463080272031,
0.));
#146501=CARTESIAN_POINT('Ctrl Pts',(-72.2319938760449,8.12281409918663,
0.));
#146502=CARTESIAN_POINT('Ctrl Pts',(-72.209683239963,8.11103713008931,0.));
#146503=CARTESIAN_POINT('Ctrl Pts',(-72.1873965584813,8.09929989616892,
0.));
#146504=CARTESIAN_POINT('Ctrl Pts',(-72.1651339513477,8.08760239807839,
0.));
#146505=CARTESIAN_POINT('Ctrl Pts',(-72.1428955387663,8.07594463638721,
0.));
#146506=CARTESIAN_POINT('Ctrl Pts',(-72.1206814413988,8.06432661158098,
0.));
#146507=CARTESIAN_POINT('Ctrl Pts',(-72.0984917803693,8.05274832405951,
0.));
#146508=CARTESIAN_POINT('Ctrl Pts',(-72.0763266772615,8.04120977412874,
0.));
#146509=CARTESIAN_POINT('Ctrl Pts',(-72.0541862541243,8.0297109620031,0.));
#146510=CARTESIAN_POINT('Ctrl Pts',(-72.032070633479,8.01825188781059,0.));
#146511=CARTESIAN_POINT('Ctrl Pts',(-72.0099799383213,8.0068325515925,0.));
#146512=CARTESIAN_POINT('Ctrl Pts',(-71.9879142921254,7.99545295330193,
0.));
#146513=CARTESIAN_POINT('Ctrl Pts',(-71.965873818843,7.98411309279615,0.));
#146514=CARTESIAN_POINT('Ctrl Pts',(-71.943858642908,7.9728129698372,0.));
#146515=CARTESIAN_POINT('Ctrl Pts',(-71.9218688892431,7.96155258409766,
0.));
#146516=CARTESIAN_POINT('Ctrl Pts',(-71.8999046832643,7.95033193516053,
0.));
#146517=CARTESIAN_POINT('Ctrl Pts',(-71.8779661508832,7.93915102251797,
0.));
#146518=CARTESIAN_POINT('Ctrl Pts',(-71.8560534185071,7.92800984556398,
0.));
#146519=CARTESIAN_POINT('Ctrl Pts',(-71.8341666130426,7.91690840359369,
0.));
#146520=CARTESIAN_POINT('Ctrl Pts',(-71.8123058619042,7.90584669580958,
0.));
#146521=CARTESIAN_POINT('Ctrl Pts',(-71.7904712930175,7.8948247213214,0.));
#146522=CARTESIAN_POINT('Ctrl Pts',(-71.7686630348238,7.88384247914526,
0.));
#146523=CARTESIAN_POINT('Ctrl Pts',(-71.7468812162788,7.87289996819656,
0.));
#146524=CARTESIAN_POINT('Ctrl Pts',(-71.7251259668563,7.86199718728829,
0.));
#146525=CARTESIAN_POINT('Ctrl Pts',(-71.7033974165568,7.85113413513738,
0.));
#146526=CARTESIAN_POINT('Ctrl Pts',(-71.6816956959117,7.84031081036492,
0.));
#146527=CARTESIAN_POINT('Ctrl Pts',(-71.6600209359872,7.8295272114951,0.));
#146528=CARTESIAN_POINT('Ctrl Pts',(-71.6383732683844,7.81878333694863,
0.));
#146529=CARTESIAN_POINT('Ctrl Pts',(-71.6167528252423,7.80807918504024,
0.));
#146530=CARTESIAN_POINT('Ctrl Pts',(-71.5951597392471,7.79741475398516,
0.));
#146531=CARTESIAN_POINT('Ctrl Pts',(-71.5735941436364,7.78679004189937,
0.));
#146532=CARTESIAN_POINT('Ctrl Pts',(-71.5520561722039,7.77620504679872,
0.));
#146533=CARTESIAN_POINT('Ctrl Pts',(-71.5305459592994,7.76565976659228,
0.));
#146534=CARTESIAN_POINT('Ctrl Pts',(-71.5090636398318,7.75515419907969,
0.));
#146535=CARTESIAN_POINT('Ctrl Pts',(-71.4876093492781,7.74468834195749,
0.));
#146536=CARTESIAN_POINT('Ctrl Pts',(-71.4661832236888,7.73426219281942,
0.));
#146537=CARTESIAN_POINT('Ctrl Pts',(-71.4447853996916,7.72387574915546,
0.));
#146538=CARTESIAN_POINT('Ctrl Pts',(-71.4234160144925,7.71352900834522,
0.));
#146539=CARTESIAN_POINT('Ctrl Pts',(-71.4020752058796,7.70322196765541,
0.));
#146540=CARTESIAN_POINT('Ctrl Pts',(-71.380763112233,7.69295462424614,0.));
#146541=CARTESIAN_POINT('Ctrl Pts',(-71.3594798725281,7.68272697517089,
0.));
#146542=CARTESIAN_POINT('Ctrl Pts',(-71.3382256263414,7.67253901737555,
0.));
#146543=CARTESIAN_POINT('Ctrl Pts',(-71.3170005138502,7.66239074769165,
0.));
#146544=CARTESIAN_POINT('Ctrl Pts',(-71.2958046758372,7.65228216283406,
0.));
#146545=CARTESIAN_POINT('Ctrl Pts',(-71.2746382537007,7.64221325940727,
0.));
#146546=CARTESIAN_POINT('Ctrl Pts',(-71.2535013894602,7.6321840339054,0.));
#146547=CARTESIAN_POINT('Ctrl Pts',(-71.2323942257609,7.62219448271111,
0.));
#146548=CARTESIAN_POINT('Ctrl Pts',(-71.211316905874,7.6122446020884,0.));
#146549=CARTESIAN_POINT('Ctrl Pts',(-71.1902695737013,7.60233438818099,
0.));
#146550=CARTESIAN_POINT('Ctrl Pts',(-71.1692523737844,7.59246383701816,
0.));
#146551=CARTESIAN_POINT('Ctrl Pts',(-71.1482654513119,7.58263294451454,
0.));
#146552=CARTESIAN_POINT('Ctrl Pts',(-71.1273089521234,7.57284170646889,
0.));
#146553=CARTESIAN_POINT('Ctrl Pts',(-71.106383022711,7.5630901185566,0.));
#146554=CARTESIAN_POINT('Ctrl Pts',(-71.0854878102243,7.55337817632919,
0.));
#146555=CARTESIAN_POINT('Ctrl Pts',(-71.0646234624811,7.54370587521982,
0.));
#146556=CARTESIAN_POINT('Ctrl Pts',(-71.043790127973,7.53407321054265,0.));
#146557=CARTESIAN_POINT('Ctrl Pts',(-71.0229879558699,7.52448017749127,
0.));
#146558=CARTESIAN_POINT('Ctrl Pts',(-71.0022170960211,7.51492677113092,
0.));
#146559=CARTESIAN_POINT('Ctrl Pts',(-70.9814776989612,7.50541298639931,
0.));
#146560=CARTESIAN_POINT('Ctrl Pts',(-70.9607699159218,7.49593881811132,
0.));
#146561=CARTESIAN_POINT('Ctrl Pts',(-70.940093898837,7.48650426095826,0.));
#146562=CARTESIAN_POINT('Ctrl Pts',(-70.9194498003493,7.47710930950564,
0.));
#146563=CARTESIAN_POINT('Ctrl Pts',(-70.8988377738104,7.46775395818529,
0.));
#146564=CARTESIAN_POINT('Ctrl Pts',(-70.87825797329,7.45843820129784,0.));
#146565=CARTESIAN_POINT('Ctrl Pts',(-70.8577105535848,7.4491620330165,0.));
#146566=CARTESIAN_POINT('Ctrl Pts',(-70.8371956702241,7.43992544738608,
0.));
#146567=CARTESIAN_POINT('Ctrl Pts',(-70.8167134794737,7.43072843832017,
0.));
#146568=CARTESIAN_POINT('Ctrl Pts',(-70.7962641383349,7.42157099959328,
0.));
#146569=CARTESIAN_POINT('Ctrl Pts',(-70.7758478045576,7.412453124845,0.));
#146570=CARTESIAN_POINT('Ctrl Pts',(-70.7554646366514,7.4033748075824,0.));
#146571=CARTESIAN_POINT('Ctrl Pts',(-70.735114793895,7.39433604117894,0.));
#146572=CARTESIAN_POINT('Ctrl Pts',(-70.7147984363423,7.3853368188703,0.));
#146573=CARTESIAN_POINT('Ctrl Pts',(-70.6945157248269,7.37637713374763,
0.));
#146574=CARTESIAN_POINT('Ctrl Pts',(-70.6742668209685,7.36745697876297,
0.));
#146575=CARTESIAN_POINT('Ctrl Pts',(-70.6540518871772,7.35857634673054,
0.));
#146576=CARTESIAN_POINT('Ctrl Pts',(-70.6338710866562,7.34973523032583,
0.));
#146577=CARTESIAN_POINT('Ctrl Pts',(-70.6137245834002,7.3409336220802,0.));
#146578=CARTESIAN_POINT('Ctrl Pts',(-70.5936125421958,7.3321715143761,0.));
#146579=CARTESIAN_POINT('Ctrl Pts',(-70.573535128649,7.3234488994524,0.));
#146580=CARTESIAN_POINT('Ctrl Pts',(-70.5534925092052,7.31476576940406,
0.));
#146581=CARTESIAN_POINT('Ctrl Pts',(-70.5334848511675,7.30612211618049,
0.));
#146582=CARTESIAN_POINT('Ctrl Pts',(-70.5135123227147,7.29751793157804,
0.));
#146583=CARTESIAN_POINT('Ctrl Pts',(-70.4935750929029,7.28895320723838,
0.));
#146584=CARTESIAN_POINT('Ctrl Pts',(-70.4736733316463,7.28042793465452,
0.));
#146585=CARTESIAN_POINT('Ctrl Pts',(-70.4538072096986,7.2719421051706,0.));
#146586=CARTESIAN_POINT('Ctrl Pts',(-70.433976898636,7.26349570998052,0.));
#146587=CARTESIAN_POINT('Ctrl Pts',(-70.4141825708207,7.25508874012078,
0.));
#146588=CARTESIAN_POINT('Ctrl Pts',(-70.3944243994532,7.24672118647119,
0.));
#146589=CARTESIAN_POINT('Ctrl Pts',(-70.3747025586569,7.23839303975629,
0.));
#146590=CARTESIAN_POINT('Ctrl Pts',(-70.3550172235486,7.23010429054233,
0.));
#146591=CARTESIAN_POINT('Ctrl Pts',(-70.3353685703097,7.2218549292318,0.));
#146592=CARTESIAN_POINT('Ctrl Pts',(-70.3157567762561,7.21364494605427,
0.));
#146593=CARTESIAN_POINT('Ctrl Pts',(-70.2961820197051,7.2054743310746,0.));
#146594=CARTESIAN_POINT('Ctrl Pts',(-70.276644479827,7.19734307419863,0.));
#146595=CARTESIAN_POINT('Ctrl Pts',(-70.2571443365198,7.18925116517565,
0.));
#146596=CARTESIAN_POINT('Ctrl Pts',(-70.2376817702239,7.18119859359803,
0.));
#146597=CARTESIAN_POINT('Ctrl Pts',(-70.2182569619028,7.1731853488975,0.));
#146598=CARTESIAN_POINT('Ctrl Pts',(-70.1988700934622,7.16521142033895,
0.));
#146599=CARTESIAN_POINT('Ctrl Pts',(-70.1795213481196,7.15727679700949,
0.));
#146600=CARTESIAN_POINT('Ctrl Pts',(-70.1602109107188,7.14938146780804,
0.));
#146601=CARTESIAN_POINT('Ctrl Pts',(-70.1409389682389,7.14152542142342,
0.));
#146602=CARTESIAN_POINT('Ctrl Pts',(-70.1217057094456,7.13370864634401,
0.));
#146603=CARTESIAN_POINT('Ctrl Pts',(-70.1025113239463,7.12593113088873,
0.));
#146604=CARTESIAN_POINT('Ctrl Pts',(-70.0833560013971,7.11819286322826,
0.));
#146605=CARTESIAN_POINT('Ctrl Pts',(-70.06423993069,7.11049383140484,0.));
#146606=CARTESIAN_POINT('Ctrl Pts',(-70.0451632990136,7.10283402335094,
0.));
#146607=CARTESIAN_POINT('Ctrl Pts',(-70.0261262936435,7.09521342684304,
0.));
#146608=CARTESIAN_POINT('Ctrl Pts',(-70.0071291040791,7.08763202944276,
0.));
#146609=CARTESIAN_POINT('Ctrl Pts',(-69.988171923787,7.08008981844645,0.));
#146610=CARTESIAN_POINT('Ctrl Pts',(-69.9692549527256,7.07258678080795,
0.));
#146611=CARTESIAN_POINT('Ctrl Pts',(-69.9503783975676,7.06512290312805,
0.));
#146612=CARTESIAN_POINT('Ctrl Pts',(-69.9315424664252,7.05769817180827,
0.));
#146613=CARTESIAN_POINT('Ctrl Pts',(-69.9127473642086,7.0503125731811,0.));
#146614=CARTESIAN_POINT('Ctrl Pts',(-69.8939932885864,7.04296609362189,
0.));
#146615=CARTESIAN_POINT('Ctrl Pts',(-69.8752804235296,7.03565871972267,
0.));
#146616=CARTESIAN_POINT('Ctrl Pts',(-69.8566089455448,7.02839043811865,
0.));
#146617=CARTESIAN_POINT('Ctrl Pts',(-69.8379790360574,7.02116123514489,
0.));
#146618=CARTESIAN_POINT('Ctrl Pts',(-69.8193908913722,7.01397109655458,
0.));
#146619=CARTESIAN_POINT('Ctrl Pts',(-69.8008447346782,7.00682000718107,
0.));
#146620=CARTESIAN_POINT('Ctrl Pts',(-69.7823408242446,6.99970795069402,
0.));
#146621=CARTESIAN_POINT('Ctrl Pts',(-69.7638794280263,6.99263491027862,
0.));
#146622=CARTESIAN_POINT('Ctrl Pts',(-69.7454607995524,6.98560086924175,
0.));
#146623=CARTESIAN_POINT('Ctrl Pts',(-69.7270851557443,6.97860581164571,
0.));
#146624=CARTESIAN_POINT('Ctrl Pts',(-69.7087526480248,6.97164972291584,
0.));
#146625=CARTESIAN_POINT('Ctrl Pts',(-69.6904633605834,6.96473259049732,
0.));
#146626=CARTESIAN_POINT('Ctrl Pts',(-69.6758665380764,6.95923004173798,
0.));
#146627=CARTESIAN_POINT('Ctrl Pts',(-69.6649383920075,6.95512065317733,
0.));
#146628=CARTESIAN_POINT('Ctrl Pts',(-69.6576616146559,6.95238884849078,
0.));
#146629=CARTESIAN_POINT('Ctrl Pts',(-69.6540253893193,6.9510248930693,0.));
#146630=CARTESIAN_POINT('Ctrl Pts',(-72.8667204369977,15.5142209845169,
0.));
#146631=CARTESIAN_POINT('Ctrl Pts',(-72.8667204369977,15.5142209845169,
12.));
#146632=CARTESIAN_POINT('Ctrl Pts',(-72.8622377860957,15.5108715869174,
0.));
#146633=CARTESIAN_POINT('Ctrl Pts',(-72.8622377860957,15.5108715869174,
12.));
#146634=CARTESIAN_POINT('Ctrl Pts',(-72.8532737732123,15.5041768664089,
0.));
#146635=CARTESIAN_POINT('Ctrl Pts',(-72.8532737732123,15.5041768664089,
12.));
#146636=CARTESIAN_POINT('Ctrl Pts',(-72.8398316206501,15.494147009717,0.));
#146637=CARTESIAN_POINT('Ctrl Pts',(-72.8398316206501,15.494147009717,12.));
#146638=CARTESIAN_POINT('Ctrl Pts',(-72.8219164844002,15.4807983165984,
0.));
#146639=CARTESIAN_POINT('Ctrl Pts',(-72.8219164844002,15.4807983165984,
12.));
#146640=CARTESIAN_POINT('Ctrl Pts',(-72.7995354604414,15.4641532053436,
0.));
#146641=CARTESIAN_POINT('Ctrl Pts',(-72.7995354604414,15.4641532053436,
12.));
#146642=CARTESIAN_POINT('Ctrl Pts',(-72.7771673494582,15.4475488590336,
0.));
#146643=CARTESIAN_POINT('Ctrl Pts',(-72.7771673494582,15.4475488590336,
12.));
#146644=CARTESIAN_POINT('Ctrl Pts',(-72.7548121825431,15.4309852897867,
0.));
#146645=CARTESIAN_POINT('Ctrl Pts',(-72.7548121825431,15.4309852897867,
12.));
#146646=CARTESIAN_POINT('Ctrl Pts',(-72.7324700089576,15.4144625111911,
0.));
#146647=CARTESIAN_POINT('Ctrl Pts',(-72.7324700089576,15.4144625111911,
12.));
#146648=CARTESIAN_POINT('Ctrl Pts',(-72.710140901746,15.397980537311,0.));
#146649=CARTESIAN_POINT('Ctrl Pts',(-72.710140901746,15.397980537311,12.));
#146650=CARTESIAN_POINT('Ctrl Pts',(-72.6878249557452,15.381539382267,0.));
#146651=CARTESIAN_POINT('Ctrl Pts',(-72.6878249557452,15.381539382267,12.));
#146652=CARTESIAN_POINT('Ctrl Pts',(-72.6655222797603,15.3651390602616,
0.));
#146653=CARTESIAN_POINT('Ctrl Pts',(-72.6655222797603,15.3651390602616,
12.));
#146654=CARTESIAN_POINT('Ctrl Pts',(-72.6432329903466,15.3487795854724,
0.));
#146655=CARTESIAN_POINT('Ctrl Pts',(-72.6432329903466,15.3487795854724,
12.));
#146656=CARTESIAN_POINT('Ctrl Pts',(-72.6209572051064,15.3324609719961,
0.));
#146657=CARTESIAN_POINT('Ctrl Pts',(-72.6209572051064,15.3324609719961,
12.));
#146658=CARTESIAN_POINT('Ctrl Pts',(-72.5986950357771,15.3161832337618,
0.));
#146659=CARTESIAN_POINT('Ctrl Pts',(-72.5986950357771,15.3161832337618,
12.));
#146660=CARTESIAN_POINT('Ctrl Pts',(-72.5764465826345,15.2999463844691,
0.));
#146661=CARTESIAN_POINT('Ctrl Pts',(-72.5764465826345,15.2999463844691,
12.));
#146662=CARTESIAN_POINT('Ctrl Pts',(-72.5542119383748,15.2837504376562,
0.));
#146663=CARTESIAN_POINT('Ctrl Pts',(-72.5542119383748,15.2837504376562,
12.));
#146664=CARTESIAN_POINT('Ctrl Pts',(-72.5319911908978,15.2675954067495,
0.));
#146665=CARTESIAN_POINT('Ctrl Pts',(-72.5319911908978,15.2675954067495,
12.));
#146666=CARTESIAN_POINT('Ctrl Pts',(-72.5097844266083,15.2514813051174,
0.));
#146667=CARTESIAN_POINT('Ctrl Pts',(-72.5097844266083,15.2514813051174,
12.));
#146668=CARTESIAN_POINT('Ctrl Pts',(-72.4875917332729,15.2354081461152,
0.));
#146669=CARTESIAN_POINT('Ctrl Pts',(-72.4875917332729,15.2354081461152,
12.));
#146670=CARTESIAN_POINT('Ctrl Pts',(-72.4654132036373,15.2193759431359,
0.));
#146671=CARTESIAN_POINT('Ctrl Pts',(-72.4654132036373,15.2193759431359,
12.));
#146672=CARTESIAN_POINT('Ctrl Pts',(-72.4432489350415,15.2033847096077,
0.));
#146673=CARTESIAN_POINT('Ctrl Pts',(-72.4432489350415,15.2033847096077,
12.));
#146674=CARTESIAN_POINT('Ctrl Pts',(-72.4210990277819,15.1874344589716,
0.));
#146675=CARTESIAN_POINT('Ctrl Pts',(-72.4210990277819,15.1874344589716,
12.));
#146676=CARTESIAN_POINT('Ctrl Pts',(-72.3989635838476,15.1715252046603,
0.));
#146677=CARTESIAN_POINT('Ctrl Pts',(-72.3989635838476,15.1715252046603,
12.));
#146678=CARTESIAN_POINT('Ctrl Pts',(-72.37684270559,15.1556569600747,0.));
#146679=CARTESIAN_POINT('Ctrl Pts',(-72.37684270559,15.1556569600747,12.));
#146680=CARTESIAN_POINT('Ctrl Pts',(-72.3547364941996,15.1398297385513,
0.));
#146681=CARTESIAN_POINT('Ctrl Pts',(-72.3547364941996,15.1398297385513,
12.));
#146682=CARTESIAN_POINT('Ctrl Pts',(-72.332645049021,15.1240435533478,0.));
#146683=CARTESIAN_POINT('Ctrl Pts',(-72.332645049021,15.1240435533478,12.));
#146684=CARTESIAN_POINT('Ctrl Pts',(-72.3105684683971,15.1082984176656,
0.));
#146685=CARTESIAN_POINT('Ctrl Pts',(-72.3105684683971,15.1082984176656,
12.));
#146686=CARTESIAN_POINT('Ctrl Pts',(-72.2885068501641,15.0925943446593,
0.));
#146687=CARTESIAN_POINT('Ctrl Pts',(-72.2885068501641,15.0925943446593,
12.));
#146688=CARTESIAN_POINT('Ctrl Pts',(-72.266460292285,15.0769313474476,0.));
#146689=CARTESIAN_POINT('Ctrl Pts',(-72.266460292285,15.0769313474476,12.));
#146690=CARTESIAN_POINT('Ctrl Pts',(-72.244428893425,15.0613094391186,0.));
#146691=CARTESIAN_POINT('Ctrl Pts',(-72.244428893425,15.0613094391186,12.));
#146692=CARTESIAN_POINT('Ctrl Pts',(-72.2224127535401,15.0457286327328,
0.));
#146693=CARTESIAN_POINT('Ctrl Pts',(-72.2224127535401,15.0457286327328,
12.));
#146694=CARTESIAN_POINT('Ctrl Pts',(-72.2004119736104,15.0301889413255,
0.));
#146695=CARTESIAN_POINT('Ctrl Pts',(-72.2004119736104,15.0301889413255,
12.));
#146696=CARTESIAN_POINT('Ctrl Pts',(-72.1784266553948,15.0146903779061,
0.));
#146697=CARTESIAN_POINT('Ctrl Pts',(-72.1784266553948,15.0146903779061,
12.));
#146698=CARTESIAN_POINT('Ctrl Pts',(-72.1564569011668,14.9992329554537,
0.));
#146699=CARTESIAN_POINT('Ctrl Pts',(-72.1564569011668,14.9992329554537,
12.));
#146700=CARTESIAN_POINT('Ctrl Pts',(-72.1345028134779,14.9838166869107,
0.));
#146701=CARTESIAN_POINT('Ctrl Pts',(-72.1345028134779,14.9838166869107,
12.));
#146702=CARTESIAN_POINT('Ctrl Pts',(-72.1125644948547,14.96844158517,0.));
#146703=CARTESIAN_POINT('Ctrl Pts',(-72.1125644948547,14.96844158517,12.));
#146704=CARTESIAN_POINT('Ctrl Pts',(-72.0906420478085,14.953107663077,0.));
#146705=CARTESIAN_POINT('Ctrl Pts',(-72.0906420478085,14.953107663077,12.));
#146706=CARTESIAN_POINT('Ctrl Pts',(-72.0687355749815,14.937814933439,0.));
#146707=CARTESIAN_POINT('Ctrl Pts',(-72.0687355749815,14.937814933439,12.));
#146708=CARTESIAN_POINT('Ctrl Pts',(-72.046845179251,14.9225634090269,0.));
#146709=CARTESIAN_POINT('Ctrl Pts',(-72.046845179251,14.9225634090269,12.));
#146710=CARTESIAN_POINT('Ctrl Pts',(-72.0249709638419,14.9073531025764,
0.));
#146711=CARTESIAN_POINT('Ctrl Pts',(-72.0249709638419,14.9073531025764,
12.));
#146712=CARTESIAN_POINT('Ctrl Pts',(-72.0031130324519,14.892184026783,0.));
#146713=CARTESIAN_POINT('Ctrl Pts',(-72.0031130324519,14.892184026783,12.));
#146714=CARTESIAN_POINT('Ctrl Pts',(-71.9812714893087,14.8770561943011,
0.));
#146715=CARTESIAN_POINT('Ctrl Pts',(-71.9812714893087,14.8770561943011,
12.));
#146716=CARTESIAN_POINT('Ctrl Pts',(-71.9594464391063,14.8619696177503,
0.));
#146717=CARTESIAN_POINT('Ctrl Pts',(-71.9594464391063,14.8619696177503,
12.));
#146718=CARTESIAN_POINT('Ctrl Pts',(-71.9376379869668,14.846924309716,0.));
#146719=CARTESIAN_POINT('Ctrl Pts',(-71.9376379869668,14.846924309716,12.));
#146720=CARTESIAN_POINT('Ctrl Pts',(-71.9158462383915,14.8319202827483,
0.));
#146721=CARTESIAN_POINT('Ctrl Pts',(-71.9158462383915,14.8319202827483,
12.));
#146722=CARTESIAN_POINT('Ctrl Pts',(-71.8940712992119,14.816957549356,0.));
#146723=CARTESIAN_POINT('Ctrl Pts',(-71.8940712992119,14.816957549356,12.));
#146724=CARTESIAN_POINT('Ctrl Pts',(-71.872313275546,14.8020361220003,0.));
#146725=CARTESIAN_POINT('Ctrl Pts',(-71.872313275546,14.8020361220003,12.));
#146726=CARTESIAN_POINT('Ctrl Pts',(-71.8505722738286,14.7871560131021,
0.));
#146727=CARTESIAN_POINT('Ctrl Pts',(-71.8505722738286,14.7871560131021,
12.));
#146728=CARTESIAN_POINT('Ctrl Pts',(-71.8288484008343,14.7723172350455,
0.));
#146729=CARTESIAN_POINT('Ctrl Pts',(-71.8288484008343,14.7723172350455,
12.));
#146730=CARTESIAN_POINT('Ctrl Pts',(-71.8071417637018,14.7575198001777,
0.));
#146731=CARTESIAN_POINT('Ctrl Pts',(-71.8071417637018,14.7575198001777,
12.));
#146732=CARTESIAN_POINT('Ctrl Pts',(-71.7854524699562,14.7427637208071,
0.));
#146733=CARTESIAN_POINT('Ctrl Pts',(-71.7854524699562,14.7427637208071,
12.));
#146734=CARTESIAN_POINT('Ctrl Pts',(-71.7637806275316,14.7280490091954,
0.));
#146735=CARTESIAN_POINT('Ctrl Pts',(-71.7637806275316,14.7280490091954,
12.));
#146736=CARTESIAN_POINT('Ctrl Pts',(-71.7421263447707,14.7133756775622,
0.));
#146737=CARTESIAN_POINT('Ctrl Pts',(-71.7421263447707,14.7133756775622,
12.));
#146738=CARTESIAN_POINT('Ctrl Pts',(-71.7204897304186,14.6987437380898,
0.));
#146739=CARTESIAN_POINT('Ctrl Pts',(-71.7204897304186,14.6987437380898,
12.));
#146740=CARTESIAN_POINT('Ctrl Pts',(-71.698870893617,14.6841532029232,0.));
#146741=CARTESIAN_POINT('Ctrl Pts',(-71.698870893617,14.6841532029232,12.));
#146742=CARTESIAN_POINT('Ctrl Pts',(-71.6772699438966,14.669604084168,0.));
#146743=CARTESIAN_POINT('Ctrl Pts',(-71.6772699438966,14.669604084168,12.));
#146744=CARTESIAN_POINT('Ctrl Pts',(-71.6556869911669,14.6550963938832,
0.));
#146745=CARTESIAN_POINT('Ctrl Pts',(-71.6556869911669,14.6550963938832,
12.));
#146746=CARTESIAN_POINT('Ctrl Pts',(-71.6341221457175,14.6406301440817,
0.));
#146747=CARTESIAN_POINT('Ctrl Pts',(-71.6341221457175,14.6406301440817,
12.));
#146748=CARTESIAN_POINT('Ctrl Pts',(-71.6125755182295,14.6262053467372,
0.));
#146749=CARTESIAN_POINT('Ctrl Pts',(-71.6125755182295,14.6262053467372,
12.));
#146750=CARTESIAN_POINT('Ctrl Pts',(-71.5910472197814,14.611822013785,0.));
#146751=CARTESIAN_POINT('Ctrl Pts',(-71.5910472197814,14.611822013785,12.));
#146752=CARTESIAN_POINT('Ctrl Pts',(-71.569537361856,14.597480157121,0.));
#146753=CARTESIAN_POINT('Ctrl Pts',(-71.569537361856,14.597480157121,12.));
#146754=CARTESIAN_POINT('Ctrl Pts',(-71.5480460563445,14.5831797885951,
0.));
#146755=CARTESIAN_POINT('Ctrl Pts',(-71.5480460563445,14.5831797885951,
12.));
#146756=CARTESIAN_POINT('Ctrl Pts',(-71.52657341555,14.5689209200091,0.));
#146757=CARTESIAN_POINT('Ctrl Pts',(-71.52657341555,14.5689209200091,12.));
#146758=CARTESIAN_POINT('Ctrl Pts',(-71.5051195521914,14.5547035631234,
0.));
#146759=CARTESIAN_POINT('Ctrl Pts',(-71.5051195521914,14.5547035631234,
12.));
#146760=CARTESIAN_POINT('Ctrl Pts',(-71.4836845794052,14.540527729659,0.));
#146761=CARTESIAN_POINT('Ctrl Pts',(-71.4836845794052,14.540527729659,12.));
#146762=CARTESIAN_POINT('Ctrl Pts',(-71.4622686107475,14.5263934312969,
0.));
#146763=CARTESIAN_POINT('Ctrl Pts',(-71.4622686107475,14.5263934312969,
12.));
#146764=CARTESIAN_POINT('Ctrl Pts',(-71.4408717601917,14.5123006796728,
0.));
#146765=CARTESIAN_POINT('Ctrl Pts',(-71.4408717601917,14.5123006796728,
12.));
#146766=CARTESIAN_POINT('Ctrl Pts',(-71.4194941421279,14.4982494863716,
0.));
#146767=CARTESIAN_POINT('Ctrl Pts',(-71.4194941421279,14.4982494863716,
12.));
#146768=CARTESIAN_POINT('Ctrl Pts',(-71.398135871371,14.4842398629354,0.));
#146769=CARTESIAN_POINT('Ctrl Pts',(-71.398135871371,14.4842398629354,12.));
#146770=CARTESIAN_POINT('Ctrl Pts',(-71.3767970631642,14.470271820865,0.));
#146771=CARTESIAN_POINT('Ctrl Pts',(-71.3767970631642,14.470271820865,12.));
#146772=CARTESIAN_POINT('Ctrl Pts',(-71.3554778331835,14.4563453716204,
0.));
#146773=CARTESIAN_POINT('Ctrl Pts',(-71.3554778331835,14.4563453716204,
12.));
#146774=CARTESIAN_POINT('Ctrl Pts',(-71.3341782975393,14.4424605266167,
0.));
#146775=CARTESIAN_POINT('Ctrl Pts',(-71.3341782975393,14.4424605266167,
12.));
#146776=CARTESIAN_POINT('Ctrl Pts',(-71.3128985727777,14.4286172972168,
0.));
#146777=CARTESIAN_POINT('Ctrl Pts',(-71.3128985727777,14.4286172972168,
12.));
#146778=CARTESIAN_POINT('Ctrl Pts',(-71.2916387758864,14.4148156947384,
0.));
#146779=CARTESIAN_POINT('Ctrl Pts',(-71.2916387758864,14.4148156947384,
12.));
#146780=CARTESIAN_POINT('Ctrl Pts',(-71.2703990242986,14.401055730457,0.));
#146781=CARTESIAN_POINT('Ctrl Pts',(-71.2703990242986,14.401055730457,12.));
#146782=CARTESIAN_POINT('Ctrl Pts',(-71.2491794358956,14.3873374156056,
0.));
#146783=CARTESIAN_POINT('Ctrl Pts',(-71.2491794358956,14.3873374156056,
12.));
#146784=CARTESIAN_POINT('Ctrl Pts',(-71.2279801290088,14.3736607613723,
0.));
#146785=CARTESIAN_POINT('Ctrl Pts',(-71.2279801290088,14.3736607613723,
12.));
#146786=CARTESIAN_POINT('Ctrl Pts',(-71.2068012224187,14.3600257788927,
0.));
#146787=CARTESIAN_POINT('Ctrl Pts',(-71.2068012224187,14.3600257788927,
12.));
#146788=CARTESIAN_POINT('Ctrl Pts',(-71.185642835361,14.3464324792537,0.));
#146789=CARTESIAN_POINT('Ctrl Pts',(-71.185642835361,14.3464324792537,12.));
#146790=CARTESIAN_POINT('Ctrl Pts',(-71.1645050875323,14.3328808734993,
0.));
#146791=CARTESIAN_POINT('Ctrl Pts',(-71.1645050875323,14.3328808734993,
12.));
#146792=CARTESIAN_POINT('Ctrl Pts',(-71.1433880990932,14.3193709726295,
0.));
#146793=CARTESIAN_POINT('Ctrl Pts',(-71.1433880990932,14.3193709726295,
12.));
#146794=CARTESIAN_POINT('Ctrl Pts',(-71.1222919906718,14.3059027875993,
0.));
#146795=CARTESIAN_POINT('Ctrl Pts',(-71.1222919906718,14.3059027875993,
12.));
#146796=CARTESIAN_POINT('Ctrl Pts',(-71.1012168833626,14.2924763293101,
0.));
#146797=CARTESIAN_POINT('Ctrl Pts',(-71.1012168833626,14.2924763293101,
12.));
#146798=CARTESIAN_POINT('Ctrl Pts',(-71.0801628987314,14.279091608613,0.));
#146799=CARTESIAN_POINT('Ctrl Pts',(-71.0801628987314,14.279091608613,12.));
#146800=CARTESIAN_POINT('Ctrl Pts',(-71.059130158822,14.2657486363137,0.));
#146801=CARTESIAN_POINT('Ctrl Pts',(-71.059130158822,14.2657486363137,12.));
#146802=CARTESIAN_POINT('Ctrl Pts',(-71.0381187861585,14.2524474231732,
0.));
#146803=CARTESIAN_POINT('Ctrl Pts',(-71.0381187861585,14.2524474231732,
12.));
#146804=CARTESIAN_POINT('Ctrl Pts',(-71.0171289037493,14.2391879799063,
0.));
#146805=CARTESIAN_POINT('Ctrl Pts',(-71.0171289037493,14.2391879799063,
12.));
#146806=CARTESIAN_POINT('Ctrl Pts',(-70.996160635087,14.2259703171739,0.));
#146807=CARTESIAN_POINT('Ctrl Pts',(-70.996160635087,14.2259703171739,12.));
#146808=CARTESIAN_POINT('Ctrl Pts',(-70.9752141041527,14.2127944455841,
0.));
#146809=CARTESIAN_POINT('Ctrl Pts',(-70.9752141041527,14.2127944455841,
12.));
#146810=CARTESIAN_POINT('Ctrl Pts',(-70.9542894354221,14.1996603756984,
0.));
#146811=CARTESIAN_POINT('Ctrl Pts',(-70.9542894354221,14.1996603756984,
12.));
#146812=CARTESIAN_POINT('Ctrl Pts',(-70.9333867538704,14.1865681180321,
0.));
#146813=CARTESIAN_POINT('Ctrl Pts',(-70.9333867538704,14.1865681180321,
12.));
#146814=CARTESIAN_POINT('Ctrl Pts',(-70.9125061849744,14.1735176830533,
0.));
#146815=CARTESIAN_POINT('Ctrl Pts',(-70.9125061849744,14.1735176830533,
12.));
#146816=CARTESIAN_POINT('Ctrl Pts',(-70.8916478547131,14.1605090811754,
0.));
#146817=CARTESIAN_POINT('Ctrl Pts',(-70.8916478547131,14.1605090811754,
12.));
#146818=CARTESIAN_POINT('Ctrl Pts',(-70.8708118895717,14.1475423227568,
0.));
#146819=CARTESIAN_POINT('Ctrl Pts',(-70.8708118895717,14.1475423227568,
12.));
#146820=CARTESIAN_POINT('Ctrl Pts',(-70.8499984165493,14.1346174181079,
0.));
#146821=CARTESIAN_POINT('Ctrl Pts',(-70.8499984165493,14.1346174181079,
12.));
#146822=CARTESIAN_POINT('Ctrl Pts',(-70.8292075631624,14.1217343774914,
0.));
#146823=CARTESIAN_POINT('Ctrl Pts',(-70.8292075631624,14.1217343774914,
12.));
#146824=CARTESIAN_POINT('Ctrl Pts',(-70.8084394574491,14.1088932111215,
0.));
#146825=CARTESIAN_POINT('Ctrl Pts',(-70.8084394574491,14.1088932111215,
12.));
#146826=CARTESIAN_POINT('Ctrl Pts',(-70.787694227969,14.0960939291569,0.));
#146827=CARTESIAN_POINT('Ctrl Pts',(-70.787694227969,14.0960939291569,12.));
#146828=CARTESIAN_POINT('Ctrl Pts',(-70.7669720038067,14.0833365416995,
0.));
#146829=CARTESIAN_POINT('Ctrl Pts',(-70.7669720038067,14.0833365416995,
12.));
#146830=CARTESIAN_POINT('Ctrl Pts',(-70.7462729145799,14.0706210588015,
0.));
#146831=CARTESIAN_POINT('Ctrl Pts',(-70.7462729145799,14.0706210588015,
12.));
#146832=CARTESIAN_POINT('Ctrl Pts',(-70.7255970904433,14.0579474904657,
0.));
#146833=CARTESIAN_POINT('Ctrl Pts',(-70.7255970904433,14.0579474904657,
12.));
#146834=CARTESIAN_POINT('Ctrl Pts',(-70.7049446620931,14.0453158466451,
0.));
#146835=CARTESIAN_POINT('Ctrl Pts',(-70.7049446620931,14.0453158466451,
12.));
#146836=CARTESIAN_POINT('Ctrl Pts',(-70.6843157607672,14.0327261372363,
0.));
#146837=CARTESIAN_POINT('Ctrl Pts',(-70.6843157607672,14.0327261372363,
12.));
#146838=CARTESIAN_POINT('Ctrl Pts',(-70.6637105182487,14.020178372077,0.));
#146839=CARTESIAN_POINT('Ctrl Pts',(-70.6637105182487,14.020178372077,12.));
#146840=CARTESIAN_POINT('Ctrl Pts',(-70.6431290668744,14.0076725609537,
0.));
#146841=CARTESIAN_POINT('Ctrl Pts',(-70.6431290668744,14.0076725609537,
12.));
#146842=CARTESIAN_POINT('Ctrl Pts',(-70.6225715395392,13.9952087136018,
0.));
#146843=CARTESIAN_POINT('Ctrl Pts',(-70.6225715395392,13.9952087136018,
12.));
#146844=CARTESIAN_POINT('Ctrl Pts',(-70.6020380697004,13.9827868397057,
0.));
#146845=CARTESIAN_POINT('Ctrl Pts',(-70.6020380697004,13.9827868397057,
12.));
#146846=CARTESIAN_POINT('Ctrl Pts',(-70.5815287913791,13.9704069488918,
0.));
#146847=CARTESIAN_POINT('Ctrl Pts',(-70.5815287913791,13.9704069488918,
12.));
#146848=CARTESIAN_POINT('Ctrl Pts',(-70.5610438391622,13.9580690507262,
0.));
#146849=CARTESIAN_POINT('Ctrl Pts',(-70.5610438391622,13.9580690507262,
12.));
#146850=CARTESIAN_POINT('Ctrl Pts',(-70.5405833482123,13.9457731547218,
0.));
#146851=CARTESIAN_POINT('Ctrl Pts',(-70.5405833482123,13.9457731547218,
12.));
#146852=CARTESIAN_POINT('Ctrl Pts',(-70.5201474542717,13.933519270339,0.));
#146853=CARTESIAN_POINT('Ctrl Pts',(-70.5201474542717,13.933519270339,12.));
#146854=CARTESIAN_POINT('Ctrl Pts',(-70.4997362936671,13.9213074069852,
0.));
#146855=CARTESIAN_POINT('Ctrl Pts',(-70.4997362936671,13.9213074069852,
12.));
#146856=CARTESIAN_POINT('Ctrl Pts',(-70.4793500033106,13.9091375740085,
0.));
#146857=CARTESIAN_POINT('Ctrl Pts',(-70.4793500033106,13.9091375740085,
12.));
#146858=CARTESIAN_POINT('Ctrl Pts',(-70.4589887207043,13.8970097806948,
0.));
#146859=CARTESIAN_POINT('Ctrl Pts',(-70.4589887207043,13.8970097806948,
12.));
#146860=CARTESIAN_POINT('Ctrl Pts',(-70.4386525839492,13.8849240362757,
0.));
#146861=CARTESIAN_POINT('Ctrl Pts',(-70.4386525839492,13.8849240362757,
12.));
#146862=CARTESIAN_POINT('Ctrl Pts',(-70.4183417317486,13.8728803499284,
0.));
#146863=CARTESIAN_POINT('Ctrl Pts',(-70.4183417317486,13.8728803499284,
12.));
#146864=CARTESIAN_POINT('Ctrl Pts',(-70.3980563034142,13.8608787307754,
0.));
#146865=CARTESIAN_POINT('Ctrl Pts',(-70.3980563034142,13.8608787307754,
12.));
#146866=CARTESIAN_POINT('Ctrl Pts',(-70.377796438866,13.8489191878774,0.));
#146867=CARTESIAN_POINT('Ctrl Pts',(-70.377796438866,13.8489191878774,12.));
#146868=CARTESIAN_POINT('Ctrl Pts',(-70.3575622786373,13.8370017302319,
0.));
#146869=CARTESIAN_POINT('Ctrl Pts',(-70.3575622786373,13.8370017302319,
12.));
#146870=CARTESIAN_POINT('Ctrl Pts',(-70.3373539638841,13.8251263667799,
0.));
#146871=CARTESIAN_POINT('Ctrl Pts',(-70.3373539638841,13.8251263667799,
12.));
#146872=CARTESIAN_POINT('Ctrl Pts',(-70.3171716363912,13.8132931064067,
0.));
#146873=CARTESIAN_POINT('Ctrl Pts',(-70.3171716363912,13.8132931064067,
12.));
#146874=CARTESIAN_POINT('Ctrl Pts',(-70.2970154385763,13.8015019579411,
0.));
#146875=CARTESIAN_POINT('Ctrl Pts',(-70.2970154385763,13.8015019579411,
12.));
#146876=CARTESIAN_POINT('Ctrl Pts',(-70.2768855134909,13.7897529301483,
0.));
#146877=CARTESIAN_POINT('Ctrl Pts',(-70.2768855134909,13.7897529301483,
12.));
#146878=CARTESIAN_POINT('Ctrl Pts',(-70.2567820048253,13.7780460317284,
0.));
#146879=CARTESIAN_POINT('Ctrl Pts',(-70.2567820048253,13.7780460317284,
12.));
#146880=CARTESIAN_POINT('Ctrl Pts',(-70.2367050569174,13.7663812713235,
0.));
#146881=CARTESIAN_POINT('Ctrl Pts',(-70.2367050569174,13.7663812713235,
12.));
#146882=CARTESIAN_POINT('Ctrl Pts',(-70.216654814759,13.7547586575178,0.));
#146883=CARTESIAN_POINT('Ctrl Pts',(-70.216654814759,13.7547586575178,12.));
#146884=CARTESIAN_POINT('Ctrl Pts',(-70.1966314240012,13.7431781988368,
0.));
#146885=CARTESIAN_POINT('Ctrl Pts',(-70.1966314240012,13.7431781988368,
12.));
#146886=CARTESIAN_POINT('Ctrl Pts',(-70.1766350309554,13.73163990374,0.));
#146887=CARTESIAN_POINT('Ctrl Pts',(-70.1766350309554,13.73163990374,12.));
#146888=CARTESIAN_POINT('Ctrl Pts',(-70.1566657825989,13.7201437806207,
0.));
#146889=CARTESIAN_POINT('Ctrl Pts',(-70.1566657825989,13.7201437806207,
12.));
#146890=CARTESIAN_POINT('Ctrl Pts',(-70.1367238265853,13.7086898378127,
0.));
#146891=CARTESIAN_POINT('Ctrl Pts',(-70.1367238265853,13.7086898378127,
12.));
#146892=CARTESIAN_POINT('Ctrl Pts',(-70.1168093112493,13.6972780835899,
0.));
#146893=CARTESIAN_POINT('Ctrl Pts',(-70.1168093112493,13.6972780835899,
12.));
#146894=CARTESIAN_POINT('Ctrl Pts',(-70.0969223856123,13.6859085261651,
0.));
#146895=CARTESIAN_POINT('Ctrl Pts',(-70.0969223856123,13.6859085261651,
12.));
#146896=CARTESIAN_POINT('Ctrl Pts',(-70.0770631993831,13.6745811736825,
0.));
#146897=CARTESIAN_POINT('Ctrl Pts',(-70.0770631993831,13.6745811736825,
12.));
#146898=CARTESIAN_POINT('Ctrl Pts',(-70.057231902965,13.6632960342192,0.));
#146899=CARTESIAN_POINT('Ctrl Pts',(-70.057231902965,13.6632960342192,12.));
#146900=CARTESIAN_POINT('Ctrl Pts',(-70.037428647466,13.6520531157904,0.));
#146901=CARTESIAN_POINT('Ctrl Pts',(-70.037428647466,13.6520531157904,12.));
#146902=CARTESIAN_POINT('Ctrl Pts',(-70.0176535847047,13.6408524263496,
0.));
#146903=CARTESIAN_POINT('Ctrl Pts',(-70.0176535847047,13.6408524263496,
12.));
#146904=CARTESIAN_POINT('Ctrl Pts',(-69.9979068672163,13.6296939737866,
0.));
#146905=CARTESIAN_POINT('Ctrl Pts',(-69.9979068672163,13.6296939737866,
12.));
#146906=CARTESIAN_POINT('Ctrl Pts',(-69.9781886482543,13.61857776592,0.));
#146907=CARTESIAN_POINT('Ctrl Pts',(-69.9781886482543,13.61857776592,12.));
#146908=CARTESIAN_POINT('Ctrl Pts',(-69.9584990817989,13.6075038105001,
0.));
#146909=CARTESIAN_POINT('Ctrl Pts',(-69.9584990817989,13.6075038105001,
12.));
#146910=CARTESIAN_POINT('Ctrl Pts',(-69.9388383225655,13.5964721152136,
0.));
#146911=CARTESIAN_POINT('Ctrl Pts',(-69.9388383225655,13.5964721152136,
12.));
#146912=CARTESIAN_POINT('Ctrl Pts',(-69.9192065260107,13.5854826876834,
0.));
#146913=CARTESIAN_POINT('Ctrl Pts',(-69.9192065260107,13.5854826876834,
12.));
#146914=CARTESIAN_POINT('Ctrl Pts',(-69.899603848336,13.5745355354657,0.));
#146915=CARTESIAN_POINT('Ctrl Pts',(-69.899603848336,13.5745355354657,12.));
#146916=CARTESIAN_POINT('Ctrl Pts',(-69.880030446488,13.5636306660423,0.));
#146917=CARTESIAN_POINT('Ctrl Pts',(-69.880030446488,13.5636306660423,12.));
#146918=CARTESIAN_POINT('Ctrl Pts',(-69.8604864781705,13.5527680868256,
0.));
#146919=CARTESIAN_POINT('Ctrl Pts',(-69.8604864781705,13.5527680868256,
12.));
#146920=CARTESIAN_POINT('Ctrl Pts',(-69.840972101856,13.5419478051626,0.));
#146921=CARTESIAN_POINT('Ctrl Pts',(-69.840972101856,13.5419478051626,12.));
#146922=CARTESIAN_POINT('Ctrl Pts',(-69.8214874767944,13.5311698283339,
0.));
#146923=CARTESIAN_POINT('Ctrl Pts',(-69.8214874767944,13.5311698283339,
12.));
#146924=CARTESIAN_POINT('Ctrl Pts',(-69.8020327630204,13.5204341635507,
0.));
#146925=CARTESIAN_POINT('Ctrl Pts',(-69.8020327630204,13.5204341635507,
12.));
#146926=CARTESIAN_POINT('Ctrl Pts',(-69.7826081213575,13.5097408179479,
0.));
#146927=CARTESIAN_POINT('Ctrl Pts',(-69.7826081213575,13.5097408179479,
12.));
#146928=CARTESIAN_POINT('Ctrl Pts',(-69.7632137134247,13.4990897985904,
0.));
#146929=CARTESIAN_POINT('Ctrl Pts',(-69.7632137134247,13.4990897985904,
12.));
#146930=CARTESIAN_POINT('Ctrl Pts',(-69.7438497016404,13.4884811124748,
0.));
#146931=CARTESIAN_POINT('Ctrl Pts',(-69.7438497016404,13.4884811124748,
12.));
#146932=CARTESIAN_POINT('Ctrl Pts',(-69.7245162492251,13.4779147665286,
0.));
#146933=CARTESIAN_POINT('Ctrl Pts',(-69.7245162492251,13.4779147665286,
12.));
#146934=CARTESIAN_POINT('Ctrl Pts',(-69.7052135202003,13.4673907676045,
0.));
#146935=CARTESIAN_POINT('Ctrl Pts',(-69.7052135202003,13.4673907676045,
12.));
#146936=CARTESIAN_POINT('Ctrl Pts',(-69.6859416793898,13.4569091224763,
0.));
#146937=CARTESIAN_POINT('Ctrl Pts',(-69.6859416793898,13.4569091224763,
12.));
#146938=CARTESIAN_POINT('Ctrl Pts',(-69.6667008924454,13.4464698378456,
0.));
#146939=CARTESIAN_POINT('Ctrl Pts',(-69.6667008924454,13.4464698378456,
12.));
#146940=CARTESIAN_POINT('Ctrl Pts',(-69.6474913258684,13.4360729203444,
0.));
#146941=CARTESIAN_POINT('Ctrl Pts',(-69.6474913258684,13.4360729203444,
12.));
#146942=CARTESIAN_POINT('Ctrl Pts',(-69.6283131470267,13.425718376534,0.));
#146943=CARTESIAN_POINT('Ctrl Pts',(-69.6283131470267,13.425718376534,12.));
#146944=CARTESIAN_POINT('Ctrl Pts',(-69.6091665241743,13.4154062128998,
0.));
#146945=CARTESIAN_POINT('Ctrl Pts',(-69.6091665241743,13.4154062128998,
12.));
#146946=CARTESIAN_POINT('Ctrl Pts',(-69.5900516264524,13.4051364358495,
0.));
#146947=CARTESIAN_POINT('Ctrl Pts',(-69.5900516264524,13.4051364358495,
12.));
#146948=CARTESIAN_POINT('Ctrl Pts',(-69.5709686238701,13.3949090517173,
0.));
#146949=CARTESIAN_POINT('Ctrl Pts',(-69.5709686238701,13.3949090517173,
12.));
#146950=CARTESIAN_POINT('Ctrl Pts',(-69.5519176872857,13.3847240667627,
0.));
#146951=CARTESIAN_POINT('Ctrl Pts',(-69.5519176872857,13.3847240667627,
12.));
#146952=CARTESIAN_POINT('Ctrl Pts',(-69.5328989883899,13.3745814871668,
0.));
#146953=CARTESIAN_POINT('Ctrl Pts',(-69.5328989883899,13.3745814871668,
12.));
#146954=CARTESIAN_POINT('Ctrl Pts',(-69.5139126996703,13.3644813190225,
0.));
#146955=CARTESIAN_POINT('Ctrl Pts',(-69.5139126996703,13.3644813190225,
12.));
#146956=CARTESIAN_POINT('Ctrl Pts',(-69.4949589944633,13.3544235683399,
0.));
#146957=CARTESIAN_POINT('Ctrl Pts',(-69.4949589944633,13.3544235683399,
12.));
#146958=CARTESIAN_POINT('Ctrl Pts',(-69.4760380470382,13.3444082410547,
0.));
#146959=CARTESIAN_POINT('Ctrl Pts',(-69.4760380470382,13.3444082410547,
12.));
#146960=CARTESIAN_POINT('Ctrl Pts',(-69.4571500326673,13.3344353430313,
0.));
#146961=CARTESIAN_POINT('Ctrl Pts',(-69.4571500326673,13.3344353430313,
12.));
#146962=CARTESIAN_POINT('Ctrl Pts',(-69.4382951276983,13.3245048800641,
0.));
#146963=CARTESIAN_POINT('Ctrl Pts',(-69.4382951276983,13.3245048800641,
12.));
#146964=CARTESIAN_POINT('Ctrl Pts',(-69.4194735096238,13.3146168578739,
0.));
#146965=CARTESIAN_POINT('Ctrl Pts',(-69.4194735096238,13.3146168578739,
12.));
#146966=CARTESIAN_POINT('Ctrl Pts',(-69.4006853569485,13.3047712821046,
0.));
#146967=CARTESIAN_POINT('Ctrl Pts',(-69.4006853569485,13.3047712821046,
12.));
#146968=CARTESIAN_POINT('Ctrl Pts',(-69.3819308490407,13.2949681583165,
0.));
#146969=CARTESIAN_POINT('Ctrl Pts',(-69.3819308490407,13.2949681583165,
12.));
#146970=CARTESIAN_POINT('Ctrl Pts',(-69.3632101660071,13.2852074919767,
0.));
#146971=CARTESIAN_POINT('Ctrl Pts',(-69.3632101660071,13.2852074919767,
12.));
#146972=CARTESIAN_POINT('Ctrl Pts',(-69.3445234885088,13.2754892884438,
0.));
#146973=CARTESIAN_POINT('Ctrl Pts',(-69.3445234885088,13.2754892884438,
12.));
#146974=CARTESIAN_POINT('Ctrl Pts',(-69.3258709977416,13.2658135529616,
0.));
#146975=CARTESIAN_POINT('Ctrl Pts',(-69.3258709977416,13.2658135529616,
12.));
#146976=CARTESIAN_POINT('Ctrl Pts',(-69.3072528758546,13.2561802906901,
0.));
#146977=CARTESIAN_POINT('Ctrl Pts',(-69.3072528758546,13.2561802906901,
12.));
#146978=CARTESIAN_POINT('Ctrl Pts',(-69.2886693063193,13.2465895067264,
0.));
#146979=CARTESIAN_POINT('Ctrl Pts',(-69.2886693063193,13.2465895067264,
12.));
#146980=CARTESIAN_POINT('Ctrl Pts',(-69.2701204742435,13.2370412061218,
0.));
#146981=CARTESIAN_POINT('Ctrl Pts',(-69.2701204742435,13.2370412061218,
12.));
#146982=CARTESIAN_POINT('Ctrl Pts',(-69.2516065668809,13.2275353939044,
0.));
#146983=CARTESIAN_POINT('Ctrl Pts',(-69.2516065668809,13.2275353939044,
12.));
#146984=CARTESIAN_POINT('Ctrl Pts',(-69.2331277732819,13.2180720750586,
0.));
#146985=CARTESIAN_POINT('Ctrl Pts',(-69.2331277732819,13.2180720750586,
12.));
#146986=CARTESIAN_POINT('Ctrl Pts',(-69.2146842833506,13.2086512544729,
0.));
#146987=CARTESIAN_POINT('Ctrl Pts',(-69.2146842833506,13.2086512544729,
12.));
#146988=CARTESIAN_POINT('Ctrl Pts',(-69.1962762870524,13.1992729368928,
0.));
#146989=CARTESIAN_POINT('Ctrl Pts',(-69.1962762870524,13.1992729368928,
12.));
#146990=CARTESIAN_POINT('Ctrl Pts',(-69.1779039736026,13.189937126869,0.));
#146991=CARTESIAN_POINT('Ctrl Pts',(-69.1779039736026,13.189937126869,12.));
#146992=CARTESIAN_POINT('Ctrl Pts',(-69.1595675305294,13.1806438286944,
0.));
#146993=CARTESIAN_POINT('Ctrl Pts',(-69.1595675305294,13.1806438286944,
12.));
#146994=CARTESIAN_POINT('Ctrl Pts',(-69.141267145461,13.1713930465142,0.));
#146995=CARTESIAN_POINT('Ctrl Pts',(-69.141267145461,13.1713930465142,12.));
#146996=CARTESIAN_POINT('Ctrl Pts',(-69.1230030082598,13.1621847844533,
0.));
#146997=CARTESIAN_POINT('Ctrl Pts',(-69.1230030082598,13.1621847844533,
12.));
#146998=CARTESIAN_POINT('Ctrl Pts',(-69.1047753127633,13.1530190467181,
0.));
#146999=CARTESIAN_POINT('Ctrl Pts',(-69.1047753127633,13.1530190467181,
12.));
#147000=CARTESIAN_POINT('Ctrl Pts',(-69.0865842593063,13.1438958377397,
0.));
#147001=CARTESIAN_POINT('Ctrl Pts',(-69.0865842593063,13.1438958377397,
12.));
#147002=CARTESIAN_POINT('Ctrl Pts',(-69.0684300549426,13.1348151621825,
0.));
#147003=CARTESIAN_POINT('Ctrl Pts',(-69.0684300549426,13.1348151621825,
12.));
#147004=CARTESIAN_POINT('Ctrl Pts',(-69.0503129081778,13.1257770246379,
0.));
#147005=CARTESIAN_POINT('Ctrl Pts',(-69.0503129081778,13.1257770246379,
12.));
#147006=CARTESIAN_POINT('Ctrl Pts',(-69.0322330243336,13.1167814293496,
0.));
#147007=CARTESIAN_POINT('Ctrl Pts',(-69.0322330243336,13.1167814293496,
12.));
#147008=CARTESIAN_POINT('Ctrl Pts',(-69.0141906015137,13.1078283799726,
0.));
#147009=CARTESIAN_POINT('Ctrl Pts',(-69.0141906015137,13.1078283799726,
12.));
#147010=CARTESIAN_POINT('Ctrl Pts',(-68.9961858241577,13.0989178791843,
0.));
#147011=CARTESIAN_POINT('Ctrl Pts',(-68.9961858241577,13.0989178791843,
12.));
#147012=CARTESIAN_POINT('Ctrl Pts',(-68.9782188692654,13.0900499290542,
0.));
#147013=CARTESIAN_POINT('Ctrl Pts',(-68.9782188692654,13.0900499290542,
12.));
#147014=CARTESIAN_POINT('Ctrl Pts',(-68.9602899187628,13.0812245317816,
0.));
#147015=CARTESIAN_POINT('Ctrl Pts',(-68.9602899187628,13.0812245317816,
12.));
#147016=CARTESIAN_POINT('Ctrl Pts',(-68.9423991694492,13.072441690283,0.));
#147017=CARTESIAN_POINT('Ctrl Pts',(-68.9423991694492,13.072441690283,12.));
#147018=CARTESIAN_POINT('Ctrl Pts',(-68.9245468449865,13.0637014089018,
0.));
#147019=CARTESIAN_POINT('Ctrl Pts',(-68.9245468449865,13.0637014089018,
12.));
#147020=CARTESIAN_POINT('Ctrl Pts',(-68.9067332040842,13.0550036938793,
0.));
#147021=CARTESIAN_POINT('Ctrl Pts',(-68.9067332040842,13.0550036938793,
12.));
#147022=CARTESIAN_POINT('Ctrl Pts',(-68.8889585151431,13.0463485518185,
0.));
#147023=CARTESIAN_POINT('Ctrl Pts',(-68.8889585151431,13.0463485518185,
12.));
#147024=CARTESIAN_POINT('Ctrl Pts',(-68.8712230321823,13.0377359881864,
0.));
#147025=CARTESIAN_POINT('Ctrl Pts',(-68.8712230321823,13.0377359881864,
12.));
#147026=CARTESIAN_POINT('Ctrl Pts',(-68.853526972687,13.0291660060118,0.));
#147027=CARTESIAN_POINT('Ctrl Pts',(-68.853526972687,13.0291660060118,12.));
#147028=CARTESIAN_POINT('Ctrl Pts',(-68.835870488774,13.0206386039729,0.));
#147029=CARTESIAN_POINT('Ctrl Pts',(-68.835870488774,13.0206386039729,12.));
#147030=CARTESIAN_POINT('Ctrl Pts',(-68.8182536654066,13.0121537769003,
0.));
#147031=CARTESIAN_POINT('Ctrl Pts',(-68.8182536654066,13.0121537769003,
12.));
#147032=CARTESIAN_POINT('Ctrl Pts',(-68.8041919669403,13.0053999700929,
0.));
#147033=CARTESIAN_POINT('Ctrl Pts',(-68.8041919669403,13.0053999700929,
12.));
#147034=CARTESIAN_POINT('Ctrl Pts',(-68.7936635625787,13.0003537683089,
0.));
#147035=CARTESIAN_POINT('Ctrl Pts',(-68.7936635625787,13.0003537683089,
12.));
#147036=CARTESIAN_POINT('Ctrl Pts',(-68.7866525680284,12.996998146029,0.));
#147037=CARTESIAN_POINT('Ctrl Pts',(-68.7866525680284,12.996998146029,12.));
#147038=CARTESIAN_POINT('Ctrl Pts',(-68.7831490561748,12.9953224629497,
0.));
#147039=CARTESIAN_POINT('Ctrl Pts',(-68.7831490561748,12.9953224629497,
12.));
#147040=CARTESIAN_POINT('',(-68.7831490561748,12.9953224629497,12.));
#147041=CARTESIAN_POINT('Ctrl Pts',(-68.7831490561748,12.9953224629497,
12.));
#147042=CARTESIAN_POINT('Ctrl Pts',(-68.7866525680284,12.996998146029,12.));
#147043=CARTESIAN_POINT('Ctrl Pts',(-68.7936635625787,13.0003537683089,
12.));
#147044=CARTESIAN_POINT('Ctrl Pts',(-68.8041919669403,13.0053999700929,
12.));
#147045=CARTESIAN_POINT('Ctrl Pts',(-68.8182536654066,13.0121537769003,
12.));
#147046=CARTESIAN_POINT('Ctrl Pts',(-68.835870488774,13.0206386039729,12.));
#147047=CARTESIAN_POINT('Ctrl Pts',(-68.853526972687,13.0291660060118,12.));
#147048=CARTESIAN_POINT('Ctrl Pts',(-68.8712230321823,13.0377359881864,
12.));
#147049=CARTESIAN_POINT('Ctrl Pts',(-68.8889585151431,13.0463485518185,
12.));
#147050=CARTESIAN_POINT('Ctrl Pts',(-68.9067332040842,13.0550036938793,
12.));
#147051=CARTESIAN_POINT('Ctrl Pts',(-68.9245468449865,13.0637014089018,
12.));
#147052=CARTESIAN_POINT('Ctrl Pts',(-68.9423991694492,13.072441690283,12.));
#147053=CARTESIAN_POINT('Ctrl Pts',(-68.9602899187628,13.0812245317816,
12.));
#147054=CARTESIAN_POINT('Ctrl Pts',(-68.9782188692654,13.0900499290542,
12.));
#147055=CARTESIAN_POINT('Ctrl Pts',(-68.9961858241577,13.0989178791843,
12.));
#147056=CARTESIAN_POINT('Ctrl Pts',(-69.0141906015137,13.1078283799726,
12.));
#147057=CARTESIAN_POINT('Ctrl Pts',(-69.0322330243336,13.1167814293496,
12.));
#147058=CARTESIAN_POINT('Ctrl Pts',(-69.0503129081778,13.1257770246379,
12.));
#147059=CARTESIAN_POINT('Ctrl Pts',(-69.0684300549426,13.1348151621825,
12.));
#147060=CARTESIAN_POINT('Ctrl Pts',(-69.0865842593063,13.1438958377397,
12.));
#147061=CARTESIAN_POINT('Ctrl Pts',(-69.1047753127633,13.1530190467181,
12.));
#147062=CARTESIAN_POINT('Ctrl Pts',(-69.1230030082598,13.1621847844533,
12.));
#147063=CARTESIAN_POINT('Ctrl Pts',(-69.141267145461,13.1713930465142,12.));
#147064=CARTESIAN_POINT('Ctrl Pts',(-69.1595675305294,13.1806438286944,
12.));
#147065=CARTESIAN_POINT('Ctrl Pts',(-69.1779039736026,13.189937126869,12.));
#147066=CARTESIAN_POINT('Ctrl Pts',(-69.1962762870524,13.1992729368928,
12.));
#147067=CARTESIAN_POINT('Ctrl Pts',(-69.2146842833506,13.2086512544729,
12.));
#147068=CARTESIAN_POINT('Ctrl Pts',(-69.2331277732819,13.2180720750586,
12.));
#147069=CARTESIAN_POINT('Ctrl Pts',(-69.2516065668809,13.2275353939044,
12.));
#147070=CARTESIAN_POINT('Ctrl Pts',(-69.2701204742435,13.2370412061218,
12.));
#147071=CARTESIAN_POINT('Ctrl Pts',(-69.2886693063193,13.2465895067264,
12.));
#147072=CARTESIAN_POINT('Ctrl Pts',(-69.3072528758546,13.2561802906901,
12.));
#147073=CARTESIAN_POINT('Ctrl Pts',(-69.3258709977416,13.2658135529616,
12.));
#147074=CARTESIAN_POINT('Ctrl Pts',(-69.3445234885088,13.2754892884438,
12.));
#147075=CARTESIAN_POINT('Ctrl Pts',(-69.3632101660071,13.2852074919767,
12.));
#147076=CARTESIAN_POINT('Ctrl Pts',(-69.3819308490407,13.2949681583165,
12.));
#147077=CARTESIAN_POINT('Ctrl Pts',(-69.4006853569485,13.3047712821046,
12.));
#147078=CARTESIAN_POINT('Ctrl Pts',(-69.4194735096238,13.3146168578739,
12.));
#147079=CARTESIAN_POINT('Ctrl Pts',(-69.4382951276983,13.3245048800641,
12.));
#147080=CARTESIAN_POINT('Ctrl Pts',(-69.4571500326673,13.3344353430313,
12.));
#147081=CARTESIAN_POINT('Ctrl Pts',(-69.4760380470382,13.3444082410547,
12.));
#147082=CARTESIAN_POINT('Ctrl Pts',(-69.4949589944633,13.3544235683399,
12.));
#147083=CARTESIAN_POINT('Ctrl Pts',(-69.5139126996703,13.3644813190225,
12.));
#147084=CARTESIAN_POINT('Ctrl Pts',(-69.5328989883899,13.3745814871668,
12.));
#147085=CARTESIAN_POINT('Ctrl Pts',(-69.5519176872857,13.3847240667627,
12.));
#147086=CARTESIAN_POINT('Ctrl Pts',(-69.5709686238701,13.3949090517173,
12.));
#147087=CARTESIAN_POINT('Ctrl Pts',(-69.5900516264524,13.4051364358495,
12.));
#147088=CARTESIAN_POINT('Ctrl Pts',(-69.6091665241743,13.4154062128998,
12.));
#147089=CARTESIAN_POINT('Ctrl Pts',(-69.6283131470267,13.425718376534,12.));
#147090=CARTESIAN_POINT('Ctrl Pts',(-69.6474913258684,13.4360729203444,
12.));
#147091=CARTESIAN_POINT('Ctrl Pts',(-69.6667008924454,13.4464698378456,
12.));
#147092=CARTESIAN_POINT('Ctrl Pts',(-69.6859416793898,13.4569091224763,
12.));
#147093=CARTESIAN_POINT('Ctrl Pts',(-69.7052135202003,13.4673907676045,
12.));
#147094=CARTESIAN_POINT('Ctrl Pts',(-69.7245162492251,13.4779147665286,
12.));
#147095=CARTESIAN_POINT('Ctrl Pts',(-69.7438497016404,13.4884811124748,
12.));
#147096=CARTESIAN_POINT('Ctrl Pts',(-69.7632137134247,13.4990897985904,
12.));
#147097=CARTESIAN_POINT('Ctrl Pts',(-69.7826081213575,13.5097408179479,
12.));
#147098=CARTESIAN_POINT('Ctrl Pts',(-69.8020327630204,13.5204341635507,
12.));
#147099=CARTESIAN_POINT('Ctrl Pts',(-69.8214874767944,13.5311698283339,
12.));
#147100=CARTESIAN_POINT('Ctrl Pts',(-69.840972101856,13.5419478051626,12.));
#147101=CARTESIAN_POINT('Ctrl Pts',(-69.8604864781705,13.5527680868256,
12.));
#147102=CARTESIAN_POINT('Ctrl Pts',(-69.880030446488,13.5636306660423,12.));
#147103=CARTESIAN_POINT('Ctrl Pts',(-69.899603848336,13.5745355354657,12.));
#147104=CARTESIAN_POINT('Ctrl Pts',(-69.9192065260107,13.5854826876834,
12.));
#147105=CARTESIAN_POINT('Ctrl Pts',(-69.9388383225655,13.5964721152136,
12.));
#147106=CARTESIAN_POINT('Ctrl Pts',(-69.9584990817989,13.6075038105001,
12.));
#147107=CARTESIAN_POINT('Ctrl Pts',(-69.9781886482543,13.61857776592,12.));
#147108=CARTESIAN_POINT('Ctrl Pts',(-69.9979068672163,13.6296939737866,
12.));
#147109=CARTESIAN_POINT('Ctrl Pts',(-70.0176535847047,13.6408524263496,
12.));
#147110=CARTESIAN_POINT('Ctrl Pts',(-70.037428647466,13.6520531157904,12.));
#147111=CARTESIAN_POINT('Ctrl Pts',(-70.057231902965,13.6632960342192,12.));
#147112=CARTESIAN_POINT('Ctrl Pts',(-70.0770631993831,13.6745811736825,
12.));
#147113=CARTESIAN_POINT('Ctrl Pts',(-70.0969223856123,13.6859085261651,
12.));
#147114=CARTESIAN_POINT('Ctrl Pts',(-70.1168093112493,13.6972780835899,
12.));
#147115=CARTESIAN_POINT('Ctrl Pts',(-70.1367238265853,13.7086898378127,
12.));
#147116=CARTESIAN_POINT('Ctrl Pts',(-70.1566657825989,13.7201437806207,
12.));
#147117=CARTESIAN_POINT('Ctrl Pts',(-70.1766350309554,13.73163990374,12.));
#147118=CARTESIAN_POINT('Ctrl Pts',(-70.1966314240012,13.7431781988368,
12.));
#147119=CARTESIAN_POINT('Ctrl Pts',(-70.216654814759,13.7547586575178,12.));
#147120=CARTESIAN_POINT('Ctrl Pts',(-70.2367050569174,13.7663812713235,
12.));
#147121=CARTESIAN_POINT('Ctrl Pts',(-70.2567820048253,13.7780460317284,
12.));
#147122=CARTESIAN_POINT('Ctrl Pts',(-70.2768855134909,13.7897529301483,
12.));
#147123=CARTESIAN_POINT('Ctrl Pts',(-70.2970154385763,13.8015019579411,
12.));
#147124=CARTESIAN_POINT('Ctrl Pts',(-70.3171716363912,13.8132931064067,
12.));
#147125=CARTESIAN_POINT('Ctrl Pts',(-70.3373539638841,13.8251263667799,
12.));
#147126=CARTESIAN_POINT('Ctrl Pts',(-70.3575622786373,13.8370017302319,
12.));
#147127=CARTESIAN_POINT('Ctrl Pts',(-70.377796438866,13.8489191878774,12.));
#147128=CARTESIAN_POINT('Ctrl Pts',(-70.3980563034142,13.8608787307754,
12.));
#147129=CARTESIAN_POINT('Ctrl Pts',(-70.4183417317486,13.8728803499284,
12.));
#147130=CARTESIAN_POINT('Ctrl Pts',(-70.4386525839492,13.8849240362757,
12.));
#147131=CARTESIAN_POINT('Ctrl Pts',(-70.4589887207043,13.8970097806948,
12.));
#147132=CARTESIAN_POINT('Ctrl Pts',(-70.4793500033106,13.9091375740085,
12.));
#147133=CARTESIAN_POINT('Ctrl Pts',(-70.4997362936671,13.9213074069852,
12.));
#147134=CARTESIAN_POINT('Ctrl Pts',(-70.5201474542717,13.933519270339,12.));
#147135=CARTESIAN_POINT('Ctrl Pts',(-70.5405833482123,13.9457731547218,
12.));
#147136=CARTESIAN_POINT('Ctrl Pts',(-70.5610438391622,13.9580690507262,
12.));
#147137=CARTESIAN_POINT('Ctrl Pts',(-70.5815287913791,13.9704069488918,
12.));
#147138=CARTESIAN_POINT('Ctrl Pts',(-70.6020380697004,13.9827868397057,
12.));
#147139=CARTESIAN_POINT('Ctrl Pts',(-70.6225715395392,13.9952087136018,
12.));
#147140=CARTESIAN_POINT('Ctrl Pts',(-70.6431290668744,14.0076725609537,
12.));
#147141=CARTESIAN_POINT('Ctrl Pts',(-70.6637105182487,14.020178372077,12.));
#147142=CARTESIAN_POINT('Ctrl Pts',(-70.6843157607672,14.0327261372363,
12.));
#147143=CARTESIAN_POINT('Ctrl Pts',(-70.7049446620931,14.0453158466451,
12.));
#147144=CARTESIAN_POINT('Ctrl Pts',(-70.7255970904433,14.0579474904657,
12.));
#147145=CARTESIAN_POINT('Ctrl Pts',(-70.7462729145799,14.0706210588015,
12.));
#147146=CARTESIAN_POINT('Ctrl Pts',(-70.7669720038067,14.0833365416995,
12.));
#147147=CARTESIAN_POINT('Ctrl Pts',(-70.787694227969,14.0960939291569,12.));
#147148=CARTESIAN_POINT('Ctrl Pts',(-70.8084394574491,14.1088932111215,
12.));
#147149=CARTESIAN_POINT('Ctrl Pts',(-70.8292075631624,14.1217343774914,
12.));
#147150=CARTESIAN_POINT('Ctrl Pts',(-70.8499984165493,14.1346174181079,
12.));
#147151=CARTESIAN_POINT('Ctrl Pts',(-70.8708118895717,14.1475423227568,
12.));
#147152=CARTESIAN_POINT('Ctrl Pts',(-70.8916478547131,14.1605090811754,
12.));
#147153=CARTESIAN_POINT('Ctrl Pts',(-70.9125061849744,14.1735176830533,
12.));
#147154=CARTESIAN_POINT('Ctrl Pts',(-70.9333867538704,14.1865681180321,
12.));
#147155=CARTESIAN_POINT('Ctrl Pts',(-70.9542894354221,14.1996603756984,
12.));
#147156=CARTESIAN_POINT('Ctrl Pts',(-70.9752141041527,14.2127944455841,
12.));
#147157=CARTESIAN_POINT('Ctrl Pts',(-70.996160635087,14.2259703171739,12.));
#147158=CARTESIAN_POINT('Ctrl Pts',(-71.0171289037493,14.2391879799063,
12.));
#147159=CARTESIAN_POINT('Ctrl Pts',(-71.0381187861585,14.2524474231732,
12.));
#147160=CARTESIAN_POINT('Ctrl Pts',(-71.059130158822,14.2657486363137,12.));
#147161=CARTESIAN_POINT('Ctrl Pts',(-71.0801628987314,14.279091608613,12.));
#147162=CARTESIAN_POINT('Ctrl Pts',(-71.1012168833626,14.2924763293101,
12.));
#147163=CARTESIAN_POINT('Ctrl Pts',(-71.1222919906718,14.3059027875993,
12.));
#147164=CARTESIAN_POINT('Ctrl Pts',(-71.1433880990932,14.3193709726295,
12.));
#147165=CARTESIAN_POINT('Ctrl Pts',(-71.1645050875323,14.3328808734993,
12.));
#147166=CARTESIAN_POINT('Ctrl Pts',(-71.185642835361,14.3464324792537,12.));
#147167=CARTESIAN_POINT('Ctrl Pts',(-71.2068012224187,14.3600257788927,
12.));
#147168=CARTESIAN_POINT('Ctrl Pts',(-71.2279801290088,14.3736607613723,
12.));
#147169=CARTESIAN_POINT('Ctrl Pts',(-71.2491794358956,14.3873374156056,
12.));
#147170=CARTESIAN_POINT('Ctrl Pts',(-71.2703990242986,14.401055730457,12.));
#147171=CARTESIAN_POINT('Ctrl Pts',(-71.2916387758864,14.4148156947384,
12.));
#147172=CARTESIAN_POINT('Ctrl Pts',(-71.3128985727777,14.4286172972168,
12.));
#147173=CARTESIAN_POINT('Ctrl Pts',(-71.3341782975393,14.4424605266167,
12.));
#147174=CARTESIAN_POINT('Ctrl Pts',(-71.3554778331835,14.4563453716204,
12.));
#147175=CARTESIAN_POINT('Ctrl Pts',(-71.3767970631642,14.470271820865,12.));
#147176=CARTESIAN_POINT('Ctrl Pts',(-71.398135871371,14.4842398629354,12.));
#147177=CARTESIAN_POINT('Ctrl Pts',(-71.4194941421279,14.4982494863716,
12.));
#147178=CARTESIAN_POINT('Ctrl Pts',(-71.4408717601917,14.5123006796728,
12.));
#147179=CARTESIAN_POINT('Ctrl Pts',(-71.4622686107475,14.5263934312969,
12.));
#147180=CARTESIAN_POINT('Ctrl Pts',(-71.4836845794052,14.540527729659,12.));
#147181=CARTESIAN_POINT('Ctrl Pts',(-71.5051195521914,14.5547035631234,
12.));
#147182=CARTESIAN_POINT('Ctrl Pts',(-71.52657341555,14.5689209200091,12.));
#147183=CARTESIAN_POINT('Ctrl Pts',(-71.5480460563445,14.5831797885951,
12.));
#147184=CARTESIAN_POINT('Ctrl Pts',(-71.569537361856,14.597480157121,12.));
#147185=CARTESIAN_POINT('Ctrl Pts',(-71.5910472197814,14.611822013785,12.));
#147186=CARTESIAN_POINT('Ctrl Pts',(-71.6125755182295,14.6262053467372,
12.));
#147187=CARTESIAN_POINT('Ctrl Pts',(-71.6341221457175,14.6406301440817,
12.));
#147188=CARTESIAN_POINT('Ctrl Pts',(-71.6556869911669,14.6550963938832,
12.));
#147189=CARTESIAN_POINT('Ctrl Pts',(-71.6772699438966,14.669604084168,12.));
#147190=CARTESIAN_POINT('Ctrl Pts',(-71.698870893617,14.6841532029232,12.));
#147191=CARTESIAN_POINT('Ctrl Pts',(-71.7204897304186,14.6987437380898,
12.));
#147192=CARTESIAN_POINT('Ctrl Pts',(-71.7421263447707,14.7133756775622,
12.));
#147193=CARTESIAN_POINT('Ctrl Pts',(-71.7637806275316,14.7280490091954,
12.));
#147194=CARTESIAN_POINT('Ctrl Pts',(-71.7854524699562,14.7427637208071,
12.));
#147195=CARTESIAN_POINT('Ctrl Pts',(-71.8071417637018,14.7575198001777,
12.));
#147196=CARTESIAN_POINT('Ctrl Pts',(-71.8288484008343,14.7723172350455,
12.));
#147197=CARTESIAN_POINT('Ctrl Pts',(-71.8505722738286,14.7871560131021,
12.));
#147198=CARTESIAN_POINT('Ctrl Pts',(-71.872313275546,14.8020361220003,12.));
#147199=CARTESIAN_POINT('Ctrl Pts',(-71.8940712992119,14.816957549356,12.));
#147200=CARTESIAN_POINT('Ctrl Pts',(-71.9158462383915,14.8319202827483,
12.));
#147201=CARTESIAN_POINT('Ctrl Pts',(-71.9376379869668,14.846924309716,12.));
#147202=CARTESIAN_POINT('Ctrl Pts',(-71.9594464391063,14.8619696177503,
12.));
#147203=CARTESIAN_POINT('Ctrl Pts',(-71.9812714893087,14.8770561943011,
12.));
#147204=CARTESIAN_POINT('Ctrl Pts',(-72.0031130324519,14.892184026783,12.));
#147205=CARTESIAN_POINT('Ctrl Pts',(-72.0249709638419,14.9073531025764,
12.));
#147206=CARTESIAN_POINT('Ctrl Pts',(-72.046845179251,14.9225634090269,12.));
#147207=CARTESIAN_POINT('Ctrl Pts',(-72.0687355749815,14.937814933439,12.));
#147208=CARTESIAN_POINT('Ctrl Pts',(-72.0906420478085,14.953107663077,12.));
#147209=CARTESIAN_POINT('Ctrl Pts',(-72.1125644948547,14.96844158517,12.));
#147210=CARTESIAN_POINT('Ctrl Pts',(-72.1345028134779,14.9838166869107,
12.));
#147211=CARTESIAN_POINT('Ctrl Pts',(-72.1564569011668,14.9992329554537,
12.));
#147212=CARTESIAN_POINT('Ctrl Pts',(-72.1784266553948,15.0146903779061,
12.));
#147213=CARTESIAN_POINT('Ctrl Pts',(-72.2004119736104,15.0301889413255,
12.));
#147214=CARTESIAN_POINT('Ctrl Pts',(-72.2224127535401,15.0457286327328,
12.));
#147215=CARTESIAN_POINT('Ctrl Pts',(-72.244428893425,15.0613094391186,12.));
#147216=CARTESIAN_POINT('Ctrl Pts',(-72.266460292285,15.0769313474476,12.));
#147217=CARTESIAN_POINT('Ctrl Pts',(-72.2885068501641,15.0925943446593,
12.));
#147218=CARTESIAN_POINT('Ctrl Pts',(-72.3105684683971,15.1082984176656,
12.));
#147219=CARTESIAN_POINT('Ctrl Pts',(-72.332645049021,15.1240435533478,12.));
#147220=CARTESIAN_POINT('Ctrl Pts',(-72.3547364941996,15.1398297385513,
12.));
#147221=CARTESIAN_POINT('Ctrl Pts',(-72.37684270559,15.1556569600747,12.));
#147222=CARTESIAN_POINT('Ctrl Pts',(-72.3989635838476,15.1715252046603,
12.));
#147223=CARTESIAN_POINT('Ctrl Pts',(-72.4210990277819,15.1874344589716,
12.));
#147224=CARTESIAN_POINT('Ctrl Pts',(-72.4432489350415,15.2033847096077,
12.));
#147225=CARTESIAN_POINT('Ctrl Pts',(-72.4654132036373,15.2193759431359,
12.));
#147226=CARTESIAN_POINT('Ctrl Pts',(-72.4875917332729,15.2354081461152,
12.));
#147227=CARTESIAN_POINT('Ctrl Pts',(-72.5097844266083,15.2514813051174,
12.));
#147228=CARTESIAN_POINT('Ctrl Pts',(-72.5319911908978,15.2675954067495,
12.));
#147229=CARTESIAN_POINT('Ctrl Pts',(-72.5542119383748,15.2837504376562,
12.));
#147230=CARTESIAN_POINT('Ctrl Pts',(-72.5732713370795,15.2976335024853,
12.));
#147231=CARTESIAN_POINT('Ctrl Pts',(-72.5878912620662,15.3082994603651,
12.));
#147232=CARTESIAN_POINT('Ctrl Pts',(-72.5980655789897,15.3157301930832,
12.));
#147233=CARTESIAN_POINT('Ctrl Pts',(-72.6037902605225,15.3199137230318,
12.));
#147234=CARTESIAN_POINT('Ctrl Pts',(-72.6050633494711,15.320844207742,12.));
#147235=CARTESIAN_POINT('',(-68.7831490561748,12.9953224629497,0.));
#147236=CARTESIAN_POINT('',(-68.7831490561748,12.9953224629497,0.));
#147237=CARTESIAN_POINT('Ctrl Pts',(-72.6050633494711,15.320844207742,0.));
#147238=CARTESIAN_POINT('Ctrl Pts',(-72.6037902605226,15.3199137230318,
0.));
#147239=CARTESIAN_POINT('Ctrl Pts',(-72.5980655789897,15.3157301930832,
0.));
#147240=CARTESIAN_POINT('Ctrl Pts',(-72.5878912620662,15.3082994603651,
0.));
#147241=CARTESIAN_POINT('Ctrl Pts',(-72.5732713370795,15.2976335024853,
0.));
#147242=CARTESIAN_POINT('Ctrl Pts',(-72.5542119383748,15.2837504376562,
0.));
#147243=CARTESIAN_POINT('Ctrl Pts',(-72.5319911908978,15.2675954067495,
0.));
#147244=CARTESIAN_POINT('Ctrl Pts',(-72.5097844266083,15.2514813051174,
0.));
#147245=CARTESIAN_POINT('Ctrl Pts',(-72.4875917332729,15.2354081461152,
0.));
#147246=CARTESIAN_POINT('Ctrl Pts',(-72.4654132036373,15.2193759431359,
0.));
#147247=CARTESIAN_POINT('Ctrl Pts',(-72.4432489350415,15.2033847096077,
0.));
#147248=CARTESIAN_POINT('Ctrl Pts',(-72.4210990277819,15.1874344589716,
0.));
#147249=CARTESIAN_POINT('Ctrl Pts',(-72.3989635838476,15.1715252046603,
0.));
#147250=CARTESIAN_POINT('Ctrl Pts',(-72.37684270559,15.1556569600747,0.));
#147251=CARTESIAN_POINT('Ctrl Pts',(-72.3547364941996,15.1398297385513,
0.));
#147252=CARTESIAN_POINT('Ctrl Pts',(-72.332645049021,15.1240435533478,0.));
#147253=CARTESIAN_POINT('Ctrl Pts',(-72.3105684683971,15.1082984176656,
0.));
#147254=CARTESIAN_POINT('Ctrl Pts',(-72.2885068501641,15.0925943446593,
0.));
#147255=CARTESIAN_POINT('Ctrl Pts',(-72.266460292285,15.0769313474476,0.));
#147256=CARTESIAN_POINT('Ctrl Pts',(-72.244428893425,15.0613094391186,0.));
#147257=CARTESIAN_POINT('Ctrl Pts',(-72.2224127535401,15.0457286327328,
0.));
#147258=CARTESIAN_POINT('Ctrl Pts',(-72.2004119736104,15.0301889413255,
0.));
#147259=CARTESIAN_POINT('Ctrl Pts',(-72.1784266553948,15.0146903779061,
0.));
#147260=CARTESIAN_POINT('Ctrl Pts',(-72.1564569011668,14.9992329554537,
0.));
#147261=CARTESIAN_POINT('Ctrl Pts',(-72.1345028134779,14.9838166869107,
0.));
#147262=CARTESIAN_POINT('Ctrl Pts',(-72.1125644948547,14.96844158517,0.));
#147263=CARTESIAN_POINT('Ctrl Pts',(-72.0906420478085,14.953107663077,0.));
#147264=CARTESIAN_POINT('Ctrl Pts',(-72.0687355749815,14.937814933439,0.));
#147265=CARTESIAN_POINT('Ctrl Pts',(-72.046845179251,14.9225634090269,0.));
#147266=CARTESIAN_POINT('Ctrl Pts',(-72.0249709638419,14.9073531025764,
0.));
#147267=CARTESIAN_POINT('Ctrl Pts',(-72.0031130324519,14.892184026783,0.));
#147268=CARTESIAN_POINT('Ctrl Pts',(-71.9812714893087,14.8770561943011,
0.));
#147269=CARTESIAN_POINT('Ctrl Pts',(-71.9594464391063,14.8619696177503,
0.));
#147270=CARTESIAN_POINT('Ctrl Pts',(-71.9376379869668,14.846924309716,0.));
#147271=CARTESIAN_POINT('Ctrl Pts',(-71.9158462383915,14.8319202827483,
0.));
#147272=CARTESIAN_POINT('Ctrl Pts',(-71.8940712992119,14.816957549356,0.));
#147273=CARTESIAN_POINT('Ctrl Pts',(-71.872313275546,14.8020361220003,0.));
#147274=CARTESIAN_POINT('Ctrl Pts',(-71.8505722738286,14.7871560131021,
0.));
#147275=CARTESIAN_POINT('Ctrl Pts',(-71.8288484008343,14.7723172350455,
0.));
#147276=CARTESIAN_POINT('Ctrl Pts',(-71.8071417637018,14.7575198001777,
0.));
#147277=CARTESIAN_POINT('Ctrl Pts',(-71.7854524699562,14.7427637208071,
0.));
#147278=CARTESIAN_POINT('Ctrl Pts',(-71.7637806275316,14.7280490091954,
0.));
#147279=CARTESIAN_POINT('Ctrl Pts',(-71.7421263447707,14.7133756775622,
0.));
#147280=CARTESIAN_POINT('Ctrl Pts',(-71.7204897304186,14.6987437380898,
0.));
#147281=CARTESIAN_POINT('Ctrl Pts',(-71.698870893617,14.6841532029232,0.));
#147282=CARTESIAN_POINT('Ctrl Pts',(-71.6772699438966,14.669604084168,0.));
#147283=CARTESIAN_POINT('Ctrl Pts',(-71.6556869911669,14.6550963938832,
0.));
#147284=CARTESIAN_POINT('Ctrl Pts',(-71.6341221457175,14.6406301440817,
0.));
#147285=CARTESIAN_POINT('Ctrl Pts',(-71.6125755182295,14.6262053467372,
0.));
#147286=CARTESIAN_POINT('Ctrl Pts',(-71.5910472197814,14.611822013785,0.));
#147287=CARTESIAN_POINT('Ctrl Pts',(-71.569537361856,14.597480157121,0.));
#147288=CARTESIAN_POINT('Ctrl Pts',(-71.5480460563445,14.5831797885951,
0.));
#147289=CARTESIAN_POINT('Ctrl Pts',(-71.52657341555,14.5689209200091,0.));
#147290=CARTESIAN_POINT('Ctrl Pts',(-71.5051195521914,14.5547035631234,
0.));
#147291=CARTESIAN_POINT('Ctrl Pts',(-71.4836845794052,14.540527729659,0.));
#147292=CARTESIAN_POINT('Ctrl Pts',(-71.4622686107475,14.5263934312969,
0.));
#147293=CARTESIAN_POINT('Ctrl Pts',(-71.4408717601917,14.5123006796728,
0.));
#147294=CARTESIAN_POINT('Ctrl Pts',(-71.4194941421279,14.4982494863716,
0.));
#147295=CARTESIAN_POINT('Ctrl Pts',(-71.398135871371,14.4842398629354,0.));
#147296=CARTESIAN_POINT('Ctrl Pts',(-71.3767970631642,14.470271820865,0.));
#147297=CARTESIAN_POINT('Ctrl Pts',(-71.3554778331835,14.4563453716204,
0.));
#147298=CARTESIAN_POINT('Ctrl Pts',(-71.3341782975393,14.4424605266167,
0.));
#147299=CARTESIAN_POINT('Ctrl Pts',(-71.3128985727777,14.4286172972168,
0.));
#147300=CARTESIAN_POINT('Ctrl Pts',(-71.2916387758864,14.4148156947384,
0.));
#147301=CARTESIAN_POINT('Ctrl Pts',(-71.2703990242986,14.401055730457,0.));
#147302=CARTESIAN_POINT('Ctrl Pts',(-71.2491794358956,14.3873374156056,
0.));
#147303=CARTESIAN_POINT('Ctrl Pts',(-71.2279801290088,14.3736607613723,
0.));
#147304=CARTESIAN_POINT('Ctrl Pts',(-71.2068012224187,14.3600257788927,
0.));
#147305=CARTESIAN_POINT('Ctrl Pts',(-71.185642835361,14.3464324792537,0.));
#147306=CARTESIAN_POINT('Ctrl Pts',(-71.1645050875323,14.3328808734993,
0.));
#147307=CARTESIAN_POINT('Ctrl Pts',(-71.1433880990932,14.3193709726295,
0.));
#147308=CARTESIAN_POINT('Ctrl Pts',(-71.1222919906718,14.3059027875993,
0.));
#147309=CARTESIAN_POINT('Ctrl Pts',(-71.1012168833626,14.2924763293101,
0.));
#147310=CARTESIAN_POINT('Ctrl Pts',(-71.0801628987314,14.279091608613,0.));
#147311=CARTESIAN_POINT('Ctrl Pts',(-71.059130158822,14.2657486363137,0.));
#147312=CARTESIAN_POINT('Ctrl Pts',(-71.0381187861585,14.2524474231732,
0.));
#147313=CARTESIAN_POINT('Ctrl Pts',(-71.0171289037493,14.2391879799063,
0.));
#147314=CARTESIAN_POINT('Ctrl Pts',(-70.996160635087,14.2259703171739,0.));
#147315=CARTESIAN_POINT('Ctrl Pts',(-70.9752141041527,14.2127944455841,
0.));
#147316=CARTESIAN_POINT('Ctrl Pts',(-70.9542894354221,14.1996603756984,
0.));
#147317=CARTESIAN_POINT('Ctrl Pts',(-70.9333867538704,14.1865681180321,
0.));
#147318=CARTESIAN_POINT('Ctrl Pts',(-70.9125061849744,14.1735176830533,
0.));
#147319=CARTESIAN_POINT('Ctrl Pts',(-70.8916478547131,14.1605090811754,
0.));
#147320=CARTESIAN_POINT('Ctrl Pts',(-70.8708118895717,14.1475423227568,
0.));
#147321=CARTESIAN_POINT('Ctrl Pts',(-70.8499984165493,14.1346174181079,
0.));
#147322=CARTESIAN_POINT('Ctrl Pts',(-70.8292075631624,14.1217343774914,
0.));
#147323=CARTESIAN_POINT('Ctrl Pts',(-70.8084394574491,14.1088932111215,
0.));
#147324=CARTESIAN_POINT('Ctrl Pts',(-70.787694227969,14.0960939291569,0.));
#147325=CARTESIAN_POINT('Ctrl Pts',(-70.7669720038067,14.0833365416995,
0.));
#147326=CARTESIAN_POINT('Ctrl Pts',(-70.7462729145799,14.0706210588015,
0.));
#147327=CARTESIAN_POINT('Ctrl Pts',(-70.7255970904433,14.0579474904657,
0.));
#147328=CARTESIAN_POINT('Ctrl Pts',(-70.7049446620931,14.0453158466451,
0.));
#147329=CARTESIAN_POINT('Ctrl Pts',(-70.6843157607672,14.0327261372363,
0.));
#147330=CARTESIAN_POINT('Ctrl Pts',(-70.6637105182487,14.020178372077,0.));
#147331=CARTESIAN_POINT('Ctrl Pts',(-70.6431290668744,14.0076725609537,
0.));
#147332=CARTESIAN_POINT('Ctrl Pts',(-70.6225715395392,13.9952087136018,
0.));
#147333=CARTESIAN_POINT('Ctrl Pts',(-70.6020380697004,13.9827868397057,
0.));
#147334=CARTESIAN_POINT('Ctrl Pts',(-70.5815287913791,13.9704069488918,
0.));
#147335=CARTESIAN_POINT('Ctrl Pts',(-70.5610438391622,13.9580690507262,
0.));
#147336=CARTESIAN_POINT('Ctrl Pts',(-70.5405833482123,13.9457731547218,
0.));
#147337=CARTESIAN_POINT('Ctrl Pts',(-70.5201474542717,13.933519270339,0.));
#147338=CARTESIAN_POINT('Ctrl Pts',(-70.4997362936671,13.9213074069852,
0.));
#147339=CARTESIAN_POINT('Ctrl Pts',(-70.4793500033106,13.9091375740085,
0.));
#147340=CARTESIAN_POINT('Ctrl Pts',(-70.4589887207043,13.8970097806948,
0.));
#147341=CARTESIAN_POINT('Ctrl Pts',(-70.4386525839492,13.8849240362757,
0.));
#147342=CARTESIAN_POINT('Ctrl Pts',(-70.4183417317486,13.8728803499284,
0.));
#147343=CARTESIAN_POINT('Ctrl Pts',(-70.3980563034142,13.8608787307754,
0.));
#147344=CARTESIAN_POINT('Ctrl Pts',(-70.377796438866,13.8489191878774,0.));
#147345=CARTESIAN_POINT('Ctrl Pts',(-70.3575622786373,13.8370017302319,
0.));
#147346=CARTESIAN_POINT('Ctrl Pts',(-70.3373539638841,13.8251263667799,
0.));
#147347=CARTESIAN_POINT('Ctrl Pts',(-70.3171716363912,13.8132931064067,
0.));
#147348=CARTESIAN_POINT('Ctrl Pts',(-70.2970154385763,13.8015019579411,
0.));
#147349=CARTESIAN_POINT('Ctrl Pts',(-70.2768855134909,13.7897529301483,
0.));
#147350=CARTESIAN_POINT('Ctrl Pts',(-70.2567820048253,13.7780460317284,
0.));
#147351=CARTESIAN_POINT('Ctrl Pts',(-70.2367050569174,13.7663812713235,
0.));
#147352=CARTESIAN_POINT('Ctrl Pts',(-70.216654814759,13.7547586575178,0.));
#147353=CARTESIAN_POINT('Ctrl Pts',(-70.1966314240012,13.7431781988368,
0.));
#147354=CARTESIAN_POINT('Ctrl Pts',(-70.1766350309554,13.73163990374,0.));
#147355=CARTESIAN_POINT('Ctrl Pts',(-70.1566657825989,13.7201437806207,
0.));
#147356=CARTESIAN_POINT('Ctrl Pts',(-70.1367238265853,13.7086898378127,
0.));
#147357=CARTESIAN_POINT('Ctrl Pts',(-70.1168093112493,13.6972780835899,
0.));
#147358=CARTESIAN_POINT('Ctrl Pts',(-70.0969223856123,13.6859085261651,
0.));
#147359=CARTESIAN_POINT('Ctrl Pts',(-70.0770631993831,13.6745811736825,
0.));
#147360=CARTESIAN_POINT('Ctrl Pts',(-70.057231902965,13.6632960342192,0.));
#147361=CARTESIAN_POINT('Ctrl Pts',(-70.037428647466,13.6520531157904,0.));
#147362=CARTESIAN_POINT('Ctrl Pts',(-70.0176535847047,13.6408524263496,
0.));
#147363=CARTESIAN_POINT('Ctrl Pts',(-69.9979068672163,13.6296939737866,
0.));
#147364=CARTESIAN_POINT('Ctrl Pts',(-69.9781886482543,13.61857776592,0.));
#147365=CARTESIAN_POINT('Ctrl Pts',(-69.9584990817989,13.6075038105001,
0.));
#147366=CARTESIAN_POINT('Ctrl Pts',(-69.9388383225655,13.5964721152136,
0.));
#147367=CARTESIAN_POINT('Ctrl Pts',(-69.9192065260107,13.5854826876834,
0.));
#147368=CARTESIAN_POINT('Ctrl Pts',(-69.899603848336,13.5745355354657,0.));
#147369=CARTESIAN_POINT('Ctrl Pts',(-69.880030446488,13.5636306660423,0.));
#147370=CARTESIAN_POINT('Ctrl Pts',(-69.8604864781705,13.5527680868256,
0.));
#147371=CARTESIAN_POINT('Ctrl Pts',(-69.840972101856,13.5419478051626,0.));
#147372=CARTESIAN_POINT('Ctrl Pts',(-69.8214874767944,13.5311698283339,
0.));
#147373=CARTESIAN_POINT('Ctrl Pts',(-69.8020327630204,13.5204341635507,
0.));
#147374=CARTESIAN_POINT('Ctrl Pts',(-69.7826081213575,13.5097408179479,
0.));
#147375=CARTESIAN_POINT('Ctrl Pts',(-69.7632137134247,13.4990897985904,
0.));
#147376=CARTESIAN_POINT('Ctrl Pts',(-69.7438497016404,13.4884811124748,
0.));
#147377=CARTESIAN_POINT('Ctrl Pts',(-69.7245162492251,13.4779147665286,
0.));
#147378=CARTESIAN_POINT('Ctrl Pts',(-69.7052135202003,13.4673907676045,
0.));
#147379=CARTESIAN_POINT('Ctrl Pts',(-69.6859416793898,13.4569091224763,
0.));
#147380=CARTESIAN_POINT('Ctrl Pts',(-69.6667008924454,13.4464698378456,
0.));
#147381=CARTESIAN_POINT('Ctrl Pts',(-69.6474913258684,13.4360729203444,
0.));
#147382=CARTESIAN_POINT('Ctrl Pts',(-69.6283131470267,13.425718376534,0.));
#147383=CARTESIAN_POINT('Ctrl Pts',(-69.6091665241743,13.4154062128998,
0.));
#147384=CARTESIAN_POINT('Ctrl Pts',(-69.5900516264524,13.4051364358495,
0.));
#147385=CARTESIAN_POINT('Ctrl Pts',(-69.5709686238701,13.3949090517173,
0.));
#147386=CARTESIAN_POINT('Ctrl Pts',(-69.5519176872857,13.3847240667627,
0.));
#147387=CARTESIAN_POINT('Ctrl Pts',(-69.5328989883899,13.3745814871668,
0.));
#147388=CARTESIAN_POINT('Ctrl Pts',(-69.5139126996703,13.3644813190225,
0.));
#147389=CARTESIAN_POINT('Ctrl Pts',(-69.4949589944633,13.3544235683399,
0.));
#147390=CARTESIAN_POINT('Ctrl Pts',(-69.4760380470382,13.3444082410547,
0.));
#147391=CARTESIAN_POINT('Ctrl Pts',(-69.4571500326673,13.3344353430313,
0.));
#147392=CARTESIAN_POINT('Ctrl Pts',(-69.4382951276983,13.3245048800641,
0.));
#147393=CARTESIAN_POINT('Ctrl Pts',(-69.4194735096238,13.3146168578739,
0.));
#147394=CARTESIAN_POINT('Ctrl Pts',(-69.4006853569485,13.3047712821046,
0.));
#147395=CARTESIAN_POINT('Ctrl Pts',(-69.3819308490407,13.2949681583165,
0.));
#147396=CARTESIAN_POINT('Ctrl Pts',(-69.3632101660071,13.2852074919767,
0.));
#147397=CARTESIAN_POINT('Ctrl Pts',(-69.3445234885088,13.2754892884438,
0.));
#147398=CARTESIAN_POINT('Ctrl Pts',(-69.3258709977416,13.2658135529616,
0.));
#147399=CARTESIAN_POINT('Ctrl Pts',(-69.3072528758546,13.2561802906901,
0.));
#147400=CARTESIAN_POINT('Ctrl Pts',(-69.2886693063193,13.2465895067264,
0.));
#147401=CARTESIAN_POINT('Ctrl Pts',(-69.2701204742435,13.2370412061218,
0.));
#147402=CARTESIAN_POINT('Ctrl Pts',(-69.2516065668809,13.2275353939044,
0.));
#147403=CARTESIAN_POINT('Ctrl Pts',(-69.2331277732819,13.2180720750586,
0.));
#147404=CARTESIAN_POINT('Ctrl Pts',(-69.2146842833506,13.2086512544729,
0.));
#147405=CARTESIAN_POINT('Ctrl Pts',(-69.1962762870524,13.1992729368928,
0.));
#147406=CARTESIAN_POINT('Ctrl Pts',(-69.1779039736026,13.189937126869,0.));
#147407=CARTESIAN_POINT('Ctrl Pts',(-69.1595675305294,13.1806438286944,
0.));
#147408=CARTESIAN_POINT('Ctrl Pts',(-69.141267145461,13.1713930465142,0.));
#147409=CARTESIAN_POINT('Ctrl Pts',(-69.1230030082598,13.1621847844533,
0.));
#147410=CARTESIAN_POINT('Ctrl Pts',(-69.1047753127633,13.1530190467181,
0.));
#147411=CARTESIAN_POINT('Ctrl Pts',(-69.0865842593063,13.1438958377397,
0.));
#147412=CARTESIAN_POINT('Ctrl Pts',(-69.0684300549426,13.1348151621825,
0.));
#147413=CARTESIAN_POINT('Ctrl Pts',(-69.0503129081778,13.1257770246379,
0.));
#147414=CARTESIAN_POINT('Ctrl Pts',(-69.0322330243336,13.1167814293496,
0.));
#147415=CARTESIAN_POINT('Ctrl Pts',(-69.0141906015137,13.1078283799726,
0.));
#147416=CARTESIAN_POINT('Ctrl Pts',(-68.9961858241577,13.0989178791843,
0.));
#147417=CARTESIAN_POINT('Ctrl Pts',(-68.9782188692654,13.0900499290542,
0.));
#147418=CARTESIAN_POINT('Ctrl Pts',(-68.9602899187628,13.0812245317816,
0.));
#147419=CARTESIAN_POINT('Ctrl Pts',(-68.9423991694492,13.072441690283,0.));
#147420=CARTESIAN_POINT('Ctrl Pts',(-68.9245468449865,13.0637014089018,
0.));
#147421=CARTESIAN_POINT('Ctrl Pts',(-68.9067332040842,13.0550036938793,
0.));
#147422=CARTESIAN_POINT('Ctrl Pts',(-68.8889585151431,13.0463485518185,
0.));
#147423=CARTESIAN_POINT('Ctrl Pts',(-68.8712230321823,13.0377359881864,
0.));
#147424=CARTESIAN_POINT('Ctrl Pts',(-68.853526972687,13.0291660060118,0.));
#147425=CARTESIAN_POINT('Ctrl Pts',(-68.835870488774,13.0206386039729,0.));
#147426=CARTESIAN_POINT('Ctrl Pts',(-68.8182536654066,13.0121537769003,
0.));
#147427=CARTESIAN_POINT('Ctrl Pts',(-68.8041919669403,13.0053999700929,
0.));
#147428=CARTESIAN_POINT('Ctrl Pts',(-68.7936635625787,13.0003537683089,
0.));
#147429=CARTESIAN_POINT('Ctrl Pts',(-68.7866525680284,12.996998146029,0.));
#147430=CARTESIAN_POINT('Ctrl Pts',(-68.7831490561748,12.9953224629497,
0.));
#147431=CARTESIAN_POINT('Ctrl Pts',(-71.2372871136137,21.8059378310719,
0.));
#147432=CARTESIAN_POINT('Ctrl Pts',(-71.2372871136137,21.8059378310719,
12.));
#147433=CARTESIAN_POINT('Ctrl Pts',(-71.2331134397872,21.8022104901727,
0.));
#147434=CARTESIAN_POINT('Ctrl Pts',(-71.2331134397872,21.8022104901727,
12.));
#147435=CARTESIAN_POINT('Ctrl Pts',(-71.2247670210176,21.794759979896,0.));
#147436=CARTESIAN_POINT('Ctrl Pts',(-71.2247670210176,21.794759979896,12.));
#147437=CARTESIAN_POINT('Ctrl Pts',(-71.2122501795138,21.7835967290463,
0.));
#147438=CARTESIAN_POINT('Ctrl Pts',(-71.2122501795138,21.7835967290463,
12.));
#147439=CARTESIAN_POINT('Ctrl Pts',(-71.1955666310295,21.7687374247287,
0.));
#147440=CARTESIAN_POINT('Ctrl Pts',(-71.1955666310295,21.7687374247287,
12.));
#147441=CARTESIAN_POINT('Ctrl Pts',(-71.1747214906585,21.750205018381,0.));
#147442=CARTESIAN_POINT('Ctrl Pts',(-71.1747214906585,21.750205018381,12.));
#147443=CARTESIAN_POINT('Ctrl Pts',(-71.1538856612261,21.7317143472951,
0.));
#147444=CARTESIAN_POINT('Ctrl Pts',(-71.1538856612261,21.7317143472951,
12.));
#147445=CARTESIAN_POINT('Ctrl Pts',(-71.1330591726507,21.7132654262531,
0.));
#147446=CARTESIAN_POINT('Ctrl Pts',(-71.1330591726507,21.7132654262531,
12.));
#147447=CARTESIAN_POINT('Ctrl Pts',(-71.1122420728217,21.694858273085,0.));
#147448=CARTESIAN_POINT('Ctrl Pts',(-71.1122420728217,21.694858273085,12.));
#147449=CARTESIAN_POINT('Ctrl Pts',(-71.0914344332798,21.6764929081677,
0.));
#147450=CARTESIAN_POINT('Ctrl Pts',(-71.0914344332798,21.6764929081677,
12.));
#147451=CARTESIAN_POINT('Ctrl Pts',(-71.0706363472704,21.6581693538335,
0.));
#147452=CARTESIAN_POINT('Ctrl Pts',(-71.0706363472704,21.6581693538335,
12.));
#147453=CARTESIAN_POINT('Ctrl Pts',(-71.0498479219467,21.639887633714,0.));
#147454=CARTESIAN_POINT('Ctrl Pts',(-71.0498479219467,21.639887633714,12.));
#147455=CARTESIAN_POINT('Ctrl Pts',(-71.0290692721848,21.6216477720912,
0.));
#147456=CARTESIAN_POINT('Ctrl Pts',(-71.0290692721848,21.6216477720912,
12.));
#147457=CARTESIAN_POINT('Ctrl Pts',(-71.0083005139107,21.6034497932581,
0.));
#147458=CARTESIAN_POINT('Ctrl Pts',(-71.0083005139107,21.6034497932581,
12.));
#147459=CARTESIAN_POINT('Ctrl Pts',(-70.987541757223,21.585293720829,0.));
#147460=CARTESIAN_POINT('Ctrl Pts',(-70.987541757223,21.585293720829,12.));
#147461=CARTESIAN_POINT('Ctrl Pts',(-70.9667931008215,21.5671795771913,
0.));
#147462=CARTESIAN_POINT('Ctrl Pts',(-70.9667931008215,21.5671795771913,
12.));
#147463=CARTESIAN_POINT('Ctrl Pts',(-70.94605463587,21.5491073839106,0.));
#147464=CARTESIAN_POINT('Ctrl Pts',(-70.94605463587,21.5491073839106,12.));
#147465=CARTESIAN_POINT('Ctrl Pts',(-70.9253264487637,21.531077162023,0.));
#147466=CARTESIAN_POINT('Ctrl Pts',(-70.9253264487637,21.531077162023,12.));
#147467=CARTESIAN_POINT('Ctrl Pts',(-70.9046086244131,21.513088932377,0.));
#147468=CARTESIAN_POINT('Ctrl Pts',(-70.9046086244131,21.513088932377,12.));
#147469=CARTESIAN_POINT('Ctrl Pts',(-70.8839012490871,21.4951427159261,
0.));
#147470=CARTESIAN_POINT('Ctrl Pts',(-70.8839012490871,21.4951427159261,
12.));
#147471=CARTESIAN_POINT('Ctrl Pts',(-70.8632044140112,21.477238534096,0.));
#147472=CARTESIAN_POINT('Ctrl Pts',(-70.8632044140112,21.477238534096,12.));
#147473=CARTESIAN_POINT('Ctrl Pts',(-70.8425182149846,21.4593764087473,
0.));
#147474=CARTESIAN_POINT('Ctrl Pts',(-70.8425182149846,21.4593764087473,
12.));
#147475=CARTESIAN_POINT('Ctrl Pts',(-70.8218427507506,21.4415563620114,
0.));
#147476=CARTESIAN_POINT('Ctrl Pts',(-70.8218427507506,21.4415563620114,
12.));
#147477=CARTESIAN_POINT('Ctrl Pts',(-70.8011781217394,21.4237784161587,
0.));
#147478=CARTESIAN_POINT('Ctrl Pts',(-70.8011781217394,21.4237784161587,
12.));
#147479=CARTESIAN_POINT('Ctrl Pts',(-70.780524428745,21.4060425934598,0.));
#147480=CARTESIAN_POINT('Ctrl Pts',(-70.780524428745,21.4060425934598,12.));
#147481=CARTESIAN_POINT('Ctrl Pts',(-70.7598817714105,21.3883489160196,
0.));
#147482=CARTESIAN_POINT('Ctrl Pts',(-70.7598817714105,21.3883489160196,
12.));
#147483=CARTESIAN_POINT('Ctrl Pts',(-70.7392502475469,21.3706974057039,
0.));
#147484=CARTESIAN_POINT('Ctrl Pts',(-70.7392502475469,21.3706974057039,
12.));
#147485=CARTESIAN_POINT('Ctrl Pts',(-70.7186299539724,21.3530880842349,
0.));
#147486=CARTESIAN_POINT('Ctrl Pts',(-70.7186299539724,21.3530880842349,
12.));
#147487=CARTESIAN_POINT('Ctrl Pts',(-70.6980209870045,21.3355209732443,
0.));
#147488=CARTESIAN_POINT('Ctrl Pts',(-70.6980209870045,21.3355209732443,
12.));
#147489=CARTESIAN_POINT('Ctrl Pts',(-70.6774234430897,21.3179960943388,
0.));
#147490=CARTESIAN_POINT('Ctrl Pts',(-70.6774234430897,21.3179960943388,
12.));
#147491=CARTESIAN_POINT('Ctrl Pts',(-70.6568374193774,21.300513469156,0.));
#147492=CARTESIAN_POINT('Ctrl Pts',(-70.6568374193774,21.300513469156,12.));
#147493=CARTESIAN_POINT('Ctrl Pts',(-70.6362630143047,21.2830731194183,
0.));
#147494=CARTESIAN_POINT('Ctrl Pts',(-70.6362630143047,21.2830731194183,
12.));
#147495=CARTESIAN_POINT('Ctrl Pts',(-70.6157003273316,21.2656750669126,
0.));
#147496=CARTESIAN_POINT('Ctrl Pts',(-70.6157003273316,21.2656750669126,
12.));
#147497=CARTESIAN_POINT('Ctrl Pts',(-70.5951494586957,21.2483193334675,
0.));
#147498=CARTESIAN_POINT('Ctrl Pts',(-70.5951494586957,21.2483193334675,
12.));
#147499=CARTESIAN_POINT('Ctrl Pts',(-70.5746105091502,21.2310059409265,
0.));
#147500=CARTESIAN_POINT('Ctrl Pts',(-70.5746105091502,21.2310059409265,
12.));
#147501=CARTESIAN_POINT('Ctrl Pts',(-70.5540835797283,21.2137349111208,
0.));
#147502=CARTESIAN_POINT('Ctrl Pts',(-70.5540835797283,21.2137349111208,
12.));
#147503=CARTESIAN_POINT('Ctrl Pts',(-70.5335687714429,21.1965062658298,
0.));
#147504=CARTESIAN_POINT('Ctrl Pts',(-70.5335687714429,21.1965062658298,
12.));
#147505=CARTESIAN_POINT('Ctrl Pts',(-70.5130661852955,21.1793200267846,
0.));
#147506=CARTESIAN_POINT('Ctrl Pts',(-70.5130661852955,21.1793200267846,
12.));
#147507=CARTESIAN_POINT('Ctrl Pts',(-70.4925759224216,21.1621762156897,
0.));
#147508=CARTESIAN_POINT('Ctrl Pts',(-70.4925759224216,21.1621762156897,
12.));
#147509=CARTESIAN_POINT('Ctrl Pts',(-70.4720980841939,21.1450748542336,
0.));
#147510=CARTESIAN_POINT('Ctrl Pts',(-70.4720980841939,21.1450748542336,
12.));
#147511=CARTESIAN_POINT('Ctrl Pts',(-70.4516327723346,21.1280159641002,
0.));
#147512=CARTESIAN_POINT('Ctrl Pts',(-70.4516327723346,21.1280159641002,
12.));
#147513=CARTESIAN_POINT('Ctrl Pts',(-70.4311800890402,21.1109995669747,
0.));
#147514=CARTESIAN_POINT('Ctrl Pts',(-70.4311800890402,21.1109995669747,
12.));
#147515=CARTESIAN_POINT('Ctrl Pts',(-70.4107401370389,21.0940256845472,
0.));
#147516=CARTESIAN_POINT('Ctrl Pts',(-70.4107401370389,21.0940256845472,
12.));
#147517=CARTESIAN_POINT('Ctrl Pts',(-70.3903130195265,21.0770943385141,
0.));
#147518=CARTESIAN_POINT('Ctrl Pts',(-70.3903130195265,21.0770943385141,
12.));
#147519=CARTESIAN_POINT('Ctrl Pts',(-70.3698988401281,21.0602055505748,
0.));
#147520=CARTESIAN_POINT('Ctrl Pts',(-70.3698988401281,21.0602055505748,
12.));
#147521=CARTESIAN_POINT('Ctrl Pts',(-70.3494977028498,21.0433593424266,
0.));
#147522=CARTESIAN_POINT('Ctrl Pts',(-70.3494977028498,21.0433593424266,
12.));
#147523=CARTESIAN_POINT('Ctrl Pts',(-70.3291097120302,21.0265557357548,
0.));
#147524=CARTESIAN_POINT('Ctrl Pts',(-70.3291097120302,21.0265557357548,
12.));
#147525=CARTESIAN_POINT('Ctrl Pts',(-70.3087349722973,21.0097947522218,
0.));
#147526=CARTESIAN_POINT('Ctrl Pts',(-70.3087349722973,21.0097947522218,
12.));
#147527=CARTESIAN_POINT('Ctrl Pts',(-70.2883735885984,20.9930764134776,
0.));
#147528=CARTESIAN_POINT('Ctrl Pts',(-70.2883735885984,20.9930764134776,
12.));
#147529=CARTESIAN_POINT('Ctrl Pts',(-70.2680256662224,20.9764007411652,
0.));
#147530=CARTESIAN_POINT('Ctrl Pts',(-70.2680256662224,20.9764007411652,
12.));
#147531=CARTESIAN_POINT('Ctrl Pts',(-70.2476913108244,20.9597677569228,
0.));
#147532=CARTESIAN_POINT('Ctrl Pts',(-70.2476913108244,20.9597677569228,
12.));
#147533=CARTESIAN_POINT('Ctrl Pts',(-70.2273706284472,20.9431774823831,
0.));
#147534=CARTESIAN_POINT('Ctrl Pts',(-70.2273706284472,20.9431774823831,
12.));
#147535=CARTESIAN_POINT('Ctrl Pts',(-70.2070637255458,20.9266299391684,
0.));
#147536=CARTESIAN_POINT('Ctrl Pts',(-70.2070637255458,20.9266299391684,
12.));
#147537=CARTESIAN_POINT('Ctrl Pts',(-70.1867707089854,20.9101251488943,
0.));
#147538=CARTESIAN_POINT('Ctrl Pts',(-70.1867707089854,20.9101251488943,
12.));
#147539=CARTESIAN_POINT('Ctrl Pts',(-70.1664916860358,20.8936631331748,
0.));
#147540=CARTESIAN_POINT('Ctrl Pts',(-70.1664916860358,20.8936631331748,
12.));
#147541=CARTESIAN_POINT('Ctrl Pts',(-70.1462267643647,20.8772439136206,
0.));
#147542=CARTESIAN_POINT('Ctrl Pts',(-70.1462267643647,20.8772439136206,
12.));
#147543=CARTESIAN_POINT('Ctrl Pts',(-70.1259760520309,20.8608675118378,
0.));
#147544=CARTESIAN_POINT('Ctrl Pts',(-70.1259760520309,20.8608675118378,
12.));
#147545=CARTESIAN_POINT('Ctrl Pts',(-70.1057396574747,20.8445339494187,
0.));
#147546=CARTESIAN_POINT('Ctrl Pts',(-70.1057396574747,20.8445339494187,
12.));
#147547=CARTESIAN_POINT('Ctrl Pts',(-70.0855176895191,20.8282432479428,
0.));
#147548=CARTESIAN_POINT('Ctrl Pts',(-70.0855176895191,20.8282432479428,
12.));
#147549=CARTESIAN_POINT('Ctrl Pts',(-70.0653102573803,20.8119954289848,
0.));
#147550=CARTESIAN_POINT('Ctrl Pts',(-70.0653102573803,20.8119954289848,
12.));
#147551=CARTESIAN_POINT('Ctrl Pts',(-70.0451174706741,20.7957905141156,
0.));
#147552=CARTESIAN_POINT('Ctrl Pts',(-70.0451174706741,20.7957905141156,
12.));
#147553=CARTESIAN_POINT('Ctrl Pts',(-70.024939439422,20.7796285249022,0.));
#147554=CARTESIAN_POINT('Ctrl Pts',(-70.024939439422,20.7796285249022,12.));
#147555=CARTESIAN_POINT('Ctrl Pts',(-70.0047762740568,20.7635094829015,
0.));
#147556=CARTESIAN_POINT('Ctrl Pts',(-70.0047762740568,20.7635094829015,
12.));
#147557=CARTESIAN_POINT('Ctrl Pts',(-69.9846280854257,20.7474334096581,
0.));
#147558=CARTESIAN_POINT('Ctrl Pts',(-69.9846280854257,20.7474334096581,
12.));
#147559=CARTESIAN_POINT('Ctrl Pts',(-69.9644949847934,20.7314003267119,
0.));
#147560=CARTESIAN_POINT('Ctrl Pts',(-69.9644949847934,20.7314003267119,
12.));
#147561=CARTESIAN_POINT('Ctrl Pts',(-69.9443770838448,20.7154102555997,
0.));
#147562=CARTESIAN_POINT('Ctrl Pts',(-69.9443770838448,20.7154102555997,
12.));
#147563=CARTESIAN_POINT('Ctrl Pts',(-69.9242744946854,20.6994632178551,
0.));
#147564=CARTESIAN_POINT('Ctrl Pts',(-69.9242744946854,20.6994632178551,
12.));
#147565=CARTESIAN_POINT('Ctrl Pts',(-69.904187329841,20.683559235003,0.));
#147566=CARTESIAN_POINT('Ctrl Pts',(-69.904187329841,20.683559235003,12.));
#147567=CARTESIAN_POINT('Ctrl Pts',(-69.8841157022568,20.667698328554,0.));
#147568=CARTESIAN_POINT('Ctrl Pts',(-69.8841157022568,20.667698328554,12.));
#147569=CARTESIAN_POINT('Ctrl Pts',(-69.8640597253045,20.6518805200129,
0.));
#147570=CARTESIAN_POINT('Ctrl Pts',(-69.8640597253045,20.6518805200129,
12.));
#147571=CARTESIAN_POINT('Ctrl Pts',(-69.8440195127866,20.636105830881,0.));
#147572=CARTESIAN_POINT('Ctrl Pts',(-69.8440195127866,20.636105830881,12.));
#147573=CARTESIAN_POINT('Ctrl Pts',(-69.8239951789402,20.6203742826566,
0.));
#147574=CARTESIAN_POINT('Ctrl Pts',(-69.8239951789402,20.6203742826566,
12.));
#147575=CARTESIAN_POINT('Ctrl Pts',(-69.8039868384389,20.6046858968307,
0.));
#147576=CARTESIAN_POINT('Ctrl Pts',(-69.8039868384389,20.6046858968307,
12.));
#147577=CARTESIAN_POINT('Ctrl Pts',(-69.7839946063949,20.5890406948811,
0.));
#147578=CARTESIAN_POINT('Ctrl Pts',(-69.7839946063949,20.5890406948811,
12.));
#147579=CARTESIAN_POINT('Ctrl Pts',(-69.7640185983644,20.5734386982782,
0.));
#147580=CARTESIAN_POINT('Ctrl Pts',(-69.7640185983644,20.5734386982782,
12.));
#147581=CARTESIAN_POINT('Ctrl Pts',(-69.744058930351,20.5578799284897,0.));
#147582=CARTESIAN_POINT('Ctrl Pts',(-69.744058930351,20.5578799284897,12.));
#147583=CARTESIAN_POINT('Ctrl Pts',(-69.7241157188083,20.5423644069799,
0.));
#147584=CARTESIAN_POINT('Ctrl Pts',(-69.7241157188083,20.5423644069799,
12.));
#147585=CARTESIAN_POINT('Ctrl Pts',(-69.7041890806425,20.5268921552077,
0.));
#147586=CARTESIAN_POINT('Ctrl Pts',(-69.7041890806425,20.5268921552077,
12.));
#147587=CARTESIAN_POINT('Ctrl Pts',(-69.6842791332115,20.5114631946184,
0.));
#147588=CARTESIAN_POINT('Ctrl Pts',(-69.6842791332115,20.5114631946184,
12.));
#147589=CARTESIAN_POINT('Ctrl Pts',(-69.6643859943308,20.4960775466492,
0.));
#147590=CARTESIAN_POINT('Ctrl Pts',(-69.6643859943308,20.4960775466492,
12.));
#147591=CARTESIAN_POINT('Ctrl Pts',(-69.6445097822792,20.480735232734,0.));
#147592=CARTESIAN_POINT('Ctrl Pts',(-69.6445097822792,20.480735232734,12.));
#147593=CARTESIAN_POINT('Ctrl Pts',(-69.6246506158013,20.4654362743037,
0.));
#147594=CARTESIAN_POINT('Ctrl Pts',(-69.6246506158013,20.4654362743037,
12.));
#147595=CARTESIAN_POINT('Ctrl Pts',(-69.6048086141113,20.4501806927851,
0.));
#147596=CARTESIAN_POINT('Ctrl Pts',(-69.6048086141113,20.4501806927851,
12.));
#147597=CARTESIAN_POINT('Ctrl Pts',(-69.5849838968928,20.4349685095923,
0.));
#147598=CARTESIAN_POINT('Ctrl Pts',(-69.5849838968928,20.4349685095923,
12.));
#147599=CARTESIAN_POINT('Ctrl Pts',(-69.5651765843033,20.41979974613,0.));
#147600=CARTESIAN_POINT('Ctrl Pts',(-69.5651765843033,20.41979974613,12.));
#147601=CARTESIAN_POINT('Ctrl Pts',(-69.5453867969804,20.4046744237999,
0.));
#147602=CARTESIAN_POINT('Ctrl Pts',(-69.5453867969804,20.4046744237999,
12.));
#147603=CARTESIAN_POINT('Ctrl Pts',(-69.5256146560441,20.3895925640005,
0.));
#147604=CARTESIAN_POINT('Ctrl Pts',(-69.5256146560441,20.3895925640005,
12.));
#147605=CARTESIAN_POINT('Ctrl Pts',(-69.5058602831008,20.3745541881268,
0.));
#147606=CARTESIAN_POINT('Ctrl Pts',(-69.5058602831008,20.3745541881268,
12.));
#147607=CARTESIAN_POINT('Ctrl Pts',(-69.4861238002441,20.3595593175623,
0.));
#147608=CARTESIAN_POINT('Ctrl Pts',(-69.4861238002441,20.3595593175623,
12.));
#147609=CARTESIAN_POINT('Ctrl Pts',(-69.4664053300587,20.3446079736802,
0.));
#147610=CARTESIAN_POINT('Ctrl Pts',(-69.4664053300587,20.3446079736802,
12.));
#147611=CARTESIAN_POINT('Ctrl Pts',(-69.4467049956262,20.3297001778507,
0.));
#147612=CARTESIAN_POINT('Ctrl Pts',(-69.4467049956262,20.3297001778507,
12.));
#147613=CARTESIAN_POINT('Ctrl Pts',(-69.4270229205297,20.3148359514415,
0.));
#147614=CARTESIAN_POINT('Ctrl Pts',(-69.4270229205297,20.3148359514415,
12.));
#147615=CARTESIAN_POINT('Ctrl Pts',(-69.407359228856,20.3000153158166,0.));
#147616=CARTESIAN_POINT('Ctrl Pts',(-69.407359228856,20.3000153158166,12.));
#147617=CARTESIAN_POINT('Ctrl Pts',(-69.3877140451975,20.2852382923299,
0.));
#147618=CARTESIAN_POINT('Ctrl Pts',(-69.3877140451975,20.2852382923299,
12.));
#147619=CARTESIAN_POINT('Ctrl Pts',(-69.368087494655,20.2705049023241,0.));
#147620=CARTESIAN_POINT('Ctrl Pts',(-69.368087494655,20.2705049023241,12.));
#147621=CARTESIAN_POINT('Ctrl Pts',(-69.3484797028458,20.2558151671391,
0.));
#147622=CARTESIAN_POINT('Ctrl Pts',(-69.3484797028458,20.2558151671391,
12.));
#147623=CARTESIAN_POINT('Ctrl Pts',(-69.3288907959067,20.2411691081123,
0.));
#147624=CARTESIAN_POINT('Ctrl Pts',(-69.3288907959067,20.2411691081123,
12.));
#147625=CARTESIAN_POINT('Ctrl Pts',(-69.3093209004984,20.2265667465784,
0.));
#147626=CARTESIAN_POINT('Ctrl Pts',(-69.3093209004984,20.2265667465784,
12.));
#147627=CARTESIAN_POINT('Ctrl Pts',(-69.2897701438059,20.212008103862,0.));
#147628=CARTESIAN_POINT('Ctrl Pts',(-69.2897701438059,20.212008103862,12.));
#147629=CARTESIAN_POINT('Ctrl Pts',(-69.2702386535422,20.1974932012773,
0.));
#147630=CARTESIAN_POINT('Ctrl Pts',(-69.2702386535422,20.1974932012773,
12.));
#147631=CARTESIAN_POINT('Ctrl Pts',(-69.2507265579554,20.1830220601348,
0.));
#147632=CARTESIAN_POINT('Ctrl Pts',(-69.2507265579554,20.1830220601348,
12.));
#147633=CARTESIAN_POINT('Ctrl Pts',(-69.2312339858335,20.1685947017433,
0.));
#147634=CARTESIAN_POINT('Ctrl Pts',(-69.2312339858335,20.1685947017433,
12.));
#147635=CARTESIAN_POINT('Ctrl Pts',(-69.2117610665076,20.1542111474087,
0.));
#147636=CARTESIAN_POINT('Ctrl Pts',(-69.2117610665076,20.1542111474087,
12.));
#147637=CARTESIAN_POINT('Ctrl Pts',(-69.1923079298538,20.1398714184279,
0.));
#147638=CARTESIAN_POINT('Ctrl Pts',(-69.1923079298538,20.1398714184279,
12.));
#147639=CARTESIAN_POINT('Ctrl Pts',(-69.1728747062963,20.1255755360872,
0.));
#147640=CARTESIAN_POINT('Ctrl Pts',(-69.1728747062963,20.1255755360872,
12.));
#147641=CARTESIAN_POINT('Ctrl Pts',(-69.1534615268153,20.1113235216694,
0.));
#147642=CARTESIAN_POINT('Ctrl Pts',(-69.1534615268153,20.1113235216694,
12.));
#147643=CARTESIAN_POINT('Ctrl Pts',(-69.1340685229515,20.0971153964557,
0.));
#147644=CARTESIAN_POINT('Ctrl Pts',(-69.1340685229515,20.0971153964557,
12.));
#147645=CARTESIAN_POINT('Ctrl Pts',(-69.1146958268104,20.0829511817251,
0.));
#147646=CARTESIAN_POINT('Ctrl Pts',(-69.1146958268104,20.0829511817251,
12.));
#147647=CARTESIAN_POINT('Ctrl Pts',(-69.095343571064,20.068830898748,0.));
#147648=CARTESIAN_POINT('Ctrl Pts',(-69.095343571064,20.068830898748,12.));
#147649=CARTESIAN_POINT('Ctrl Pts',(-69.0760118889535,20.0547545687842,
0.));
#147650=CARTESIAN_POINT('Ctrl Pts',(-69.0760118889535,20.0547545687842,
12.));
#147651=CARTESIAN_POINT('Ctrl Pts',(-69.0567009142978,20.0407222130905,
0.));
#147652=CARTESIAN_POINT('Ctrl Pts',(-69.0567009142978,20.0407222130905,
12.));
#147653=CARTESIAN_POINT('Ctrl Pts',(-69.0374107814984,20.0267338529223,
0.));
#147654=CARTESIAN_POINT('Ctrl Pts',(-69.0374107814984,20.0267338529223,
12.));
#147655=CARTESIAN_POINT('Ctrl Pts',(-69.0181416255431,20.0127895095326,
0.));
#147656=CARTESIAN_POINT('Ctrl Pts',(-69.0181416255431,20.0127895095326,
12.));
#147657=CARTESIAN_POINT('Ctrl Pts',(-68.9988935820084,19.9988892041666,
0.));
#147658=CARTESIAN_POINT('Ctrl Pts',(-68.9988935820084,19.9988892041666,
12.));
#147659=CARTESIAN_POINT('Ctrl Pts',(-68.9796667870638,19.9850329580591,
0.));
#147660=CARTESIAN_POINT('Ctrl Pts',(-68.9796667870638,19.9850329580591,
12.));
#147661=CARTESIAN_POINT('Ctrl Pts',(-68.9604613774802,19.9712207924428,
0.));
#147662=CARTESIAN_POINT('Ctrl Pts',(-68.9604613774802,19.9712207924428,
12.));
#147663=CARTESIAN_POINT('Ctrl Pts',(-68.9412774906333,19.9574527285488,
0.));
#147664=CARTESIAN_POINT('Ctrl Pts',(-68.9412774906333,19.9574527285488,
12.));
#147665=CARTESIAN_POINT('Ctrl Pts',(-68.9221152645095,19.9437287876066,
0.));
#147666=CARTESIAN_POINT('Ctrl Pts',(-68.9221152645095,19.9437287876066,
12.));
#147667=CARTESIAN_POINT('Ctrl Pts',(-68.9029748377067,19.9300489908374,
0.));
#147668=CARTESIAN_POINT('Ctrl Pts',(-68.9029748377067,19.9300489908374,
12.));
#147669=CARTESIAN_POINT('Ctrl Pts',(-68.8838563494393,19.9164133594525,
0.));
#147670=CARTESIAN_POINT('Ctrl Pts',(-68.8838563494393,19.9164133594525,
12.));
#147671=CARTESIAN_POINT('Ctrl Pts',(-68.8647599395469,19.9028219146618,
0.));
#147672=CARTESIAN_POINT('Ctrl Pts',(-68.8647599395469,19.9028219146618,
12.));
#147673=CARTESIAN_POINT('Ctrl Pts',(-68.8456857485002,19.8892746776739,
0.));
#147674=CARTESIAN_POINT('Ctrl Pts',(-68.8456857485002,19.8892746776739,
12.));
#147675=CARTESIAN_POINT('Ctrl Pts',(-68.8266339174056,19.8757716696965,
0.));
#147676=CARTESIAN_POINT('Ctrl Pts',(-68.8266339174056,19.8757716696965,
12.));
#147677=CARTESIAN_POINT('Ctrl Pts',(-68.8076045880065,19.8623129119293,
0.));
#147678=CARTESIAN_POINT('Ctrl Pts',(-68.8076045880065,19.8623129119293,
12.));
#147679=CARTESIAN_POINT('Ctrl Pts',(-68.7885979026879,19.8488984255627,
0.));
#147680=CARTESIAN_POINT('Ctrl Pts',(-68.7885979026879,19.8488984255627,
12.));
#147681=CARTESIAN_POINT('Ctrl Pts',(-68.7696140044851,19.8355282317858,
0.));
#147682=CARTESIAN_POINT('Ctrl Pts',(-68.7696140044851,19.8355282317858,
12.));
#147683=CARTESIAN_POINT('Ctrl Pts',(-68.7506530370904,19.822202351787,0.));
#147684=CARTESIAN_POINT('Ctrl Pts',(-68.7506530370904,19.822202351787,12.));
#147685=CARTESIAN_POINT('Ctrl Pts',(-68.7317151448573,19.8089208067537,
0.));
#147686=CARTESIAN_POINT('Ctrl Pts',(-68.7317151448573,19.8089208067537,
12.));
#147687=CARTESIAN_POINT('Ctrl Pts',(-68.7128004728034,19.7956836178651,
0.));
#147688=CARTESIAN_POINT('Ctrl Pts',(-68.7128004728034,19.7956836178651,
12.));
#147689=CARTESIAN_POINT('Ctrl Pts',(-68.693909166615,19.7824908062924,0.));
#147690=CARTESIAN_POINT('Ctrl Pts',(-68.693909166615,19.7824908062924,12.));
#147691=CARTESIAN_POINT('Ctrl Pts',(-68.6750413726575,19.7693423932066,
0.));
#147692=CARTESIAN_POINT('Ctrl Pts',(-68.6750413726575,19.7693423932066,
12.));
#147693=CARTESIAN_POINT('Ctrl Pts',(-68.65619723798,19.7562383997783,0.));
#147694=CARTESIAN_POINT('Ctrl Pts',(-68.65619723798,19.7562383997783,12.));
#147695=CARTESIAN_POINT('Ctrl Pts',(-68.6373769103211,19.7431788471772,
0.));
#147696=CARTESIAN_POINT('Ctrl Pts',(-68.6373769103211,19.7431788471772,
12.));
#147697=CARTESIAN_POINT('Ctrl Pts',(-68.6185805381102,19.7301637565645,
0.));
#147698=CARTESIAN_POINT('Ctrl Pts',(-68.6185805381102,19.7301637565645,
12.));
#147699=CARTESIAN_POINT('Ctrl Pts',(-68.5998082704741,19.717193149095,0.));
#147700=CARTESIAN_POINT('Ctrl Pts',(-68.5998082704741,19.717193149095,12.));
#147701=CARTESIAN_POINT('Ctrl Pts',(-68.5810602572474,19.7042670459233,
0.));
#147702=CARTESIAN_POINT('Ctrl Pts',(-68.5810602572474,19.7042670459233,
12.));
#147703=CARTESIAN_POINT('Ctrl Pts',(-68.5623366489776,19.6913854682046,
0.));
#147704=CARTESIAN_POINT('Ctrl Pts',(-68.5623366489776,19.6913854682046,
12.));
#147705=CARTESIAN_POINT('Ctrl Pts',(-68.543637596932,19.6785484370929,0.));
#147706=CARTESIAN_POINT('Ctrl Pts',(-68.543637596932,19.6785484370929,12.));
#147707=CARTESIAN_POINT('Ctrl Pts',(-68.5249632530994,19.665755973734,0.));
#147708=CARTESIAN_POINT('Ctrl Pts',(-68.5249632530994,19.665755973734,12.));
#147709=CARTESIAN_POINT('Ctrl Pts',(-68.5063137701986,19.6530080992689,
0.));
#147710=CARTESIAN_POINT('Ctrl Pts',(-68.5063137701986,19.6530080992689,
12.));
#147711=CARTESIAN_POINT('Ctrl Pts',(-68.4876893016863,19.6403048348396,
0.));
#147712=CARTESIAN_POINT('Ctrl Pts',(-68.4876893016863,19.6403048348396,
12.));
#147713=CARTESIAN_POINT('Ctrl Pts',(-68.4690900017631,19.6276462015888,
0.));
#147714=CARTESIAN_POINT('Ctrl Pts',(-68.4690900017631,19.6276462015888,
12.));
#147715=CARTESIAN_POINT('Ctrl Pts',(-68.4505160253777,19.6150322206577,
0.));
#147716=CARTESIAN_POINT('Ctrl Pts',(-68.4505160253777,19.6150322206577,
12.));
#147717=CARTESIAN_POINT('Ctrl Pts',(-68.4319675282273,19.6024629131785,
0.));
#147718=CARTESIAN_POINT('Ctrl Pts',(-68.4319675282273,19.6024629131785,
12.));
#147719=CARTESIAN_POINT('Ctrl Pts',(-68.4134446667695,19.5899383002803,
0.));
#147720=CARTESIAN_POINT('Ctrl Pts',(-68.4134446667695,19.5899383002803,
12.));
#147721=CARTESIAN_POINT('Ctrl Pts',(-68.3949475982334,19.5774584030938,
0.));
#147722=CARTESIAN_POINT('Ctrl Pts',(-68.3949475982334,19.5774584030938,
12.));
#147723=CARTESIAN_POINT('Ctrl Pts',(-68.3764764806287,19.5650232427516,
0.));
#147724=CARTESIAN_POINT('Ctrl Pts',(-68.3764764806287,19.5650232427516,
12.));
#147725=CARTESIAN_POINT('Ctrl Pts',(-68.3580314727522,19.5526328403851,
0.));
#147726=CARTESIAN_POINT('Ctrl Pts',(-68.3580314727522,19.5526328403851,
12.));
#147727=CARTESIAN_POINT('Ctrl Pts',(-68.3396127341937,19.540287217119,0.));
#147728=CARTESIAN_POINT('Ctrl Pts',(-68.3396127341937,19.540287217119,12.));
#147729=CARTESIAN_POINT('Ctrl Pts',(-68.3212204253416,19.5279863940772,
0.));
#147730=CARTESIAN_POINT('Ctrl Pts',(-68.3212204253416,19.5279863940772,
12.));
#147731=CARTESIAN_POINT('Ctrl Pts',(-68.3028547073862,19.5157303923855,
0.));
#147732=CARTESIAN_POINT('Ctrl Pts',(-68.3028547073862,19.5157303923855,
12.));
#147733=CARTESIAN_POINT('Ctrl Pts',(-68.2845157423234,19.5035192331706,
0.));
#147734=CARTESIAN_POINT('Ctrl Pts',(-68.2845157423234,19.5035192331706,
12.));
#147735=CARTESIAN_POINT('Ctrl Pts',(-68.2662036929531,19.4913529375545,
0.));
#147736=CARTESIAN_POINT('Ctrl Pts',(-68.2662036929531,19.4913529375545,
12.));
#147737=CARTESIAN_POINT('Ctrl Pts',(-68.2479187228815,19.4792315266505,
0.));
#147738=CARTESIAN_POINT('Ctrl Pts',(-68.2479187228815,19.4792315266505,
12.));
#147739=CARTESIAN_POINT('Ctrl Pts',(-68.2296609965461,19.4671550215724,
0.));
#147740=CARTESIAN_POINT('Ctrl Pts',(-68.2296609965461,19.4671550215724,
12.));
#147741=CARTESIAN_POINT('Ctrl Pts',(-68.2114306792366,19.4551234434383,
0.));
#147742=CARTESIAN_POINT('Ctrl Pts',(-68.2114306792366,19.4551234434383,
12.));
#147743=CARTESIAN_POINT('Ctrl Pts',(-68.1932279371121,19.4431368133718,
0.));
#147744=CARTESIAN_POINT('Ctrl Pts',(-68.1932279371121,19.4431368133718,
12.));
#147745=CARTESIAN_POINT('Ctrl Pts',(-68.1750529372211,19.4311951524977,
0.));
#147746=CARTESIAN_POINT('Ctrl Pts',(-68.1750529372211,19.4311951524977,
12.));
#147747=CARTESIAN_POINT('Ctrl Pts',(-68.1569058475026,19.419298481941,0.));
#147748=CARTESIAN_POINT('Ctrl Pts',(-68.1569058475026,19.419298481941,12.));
#147749=CARTESIAN_POINT('Ctrl Pts',(-68.1387868367668,19.4074468228293,
0.));
#147750=CARTESIAN_POINT('Ctrl Pts',(-68.1387868367668,19.4074468228293,
12.));
#147751=CARTESIAN_POINT('Ctrl Pts',(-68.1206960746763,19.3956401962893,
0.));
#147752=CARTESIAN_POINT('Ctrl Pts',(-68.1206960746763,19.3956401962893,
12.));
#147753=CARTESIAN_POINT('Ctrl Pts',(-68.1026337317298,19.3838786234425,
0.));
#147754=CARTESIAN_POINT('Ctrl Pts',(-68.1026337317298,19.3838786234425,
12.));
#147755=CARTESIAN_POINT('Ctrl Pts',(-68.0845999792274,19.372162125392,0.));
#147756=CARTESIAN_POINT('Ctrl Pts',(-68.0845999792274,19.372162125392,12.));
#147757=CARTESIAN_POINT('Ctrl Pts',(-68.0665949893222,19.3604907232322,
0.));
#147758=CARTESIAN_POINT('Ctrl Pts',(-68.0665949893222,19.3604907232322,
12.));
#147759=CARTESIAN_POINT('Ctrl Pts',(-68.0486189351027,19.3488644380646,
0.));
#147760=CARTESIAN_POINT('Ctrl Pts',(-68.0486189351027,19.3488644380646,
12.));
#147761=CARTESIAN_POINT('Ctrl Pts',(-68.0306719906636,19.3372832910076,
0.));
#147762=CARTESIAN_POINT('Ctrl Pts',(-68.0306719906636,19.3372832910076,
12.));
#147763=CARTESIAN_POINT('Ctrl Pts',(-68.0127543311761,19.3257473032031,
0.));
#147764=CARTESIAN_POINT('Ctrl Pts',(-68.0127543311761,19.3257473032031,
12.));
#147765=CARTESIAN_POINT('Ctrl Pts',(-67.9948661329592,19.3142564958195,
0.));
#147766=CARTESIAN_POINT('Ctrl Pts',(-67.9948661329592,19.3142564958195,
12.));
#147767=CARTESIAN_POINT('Ctrl Pts',(-67.977007573346,19.3028108900373,0.));
#147768=CARTESIAN_POINT('Ctrl Pts',(-67.977007573346,19.3028108900373,12.));
#147769=CARTESIAN_POINT('Ctrl Pts',(-67.959178830538,19.2914105070282,0.));
#147770=CARTESIAN_POINT('Ctrl Pts',(-67.959178830538,19.2914105070282,12.));
#147771=CARTESIAN_POINT('Ctrl Pts',(-67.9413800834798,19.2800553679362,
0.));
#147772=CARTESIAN_POINT('Ctrl Pts',(-67.9413800834798,19.2800553679362,
12.));
#147773=CARTESIAN_POINT('Ctrl Pts',(-67.9236115116781,19.2687454938448,
0.));
#147774=CARTESIAN_POINT('Ctrl Pts',(-67.9236115116781,19.2687454938448,
12.));
#147775=CARTESIAN_POINT('Ctrl Pts',(-67.9058732951822,19.2574809057705,
0.));
#147776=CARTESIAN_POINT('Ctrl Pts',(-67.9058732951822,19.2574809057705,
12.));
#147777=CARTESIAN_POINT('Ctrl Pts',(-67.8881656149983,19.2462616247287,
0.));
#147778=CARTESIAN_POINT('Ctrl Pts',(-67.8881656149983,19.2462616247287,
12.));
#147779=CARTESIAN_POINT('Ctrl Pts',(-67.8704886534555,19.2350876717877,
0.));
#147780=CARTESIAN_POINT('Ctrl Pts',(-67.8704886534555,19.2350876717877,
12.));
#147781=CARTESIAN_POINT('Ctrl Pts',(-67.852842594517,19.2239590681129,0.));
#147782=CARTESIAN_POINT('Ctrl Pts',(-67.852842594517,19.2239590681129,12.));
#147783=CARTESIAN_POINT('Ctrl Pts',(-67.8352276242856,19.2128758350336,
0.));
#147784=CARTESIAN_POINT('Ctrl Pts',(-67.8352276242856,19.2128758350336,
12.));
#147785=CARTESIAN_POINT('Ctrl Pts',(-67.817643930658,19.2018379939918,0.));
#147786=CARTESIAN_POINT('Ctrl Pts',(-67.817643930658,19.2018379939918,12.));
#147787=CARTESIAN_POINT('Ctrl Pts',(-67.8000917023896,19.1908455664089,
0.));
#147788=CARTESIAN_POINT('Ctrl Pts',(-67.8000917023896,19.1908455664089,
12.));
#147789=CARTESIAN_POINT('Ctrl Pts',(-67.7825711283092,19.1798985735687,
0.));
#147790=CARTESIAN_POINT('Ctrl Pts',(-67.7825711283092,19.1798985735687,
12.));
#147791=CARTESIAN_POINT('Ctrl Pts',(-67.7650823965156,19.1689970364958,
0.));
#147792=CARTESIAN_POINT('Ctrl Pts',(-67.7650823965156,19.1689970364958,
12.));
#147793=CARTESIAN_POINT('Ctrl Pts',(-67.7476256934493,19.1581409758112,
0.));
#147794=CARTESIAN_POINT('Ctrl Pts',(-67.7476256934493,19.1581409758112,
12.));
#147795=CARTESIAN_POINT('Ctrl Pts',(-67.730201205663,19.1473304119968,0.));
#147796=CARTESIAN_POINT('Ctrl Pts',(-67.730201205663,19.1473304119968,12.));
#147797=CARTESIAN_POINT('Ctrl Pts',(-67.7128091219372,19.1365653657097,
0.));
#147798=CARTESIAN_POINT('Ctrl Pts',(-67.7128091219372,19.1365653657097,
12.));
#147799=CARTESIAN_POINT('Ctrl Pts',(-67.6954496350053,19.1258458580343,
0.));
#147800=CARTESIAN_POINT('Ctrl Pts',(-67.6954496350053,19.1258458580343,
12.));
#147801=CARTESIAN_POINT('Ctrl Pts',(-67.6781229440535,19.115171910845,0.));
#147802=CARTESIAN_POINT('Ctrl Pts',(-67.6781229440535,19.115171910845,12.));
#147803=CARTESIAN_POINT('Ctrl Pts',(-67.6608292549412,19.1045435468344,
0.));
#147804=CARTESIAN_POINT('Ctrl Pts',(-67.6608292549412,19.1045435468344,
12.));
#147805=CARTESIAN_POINT('Ctrl Pts',(-67.6435687749803,19.0939607887491,
0.));
#147806=CARTESIAN_POINT('Ctrl Pts',(-67.6435687749803,19.0939607887491,
12.));
#147807=CARTESIAN_POINT('Ctrl Pts',(-67.6263417083414,19.0834236587115,
0.));
#147808=CARTESIAN_POINT('Ctrl Pts',(-67.6263417083414,19.0834236587115,
12.));
#147809=CARTESIAN_POINT('Ctrl Pts',(-67.6091482520558,19.0729321776286,
0.));
#147810=CARTESIAN_POINT('Ctrl Pts',(-67.6091482520558,19.0729321776286,
12.));
#147811=CARTESIAN_POINT('Ctrl Pts',(-67.5919885896278,19.0624863642425,
0.));
#147812=CARTESIAN_POINT('Ctrl Pts',(-67.5919885896278,19.0624863642425,
12.));
#147813=CARTESIAN_POINT('Ctrl Pts',(-67.5748628972035,19.0520862360413,
0.));
#147814=CARTESIAN_POINT('Ctrl Pts',(-67.5748628972035,19.0520862360413,
12.));
#147815=CARTESIAN_POINT('Ctrl Pts',(-67.5577713558248,19.0417318110721,
0.));
#147816=CARTESIAN_POINT('Ctrl Pts',(-67.5577713558248,19.0417318110721,
12.));
#147817=CARTESIAN_POINT('Ctrl Pts',(-67.5407141612881,19.0314231093923,
0.));
#147818=CARTESIAN_POINT('Ctrl Pts',(-67.5407141612881,19.0314231093923,
12.));
#147819=CARTESIAN_POINT('Ctrl Pts',(-67.5236915360253,19.0211601548222,
0.));
#147820=CARTESIAN_POINT('Ctrl Pts',(-67.5236915360253,19.0211601548222,
12.));
#147821=CARTESIAN_POINT('Ctrl Pts',(-67.5067037372177,19.0109429761274,
0.));
#147822=CARTESIAN_POINT('Ctrl Pts',(-67.5067037372177,19.0109429761274,
12.));
#147823=CARTESIAN_POINT('Ctrl Pts',(-67.4897510316692,19.0007716032784,
0.));
#147824=CARTESIAN_POINT('Ctrl Pts',(-67.4897510316692,19.0007716032784,
12.));
#147825=CARTESIAN_POINT('Ctrl Pts',(-67.4728336719559,18.9906460638607,
0.));
#147826=CARTESIAN_POINT('Ctrl Pts',(-67.4728336719559,18.9906460638607,
12.));
#147827=CARTESIAN_POINT('Ctrl Pts',(-67.4559518744714,18.9805663798466,
0.));
#147828=CARTESIAN_POINT('Ctrl Pts',(-67.4559518744714,18.9805663798466,
12.));
#147829=CARTESIAN_POINT('Ctrl Pts',(-67.4391057908687,18.9705325631772,
0.));
#147830=CARTESIAN_POINT('Ctrl Pts',(-67.4391057908687,18.9705325631772,
12.));
#147831=CARTESIAN_POINT('Ctrl Pts',(-67.4222955062385,18.9605446161078,
0.));
#147832=CARTESIAN_POINT('Ctrl Pts',(-67.4222955062385,18.9605446161078,
12.));
#147833=CARTESIAN_POINT('Ctrl Pts',(-67.4088759498287,18.9525909518002,
0.));
#147834=CARTESIAN_POINT('Ctrl Pts',(-67.4088759498287,18.9525909518002,
12.));
#147835=CARTESIAN_POINT('Ctrl Pts',(-67.398827414689,18.9466463414354,0.));
#147836=CARTESIAN_POINT('Ctrl Pts',(-67.398827414689,18.9466463414354,12.));
#147837=CARTESIAN_POINT('Ctrl Pts',(-67.3921355608417,18.942692439874,0.));
#147838=CARTESIAN_POINT('Ctrl Pts',(-67.3921355608417,18.942692439874,12.));
#147839=CARTESIAN_POINT('Ctrl Pts',(-67.3887914263119,18.9407177820969,
0.));
#147840=CARTESIAN_POINT('Ctrl Pts',(-67.3887914263119,18.9407177820969,
12.));
#147841=CARTESIAN_POINT('',(-67.3887914263119,18.9407177820969,12.));
#147842=CARTESIAN_POINT('Ctrl Pts',(-67.3887914263119,18.9407177820969,
12.));
#147843=CARTESIAN_POINT('Ctrl Pts',(-67.3921355608417,18.942692439874,12.));
#147844=CARTESIAN_POINT('Ctrl Pts',(-67.398827414689,18.9466463414354,12.));
#147845=CARTESIAN_POINT('Ctrl Pts',(-67.4088759498287,18.9525909518002,
12.));
#147846=CARTESIAN_POINT('Ctrl Pts',(-67.4222955062385,18.9605446161078,
12.));
#147847=CARTESIAN_POINT('Ctrl Pts',(-67.4391057908687,18.9705325631772,
12.));
#147848=CARTESIAN_POINT('Ctrl Pts',(-67.4559518744714,18.9805663798466,
12.));
#147849=CARTESIAN_POINT('Ctrl Pts',(-67.4728336719559,18.9906460638607,
12.));
#147850=CARTESIAN_POINT('Ctrl Pts',(-67.4897510316692,19.0007716032784,
12.));
#147851=CARTESIAN_POINT('Ctrl Pts',(-67.5067037372177,19.0109429761274,
12.));
#147852=CARTESIAN_POINT('Ctrl Pts',(-67.5236915360253,19.0211601548222,
12.));
#147853=CARTESIAN_POINT('Ctrl Pts',(-67.5407141612881,19.0314231093923,
12.));
#147854=CARTESIAN_POINT('Ctrl Pts',(-67.5577713558248,19.0417318110721,
12.));
#147855=CARTESIAN_POINT('Ctrl Pts',(-67.5748628972035,19.0520862360413,
12.));
#147856=CARTESIAN_POINT('Ctrl Pts',(-67.5919885896278,19.0624863642425,
12.));
#147857=CARTESIAN_POINT('Ctrl Pts',(-67.6091482520558,19.0729321776286,
12.));
#147858=CARTESIAN_POINT('Ctrl Pts',(-67.6263417083414,19.0834236587115,
12.));
#147859=CARTESIAN_POINT('Ctrl Pts',(-67.6435687749803,19.0939607887491,
12.));
#147860=CARTESIAN_POINT('Ctrl Pts',(-67.6608292549412,19.1045435468344,
12.));
#147861=CARTESIAN_POINT('Ctrl Pts',(-67.6781229440535,19.115171910845,12.));
#147862=CARTESIAN_POINT('Ctrl Pts',(-67.6954496350053,19.1258458580343,
12.));
#147863=CARTESIAN_POINT('Ctrl Pts',(-67.7128091219372,19.1365653657097,
12.));
#147864=CARTESIAN_POINT('Ctrl Pts',(-67.730201205663,19.1473304119968,12.));
#147865=CARTESIAN_POINT('Ctrl Pts',(-67.7476256934493,19.1581409758112,
12.));
#147866=CARTESIAN_POINT('Ctrl Pts',(-67.7650823965156,19.1689970364958,
12.));
#147867=CARTESIAN_POINT('Ctrl Pts',(-67.7825711283092,19.1798985735687,
12.));
#147868=CARTESIAN_POINT('Ctrl Pts',(-67.8000917023896,19.1908455664089,
12.));
#147869=CARTESIAN_POINT('Ctrl Pts',(-67.817643930658,19.2018379939918,12.));
#147870=CARTESIAN_POINT('Ctrl Pts',(-67.8352276242856,19.2128758350336,
12.));
#147871=CARTESIAN_POINT('Ctrl Pts',(-67.852842594517,19.2239590681129,12.));
#147872=CARTESIAN_POINT('Ctrl Pts',(-67.8704886534555,19.2350876717877,
12.));
#147873=CARTESIAN_POINT('Ctrl Pts',(-67.8881656149983,19.2462616247287,
12.));
#147874=CARTESIAN_POINT('Ctrl Pts',(-67.9058732951822,19.2574809057705,
12.));
#147875=CARTESIAN_POINT('Ctrl Pts',(-67.9236115116781,19.2687454938448,
12.));
#147876=CARTESIAN_POINT('Ctrl Pts',(-67.9413800834798,19.2800553679362,
12.));
#147877=CARTESIAN_POINT('Ctrl Pts',(-67.959178830538,19.2914105070282,12.));
#147878=CARTESIAN_POINT('Ctrl Pts',(-67.977007573346,19.3028108900373,12.));
#147879=CARTESIAN_POINT('Ctrl Pts',(-67.9948661329592,19.3142564958195,
12.));
#147880=CARTESIAN_POINT('Ctrl Pts',(-68.0127543311761,19.3257473032031,
12.));
#147881=CARTESIAN_POINT('Ctrl Pts',(-68.0306719906636,19.3372832910076,
12.));
#147882=CARTESIAN_POINT('Ctrl Pts',(-68.0486189351027,19.3488644380646,
12.));
#147883=CARTESIAN_POINT('Ctrl Pts',(-68.0665949893222,19.3604907232322,
12.));
#147884=CARTESIAN_POINT('Ctrl Pts',(-68.0845999792274,19.372162125392,12.));
#147885=CARTESIAN_POINT('Ctrl Pts',(-68.1026337317298,19.3838786234425,
12.));
#147886=CARTESIAN_POINT('Ctrl Pts',(-68.1206960746763,19.3956401962893,
12.));
#147887=CARTESIAN_POINT('Ctrl Pts',(-68.1387868367668,19.4074468228293,
12.));
#147888=CARTESIAN_POINT('Ctrl Pts',(-68.1569058475026,19.419298481941,12.));
#147889=CARTESIAN_POINT('Ctrl Pts',(-68.1750529372211,19.4311951524977,
12.));
#147890=CARTESIAN_POINT('Ctrl Pts',(-68.1932279371121,19.4431368133718,
12.));
#147891=CARTESIAN_POINT('Ctrl Pts',(-68.2114306792366,19.4551234434383,
12.));
#147892=CARTESIAN_POINT('Ctrl Pts',(-68.2296609965461,19.4671550215724,
12.));
#147893=CARTESIAN_POINT('Ctrl Pts',(-68.2479187228815,19.4792315266505,
12.));
#147894=CARTESIAN_POINT('Ctrl Pts',(-68.2662036929531,19.4913529375545,
12.));
#147895=CARTESIAN_POINT('Ctrl Pts',(-68.2845157423234,19.5035192331706,
12.));
#147896=CARTESIAN_POINT('Ctrl Pts',(-68.3028547073862,19.5157303923855,
12.));
#147897=CARTESIAN_POINT('Ctrl Pts',(-68.3212204253416,19.5279863940772,
12.));
#147898=CARTESIAN_POINT('Ctrl Pts',(-68.3396127341937,19.540287217119,12.));
#147899=CARTESIAN_POINT('Ctrl Pts',(-68.3580314727522,19.5526328403851,
12.));
#147900=CARTESIAN_POINT('Ctrl Pts',(-68.3764764806287,19.5650232427516,
12.));
#147901=CARTESIAN_POINT('Ctrl Pts',(-68.3949475982334,19.5774584030938,
12.));
#147902=CARTESIAN_POINT('Ctrl Pts',(-68.4134446667695,19.5899383002803,
12.));
#147903=CARTESIAN_POINT('Ctrl Pts',(-68.4319675282273,19.6024629131785,
12.));
#147904=CARTESIAN_POINT('Ctrl Pts',(-68.4505160253777,19.6150322206577,
12.));
#147905=CARTESIAN_POINT('Ctrl Pts',(-68.4690900017631,19.6276462015888,
12.));
#147906=CARTESIAN_POINT('Ctrl Pts',(-68.4876893016863,19.6403048348396,
12.));
#147907=CARTESIAN_POINT('Ctrl Pts',(-68.5063137701986,19.6530080992689,
12.));
#147908=CARTESIAN_POINT('Ctrl Pts',(-68.5249632530994,19.665755973734,12.));
#147909=CARTESIAN_POINT('Ctrl Pts',(-68.543637596932,19.6785484370929,12.));
#147910=CARTESIAN_POINT('Ctrl Pts',(-68.5623366489776,19.6913854682046,
12.));
#147911=CARTESIAN_POINT('Ctrl Pts',(-68.5810602572474,19.7042670459233,
12.));
#147912=CARTESIAN_POINT('Ctrl Pts',(-68.5998082704741,19.717193149095,12.));
#147913=CARTESIAN_POINT('Ctrl Pts',(-68.6185805381102,19.7301637565645,
12.));
#147914=CARTESIAN_POINT('Ctrl Pts',(-68.6373769103211,19.7431788471772,
12.));
#147915=CARTESIAN_POINT('Ctrl Pts',(-68.65619723798,19.7562383997783,12.));
#147916=CARTESIAN_POINT('Ctrl Pts',(-68.6750413726575,19.7693423932066,
12.));
#147917=CARTESIAN_POINT('Ctrl Pts',(-68.693909166615,19.7824908062924,12.));
#147918=CARTESIAN_POINT('Ctrl Pts',(-68.7128004728034,19.7956836178651,
12.));
#147919=CARTESIAN_POINT('Ctrl Pts',(-68.7317151448573,19.8089208067537,
12.));
#147920=CARTESIAN_POINT('Ctrl Pts',(-68.7506530370904,19.822202351787,12.));
#147921=CARTESIAN_POINT('Ctrl Pts',(-68.7696140044851,19.8355282317858,
12.));
#147922=CARTESIAN_POINT('Ctrl Pts',(-68.7885979026879,19.8488984255627,
12.));
#147923=CARTESIAN_POINT('Ctrl Pts',(-68.8076045880065,19.8623129119293,
12.));
#147924=CARTESIAN_POINT('Ctrl Pts',(-68.8266339174056,19.8757716696965,
12.));
#147925=CARTESIAN_POINT('Ctrl Pts',(-68.8456857485002,19.8892746776739,
12.));
#147926=CARTESIAN_POINT('Ctrl Pts',(-68.8647599395469,19.9028219146618,
12.));
#147927=CARTESIAN_POINT('Ctrl Pts',(-68.8838563494393,19.9164133594525,
12.));
#147928=CARTESIAN_POINT('Ctrl Pts',(-68.9029748377067,19.9300489908374,
12.));
#147929=CARTESIAN_POINT('Ctrl Pts',(-68.9221152645095,19.9437287876066,
12.));
#147930=CARTESIAN_POINT('Ctrl Pts',(-68.9412774906333,19.9574527285488,
12.));
#147931=CARTESIAN_POINT('Ctrl Pts',(-68.9604613774802,19.9712207924428,
12.));
#147932=CARTESIAN_POINT('Ctrl Pts',(-68.9796667870638,19.9850329580591,
12.));
#147933=CARTESIAN_POINT('Ctrl Pts',(-68.9988935820084,19.9988892041666,
12.));
#147934=CARTESIAN_POINT('Ctrl Pts',(-69.0181416255431,20.0127895095326,
12.));
#147935=CARTESIAN_POINT('Ctrl Pts',(-69.0374107814984,20.0267338529223,
12.));
#147936=CARTESIAN_POINT('Ctrl Pts',(-69.0567009142978,20.0407222130905,
12.));
#147937=CARTESIAN_POINT('Ctrl Pts',(-69.0760118889535,20.0547545687842,
12.));
#147938=CARTESIAN_POINT('Ctrl Pts',(-69.095343571064,20.068830898748,12.));
#147939=CARTESIAN_POINT('Ctrl Pts',(-69.1146958268104,20.0829511817251,
12.));
#147940=CARTESIAN_POINT('Ctrl Pts',(-69.1340685229515,20.0971153964557,
12.));
#147941=CARTESIAN_POINT('Ctrl Pts',(-69.1534615268153,20.1113235216694,
12.));
#147942=CARTESIAN_POINT('Ctrl Pts',(-69.1728747062963,20.1255755360872,
12.));
#147943=CARTESIAN_POINT('Ctrl Pts',(-69.1923079298538,20.1398714184279,
12.));
#147944=CARTESIAN_POINT('Ctrl Pts',(-69.2117610665076,20.1542111474087,
12.));
#147945=CARTESIAN_POINT('Ctrl Pts',(-69.2312339858335,20.1685947017433,
12.));
#147946=CARTESIAN_POINT('Ctrl Pts',(-69.2507265579554,20.1830220601348,
12.));
#147947=CARTESIAN_POINT('Ctrl Pts',(-69.2702386535422,20.1974932012773,
12.));
#147948=CARTESIAN_POINT('Ctrl Pts',(-69.2897701438059,20.212008103862,12.));
#147949=CARTESIAN_POINT('Ctrl Pts',(-69.3093209004984,20.2265667465784,
12.));
#147950=CARTESIAN_POINT('Ctrl Pts',(-69.3288907959067,20.2411691081123,
12.));
#147951=CARTESIAN_POINT('Ctrl Pts',(-69.3484797028458,20.2558151671391,
12.));
#147952=CARTESIAN_POINT('Ctrl Pts',(-69.368087494655,20.2705049023241,12.));
#147953=CARTESIAN_POINT('Ctrl Pts',(-69.3877140451975,20.2852382923299,
12.));
#147954=CARTESIAN_POINT('Ctrl Pts',(-69.407359228856,20.3000153158166,12.));
#147955=CARTESIAN_POINT('Ctrl Pts',(-69.4270229205297,20.3148359514415,
12.));
#147956=CARTESIAN_POINT('Ctrl Pts',(-69.4467049956262,20.3297001778507,
12.));
#147957=CARTESIAN_POINT('Ctrl Pts',(-69.4664053300587,20.3446079736802,
12.));
#147958=CARTESIAN_POINT('Ctrl Pts',(-69.4861238002441,20.3595593175623,
12.));
#147959=CARTESIAN_POINT('Ctrl Pts',(-69.5058602831008,20.3745541881268,
12.));
#147960=CARTESIAN_POINT('Ctrl Pts',(-69.5256146560441,20.3895925640005,
12.));
#147961=CARTESIAN_POINT('Ctrl Pts',(-69.5453867969804,20.4046744237999,
12.));
#147962=CARTESIAN_POINT('Ctrl Pts',(-69.5651765843033,20.41979974613,12.));
#147963=CARTESIAN_POINT('Ctrl Pts',(-69.5849838968928,20.4349685095923,
12.));
#147964=CARTESIAN_POINT('Ctrl Pts',(-69.6048086141113,20.4501806927851,
12.));
#147965=CARTESIAN_POINT('Ctrl Pts',(-69.6246506158013,20.4654362743037,
12.));
#147966=CARTESIAN_POINT('Ctrl Pts',(-69.6445097822792,20.480735232734,12.));
#147967=CARTESIAN_POINT('Ctrl Pts',(-69.6643859943308,20.4960775466492,
12.));
#147968=CARTESIAN_POINT('Ctrl Pts',(-69.6842791332115,20.5114631946184,
12.));
#147969=CARTESIAN_POINT('Ctrl Pts',(-69.7041890806425,20.5268921552077,
12.));
#147970=CARTESIAN_POINT('Ctrl Pts',(-69.7241157188083,20.5423644069799,
12.));
#147971=CARTESIAN_POINT('Ctrl Pts',(-69.744058930351,20.5578799284897,12.));
#147972=CARTESIAN_POINT('Ctrl Pts',(-69.7640185983644,20.5734386982782,
12.));
#147973=CARTESIAN_POINT('Ctrl Pts',(-69.7839946063949,20.5890406948811,
12.));
#147974=CARTESIAN_POINT('Ctrl Pts',(-69.8039868384389,20.6046858968307,
12.));
#147975=CARTESIAN_POINT('Ctrl Pts',(-69.8239951789402,20.6203742826566,
12.));
#147976=CARTESIAN_POINT('Ctrl Pts',(-69.8440195127866,20.636105830881,12.));
#147977=CARTESIAN_POINT('Ctrl Pts',(-69.8640597253045,20.6518805200129,
12.));
#147978=CARTESIAN_POINT('Ctrl Pts',(-69.8841157022568,20.667698328554,12.));
#147979=CARTESIAN_POINT('Ctrl Pts',(-69.904187329841,20.683559235003,12.));
#147980=CARTESIAN_POINT('Ctrl Pts',(-69.9242744946854,20.6994632178551,
12.));
#147981=CARTESIAN_POINT('Ctrl Pts',(-69.9443770838448,20.7154102555997,
12.));
#147982=CARTESIAN_POINT('Ctrl Pts',(-69.9644949847934,20.7314003267119,
12.));
#147983=CARTESIAN_POINT('Ctrl Pts',(-69.9846280854257,20.7474334096581,
12.));
#147984=CARTESIAN_POINT('Ctrl Pts',(-70.0047762740568,20.7635094829015,
12.));
#147985=CARTESIAN_POINT('Ctrl Pts',(-70.024939439422,20.7796285249022,12.));
#147986=CARTESIAN_POINT('Ctrl Pts',(-70.0451174706741,20.7957905141156,
12.));
#147987=CARTESIAN_POINT('Ctrl Pts',(-70.0653102573803,20.8119954289848,
12.));
#147988=CARTESIAN_POINT('Ctrl Pts',(-70.0855176895191,20.8282432479428,
12.));
#147989=CARTESIAN_POINT('Ctrl Pts',(-70.1057396574747,20.8445339494187,
12.));
#147990=CARTESIAN_POINT('Ctrl Pts',(-70.1259760520309,20.8608675118378,
12.));
#147991=CARTESIAN_POINT('Ctrl Pts',(-70.1462267643647,20.8772439136206,
12.));
#147992=CARTESIAN_POINT('Ctrl Pts',(-70.1664916860358,20.8936631331748,
12.));
#147993=CARTESIAN_POINT('Ctrl Pts',(-70.1867707089854,20.9101251488943,
12.));
#147994=CARTESIAN_POINT('Ctrl Pts',(-70.2070637255458,20.9266299391684,
12.));
#147995=CARTESIAN_POINT('Ctrl Pts',(-70.2273706284472,20.9431774823831,
12.));
#147996=CARTESIAN_POINT('Ctrl Pts',(-70.2476913108244,20.9597677569228,
12.));
#147997=CARTESIAN_POINT('Ctrl Pts',(-70.2680256662224,20.9764007411652,
12.));
#147998=CARTESIAN_POINT('Ctrl Pts',(-70.2883735885984,20.9930764134776,
12.));
#147999=CARTESIAN_POINT('Ctrl Pts',(-70.3087349722973,21.0097947522218,
12.));
#148000=CARTESIAN_POINT('Ctrl Pts',(-70.3291097120302,21.0265557357548,
12.));
#148001=CARTESIAN_POINT('Ctrl Pts',(-70.3494977028498,21.0433593424266,
12.));
#148002=CARTESIAN_POINT('Ctrl Pts',(-70.3698988401281,21.0602055505748,
12.));
#148003=CARTESIAN_POINT('Ctrl Pts',(-70.3903130195265,21.0770943385141,
12.));
#148004=CARTESIAN_POINT('Ctrl Pts',(-70.4107401370389,21.0940256845472,
12.));
#148005=CARTESIAN_POINT('Ctrl Pts',(-70.4311800890402,21.1109995669747,
12.));
#148006=CARTESIAN_POINT('Ctrl Pts',(-70.4516327723346,21.1280159641002,
12.));
#148007=CARTESIAN_POINT('Ctrl Pts',(-70.4720980841939,21.1450748542336,
12.));
#148008=CARTESIAN_POINT('Ctrl Pts',(-70.4925759224216,21.1621762156897,
12.));
#148009=CARTESIAN_POINT('Ctrl Pts',(-70.5130661852955,21.1793200267846,
12.));
#148010=CARTESIAN_POINT('Ctrl Pts',(-70.5335687714429,21.1965062658298,
12.));
#148011=CARTESIAN_POINT('Ctrl Pts',(-70.5540835797283,21.2137349111208,
12.));
#148012=CARTESIAN_POINT('Ctrl Pts',(-70.5746105091502,21.2310059409265,
12.));
#148013=CARTESIAN_POINT('Ctrl Pts',(-70.5951494586957,21.2483193334675,
12.));
#148014=CARTESIAN_POINT('Ctrl Pts',(-70.6157003273316,21.2656750669126,
12.));
#148015=CARTESIAN_POINT('Ctrl Pts',(-70.6362630143047,21.2830731194183,
12.));
#148016=CARTESIAN_POINT('Ctrl Pts',(-70.6568374193774,21.300513469156,12.));
#148017=CARTESIAN_POINT('Ctrl Pts',(-70.6774234430897,21.3179960943388,
12.));
#148018=CARTESIAN_POINT('Ctrl Pts',(-70.6980209870045,21.3355209732443,
12.));
#148019=CARTESIAN_POINT('Ctrl Pts',(-70.7186299539724,21.3530880842349,
12.));
#148020=CARTESIAN_POINT('Ctrl Pts',(-70.7392502475469,21.3706974057039,
12.));
#148021=CARTESIAN_POINT('Ctrl Pts',(-70.7598817714105,21.3883489160196,
12.));
#148022=CARTESIAN_POINT('Ctrl Pts',(-70.780524428745,21.4060425934598,12.));
#148023=CARTESIAN_POINT('Ctrl Pts',(-70.8011781217394,21.4237784161587,
12.));
#148024=CARTESIAN_POINT('Ctrl Pts',(-70.8218427507506,21.4415563620114,
12.));
#148025=CARTESIAN_POINT('Ctrl Pts',(-70.8425182149846,21.4593764087473,
12.));
#148026=CARTESIAN_POINT('Ctrl Pts',(-70.8632044140112,21.477238534096,12.));
#148027=CARTESIAN_POINT('Ctrl Pts',(-70.8839012490871,21.4951427159261,
12.));
#148028=CARTESIAN_POINT('Ctrl Pts',(-70.9046086244131,21.513088932377,12.));
#148029=CARTESIAN_POINT('Ctrl Pts',(-70.9253264487637,21.531077162023,12.));
#148030=CARTESIAN_POINT('Ctrl Pts',(-70.94605463587,21.5491073839106,12.));
#148031=CARTESIAN_POINT('Ctrl Pts',(-70.9638315189817,21.5645987555369,
12.));
#148032=CARTESIAN_POINT('Ctrl Pts',(-70.9774662112587,21.576498336648,12.));
#148033=CARTESIAN_POINT('Ctrl Pts',(-70.9869541808053,21.584787543333,12.));
#148034=CARTESIAN_POINT('Ctrl Pts',(-70.9922924595366,21.5894540925581,
12.));
#148035=CARTESIAN_POINT('Ctrl Pts',(-70.9934796069113,21.5904919935059,
12.));
#148036=CARTESIAN_POINT('',(-67.3887914263119,18.9407177820969,0.));
#148037=CARTESIAN_POINT('',(-67.3887914263118,18.9407177820969,0.));
#148038=CARTESIAN_POINT('Ctrl Pts',(-70.9934796069113,21.5904919935059,
0.));
#148039=CARTESIAN_POINT('Ctrl Pts',(-70.9922924595366,21.5894540925581,
0.));
#148040=CARTESIAN_POINT('Ctrl Pts',(-70.9869541808053,21.584787543333,0.));
#148041=CARTESIAN_POINT('Ctrl Pts',(-70.9774662112587,21.576498336648,0.));
#148042=CARTESIAN_POINT('Ctrl Pts',(-70.9638315189817,21.5645987555369,
0.));
#148043=CARTESIAN_POINT('Ctrl Pts',(-70.94605463587,21.5491073839106,0.));
#148044=CARTESIAN_POINT('Ctrl Pts',(-70.9253264487637,21.531077162023,0.));
#148045=CARTESIAN_POINT('Ctrl Pts',(-70.9046086244131,21.513088932377,0.));
#148046=CARTESIAN_POINT('Ctrl Pts',(-70.8839012490871,21.4951427159261,
0.));
#148047=CARTESIAN_POINT('Ctrl Pts',(-70.8632044140112,21.477238534096,0.));
#148048=CARTESIAN_POINT('Ctrl Pts',(-70.8425182149846,21.4593764087473,
0.));
#148049=CARTESIAN_POINT('Ctrl Pts',(-70.8218427507506,21.4415563620114,
0.));
#148050=CARTESIAN_POINT('Ctrl Pts',(-70.8011781217394,21.4237784161587,
0.));
#148051=CARTESIAN_POINT('Ctrl Pts',(-70.780524428745,21.4060425934598,0.));
#148052=CARTESIAN_POINT('Ctrl Pts',(-70.7598817714105,21.3883489160196,
0.));
#148053=CARTESIAN_POINT('Ctrl Pts',(-70.7392502475469,21.3706974057039,
0.));
#148054=CARTESIAN_POINT('Ctrl Pts',(-70.7186299539724,21.3530880842349,
0.));
#148055=CARTESIAN_POINT('Ctrl Pts',(-70.6980209870045,21.3355209732443,
0.));
#148056=CARTESIAN_POINT('Ctrl Pts',(-70.6774234430897,21.3179960943388,
0.));
#148057=CARTESIAN_POINT('Ctrl Pts',(-70.6568374193774,21.300513469156,0.));
#148058=CARTESIAN_POINT('Ctrl Pts',(-70.6362630143047,21.2830731194183,
0.));
#148059=CARTESIAN_POINT('Ctrl Pts',(-70.6157003273316,21.2656750669126,
0.));
#148060=CARTESIAN_POINT('Ctrl Pts',(-70.5951494586957,21.2483193334675,
0.));
#148061=CARTESIAN_POINT('Ctrl Pts',(-70.5746105091502,21.2310059409265,
0.));
#148062=CARTESIAN_POINT('Ctrl Pts',(-70.5540835797283,21.2137349111208,
0.));
#148063=CARTESIAN_POINT('Ctrl Pts',(-70.5335687714429,21.1965062658298,
0.));
#148064=CARTESIAN_POINT('Ctrl Pts',(-70.5130661852955,21.1793200267846,
0.));
#148065=CARTESIAN_POINT('Ctrl Pts',(-70.4925759224216,21.1621762156897,
0.));
#148066=CARTESIAN_POINT('Ctrl Pts',(-70.4720980841939,21.1450748542336,
0.));
#148067=CARTESIAN_POINT('Ctrl Pts',(-70.4516327723346,21.1280159641002,
0.));
#148068=CARTESIAN_POINT('Ctrl Pts',(-70.4311800890402,21.1109995669747,
0.));
#148069=CARTESIAN_POINT('Ctrl Pts',(-70.4107401370389,21.0940256845472,
0.));
#148070=CARTESIAN_POINT('Ctrl Pts',(-70.3903130195265,21.0770943385141,
0.));
#148071=CARTESIAN_POINT('Ctrl Pts',(-70.3698988401281,21.0602055505748,
0.));
#148072=CARTESIAN_POINT('Ctrl Pts',(-70.3494977028498,21.0433593424266,
0.));
#148073=CARTESIAN_POINT('Ctrl Pts',(-70.3291097120302,21.0265557357548,
0.));
#148074=CARTESIAN_POINT('Ctrl Pts',(-70.3087349722973,21.0097947522218,
0.));
#148075=CARTESIAN_POINT('Ctrl Pts',(-70.2883735885984,20.9930764134776,
0.));
#148076=CARTESIAN_POINT('Ctrl Pts',(-70.2680256662224,20.9764007411652,
0.));
#148077=CARTESIAN_POINT('Ctrl Pts',(-70.2476913108244,20.9597677569228,
0.));
#148078=CARTESIAN_POINT('Ctrl Pts',(-70.2273706284472,20.9431774823831,
0.));
#148079=CARTESIAN_POINT('Ctrl Pts',(-70.2070637255458,20.9266299391684,
0.));
#148080=CARTESIAN_POINT('Ctrl Pts',(-70.1867707089854,20.9101251488943,
0.));
#148081=CARTESIAN_POINT('Ctrl Pts',(-70.1664916860358,20.8936631331748,
0.));
#148082=CARTESIAN_POINT('Ctrl Pts',(-70.1462267643647,20.8772439136206,
0.));
#148083=CARTESIAN_POINT('Ctrl Pts',(-70.1259760520309,20.8608675118378,
0.));
#148084=CARTESIAN_POINT('Ctrl Pts',(-70.1057396574747,20.8445339494187,
0.));
#148085=CARTESIAN_POINT('Ctrl Pts',(-70.0855176895191,20.8282432479428,
0.));
#148086=CARTESIAN_POINT('Ctrl Pts',(-70.0653102573803,20.8119954289848,
0.));
#148087=CARTESIAN_POINT('Ctrl Pts',(-70.0451174706741,20.7957905141156,
0.));
#148088=CARTESIAN_POINT('Ctrl Pts',(-70.024939439422,20.7796285249022,0.));
#148089=CARTESIAN_POINT('Ctrl Pts',(-70.0047762740568,20.7635094829015,
0.));
#148090=CARTESIAN_POINT('Ctrl Pts',(-69.9846280854257,20.7474334096581,
0.));
#148091=CARTESIAN_POINT('Ctrl Pts',(-69.9644949847934,20.7314003267119,
0.));
#148092=CARTESIAN_POINT('Ctrl Pts',(-69.9443770838448,20.7154102555997,
0.));
#148093=CARTESIAN_POINT('Ctrl Pts',(-69.9242744946854,20.6994632178551,
0.));
#148094=CARTESIAN_POINT('Ctrl Pts',(-69.904187329841,20.683559235003,0.));
#148095=CARTESIAN_POINT('Ctrl Pts',(-69.8841157022568,20.667698328554,0.));
#148096=CARTESIAN_POINT('Ctrl Pts',(-69.8640597253045,20.6518805200129,
0.));
#148097=CARTESIAN_POINT('Ctrl Pts',(-69.8440195127866,20.636105830881,0.));
#148098=CARTESIAN_POINT('Ctrl Pts',(-69.8239951789402,20.6203742826566,
0.));
#148099=CARTESIAN_POINT('Ctrl Pts',(-69.8039868384389,20.6046858968307,
0.));
#148100=CARTESIAN_POINT('Ctrl Pts',(-69.7839946063949,20.5890406948811,
0.));
#148101=CARTESIAN_POINT('Ctrl Pts',(-69.7640185983644,20.5734386982782,
0.));
#148102=CARTESIAN_POINT('Ctrl Pts',(-69.744058930351,20.5578799284897,0.));
#148103=CARTESIAN_POINT('Ctrl Pts',(-69.7241157188083,20.5423644069799,
0.));
#148104=CARTESIAN_POINT('Ctrl Pts',(-69.7041890806425,20.5268921552077,
0.));
#148105=CARTESIAN_POINT('Ctrl Pts',(-69.6842791332115,20.5114631946184,
0.));
#148106=CARTESIAN_POINT('Ctrl Pts',(-69.6643859943308,20.4960775466492,
0.));
#148107=CARTESIAN_POINT('Ctrl Pts',(-69.6445097822792,20.480735232734,0.));
#148108=CARTESIAN_POINT('Ctrl Pts',(-69.6246506158013,20.4654362743037,
0.));
#148109=CARTESIAN_POINT('Ctrl Pts',(-69.6048086141113,20.4501806927851,
0.));
#148110=CARTESIAN_POINT('Ctrl Pts',(-69.5849838968928,20.4349685095923,
0.));
#148111=CARTESIAN_POINT('Ctrl Pts',(-69.5651765843033,20.41979974613,0.));
#148112=CARTESIAN_POINT('Ctrl Pts',(-69.5453867969804,20.4046744237999,
0.));
#148113=CARTESIAN_POINT('Ctrl Pts',(-69.5256146560441,20.3895925640005,
0.));
#148114=CARTESIAN_POINT('Ctrl Pts',(-69.5058602831008,20.3745541881268,
0.));
#148115=CARTESIAN_POINT('Ctrl Pts',(-69.4861238002441,20.3595593175623,
0.));
#148116=CARTESIAN_POINT('Ctrl Pts',(-69.4664053300587,20.3446079736802,
0.));
#148117=CARTESIAN_POINT('Ctrl Pts',(-69.4467049956262,20.3297001778507,
0.));
#148118=CARTESIAN_POINT('Ctrl Pts',(-69.4270229205297,20.3148359514415,
0.));
#148119=CARTESIAN_POINT('Ctrl Pts',(-69.407359228856,20.3000153158166,0.));
#148120=CARTESIAN_POINT('Ctrl Pts',(-69.3877140451975,20.2852382923299,
0.));
#148121=CARTESIAN_POINT('Ctrl Pts',(-69.368087494655,20.2705049023241,0.));
#148122=CARTESIAN_POINT('Ctrl Pts',(-69.3484797028458,20.2558151671391,
0.));
#148123=CARTESIAN_POINT('Ctrl Pts',(-69.3288907959067,20.2411691081123,
0.));
#148124=CARTESIAN_POINT('Ctrl Pts',(-69.3093209004984,20.2265667465784,
0.));
#148125=CARTESIAN_POINT('Ctrl Pts',(-69.2897701438059,20.212008103862,0.));
#148126=CARTESIAN_POINT('Ctrl Pts',(-69.2702386535422,20.1974932012773,
0.));
#148127=CARTESIAN_POINT('Ctrl Pts',(-69.2507265579554,20.1830220601348,
0.));
#148128=CARTESIAN_POINT('Ctrl Pts',(-69.2312339858335,20.1685947017433,
0.));
#148129=CARTESIAN_POINT('Ctrl Pts',(-69.2117610665076,20.1542111474087,
0.));
#148130=CARTESIAN_POINT('Ctrl Pts',(-69.1923079298538,20.1398714184279,
0.));
#148131=CARTESIAN_POINT('Ctrl Pts',(-69.1728747062963,20.1255755360872,
0.));
#148132=CARTESIAN_POINT('Ctrl Pts',(-69.1534615268153,20.1113235216694,
0.));
#148133=CARTESIAN_POINT('Ctrl Pts',(-69.1340685229515,20.0971153964557,
0.));
#148134=CARTESIAN_POINT('Ctrl Pts',(-69.1146958268104,20.0829511817251,
0.));
#148135=CARTESIAN_POINT('Ctrl Pts',(-69.095343571064,20.068830898748,0.));
#148136=CARTESIAN_POINT('Ctrl Pts',(-69.0760118889535,20.0547545687842,
0.));
#148137=CARTESIAN_POINT('Ctrl Pts',(-69.0567009142978,20.0407222130905,
0.));
#148138=CARTESIAN_POINT('Ctrl Pts',(-69.0374107814984,20.0267338529223,
0.));
#148139=CARTESIAN_POINT('Ctrl Pts',(-69.0181416255431,20.0127895095326,
0.));
#148140=CARTESIAN_POINT('Ctrl Pts',(-68.9988935820084,19.9988892041666,
0.));
#148141=CARTESIAN_POINT('Ctrl Pts',(-68.9796667870638,19.9850329580591,
0.));
#148142=CARTESIAN_POINT('Ctrl Pts',(-68.9604613774802,19.9712207924428,
0.));
#148143=CARTESIAN_POINT('Ctrl Pts',(-68.9412774906333,19.9574527285488,
0.));
#148144=CARTESIAN_POINT('Ctrl Pts',(-68.9221152645095,19.9437287876066,
0.));
#148145=CARTESIAN_POINT('Ctrl Pts',(-68.9029748377067,19.9300489908374,
0.));
#148146=CARTESIAN_POINT('Ctrl Pts',(-68.8838563494393,19.9164133594525,
0.));
#148147=CARTESIAN_POINT('Ctrl Pts',(-68.8647599395469,19.9028219146618,
0.));
#148148=CARTESIAN_POINT('Ctrl Pts',(-68.8456857485002,19.8892746776739,
0.));
#148149=CARTESIAN_POINT('Ctrl Pts',(-68.8266339174056,19.8757716696965,
0.));
#148150=CARTESIAN_POINT('Ctrl Pts',(-68.8076045880065,19.8623129119293,
0.));
#148151=CARTESIAN_POINT('Ctrl Pts',(-68.7885979026879,19.8488984255627,
0.));
#148152=CARTESIAN_POINT('Ctrl Pts',(-68.7696140044851,19.8355282317858,
0.));
#148153=CARTESIAN_POINT('Ctrl Pts',(-68.7506530370904,19.822202351787,0.));
#148154=CARTESIAN_POINT('Ctrl Pts',(-68.7317151448573,19.8089208067537,
0.));
#148155=CARTESIAN_POINT('Ctrl Pts',(-68.7128004728034,19.7956836178651,
0.));
#148156=CARTESIAN_POINT('Ctrl Pts',(-68.693909166615,19.7824908062924,0.));
#148157=CARTESIAN_POINT('Ctrl Pts',(-68.6750413726575,19.7693423932066,
0.));
#148158=CARTESIAN_POINT('Ctrl Pts',(-68.65619723798,19.7562383997783,0.));
#148159=CARTESIAN_POINT('Ctrl Pts',(-68.6373769103211,19.7431788471772,
0.));
#148160=CARTESIAN_POINT('Ctrl Pts',(-68.6185805381102,19.7301637565645,
0.));
#148161=CARTESIAN_POINT('Ctrl Pts',(-68.5998082704741,19.717193149095,0.));
#148162=CARTESIAN_POINT('Ctrl Pts',(-68.5810602572474,19.7042670459233,
0.));
#148163=CARTESIAN_POINT('Ctrl Pts',(-68.5623366489776,19.6913854682046,
0.));
#148164=CARTESIAN_POINT('Ctrl Pts',(-68.543637596932,19.6785484370929,0.));
#148165=CARTESIAN_POINT('Ctrl Pts',(-68.5249632530994,19.665755973734,0.));
#148166=CARTESIAN_POINT('Ctrl Pts',(-68.5063137701986,19.6530080992689,
0.));
#148167=CARTESIAN_POINT('Ctrl Pts',(-68.4876893016863,19.6403048348396,
0.));
#148168=CARTESIAN_POINT('Ctrl Pts',(-68.4690900017631,19.6276462015888,
0.));
#148169=CARTESIAN_POINT('Ctrl Pts',(-68.4505160253777,19.6150322206577,
0.));
#148170=CARTESIAN_POINT('Ctrl Pts',(-68.4319675282273,19.6024629131785,
0.));
#148171=CARTESIAN_POINT('Ctrl Pts',(-68.4134446667695,19.5899383002803,
0.));
#148172=CARTESIAN_POINT('Ctrl Pts',(-68.3949475982334,19.5774584030938,
0.));
#148173=CARTESIAN_POINT('Ctrl Pts',(-68.3764764806287,19.5650232427516,
0.));
#148174=CARTESIAN_POINT('Ctrl Pts',(-68.3580314727522,19.5526328403851,
0.));
#148175=CARTESIAN_POINT('Ctrl Pts',(-68.3396127341937,19.540287217119,0.));
#148176=CARTESIAN_POINT('Ctrl Pts',(-68.3212204253416,19.5279863940772,
0.));
#148177=CARTESIAN_POINT('Ctrl Pts',(-68.3028547073862,19.5157303923855,
0.));
#148178=CARTESIAN_POINT('Ctrl Pts',(-68.2845157423234,19.5035192331706,
0.));
#148179=CARTESIAN_POINT('Ctrl Pts',(-68.2662036929531,19.4913529375545,
0.));
#148180=CARTESIAN_POINT('Ctrl Pts',(-68.2479187228815,19.4792315266505,
0.));
#148181=CARTESIAN_POINT('Ctrl Pts',(-68.2296609965461,19.4671550215724,
0.));
#148182=CARTESIAN_POINT('Ctrl Pts',(-68.2114306792366,19.4551234434383,
0.));
#148183=CARTESIAN_POINT('Ctrl Pts',(-68.1932279371121,19.4431368133718,
0.));
#148184=CARTESIAN_POINT('Ctrl Pts',(-68.1750529372211,19.4311951524977,
0.));
#148185=CARTESIAN_POINT('Ctrl Pts',(-68.1569058475026,19.419298481941,0.));
#148186=CARTESIAN_POINT('Ctrl Pts',(-68.1387868367668,19.4074468228293,
0.));
#148187=CARTESIAN_POINT('Ctrl Pts',(-68.1206960746763,19.3956401962893,
0.));
#148188=CARTESIAN_POINT('Ctrl Pts',(-68.1026337317298,19.3838786234425,
0.));
#148189=CARTESIAN_POINT('Ctrl Pts',(-68.0845999792274,19.372162125392,0.));
#148190=CARTESIAN_POINT('Ctrl Pts',(-68.0665949893222,19.3604907232322,
0.));
#148191=CARTESIAN_POINT('Ctrl Pts',(-68.0486189351027,19.3488644380646,
0.));
#148192=CARTESIAN_POINT('Ctrl Pts',(-68.0306719906636,19.3372832910076,
0.));
#148193=CARTESIAN_POINT('Ctrl Pts',(-68.0127543311761,19.3257473032031,
0.));
#148194=CARTESIAN_POINT('Ctrl Pts',(-67.9948661329592,19.3142564958195,
0.));
#148195=CARTESIAN_POINT('Ctrl Pts',(-67.977007573346,19.3028108900373,0.));
#148196=CARTESIAN_POINT('Ctrl Pts',(-67.959178830538,19.2914105070282,0.));
#148197=CARTESIAN_POINT('Ctrl Pts',(-67.9413800834798,19.2800553679362,
0.));
#148198=CARTESIAN_POINT('Ctrl Pts',(-67.9236115116781,19.2687454938448,
0.));
#148199=CARTESIAN_POINT('Ctrl Pts',(-67.9058732951822,19.2574809057705,
0.));
#148200=CARTESIAN_POINT('Ctrl Pts',(-67.8881656149983,19.2462616247287,
0.));
#148201=CARTESIAN_POINT('Ctrl Pts',(-67.8704886534555,19.2350876717877,
0.));
#148202=CARTESIAN_POINT('Ctrl Pts',(-67.852842594517,19.2239590681129,0.));
#148203=CARTESIAN_POINT('Ctrl Pts',(-67.8352276242856,19.2128758350336,
0.));
#148204=CARTESIAN_POINT('Ctrl Pts',(-67.817643930658,19.2018379939918,0.));
#148205=CARTESIAN_POINT('Ctrl Pts',(-67.8000917023896,19.1908455664089,
0.));
#148206=CARTESIAN_POINT('Ctrl Pts',(-67.7825711283092,19.1798985735687,
0.));
#148207=CARTESIAN_POINT('Ctrl Pts',(-67.7650823965156,19.1689970364958,
0.));
#148208=CARTESIAN_POINT('Ctrl Pts',(-67.7476256934493,19.1581409758112,
0.));
#148209=CARTESIAN_POINT('Ctrl Pts',(-67.730201205663,19.1473304119968,0.));
#148210=CARTESIAN_POINT('Ctrl Pts',(-67.7128091219372,19.1365653657097,
0.));
#148211=CARTESIAN_POINT('Ctrl Pts',(-67.6954496350053,19.1258458580343,
0.));
#148212=CARTESIAN_POINT('Ctrl Pts',(-67.6781229440535,19.115171910845,0.));
#148213=CARTESIAN_POINT('Ctrl Pts',(-67.6608292549412,19.1045435468344,
0.));
#148214=CARTESIAN_POINT('Ctrl Pts',(-67.6435687749803,19.0939607887491,
0.));
#148215=CARTESIAN_POINT('Ctrl Pts',(-67.6263417083414,19.0834236587115,
0.));
#148216=CARTESIAN_POINT('Ctrl Pts',(-67.6091482520558,19.0729321776286,
0.));
#148217=CARTESIAN_POINT('Ctrl Pts',(-67.5919885896278,19.0624863642425,
0.));
#148218=CARTESIAN_POINT('Ctrl Pts',(-67.5748628972035,19.0520862360413,
0.));
#148219=CARTESIAN_POINT('Ctrl Pts',(-67.5577713558248,19.0417318110721,
0.));
#148220=CARTESIAN_POINT('Ctrl Pts',(-67.5407141612881,19.0314231093923,
0.));
#148221=CARTESIAN_POINT('Ctrl Pts',(-67.5236915360253,19.0211601548222,
0.));
#148222=CARTESIAN_POINT('Ctrl Pts',(-67.5067037372177,19.0109429761274,
0.));
#148223=CARTESIAN_POINT('Ctrl Pts',(-67.4897510316692,19.0007716032784,
0.));
#148224=CARTESIAN_POINT('Ctrl Pts',(-67.4728336719559,18.9906460638607,
0.));
#148225=CARTESIAN_POINT('Ctrl Pts',(-67.4559518744714,18.9805663798466,
0.));
#148226=CARTESIAN_POINT('Ctrl Pts',(-67.4391057908687,18.9705325631772,
0.));
#148227=CARTESIAN_POINT('Ctrl Pts',(-67.4222955062385,18.9605446161078,
0.));
#148228=CARTESIAN_POINT('Ctrl Pts',(-67.4088759498287,18.9525909518002,
0.));
#148229=CARTESIAN_POINT('Ctrl Pts',(-67.398827414689,18.9466463414354,0.));
#148230=CARTESIAN_POINT('Ctrl Pts',(-67.3921355608417,18.942692439874,0.));
#148231=CARTESIAN_POINT('Ctrl Pts',(-67.3887914263119,18.9407177820969,
0.));
#148232=CARTESIAN_POINT('Ctrl Pts',(-69.065695021045,27.9316983239472,0.));
#148233=CARTESIAN_POINT('Ctrl Pts',(-69.065695021045,27.9316983239472,12.));
#148234=CARTESIAN_POINT('Ctrl Pts',(-69.0618620884721,27.9276214070631,
0.));
#148235=CARTESIAN_POINT('Ctrl Pts',(-69.0618620884721,27.9276214070631,
12.));
#148236=CARTESIAN_POINT('Ctrl Pts',(-69.0541967851028,27.9194718099003,
0.));
#148237=CARTESIAN_POINT('Ctrl Pts',(-69.0541967851028,27.9194718099003,
12.));
#148238=CARTESIAN_POINT('Ctrl Pts',(-69.0427005153791,27.9072601239722,
0.));
#148239=CARTESIAN_POINT('Ctrl Pts',(-69.0427005153791,27.9072601239722,
12.));
#148240=CARTESIAN_POINT('Ctrl Pts',(-69.0273755265383,27.8910032967339,
0.));
#148241=CARTESIAN_POINT('Ctrl Pts',(-69.0273755265383,27.8910032967339,
12.));
#148242=CARTESIAN_POINT('Ctrl Pts',(-69.0082249138598,27.8707246380957,
0.));
#148243=CARTESIAN_POINT('Ctrl Pts',(-69.0082249138598,27.8707246380957,
12.));
#148244=CARTESIAN_POINT('Ctrl Pts',(-68.9890799392213,27.8504883674058,
0.));
#148245=CARTESIAN_POINT('Ctrl Pts',(-68.9890799392213,27.8504883674058,
12.));
#148246=CARTESIAN_POINT('Ctrl Pts',(-68.9699406311389,27.8302945019976,
0.));
#148247=CARTESIAN_POINT('Ctrl Pts',(-68.9699406311389,27.8302945019976,
12.));
#148248=CARTESIAN_POINT('Ctrl Pts',(-68.9508070357658,27.8101430638071,
0.));
#148249=CARTESIAN_POINT('Ctrl Pts',(-68.9508070357658,27.8101430638071,
12.));
#148250=CARTESIAN_POINT('Ctrl Pts',(-68.9316792225946,27.7900340793689,
0.));
#148251=CARTESIAN_POINT('Ctrl Pts',(-68.9316792225946,27.7900340793689,
12.));
#148252=CARTESIAN_POINT('Ctrl Pts',(-68.9125572825694,27.7699675790571,
0.));
#148253=CARTESIAN_POINT('Ctrl Pts',(-68.9125572825694,27.7699675790571,
12.));
#148254=CARTESIAN_POINT('Ctrl Pts',(-68.8934413203759,27.7499435957525,
0.));
#148255=CARTESIAN_POINT('Ctrl Pts',(-68.8934413203759,27.7499435957525,
12.));
#148256=CARTESIAN_POINT('Ctrl Pts',(-68.8743314483369,27.7299621636566,
0.));
#148257=CARTESIAN_POINT('Ctrl Pts',(-68.8743314483369,27.7299621636566,
12.));
#148258=CARTESIAN_POINT('Ctrl Pts',(-68.85522777982,27.7100233170737,0.));
#148259=CARTESIAN_POINT('Ctrl Pts',(-68.85522777982,27.7100233170737,12.));
#148260=CARTESIAN_POINT('Ctrl Pts',(-68.8361304224467,27.6901270891241,
0.));
#148261=CARTESIAN_POINT('Ctrl Pts',(-68.8361304224467,27.6901270891241,
12.));
#148262=CARTESIAN_POINT('Ctrl Pts',(-68.81703947259,27.6702735107121,0.));
#148263=CARTESIAN_POINT('Ctrl Pts',(-68.81703947259,27.6702735107121,12.));
#148264=CARTESIAN_POINT('Ctrl Pts',(-68.7979550191872,27.6504626112666,
0.));
#148265=CARTESIAN_POINT('Ctrl Pts',(-68.7979550191872,27.6504626112666,
12.));
#148266=CARTESIAN_POINT('Ctrl Pts',(-68.7788771464713,27.6306944192737,
0.));
#148267=CARTESIAN_POINT('Ctrl Pts',(-68.7788771464713,27.6306944192737,
12.));
#148268=CARTESIAN_POINT('Ctrl Pts',(-68.7598059372129,27.6109689629029,
0.));
#148269=CARTESIAN_POINT('Ctrl Pts',(-68.7598059372129,27.6109689629029,
12.));
#148270=CARTESIAN_POINT('Ctrl Pts',(-68.740741475526,27.5912862705468,0.));
#148271=CARTESIAN_POINT('Ctrl Pts',(-68.740741475526,27.5912862705468,12.));
#148272=CARTESIAN_POINT('Ctrl Pts',(-68.7216838504218,27.5716463715004,
0.));
#148273=CARTESIAN_POINT('Ctrl Pts',(-68.7216838504218,27.5716463715004,
12.));
#148274=CARTESIAN_POINT('Ctrl Pts',(-68.7026331554296,27.5520492958907,
0.));
#148275=CARTESIAN_POINT('Ctrl Pts',(-68.7026331554296,27.5520492958907,
12.));
#148276=CARTESIAN_POINT('Ctrl Pts',(-68.6835894869882,27.5324950743706,
0.));
#148277=CARTESIAN_POINT('Ctrl Pts',(-68.6835894869882,27.5324950743706,
12.));
#148278=CARTESIAN_POINT('Ctrl Pts',(-68.6645529432045,27.5129837378791,
0.));
#148279=CARTESIAN_POINT('Ctrl Pts',(-68.6645529432045,27.5129837378791,
12.));
#148280=CARTESIAN_POINT('Ctrl Pts',(-68.645523622548,27.4935153173868,0.));
#148281=CARTESIAN_POINT('Ctrl Pts',(-68.645523622548,27.4935153173868,12.));
#148282=CARTESIAN_POINT('Ctrl Pts',(-68.6265016223561,27.4740898435988,
0.));
#148283=CARTESIAN_POINT('Ctrl Pts',(-68.6265016223561,27.4740898435988,
12.));
#148284=CARTESIAN_POINT('Ctrl Pts',(-68.6074870381619,27.4547073468226,
0.));
#148285=CARTESIAN_POINT('Ctrl Pts',(-68.6074870381619,27.4547073468226,
12.));
#148286=CARTESIAN_POINT('Ctrl Pts',(-68.5884799645218,27.4353678571361,
0.));
#148287=CARTESIAN_POINT('Ctrl Pts',(-68.5884799645218,27.4353678571361,
12.));
#148288=CARTESIAN_POINT('Ctrl Pts',(-68.5694804955014,27.4160714044831,
0.));
#148289=CARTESIAN_POINT('Ctrl Pts',(-68.5694804955014,27.4160714044831,
12.));
#148290=CARTESIAN_POINT('Ctrl Pts',(-68.5504887252975,27.3968180187941,
0.));
#148291=CARTESIAN_POINT('Ctrl Pts',(-68.5504887252975,27.3968180187941,
12.));
#148292=CARTESIAN_POINT('Ctrl Pts',(-68.5315047488035,27.3776077300914,
0.));
#148293=CARTESIAN_POINT('Ctrl Pts',(-68.5315047488035,27.3776077300914,
12.));
#148294=CARTESIAN_POINT('Ctrl Pts',(-68.5125286621888,27.3584405685941,
0.));
#148295=CARTESIAN_POINT('Ctrl Pts',(-68.5125286621888,27.3584405685941,
12.));
#148296=CARTESIAN_POINT('Ctrl Pts',(-68.4935605626362,27.3393165646748,
0.));
#148297=CARTESIAN_POINT('Ctrl Pts',(-68.4935605626362,27.3393165646748,
12.));
#148298=CARTESIAN_POINT('Ctrl Pts',(-68.4746005480993,27.3202357488153,
0.));
#148299=CARTESIAN_POINT('Ctrl Pts',(-68.4746005480993,27.3202357488153,
12.));
#148300=CARTESIAN_POINT('Ctrl Pts',(-68.455648717044,27.301198151557,0.));
#148301=CARTESIAN_POINT('Ctrl Pts',(-68.455648717044,27.301198151557,12.));
#148302=CARTESIAN_POINT('Ctrl Pts',(-68.4367051682166,27.2822038034539,
0.));
#148303=CARTESIAN_POINT('Ctrl Pts',(-68.4367051682166,27.2822038034539,
12.));
#148304=CARTESIAN_POINT('Ctrl Pts',(-68.4177700003471,27.2632527350062,
0.));
#148305=CARTESIAN_POINT('Ctrl Pts',(-68.4177700003471,27.2632527350062,
12.));
#148306=CARTESIAN_POINT('Ctrl Pts',(-68.398843312159,27.2443449766654,0.));
#148307=CARTESIAN_POINT('Ctrl Pts',(-68.398843312159,27.2443449766654,12.));
#148308=CARTESIAN_POINT('Ctrl Pts',(-68.379925202511,27.2254805588677,0.));
#148309=CARTESIAN_POINT('Ctrl Pts',(-68.379925202511,27.2254805588677,12.));
#148310=CARTESIAN_POINT('Ctrl Pts',(-68.3610157704999,27.2066595120544,
0.));
#148311=CARTESIAN_POINT('Ctrl Pts',(-68.3610157704999,27.2066595120544,
12.));
#148312=CARTESIAN_POINT('Ctrl Pts',(-68.3421151155708,27.1878818666925,
0.));
#148313=CARTESIAN_POINT('Ctrl Pts',(-68.3421151155708,27.1878818666925,
12.));
#148314=CARTESIAN_POINT('Ctrl Pts',(-68.3232233376415,27.1691476532917,
0.));
#148315=CARTESIAN_POINT('Ctrl Pts',(-68.3232233376415,27.1691476532917,
12.));
#148316=CARTESIAN_POINT('Ctrl Pts',(-68.3043405371589,27.150456902413,0.));
#148317=CARTESIAN_POINT('Ctrl Pts',(-68.3043405371589,27.150456902413,12.));
#148318=CARTESIAN_POINT('Ctrl Pts',(-68.285466815035,27.1318096446643,0.));
#148319=CARTESIAN_POINT('Ctrl Pts',(-68.285466815035,27.1318096446643,12.));
#148320=CARTESIAN_POINT('Ctrl Pts',(-68.2666022726094,27.1132059106939,
0.));
#148321=CARTESIAN_POINT('Ctrl Pts',(-68.2666022726094,27.1132059106939,
12.));
#148322=CARTESIAN_POINT('Ctrl Pts',(-68.2477470116014,27.0946457311813,
0.));
#148323=CARTESIAN_POINT('Ctrl Pts',(-68.2477470116014,27.0946457311813,
12.));
#148324=CARTESIAN_POINT('Ctrl Pts',(-68.2289011340624,27.076129136823,0.));
#148325=CARTESIAN_POINT('Ctrl Pts',(-68.2289011340624,27.076129136823,12.));
#148326=CARTESIAN_POINT('Ctrl Pts',(-68.2100647423345,27.0576561583179,
0.));
#148327=CARTESIAN_POINT('Ctrl Pts',(-68.2100647423345,27.0576561583179,
12.));
#148328=CARTESIAN_POINT('Ctrl Pts',(-68.1912379390787,27.0392268263804,
0.));
#148329=CARTESIAN_POINT('Ctrl Pts',(-68.1912379390787,27.0392268263804,
12.));
#148330=CARTESIAN_POINT('Ctrl Pts',(-68.1724208272967,27.0208411717477,
0.));
#148331=CARTESIAN_POINT('Ctrl Pts',(-68.1724208272967,27.0208411717477,
12.));
#148332=CARTESIAN_POINT('Ctrl Pts',(-68.1536135103558,27.0024992251839,
0.));
#148333=CARTESIAN_POINT('Ctrl Pts',(-68.1536135103558,27.0024992251839,
12.));
#148334=CARTESIAN_POINT('Ctrl Pts',(-68.13481609201,26.9842010174819,0.));
#148335=CARTESIAN_POINT('Ctrl Pts',(-68.13481609201,26.9842010174819,12.));
#148336=CARTESIAN_POINT('Ctrl Pts',(-68.1160286764244,26.9659465794596,
0.));
#148337=CARTESIAN_POINT('Ctrl Pts',(-68.1160286764244,26.9659465794596,
12.));
#148338=CARTESIAN_POINT('Ctrl Pts',(-68.0972513681739,26.9477359419646,
0.));
#148339=CARTESIAN_POINT('Ctrl Pts',(-68.0972513681739,26.9477359419646,
12.));
#148340=CARTESIAN_POINT('Ctrl Pts',(-68.0784842722362,26.9295691358775,
0.));
#148341=CARTESIAN_POINT('Ctrl Pts',(-68.0784842722362,26.9295691358775,
12.));
#148342=CARTESIAN_POINT('Ctrl Pts',(-68.0597274939857,26.9114461921109,
0.));
#148343=CARTESIAN_POINT('Ctrl Pts',(-68.0597274939857,26.9114461921109,
12.));
#148344=CARTESIAN_POINT('Ctrl Pts',(-68.0409811391872,26.8933671416064,
0.));
#148345=CARTESIAN_POINT('Ctrl Pts',(-68.0409811391872,26.8933671416064,
12.));
#148346=CARTESIAN_POINT('Ctrl Pts',(-68.0222453139862,26.8753320153255,
0.));
#148347=CARTESIAN_POINT('Ctrl Pts',(-68.0222453139862,26.8753320153255,
12.));
#148348=CARTESIAN_POINT('Ctrl Pts',(-68.0035201249108,26.85734084425,0.));
#148349=CARTESIAN_POINT('Ctrl Pts',(-68.0035201249108,26.85734084425,12.));
#148350=CARTESIAN_POINT('Ctrl Pts',(-67.9848056788814,26.8393936593914,
0.));
#148351=CARTESIAN_POINT('Ctrl Pts',(-67.9848056788814,26.8393936593914,
12.));
#148352=CARTESIAN_POINT('Ctrl Pts',(-67.9661020832165,26.8214904917922,
0.));
#148353=CARTESIAN_POINT('Ctrl Pts',(-67.9661020832165,26.8214904917922,
12.));
#148354=CARTESIAN_POINT('Ctrl Pts',(-67.9474094456395,26.8036313725262,
0.));
#148355=CARTESIAN_POINT('Ctrl Pts',(-67.9474094456395,26.8036313725262,
12.));
#148356=CARTESIAN_POINT('Ctrl Pts',(-67.9287278742839,26.7858163326932,
0.));
#148357=CARTESIAN_POINT('Ctrl Pts',(-67.9287278742839,26.7858163326932,
12.));
#148358=CARTESIAN_POINT('Ctrl Pts',(-67.9100574776974,26.7680454034168,
0.));
#148359=CARTESIAN_POINT('Ctrl Pts',(-67.9100574776974,26.7680454034168,
12.));
#148360=CARTESIAN_POINT('Ctrl Pts',(-67.8913983648441,26.7503186158523,
0.));
#148361=CARTESIAN_POINT('Ctrl Pts',(-67.8913983648441,26.7503186158523,
12.));
#148362=CARTESIAN_POINT('Ctrl Pts',(-67.8727506451068,26.7326360011886,
0.));
#148363=CARTESIAN_POINT('Ctrl Pts',(-67.8727506451068,26.7326360011886,
12.));
#148364=CARTESIAN_POINT('Ctrl Pts',(-67.8541144282875,26.7149975906478,
0.));
#148365=CARTESIAN_POINT('Ctrl Pts',(-67.8541144282875,26.7149975906478,
12.));
#148366=CARTESIAN_POINT('Ctrl Pts',(-67.8354898246079,26.6974034154803,
0.));
#148367=CARTESIAN_POINT('Ctrl Pts',(-67.8354898246079,26.6974034154803,
12.));
#148368=CARTESIAN_POINT('Ctrl Pts',(-67.8168769447086,26.6798535069586,
0.));
#148369=CARTESIAN_POINT('Ctrl Pts',(-67.8168769447086,26.6798535069586,
12.));
#148370=CARTESIAN_POINT('Ctrl Pts',(-67.7982758996557,26.6623478963867,
0.));
#148371=CARTESIAN_POINT('Ctrl Pts',(-67.7982758996557,26.6623478963867,
12.));
#148372=CARTESIAN_POINT('Ctrl Pts',(-67.7796868009447,26.6448866151027,
0.));
#148373=CARTESIAN_POINT('Ctrl Pts',(-67.7796868009447,26.6448866151027,
12.));
#148374=CARTESIAN_POINT('Ctrl Pts',(-67.7611097605042,26.6274696944793,
0.));
#148375=CARTESIAN_POINT('Ctrl Pts',(-67.7611097605042,26.6274696944793,
12.));
#148376=CARTESIAN_POINT('Ctrl Pts',(-67.7425448906983,26.6100971659204,
0.));
#148377=CARTESIAN_POINT('Ctrl Pts',(-67.7425448906983,26.6100971659204,
12.));
#148378=CARTESIAN_POINT('Ctrl Pts',(-67.7239923043295,26.5927690608546,
0.));
#148379=CARTESIAN_POINT('Ctrl Pts',(-67.7239923043295,26.5927690608546,
12.));
#148380=CARTESIAN_POINT('Ctrl Pts',(-67.7054521146427,26.5754854107422,
0.));
#148381=CARTESIAN_POINT('Ctrl Pts',(-67.7054521146427,26.5754854107422,
12.));
#148382=CARTESIAN_POINT('Ctrl Pts',(-67.6869244353292,26.5582462470794,
0.));
#148383=CARTESIAN_POINT('Ctrl Pts',(-67.6869244353292,26.5582462470794,
12.));
#148384=CARTESIAN_POINT('Ctrl Pts',(-67.6684093805288,26.5410516013984,
0.));
#148385=CARTESIAN_POINT('Ctrl Pts',(-67.6684093805288,26.5410516013984,
12.));
#148386=CARTESIAN_POINT('Ctrl Pts',(-67.6499070648323,26.5239015052655,
0.));
#148387=CARTESIAN_POINT('Ctrl Pts',(-67.6499070648323,26.5239015052655,
12.));
#148388=CARTESIAN_POINT('Ctrl Pts',(-67.6314176032823,26.506795990273,0.));
#148389=CARTESIAN_POINT('Ctrl Pts',(-67.6314176032823,26.506795990273,12.));
#148390=CARTESIAN_POINT('Ctrl Pts',(-67.6129411113774,26.4897350880446,
0.));
#148391=CARTESIAN_POINT('Ctrl Pts',(-67.6129411113774,26.4897350880446,
12.));
#148392=CARTESIAN_POINT('Ctrl Pts',(-67.5944777050782,26.4727188302415,
0.));
#148393=CARTESIAN_POINT('Ctrl Pts',(-67.5944777050782,26.4727188302415,
12.));
#148394=CARTESIAN_POINT('Ctrl Pts',(-67.5760275008096,26.4557472485622,
0.));
#148395=CARTESIAN_POINT('Ctrl Pts',(-67.5760275008096,26.4557472485622,
12.));
#148396=CARTESIAN_POINT('Ctrl Pts',(-67.5575906154648,26.4388203747422,
0.));
#148397=CARTESIAN_POINT('Ctrl Pts',(-67.5575906154648,26.4388203747422,
12.));
#148398=CARTESIAN_POINT('Ctrl Pts',(-67.5391671664055,26.4219382405452,
0.));
#148399=CARTESIAN_POINT('Ctrl Pts',(-67.5391671664055,26.4219382405452,
12.));
#148400=CARTESIAN_POINT('Ctrl Pts',(-67.5207572714666,26.4051008777669,
0.));
#148401=CARTESIAN_POINT('Ctrl Pts',(-67.5207572714666,26.4051008777669,
12.));
#148402=CARTESIAN_POINT('Ctrl Pts',(-67.5023610489611,26.3883083182417,
0.));
#148403=CARTESIAN_POINT('Ctrl Pts',(-67.5023610489611,26.3883083182417,
12.));
#148404=CARTESIAN_POINT('Ctrl Pts',(-67.4839786176833,26.3715605938432,
0.));
#148405=CARTESIAN_POINT('Ctrl Pts',(-67.4839786176833,26.3715605938432,
12.));
#148406=CARTESIAN_POINT('Ctrl Pts',(-67.4656100969121,26.3548577364835,
0.));
#148407=CARTESIAN_POINT('Ctrl Pts',(-67.4656100969121,26.3548577364835,
12.));
#148408=CARTESIAN_POINT('Ctrl Pts',(-67.4472556064127,26.3381997781059,
0.));
#148409=CARTESIAN_POINT('Ctrl Pts',(-67.4472556064127,26.3381997781059,
12.));
#148410=CARTESIAN_POINT('Ctrl Pts',(-67.4289152664406,26.3215867506864,
0.));
#148411=CARTESIAN_POINT('Ctrl Pts',(-67.4289152664406,26.3215867506864,
12.));
#148412=CARTESIAN_POINT('Ctrl Pts',(-67.4105891977465,26.305018686241,0.));
#148413=CARTESIAN_POINT('Ctrl Pts',(-67.4105891977465,26.305018686241,12.));
#148414=CARTESIAN_POINT('Ctrl Pts',(-67.392277521581,26.288495616827,0.));
#148415=CARTESIAN_POINT('Ctrl Pts',(-67.392277521581,26.288495616827,12.));
#148416=CARTESIAN_POINT('Ctrl Pts',(-67.3739803596967,26.2720175745422,
0.));
#148417=CARTESIAN_POINT('Ctrl Pts',(-67.3739803596967,26.2720175745422,
12.));
#148418=CARTESIAN_POINT('Ctrl Pts',(-67.3556978343506,26.255584591518,0.));
#148419=CARTESIAN_POINT('Ctrl Pts',(-67.3556978343506,26.255584591518,12.));
#148420=CARTESIAN_POINT('Ctrl Pts',(-67.3374300683076,26.2391966999192,
0.));
#148421=CARTESIAN_POINT('Ctrl Pts',(-67.3374300683076,26.2391966999192,
12.));
#148422=CARTESIAN_POINT('Ctrl Pts',(-67.3191771848468,26.2228539319527,
0.));
#148423=CARTESIAN_POINT('Ctrl Pts',(-67.3191771848468,26.2228539319527,
12.));
#148424=CARTESIAN_POINT('Ctrl Pts',(-67.3009393077654,26.2065563198684,
0.));
#148425=CARTESIAN_POINT('Ctrl Pts',(-67.3009393077654,26.2065563198684,
12.));
#148426=CARTESIAN_POINT('Ctrl Pts',(-67.2827165613828,26.1903038959589,
0.));
#148427=CARTESIAN_POINT('Ctrl Pts',(-67.2827165613828,26.1903038959589,
12.));
#148428=CARTESIAN_POINT('Ctrl Pts',(-67.2645090705414,26.1740966925527,
0.));
#148429=CARTESIAN_POINT('Ctrl Pts',(-67.2645090705414,26.1740966925527,
12.));
#148430=CARTESIAN_POINT('Ctrl Pts',(-67.2463169606105,26.1579347420135,
0.));
#148431=CARTESIAN_POINT('Ctrl Pts',(-67.2463169606105,26.1579347420135,
12.));
#148432=CARTESIAN_POINT('Ctrl Pts',(-67.228140357493,26.1418180767487,0.));
#148433=CARTESIAN_POINT('Ctrl Pts',(-67.228140357493,26.1418180767487,12.));
#148434=CARTESIAN_POINT('Ctrl Pts',(-67.2099793876295,26.1257467292102,
0.));
#148435=CARTESIAN_POINT('Ctrl Pts',(-67.2099793876295,26.1257467292102,
12.));
#148436=CARTESIAN_POINT('Ctrl Pts',(-67.191834178002,26.109720731895,0.));
#148437=CARTESIAN_POINT('Ctrl Pts',(-67.191834178002,26.109720731895,12.));
#148438=CARTESIAN_POINT('Ctrl Pts',(-67.1737048561364,26.0937401173385,
0.));
#148439=CARTESIAN_POINT('Ctrl Pts',(-67.1737048561364,26.0937401173385,
12.));
#148440=CARTESIAN_POINT('Ctrl Pts',(-67.1555915501052,26.0778049181129,
0.));
#148441=CARTESIAN_POINT('Ctrl Pts',(-67.1555915501052,26.0778049181129,
12.));
#148442=CARTESIAN_POINT('Ctrl Pts',(-67.1374943885353,26.061915166836,0.));
#148443=CARTESIAN_POINT('Ctrl Pts',(-67.1374943885353,26.061915166836,12.));
#148444=CARTESIAN_POINT('Ctrl Pts',(-67.1194135006122,26.0460708961725,
0.));
#148445=CARTESIAN_POINT('Ctrl Pts',(-67.1194135006122,26.0460708961725,
12.));
#148446=CARTESIAN_POINT('Ctrl Pts',(-67.101349016084,26.030272138834,0.));
#148447=CARTESIAN_POINT('Ctrl Pts',(-67.101349016084,26.030272138834,12.));
#148448=CARTESIAN_POINT('Ctrl Pts',(-67.083301065264,26.0145189275733,0.));
#148449=CARTESIAN_POINT('Ctrl Pts',(-67.083301065264,26.0145189275733,12.));
#148450=CARTESIAN_POINT('Ctrl Pts',(-67.0652697790335,25.9988112951818,
0.));
#148451=CARTESIAN_POINT('Ctrl Pts',(-67.0652697790335,25.9988112951818,
12.));
#148452=CARTESIAN_POINT('Ctrl Pts',(-67.0472552888495,25.9831492744988,
0.));
#148453=CARTESIAN_POINT('Ctrl Pts',(-67.0472552888495,25.9831492744988,
12.));
#148454=CARTESIAN_POINT('Ctrl Pts',(-67.0292577267495,25.9675328984123,
0.));
#148455=CARTESIAN_POINT('Ctrl Pts',(-67.0292577267495,25.9675328984123,
12.));
#148456=CARTESIAN_POINT('Ctrl Pts',(-67.0112772253553,25.9519621998598,
0.));
#148457=CARTESIAN_POINT('Ctrl Pts',(-67.0112772253553,25.9519621998598,
12.));
#148458=CARTESIAN_POINT('Ctrl Pts',(-66.993313917876,25.9364372118216,0.));
#148459=CARTESIAN_POINT('Ctrl Pts',(-66.993313917876,25.9364372118216,12.));
#148460=CARTESIAN_POINT('Ctrl Pts',(-66.9753679381122,25.9209579673198,
0.));
#148461=CARTESIAN_POINT('Ctrl Pts',(-66.9753679381122,25.9209579673198,
12.));
#148462=CARTESIAN_POINT('Ctrl Pts',(-66.9574394204635,25.9055244994266,
0.));
#148463=CARTESIAN_POINT('Ctrl Pts',(-66.9574394204635,25.9055244994266,
12.));
#148464=CARTESIAN_POINT('Ctrl Pts',(-66.9395284999327,25.8901368412655,
0.));
#148465=CARTESIAN_POINT('Ctrl Pts',(-66.9395284999327,25.8901368412655,
12.));
#148466=CARTESIAN_POINT('Ctrl Pts',(-66.9216353121308,25.8747950260114,
0.));
#148467=CARTESIAN_POINT('Ctrl Pts',(-66.9216353121308,25.8747950260114,
12.));
#148468=CARTESIAN_POINT('Ctrl Pts',(-66.9037599932787,25.8594990868845,
0.));
#148469=CARTESIAN_POINT('Ctrl Pts',(-66.9037599932787,25.8594990868845,
12.));
#148470=CARTESIAN_POINT('Ctrl Pts',(-66.8859026802123,25.8442490571486,
0.));
#148471=CARTESIAN_POINT('Ctrl Pts',(-66.8859026802123,25.8442490571486,
12.));
#148472=CARTESIAN_POINT('Ctrl Pts',(-66.8680635103907,25.8290449701206,
0.));
#148473=CARTESIAN_POINT('Ctrl Pts',(-66.8680635103907,25.8290449701206,
12.));
#148474=CARTESIAN_POINT('Ctrl Pts',(-66.8502426219015,25.8138868591715,
0.));
#148475=CARTESIAN_POINT('Ctrl Pts',(-66.8502426219015,25.8138868591715,
12.));
#148476=CARTESIAN_POINT('Ctrl Pts',(-66.8324401534658,25.7987747577264,
0.));
#148477=CARTESIAN_POINT('Ctrl Pts',(-66.8324401534658,25.7987747577264,
12.));
#148478=CARTESIAN_POINT('Ctrl Pts',(-66.8146562444397,25.783708699258,0.));
#148479=CARTESIAN_POINT('Ctrl Pts',(-66.8146562444397,25.783708699258,12.));
#148480=CARTESIAN_POINT('Ctrl Pts',(-66.7968910348199,25.7686887172859,
0.));
#148481=CARTESIAN_POINT('Ctrl Pts',(-66.7968910348199,25.7686887172859,
12.));
#148482=CARTESIAN_POINT('Ctrl Pts',(-66.7791446652505,25.7537148453848,
0.));
#148483=CARTESIAN_POINT('Ctrl Pts',(-66.7791446652505,25.7537148453848,
12.));
#148484=CARTESIAN_POINT('Ctrl Pts',(-66.7614172770302,25.7387871171861,
0.));
#148485=CARTESIAN_POINT('Ctrl Pts',(-66.7614172770302,25.7387871171861,
12.));
#148486=CARTESIAN_POINT('Ctrl Pts',(-66.7437090121168,25.7239055663778,
0.));
#148487=CARTESIAN_POINT('Ctrl Pts',(-66.7437090121168,25.7239055663778,
12.));
#148488=CARTESIAN_POINT('Ctrl Pts',(-66.72602001313,25.7090702266976,0.));
#148489=CARTESIAN_POINT('Ctrl Pts',(-66.72602001313,25.7090702266976,12.));
#148490=CARTESIAN_POINT('Ctrl Pts',(-66.7083504233566,25.6942811319337,
0.));
#148491=CARTESIAN_POINT('Ctrl Pts',(-66.7083504233566,25.6942811319337,
12.));
#148492=CARTESIAN_POINT('Ctrl Pts',(-66.6907003867599,25.6795383159329,
0.));
#148493=CARTESIAN_POINT('Ctrl Pts',(-66.6907003867599,25.6795383159329,
12.));
#148494=CARTESIAN_POINT('Ctrl Pts',(-66.6730700479844,25.6648418126016,
0.));
#148495=CARTESIAN_POINT('Ctrl Pts',(-66.6730700479844,25.6648418126016,
12.));
#148496=CARTESIAN_POINT('Ctrl Pts',(-66.6554595523611,25.650191655905,0.));
#148497=CARTESIAN_POINT('Ctrl Pts',(-66.6554595523611,25.650191655905,12.));
#148498=CARTESIAN_POINT('Ctrl Pts',(-66.6378690459105,25.6355878798605,
0.));
#148499=CARTESIAN_POINT('Ctrl Pts',(-66.6378690459105,25.6355878798605,
12.));
#148500=CARTESIAN_POINT('Ctrl Pts',(-66.6202986753482,25.6210305185394,
0.));
#148501=CARTESIAN_POINT('Ctrl Pts',(-66.6202986753482,25.6210305185394,
12.));
#148502=CARTESIAN_POINT('Ctrl Pts',(-66.6027485880947,25.606519606075,0.));
#148503=CARTESIAN_POINT('Ctrl Pts',(-66.6027485880947,25.606519606075,12.));
#148504=CARTESIAN_POINT('Ctrl Pts',(-66.5852189322811,25.5920551766629,
0.));
#148505=CARTESIAN_POINT('Ctrl Pts',(-66.5852189322811,25.5920551766629,
12.));
#148506=CARTESIAN_POINT('Ctrl Pts',(-66.5677098567551,25.5776372645605,
0.));
#148507=CARTESIAN_POINT('Ctrl Pts',(-66.5677098567551,25.5776372645605,
12.));
#148508=CARTESIAN_POINT('Ctrl Pts',(-66.5502215110843,25.5632659040797,
0.));
#148509=CARTESIAN_POINT('Ctrl Pts',(-66.5502215110843,25.5632659040797,
12.));
#148510=CARTESIAN_POINT('Ctrl Pts',(-66.5327540455639,25.5489411295916,
0.));
#148511=CARTESIAN_POINT('Ctrl Pts',(-66.5327540455639,25.5489411295916,
12.));
#148512=CARTESIAN_POINT('Ctrl Pts',(-66.5153076112237,25.5346629755322,
0.));
#148513=CARTESIAN_POINT('Ctrl Pts',(-66.5153076112237,25.5346629755322,
12.));
#148514=CARTESIAN_POINT('Ctrl Pts',(-66.4978823598352,25.5204314764033,
0.));
#148515=CARTESIAN_POINT('Ctrl Pts',(-66.4978823598352,25.5204314764033,
12.));
#148516=CARTESIAN_POINT('Ctrl Pts',(-66.4804784439146,25.5062466667703,
0.));
#148517=CARTESIAN_POINT('Ctrl Pts',(-66.4804784439146,25.5062466667703,
12.));
#148518=CARTESIAN_POINT('Ctrl Pts',(-66.463096016725,25.4921085812548,0.));
#148519=CARTESIAN_POINT('Ctrl Pts',(-66.463096016725,25.4921085812548,12.));
#148520=CARTESIAN_POINT('Ctrl Pts',(-66.445735232287,25.4780172545418,0.));
#148521=CARTESIAN_POINT('Ctrl Pts',(-66.445735232287,25.4780172545418,12.));
#148522=CARTESIAN_POINT('Ctrl Pts',(-66.4283962453899,25.463972721385,0.));
#148523=CARTESIAN_POINT('Ctrl Pts',(-66.4283962453899,25.463972721385,12.));
#148524=CARTESIAN_POINT('Ctrl Pts',(-66.4110792116,25.4499750166079,0.));
#148525=CARTESIAN_POINT('Ctrl Pts',(-66.4110792116,25.4499750166079,12.));
#148526=CARTESIAN_POINT('Ctrl Pts',(-66.3937842872684,25.4360241751017,
0.));
#148527=CARTESIAN_POINT('Ctrl Pts',(-66.3937842872684,25.4360241751017,
12.));
#148528=CARTESIAN_POINT('Ctrl Pts',(-66.3765116295364,25.4221202318198,
0.));
#148529=CARTESIAN_POINT('Ctrl Pts',(-66.3765116295364,25.4221202318198,
12.));
#148530=CARTESIAN_POINT('Ctrl Pts',(-66.3592613963407,25.4082632217846,
0.));
#148531=CARTESIAN_POINT('Ctrl Pts',(-66.3592613963407,25.4082632217846,
12.));
#148532=CARTESIAN_POINT('Ctrl Pts',(-66.3420337464176,25.39445318009,0.));
#148533=CARTESIAN_POINT('Ctrl Pts',(-66.3420337464176,25.39445318009,12.));
#148534=CARTESIAN_POINT('Ctrl Pts',(-66.3248288393046,25.3806901419012,
0.));
#148535=CARTESIAN_POINT('Ctrl Pts',(-66.3248288393046,25.3806901419012,
12.));
#148536=CARTESIAN_POINT('Ctrl Pts',(-66.3076468353417,25.366974142449,0.));
#148537=CARTESIAN_POINT('Ctrl Pts',(-66.3076468353417,25.366974142449,12.));
#148538=CARTESIAN_POINT('Ctrl Pts',(-66.2904878956721,25.3533052170253,
0.));
#148539=CARTESIAN_POINT('Ctrl Pts',(-66.2904878956721,25.3533052170253,
12.));
#148540=CARTESIAN_POINT('Ctrl Pts',(-66.2733521822675,25.3396834009954,
0.));
#148541=CARTESIAN_POINT('Ctrl Pts',(-66.2733521822675,25.3396834009954,
12.));
#148542=CARTESIAN_POINT('Ctrl Pts',(-66.2562398579479,25.3261087298029,
0.));
#148543=CARTESIAN_POINT('Ctrl Pts',(-66.2562398579479,25.3261087298029,
12.));
#148544=CARTESIAN_POINT('Ctrl Pts',(-66.2391510863992,25.3125812389727,
0.));
#148545=CARTESIAN_POINT('Ctrl Pts',(-66.2391510863992,25.3125812389727,
12.));
#148546=CARTESIAN_POINT('Ctrl Pts',(-66.2220860321931,25.2991009641086,
0.));
#148547=CARTESIAN_POINT('Ctrl Pts',(-66.2220860321931,25.2991009641086,
12.));
#148548=CARTESIAN_POINT('Ctrl Pts',(-66.2050448607883,25.285667940892,0.));
#148549=CARTESIAN_POINT('Ctrl Pts',(-66.2050448607883,25.285667940892,12.));
#148550=CARTESIAN_POINT('Ctrl Pts',(-66.1880277385114,25.2722822050828,
0.));
#148551=CARTESIAN_POINT('Ctrl Pts',(-66.1880277385114,25.2722822050828,
12.));
#148552=CARTESIAN_POINT('Ctrl Pts',(-66.1710348325378,25.2589437925145,
0.));
#148553=CARTESIAN_POINT('Ctrl Pts',(-66.1710348325378,25.2589437925145,
12.));
#148554=CARTESIAN_POINT('Ctrl Pts',(-66.1540663108767,25.245652739088,0.));
#148555=CARTESIAN_POINT('Ctrl Pts',(-66.1540663108767,25.245652739088,12.));
#148556=CARTESIAN_POINT('Ctrl Pts',(-66.1371223423372,25.232409080756,0.));
#148557=CARTESIAN_POINT('Ctrl Pts',(-66.1371223423372,25.232409080756,12.));
#148558=CARTESIAN_POINT('Ctrl Pts',(-66.1202030965785,25.2192128535367,
0.));
#148559=CARTESIAN_POINT('Ctrl Pts',(-66.1202030965785,25.2192128535367,
12.));
#148560=CARTESIAN_POINT('Ctrl Pts',(-66.1033087441916,25.2060640935371,
0.));
#148561=CARTESIAN_POINT('Ctrl Pts',(-66.1033087441916,25.2060640935371,
12.));
#148562=CARTESIAN_POINT('Ctrl Pts',(-66.086439456768,25.1929628369685,0.));
#148563=CARTESIAN_POINT('Ctrl Pts',(-66.086439456768,25.1929628369685,12.));
#148564=CARTESIAN_POINT('Ctrl Pts',(-66.0695954069699,25.1799091201594,
0.));
#148565=CARTESIAN_POINT('Ctrl Pts',(-66.0695954069699,25.1799091201594,
12.));
#148566=CARTESIAN_POINT('Ctrl Pts',(-66.0527767686,25.1669029795651,0.));
#148567=CARTESIAN_POINT('Ctrl Pts',(-66.0527767686,25.1669029795651,12.));
#148568=CARTESIAN_POINT('Ctrl Pts',(-66.0359837164709,25.1539444517409,
0.));
#148569=CARTESIAN_POINT('Ctrl Pts',(-66.0359837164709,25.1539444517409,
12.));
#148570=CARTESIAN_POINT('Ctrl Pts',(-66.0192164262607,25.1410335733094,
0.));
#148571=CARTESIAN_POINT('Ctrl Pts',(-66.0192164262607,25.1410335733094,
12.));
#148572=CARTESIAN_POINT('Ctrl Pts',(-66.0024750743902,25.1281703809299,
0.));
#148573=CARTESIAN_POINT('Ctrl Pts',(-66.0024750743902,25.1281703809299,
12.));
#148574=CARTESIAN_POINT('Ctrl Pts',(-65.9857598378455,25.1153549112511,
0.));
#148575=CARTESIAN_POINT('Ctrl Pts',(-65.9857598378455,25.1153549112511,
12.));
#148576=CARTESIAN_POINT('Ctrl Pts',(-65.9690708941591,25.1025872009016,
0.));
#148577=CARTESIAN_POINT('Ctrl Pts',(-65.9690708941591,25.1025872009016,
12.));
#148578=CARTESIAN_POINT('Ctrl Pts',(-65.9524084218167,25.0898672865926,
0.));
#148579=CARTESIAN_POINT('Ctrl Pts',(-65.9524084218167,25.0898672865926,
12.));
#148580=CARTESIAN_POINT('Ctrl Pts',(-65.9357726006174,25.0771952052032,
0.));
#148581=CARTESIAN_POINT('Ctrl Pts',(-65.9357726006174,25.0771952052032,
12.));
#148582=CARTESIAN_POINT('Ctrl Pts',(-65.9191636119796,25.0645709938519,
0.));
#148583=CARTESIAN_POINT('Ctrl Pts',(-65.9191636119796,25.0645709938519,
12.));
#148584=CARTESIAN_POINT('Ctrl Pts',(-65.9025816394391,25.0519946900066,
0.));
#148585=CARTESIAN_POINT('Ctrl Pts',(-65.9025816394391,25.0519946900066,
12.));
#148586=CARTESIAN_POINT('Ctrl Pts',(-65.8860268683088,25.039466331404,0.));
#148587=CARTESIAN_POINT('Ctrl Pts',(-65.8860268683088,25.039466331404,12.));
#148588=CARTESIAN_POINT('Ctrl Pts',(-65.8694994847587,25.0269859558351,
0.));
#148589=CARTESIAN_POINT('Ctrl Pts',(-65.8694994847587,25.0269859558351,
12.));
#148590=CARTESIAN_POINT('Ctrl Pts',(-65.8529996750441,25.0145536009603,
0.));
#148591=CARTESIAN_POINT('Ctrl Pts',(-65.8529996750441,25.0145536009603,
12.));
#148592=CARTESIAN_POINT('Ctrl Pts',(-65.8365276247157,25.0021693041181,
0.));
#148593=CARTESIAN_POINT('Ctrl Pts',(-65.8365276247157,25.0021693041181,
12.));
#148594=CARTESIAN_POINT('Ctrl Pts',(-65.8200835177071,24.9898331021002,
0.));
#148595=CARTESIAN_POINT('Ctrl Pts',(-65.8200835177071,24.9898331021002,
12.));
#148596=CARTESIAN_POINT('Ctrl Pts',(-65.8036675380761,24.97754503157,0.));
#148597=CARTESIAN_POINT('Ctrl Pts',(-65.8036675380761,24.97754503157,12.));
#148598=CARTESIAN_POINT('Ctrl Pts',(-65.7872798720847,24.965305129559,0.));
#148599=CARTESIAN_POINT('Ctrl Pts',(-65.7872798720847,24.965305129559,12.));
#148600=CARTESIAN_POINT('Ctrl Pts',(-65.7709207098949,24.9531134338693,
0.));
#148601=CARTESIAN_POINT('Ctrl Pts',(-65.7709207098949,24.9531134338693,
12.));
#148602=CARTESIAN_POINT('Ctrl Pts',(-65.7545902480286,24.9409699836523,
0.));
#148603=CARTESIAN_POINT('Ctrl Pts',(-65.7545902480286,24.9409699836523,
12.));
#148604=CARTESIAN_POINT('Ctrl Pts',(-65.7382886895839,24.9288748194562,
0.));
#148605=CARTESIAN_POINT('Ctrl Pts',(-65.7382886895839,24.9288748194562,
12.));
#148606=CARTESIAN_POINT('Ctrl Pts',(-65.7220162391016,24.9168279820093,
0.));
#148607=CARTESIAN_POINT('Ctrl Pts',(-65.7220162391016,24.9168279820093,
12.));
#148608=CARTESIAN_POINT('Ctrl Pts',(-65.7057730980471,24.9048295111444,
0.));
#148609=CARTESIAN_POINT('Ctrl Pts',(-65.7057730980471,24.9048295111444,
12.));
#148610=CARTESIAN_POINT('Ctrl Pts',(-65.6895594608798,24.8928794448615,
0.));
#148611=CARTESIAN_POINT('Ctrl Pts',(-65.6895594608798,24.8928794448615,
12.));
#148612=CARTESIAN_POINT('Ctrl Pts',(-65.6733755087724,24.8809778178248,
0.));
#148613=CARTESIAN_POINT('Ctrl Pts',(-65.6733755087724,24.8809778178248,
12.));
#148614=CARTESIAN_POINT('Ctrl Pts',(-65.6572214156761,24.869124662808,0.));
#148615=CARTESIAN_POINT('Ctrl Pts',(-65.6572214156761,24.869124662808,12.));
#148616=CARTESIAN_POINT('Ctrl Pts',(-65.6410973603713,24.8573200135683,
0.));
#148617=CARTESIAN_POINT('Ctrl Pts',(-65.6410973603713,24.8573200135683,
12.));
#148618=CARTESIAN_POINT('Ctrl Pts',(-65.6250035361612,24.8455639071517,
0.));
#148619=CARTESIAN_POINT('Ctrl Pts',(-65.6250035361612,24.8455639071517,
12.));
#148620=CARTESIAN_POINT('Ctrl Pts',(-65.6089401625552,24.8338563866739,
0.));
#148621=CARTESIAN_POINT('Ctrl Pts',(-65.6089401625552,24.8338563866739,
12.));
#148622=CARTESIAN_POINT('Ctrl Pts',(-65.5929074932487,24.8221975032059,
0.));
#148623=CARTESIAN_POINT('Ctrl Pts',(-65.5929074932487,24.8221975032059,
12.));
#148624=CARTESIAN_POINT('Ctrl Pts',(-65.5769057914184,24.8105873098578,
0.));
#148625=CARTESIAN_POINT('Ctrl Pts',(-65.5769057914184,24.8105873098578,
12.));
#148626=CARTESIAN_POINT('Ctrl Pts',(-65.560935306275,24.7990258561234,0.));
#148627=CARTESIAN_POINT('Ctrl Pts',(-65.560935306275,24.7990258561234,12.));
#148628=CARTESIAN_POINT('Ctrl Pts',(-65.5449962514735,24.7875131827515,
0.));
#148629=CARTESIAN_POINT('Ctrl Pts',(-65.5449962514735,24.7875131827515,
12.));
#148630=CARTESIAN_POINT('Ctrl Pts',(-65.5290887770494,24.776049314855,0.));
#148631=CARTESIAN_POINT('Ctrl Pts',(-65.5290887770494,24.776049314855,12.));
#148632=CARTESIAN_POINT('Ctrl Pts',(-65.5132129675727,24.7646342620969,
0.));
#148633=CARTESIAN_POINT('Ctrl Pts',(-65.5132129675727,24.7646342620969,
12.));
#148634=CARTESIAN_POINT('Ctrl Pts',(-65.5005376841469,24.755541272477,0.));
#148635=CARTESIAN_POINT('Ctrl Pts',(-65.5005376841469,24.755541272477,12.));
#148636=CARTESIAN_POINT('Ctrl Pts',(-65.4910454936487,24.7487434956058,
0.));
#148637=CARTESIAN_POINT('Ctrl Pts',(-65.4910454936487,24.7487434956058,
12.));
#148638=CARTESIAN_POINT('Ctrl Pts',(-65.484723709553,24.7442214063411,0.));
#148639=CARTESIAN_POINT('Ctrl Pts',(-65.484723709553,24.7442214063411,12.));
#148640=CARTESIAN_POINT('Ctrl Pts',(-65.4815644032299,24.7419628022042,
0.));
#148641=CARTESIAN_POINT('Ctrl Pts',(-65.4815644032299,24.7419628022042,
12.));
#148642=CARTESIAN_POINT('',(-65.4815644032299,24.7419628022042,12.));
#148643=CARTESIAN_POINT('Ctrl Pts',(-65.4815644032299,24.7419628022042,
12.));
#148644=CARTESIAN_POINT('Ctrl Pts',(-65.484723709553,24.7442214063411,12.));
#148645=CARTESIAN_POINT('Ctrl Pts',(-65.4910454936487,24.7487434956058,
12.));
#148646=CARTESIAN_POINT('Ctrl Pts',(-65.5005376841469,24.755541272477,12.));
#148647=CARTESIAN_POINT('Ctrl Pts',(-65.5132129675727,24.7646342620969,
12.));
#148648=CARTESIAN_POINT('Ctrl Pts',(-65.5290887770494,24.776049314855,12.));
#148649=CARTESIAN_POINT('Ctrl Pts',(-65.5449962514735,24.7875131827515,
12.));
#148650=CARTESIAN_POINT('Ctrl Pts',(-65.560935306275,24.7990258561234,12.));
#148651=CARTESIAN_POINT('Ctrl Pts',(-65.5769057914184,24.8105873098578,
12.));
#148652=CARTESIAN_POINT('Ctrl Pts',(-65.5929074932487,24.8221975032059,
12.));
#148653=CARTESIAN_POINT('Ctrl Pts',(-65.6089401625552,24.8338563866739,
12.));
#148654=CARTESIAN_POINT('Ctrl Pts',(-65.6250035361612,24.8455639071517,
12.));
#148655=CARTESIAN_POINT('Ctrl Pts',(-65.6410973603713,24.8573200135683,
12.));
#148656=CARTESIAN_POINT('Ctrl Pts',(-65.6572214156761,24.869124662808,12.));
#148657=CARTESIAN_POINT('Ctrl Pts',(-65.6733755087724,24.8809778178248,
12.));
#148658=CARTESIAN_POINT('Ctrl Pts',(-65.6895594608798,24.8928794448615,
12.));
#148659=CARTESIAN_POINT('Ctrl Pts',(-65.7057730980471,24.9048295111444,
12.));
#148660=CARTESIAN_POINT('Ctrl Pts',(-65.7220162391016,24.9168279820093,
12.));
#148661=CARTESIAN_POINT('Ctrl Pts',(-65.7382886895839,24.9288748194562,
12.));
#148662=CARTESIAN_POINT('Ctrl Pts',(-65.7545902480286,24.9409699836523,
12.));
#148663=CARTESIAN_POINT('Ctrl Pts',(-65.7709207098949,24.9531134338693,
12.));
#148664=CARTESIAN_POINT('Ctrl Pts',(-65.7872798720847,24.965305129559,12.));
#148665=CARTESIAN_POINT('Ctrl Pts',(-65.8036675380761,24.97754503157,12.));
#148666=CARTESIAN_POINT('Ctrl Pts',(-65.8200835177071,24.9898331021002,
12.));
#148667=CARTESIAN_POINT('Ctrl Pts',(-65.8365276247157,25.0021693041181,
12.));
#148668=CARTESIAN_POINT('Ctrl Pts',(-65.8529996750441,25.0145536009603,
12.));
#148669=CARTESIAN_POINT('Ctrl Pts',(-65.8694994847587,25.0269859558351,
12.));
#148670=CARTESIAN_POINT('Ctrl Pts',(-65.8860268683088,25.039466331404,12.));
#148671=CARTESIAN_POINT('Ctrl Pts',(-65.9025816394391,25.0519946900066,
12.));
#148672=CARTESIAN_POINT('Ctrl Pts',(-65.9191636119796,25.0645709938519,
12.));
#148673=CARTESIAN_POINT('Ctrl Pts',(-65.9357726006174,25.0771952052032,
12.));
#148674=CARTESIAN_POINT('Ctrl Pts',(-65.9524084218167,25.0898672865926,
12.));
#148675=CARTESIAN_POINT('Ctrl Pts',(-65.9690708941591,25.1025872009016,
12.));
#148676=CARTESIAN_POINT('Ctrl Pts',(-65.9857598378455,25.1153549112511,
12.));
#148677=CARTESIAN_POINT('Ctrl Pts',(-66.0024750743902,25.1281703809299,
12.));
#148678=CARTESIAN_POINT('Ctrl Pts',(-66.0192164262607,25.1410335733094,
12.));
#148679=CARTESIAN_POINT('Ctrl Pts',(-66.0359837164709,25.1539444517409,
12.));
#148680=CARTESIAN_POINT('Ctrl Pts',(-66.0527767686,25.1669029795651,12.));
#148681=CARTESIAN_POINT('Ctrl Pts',(-66.0695954069699,25.1799091201594,
12.));
#148682=CARTESIAN_POINT('Ctrl Pts',(-66.086439456768,25.1929628369685,12.));
#148683=CARTESIAN_POINT('Ctrl Pts',(-66.1033087441916,25.2060640935371,
12.));
#148684=CARTESIAN_POINT('Ctrl Pts',(-66.1202030965785,25.2192128535367,
12.));
#148685=CARTESIAN_POINT('Ctrl Pts',(-66.1371223423372,25.232409080756,12.));
#148686=CARTESIAN_POINT('Ctrl Pts',(-66.1540663108767,25.245652739088,12.));
#148687=CARTESIAN_POINT('Ctrl Pts',(-66.1710348325378,25.2589437925145,
12.));
#148688=CARTESIAN_POINT('Ctrl Pts',(-66.1880277385114,25.2722822050828,
12.));
#148689=CARTESIAN_POINT('Ctrl Pts',(-66.2050448607883,25.285667940892,12.));
#148690=CARTESIAN_POINT('Ctrl Pts',(-66.2220860321931,25.2991009641086,
12.));
#148691=CARTESIAN_POINT('Ctrl Pts',(-66.2391510863992,25.3125812389727,
12.));
#148692=CARTESIAN_POINT('Ctrl Pts',(-66.2562398579479,25.3261087298029,
12.));
#148693=CARTESIAN_POINT('Ctrl Pts',(-66.2733521822675,25.3396834009954,
12.));
#148694=CARTESIAN_POINT('Ctrl Pts',(-66.2904878956721,25.3533052170253,
12.));
#148695=CARTESIAN_POINT('Ctrl Pts',(-66.3076468353417,25.366974142449,12.));
#148696=CARTESIAN_POINT('Ctrl Pts',(-66.3248288393046,25.3806901419012,
12.));
#148697=CARTESIAN_POINT('Ctrl Pts',(-66.3420337464176,25.39445318009,12.));
#148698=CARTESIAN_POINT('Ctrl Pts',(-66.3592613963407,25.4082632217846,
12.));
#148699=CARTESIAN_POINT('Ctrl Pts',(-66.3765116295364,25.4221202318198,
12.));
#148700=CARTESIAN_POINT('Ctrl Pts',(-66.3937842872684,25.4360241751017,
12.));
#148701=CARTESIAN_POINT('Ctrl Pts',(-66.4110792116,25.4499750166079,12.));
#148702=CARTESIAN_POINT('Ctrl Pts',(-66.4283962453899,25.463972721385,12.));
#148703=CARTESIAN_POINT('Ctrl Pts',(-66.445735232287,25.4780172545418,12.));
#148704=CARTESIAN_POINT('Ctrl Pts',(-66.463096016725,25.4921085812548,12.));
#148705=CARTESIAN_POINT('Ctrl Pts',(-66.4804784439146,25.5062466667703,
12.));
#148706=CARTESIAN_POINT('Ctrl Pts',(-66.4978823598352,25.5204314764033,
12.));
#148707=CARTESIAN_POINT('Ctrl Pts',(-66.5153076112237,25.5346629755322,
12.));
#148708=CARTESIAN_POINT('Ctrl Pts',(-66.5327540455639,25.5489411295916,
12.));
#148709=CARTESIAN_POINT('Ctrl Pts',(-66.5502215110843,25.5632659040797,
12.));
#148710=CARTESIAN_POINT('Ctrl Pts',(-66.5677098567551,25.5776372645605,
12.));
#148711=CARTESIAN_POINT('Ctrl Pts',(-66.5852189322811,25.5920551766629,
12.));
#148712=CARTESIAN_POINT('Ctrl Pts',(-66.6027485880947,25.606519606075,12.));
#148713=CARTESIAN_POINT('Ctrl Pts',(-66.6202986753482,25.6210305185394,
12.));
#148714=CARTESIAN_POINT('Ctrl Pts',(-66.6378690459105,25.6355878798605,
12.));
#148715=CARTESIAN_POINT('Ctrl Pts',(-66.6554595523611,25.650191655905,12.));
#148716=CARTESIAN_POINT('Ctrl Pts',(-66.6730700479844,25.6648418126016,
12.));
#148717=CARTESIAN_POINT('Ctrl Pts',(-66.6907003867599,25.6795383159329,
12.));
#148718=CARTESIAN_POINT('Ctrl Pts',(-66.7083504233566,25.6942811319337,
12.));
#148719=CARTESIAN_POINT('Ctrl Pts',(-66.72602001313,25.7090702266976,12.));
#148720=CARTESIAN_POINT('Ctrl Pts',(-66.7437090121168,25.7239055663778,
12.));
#148721=CARTESIAN_POINT('Ctrl Pts',(-66.7614172770302,25.7387871171861,
12.));
#148722=CARTESIAN_POINT('Ctrl Pts',(-66.7791446652505,25.7537148453848,
12.));
#148723=CARTESIAN_POINT('Ctrl Pts',(-66.7968910348199,25.7686887172859,
12.));
#148724=CARTESIAN_POINT('Ctrl Pts',(-66.8146562444397,25.783708699258,12.));
#148725=CARTESIAN_POINT('Ctrl Pts',(-66.8324401534658,25.7987747577264,
12.));
#148726=CARTESIAN_POINT('Ctrl Pts',(-66.8502426219015,25.8138868591715,
12.));
#148727=CARTESIAN_POINT('Ctrl Pts',(-66.8680635103907,25.8290449701206,
12.));
#148728=CARTESIAN_POINT('Ctrl Pts',(-66.8859026802123,25.8442490571486,
12.));
#148729=CARTESIAN_POINT('Ctrl Pts',(-66.9037599932787,25.8594990868845,
12.));
#148730=CARTESIAN_POINT('Ctrl Pts',(-66.9216353121308,25.8747950260114,
12.));
#148731=CARTESIAN_POINT('Ctrl Pts',(-66.9395284999327,25.8901368412655,
12.));
#148732=CARTESIAN_POINT('Ctrl Pts',(-66.9574394204635,25.9055244994266,
12.));
#148733=CARTESIAN_POINT('Ctrl Pts',(-66.9753679381122,25.9209579673198,
12.));
#148734=CARTESIAN_POINT('Ctrl Pts',(-66.993313917876,25.9364372118216,12.));
#148735=CARTESIAN_POINT('Ctrl Pts',(-67.0112772253553,25.9519621998598,
12.));
#148736=CARTESIAN_POINT('Ctrl Pts',(-67.0292577267495,25.9675328984123,
12.));
#148737=CARTESIAN_POINT('Ctrl Pts',(-67.0472552888495,25.9831492744988,
12.));
#148738=CARTESIAN_POINT('Ctrl Pts',(-67.0652697790335,25.9988112951818,
12.));
#148739=CARTESIAN_POINT('Ctrl Pts',(-67.083301065264,26.0145189275733,12.));
#148740=CARTESIAN_POINT('Ctrl Pts',(-67.101349016084,26.030272138834,12.));
#148741=CARTESIAN_POINT('Ctrl Pts',(-67.1194135006122,26.0460708961725,
12.));
#148742=CARTESIAN_POINT('Ctrl Pts',(-67.1374943885353,26.061915166836,12.));
#148743=CARTESIAN_POINT('Ctrl Pts',(-67.1555915501052,26.0778049181129,
12.));
#148744=CARTESIAN_POINT('Ctrl Pts',(-67.1737048561364,26.0937401173385,
12.));
#148745=CARTESIAN_POINT('Ctrl Pts',(-67.191834178002,26.109720731895,12.));
#148746=CARTESIAN_POINT('Ctrl Pts',(-67.2099793876295,26.1257467292102,
12.));
#148747=CARTESIAN_POINT('Ctrl Pts',(-67.228140357493,26.1418180767487,12.));
#148748=CARTESIAN_POINT('Ctrl Pts',(-67.2463169606105,26.1579347420135,
12.));
#148749=CARTESIAN_POINT('Ctrl Pts',(-67.2645090705414,26.1740966925527,
12.));
#148750=CARTESIAN_POINT('Ctrl Pts',(-67.2827165613828,26.1903038959589,
12.));
#148751=CARTESIAN_POINT('Ctrl Pts',(-67.3009393077654,26.2065563198684,
12.));
#148752=CARTESIAN_POINT('Ctrl Pts',(-67.3191771848468,26.2228539319527,
12.));
#148753=CARTESIAN_POINT('Ctrl Pts',(-67.3374300683076,26.2391966999192,
12.));
#148754=CARTESIAN_POINT('Ctrl Pts',(-67.3556978343506,26.255584591518,12.));
#148755=CARTESIAN_POINT('Ctrl Pts',(-67.3739803596967,26.2720175745422,
12.));
#148756=CARTESIAN_POINT('Ctrl Pts',(-67.392277521581,26.288495616827,12.));
#148757=CARTESIAN_POINT('Ctrl Pts',(-67.4105891977465,26.305018686241,12.));
#148758=CARTESIAN_POINT('Ctrl Pts',(-67.4289152664406,26.3215867506864,
12.));
#148759=CARTESIAN_POINT('Ctrl Pts',(-67.4472556064127,26.3381997781059,
12.));
#148760=CARTESIAN_POINT('Ctrl Pts',(-67.4656100969121,26.3548577364835,
12.));
#148761=CARTESIAN_POINT('Ctrl Pts',(-67.4839786176833,26.3715605938432,
12.));
#148762=CARTESIAN_POINT('Ctrl Pts',(-67.5023610489611,26.3883083182417,
12.));
#148763=CARTESIAN_POINT('Ctrl Pts',(-67.5207572714666,26.4051008777669,
12.));
#148764=CARTESIAN_POINT('Ctrl Pts',(-67.5391671664055,26.4219382405452,
12.));
#148765=CARTESIAN_POINT('Ctrl Pts',(-67.5575906154648,26.4388203747422,
12.));
#148766=CARTESIAN_POINT('Ctrl Pts',(-67.5760275008096,26.4557472485622,
12.));
#148767=CARTESIAN_POINT('Ctrl Pts',(-67.5944777050782,26.4727188302415,
12.));
#148768=CARTESIAN_POINT('Ctrl Pts',(-67.6129411113774,26.4897350880446,
12.));
#148769=CARTESIAN_POINT('Ctrl Pts',(-67.6314176032823,26.506795990273,12.));
#148770=CARTESIAN_POINT('Ctrl Pts',(-67.6499070648323,26.5239015052655,
12.));
#148771=CARTESIAN_POINT('Ctrl Pts',(-67.6684093805288,26.5410516013984,
12.));
#148772=CARTESIAN_POINT('Ctrl Pts',(-67.6869244353292,26.5582462470794,
12.));
#148773=CARTESIAN_POINT('Ctrl Pts',(-67.7054521146427,26.5754854107422,
12.));
#148774=CARTESIAN_POINT('Ctrl Pts',(-67.7239923043295,26.5927690608546,
12.));
#148775=CARTESIAN_POINT('Ctrl Pts',(-67.7425448906983,26.6100971659204,
12.));
#148776=CARTESIAN_POINT('Ctrl Pts',(-67.7611097605042,26.6274696944793,
12.));
#148777=CARTESIAN_POINT('Ctrl Pts',(-67.7796868009447,26.6448866151027,
12.));
#148778=CARTESIAN_POINT('Ctrl Pts',(-67.7982758996557,26.6623478963867,
12.));
#148779=CARTESIAN_POINT('Ctrl Pts',(-67.8168769447086,26.6798535069586,
12.));
#148780=CARTESIAN_POINT('Ctrl Pts',(-67.8354898246079,26.6974034154803,
12.));
#148781=CARTESIAN_POINT('Ctrl Pts',(-67.8541144282875,26.7149975906478,
12.));
#148782=CARTESIAN_POINT('Ctrl Pts',(-67.8727506451068,26.7326360011886,
12.));
#148783=CARTESIAN_POINT('Ctrl Pts',(-67.8913983648441,26.7503186158523,
12.));
#148784=CARTESIAN_POINT('Ctrl Pts',(-67.9100574776974,26.7680454034168,
12.));
#148785=CARTESIAN_POINT('Ctrl Pts',(-67.9287278742839,26.7858163326932,
12.));
#148786=CARTESIAN_POINT('Ctrl Pts',(-67.9474094456395,26.8036313725262,
12.));
#148787=CARTESIAN_POINT('Ctrl Pts',(-67.9661020832165,26.8214904917922,
12.));
#148788=CARTESIAN_POINT('Ctrl Pts',(-67.9848056788814,26.8393936593914,
12.));
#148789=CARTESIAN_POINT('Ctrl Pts',(-68.0035201249108,26.85734084425,12.));
#148790=CARTESIAN_POINT('Ctrl Pts',(-68.0222453139862,26.8753320153255,
12.));
#148791=CARTESIAN_POINT('Ctrl Pts',(-68.0409811391872,26.8933671416064,
12.));
#148792=CARTESIAN_POINT('Ctrl Pts',(-68.0597274939857,26.9114461921109,
12.));
#148793=CARTESIAN_POINT('Ctrl Pts',(-68.0784842722362,26.9295691358775,
12.));
#148794=CARTESIAN_POINT('Ctrl Pts',(-68.0972513681739,26.9477359419646,
12.));
#148795=CARTESIAN_POINT('Ctrl Pts',(-68.1160286764244,26.9659465794596,
12.));
#148796=CARTESIAN_POINT('Ctrl Pts',(-68.13481609201,26.9842010174819,12.));
#148797=CARTESIAN_POINT('Ctrl Pts',(-68.1536135103558,27.0024992251839,
12.));
#148798=CARTESIAN_POINT('Ctrl Pts',(-68.1724208272967,27.0208411717477,
12.));
#148799=CARTESIAN_POINT('Ctrl Pts',(-68.1912379390787,27.0392268263804,
12.));
#148800=CARTESIAN_POINT('Ctrl Pts',(-68.2100647423345,27.0576561583179,
12.));
#148801=CARTESIAN_POINT('Ctrl Pts',(-68.2289011340624,27.076129136823,12.));
#148802=CARTESIAN_POINT('Ctrl Pts',(-68.2477470116014,27.0946457311813,
12.));
#148803=CARTESIAN_POINT('Ctrl Pts',(-68.2666022726094,27.1132059106939,
12.));
#148804=CARTESIAN_POINT('Ctrl Pts',(-68.285466815035,27.1318096446643,12.));
#148805=CARTESIAN_POINT('Ctrl Pts',(-68.3043405371589,27.150456902413,12.));
#148806=CARTESIAN_POINT('Ctrl Pts',(-68.3232233376415,27.1691476532917,
12.));
#148807=CARTESIAN_POINT('Ctrl Pts',(-68.3421151155708,27.1878818666925,
12.));
#148808=CARTESIAN_POINT('Ctrl Pts',(-68.3610157704999,27.2066595120544,
12.));
#148809=CARTESIAN_POINT('Ctrl Pts',(-68.379925202511,27.2254805588677,12.));
#148810=CARTESIAN_POINT('Ctrl Pts',(-68.398843312159,27.2443449766654,12.));
#148811=CARTESIAN_POINT('Ctrl Pts',(-68.4177700003471,27.2632527350062,
12.));
#148812=CARTESIAN_POINT('Ctrl Pts',(-68.4367051682166,27.2822038034539,
12.));
#148813=CARTESIAN_POINT('Ctrl Pts',(-68.455648717044,27.301198151557,12.));
#148814=CARTESIAN_POINT('Ctrl Pts',(-68.4746005480993,27.3202357488153,
12.));
#148815=CARTESIAN_POINT('Ctrl Pts',(-68.4935605626362,27.3393165646748,
12.));
#148816=CARTESIAN_POINT('Ctrl Pts',(-68.5125286621888,27.3584405685941,
12.));
#148817=CARTESIAN_POINT('Ctrl Pts',(-68.5315047488035,27.3776077300914,
12.));
#148818=CARTESIAN_POINT('Ctrl Pts',(-68.5504887252975,27.3968180187941,
12.));
#148819=CARTESIAN_POINT('Ctrl Pts',(-68.5694804955014,27.4160714044831,
12.));
#148820=CARTESIAN_POINT('Ctrl Pts',(-68.5884799645218,27.4353678571361,
12.));
#148821=CARTESIAN_POINT('Ctrl Pts',(-68.6074870381619,27.4547073468226,
12.));
#148822=CARTESIAN_POINT('Ctrl Pts',(-68.6265016223561,27.4740898435988,
12.));
#148823=CARTESIAN_POINT('Ctrl Pts',(-68.645523622548,27.4935153173868,12.));
#148824=CARTESIAN_POINT('Ctrl Pts',(-68.6645529432045,27.5129837378791,
12.));
#148825=CARTESIAN_POINT('Ctrl Pts',(-68.6835894869882,27.5324950743706,
12.));
#148826=CARTESIAN_POINT('Ctrl Pts',(-68.7026331554296,27.5520492958907,
12.));
#148827=CARTESIAN_POINT('Ctrl Pts',(-68.7216838504218,27.5716463715004,
12.));
#148828=CARTESIAN_POINT('Ctrl Pts',(-68.740741475526,27.5912862705468,12.));
#148829=CARTESIAN_POINT('Ctrl Pts',(-68.7598059372129,27.6109689629029,
12.));
#148830=CARTESIAN_POINT('Ctrl Pts',(-68.7788771464713,27.6306944192737,
12.));
#148831=CARTESIAN_POINT('Ctrl Pts',(-68.7979550191872,27.6504626112666,
12.));
#148832=CARTESIAN_POINT('Ctrl Pts',(-68.8143140938915,27.6674443909983,
12.));
#148833=CARTESIAN_POINT('Ctrl Pts',(-68.8268597852179,27.6804870323434,
12.));
#148834=CARTESIAN_POINT('Ctrl Pts',(-68.8355891982106,27.6895716271274,
12.));
#148835=CARTESIAN_POINT('Ctrl Pts',(-68.8405004466159,27.6946856803718,
12.));
#148836=CARTESIAN_POINT('Ctrl Pts',(-68.8415926175085,27.6958230985044,
12.));
#148837=CARTESIAN_POINT('',(-65.4815644032299,24.7419628022042,0.));
#148838=CARTESIAN_POINT('',(-65.4815644032299,24.7419628022042,0.));
#148839=CARTESIAN_POINT('Ctrl Pts',(-68.8415926175085,27.6958230985044,
0.));
#148840=CARTESIAN_POINT('Ctrl Pts',(-68.8405004466159,27.6946856803718,
0.));
#148841=CARTESIAN_POINT('Ctrl Pts',(-68.8355891982106,27.6895716271274,
0.));
#148842=CARTESIAN_POINT('Ctrl Pts',(-68.8268597852179,27.6804870323434,
0.));
#148843=CARTESIAN_POINT('Ctrl Pts',(-68.8143140938915,27.6674443909983,
0.));
#148844=CARTESIAN_POINT('Ctrl Pts',(-68.7979550191872,27.6504626112666,
0.));
#148845=CARTESIAN_POINT('Ctrl Pts',(-68.7788771464713,27.6306944192737,
0.));
#148846=CARTESIAN_POINT('Ctrl Pts',(-68.7598059372129,27.6109689629029,
0.));
#148847=CARTESIAN_POINT('Ctrl Pts',(-68.740741475526,27.5912862705468,0.));
#148848=CARTESIAN_POINT('Ctrl Pts',(-68.7216838504218,27.5716463715004,
0.));
#148849=CARTESIAN_POINT('Ctrl Pts',(-68.7026331554296,27.5520492958907,
0.));
#148850=CARTESIAN_POINT('Ctrl Pts',(-68.6835894869882,27.5324950743706,
0.));
#148851=CARTESIAN_POINT('Ctrl Pts',(-68.6645529432045,27.5129837378791,
0.));
#148852=CARTESIAN_POINT('Ctrl Pts',(-68.645523622548,27.4935153173868,0.));
#148853=CARTESIAN_POINT('Ctrl Pts',(-68.6265016223561,27.4740898435988,
0.));
#148854=CARTESIAN_POINT('Ctrl Pts',(-68.6074870381619,27.4547073468226,
0.));
#148855=CARTESIAN_POINT('Ctrl Pts',(-68.5884799645218,27.4353678571361,
0.));
#148856=CARTESIAN_POINT('Ctrl Pts',(-68.5694804955014,27.4160714044831,
0.));
#148857=CARTESIAN_POINT('Ctrl Pts',(-68.5504887252975,27.3968180187941,
0.));
#148858=CARTESIAN_POINT('Ctrl Pts',(-68.5315047488035,27.3776077300914,
0.));
#148859=CARTESIAN_POINT('Ctrl Pts',(-68.5125286621888,27.3584405685941,
0.));
#148860=CARTESIAN_POINT('Ctrl Pts',(-68.4935605626362,27.3393165646748,
0.));
#148861=CARTESIAN_POINT('Ctrl Pts',(-68.4746005480993,27.3202357488153,
0.));
#148862=CARTESIAN_POINT('Ctrl Pts',(-68.455648717044,27.301198151557,0.));
#148863=CARTESIAN_POINT('Ctrl Pts',(-68.4367051682166,27.2822038034539,
0.));
#148864=CARTESIAN_POINT('Ctrl Pts',(-68.4177700003471,27.2632527350062,
0.));
#148865=CARTESIAN_POINT('Ctrl Pts',(-68.398843312159,27.2443449766654,0.));
#148866=CARTESIAN_POINT('Ctrl Pts',(-68.379925202511,27.2254805588677,0.));
#148867=CARTESIAN_POINT('Ctrl Pts',(-68.3610157704999,27.2066595120544,
0.));
#148868=CARTESIAN_POINT('Ctrl Pts',(-68.3421151155708,27.1878818666925,
0.));
#148869=CARTESIAN_POINT('Ctrl Pts',(-68.3232233376415,27.1691476532917,
0.));
#148870=CARTESIAN_POINT('Ctrl Pts',(-68.3043405371589,27.150456902413,0.));
#148871=CARTESIAN_POINT('Ctrl Pts',(-68.285466815035,27.1318096446643,0.));
#148872=CARTESIAN_POINT('Ctrl Pts',(-68.2666022726094,27.1132059106939,
0.));
#148873=CARTESIAN_POINT('Ctrl Pts',(-68.2477470116014,27.0946457311813,
0.));
#148874=CARTESIAN_POINT('Ctrl Pts',(-68.2289011340624,27.076129136823,0.));
#148875=CARTESIAN_POINT('Ctrl Pts',(-68.2100647423345,27.0576561583179,
0.));
#148876=CARTESIAN_POINT('Ctrl Pts',(-68.1912379390787,27.0392268263804,
0.));
#148877=CARTESIAN_POINT('Ctrl Pts',(-68.1724208272967,27.0208411717477,
0.));
#148878=CARTESIAN_POINT('Ctrl Pts',(-68.1536135103558,27.0024992251839,
0.));
#148879=CARTESIAN_POINT('Ctrl Pts',(-68.13481609201,26.9842010174819,0.));
#148880=CARTESIAN_POINT('Ctrl Pts',(-68.1160286764244,26.9659465794596,
0.));
#148881=CARTESIAN_POINT('Ctrl Pts',(-68.0972513681739,26.9477359419646,
0.));
#148882=CARTESIAN_POINT('Ctrl Pts',(-68.0784842722362,26.9295691358775,
0.));
#148883=CARTESIAN_POINT('Ctrl Pts',(-68.0597274939857,26.9114461921109,
0.));
#148884=CARTESIAN_POINT('Ctrl Pts',(-68.0409811391872,26.8933671416064,
0.));
#148885=CARTESIAN_POINT('Ctrl Pts',(-68.0222453139862,26.8753320153255,
0.));
#148886=CARTESIAN_POINT('Ctrl Pts',(-68.0035201249108,26.85734084425,0.));
#148887=CARTESIAN_POINT('Ctrl Pts',(-67.9848056788814,26.8393936593914,
0.));
#148888=CARTESIAN_POINT('Ctrl Pts',(-67.9661020832165,26.8214904917922,
0.));
#148889=CARTESIAN_POINT('Ctrl Pts',(-67.9474094456395,26.8036313725262,
0.));
#148890=CARTESIAN_POINT('Ctrl Pts',(-67.9287278742839,26.7858163326932,
0.));
#148891=CARTESIAN_POINT('Ctrl Pts',(-67.9100574776974,26.7680454034168,
0.));
#148892=CARTESIAN_POINT('Ctrl Pts',(-67.8913983648441,26.7503186158523,
0.));
#148893=CARTESIAN_POINT('Ctrl Pts',(-67.8727506451068,26.7326360011886,
0.));
#148894=CARTESIAN_POINT('Ctrl Pts',(-67.8541144282875,26.7149975906478,
0.));
#148895=CARTESIAN_POINT('Ctrl Pts',(-67.8354898246079,26.6974034154803,
0.));
#148896=CARTESIAN_POINT('Ctrl Pts',(-67.8168769447086,26.6798535069586,
0.));
#148897=CARTESIAN_POINT('Ctrl Pts',(-67.7982758996557,26.6623478963867,
0.));
#148898=CARTESIAN_POINT('Ctrl Pts',(-67.7796868009447,26.6448866151027,
0.));
#148899=CARTESIAN_POINT('Ctrl Pts',(-67.7611097605042,26.6274696944793,
0.));
#148900=CARTESIAN_POINT('Ctrl Pts',(-67.7425448906983,26.6100971659204,
0.));
#148901=CARTESIAN_POINT('Ctrl Pts',(-67.7239923043295,26.5927690608546,
0.));
#148902=CARTESIAN_POINT('Ctrl Pts',(-67.7054521146427,26.5754854107422,
0.));
#148903=CARTESIAN_POINT('Ctrl Pts',(-67.6869244353292,26.5582462470794,
0.));
#148904=CARTESIAN_POINT('Ctrl Pts',(-67.6684093805288,26.5410516013984,
0.));
#148905=CARTESIAN_POINT('Ctrl Pts',(-67.6499070648323,26.5239015052655,
0.));
#148906=CARTESIAN_POINT('Ctrl Pts',(-67.6314176032823,26.506795990273,0.));
#148907=CARTESIAN_POINT('Ctrl Pts',(-67.6129411113774,26.4897350880446,
0.));
#148908=CARTESIAN_POINT('Ctrl Pts',(-67.5944777050782,26.4727188302415,
0.));
#148909=CARTESIAN_POINT('Ctrl Pts',(-67.5760275008096,26.4557472485622,
0.));
#148910=CARTESIAN_POINT('Ctrl Pts',(-67.5575906154648,26.4388203747422,
0.));
#148911=CARTESIAN_POINT('Ctrl Pts',(-67.5391671664055,26.4219382405452,
0.));
#148912=CARTESIAN_POINT('Ctrl Pts',(-67.5207572714666,26.4051008777669,
0.));
#148913=CARTESIAN_POINT('Ctrl Pts',(-67.5023610489611,26.3883083182417,
0.));
#148914=CARTESIAN_POINT('Ctrl Pts',(-67.4839786176833,26.3715605938432,
0.));
#148915=CARTESIAN_POINT('Ctrl Pts',(-67.4656100969121,26.3548577364835,
0.));
#148916=CARTESIAN_POINT('Ctrl Pts',(-67.4472556064127,26.3381997781059,
0.));
#148917=CARTESIAN_POINT('Ctrl Pts',(-67.4289152664406,26.3215867506864,
0.));
#148918=CARTESIAN_POINT('Ctrl Pts',(-67.4105891977465,26.305018686241,0.));
#148919=CARTESIAN_POINT('Ctrl Pts',(-67.392277521581,26.288495616827,0.));
#148920=CARTESIAN_POINT('Ctrl Pts',(-67.3739803596967,26.2720175745422,
0.));
#148921=CARTESIAN_POINT('Ctrl Pts',(-67.3556978343506,26.255584591518,0.));
#148922=CARTESIAN_POINT('Ctrl Pts',(-67.3374300683076,26.2391966999192,
0.));
#148923=CARTESIAN_POINT('Ctrl Pts',(-67.3191771848468,26.2228539319527,
0.));
#148924=CARTESIAN_POINT('Ctrl Pts',(-67.3009393077654,26.2065563198684,
0.));
#148925=CARTESIAN_POINT('Ctrl Pts',(-67.2827165613828,26.1903038959589,
0.));
#148926=CARTESIAN_POINT('Ctrl Pts',(-67.2645090705414,26.1740966925527,
0.));
#148927=CARTESIAN_POINT('Ctrl Pts',(-67.2463169606105,26.1579347420135,
0.));
#148928=CARTESIAN_POINT('Ctrl Pts',(-67.228140357493,26.1418180767487,0.));
#148929=CARTESIAN_POINT('Ctrl Pts',(-67.2099793876295,26.1257467292102,
0.));
#148930=CARTESIAN_POINT('Ctrl Pts',(-67.191834178002,26.109720731895,0.));
#148931=CARTESIAN_POINT('Ctrl Pts',(-67.1737048561364,26.0937401173385,
0.));
#148932=CARTESIAN_POINT('Ctrl Pts',(-67.1555915501052,26.0778049181129,
0.));
#148933=CARTESIAN_POINT('Ctrl Pts',(-67.1374943885353,26.061915166836,0.));
#148934=CARTESIAN_POINT('Ctrl Pts',(-67.1194135006122,26.0460708961725,
0.));
#148935=CARTESIAN_POINT('Ctrl Pts',(-67.101349016084,26.030272138834,0.));
#148936=CARTESIAN_POINT('Ctrl Pts',(-67.083301065264,26.0145189275733,0.));
#148937=CARTESIAN_POINT('Ctrl Pts',(-67.0652697790335,25.9988112951818,
0.));
#148938=CARTESIAN_POINT('Ctrl Pts',(-67.0472552888495,25.9831492744988,
0.));
#148939=CARTESIAN_POINT('Ctrl Pts',(-67.0292577267495,25.9675328984123,
0.));
#148940=CARTESIAN_POINT('Ctrl Pts',(-67.0112772253553,25.9519621998598,
0.));
#148941=CARTESIAN_POINT('Ctrl Pts',(-66.993313917876,25.9364372118216,0.));
#148942=CARTESIAN_POINT('Ctrl Pts',(-66.9753679381122,25.9209579673198,
0.));
#148943=CARTESIAN_POINT('Ctrl Pts',(-66.9574394204635,25.9055244994266,
0.));
#148944=CARTESIAN_POINT('Ctrl Pts',(-66.9395284999327,25.8901368412655,
0.));
#148945=CARTESIAN_POINT('Ctrl Pts',(-66.9216353121308,25.8747950260114,
0.));
#148946=CARTESIAN_POINT('Ctrl Pts',(-66.9037599932787,25.8594990868845,
0.));
#148947=CARTESIAN_POINT('Ctrl Pts',(-66.8859026802123,25.8442490571486,
0.));
#148948=CARTESIAN_POINT('Ctrl Pts',(-66.8680635103907,25.8290449701206,
0.));
#148949=CARTESIAN_POINT('Ctrl Pts',(-66.8502426219015,25.8138868591715,
0.));
#148950=CARTESIAN_POINT('Ctrl Pts',(-66.8324401534658,25.7987747577264,
0.));
#148951=CARTESIAN_POINT('Ctrl Pts',(-66.8146562444397,25.783708699258,0.));
#148952=CARTESIAN_POINT('Ctrl Pts',(-66.7968910348199,25.7686887172859,
0.));
#148953=CARTESIAN_POINT('Ctrl Pts',(-66.7791446652505,25.7537148453848,
0.));
#148954=CARTESIAN_POINT('Ctrl Pts',(-66.7614172770302,25.7387871171861,
0.));
#148955=CARTESIAN_POINT('Ctrl Pts',(-66.7437090121168,25.7239055663778,
0.));
#148956=CARTESIAN_POINT('Ctrl Pts',(-66.72602001313,25.7090702266976,0.));
#148957=CARTESIAN_POINT('Ctrl Pts',(-66.7083504233566,25.6942811319337,
0.));
#148958=CARTESIAN_POINT('Ctrl Pts',(-66.6907003867599,25.6795383159329,
0.));
#148959=CARTESIAN_POINT('Ctrl Pts',(-66.6730700479844,25.6648418126016,
0.));
#148960=CARTESIAN_POINT('Ctrl Pts',(-66.6554595523611,25.650191655905,0.));
#148961=CARTESIAN_POINT('Ctrl Pts',(-66.6378690459105,25.6355878798605,
0.));
#148962=CARTESIAN_POINT('Ctrl Pts',(-66.6202986753482,25.6210305185394,
0.));
#148963=CARTESIAN_POINT('Ctrl Pts',(-66.6027485880947,25.606519606075,0.));
#148964=CARTESIAN_POINT('Ctrl Pts',(-66.5852189322811,25.5920551766629,
0.));
#148965=CARTESIAN_POINT('Ctrl Pts',(-66.5677098567551,25.5776372645605,
0.));
#148966=CARTESIAN_POINT('Ctrl Pts',(-66.5502215110843,25.5632659040797,
0.));
#148967=CARTESIAN_POINT('Ctrl Pts',(-66.5327540455639,25.5489411295916,
0.));
#148968=CARTESIAN_POINT('Ctrl Pts',(-66.5153076112237,25.5346629755322,
0.));
#148969=CARTESIAN_POINT('Ctrl Pts',(-66.4978823598352,25.5204314764033,
0.));
#148970=CARTESIAN_POINT('Ctrl Pts',(-66.4804784439146,25.5062466667703,
0.));
#148971=CARTESIAN_POINT('Ctrl Pts',(-66.463096016725,25.4921085812548,0.));
#148972=CARTESIAN_POINT('Ctrl Pts',(-66.445735232287,25.4780172545418,0.));
#148973=CARTESIAN_POINT('Ctrl Pts',(-66.4283962453899,25.463972721385,0.));
#148974=CARTESIAN_POINT('Ctrl Pts',(-66.4110792116,25.4499750166079,0.));
#148975=CARTESIAN_POINT('Ctrl Pts',(-66.3937842872684,25.4360241751017,
0.));
#148976=CARTESIAN_POINT('Ctrl Pts',(-66.3765116295364,25.4221202318198,
0.));
#148977=CARTESIAN_POINT('Ctrl Pts',(-66.3592613963407,25.4082632217846,
0.));
#148978=CARTESIAN_POINT('Ctrl Pts',(-66.3420337464176,25.39445318009,0.));
#148979=CARTESIAN_POINT('Ctrl Pts',(-66.3248288393046,25.3806901419012,
0.));
#148980=CARTESIAN_POINT('Ctrl Pts',(-66.3076468353417,25.366974142449,0.));
#148981=CARTESIAN_POINT('Ctrl Pts',(-66.2904878956721,25.3533052170253,
0.));
#148982=CARTESIAN_POINT('Ctrl Pts',(-66.2733521822675,25.3396834009954,
0.));
#148983=CARTESIAN_POINT('Ctrl Pts',(-66.2562398579479,25.3261087298029,
0.));
#148984=CARTESIAN_POINT('Ctrl Pts',(-66.2391510863992,25.3125812389727,
0.));
#148985=CARTESIAN_POINT('Ctrl Pts',(-66.2220860321931,25.2991009641086,
0.));
#148986=CARTESIAN_POINT('Ctrl Pts',(-66.2050448607883,25.285667940892,0.));
#148987=CARTESIAN_POINT('Ctrl Pts',(-66.1880277385114,25.2722822050828,
0.));
#148988=CARTESIAN_POINT('Ctrl Pts',(-66.1710348325378,25.2589437925145,
0.));
#148989=CARTESIAN_POINT('Ctrl Pts',(-66.1540663108767,25.245652739088,0.));
#148990=CARTESIAN_POINT('Ctrl Pts',(-66.1371223423372,25.232409080756,0.));
#148991=CARTESIAN_POINT('Ctrl Pts',(-66.1202030965785,25.2192128535367,
0.));
#148992=CARTESIAN_POINT('Ctrl Pts',(-66.1033087441916,25.2060640935371,
0.));
#148993=CARTESIAN_POINT('Ctrl Pts',(-66.086439456768,25.1929628369685,0.));
#148994=CARTESIAN_POINT('Ctrl Pts',(-66.0695954069699,25.1799091201594,
0.));
#148995=CARTESIAN_POINT('Ctrl Pts',(-66.0527767686,25.1669029795651,0.));
#148996=CARTESIAN_POINT('Ctrl Pts',(-66.0359837164709,25.1539444517409,
0.));
#148997=CARTESIAN_POINT('Ctrl Pts',(-66.0192164262607,25.1410335733094,
0.));
#148998=CARTESIAN_POINT('Ctrl Pts',(-66.0024750743902,25.1281703809299,
0.));
#148999=CARTESIAN_POINT('Ctrl Pts',(-65.9857598378455,25.1153549112511,
0.));
#149000=CARTESIAN_POINT('Ctrl Pts',(-65.9690708941591,25.1025872009016,
0.));
#149001=CARTESIAN_POINT('Ctrl Pts',(-65.9524084218167,25.0898672865926,
0.));
#149002=CARTESIAN_POINT('Ctrl Pts',(-65.9357726006174,25.0771952052032,
0.));
#149003=CARTESIAN_POINT('Ctrl Pts',(-65.9191636119796,25.0645709938519,
0.));
#149004=CARTESIAN_POINT('Ctrl Pts',(-65.9025816394391,25.0519946900066,
0.));
#149005=CARTESIAN_POINT('Ctrl Pts',(-65.8860268683088,25.039466331404,0.));
#149006=CARTESIAN_POINT('Ctrl Pts',(-65.8694994847587,25.0269859558351,
0.));
#149007=CARTESIAN_POINT('Ctrl Pts',(-65.8529996750441,25.0145536009603,
0.));
#149008=CARTESIAN_POINT('Ctrl Pts',(-65.8365276247157,25.0021693041181,
0.));
#149009=CARTESIAN_POINT('Ctrl Pts',(-65.8200835177071,24.9898331021002,
0.));
#149010=CARTESIAN_POINT('Ctrl Pts',(-65.8036675380761,24.97754503157,0.));
#149011=CARTESIAN_POINT('Ctrl Pts',(-65.7872798720847,24.965305129559,0.));
#149012=CARTESIAN_POINT('Ctrl Pts',(-65.7709207098949,24.9531134338693,
0.));
#149013=CARTESIAN_POINT('Ctrl Pts',(-65.7545902480286,24.9409699836523,
0.));
#149014=CARTESIAN_POINT('Ctrl Pts',(-65.7382886895839,24.9288748194562,
0.));
#149015=CARTESIAN_POINT('Ctrl Pts',(-65.7220162391016,24.9168279820093,
0.));
#149016=CARTESIAN_POINT('Ctrl Pts',(-65.7057730980471,24.9048295111444,
0.));
#149017=CARTESIAN_POINT('Ctrl Pts',(-65.6895594608798,24.8928794448615,
0.));
#149018=CARTESIAN_POINT('Ctrl Pts',(-65.6733755087724,24.8809778178248,
0.));
#149019=CARTESIAN_POINT('Ctrl Pts',(-65.6572214156761,24.869124662808,0.));
#149020=CARTESIAN_POINT('Ctrl Pts',(-65.6410973603713,24.8573200135683,
0.));
#149021=CARTESIAN_POINT('Ctrl Pts',(-65.6250035361612,24.8455639071517,
0.));
#149022=CARTESIAN_POINT('Ctrl Pts',(-65.6089401625552,24.8338563866739,
0.));
#149023=CARTESIAN_POINT('Ctrl Pts',(-65.5929074932487,24.8221975032059,
0.));
#149024=CARTESIAN_POINT('Ctrl Pts',(-65.5769057914184,24.8105873098578,
0.));
#149025=CARTESIAN_POINT('Ctrl Pts',(-65.560935306275,24.7990258561234,0.));
#149026=CARTESIAN_POINT('Ctrl Pts',(-65.5449962514735,24.7875131827515,
0.));
#149027=CARTESIAN_POINT('Ctrl Pts',(-65.5290887770494,24.776049314855,0.));
#149028=CARTESIAN_POINT('Ctrl Pts',(-65.5132129675727,24.7646342620969,
0.));
#149029=CARTESIAN_POINT('Ctrl Pts',(-65.5005376841469,24.755541272477,0.));
#149030=CARTESIAN_POINT('Ctrl Pts',(-65.4910454936487,24.7487434956058,
0.));
#149031=CARTESIAN_POINT('Ctrl Pts',(-65.484723709553,24.7442214063411,0.));
#149032=CARTESIAN_POINT('Ctrl Pts',(-65.4815644032299,24.7419628022042,
0.));
#149033=CARTESIAN_POINT('Ctrl Pts',(-66.3684712863594,33.8448817269567,
0.));
#149034=CARTESIAN_POINT('Ctrl Pts',(-66.3684712863594,33.8448817269567,
12.));
#149035=CARTESIAN_POINT('Ctrl Pts',(-66.3650082659713,33.8404862618869,
0.));
#149036=CARTESIAN_POINT('Ctrl Pts',(-66.3650082659713,33.8404862618869,
12.));
#149037=CARTESIAN_POINT('Ctrl Pts',(-66.3580824155893,33.8316996011932,
0.));
#149038=CARTESIAN_POINT('Ctrl Pts',(-66.3580824155893,33.8316996011932,
12.));
#149039=CARTESIAN_POINT('Ctrl Pts',(-66.3476942112,33.8185324184903,0.));
#149040=CARTESIAN_POINT('Ctrl Pts',(-66.3476942112,33.8185324184903,12.));
#149041=CARTESIAN_POINT('Ctrl Pts',(-66.3338444144211,33.8010017926027,
0.));
#149042=CARTESIAN_POINT('Ctrl Pts',(-66.3338444144211,33.8010017926027,
12.));
#149043=CARTESIAN_POINT('Ctrl Pts',(-66.3165340771611,33.7791312145108,
0.));
#149044=CARTESIAN_POINT('Ctrl Pts',(-66.3165340771611,33.7791312145108,
12.));
#149045=CARTESIAN_POINT('Ctrl Pts',(-66.2992256621336,33.7573033544559,
0.));
#149046=CARTESIAN_POINT('Ctrl Pts',(-66.2992256621336,33.7573033544559,
12.));
#149047=CARTESIAN_POINT('Ctrl Pts',(-66.2819191962353,33.7355182321907,
0.));
#149048=CARTESIAN_POINT('Ctrl Pts',(-66.2819191962353,33.7355182321907,
12.));
#149049=CARTESIAN_POINT('Ctrl Pts',(-66.2646147235322,33.7137758735902,
0.));
#149050=CARTESIAN_POINT('Ctrl Pts',(-66.2646147235322,33.7137758735902,
12.));
#149051=CARTESIAN_POINT('Ctrl Pts',(-66.2473123109395,33.6920763111448,
0.));
#149052=CARTESIAN_POINT('Ctrl Pts',(-66.2473123109395,33.6920763111448,
12.));
#149053=CARTESIAN_POINT('Ctrl Pts',(-66.2300120464082,33.6704195830392,
0.));
#149054=CARTESIAN_POINT('Ctrl Pts',(-66.2300120464082,33.6704195830392,
12.));
#149055=CARTESIAN_POINT('Ctrl Pts',(-66.2127140313598,33.6488057311532,
0.));
#149056=CARTESIAN_POINT('Ctrl Pts',(-66.2127140313598,33.6488057311532,
12.));
#149057=CARTESIAN_POINT('Ctrl Pts',(-66.1954183747089,33.6272347993476,
0.));
#149058=CARTESIAN_POINT('Ctrl Pts',(-66.1954183747089,33.6272347993476,
12.));
#149059=CARTESIAN_POINT('Ctrl Pts',(-66.1781251864017,33.6057068316769,
0.));
#149060=CARTESIAN_POINT('Ctrl Pts',(-66.1781251864017,33.6057068316769,
12.));
#149061=CARTESIAN_POINT('Ctrl Pts',(-66.1608345707637,33.584221870515,0.));
#149062=CARTESIAN_POINT('Ctrl Pts',(-66.1608345707637,33.584221870515,12.));
#149063=CARTESIAN_POINT('Ctrl Pts',(-66.1435466211076,33.5627799550483,
0.));
#149064=CARTESIAN_POINT('Ctrl Pts',(-66.1435466211076,33.5627799550483,
12.));
#149065=CARTESIAN_POINT('Ctrl Pts',(-66.1262614234675,33.541381122345,0.));
#149066=CARTESIAN_POINT('Ctrl Pts',(-66.1262614234675,33.541381122345,12.));
#149067=CARTESIAN_POINT('Ctrl Pts',(-66.1089790592729,33.5200254081243,
0.));
#149068=CARTESIAN_POINT('Ctrl Pts',(-66.1089790592729,33.5200254081243,
12.));
#149069=CARTESIAN_POINT('Ctrl Pts',(-66.0916996085245,33.4987128476622,
0.));
#149070=CARTESIAN_POINT('Ctrl Pts',(-66.0916996085245,33.4987128476622,
12.));
#149071=CARTESIAN_POINT('Ctrl Pts',(-66.0744231525415,33.4774434765745,
0.));
#149072=CARTESIAN_POINT('Ctrl Pts',(-66.0744231525415,33.4774434765745,
12.));
#149073=CARTESIAN_POINT('Ctrl Pts',(-66.0571497774434,33.4562173318025,
0.));
#149074=CARTESIAN_POINT('Ctrl Pts',(-66.0571497774434,33.4562173318025,
12.));
#149075=CARTESIAN_POINT('Ctrl Pts',(-66.0398795737777,33.43503445151,0.));
#149076=CARTESIAN_POINT('Ctrl Pts',(-66.0398795737777,33.43503445151,12.));
#149077=CARTESIAN_POINT('Ctrl Pts',(-66.0226126349446,33.4138948746388,
0.));
#149078=CARTESIAN_POINT('Ctrl Pts',(-66.0226126349446,33.4138948746388,
12.));
#149079=CARTESIAN_POINT('Ctrl Pts',(-66.0053490559812,33.3927986405605,
0.));
#149080=CARTESIAN_POINT('Ctrl Pts',(-66.0053490559812,33.3927986405605,
12.));
#149081=CARTESIAN_POINT('Ctrl Pts',(-65.9880889322831,33.37174578871,0.));
#149082=CARTESIAN_POINT('Ctrl Pts',(-65.9880889322831,33.37174578871,12.));
#149083=CARTESIAN_POINT('Ctrl Pts',(-65.970832358141,33.3507363581592,0.));
#149084=CARTESIAN_POINT('Ctrl Pts',(-65.970832358141,33.3507363581592,12.));
#149085=CARTESIAN_POINT('Ctrl Pts',(-65.9535794260831,33.3297703874265,
0.));
#149086=CARTESIAN_POINT('Ctrl Pts',(-65.9535794260831,33.3297703874265,
12.));
#149087=CARTESIAN_POINT('Ctrl Pts',(-65.9363302276846,33.3088479147164,
0.));
#149088=CARTESIAN_POINT('Ctrl Pts',(-65.9363302276846,33.3088479147164,
12.));
#149089=CARTESIAN_POINT('Ctrl Pts',(-65.9190848540433,33.2879689780572,
0.));
#149090=CARTESIAN_POINT('Ctrl Pts',(-65.9190848540433,33.2879689780572,
12.));
#149091=CARTESIAN_POINT('Ctrl Pts',(-65.9018433963889,33.2671336154753,
0.));
#149092=CARTESIAN_POINT('Ctrl Pts',(-65.9018433963889,33.2671336154753,
12.));
#149093=CARTESIAN_POINT('Ctrl Pts',(-65.8846059466372,33.2463418651492,
0.));
#149094=CARTESIAN_POINT('Ctrl Pts',(-65.8846059466372,33.2463418651492,
12.));
#149095=CARTESIAN_POINT('Ctrl Pts',(-65.8673725979578,33.2255937655649,
0.));
#149096=CARTESIAN_POINT('Ctrl Pts',(-65.8673725979578,33.2255937655649,
12.));
#149097=CARTESIAN_POINT('Ctrl Pts',(-65.8501434445164,33.2048893554491,
0.));
#149098=CARTESIAN_POINT('Ctrl Pts',(-65.8501434445164,33.2048893554491,
12.));
#149099=CARTESIAN_POINT('Ctrl Pts',(-65.8329185812375,33.1842286737051,
0.));
#149100=CARTESIAN_POINT('Ctrl Pts',(-65.8329185812375,33.1842286737051,
12.));
#149101=CARTESIAN_POINT('Ctrl Pts',(-65.8156981035503,33.16361175934,0.));
#149102=CARTESIAN_POINT('Ctrl Pts',(-65.8156981035503,33.16361175934,12.));
#149103=CARTESIAN_POINT('Ctrl Pts',(-65.7984821071623,33.1430386513976,
0.));
#149104=CARTESIAN_POINT('Ctrl Pts',(-65.7984821071623,33.1430386513976,
12.));
#149105=CARTESIAN_POINT('Ctrl Pts',(-65.7812706877697,33.1225093888671,
0.));
#149106=CARTESIAN_POINT('Ctrl Pts',(-65.7812706877697,33.1225093888671,
12.));
#149107=CARTESIAN_POINT('Ctrl Pts',(-65.7640639410661,33.1020240106884,
0.));
#149108=CARTESIAN_POINT('Ctrl Pts',(-65.7640639410661,33.1020240106884,
12.));
#149109=CARTESIAN_POINT('Ctrl Pts',(-65.7468619628816,33.081582555798,0.));
#149110=CARTESIAN_POINT('Ctrl Pts',(-65.7468619628816,33.081582555798,12.));
#149111=CARTESIAN_POINT('Ctrl Pts',(-65.7296648492825,33.0611850631582,
0.));
#149112=CARTESIAN_POINT('Ctrl Pts',(-65.7296648492825,33.0611850631582,
12.));
#149113=CARTESIAN_POINT('Ctrl Pts',(-65.7124726966802,33.0408315717873,
0.));
#149114=CARTESIAN_POINT('Ctrl Pts',(-65.7124726966802,33.0408315717873,
12.));
#149115=CARTESIAN_POINT('Ctrl Pts',(-65.6952856019533,33.0205221207872,
0.));
#149116=CARTESIAN_POINT('Ctrl Pts',(-65.6952856019533,33.0205221207872,
12.));
#149117=CARTESIAN_POINT('Ctrl Pts',(-65.6781036625027,33.0002567493573,
0.));
#149118=CARTESIAN_POINT('Ctrl Pts',(-65.6781036625027,33.0002567493573,
12.));
#149119=CARTESIAN_POINT('Ctrl Pts',(-65.6609269761889,32.9800354967839,
0.));
#149120=CARTESIAN_POINT('Ctrl Pts',(-65.6609269761889,32.9800354967839,
12.));
#149121=CARTESIAN_POINT('Ctrl Pts',(-65.6437556412947,32.9598584024312,
0.));
#149122=CARTESIAN_POINT('Ctrl Pts',(-65.6437556412947,32.9598584024312,
12.));
#149123=CARTESIAN_POINT('Ctrl Pts',(-65.6265897564783,32.9397255057274,
0.));
#149124=CARTESIAN_POINT('Ctrl Pts',(-65.6265897564783,32.9397255057274,
12.));
#149125=CARTESIAN_POINT('Ctrl Pts',(-65.6094294207276,32.9196368461463,
0.));
#149126=CARTESIAN_POINT('Ctrl Pts',(-65.6094294207276,32.9196368461463,
12.));
#149127=CARTESIAN_POINT('Ctrl Pts',(-65.5922747333194,32.8995924631898,
0.));
#149128=CARTESIAN_POINT('Ctrl Pts',(-65.5922747333194,32.8995924631898,
12.));
#149129=CARTESIAN_POINT('Ctrl Pts',(-65.5751257938473,32.879592396403,0.));
#149130=CARTESIAN_POINT('Ctrl Pts',(-65.5751257938473,32.879592396403,12.));
#149131=CARTESIAN_POINT('Ctrl Pts',(-65.5579827022421,32.8596366853832,
0.));
#149132=CARTESIAN_POINT('Ctrl Pts',(-65.5579827022421,32.8596366853832,
12.));
#149133=CARTESIAN_POINT('Ctrl Pts',(-65.5408455587965,32.8397253697865,
0.));
#149134=CARTESIAN_POINT('Ctrl Pts',(-65.5408455587965,32.8397253697865,
12.));
#149135=CARTESIAN_POINT('Ctrl Pts',(-65.5237144641858,32.8198584893315,
0.));
#149136=CARTESIAN_POINT('Ctrl Pts',(-65.5237144641858,32.8198584893315,
12.));
#149137=CARTESIAN_POINT('Ctrl Pts',(-65.5065895194929,32.8000360837974,
0.));
#149138=CARTESIAN_POINT('Ctrl Pts',(-65.5065895194929,32.8000360837974,
12.));
#149139=CARTESIAN_POINT('Ctrl Pts',(-65.4894708262061,32.7802581930287,
0.));
#149140=CARTESIAN_POINT('Ctrl Pts',(-65.4894708262061,32.7802581930287,
12.));
#149141=CARTESIAN_POINT('Ctrl Pts',(-65.4723584862122,32.7605248569378,
0.));
#149142=CARTESIAN_POINT('Ctrl Pts',(-65.4723584862122,32.7605248569378,
12.));
#149143=CARTESIAN_POINT('Ctrl Pts',(-65.4552526017905,32.7408361155037,
0.));
#149144=CARTESIAN_POINT('Ctrl Pts',(-65.4552526017905,32.7408361155037,
12.));
#149145=CARTESIAN_POINT('Ctrl Pts',(-65.4381532756065,32.7211920087683,
0.));
#149146=CARTESIAN_POINT('Ctrl Pts',(-65.4381532756065,32.7211920087683,
12.));
#149147=CARTESIAN_POINT('Ctrl Pts',(-65.4210606107035,32.7015925768265,
0.));
#149148=CARTESIAN_POINT('Ctrl Pts',(-65.4210606107035,32.7015925768265,
12.));
#149149=CARTESIAN_POINT('Ctrl Pts',(-65.4039747105039,32.6820378598267,
0.));
#149150=CARTESIAN_POINT('Ctrl Pts',(-65.4039747105039,32.6820378598267,
12.));
#149151=CARTESIAN_POINT('Ctrl Pts',(-65.3868956788182,32.662527897981,0.));
#149152=CARTESIAN_POINT('Ctrl Pts',(-65.3868956788182,32.662527897981,12.));
#149153=CARTESIAN_POINT('Ctrl Pts',(-65.3698236198513,32.6430627315674,
0.));
#149154=CARTESIAN_POINT('Ctrl Pts',(-65.3698236198513,32.6430627315674,
12.));
#149155=CARTESIAN_POINT('Ctrl Pts',(-65.3527586382081,32.6236424009301,
0.));
#149156=CARTESIAN_POINT('Ctrl Pts',(-65.3527586382081,32.6236424009301,
12.));
#149157=CARTESIAN_POINT('Ctrl Pts',(-65.3357008389004,32.604266946475,0.));
#149158=CARTESIAN_POINT('Ctrl Pts',(-65.3357008389004,32.604266946475,12.));
#149159=CARTESIAN_POINT('Ctrl Pts',(-65.31865032735,32.5849364086678,0.));
#149160=CARTESIAN_POINT('Ctrl Pts',(-65.31865032735,32.5849364086678,12.));
#149161=CARTESIAN_POINT('Ctrl Pts',(-65.3016072093912,32.5656508280421,
0.));
#149162=CARTESIAN_POINT('Ctrl Pts',(-65.3016072093912,32.5656508280421,
12.));
#149163=CARTESIAN_POINT('Ctrl Pts',(-65.2845715912721,32.5464102452014,
0.));
#149164=CARTESIAN_POINT('Ctrl Pts',(-65.2845715912721,32.5464102452014,
12.));
#149165=CARTESIAN_POINT('Ctrl Pts',(-65.2675435796558,32.5272147008191,
0.));
#149166=CARTESIAN_POINT('Ctrl Pts',(-65.2675435796558,32.5272147008191,
12.));
#149167=CARTESIAN_POINT('Ctrl Pts',(-65.2505232816209,32.5080642356328,
0.));
#149168=CARTESIAN_POINT('Ctrl Pts',(-65.2505232816209,32.5080642356328,
12.));
#149169=CARTESIAN_POINT('Ctrl Pts',(-65.2335108046614,32.4889588904392,
0.));
#149170=CARTESIAN_POINT('Ctrl Pts',(-65.2335108046614,32.4889588904392,
12.));
#149171=CARTESIAN_POINT('Ctrl Pts',(-65.2165062566924,32.4698987061032,
0.));
#149172=CARTESIAN_POINT('Ctrl Pts',(-65.2165062566924,32.4698987061032,
12.));
#149173=CARTESIAN_POINT('Ctrl Pts',(-65.1995097460538,32.450883723561,0.));
#149174=CARTESIAN_POINT('Ctrl Pts',(-65.1995097460538,32.450883723561,12.));
#149175=CARTESIAN_POINT('Ctrl Pts',(-65.182521381514,32.4319139838212,0.));
#149176=CARTESIAN_POINT('Ctrl Pts',(-65.182521381514,32.4319139838212,12.));
#149177=CARTESIAN_POINT('Ctrl Pts',(-65.1655412722726,32.4129895279615,
0.));
#149178=CARTESIAN_POINT('Ctrl Pts',(-65.1655412722726,32.4129895279615,
12.));
#149179=CARTESIAN_POINT('Ctrl Pts',(-65.1485695279635,32.3941103971221,
0.));
#149180=CARTESIAN_POINT('Ctrl Pts',(-65.1485695279635,32.3941103971221,
12.));
#149181=CARTESIAN_POINT('Ctrl Pts',(-65.1316062586588,32.3752766325136,
0.));
#149182=CARTESIAN_POINT('Ctrl Pts',(-65.1316062586588,32.3752766325136,
12.));
#149183=CARTESIAN_POINT('Ctrl Pts',(-65.1146515748722,32.3564882754212,
0.));
#149184=CARTESIAN_POINT('Ctrl Pts',(-65.1146515748722,32.3564882754212,
12.));
#149185=CARTESIAN_POINT('Ctrl Pts',(-65.0977055875608,32.3377453672051,
0.));
#149186=CARTESIAN_POINT('Ctrl Pts',(-65.0977055875608,32.3377453672051,
12.));
#149187=CARTESIAN_POINT('Ctrl Pts',(-65.0807684081282,32.3190479492987,
0.));
#149188=CARTESIAN_POINT('Ctrl Pts',(-65.0807684081282,32.3190479492987,
12.));
#149189=CARTESIAN_POINT('Ctrl Pts',(-65.0638401484257,32.3003960632006,
0.));
#149190=CARTESIAN_POINT('Ctrl Pts',(-65.0638401484257,32.3003960632006,
12.));
#149191=CARTESIAN_POINT('Ctrl Pts',(-65.0469209207563,32.2817897504807,
0.));
#149192=CARTESIAN_POINT('Ctrl Pts',(-65.0469209207563,32.2817897504807,
12.));
#149193=CARTESIAN_POINT('Ctrl Pts',(-65.03001083788,32.2632290527862,0.));
#149194=CARTESIAN_POINT('Ctrl Pts',(-65.03001083788,32.2632290527862,12.));
#149195=CARTESIAN_POINT('Ctrl Pts',(-65.0131100130158,32.2447140118422,
0.));
#149196=CARTESIAN_POINT('Ctrl Pts',(-65.0131100130158,32.2447140118422,
12.));
#149197=CARTESIAN_POINT('Ctrl Pts',(-64.9962185598462,32.2262446694512,
0.));
#149198=CARTESIAN_POINT('Ctrl Pts',(-64.9962185598462,32.2262446694512,
12.));
#149199=CARTESIAN_POINT('Ctrl Pts',(-64.9793365925178,32.207821067485,0.));
#149200=CARTESIAN_POINT('Ctrl Pts',(-64.9793365925178,32.207821067485,12.));
#149201=CARTESIAN_POINT('Ctrl Pts',(-64.9624642256461,32.189443247888,0.));
#149202=CARTESIAN_POINT('Ctrl Pts',(-64.9624642256461,32.189443247888,12.));
#149203=CARTESIAN_POINT('Ctrl Pts',(-64.9456015743193,32.1711112526854,
0.));
#149204=CARTESIAN_POINT('Ctrl Pts',(-64.9456015743193,32.1711112526854,
12.));
#149205=CARTESIAN_POINT('Ctrl Pts',(-64.9287487541015,32.152825123983,0.));
#149206=CARTESIAN_POINT('Ctrl Pts',(-64.9287487541015,32.152825123983,12.));
#149207=CARTESIAN_POINT('Ctrl Pts',(-64.9119058810367,32.1345849039674,
0.));
#149208=CARTESIAN_POINT('Ctrl Pts',(-64.9119058810367,32.1345849039674,
12.));
#149209=CARTESIAN_POINT('Ctrl Pts',(-64.8950730716501,32.1163906348983,
0.));
#149210=CARTESIAN_POINT('Ctrl Pts',(-64.8950730716501,32.1163906348983,
12.));
#149211=CARTESIAN_POINT('Ctrl Pts',(-64.8782504429527,32.0982423591112,
0.));
#149212=CARTESIAN_POINT('Ctrl Pts',(-64.8782504429527,32.0982423591112,
12.));
#149213=CARTESIAN_POINT('Ctrl Pts',(-64.8614381124455,32.0801401190244,
0.));
#149214=CARTESIAN_POINT('Ctrl Pts',(-64.8614381124455,32.0801401190244,
12.));
#149215=CARTESIAN_POINT('Ctrl Pts',(-64.8446361981234,32.0620839571409,
0.));
#149216=CARTESIAN_POINT('Ctrl Pts',(-64.8446361981234,32.0620839571409,
12.));
#149217=CARTESIAN_POINT('Ctrl Pts',(-64.8278448184785,32.0440739160476,
0.));
#149218=CARTESIAN_POINT('Ctrl Pts',(-64.8278448184785,32.0440739160476,
12.));
#149219=CARTESIAN_POINT('Ctrl Pts',(-64.8110640925021,32.0261100384092,
0.));
#149220=CARTESIAN_POINT('Ctrl Pts',(-64.8110640925021,32.0261100384092,
12.));
#149221=CARTESIAN_POINT('Ctrl Pts',(-64.7942941396883,32.0081923669677,
0.));
#149222=CARTESIAN_POINT('Ctrl Pts',(-64.7942941396883,32.0081923669677,
12.));
#149223=CARTESIAN_POINT('Ctrl Pts',(-64.7775350800405,31.9903209445521,
0.));
#149224=CARTESIAN_POINT('Ctrl Pts',(-64.7775350800405,31.9903209445521,
12.));
#149225=CARTESIAN_POINT('Ctrl Pts',(-64.7607870340738,31.972495814079,0.));
#149226=CARTESIAN_POINT('Ctrl Pts',(-64.7607870340738,31.972495814079,12.));
#149227=CARTESIAN_POINT('Ctrl Pts',(-64.7440501228201,31.9547170185533,
0.));
#149228=CARTESIAN_POINT('Ctrl Pts',(-64.7440501228201,31.9547170185533,
12.));
#149229=CARTESIAN_POINT('Ctrl Pts',(-64.727324467829,31.9369846010613,0.));
#149230=CARTESIAN_POINT('Ctrl Pts',(-64.727324467829,31.9369846010613,12.));
#149231=CARTESIAN_POINT('Ctrl Pts',(-64.7106101911723,31.9192986047702,
0.));
#149232=CARTESIAN_POINT('Ctrl Pts',(-64.7106101911723,31.9192986047702,
12.));
#149233=CARTESIAN_POINT('Ctrl Pts',(-64.6939074154491,31.9016590729371,
0.));
#149234=CARTESIAN_POINT('Ctrl Pts',(-64.6939074154491,31.9016590729371,
12.));
#149235=CARTESIAN_POINT('Ctrl Pts',(-64.6772162637905,31.8840660489106,
0.));
#149236=CARTESIAN_POINT('Ctrl Pts',(-64.6772162637905,31.8840660489106,
12.));
#149237=CARTESIAN_POINT('Ctrl Pts',(-64.6605368598631,31.8665195761311,
0.));
#149238=CARTESIAN_POINT('Ctrl Pts',(-64.6605368598631,31.8665195761311,
12.));
#149239=CARTESIAN_POINT('Ctrl Pts',(-64.6438693278718,31.849019698125,0.));
#149240=CARTESIAN_POINT('Ctrl Pts',(-64.6438693278718,31.849019698125,12.));
#149241=CARTESIAN_POINT('Ctrl Pts',(-64.627213792563,31.8315664585027,0.));
#149242=CARTESIAN_POINT('Ctrl Pts',(-64.627213792563,31.8315664585027,12.));
#149243=CARTESIAN_POINT('Ctrl Pts',(-64.6105703792312,31.8141599009684,
0.));
#149244=CARTESIAN_POINT('Ctrl Pts',(-64.6105703792312,31.8141599009684,
12.));
#149245=CARTESIAN_POINT('Ctrl Pts',(-64.5939392137233,31.7968000693218,
0.));
#149246=CARTESIAN_POINT('Ctrl Pts',(-64.5939392137233,31.7968000693218,
12.));
#149247=CARTESIAN_POINT('Ctrl Pts',(-64.5773204224429,31.7794870074583,
0.));
#149248=CARTESIAN_POINT('Ctrl Pts',(-64.5773204224429,31.7794870074583,
12.));
#149249=CARTESIAN_POINT('Ctrl Pts',(-64.5607141323527,31.7622207593637,
0.));
#149250=CARTESIAN_POINT('Ctrl Pts',(-64.5607141323527,31.7622207593637,
12.));
#149251=CARTESIAN_POINT('Ctrl Pts',(-64.544120470978,31.7450013691116,0.));
#149252=CARTESIAN_POINT('Ctrl Pts',(-64.544120470978,31.7450013691116,12.));
#149253=CARTESIAN_POINT('Ctrl Pts',(-64.5275395664134,31.7278288808736,
0.));
#149254=CARTESIAN_POINT('Ctrl Pts',(-64.5275395664134,31.7278288808736,
12.));
#149255=CARTESIAN_POINT('Ctrl Pts',(-64.5109715473277,31.7107033389204,
0.));
#149256=CARTESIAN_POINT('Ctrl Pts',(-64.5109715473277,31.7107033389204,
12.));
#149257=CARTESIAN_POINT('Ctrl Pts',(-64.4944165429672,31.6936247876228,
0.));
#149258=CARTESIAN_POINT('Ctrl Pts',(-64.4944165429672,31.6936247876228,
12.));
#149259=CARTESIAN_POINT('Ctrl Pts',(-64.4778746831598,31.6765932714456,
0.));
#149260=CARTESIAN_POINT('Ctrl Pts',(-64.4778746831598,31.6765932714456,
12.));
#149261=CARTESIAN_POINT('Ctrl Pts',(-64.4613460983186,31.6596088349468,
0.));
#149262=CARTESIAN_POINT('Ctrl Pts',(-64.4613460983186,31.6596088349468,
12.));
#149263=CARTESIAN_POINT('Ctrl Pts',(-64.4448309194499,31.6426715227865,
0.));
#149264=CARTESIAN_POINT('Ctrl Pts',(-64.4448309194499,31.6426715227865,
12.));
#149265=CARTESIAN_POINT('Ctrl Pts',(-64.4283292781553,31.6257813797281,
0.));
#149266=CARTESIAN_POINT('Ctrl Pts',(-64.4283292781553,31.6257813797281,
12.));
#149267=CARTESIAN_POINT('Ctrl Pts',(-64.4118413066386,31.6089384506399,
0.));
#149268=CARTESIAN_POINT('Ctrl Pts',(-64.4118413066386,31.6089384506399,
12.));
#149269=CARTESIAN_POINT('Ctrl Pts',(-64.3953671377071,31.5921427804879,
0.));
#149270=CARTESIAN_POINT('Ctrl Pts',(-64.3953671377071,31.5921427804879,
12.));
#149271=CARTESIAN_POINT('Ctrl Pts',(-64.3789069047768,31.5753944143355,
0.));
#149272=CARTESIAN_POINT('Ctrl Pts',(-64.3789069047768,31.5753944143355,
12.));
#149273=CARTESIAN_POINT('Ctrl Pts',(-64.3624607418798,31.5586933973531,
0.));
#149274=CARTESIAN_POINT('Ctrl Pts',(-64.3624607418798,31.5586933973531,
12.));
#149275=CARTESIAN_POINT('Ctrl Pts',(-64.34602878367,31.5420397748198,0.));
#149276=CARTESIAN_POINT('Ctrl Pts',(-64.34602878367,31.5420397748198,12.));
#149277=CARTESIAN_POINT('Ctrl Pts',(-64.3296111654273,31.5254335921239,
0.));
#149278=CARTESIAN_POINT('Ctrl Pts',(-64.3296111654273,31.5254335921239,
12.));
#149279=CARTESIAN_POINT('Ctrl Pts',(-64.3132080230603,31.5088748947564,
0.));
#149280=CARTESIAN_POINT('Ctrl Pts',(-64.3132080230603,31.5088748947564,
12.));
#149281=CARTESIAN_POINT('Ctrl Pts',(-64.2968194931113,31.4923637283109,
0.));
#149282=CARTESIAN_POINT('Ctrl Pts',(-64.2968194931113,31.4923637283109,
12.));
#149283=CARTESIAN_POINT('Ctrl Pts',(-64.2804457127633,31.4759001384922,
0.));
#149284=CARTESIAN_POINT('Ctrl Pts',(-64.2804457127633,31.4759001384922,
12.));
#149285=CARTESIAN_POINT('Ctrl Pts',(-64.264086819846,31.4594841711188,0.));
#149286=CARTESIAN_POINT('Ctrl Pts',(-64.264086819846,31.4594841711188,12.));
#149287=CARTESIAN_POINT('Ctrl Pts',(-64.2477429528408,31.4431158721229,
0.));
#149288=CARTESIAN_POINT('Ctrl Pts',(-64.2477429528408,31.4431158721229,
12.));
#149289=CARTESIAN_POINT('Ctrl Pts',(-64.2314142508843,31.4267952875439,
0.));
#149290=CARTESIAN_POINT('Ctrl Pts',(-64.2314142508843,31.4267952875439,
12.));
#149291=CARTESIAN_POINT('Ctrl Pts',(-64.2151008537733,31.4105224635298,
0.));
#149292=CARTESIAN_POINT('Ctrl Pts',(-64.2151008537733,31.4105224635298,
12.));
#149293=CARTESIAN_POINT('Ctrl Pts',(-64.1988029019733,31.3942974463458,
0.));
#149294=CARTESIAN_POINT('Ctrl Pts',(-64.1988029019733,31.3942974463458,
12.));
#149295=CARTESIAN_POINT('Ctrl Pts',(-64.1825205366231,31.3781202823758,
0.));
#149296=CARTESIAN_POINT('Ctrl Pts',(-64.1825205366231,31.3781202823758,
12.));
#149297=CARTESIAN_POINT('Ctrl Pts',(-64.1662538995407,31.3619910181222,
0.));
#149298=CARTESIAN_POINT('Ctrl Pts',(-64.1662538995407,31.3619910181222,
12.));
#149299=CARTESIAN_POINT('Ctrl Pts',(-64.150003133226,31.3459097001995,0.));
#149300=CARTESIAN_POINT('Ctrl Pts',(-64.150003133226,31.3459097001995,12.));
#149301=CARTESIAN_POINT('Ctrl Pts',(-64.1337683808667,31.3298763753366,
0.));
#149302=CARTESIAN_POINT('Ctrl Pts',(-64.1337683808667,31.3298763753366,
12.));
#149303=CARTESIAN_POINT('Ctrl Pts',(-64.1175497863475,31.3138910903852,
0.));
#149304=CARTESIAN_POINT('Ctrl Pts',(-64.1175497863475,31.3138910903852,
12.));
#149305=CARTESIAN_POINT('Ctrl Pts',(-64.1013474942554,31.2979538923213,
0.));
#149306=CARTESIAN_POINT('Ctrl Pts',(-64.1013474942554,31.2979538923213,
12.));
#149307=CARTESIAN_POINT('Ctrl Pts',(-64.0851616498861,31.2820648282451,
0.));
#149308=CARTESIAN_POINT('Ctrl Pts',(-64.0851616498861,31.2820648282451,
12.));
#149309=CARTESIAN_POINT('Ctrl Pts',(-64.0689923992475,31.2662239453734,
0.));
#149310=CARTESIAN_POINT('Ctrl Pts',(-64.0689923992475,31.2662239453734,
12.));
#149311=CARTESIAN_POINT('Ctrl Pts',(-64.0528398890671,31.2504312910457,
0.));
#149312=CARTESIAN_POINT('Ctrl Pts',(-64.0528398890671,31.2504312910457,
12.));
#149313=CARTESIAN_POINT('Ctrl Pts',(-64.036704266799,31.23468691273,0.));
#149314=CARTESIAN_POINT('Ctrl Pts',(-64.036704266799,31.23468691273,12.));
#149315=CARTESIAN_POINT('Ctrl Pts',(-64.0205856806298,31.2189908580245,
0.));
#149316=CARTESIAN_POINT('Ctrl Pts',(-64.0205856806298,31.2189908580245,
12.));
#149317=CARTESIAN_POINT('Ctrl Pts',(-64.004484279483,31.2033431746558,0.));
#149318=CARTESIAN_POINT('Ctrl Pts',(-64.004484279483,31.2033431746558,12.));
#149319=CARTESIAN_POINT('Ctrl Pts',(-63.9884002130209,31.1877439104717,
0.));
#149320=CARTESIAN_POINT('Ctrl Pts',(-63.9884002130209,31.1877439104717,
12.));
#149321=CARTESIAN_POINT('Ctrl Pts',(-63.972333631655,31.1721931134488,0.));
#149322=CARTESIAN_POINT('Ctrl Pts',(-63.972333631655,31.1721931134488,12.));
#149323=CARTESIAN_POINT('Ctrl Pts',(-63.9562846865566,31.1566908316992,
0.));
#149324=CARTESIAN_POINT('Ctrl Pts',(-63.9562846865566,31.1566908316992,
12.));
#149325=CARTESIAN_POINT('Ctrl Pts',(-63.9402535296651,31.1412371134727,
0.));
#149326=CARTESIAN_POINT('Ctrl Pts',(-63.9402535296651,31.1412371134727,
12.));
#149327=CARTESIAN_POINT('Ctrl Pts',(-63.9242403136955,31.1258320071545,
0.));
#149328=CARTESIAN_POINT('Ctrl Pts',(-63.9242403136955,31.1258320071545,
12.));
#149329=CARTESIAN_POINT('Ctrl Pts',(-63.9082451921447,31.1104755612606,
0.));
#149330=CARTESIAN_POINT('Ctrl Pts',(-63.9082451921447,31.1104755612606,
12.));
#149331=CARTESIAN_POINT('Ctrl Pts',(-63.8922683192963,31.0951678244454,
0.));
#149332=CARTESIAN_POINT('Ctrl Pts',(-63.8922683192963,31.0951678244454,
12.));
#149333=CARTESIAN_POINT('Ctrl Pts',(-63.8763098502235,31.079908845504,0.));
#149334=CARTESIAN_POINT('Ctrl Pts',(-63.8763098502235,31.079908845504,12.));
#149335=CARTESIAN_POINT('Ctrl Pts',(-63.8603699407922,31.0646986733723,
0.));
#149336=CARTESIAN_POINT('Ctrl Pts',(-63.8603699407922,31.0646986733723,
12.));
#149337=CARTESIAN_POINT('Ctrl Pts',(-63.8444487476615,31.0495373571217,
0.));
#149338=CARTESIAN_POINT('Ctrl Pts',(-63.8444487476615,31.0495373571217,
12.));
#149339=CARTESIAN_POINT('Ctrl Pts',(-63.8285464282857,31.0344249459544,
0.));
#149340=CARTESIAN_POINT('Ctrl Pts',(-63.8285464282857,31.0344249459544,
12.));
#149341=CARTESIAN_POINT('Ctrl Pts',(-63.8126631409376,31.0193614892177,
0.));
#149342=CARTESIAN_POINT('Ctrl Pts',(-63.8126631409376,31.0193614892177,
12.));
#149343=CARTESIAN_POINT('Ctrl Pts',(-63.7967990447288,31.0043470364112,
0.));
#149344=CARTESIAN_POINT('Ctrl Pts',(-63.7967990447288,31.0043470364112,
12.));
#149345=CARTESIAN_POINT('Ctrl Pts',(-63.7809542996258,30.9893816371907,
0.));
#149346=CARTESIAN_POINT('Ctrl Pts',(-63.7809542996258,30.9893816371907,
12.));
#149347=CARTESIAN_POINT('Ctrl Pts',(-63.7651290664713,30.9744653413679,
0.));
#149348=CARTESIAN_POINT('Ctrl Pts',(-63.7651290664713,30.9744653413679,
12.));
#149349=CARTESIAN_POINT('Ctrl Pts',(-63.7493235069844,30.9595981989091,
0.));
#149350=CARTESIAN_POINT('Ctrl Pts',(-63.7493235069844,30.9595981989091,
12.));
#149351=CARTESIAN_POINT('Ctrl Pts',(-63.733537783742,30.9447802599345,0.));
#149352=CARTESIAN_POINT('Ctrl Pts',(-63.733537783742,30.9447802599345,12.));
#149353=CARTESIAN_POINT('Ctrl Pts',(-63.7177720601604,30.9300115747113,
0.));
#149354=CARTESIAN_POINT('Ctrl Pts',(-63.7177720601604,30.9300115747113,
12.));
#149355=CARTESIAN_POINT('Ctrl Pts',(-63.7020265004805,30.9152921936471,
0.));
#149356=CARTESIAN_POINT('Ctrl Pts',(-63.7020265004805,30.9152921936471,
12.));
#149357=CARTESIAN_POINT('Ctrl Pts',(-63.6863012697354,30.9006221672703,
0.));
#149358=CARTESIAN_POINT('Ctrl Pts',(-63.6863012697354,30.9006221672703,
12.));
#149359=CARTESIAN_POINT('Ctrl Pts',(-63.6705965337996,30.8860015462488,
0.));
#149360=CARTESIAN_POINT('Ctrl Pts',(-63.6705965337996,30.8860015462488,
12.));
#149361=CARTESIAN_POINT('Ctrl Pts',(-63.6549124594681,30.8714303814202,
0.));
#149362=CARTESIAN_POINT('Ctrl Pts',(-63.6549124594681,30.8714303814202,
12.));
#149363=CARTESIAN_POINT('Ctrl Pts',(-63.6392492145233,30.8569087238131,
0.));
#149364=CARTESIAN_POINT('Ctrl Pts',(-63.6392492145233,30.8569087238131,
12.));
#149365=CARTESIAN_POINT('Ctrl Pts',(-63.6236069678041,30.8424366246665,
0.));
#149366=CARTESIAN_POINT('Ctrl Pts',(-63.6236069678041,30.8424366246665,
12.));
#149367=CARTESIAN_POINT('Ctrl Pts',(-63.6079858892747,30.8280141354447,
0.));
#149368=CARTESIAN_POINT('Ctrl Pts',(-63.6079858892747,30.8280141354447,
12.));
#149369=CARTESIAN_POINT('Ctrl Pts',(-63.5923861498964,30.8136413077999,
0.));
#149370=CARTESIAN_POINT('Ctrl Pts',(-63.5923861498964,30.8136413077999,
12.));
#149371=CARTESIAN_POINT('Ctrl Pts',(-63.5768079214868,30.7993181935265,
0.));
#149372=CARTESIAN_POINT('Ctrl Pts',(-63.5768079214868,30.7993181935265,
12.));
#149373=CARTESIAN_POINT('Ctrl Pts',(-63.5612513766005,30.7850448445207,
0.));
#149374=CARTESIAN_POINT('Ctrl Pts',(-63.5612513766005,30.7850448445207,
12.));
#149375=CARTESIAN_POINT('Ctrl Pts',(-63.5457166883558,30.7708213127169,
0.));
#149376=CARTESIAN_POINT('Ctrl Pts',(-63.5457166883558,30.7708213127169,
12.));
#149377=CARTESIAN_POINT('Ctrl Pts',(-63.5302040304174,30.7566476500772,
0.));
#149378=CARTESIAN_POINT('Ctrl Pts',(-63.5302040304174,30.7566476500772,
12.));
#149379=CARTESIAN_POINT('Ctrl Pts',(-63.514713577392,30.7425239087294,0.));
#149380=CARTESIAN_POINT('Ctrl Pts',(-63.514713577392,30.7425239087294,12.));
#149381=CARTESIAN_POINT('Ctrl Pts',(-63.4992455051805,30.7284501410827,
0.));
#149382=CARTESIAN_POINT('Ctrl Pts',(-63.4992455051805,30.7284501410827,
12.));
#149383=CARTESIAN_POINT('Ctrl Pts',(-63.4837999912759,30.7144263999259,
0.));
#149384=CARTESIAN_POINT('Ctrl Pts',(-63.4837999912759,30.7144263999259,
12.));
#149385=CARTESIAN_POINT('Ctrl Pts',(-63.4683772152497,30.7004527385806,
0.));
#149386=CARTESIAN_POINT('Ctrl Pts',(-63.4683772152497,30.7004527385806,
12.));
#149387=CARTESIAN_POINT('Ctrl Pts',(-63.4529773584211,30.686529210791,0.));
#149388=CARTESIAN_POINT('Ctrl Pts',(-63.4529773584211,30.686529210791,12.));
#149389=CARTESIAN_POINT('Ctrl Pts',(-63.4376006029575,30.6726558704301,
0.));
#149390=CARTESIAN_POINT('Ctrl Pts',(-63.4376006029575,30.6726558704301,
12.));
#149391=CARTESIAN_POINT('Ctrl Pts',(-63.4222471311236,30.6588327712482,
0.));
#149392=CARTESIAN_POINT('Ctrl Pts',(-63.4222471311236,30.6588327712482,
12.));
#149393=CARTESIAN_POINT('Ctrl Pts',(-63.4069171245094,30.6450599666134,
0.));
#149394=CARTESIAN_POINT('Ctrl Pts',(-63.4069171245094,30.6450599666134,
12.));
#149395=CARTESIAN_POINT('Ctrl Pts',(-63.3916107631421,30.6313375092084,
0.));
#149396=CARTESIAN_POINT('Ctrl Pts',(-63.3916107631421,30.6313375092084,
12.));
#149397=CARTESIAN_POINT('Ctrl Pts',(-63.3763282271838,30.6176654515988,
0.));
#149398=CARTESIAN_POINT('Ctrl Pts',(-63.3763282271838,30.6176654515988,
12.));
#149399=CARTESIAN_POINT('Ctrl Pts',(-63.3610696989599,30.6040438469089,
0.));
#149400=CARTESIAN_POINT('Ctrl Pts',(-63.3610696989599,30.6040438469089,
12.));
#149401=CARTESIAN_POINT('Ctrl Pts',(-63.3458353646145,30.5904727493707,
0.));
#149402=CARTESIAN_POINT('Ctrl Pts',(-63.3458353646145,30.5904727493707,
12.));
#149403=CARTESIAN_POINT('Ctrl Pts',(-63.330625416509,30.5769522151147,0.));
#149404=CARTESIAN_POINT('Ctrl Pts',(-63.330625416509,30.5769522151147,12.));
#149405=CARTESIAN_POINT('Ctrl Pts',(-63.315440053435,30.5634823022357,0.));
#149406=CARTESIAN_POINT('Ctrl Pts',(-63.315440053435,30.5634823022357,12.));
#149407=CARTESIAN_POINT('Ctrl Pts',(-63.300279475605,30.5500630691342,0.));
#149408=CARTESIAN_POINT('Ctrl Pts',(-63.300279475605,30.5500630691342,12.));
#149409=CARTESIAN_POINT('Ctrl Pts',(-63.2851438802462,30.5366945730503,
0.));
#149410=CARTESIAN_POINT('Ctrl Pts',(-63.2851438802462,30.5366945730503,
12.));
#149411=CARTESIAN_POINT('Ctrl Pts',(-63.2700334577661,30.5233768687875,
0.));
#149412=CARTESIAN_POINT('Ctrl Pts',(-63.2700334577661,30.5233768687875,
12.));
#149413=CARTESIAN_POINT('Ctrl Pts',(-63.2549483856268,30.5101100066683,
0.));
#149414=CARTESIAN_POINT('Ctrl Pts',(-63.2549483856268,30.5101100066683,
12.));
#149415=CARTESIAN_POINT('Ctrl Pts',(-63.2398888342612,30.4968940345027,
0.));
#149416=CARTESIAN_POINT('Ctrl Pts',(-63.2398888342612,30.4968940345027,
12.));
#149417=CARTESIAN_POINT('Ctrl Pts',(-63.2248549788272,30.4837290015011,
0.));
#149418=CARTESIAN_POINT('Ctrl Pts',(-63.2248549788272,30.4837290015011,
12.));
#149419=CARTESIAN_POINT('Ctrl Pts',(-63.2098470086636,30.470614961416,0.));
#149420=CARTESIAN_POINT('Ctrl Pts',(-63.2098470086636,30.470614961416,12.));
#149421=CARTESIAN_POINT('Ctrl Pts',(-63.1948651386868,30.4575519763305,
0.));
#149422=CARTESIAN_POINT('Ctrl Pts',(-63.1948651386868,30.4575519763305,
12.));
#149423=CARTESIAN_POINT('Ctrl Pts',(-63.1799096171757,30.4445401192324,
0.));
#149424=CARTESIAN_POINT('Ctrl Pts',(-63.1799096171757,30.4445401192324,
12.));
#149425=CARTESIAN_POINT('Ctrl Pts',(-63.1649807016766,30.431579465967,0.));
#149426=CARTESIAN_POINT('Ctrl Pts',(-63.1649807016766,30.431579465967,12.));
#149427=CARTESIAN_POINT('Ctrl Pts',(-63.1500786361382,30.4186700875598,
0.));
#149428=CARTESIAN_POINT('Ctrl Pts',(-63.1500786361382,30.4186700875598,
12.));
#149429=CARTESIAN_POINT('Ctrl Pts',(-63.1352036298512,30.4058120432259,
0.));
#149430=CARTESIAN_POINT('Ctrl Pts',(-63.1352036298512,30.4058120432259,
12.));
#149431=CARTESIAN_POINT('Ctrl Pts',(-63.1203558300911,30.3930053710592,
0.));
#149432=CARTESIAN_POINT('Ctrl Pts',(-63.1203558300911,30.3930053710592,
12.));
#149433=CARTESIAN_POINT('Ctrl Pts',(-63.1055353202641,30.3802500880564,
0.));
#149434=CARTESIAN_POINT('Ctrl Pts',(-63.1055353202641,30.3802500880564,
12.));
#149435=CARTESIAN_POINT('Ctrl Pts',(-63.0937007763826,30.3700869762658,
0.));
#149436=CARTESIAN_POINT('Ctrl Pts',(-63.0937007763826,30.3700869762658,
12.));
#149437=CARTESIAN_POINT('Ctrl Pts',(-63.0848371718274,30.3624877680747,
0.));
#149438=CARTESIAN_POINT('Ctrl Pts',(-63.0848371718274,30.3624877680747,
12.));
#149439=CARTESIAN_POINT('Ctrl Pts',(-63.0789335700774,30.3574319069365,
0.));
#149440=CARTESIAN_POINT('Ctrl Pts',(-63.0789335700774,30.3574319069365,
12.));
#149441=CARTESIAN_POINT('Ctrl Pts',(-63.0759831361898,30.3549065457811,
0.));
#149442=CARTESIAN_POINT('Ctrl Pts',(-63.0759831361898,30.3549065457811,
12.));
#149443=CARTESIAN_POINT('',(-63.0759831361898,30.3549065457811,12.));
#149444=CARTESIAN_POINT('Ctrl Pts',(-63.0759831361898,30.3549065457811,
12.));
#149445=CARTESIAN_POINT('Ctrl Pts',(-63.0789335700774,30.3574319069365,
12.));
#149446=CARTESIAN_POINT('Ctrl Pts',(-63.0848371718274,30.3624877680747,
12.));
#149447=CARTESIAN_POINT('Ctrl Pts',(-63.0937007763826,30.3700869762658,
12.));
#149448=CARTESIAN_POINT('Ctrl Pts',(-63.1055353202641,30.3802500880564,
12.));
#149449=CARTESIAN_POINT('Ctrl Pts',(-63.1203558300911,30.3930053710592,
12.));
#149450=CARTESIAN_POINT('Ctrl Pts',(-63.1352036298512,30.4058120432259,
12.));
#149451=CARTESIAN_POINT('Ctrl Pts',(-63.1500786361382,30.4186700875598,
12.));
#149452=CARTESIAN_POINT('Ctrl Pts',(-63.1649807016766,30.431579465967,12.));
#149453=CARTESIAN_POINT('Ctrl Pts',(-63.1799096171757,30.4445401192324,
12.));
#149454=CARTESIAN_POINT('Ctrl Pts',(-63.1948651386868,30.4575519763305,
12.));
#149455=CARTESIAN_POINT('Ctrl Pts',(-63.2098470086636,30.470614961416,12.));
#149456=CARTESIAN_POINT('Ctrl Pts',(-63.2248549788272,30.4837290015011,
12.));
#149457=CARTESIAN_POINT('Ctrl Pts',(-63.2398888342612,30.4968940345027,
12.));
#149458=CARTESIAN_POINT('Ctrl Pts',(-63.2549483856268,30.5101100066683,
12.));
#149459=CARTESIAN_POINT('Ctrl Pts',(-63.2700334577661,30.5233768687875,
12.));
#149460=CARTESIAN_POINT('Ctrl Pts',(-63.2851438802462,30.5366945730503,
12.));
#149461=CARTESIAN_POINT('Ctrl Pts',(-63.300279475605,30.5500630691342,12.));
#149462=CARTESIAN_POINT('Ctrl Pts',(-63.315440053435,30.5634823022357,12.));
#149463=CARTESIAN_POINT('Ctrl Pts',(-63.330625416509,30.5769522151147,12.));
#149464=CARTESIAN_POINT('Ctrl Pts',(-63.3458353646145,30.5904727493707,
12.));
#149465=CARTESIAN_POINT('Ctrl Pts',(-63.3610696989599,30.6040438469089,
12.));
#149466=CARTESIAN_POINT('Ctrl Pts',(-63.3763282271838,30.6176654515988,
12.));
#149467=CARTESIAN_POINT('Ctrl Pts',(-63.3916107631421,30.6313375092084,
12.));
#149468=CARTESIAN_POINT('Ctrl Pts',(-63.4069171245094,30.6450599666134,
12.));
#149469=CARTESIAN_POINT('Ctrl Pts',(-63.4222471311236,30.6588327712482,
12.));
#149470=CARTESIAN_POINT('Ctrl Pts',(-63.4376006029575,30.6726558704301,
12.));
#149471=CARTESIAN_POINT('Ctrl Pts',(-63.4529773584211,30.686529210791,12.));
#149472=CARTESIAN_POINT('Ctrl Pts',(-63.4683772152497,30.7004527385806,
12.));
#149473=CARTESIAN_POINT('Ctrl Pts',(-63.4837999912759,30.7144263999259,
12.));
#149474=CARTESIAN_POINT('Ctrl Pts',(-63.4992455051805,30.7284501410827,
12.));
#149475=CARTESIAN_POINT('Ctrl Pts',(-63.514713577392,30.7425239087294,12.));
#149476=CARTESIAN_POINT('Ctrl Pts',(-63.5302040304174,30.7566476500772,
12.));
#149477=CARTESIAN_POINT('Ctrl Pts',(-63.5457166883558,30.7708213127169,
12.));
#149478=CARTESIAN_POINT('Ctrl Pts',(-63.5612513766005,30.7850448445207,
12.));
#149479=CARTESIAN_POINT('Ctrl Pts',(-63.5768079214868,30.7993181935265,
12.));
#149480=CARTESIAN_POINT('Ctrl Pts',(-63.5923861498964,30.8136413077999,
12.));
#149481=CARTESIAN_POINT('Ctrl Pts',(-63.6079858892747,30.8280141354447,
12.));
#149482=CARTESIAN_POINT('Ctrl Pts',(-63.6236069678041,30.8424366246665,
12.));
#149483=CARTESIAN_POINT('Ctrl Pts',(-63.6392492145233,30.8569087238131,
12.));
#149484=CARTESIAN_POINT('Ctrl Pts',(-63.6549124594681,30.8714303814202,
12.));
#149485=CARTESIAN_POINT('Ctrl Pts',(-63.6705965337996,30.8860015462488,
12.));
#149486=CARTESIAN_POINT('Ctrl Pts',(-63.6863012697354,30.9006221672703,
12.));
#149487=CARTESIAN_POINT('Ctrl Pts',(-63.7020265004805,30.9152921936471,
12.));
#149488=CARTESIAN_POINT('Ctrl Pts',(-63.7177720601604,30.9300115747113,
12.));
#149489=CARTESIAN_POINT('Ctrl Pts',(-63.733537783742,30.9447802599345,12.));
#149490=CARTESIAN_POINT('Ctrl Pts',(-63.7493235069844,30.9595981989091,
12.));
#149491=CARTESIAN_POINT('Ctrl Pts',(-63.7651290664713,30.9744653413679,
12.));
#149492=CARTESIAN_POINT('Ctrl Pts',(-63.7809542996258,30.9893816371907,
12.));
#149493=CARTESIAN_POINT('Ctrl Pts',(-63.7967990447288,31.0043470364112,
12.));
#149494=CARTESIAN_POINT('Ctrl Pts',(-63.8126631409376,31.0193614892177,
12.));
#149495=CARTESIAN_POINT('Ctrl Pts',(-63.8285464282857,31.0344249459544,
12.));
#149496=CARTESIAN_POINT('Ctrl Pts',(-63.8444487476615,31.0495373571217,
12.));
#149497=CARTESIAN_POINT('Ctrl Pts',(-63.8603699407922,31.0646986733723,
12.));
#149498=CARTESIAN_POINT('Ctrl Pts',(-63.8763098502235,31.079908845504,12.));
#149499=CARTESIAN_POINT('Ctrl Pts',(-63.8922683192963,31.0951678244454,
12.));
#149500=CARTESIAN_POINT('Ctrl Pts',(-63.9082451921447,31.1104755612606,
12.));
#149501=CARTESIAN_POINT('Ctrl Pts',(-63.9242403136955,31.1258320071545,
12.));
#149502=CARTESIAN_POINT('Ctrl Pts',(-63.9402535296651,31.1412371134727,
12.));
#149503=CARTESIAN_POINT('Ctrl Pts',(-63.9562846865566,31.1566908316992,
12.));
#149504=CARTESIAN_POINT('Ctrl Pts',(-63.972333631655,31.1721931134488,12.));
#149505=CARTESIAN_POINT('Ctrl Pts',(-63.9884002130209,31.1877439104717,
12.));
#149506=CARTESIAN_POINT('Ctrl Pts',(-64.004484279483,31.2033431746558,12.));
#149507=CARTESIAN_POINT('Ctrl Pts',(-64.0205856806298,31.2189908580245,
12.));
#149508=CARTESIAN_POINT('Ctrl Pts',(-64.036704266799,31.23468691273,12.));
#149509=CARTESIAN_POINT('Ctrl Pts',(-64.0528398890671,31.2504312910457,
12.));
#149510=CARTESIAN_POINT('Ctrl Pts',(-64.0689923992475,31.2662239453734,
12.));
#149511=CARTESIAN_POINT('Ctrl Pts',(-64.0851616498861,31.2820648282451,
12.));
#149512=CARTESIAN_POINT('Ctrl Pts',(-64.1013474942554,31.2979538923213,
12.));
#149513=CARTESIAN_POINT('Ctrl Pts',(-64.1175497863475,31.3138910903852,
12.));
#149514=CARTESIAN_POINT('Ctrl Pts',(-64.1337683808667,31.3298763753366,
12.));
#149515=CARTESIAN_POINT('Ctrl Pts',(-64.150003133226,31.3459097001995,12.));
#149516=CARTESIAN_POINT('Ctrl Pts',(-64.1662538995407,31.3619910181222,
12.));
#149517=CARTESIAN_POINT('Ctrl Pts',(-64.1825205366231,31.3781202823758,
12.));
#149518=CARTESIAN_POINT('Ctrl Pts',(-64.1988029019733,31.3942974463458,
12.));
#149519=CARTESIAN_POINT('Ctrl Pts',(-64.2151008537733,31.4105224635298,
12.));
#149520=CARTESIAN_POINT('Ctrl Pts',(-64.2314142508843,31.4267952875439,
12.));
#149521=CARTESIAN_POINT('Ctrl Pts',(-64.2477429528408,31.4431158721229,
12.));
#149522=CARTESIAN_POINT('Ctrl Pts',(-64.264086819846,31.4594841711188,12.));
#149523=CARTESIAN_POINT('Ctrl Pts',(-64.2804457127633,31.4759001384922,
12.));
#149524=CARTESIAN_POINT('Ctrl Pts',(-64.2968194931113,31.4923637283109,
12.));
#149525=CARTESIAN_POINT('Ctrl Pts',(-64.3132080230603,31.5088748947564,
12.));
#149526=CARTESIAN_POINT('Ctrl Pts',(-64.3296111654273,31.5254335921239,
12.));
#149527=CARTESIAN_POINT('Ctrl Pts',(-64.34602878367,31.5420397748198,12.));
#149528=CARTESIAN_POINT('Ctrl Pts',(-64.3624607418798,31.5586933973531,
12.));
#149529=CARTESIAN_POINT('Ctrl Pts',(-64.3789069047768,31.5753944143355,
12.));
#149530=CARTESIAN_POINT('Ctrl Pts',(-64.3953671377071,31.5921427804879,
12.));
#149531=CARTESIAN_POINT('Ctrl Pts',(-64.4118413066386,31.6089384506399,
12.));
#149532=CARTESIAN_POINT('Ctrl Pts',(-64.4283292781553,31.6257813797281,
12.));
#149533=CARTESIAN_POINT('Ctrl Pts',(-64.4448309194499,31.6426715227865,
12.));
#149534=CARTESIAN_POINT('Ctrl Pts',(-64.4613460983186,31.6596088349468,
12.));
#149535=CARTESIAN_POINT('Ctrl Pts',(-64.4778746831598,31.6765932714456,
12.));
#149536=CARTESIAN_POINT('Ctrl Pts',(-64.4944165429672,31.6936247876228,
12.));
#149537=CARTESIAN_POINT('Ctrl Pts',(-64.5109715473277,31.7107033389204,
12.));
#149538=CARTESIAN_POINT('Ctrl Pts',(-64.5275395664134,31.7278288808736,
12.));
#149539=CARTESIAN_POINT('Ctrl Pts',(-64.544120470978,31.7450013691116,12.));
#149540=CARTESIAN_POINT('Ctrl Pts',(-64.5607141323527,31.7622207593637,
12.));
#149541=CARTESIAN_POINT('Ctrl Pts',(-64.5773204224429,31.7794870074583,
12.));
#149542=CARTESIAN_POINT('Ctrl Pts',(-64.5939392137233,31.7968000693218,
12.));
#149543=CARTESIAN_POINT('Ctrl Pts',(-64.6105703792312,31.8141599009684,
12.));
#149544=CARTESIAN_POINT('Ctrl Pts',(-64.627213792563,31.8315664585027,12.));
#149545=CARTESIAN_POINT('Ctrl Pts',(-64.6438693278718,31.849019698125,12.));
#149546=CARTESIAN_POINT('Ctrl Pts',(-64.6605368598631,31.8665195761311,
12.));
#149547=CARTESIAN_POINT('Ctrl Pts',(-64.6772162637905,31.8840660489106,
12.));
#149548=CARTESIAN_POINT('Ctrl Pts',(-64.6939074154491,31.9016590729371,
12.));
#149549=CARTESIAN_POINT('Ctrl Pts',(-64.7106101911723,31.9192986047702,
12.));
#149550=CARTESIAN_POINT('Ctrl Pts',(-64.727324467829,31.9369846010613,12.));
#149551=CARTESIAN_POINT('Ctrl Pts',(-64.7440501228201,31.9547170185533,
12.));
#149552=CARTESIAN_POINT('Ctrl Pts',(-64.7607870340738,31.972495814079,12.));
#149553=CARTESIAN_POINT('Ctrl Pts',(-64.7775350800405,31.9903209445521,
12.));
#149554=CARTESIAN_POINT('Ctrl Pts',(-64.7942941396883,32.0081923669677,
12.));
#149555=CARTESIAN_POINT('Ctrl Pts',(-64.8110640925021,32.0261100384092,
12.));
#149556=CARTESIAN_POINT('Ctrl Pts',(-64.8278448184785,32.0440739160476,
12.));
#149557=CARTESIAN_POINT('Ctrl Pts',(-64.8446361981234,32.0620839571409,
12.));
#149558=CARTESIAN_POINT('Ctrl Pts',(-64.8614381124455,32.0801401190244,
12.));
#149559=CARTESIAN_POINT('Ctrl Pts',(-64.8782504429527,32.0982423591112,
12.));
#149560=CARTESIAN_POINT('Ctrl Pts',(-64.8950730716501,32.1163906348983,
12.));
#149561=CARTESIAN_POINT('Ctrl Pts',(-64.9119058810367,32.1345849039674,
12.));
#149562=CARTESIAN_POINT('Ctrl Pts',(-64.9287487541015,32.152825123983,12.));
#149563=CARTESIAN_POINT('Ctrl Pts',(-64.9456015743193,32.1711112526854,
12.));
#149564=CARTESIAN_POINT('Ctrl Pts',(-64.9624642256461,32.189443247888,12.));
#149565=CARTESIAN_POINT('Ctrl Pts',(-64.9793365925178,32.207821067485,12.));
#149566=CARTESIAN_POINT('Ctrl Pts',(-64.9962185598462,32.2262446694512,
12.));
#149567=CARTESIAN_POINT('Ctrl Pts',(-65.0131100130158,32.2447140118422,
12.));
#149568=CARTESIAN_POINT('Ctrl Pts',(-65.03001083788,32.2632290527862,12.));
#149569=CARTESIAN_POINT('Ctrl Pts',(-65.0469209207563,32.2817897504807,
12.));
#149570=CARTESIAN_POINT('Ctrl Pts',(-65.0638401484257,32.3003960632006,
12.));
#149571=CARTESIAN_POINT('Ctrl Pts',(-65.0807684081282,32.3190479492987,
12.));
#149572=CARTESIAN_POINT('Ctrl Pts',(-65.0977055875608,32.3377453672051,
12.));
#149573=CARTESIAN_POINT('Ctrl Pts',(-65.1146515748722,32.3564882754212,
12.));
#149574=CARTESIAN_POINT('Ctrl Pts',(-65.1316062586588,32.3752766325136,
12.));
#149575=CARTESIAN_POINT('Ctrl Pts',(-65.1485695279635,32.3941103971221,
12.));
#149576=CARTESIAN_POINT('Ctrl Pts',(-65.1655412722726,32.4129895279615,
12.));
#149577=CARTESIAN_POINT('Ctrl Pts',(-65.182521381514,32.4319139838212,12.));
#149578=CARTESIAN_POINT('Ctrl Pts',(-65.1995097460538,32.450883723561,12.));
#149579=CARTESIAN_POINT('Ctrl Pts',(-65.2165062566924,32.4698987061032,
12.));
#149580=CARTESIAN_POINT('Ctrl Pts',(-65.2335108046614,32.4889588904392,
12.));
#149581=CARTESIAN_POINT('Ctrl Pts',(-65.2505232816209,32.5080642356328,
12.));
#149582=CARTESIAN_POINT('Ctrl Pts',(-65.2675435796558,32.5272147008191,
12.));
#149583=CARTESIAN_POINT('Ctrl Pts',(-65.2845715912721,32.5464102452014,
12.));
#149584=CARTESIAN_POINT('Ctrl Pts',(-65.3016072093912,32.5656508280421,
12.));
#149585=CARTESIAN_POINT('Ctrl Pts',(-65.31865032735,32.5849364086678,12.));
#149586=CARTESIAN_POINT('Ctrl Pts',(-65.3357008389004,32.604266946475,12.));
#149587=CARTESIAN_POINT('Ctrl Pts',(-65.3527586382081,32.6236424009301,
12.));
#149588=CARTESIAN_POINT('Ctrl Pts',(-65.3698236198513,32.6430627315674,
12.));
#149589=CARTESIAN_POINT('Ctrl Pts',(-65.3868956788182,32.662527897981,12.));
#149590=CARTESIAN_POINT('Ctrl Pts',(-65.4039747105039,32.6820378598267,
12.));
#149591=CARTESIAN_POINT('Ctrl Pts',(-65.4210606107035,32.7015925768265,
12.));
#149592=CARTESIAN_POINT('Ctrl Pts',(-65.4381532756065,32.7211920087683,
12.));
#149593=CARTESIAN_POINT('Ctrl Pts',(-65.4552526017905,32.7408361155037,
12.));
#149594=CARTESIAN_POINT('Ctrl Pts',(-65.4723584862122,32.7605248569378,
12.));
#149595=CARTESIAN_POINT('Ctrl Pts',(-65.4894708262061,32.7802581930287,
12.));
#149596=CARTESIAN_POINT('Ctrl Pts',(-65.5065895194929,32.8000360837974,
12.));
#149597=CARTESIAN_POINT('Ctrl Pts',(-65.5237144641858,32.8198584893315,
12.));
#149598=CARTESIAN_POINT('Ctrl Pts',(-65.5408455587965,32.8397253697865,
12.));
#149599=CARTESIAN_POINT('Ctrl Pts',(-65.5579827022421,32.8596366853832,
12.));
#149600=CARTESIAN_POINT('Ctrl Pts',(-65.5751257938473,32.879592396403,12.));
#149601=CARTESIAN_POINT('Ctrl Pts',(-65.5922747333194,32.8995924631898,
12.));
#149602=CARTESIAN_POINT('Ctrl Pts',(-65.6094294207276,32.9196368461463,
12.));
#149603=CARTESIAN_POINT('Ctrl Pts',(-65.6265897564783,32.9397255057274,
12.));
#149604=CARTESIAN_POINT('Ctrl Pts',(-65.6437556412947,32.9598584024312,
12.));
#149605=CARTESIAN_POINT('Ctrl Pts',(-65.6609269761889,32.9800354967839,
12.));
#149606=CARTESIAN_POINT('Ctrl Pts',(-65.6781036625027,33.0002567493573,
12.));
#149607=CARTESIAN_POINT('Ctrl Pts',(-65.6952856019533,33.0205221207872,
12.));
#149608=CARTESIAN_POINT('Ctrl Pts',(-65.7124726966802,33.0408315717873,
12.));
#149609=CARTESIAN_POINT('Ctrl Pts',(-65.7296648492825,33.0611850631582,
12.));
#149610=CARTESIAN_POINT('Ctrl Pts',(-65.7468619628816,33.081582555798,12.));
#149611=CARTESIAN_POINT('Ctrl Pts',(-65.7640639410661,33.1020240106884,
12.));
#149612=CARTESIAN_POINT('Ctrl Pts',(-65.7812706877697,33.1225093888671,
12.));
#149613=CARTESIAN_POINT('Ctrl Pts',(-65.7984821071623,33.1430386513976,
12.));
#149614=CARTESIAN_POINT('Ctrl Pts',(-65.8156981035503,33.16361175934,12.));
#149615=CARTESIAN_POINT('Ctrl Pts',(-65.8329185812375,33.1842286737051,
12.));
#149616=CARTESIAN_POINT('Ctrl Pts',(-65.8501434445164,33.2048893554491,
12.));
#149617=CARTESIAN_POINT('Ctrl Pts',(-65.8673725979578,33.2255937655649,
12.));
#149618=CARTESIAN_POINT('Ctrl Pts',(-65.8846059466372,33.2463418651492,
12.));
#149619=CARTESIAN_POINT('Ctrl Pts',(-65.9018433963889,33.2671336154753,
12.));
#149620=CARTESIAN_POINT('Ctrl Pts',(-65.9190848540433,33.2879689780572,
12.));
#149621=CARTESIAN_POINT('Ctrl Pts',(-65.9363302276846,33.3088479147164,
12.));
#149622=CARTESIAN_POINT('Ctrl Pts',(-65.9535794260831,33.3297703874265,
12.));
#149623=CARTESIAN_POINT('Ctrl Pts',(-65.970832358141,33.3507363581592,12.));
#149624=CARTESIAN_POINT('Ctrl Pts',(-65.9880889322831,33.37174578871,12.));
#149625=CARTESIAN_POINT('Ctrl Pts',(-66.0053490559812,33.3927986405605,
12.));
#149626=CARTESIAN_POINT('Ctrl Pts',(-66.0226126349446,33.4138948746388,
12.));
#149627=CARTESIAN_POINT('Ctrl Pts',(-66.0398795737777,33.43503445151,12.));
#149628=CARTESIAN_POINT('Ctrl Pts',(-66.0571497774434,33.4562173318025,
12.));
#149629=CARTESIAN_POINT('Ctrl Pts',(-66.0744231525415,33.4774434765745,
12.));
#149630=CARTESIAN_POINT('Ctrl Pts',(-66.0916996085245,33.4987128476622,
12.));
#149631=CARTESIAN_POINT('Ctrl Pts',(-66.1089790592729,33.5200254081243,
12.));
#149632=CARTESIAN_POINT('Ctrl Pts',(-66.1262614234675,33.541381122345,12.));
#149633=CARTESIAN_POINT('Ctrl Pts',(-66.1410781873279,33.5597240685847,
12.));
#149634=CARTESIAN_POINT('Ctrl Pts',(-66.1524393974176,33.5738105077877,
12.));
#149635=CARTESIAN_POINT('Ctrl Pts',(-66.1603438177524,33.5836213514192,
12.));
#149636=CARTESIAN_POINT('Ctrl Pts',(-66.1647906582661,33.5891439876497,
12.));
#149637=CARTESIAN_POINT('Ctrl Pts',(-66.1657795405966,33.5903722665284,
12.));
#149638=CARTESIAN_POINT('',(-63.0759831361898,30.3549065457811,0.));
#149639=CARTESIAN_POINT('',(-63.0759831361898,30.3549065457811,0.));
#149640=CARTESIAN_POINT('Ctrl Pts',(-66.1657795405966,33.5903722665284,
0.));
#149641=CARTESIAN_POINT('Ctrl Pts',(-66.1647906582661,33.5891439876497,
0.));
#149642=CARTESIAN_POINT('Ctrl Pts',(-66.1603438177524,33.5836213514192,
0.));
#149643=CARTESIAN_POINT('Ctrl Pts',(-66.1524393974176,33.5738105077877,
0.));
#149644=CARTESIAN_POINT('Ctrl Pts',(-66.1410781873279,33.5597240685847,
0.));
#149645=CARTESIAN_POINT('Ctrl Pts',(-66.1262614234675,33.541381122345,0.));
#149646=CARTESIAN_POINT('Ctrl Pts',(-66.1089790592729,33.5200254081243,
0.));
#149647=CARTESIAN_POINT('Ctrl Pts',(-66.0916996085245,33.4987128476622,
0.));
#149648=CARTESIAN_POINT('Ctrl Pts',(-66.0744231525415,33.4774434765745,
0.));
#149649=CARTESIAN_POINT('Ctrl Pts',(-66.0571497774434,33.4562173318025,
0.));
#149650=CARTESIAN_POINT('Ctrl Pts',(-66.0398795737777,33.43503445151,0.));
#149651=CARTESIAN_POINT('Ctrl Pts',(-66.0226126349446,33.4138948746388,
0.));
#149652=CARTESIAN_POINT('Ctrl Pts',(-66.0053490559812,33.3927986405605,
0.));
#149653=CARTESIAN_POINT('Ctrl Pts',(-65.9880889322831,33.37174578871,0.));
#149654=CARTESIAN_POINT('Ctrl Pts',(-65.970832358141,33.3507363581592,0.));
#149655=CARTESIAN_POINT('Ctrl Pts',(-65.9535794260831,33.3297703874265,
0.));
#149656=CARTESIAN_POINT('Ctrl Pts',(-65.9363302276846,33.3088479147164,
0.));
#149657=CARTESIAN_POINT('Ctrl Pts',(-65.9190848540433,33.2879689780572,
0.));
#149658=CARTESIAN_POINT('Ctrl Pts',(-65.9018433963889,33.2671336154753,
0.));
#149659=CARTESIAN_POINT('Ctrl Pts',(-65.8846059466372,33.2463418651492,
0.));
#149660=CARTESIAN_POINT('Ctrl Pts',(-65.8673725979578,33.2255937655649,
0.));
#149661=CARTESIAN_POINT('Ctrl Pts',(-65.8501434445164,33.2048893554491,
0.));
#149662=CARTESIAN_POINT('Ctrl Pts',(-65.8329185812375,33.1842286737051,
0.));
#149663=CARTESIAN_POINT('Ctrl Pts',(-65.8156981035503,33.16361175934,0.));
#149664=CARTESIAN_POINT('Ctrl Pts',(-65.7984821071623,33.1430386513976,
0.));
#149665=CARTESIAN_POINT('Ctrl Pts',(-65.7812706877697,33.1225093888671,
0.));
#149666=CARTESIAN_POINT('Ctrl Pts',(-65.7640639410661,33.1020240106884,
0.));
#149667=CARTESIAN_POINT('Ctrl Pts',(-65.7468619628816,33.081582555798,0.));
#149668=CARTESIAN_POINT('Ctrl Pts',(-65.7296648492825,33.0611850631582,
0.));
#149669=CARTESIAN_POINT('Ctrl Pts',(-65.7124726966802,33.0408315717873,
0.));
#149670=CARTESIAN_POINT('Ctrl Pts',(-65.6952856019533,33.0205221207872,
0.));
#149671=CARTESIAN_POINT('Ctrl Pts',(-65.6781036625027,33.0002567493573,
0.));
#149672=CARTESIAN_POINT('Ctrl Pts',(-65.6609269761889,32.9800354967839,
0.));
#149673=CARTESIAN_POINT('Ctrl Pts',(-65.6437556412947,32.9598584024312,
0.));
#149674=CARTESIAN_POINT('Ctrl Pts',(-65.6265897564783,32.9397255057274,
0.));
#149675=CARTESIAN_POINT('Ctrl Pts',(-65.6094294207276,32.9196368461463,
0.));
#149676=CARTESIAN_POINT('Ctrl Pts',(-65.5922747333194,32.8995924631898,
0.));
#149677=CARTESIAN_POINT('Ctrl Pts',(-65.5751257938473,32.879592396403,0.));
#149678=CARTESIAN_POINT('Ctrl Pts',(-65.5579827022421,32.8596366853832,
0.));
#149679=CARTESIAN_POINT('Ctrl Pts',(-65.5408455587965,32.8397253697865,
0.));
#149680=CARTESIAN_POINT('Ctrl Pts',(-65.5237144641858,32.8198584893315,
0.));
#149681=CARTESIAN_POINT('Ctrl Pts',(-65.5065895194929,32.8000360837974,
0.));
#149682=CARTESIAN_POINT('Ctrl Pts',(-65.4894708262061,32.7802581930287,
0.));
#149683=CARTESIAN_POINT('Ctrl Pts',(-65.4723584862122,32.7605248569378,
0.));
#149684=CARTESIAN_POINT('Ctrl Pts',(-65.4552526017905,32.7408361155037,
0.));
#149685=CARTESIAN_POINT('Ctrl Pts',(-65.4381532756065,32.7211920087683,
0.));
#149686=CARTESIAN_POINT('Ctrl Pts',(-65.4210606107035,32.7015925768265,
0.));
#149687=CARTESIAN_POINT('Ctrl Pts',(-65.4039747105039,32.6820378598267,
0.));
#149688=CARTESIAN_POINT('Ctrl Pts',(-65.3868956788182,32.662527897981,0.));
#149689=CARTESIAN_POINT('Ctrl Pts',(-65.3698236198513,32.6430627315674,
0.));
#149690=CARTESIAN_POINT('Ctrl Pts',(-65.3527586382081,32.6236424009301,
0.));
#149691=CARTESIAN_POINT('Ctrl Pts',(-65.3357008389004,32.604266946475,0.));
#149692=CARTESIAN_POINT('Ctrl Pts',(-65.31865032735,32.5849364086678,0.));
#149693=CARTESIAN_POINT('Ctrl Pts',(-65.3016072093912,32.5656508280421,
0.));
#149694=CARTESIAN_POINT('Ctrl Pts',(-65.2845715912721,32.5464102452014,
0.));
#149695=CARTESIAN_POINT('Ctrl Pts',(-65.2675435796558,32.5272147008191,
0.));
#149696=CARTESIAN_POINT('Ctrl Pts',(-65.2505232816209,32.5080642356328,
0.));
#149697=CARTESIAN_POINT('Ctrl Pts',(-65.2335108046614,32.4889588904392,
0.));
#149698=CARTESIAN_POINT('Ctrl Pts',(-65.2165062566924,32.4698987061032,
0.));
#149699=CARTESIAN_POINT('Ctrl Pts',(-65.1995097460538,32.450883723561,0.));
#149700=CARTESIAN_POINT('Ctrl Pts',(-65.182521381514,32.4319139838212,0.));
#149701=CARTESIAN_POINT('Ctrl Pts',(-65.1655412722726,32.4129895279615,
0.));
#149702=CARTESIAN_POINT('Ctrl Pts',(-65.1485695279635,32.3941103971221,
0.));
#149703=CARTESIAN_POINT('Ctrl Pts',(-65.1316062586588,32.3752766325136,
0.));
#149704=CARTESIAN_POINT('Ctrl Pts',(-65.1146515748722,32.3564882754212,
0.));
#149705=CARTESIAN_POINT('Ctrl Pts',(-65.0977055875608,32.3377453672051,
0.));
#149706=CARTESIAN_POINT('Ctrl Pts',(-65.0807684081282,32.3190479492987,
0.));
#149707=CARTESIAN_POINT('Ctrl Pts',(-65.0638401484257,32.3003960632006,
0.));
#149708=CARTESIAN_POINT('Ctrl Pts',(-65.0469209207563,32.2817897504807,
0.));
#149709=CARTESIAN_POINT('Ctrl Pts',(-65.03001083788,32.2632290527862,0.));
#149710=CARTESIAN_POINT('Ctrl Pts',(-65.0131100130158,32.2447140118422,
0.));
#149711=CARTESIAN_POINT('Ctrl Pts',(-64.9962185598462,32.2262446694512,
0.));
#149712=CARTESIAN_POINT('Ctrl Pts',(-64.9793365925178,32.207821067485,0.));
#149713=CARTESIAN_POINT('Ctrl Pts',(-64.9624642256461,32.189443247888,0.));
#149714=CARTESIAN_POINT('Ctrl Pts',(-64.9456015743193,32.1711112526854,
0.));
#149715=CARTESIAN_POINT('Ctrl Pts',(-64.9287487541015,32.152825123983,0.));
#149716=CARTESIAN_POINT('Ctrl Pts',(-64.9119058810367,32.1345849039674,
0.));
#149717=CARTESIAN_POINT('Ctrl Pts',(-64.8950730716501,32.1163906348983,
0.));
#149718=CARTESIAN_POINT('Ctrl Pts',(-64.8782504429527,32.0982423591112,
0.));
#149719=CARTESIAN_POINT('Ctrl Pts',(-64.8614381124455,32.0801401190244,
0.));
#149720=CARTESIAN_POINT('Ctrl Pts',(-64.8446361981234,32.0620839571409,
0.));
#149721=CARTESIAN_POINT('Ctrl Pts',(-64.8278448184785,32.0440739160476,
0.));
#149722=CARTESIAN_POINT('Ctrl Pts',(-64.8110640925021,32.0261100384092,
0.));
#149723=CARTESIAN_POINT('Ctrl Pts',(-64.7942941396883,32.0081923669677,
0.));
#149724=CARTESIAN_POINT('Ctrl Pts',(-64.7775350800405,31.9903209445521,
0.));
#149725=CARTESIAN_POINT('Ctrl Pts',(-64.7607870340738,31.972495814079,0.));
#149726=CARTESIAN_POINT('Ctrl Pts',(-64.7440501228201,31.9547170185533,
0.));
#149727=CARTESIAN_POINT('Ctrl Pts',(-64.727324467829,31.9369846010613,0.));
#149728=CARTESIAN_POINT('Ctrl Pts',(-64.7106101911723,31.9192986047702,
0.));
#149729=CARTESIAN_POINT('Ctrl Pts',(-64.6939074154491,31.9016590729371,
0.));
#149730=CARTESIAN_POINT('Ctrl Pts',(-64.6772162637905,31.8840660489106,
0.));
#149731=CARTESIAN_POINT('Ctrl Pts',(-64.6605368598631,31.8665195761311,
0.));
#149732=CARTESIAN_POINT('Ctrl Pts',(-64.6438693278718,31.849019698125,0.));
#149733=CARTESIAN_POINT('Ctrl Pts',(-64.627213792563,31.8315664585027,0.));
#149734=CARTESIAN_POINT('Ctrl Pts',(-64.6105703792312,31.8141599009684,
0.));
#149735=CARTESIAN_POINT('Ctrl Pts',(-64.5939392137233,31.7968000693218,
0.));
#149736=CARTESIAN_POINT('Ctrl Pts',(-64.5773204224429,31.7794870074583,
0.));
#149737=CARTESIAN_POINT('Ctrl Pts',(-64.5607141323527,31.7622207593637,
0.));
#149738=CARTESIAN_POINT('Ctrl Pts',(-64.544120470978,31.7450013691116,0.));
#149739=CARTESIAN_POINT('Ctrl Pts',(-64.5275395664134,31.7278288808736,
0.));
#149740=CARTESIAN_POINT('Ctrl Pts',(-64.5109715473277,31.7107033389204,
0.));
#149741=CARTESIAN_POINT('Ctrl Pts',(-64.4944165429672,31.6936247876228,
0.));
#149742=CARTESIAN_POINT('Ctrl Pts',(-64.4778746831598,31.6765932714456,
0.));
#149743=CARTESIAN_POINT('Ctrl Pts',(-64.4613460983186,31.6596088349468,
0.));
#149744=CARTESIAN_POINT('Ctrl Pts',(-64.4448309194499,31.6426715227865,
0.));
#149745=CARTESIAN_POINT('Ctrl Pts',(-64.4283292781553,31.6257813797281,
0.));
#149746=CARTESIAN_POINT('Ctrl Pts',(-64.4118413066386,31.6089384506399,
0.));
#149747=CARTESIAN_POINT('Ctrl Pts',(-64.3953671377071,31.5921427804879,
0.));
#149748=CARTESIAN_POINT('Ctrl Pts',(-64.3789069047768,31.5753944143355,
0.));
#149749=CARTESIAN_POINT('Ctrl Pts',(-64.3624607418798,31.5586933973531,
0.));
#149750=CARTESIAN_POINT('Ctrl Pts',(-64.34602878367,31.5420397748198,0.));
#149751=CARTESIAN_POINT('Ctrl Pts',(-64.3296111654273,31.5254335921239,
0.));
#149752=CARTESIAN_POINT('Ctrl Pts',(-64.3132080230603,31.5088748947564,
0.));
#149753=CARTESIAN_POINT('Ctrl Pts',(-64.2968194931113,31.4923637283109,
0.));
#149754=CARTESIAN_POINT('Ctrl Pts',(-64.2804457127633,31.4759001384922,
0.));
#149755=CARTESIAN_POINT('Ctrl Pts',(-64.264086819846,31.4594841711188,0.));
#149756=CARTESIAN_POINT('Ctrl Pts',(-64.2477429528408,31.4431158721229,
0.));
#149757=CARTESIAN_POINT('Ctrl Pts',(-64.2314142508843,31.4267952875439,
0.));
#149758=CARTESIAN_POINT('Ctrl Pts',(-64.2151008537733,31.4105224635298,
0.));
#149759=CARTESIAN_POINT('Ctrl Pts',(-64.1988029019733,31.3942974463458,
0.));
#149760=CARTESIAN_POINT('Ctrl Pts',(-64.1825205366231,31.3781202823758,
0.));
#149761=CARTESIAN_POINT('Ctrl Pts',(-64.1662538995407,31.3619910181222,
0.));
#149762=CARTESIAN_POINT('Ctrl Pts',(-64.150003133226,31.3459097001995,0.));
#149763=CARTESIAN_POINT('Ctrl Pts',(-64.1337683808667,31.3298763753366,
0.));
#149764=CARTESIAN_POINT('Ctrl Pts',(-64.1175497863475,31.3138910903852,
0.));
#149765=CARTESIAN_POINT('Ctrl Pts',(-64.1013474942554,31.2979538923213,
0.));
#149766=CARTESIAN_POINT('Ctrl Pts',(-64.0851616498861,31.2820648282451,
0.));
#149767=CARTESIAN_POINT('Ctrl Pts',(-64.0689923992475,31.2662239453734,
0.));
#149768=CARTESIAN_POINT('Ctrl Pts',(-64.0528398890671,31.2504312910457,
0.));
#149769=CARTESIAN_POINT('Ctrl Pts',(-64.036704266799,31.23468691273,0.));
#149770=CARTESIAN_POINT('Ctrl Pts',(-64.0205856806298,31.2189908580245,
0.));
#149771=CARTESIAN_POINT('Ctrl Pts',(-64.004484279483,31.2033431746558,0.));
#149772=CARTESIAN_POINT('Ctrl Pts',(-63.9884002130209,31.1877439104717,
0.));
#149773=CARTESIAN_POINT('Ctrl Pts',(-63.972333631655,31.1721931134488,0.));
#149774=CARTESIAN_POINT('Ctrl Pts',(-63.9562846865566,31.1566908316992,
0.));
#149775=CARTESIAN_POINT('Ctrl Pts',(-63.9402535296651,31.1412371134727,
0.));
#149776=CARTESIAN_POINT('Ctrl Pts',(-63.9242403136955,31.1258320071545,
0.));
#149777=CARTESIAN_POINT('Ctrl Pts',(-63.9082451921447,31.1104755612606,
0.));
#149778=CARTESIAN_POINT('Ctrl Pts',(-63.8922683192963,31.0951678244454,
0.));
#149779=CARTESIAN_POINT('Ctrl Pts',(-63.8763098502235,31.079908845504,0.));
#149780=CARTESIAN_POINT('Ctrl Pts',(-63.8603699407922,31.0646986733723,
0.));
#149781=CARTESIAN_POINT('Ctrl Pts',(-63.8444487476615,31.0495373571217,
0.));
#149782=CARTESIAN_POINT('Ctrl Pts',(-63.8285464282857,31.0344249459544,
0.));
#149783=CARTESIAN_POINT('Ctrl Pts',(-63.8126631409376,31.0193614892177,
0.));
#149784=CARTESIAN_POINT('Ctrl Pts',(-63.7967990447288,31.0043470364112,
0.));
#149785=CARTESIAN_POINT('Ctrl Pts',(-63.7809542996258,30.9893816371907,
0.));
#149786=CARTESIAN_POINT('Ctrl Pts',(-63.7651290664713,30.9744653413679,
0.));
#149787=CARTESIAN_POINT('Ctrl Pts',(-63.7493235069844,30.9595981989091,
0.));
#149788=CARTESIAN_POINT('Ctrl Pts',(-63.733537783742,30.9447802599345,0.));
#149789=CARTESIAN_POINT('Ctrl Pts',(-63.7177720601604,30.9300115747113,
0.));
#149790=CARTESIAN_POINT('Ctrl Pts',(-63.7020265004805,30.9152921936471,
0.));
#149791=CARTESIAN_POINT('Ctrl Pts',(-63.6863012697354,30.9006221672703,
0.));
#149792=CARTESIAN_POINT('Ctrl Pts',(-63.6705965337996,30.8860015462488,
0.));
#149793=CARTESIAN_POINT('Ctrl Pts',(-63.6549124594681,30.8714303814202,
0.));
#149794=CARTESIAN_POINT('Ctrl Pts',(-63.6392492145233,30.8569087238131,
0.));
#149795=CARTESIAN_POINT('Ctrl Pts',(-63.6236069678041,30.8424366246665,
0.));
#149796=CARTESIAN_POINT('Ctrl Pts',(-63.6079858892747,30.8280141354447,
0.));
#149797=CARTESIAN_POINT('Ctrl Pts',(-63.5923861498964,30.8136413077999,
0.));
#149798=CARTESIAN_POINT('Ctrl Pts',(-63.5768079214868,30.7993181935265,
0.));
#149799=CARTESIAN_POINT('Ctrl Pts',(-63.5612513766005,30.7850448445207,
0.));
#149800=CARTESIAN_POINT('Ctrl Pts',(-63.5457166883558,30.7708213127169,
0.));
#149801=CARTESIAN_POINT('Ctrl Pts',(-63.5302040304174,30.7566476500772,
0.));
#149802=CARTESIAN_POINT('Ctrl Pts',(-63.514713577392,30.7425239087294,0.));
#149803=CARTESIAN_POINT('Ctrl Pts',(-63.4992455051805,30.7284501410827,
0.));
#149804=CARTESIAN_POINT('Ctrl Pts',(-63.4837999912759,30.7144263999259,
0.));
#149805=CARTESIAN_POINT('Ctrl Pts',(-63.4683772152497,30.7004527385806,
0.));
#149806=CARTESIAN_POINT('Ctrl Pts',(-63.4529773584211,30.686529210791,0.));
#149807=CARTESIAN_POINT('Ctrl Pts',(-63.4376006029575,30.6726558704301,
0.));
#149808=CARTESIAN_POINT('Ctrl Pts',(-63.4222471311236,30.6588327712482,
0.));
#149809=CARTESIAN_POINT('Ctrl Pts',(-63.4069171245094,30.6450599666134,
0.));
#149810=CARTESIAN_POINT('Ctrl Pts',(-63.3916107631421,30.6313375092084,
0.));
#149811=CARTESIAN_POINT('Ctrl Pts',(-63.3763282271838,30.6176654515988,
0.));
#149812=CARTESIAN_POINT('Ctrl Pts',(-63.3610696989599,30.6040438469089,
0.));
#149813=CARTESIAN_POINT('Ctrl Pts',(-63.3458353646145,30.5904727493707,
0.));
#149814=CARTESIAN_POINT('Ctrl Pts',(-63.330625416509,30.5769522151147,0.));
#149815=CARTESIAN_POINT('Ctrl Pts',(-63.315440053435,30.5634823022357,0.));
#149816=CARTESIAN_POINT('Ctrl Pts',(-63.300279475605,30.5500630691342,0.));
#149817=CARTESIAN_POINT('Ctrl Pts',(-63.2851438802462,30.5366945730503,
0.));
#149818=CARTESIAN_POINT('Ctrl Pts',(-63.2700334577661,30.5233768687875,
0.));
#149819=CARTESIAN_POINT('Ctrl Pts',(-63.2549483856268,30.5101100066683,
0.));
#149820=CARTESIAN_POINT('Ctrl Pts',(-63.2398888342612,30.4968940345027,
0.));
#149821=CARTESIAN_POINT('Ctrl Pts',(-63.2248549788272,30.4837290015011,
0.));
#149822=CARTESIAN_POINT('Ctrl Pts',(-63.2098470086636,30.470614961416,0.));
#149823=CARTESIAN_POINT('Ctrl Pts',(-63.1948651386868,30.4575519763305,
0.));
#149824=CARTESIAN_POINT('Ctrl Pts',(-63.1799096171757,30.4445401192324,
0.));
#149825=CARTESIAN_POINT('Ctrl Pts',(-63.1649807016766,30.431579465967,0.));
#149826=CARTESIAN_POINT('Ctrl Pts',(-63.1500786361382,30.4186700875598,
0.));
#149827=CARTESIAN_POINT('Ctrl Pts',(-63.1352036298512,30.4058120432259,
0.));
#149828=CARTESIAN_POINT('Ctrl Pts',(-63.1203558300911,30.3930053710592,
0.));
#149829=CARTESIAN_POINT('Ctrl Pts',(-63.1055353202641,30.3802500880564,
0.));
#149830=CARTESIAN_POINT('Ctrl Pts',(-63.0937007763826,30.3700869762658,
0.));
#149831=CARTESIAN_POINT('Ctrl Pts',(-63.0848371718274,30.3624877680747,
0.));
#149832=CARTESIAN_POINT('Ctrl Pts',(-63.0789335700774,30.3574319069365,
0.));
#149833=CARTESIAN_POINT('Ctrl Pts',(-63.0759831361898,30.3549065457811,
0.));
#149834=CARTESIAN_POINT('Ctrl Pts',(-63.1661434108059,39.5004851439258,
0.));
#149835=CARTESIAN_POINT('Ctrl Pts',(-63.1661434108059,39.5004851439258,
12.));
#149836=CARTESIAN_POINT('Ctrl Pts',(-63.1630766582788,39.4958045828135,
0.));
#149837=CARTESIAN_POINT('Ctrl Pts',(-63.1630766582788,39.4958045828135,
12.));
#149838=CARTESIAN_POINT('Ctrl Pts',(-63.1569429707875,39.4864477303823,
0.));
#149839=CARTESIAN_POINT('Ctrl Pts',(-63.1569429707875,39.4864477303823,
12.));
#149840=CARTESIAN_POINT('Ctrl Pts',(-63.1477418922406,39.4724252611155,
0.));
#149841=CARTESIAN_POINT('Ctrl Pts',(-63.1477418922406,39.4724252611155,
12.));
#149842=CARTESIAN_POINT('Ctrl Pts',(-63.1354726928398,39.4537542552268,
0.));
#149843=CARTESIAN_POINT('Ctrl Pts',(-63.1354726928398,39.4537542552268,
12.));
#149844=CARTESIAN_POINT('Ctrl Pts',(-63.1201343731172,39.4304582059864,
0.));
#149845=CARTESIAN_POINT('Ctrl Pts',(-63.1201343731172,39.4304582059864,
12.));
#149846=CARTESIAN_POINT('Ctrl Pts',(-63.10479424519,39.4072048797616,0.));
#149847=CARTESIAN_POINT('Ctrl Pts',(-63.10479424519,39.4072048797616,12.));
#149848=CARTESIAN_POINT('Ctrl Pts',(-63.0894523341314,39.383994298574,0.));
#149849=CARTESIAN_POINT('Ctrl Pts',(-63.0894523341314,39.383994298574,12.));
#149850=CARTESIAN_POINT('Ctrl Pts',(-63.0741086815841,39.3608264920409,
0.));
#149851=CARTESIAN_POINT('Ctrl Pts',(-63.0741086815841,39.3608264920409,
12.));
#149852=CARTESIAN_POINT('Ctrl Pts',(-63.0587633513774,39.3377014983609,
0.));
#149853=CARTESIAN_POINT('Ctrl Pts',(-63.0587633513774,39.3377014983609,
12.));
#149854=CARTESIAN_POINT('Ctrl Pts',(-63.0434164277992,39.3146193632392,
0.));
#149855=CARTESIAN_POINT('Ctrl Pts',(-63.0434164277992,39.3146193632392,
12.));
#149856=CARTESIAN_POINT('Ctrl Pts',(-63.0280680082353,39.2915801372354,
0.));
#149857=CARTESIAN_POINT('Ctrl Pts',(-63.0280680082353,39.2915801372354,
12.));
#149858=CARTESIAN_POINT('Ctrl Pts',(-63.0127181973628,39.2685838735361,
0.));
#149859=CARTESIAN_POINT('Ctrl Pts',(-63.0127181973628,39.2685838735361,
12.));
#149860=CARTESIAN_POINT('Ctrl Pts',(-62.9973671008703,39.2456306256104,
0.));
#149861=CARTESIAN_POINT('Ctrl Pts',(-62.9973671008703,39.2456306256104,
12.));
#149862=CARTESIAN_POINT('Ctrl Pts',(-62.9820148189929,39.2227204447638,
0.));
#149863=CARTESIAN_POINT('Ctrl Pts',(-62.9820148189929,39.2227204447638,
12.));
#149864=CARTESIAN_POINT('Ctrl Pts',(-62.9666614412731,39.1998533781661,
0.));
#149865=CARTESIAN_POINT('Ctrl Pts',(-62.9666614412731,39.1998533781661,
12.));
#149866=CARTESIAN_POINT('Ctrl Pts',(-62.9513070501867,39.1770294702428,
0.));
#149867=CARTESIAN_POINT('Ctrl Pts',(-62.9513070501867,39.1770294702428,
12.));
#149868=CARTESIAN_POINT('Ctrl Pts',(-62.9359517237404,39.1542487636744,
0.));
#149869=CARTESIAN_POINT('Ctrl Pts',(-62.9359517237404,39.1542487636744,
12.));
#149870=CARTESIAN_POINT('Ctrl Pts',(-62.9205955385558,39.131511300575,0.));
#149871=CARTESIAN_POINT('Ctrl Pts',(-62.9205955385558,39.131511300575,12.));
#149872=CARTESIAN_POINT('Ctrl Pts',(-62.9052385725387,39.1088171235125,
0.));
#149873=CARTESIAN_POINT('Ctrl Pts',(-62.9052385725387,39.1088171235125,
12.));
#149874=CARTESIAN_POINT('Ctrl Pts',(-62.8898809082612,39.0861662767932,
0.));
#149875=CARTESIAN_POINT('Ctrl Pts',(-62.8898809082612,39.0861662767932,
12.));
#149876=CARTESIAN_POINT('Ctrl Pts',(-62.8745226325998,39.0635588063276,
0.));
#149877=CARTESIAN_POINT('Ctrl Pts',(-62.8745226325998,39.0635588063276,
12.));
#149878=CARTESIAN_POINT('Ctrl Pts',(-62.8591638352056,39.0409947590497,
0.));
#149879=CARTESIAN_POINT('Ctrl Pts',(-62.8591638352056,39.0409947590497,
12.));
#149880=CARTESIAN_POINT('Ctrl Pts',(-62.8438046073224,39.0184741824641,
0.));
#149881=CARTESIAN_POINT('Ctrl Pts',(-62.8438046073224,39.0184741824641,
12.));
#149882=CARTESIAN_POINT('Ctrl Pts',(-62.8284450405459,38.9959971241701,
0.));
#149883=CARTESIAN_POINT('Ctrl Pts',(-62.8284450405459,38.9959971241701,
12.));
#149884=CARTESIAN_POINT('Ctrl Pts',(-62.8130852254027,38.9735636313089,
0.));
#149885=CARTESIAN_POINT('Ctrl Pts',(-62.8130852254027,38.9735636313089,
12.));
#149886=CARTESIAN_POINT('Ctrl Pts',(-62.7977252507118,38.9511737503165,
0.));
#149887=CARTESIAN_POINT('Ctrl Pts',(-62.7977252507118,38.9511737503165,
12.));
#149888=CARTESIAN_POINT('Ctrl Pts',(-62.78236520437,38.9288275272335,0.));
#149889=CARTESIAN_POINT('Ctrl Pts',(-62.78236520437,38.9288275272335,12.));
#149890=CARTESIAN_POINT('Ctrl Pts',(-62.7670051738143,38.9065250078832,
0.));
#149891=CARTESIAN_POINT('Ctrl Pts',(-62.7670051738143,38.9065250078832,
12.));
#149892=CARTESIAN_POINT('Ctrl Pts',(-62.7516452466128,38.8842662380984,
0.));
#149893=CARTESIAN_POINT('Ctrl Pts',(-62.7516452466128,38.8842662380984,
12.));
#149894=CARTESIAN_POINT('Ctrl Pts',(-62.7362855110042,38.8620512639232,
0.));
#149895=CARTESIAN_POINT('Ctrl Pts',(-62.7362855110042,38.8620512639232,
12.));
#149896=CARTESIAN_POINT('Ctrl Pts',(-62.7209260564493,38.8398801318177,
0.));
#149897=CARTESIAN_POINT('Ctrl Pts',(-62.7209260564493,38.8398801318177,
12.));
#149898=CARTESIAN_POINT('Ctrl Pts',(-62.7055669733802,38.8177528885681,
0.));
#149899=CARTESIAN_POINT('Ctrl Pts',(-62.7055669733802,38.8177528885681,
12.));
#149900=CARTESIAN_POINT('Ctrl Pts',(-62.6902083529694,38.795669581203,0.));
#149901=CARTESIAN_POINT('Ctrl Pts',(-62.6902083529694,38.795669581203,12.));
#149902=CARTESIAN_POINT('Ctrl Pts',(-62.6748502868835,38.7736302568982,
0.));
#149903=CARTESIAN_POINT('Ctrl Pts',(-62.6748502868835,38.7736302568982,
12.));
#149904=CARTESIAN_POINT('Ctrl Pts',(-62.6594928670628,38.7516349628904,
0.));
#149905=CARTESIAN_POINT('Ctrl Pts',(-62.6594928670628,38.7516349628904,
12.));
#149906=CARTESIAN_POINT('Ctrl Pts',(-62.6441361854411,38.7296837463609,
0.));
#149907=CARTESIAN_POINT('Ctrl Pts',(-62.6441361854411,38.7296837463609,
12.));
#149908=CARTESIAN_POINT('Ctrl Pts',(-62.6287803339542,38.7077766544416,
0.));
#149909=CARTESIAN_POINT('Ctrl Pts',(-62.6287803339542,38.7077766544416,
12.));
#149910=CARTESIAN_POINT('Ctrl Pts',(-62.6134254046739,38.6859137342731,
0.));
#149911=CARTESIAN_POINT('Ctrl Pts',(-62.6134254046739,38.6859137342731,
12.));
#149912=CARTESIAN_POINT('Ctrl Pts',(-62.5980714899052,38.6640950330421,
0.));
#149913=CARTESIAN_POINT('Ctrl Pts',(-62.5980714899052,38.6640950330421,
12.));
#149914=CARTESIAN_POINT('Ctrl Pts',(-62.5827186822921,38.6423205980213,
0.));
#149915=CARTESIAN_POINT('Ctrl Pts',(-62.5827186822921,38.6423205980213,
12.));
#149916=CARTESIAN_POINT('Ctrl Pts',(-62.5673670749361,38.6205904766073,
0.));
#149917=CARTESIAN_POINT('Ctrl Pts',(-62.5673670749361,38.6205904766073,
12.));
#149918=CARTESIAN_POINT('Ctrl Pts',(-62.5520167614516,38.5989047163393,
0.));
#149919=CARTESIAN_POINT('Ctrl Pts',(-62.5520167614516,38.5989047163393,
12.));
#149920=CARTESIAN_POINT('Ctrl Pts',(-62.5366678359023,38.5772633648832,
0.));
#149921=CARTESIAN_POINT('Ctrl Pts',(-62.5366678359023,38.5772633648832,
12.));
#149922=CARTESIAN_POINT('Ctrl Pts',(-62.5213203927663,38.5556664700195,
0.));
#149923=CARTESIAN_POINT('Ctrl Pts',(-62.5213203927663,38.5556664700195,
12.));
#149924=CARTESIAN_POINT('Ctrl Pts',(-62.5059745268901,38.5341140796248,
0.));
#149925=CARTESIAN_POINT('Ctrl Pts',(-62.5059745268901,38.5341140796248,
12.));
#149926=CARTESIAN_POINT('Ctrl Pts',(-62.4906303334443,38.5126062416502,
0.));
#149927=CARTESIAN_POINT('Ctrl Pts',(-62.4906303334443,38.5126062416502,
12.));
#149928=CARTESIAN_POINT('Ctrl Pts',(-62.4752879078854,38.4911430040997,
0.));
#149929=CARTESIAN_POINT('Ctrl Pts',(-62.4752879078854,38.4911430040997,
12.));
#149930=CARTESIAN_POINT('Ctrl Pts',(-62.4599473459811,38.4697244150482,
0.));
#149931=CARTESIAN_POINT('Ctrl Pts',(-62.4599473459811,38.4697244150482,
12.));
#149932=CARTESIAN_POINT('Ctrl Pts',(-62.4446087438312,38.4483505226518,
0.));
#149933=CARTESIAN_POINT('Ctrl Pts',(-62.4446087438312,38.4483505226518,
12.));
#149934=CARTESIAN_POINT('Ctrl Pts',(-62.4292721978901,38.4270213751568,
0.));
#149935=CARTESIAN_POINT('Ctrl Pts',(-62.4292721978901,38.4270213751568,
12.));
#149936=CARTESIAN_POINT('Ctrl Pts',(-62.4139378049885,38.405737020905,0.));
#149937=CARTESIAN_POINT('Ctrl Pts',(-62.4139378049885,38.405737020905,12.));
#149938=CARTESIAN_POINT('Ctrl Pts',(-62.3986056623577,38.3844975083343,
0.));
#149939=CARTESIAN_POINT('Ctrl Pts',(-62.3986056623577,38.3844975083343,
12.));
#149940=CARTESIAN_POINT('Ctrl Pts',(-62.3832758676271,38.3633028859828,
0.));
#149941=CARTESIAN_POINT('Ctrl Pts',(-62.3832758676271,38.3633028859828,
12.));
#149942=CARTESIAN_POINT('Ctrl Pts',(-62.3679485188172,38.342153202491,0.));
#149943=CARTESIAN_POINT('Ctrl Pts',(-62.3679485188172,38.342153202491,12.));
#149944=CARTESIAN_POINT('Ctrl Pts',(-62.3526237143336,38.3210485066001,
0.));
#149945=CARTESIAN_POINT('Ctrl Pts',(-62.3526237143336,38.3210485066001,
12.));
#149946=CARTESIAN_POINT('Ctrl Pts',(-62.3373015529613,38.2999888471476,
0.));
#149947=CARTESIAN_POINT('Ctrl Pts',(-62.3373015529613,38.2999888471476,
12.));
#149948=CARTESIAN_POINT('Ctrl Pts',(-62.3219821338569,38.2789742730564,
0.));
#149949=CARTESIAN_POINT('Ctrl Pts',(-62.3219821338569,38.2789742730564,
12.));
#149950=CARTESIAN_POINT('Ctrl Pts',(-62.3066655565503,38.2580048333361,
0.));
#149951=CARTESIAN_POINT('Ctrl Pts',(-62.3066655565503,38.2580048333361,
12.));
#149952=CARTESIAN_POINT('Ctrl Pts',(-62.2913519209521,38.2370805770935,
0.));
#149953=CARTESIAN_POINT('Ctrl Pts',(-62.2913519209521,38.2370805770935,
12.));
#149954=CARTESIAN_POINT('Ctrl Pts',(-62.2760413273602,38.2162015535353,
0.));
#149955=CARTESIAN_POINT('Ctrl Pts',(-62.2760413273602,38.2162015535353,
12.));
#149956=CARTESIAN_POINT('Ctrl Pts',(-62.2607338764654,38.1953678119691,
0.));
#149957=CARTESIAN_POINT('Ctrl Pts',(-62.2607338764654,38.1953678119691,
12.));
#149958=CARTESIAN_POINT('Ctrl Pts',(-62.245429669358,38.1745794017996,0.));
#149959=CARTESIAN_POINT('Ctrl Pts',(-62.245429669358,38.1745794017996,12.));
#149960=CARTESIAN_POINT('Ctrl Pts',(-62.2301288075321,38.1538363725264,
0.));
#149961=CARTESIAN_POINT('Ctrl Pts',(-62.2301288075321,38.1538363725264,
12.));
#149962=CARTESIAN_POINT('Ctrl Pts',(-62.2148313928863,38.133138773753,0.));
#149963=CARTESIAN_POINT('Ctrl Pts',(-62.2148313928863,38.133138773753,12.));
#149964=CARTESIAN_POINT('Ctrl Pts',(-62.1995375277257,38.1124866551886,
0.));
#149965=CARTESIAN_POINT('Ctrl Pts',(-62.1995375277257,38.1124866551886,
12.));
#149966=CARTESIAN_POINT('Ctrl Pts',(-62.1842473147626,38.0918800666479,
0.));
#149967=CARTESIAN_POINT('Ctrl Pts',(-62.1842473147626,38.0918800666479,
12.));
#149968=CARTESIAN_POINT('Ctrl Pts',(-62.1689608571176,38.0713190580463,
0.));
#149969=CARTESIAN_POINT('Ctrl Pts',(-62.1689608571176,38.0713190580463,
12.));
#149970=CARTESIAN_POINT('Ctrl Pts',(-62.1536782583199,38.0508036793939,
0.));
#149971=CARTESIAN_POINT('Ctrl Pts',(-62.1536782583199,38.0508036793939,
12.));
#149972=CARTESIAN_POINT('Ctrl Pts',(-62.1383996223125,38.0303339808053,
0.));
#149973=CARTESIAN_POINT('Ctrl Pts',(-62.1383996223125,38.0303339808053,
12.));
#149974=CARTESIAN_POINT('Ctrl Pts',(-62.123125053455,38.0099100125037,0.));
#149975=CARTESIAN_POINT('Ctrl Pts',(-62.123125053455,38.0099100125037,12.));
#149976=CARTESIAN_POINT('Ctrl Pts',(-62.107854656528,37.9895318248212,0.));
#149977=CARTESIAN_POINT('Ctrl Pts',(-62.107854656528,37.9895318248212,12.));
#149978=CARTESIAN_POINT('Ctrl Pts',(-62.0925885367352,37.9691994681966,
0.));
#149979=CARTESIAN_POINT('Ctrl Pts',(-62.0925885367352,37.9691994681966,
12.));
#149980=CARTESIAN_POINT('Ctrl Pts',(-62.0773267997079,37.9489129931689,
0.));
#149981=CARTESIAN_POINT('Ctrl Pts',(-62.0773267997079,37.9489129931689,
12.));
#149982=CARTESIAN_POINT('Ctrl Pts',(-62.0620695515074,37.9286724503851,
0.));
#149983=CARTESIAN_POINT('Ctrl Pts',(-62.0620695515074,37.9286724503851,
12.));
#149984=CARTESIAN_POINT('Ctrl Pts',(-62.0468168986288,37.9084778906053,
0.));
#149985=CARTESIAN_POINT('Ctrl Pts',(-62.0468168986288,37.9084778906053,
12.));
#149986=CARTESIAN_POINT('Ctrl Pts',(-62.031568948002,37.8883293647029,0.));
#149987=CARTESIAN_POINT('Ctrl Pts',(-62.031568948002,37.8883293647029,12.));
#149988=CARTESIAN_POINT('Ctrl Pts',(-62.0163258069957,37.868226923663,0.));
#149989=CARTESIAN_POINT('Ctrl Pts',(-62.0163258069957,37.868226923663,12.));
#149990=CARTESIAN_POINT('Ctrl Pts',(-62.0010875834187,37.8481706185749,
0.));
#149991=CARTESIAN_POINT('Ctrl Pts',(-62.0010875834187,37.8481706185749,
12.));
#149992=CARTESIAN_POINT('Ctrl Pts',(-61.9858543855236,37.828160500638,0.));
#149993=CARTESIAN_POINT('Ctrl Pts',(-61.9858543855236,37.828160500638,12.));
#149994=CARTESIAN_POINT('Ctrl Pts',(-61.9706263220114,37.8081966211689,
0.));
#149995=CARTESIAN_POINT('Ctrl Pts',(-61.9706263220114,37.8081966211689,
12.));
#149996=CARTESIAN_POINT('Ctrl Pts',(-61.9554035020338,37.7882790316014,
0.));
#149997=CARTESIAN_POINT('Ctrl Pts',(-61.9554035020338,37.7882790316014,
12.));
#149998=CARTESIAN_POINT('Ctrl Pts',(-61.9401860351972,37.7684077834872,
0.));
#149999=CARTESIAN_POINT('Ctrl Pts',(-61.9401860351972,37.7684077834872,
12.));
#150000=CARTESIAN_POINT('Ctrl Pts',(-61.9249740315649,37.7485829284871,
0.));
#150001=CARTESIAN_POINT('Ctrl Pts',(-61.9249740315649,37.7485829284871,
12.));
#150002=CARTESIAN_POINT('Ctrl Pts',(-61.9097676016601,37.7288045183756,
0.));
#150003=CARTESIAN_POINT('Ctrl Pts',(-61.9097676016601,37.7288045183756,
12.));
#150004=CARTESIAN_POINT('Ctrl Pts',(-61.8945668564704,37.7090726050482,
0.));
#150005=CARTESIAN_POINT('Ctrl Pts',(-61.8945668564704,37.7090726050482,
12.));
#150006=CARTESIAN_POINT('Ctrl Pts',(-61.8793719074507,37.6893872405228,
0.));
#150007=CARTESIAN_POINT('Ctrl Pts',(-61.8793719074507,37.6893872405228,
12.));
#150008=CARTESIAN_POINT('Ctrl Pts',(-61.8641828665261,37.6697484769392,
0.));
#150009=CARTESIAN_POINT('Ctrl Pts',(-61.8641828665261,37.6697484769392,
12.));
#150010=CARTESIAN_POINT('Ctrl Pts',(-61.8489998460957,37.6501563665523,
0.));
#150011=CARTESIAN_POINT('Ctrl Pts',(-61.8489998460957,37.6501563665523,
12.));
#150012=CARTESIAN_POINT('Ctrl Pts',(-61.8338229590353,37.6306109617346,
0.));
#150013=CARTESIAN_POINT('Ctrl Pts',(-61.8338229590353,37.6306109617346,
12.));
#150014=CARTESIAN_POINT('Ctrl Pts',(-61.8186523187015,37.6111123149839,
0.));
#150015=CARTESIAN_POINT('Ctrl Pts',(-61.8186523187015,37.6111123149839,
12.));
#150016=CARTESIAN_POINT('Ctrl Pts',(-61.8034880389362,37.5916604789253,
0.));
#150017=CARTESIAN_POINT('Ctrl Pts',(-61.8034880389362,37.5916604789253,
12.));
#150018=CARTESIAN_POINT('Ctrl Pts',(-61.7883302340687,37.5722555063111,
0.));
#150019=CARTESIAN_POINT('Ctrl Pts',(-61.7883302340687,37.5722555063111,
12.));
#150020=CARTESIAN_POINT('Ctrl Pts',(-61.7731790189191,37.5528974500142,
0.));
#150021=CARTESIAN_POINT('Ctrl Pts',(-61.7731790189191,37.5528974500142,
12.));
#150022=CARTESIAN_POINT('Ctrl Pts',(-61.7580345088016,37.5335863630287,
0.));
#150023=CARTESIAN_POINT('Ctrl Pts',(-61.7580345088016,37.5335863630287,
12.));
#150024=CARTESIAN_POINT('Ctrl Pts',(-61.7428968195299,37.5143222984796,
0.));
#150025=CARTESIAN_POINT('Ctrl Pts',(-61.7428968195299,37.5143222984796,
12.));
#150026=CARTESIAN_POINT('Ctrl Pts',(-61.7277660674205,37.4951053096237,
0.));
#150027=CARTESIAN_POINT('Ctrl Pts',(-61.7277660674205,37.4951053096237,
12.));
#150028=CARTESIAN_POINT('Ctrl Pts',(-61.7126423692963,37.4759354498509,
0.));
#150029=CARTESIAN_POINT('Ctrl Pts',(-61.7126423692963,37.4759354498509,
12.));
#150030=CARTESIAN_POINT('Ctrl Pts',(-61.6975258424894,37.4568127726773,
0.));
#150031=CARTESIAN_POINT('Ctrl Pts',(-61.6975258424894,37.4568127726773,
12.));
#150032=CARTESIAN_POINT('Ctrl Pts',(-61.6824166048444,37.4377373317451,
0.));
#150033=CARTESIAN_POINT('Ctrl Pts',(-61.6824166048444,37.4377373317451,
12.));
#150034=CARTESIAN_POINT('Ctrl Pts',(-61.6673147747242,37.4187091808321,
0.));
#150035=CARTESIAN_POINT('Ctrl Pts',(-61.6673147747242,37.4187091808321,
12.));
#150036=CARTESIAN_POINT('Ctrl Pts',(-61.6522204710131,37.3997283738533,
0.));
#150037=CARTESIAN_POINT('Ctrl Pts',(-61.6522204710131,37.3997283738533,
12.));
#150038=CARTESIAN_POINT('Ctrl Pts',(-61.637133813121,37.3807949648624,0.));
#150039=CARTESIAN_POINT('Ctrl Pts',(-61.637133813121,37.3807949648624,12.));
#150040=CARTESIAN_POINT('Ctrl Pts',(-61.6220549209866,37.361909008045,0.));
#150041=CARTESIAN_POINT('Ctrl Pts',(-61.6220549209866,37.361909008045,12.));
#150042=CARTESIAN_POINT('Ctrl Pts',(-61.6069839150807,37.343070557718,0.));
#150043=CARTESIAN_POINT('Ctrl Pts',(-61.6069839150807,37.343070557718,12.));
#150044=CARTESIAN_POINT('Ctrl Pts',(-61.591920916412,37.3242796683395,0.));
#150045=CARTESIAN_POINT('Ctrl Pts',(-61.591920916412,37.3242796683395,12.));
#150046=CARTESIAN_POINT('Ctrl Pts',(-61.5768660465311,37.3055363945107,
0.));
#150047=CARTESIAN_POINT('Ctrl Pts',(-61.5768660465311,37.3055363945107,
12.));
#150048=CARTESIAN_POINT('Ctrl Pts',(-61.5618194275348,37.286840790977,0.));
#150049=CARTESIAN_POINT('Ctrl Pts',(-61.5618194275348,37.286840790977,12.));
#150050=CARTESIAN_POINT('Ctrl Pts',(-61.5467811820691,37.2681929126221,
0.));
#150051=CARTESIAN_POINT('Ctrl Pts',(-61.5467811820691,37.2681929126221,
12.));
#150052=CARTESIAN_POINT('Ctrl Pts',(-61.5317514333328,37.2495928144667,
0.));
#150053=CARTESIAN_POINT('Ctrl Pts',(-61.5317514333328,37.2495928144667,
12.));
#150054=CARTESIAN_POINT('Ctrl Pts',(-61.5167303050832,37.2310405516781,
0.));
#150055=CARTESIAN_POINT('Ctrl Pts',(-61.5167303050832,37.2310405516781,
12.));
#150056=CARTESIAN_POINT('Ctrl Pts',(-61.501717921641,37.2125361795731,0.));
#150057=CARTESIAN_POINT('Ctrl Pts',(-61.501717921641,37.2125361795731,12.));
#150058=CARTESIAN_POINT('Ctrl Pts',(-61.4867144078936,37.1940797536181,
0.));
#150059=CARTESIAN_POINT('Ctrl Pts',(-61.4867144078936,37.1940797536181,
12.));
#150060=CARTESIAN_POINT('Ctrl Pts',(-61.4717198892994,37.175671329424,0.));
#150061=CARTESIAN_POINT('Ctrl Pts',(-61.4717198892994,37.175671329424,12.));
#150062=CARTESIAN_POINT('Ctrl Pts',(-61.4567344918919,37.1573109627454,
0.));
#150063=CARTESIAN_POINT('Ctrl Pts',(-61.4567344918919,37.1573109627454,
12.));
#150064=CARTESIAN_POINT('Ctrl Pts',(-61.4417583422863,37.1389987094905,
0.));
#150065=CARTESIAN_POINT('Ctrl Pts',(-61.4417583422863,37.1389987094905,
12.));
#150066=CARTESIAN_POINT('Ctrl Pts',(-61.4267915676822,37.1207346257222,
0.));
#150067=CARTESIAN_POINT('Ctrl Pts',(-61.4267915676822,37.1207346257222,
12.));
#150068=CARTESIAN_POINT('Ctrl Pts',(-61.4118342958697,37.1025187676602,
0.));
#150069=CARTESIAN_POINT('Ctrl Pts',(-61.4118342958697,37.1025187676602,
12.));
#150070=CARTESIAN_POINT('Ctrl Pts',(-61.3968866552317,37.0843511916745,
0.));
#150071=CARTESIAN_POINT('Ctrl Pts',(-61.3968866552317,37.0843511916745,
12.));
#150072=CARTESIAN_POINT('Ctrl Pts',(-61.381948774749,37.0662319542849,0.));
#150073=CARTESIAN_POINT('Ctrl Pts',(-61.381948774749,37.0662319542849,12.));
#150074=CARTESIAN_POINT('Ctrl Pts',(-61.3670207840069,37.0481611121717,
0.));
#150075=CARTESIAN_POINT('Ctrl Pts',(-61.3670207840069,37.0481611121717,
12.));
#150076=CARTESIAN_POINT('Ctrl Pts',(-61.3521028132003,37.0301387221774,
0.));
#150077=CARTESIAN_POINT('Ctrl Pts',(-61.3521028132003,37.0301387221774,
12.));
#150078=CARTESIAN_POINT('Ctrl Pts',(-61.3371949931387,37.0121648413082,
0.));
#150079=CARTESIAN_POINT('Ctrl Pts',(-61.3371949931387,37.0121648413082,
12.));
#150080=CARTESIAN_POINT('Ctrl Pts',(-61.3222974552487,36.994239526727,0.));
#150081=CARTESIAN_POINT('Ctrl Pts',(-61.3222974552487,36.994239526727,12.));
#150082=CARTESIAN_POINT('Ctrl Pts',(-61.3074103315792,36.9763628357544,
0.));
#150083=CARTESIAN_POINT('Ctrl Pts',(-61.3074103315792,36.9763628357544,
12.));
#150084=CARTESIAN_POINT('Ctrl Pts',(-61.2925337548077,36.9585348258776,
0.));
#150085=CARTESIAN_POINT('Ctrl Pts',(-61.2925337548077,36.9585348258776,
12.));
#150086=CARTESIAN_POINT('Ctrl Pts',(-61.2776678582461,36.9407555547535,
0.));
#150087=CARTESIAN_POINT('Ctrl Pts',(-61.2776678582461,36.9407555547535,
12.));
#150088=CARTESIAN_POINT('Ctrl Pts',(-61.2628127758457,36.9230250802087,
0.));
#150089=CARTESIAN_POINT('Ctrl Pts',(-61.2628127758457,36.9230250802087,
12.));
#150090=CARTESIAN_POINT('Ctrl Pts',(-61.247968642201,36.9053434602343,0.));
#150091=CARTESIAN_POINT('Ctrl Pts',(-61.247968642201,36.9053434602343,12.));
#150092=CARTESIAN_POINT('Ctrl Pts',(-61.2331355925547,36.8877107529865,
0.));
#150093=CARTESIAN_POINT('Ctrl Pts',(-61.2331355925547,36.8877107529865,
12.));
#150094=CARTESIAN_POINT('Ctrl Pts',(-61.2183137628056,36.8701270167969,
0.));
#150095=CARTESIAN_POINT('Ctrl Pts',(-61.2183137628056,36.8701270167969,
12.));
#150096=CARTESIAN_POINT('Ctrl Pts',(-61.2035032895127,36.852592310174,0.));
#150097=CARTESIAN_POINT('Ctrl Pts',(-61.2035032895127,36.852592310174,12.));
#150098=CARTESIAN_POINT('Ctrl Pts',(-61.1887043099014,36.8351066918036,
0.));
#150099=CARTESIAN_POINT('Ctrl Pts',(-61.1887043099014,36.8351066918036,
12.));
#150100=CARTESIAN_POINT('Ctrl Pts',(-61.1739169618666,36.8176702205423,
0.));
#150101=CARTESIAN_POINT('Ctrl Pts',(-61.1739169618666,36.8176702205423,
12.));
#150102=CARTESIAN_POINT('Ctrl Pts',(-61.1591413839787,36.8002829554209,
0.));
#150103=CARTESIAN_POINT('Ctrl Pts',(-61.1591413839787,36.8002829554209,
12.));
#150104=CARTESIAN_POINT('Ctrl Pts',(-61.1443777154911,36.7829449556532,
0.));
#150105=CARTESIAN_POINT('Ctrl Pts',(-61.1443777154911,36.7829449556532,
12.));
#150106=CARTESIAN_POINT('Ctrl Pts',(-61.1296260963466,36.765656280638,0.));
#150107=CARTESIAN_POINT('Ctrl Pts',(-61.1296260963466,36.765656280638,12.));
#150108=CARTESIAN_POINT('Ctrl Pts',(-61.1148866671829,36.7484169899596,
0.));
#150109=CARTESIAN_POINT('Ctrl Pts',(-61.1148866671829,36.7484169899596,
12.));
#150110=CARTESIAN_POINT('Ctrl Pts',(-61.100159569337,36.7312271433807,0.));
#150111=CARTESIAN_POINT('Ctrl Pts',(-61.100159569337,36.7312271433807,12.));
#150112=CARTESIAN_POINT('Ctrl Pts',(-61.0854449448524,36.7140868008486,
0.));
#150113=CARTESIAN_POINT('Ctrl Pts',(-61.0854449448524,36.7140868008486,
12.));
#150114=CARTESIAN_POINT('Ctrl Pts',(-61.0707429364847,36.6969960225022,
0.));
#150115=CARTESIAN_POINT('Ctrl Pts',(-61.0707429364847,36.6969960225022,
12.));
#150116=CARTESIAN_POINT('Ctrl Pts',(-61.0560536877083,36.679954868674,0.));
#150117=CARTESIAN_POINT('Ctrl Pts',(-61.0560536877083,36.679954868674,12.));
#150118=CARTESIAN_POINT('Ctrl Pts',(-61.0413773427203,36.6629633998886,
0.));
#150119=CARTESIAN_POINT('Ctrl Pts',(-61.0413773427203,36.6629633998886,
12.));
#150120=CARTESIAN_POINT('Ctrl Pts',(-61.0267140464432,36.6460216768553,
0.));
#150121=CARTESIAN_POINT('Ctrl Pts',(-61.0267140464432,36.6460216768553,
12.));
#150122=CARTESIAN_POINT('Ctrl Pts',(-61.0120639445349,36.6291297604776,
0.));
#150123=CARTESIAN_POINT('Ctrl Pts',(-61.0120639445349,36.6291297604776,
12.));
#150124=CARTESIAN_POINT('Ctrl Pts',(-60.9974271833981,36.61228771186,0.));
#150125=CARTESIAN_POINT('Ctrl Pts',(-60.9974271833981,36.61228771186,12.));
#150126=CARTESIAN_POINT('Ctrl Pts',(-60.9828039101887,36.5954955923109,
0.));
#150127=CARTESIAN_POINT('Ctrl Pts',(-60.9828039101887,36.5954955923109,
12.));
#150128=CARTESIAN_POINT('Ctrl Pts',(-60.9681942728236,36.5787534633416,
0.));
#150129=CARTESIAN_POINT('Ctrl Pts',(-60.9681942728236,36.5787534633416,
12.));
#150130=CARTESIAN_POINT('Ctrl Pts',(-60.9535984199873,36.5620613866615,
0.));
#150131=CARTESIAN_POINT('Ctrl Pts',(-60.9535984199873,36.5620613866615,
12.));
#150132=CARTESIAN_POINT('Ctrl Pts',(-60.9390165011355,36.5454194241865,
0.));
#150133=CARTESIAN_POINT('Ctrl Pts',(-60.9390165011355,36.5454194241865,
12.));
#150134=CARTESIAN_POINT('Ctrl Pts',(-60.9244486664988,36.5288276380416,
0.));
#150135=CARTESIAN_POINT('Ctrl Pts',(-60.9244486664988,36.5288276380416,
12.));
#150136=CARTESIAN_POINT('Ctrl Pts',(-60.9098950670847,36.5122860905612,
0.));
#150137=CARTESIAN_POINT('Ctrl Pts',(-60.9098950670847,36.5122860905612,
12.));
#150138=CARTESIAN_POINT('Ctrl Pts',(-60.8953558546795,36.4957948442835,
0.));
#150139=CARTESIAN_POINT('Ctrl Pts',(-60.8953558546795,36.4957948442835,
12.));
#150140=CARTESIAN_POINT('Ctrl Pts',(-60.8808311818499,36.4793539619466,
0.));
#150141=CARTESIAN_POINT('Ctrl Pts',(-60.8808311818499,36.4793539619466,
12.));
#150142=CARTESIAN_POINT('Ctrl Pts',(-60.8663212019657,36.4629635065045,
0.));
#150143=CARTESIAN_POINT('Ctrl Pts',(-60.8663212019657,36.4629635065045,
12.));
#150144=CARTESIAN_POINT('Ctrl Pts',(-60.8518260692188,36.4466235411358,
0.));
#150145=CARTESIAN_POINT('Ctrl Pts',(-60.8518260692188,36.4466235411358,
12.));
#150146=CARTESIAN_POINT('Ctrl Pts',(-60.8373459386392,36.4303341292494,
0.));
#150147=CARTESIAN_POINT('Ctrl Pts',(-60.8373459386392,36.4303341292494,
12.));
#150148=CARTESIAN_POINT('Ctrl Pts',(-60.822880966116,36.4140953344858,0.));
#150149=CARTESIAN_POINT('Ctrl Pts',(-60.822880966116,36.4140953344858,12.));
#150150=CARTESIAN_POINT('Ctrl Pts',(-60.8084313083984,36.397907220716,0.));
#150151=CARTESIAN_POINT('Ctrl Pts',(-60.8084313083984,36.397907220716,12.));
#150152=CARTESIAN_POINT('Ctrl Pts',(-60.793997123076,36.3817698520388,0.));
#150153=CARTESIAN_POINT('Ctrl Pts',(-60.793997123076,36.3817698520388,12.));
#150154=CARTESIAN_POINT('Ctrl Pts',(-60.7795785685625,36.365683292773,0.));
#150155=CARTESIAN_POINT('Ctrl Pts',(-60.7795785685625,36.365683292773,12.));
#150156=CARTESIAN_POINT('Ctrl Pts',(-60.7651758040803,36.3496476074488,
0.));
#150157=CARTESIAN_POINT('Ctrl Pts',(-60.7651758040803,36.3496476074488,
12.));
#150158=CARTESIAN_POINT('Ctrl Pts',(-60.7507889896308,36.3336628607859,
0.));
#150159=CARTESIAN_POINT('Ctrl Pts',(-60.7507889896308,36.3336628607859,
12.));
#150160=CARTESIAN_POINT('Ctrl Pts',(-60.7364182860412,36.3177291177163,
0.));
#150161=CARTESIAN_POINT('Ctrl Pts',(-60.7364182860412,36.3177291177163,
12.));
#150162=CARTESIAN_POINT('Ctrl Pts',(-60.722063855041,36.3018464434213,0.));
#150163=CARTESIAN_POINT('Ctrl Pts',(-60.722063855041,36.3018464434213,12.));
#150164=CARTESIAN_POINT('Ctrl Pts',(-60.7077258593268,36.2860149033587,
0.));
#150165=CARTESIAN_POINT('Ctrl Pts',(-60.7077258593268,36.2860149033587,
12.));
#150166=CARTESIAN_POINT('Ctrl Pts',(-60.6934044626291,36.2702345632875,
0.));
#150167=CARTESIAN_POINT('Ctrl Pts',(-60.6934044626291,36.2702345632875,
12.));
#150168=CARTESIAN_POINT('Ctrl Pts',(-60.67909982978,36.2545054892897,0.));
#150169=CARTESIAN_POINT('Ctrl Pts',(-60.67909982978,36.2545054892897,12.));
#150170=CARTESIAN_POINT('Ctrl Pts',(-60.6648121265885,36.2388277477212,
0.));
#150171=CARTESIAN_POINT('Ctrl Pts',(-60.6648121265885,36.2388277477212,
12.));
#150172=CARTESIAN_POINT('Ctrl Pts',(-60.6505415197042,36.2232014051541,
0.));
#150173=CARTESIAN_POINT('Ctrl Pts',(-60.6505415197042,36.2232014051541,
12.));
#150174=CARTESIAN_POINT('Ctrl Pts',(-60.6362881765019,36.2076265283264,
0.));
#150175=CARTESIAN_POINT('Ctrl Pts',(-60.6362881765019,36.2076265283264,
12.));
#150176=CARTESIAN_POINT('Ctrl Pts',(-60.6220522649149,36.192103184063,0.));
#150177=CARTESIAN_POINT('Ctrl Pts',(-60.6220522649149,36.192103184063,12.));
#150178=CARTESIAN_POINT('Ctrl Pts',(-60.6078339534181,36.1766314392641,
0.));
#150179=CARTESIAN_POINT('Ctrl Pts',(-60.6078339534181,36.1766314392641,
12.));
#150180=CARTESIAN_POINT('Ctrl Pts',(-60.5936334114108,36.1612113610773,
0.));
#150181=CARTESIAN_POINT('Ctrl Pts',(-60.5936334114108,36.1612113610773,
12.));
#150182=CARTESIAN_POINT('Ctrl Pts',(-60.5794508095565,36.1458430170431,
0.));
#150183=CARTESIAN_POINT('Ctrl Pts',(-60.5794508095565,36.1458430170431,
12.));
#150184=CARTESIAN_POINT('Ctrl Pts',(-60.565286320072,36.1305264752188,0.));
#150185=CARTESIAN_POINT('Ctrl Pts',(-60.565286320072,36.1305264752188,12.));
#150186=CARTESIAN_POINT('Ctrl Pts',(-60.5511401171984,36.1152618043739,
0.));
#150187=CARTESIAN_POINT('Ctrl Pts',(-60.5511401171984,36.1152618043739,
12.));
#150188=CARTESIAN_POINT('Ctrl Pts',(-60.5370123768804,36.100049073851,0.));
#150189=CARTESIAN_POINT('Ctrl Pts',(-60.5370123768804,36.100049073851,12.));
#150190=CARTESIAN_POINT('Ctrl Pts',(-60.5229032758974,36.0848883531952,
0.));
#150191=CARTESIAN_POINT('Ctrl Pts',(-60.5229032758974,36.0848883531952,
12.));
#150192=CARTESIAN_POINT('Ctrl Pts',(-60.5088129911354,36.0697797118376,
0.));
#150193=CARTESIAN_POINT('Ctrl Pts',(-60.5088129911354,36.0697797118376,
12.));
#150194=CARTESIAN_POINT('Ctrl Pts',(-60.4947416988422,36.0547232187698,
0.));
#150195=CARTESIAN_POINT('Ctrl Pts',(-60.4947416988422,36.0547232187698,
12.));
#150196=CARTESIAN_POINT('Ctrl Pts',(-60.4806895737686,36.0397189421644,
0.));
#150197=CARTESIAN_POINT('Ctrl Pts',(-60.4806895737686,36.0397189421644,
12.));
#150198=CARTESIAN_POINT('Ctrl Pts',(-60.4666567908093,36.0247669500891,
0.));
#150199=CARTESIAN_POINT('Ctrl Pts',(-60.4666567908093,36.0247669500891,
12.));
#150200=CARTESIAN_POINT('Ctrl Pts',(-60.4526435269662,36.009867311357,0.));
#150201=CARTESIAN_POINT('Ctrl Pts',(-60.4526435269662,36.009867311357,12.));
#150202=CARTESIAN_POINT('Ctrl Pts',(-60.4386499629481,35.995020096217,0.));
#150203=CARTESIAN_POINT('Ctrl Pts',(-60.4386499629481,35.995020096217,12.));
#150204=CARTESIAN_POINT('Ctrl Pts',(-60.4246762854926,35.9802253773515,
0.));
#150205=CARTESIAN_POINT('Ctrl Pts',(-60.4246762854926,35.9802253773515,
12.));
#150206=CARTESIAN_POINT('Ctrl Pts',(-60.4107226875714,35.9654832299601,
0.));
#150207=CARTESIAN_POINT('Ctrl Pts',(-60.4107226875714,35.9654832299601,
12.));
#150208=CARTESIAN_POINT('Ctrl Pts',(-60.3967893635452,35.9507937296707,
0.));
#150209=CARTESIAN_POINT('Ctrl Pts',(-60.3967893635452,35.9507937296707,
12.));
#150210=CARTESIAN_POINT('Ctrl Pts',(-60.3828765049019,35.936156950695,0.));
#150211=CARTESIAN_POINT('Ctrl Pts',(-60.3828765049019,35.936156950695,12.));
#150212=CARTESIAN_POINT('Ctrl Pts',(-60.3689842965481,35.9215729642231,
0.));
#150213=CARTESIAN_POINT('Ctrl Pts',(-60.3689842965481,35.9215729642231,
12.));
#150214=CARTESIAN_POINT('Ctrl Pts',(-60.3551129108845,35.907041835853,0.));
#150215=CARTESIAN_POINT('Ctrl Pts',(-60.3551129108845,35.907041835853,12.));
#150216=CARTESIAN_POINT('Ctrl Pts',(-60.3412625135287,35.8925636280668,
0.));
#150217=CARTESIAN_POINT('Ctrl Pts',(-60.3412625135287,35.8925636280668,
12.));
#150218=CARTESIAN_POINT('Ctrl Pts',(-60.327433274683,35.8781384051537,0.));
#150219=CARTESIAN_POINT('Ctrl Pts',(-60.327433274683,35.8781384051537,12.));
#150220=CARTESIAN_POINT('Ctrl Pts',(-60.313625378281,35.8637662371635,0.));
#150221=CARTESIAN_POINT('Ctrl Pts',(-60.313625378281,35.8637662371635,12.));
#150222=CARTESIAN_POINT('Ctrl Pts',(-60.2998390330102,35.8494472046745,
0.));
#150223=CARTESIAN_POINT('Ctrl Pts',(-60.2998390330102,35.8494472046745,
12.));
#150224=CARTESIAN_POINT('Ctrl Pts',(-60.2860744798436,35.8351814020357,
0.));
#150225=CARTESIAN_POINT('Ctrl Pts',(-60.2860744798436,35.8351814020357,
12.));
#150226=CARTESIAN_POINT('Ctrl Pts',(-60.2723319687369,35.8209689272501,
0.));
#150227=CARTESIAN_POINT('Ctrl Pts',(-60.2723319687369,35.8209689272501,
12.));
#150228=CARTESIAN_POINT('Ctrl Pts',(-60.2586117365205,35.8068098723347,
0.));
#150229=CARTESIAN_POINT('Ctrl Pts',(-60.2586117365205,35.8068098723347,
12.));
#150230=CARTESIAN_POINT('Ctrl Pts',(-60.2449139865275,35.7927043145201,
0.));
#150231=CARTESIAN_POINT('Ctrl Pts',(-60.2449139865275,35.7927043145201,
12.));
#150232=CARTESIAN_POINT('Ctrl Pts',(-60.2312388621529,35.7786523045912,
0.));
#150233=CARTESIAN_POINT('Ctrl Pts',(-60.2312388621529,35.7786523045912,
12.));
#150234=CARTESIAN_POINT('Ctrl Pts',(-60.2175864450043,35.7646538667493,
0.));
#150235=CARTESIAN_POINT('Ctrl Pts',(-60.2175864450043,35.7646538667493,
12.));
#150236=CARTESIAN_POINT('Ctrl Pts',(-60.206682708692,35.7534979802053,0.));
#150237=CARTESIAN_POINT('Ctrl Pts',(-60.206682708692,35.7534979802053,12.));
#150238=CARTESIAN_POINT('Ctrl Pts',(-60.1985151474623,35.7451551752572,
0.));
#150239=CARTESIAN_POINT('Ctrl Pts',(-60.1985151474623,35.7451551752572,
12.));
#150240=CARTESIAN_POINT('Ctrl Pts',(-60.193074658032,35.7396040204017,0.));
#150241=CARTESIAN_POINT('Ctrl Pts',(-60.193074658032,35.7396040204017,12.));
#150242=CARTESIAN_POINT('Ctrl Pts',(-60.1903555511633,35.736831121751,0.));
#150243=CARTESIAN_POINT('Ctrl Pts',(-60.1903555511633,35.736831121751,12.));
#150244=CARTESIAN_POINT('',(-60.1903555511633,35.736831121751,12.));
#150245=CARTESIAN_POINT('Ctrl Pts',(-60.1903555511633,35.736831121751,12.));
#150246=CARTESIAN_POINT('Ctrl Pts',(-60.193074658032,35.7396040204017,12.));
#150247=CARTESIAN_POINT('Ctrl Pts',(-60.1985151474623,35.7451551752572,
12.));
#150248=CARTESIAN_POINT('Ctrl Pts',(-60.206682708692,35.7534979802053,12.));
#150249=CARTESIAN_POINT('Ctrl Pts',(-60.2175864450043,35.7646538667493,
12.));
#150250=CARTESIAN_POINT('Ctrl Pts',(-60.2312388621529,35.7786523045912,
12.));
#150251=CARTESIAN_POINT('Ctrl Pts',(-60.2449139865275,35.7927043145201,
12.));
#150252=CARTESIAN_POINT('Ctrl Pts',(-60.2586117365205,35.8068098723347,
12.));
#150253=CARTESIAN_POINT('Ctrl Pts',(-60.2723319687369,35.8209689272501,
12.));
#150254=CARTESIAN_POINT('Ctrl Pts',(-60.2860744798436,35.8351814020357,
12.));
#150255=CARTESIAN_POINT('Ctrl Pts',(-60.2998390330102,35.8494472046745,
12.));
#150256=CARTESIAN_POINT('Ctrl Pts',(-60.313625378281,35.8637662371635,12.));
#150257=CARTESIAN_POINT('Ctrl Pts',(-60.327433274683,35.8781384051537,12.));
#150258=CARTESIAN_POINT('Ctrl Pts',(-60.3412625135287,35.8925636280668,
12.));
#150259=CARTESIAN_POINT('Ctrl Pts',(-60.3551129108845,35.907041835853,12.));
#150260=CARTESIAN_POINT('Ctrl Pts',(-60.3689842965481,35.9215729642231,
12.));
#150261=CARTESIAN_POINT('Ctrl Pts',(-60.3828765049019,35.936156950695,12.));
#150262=CARTESIAN_POINT('Ctrl Pts',(-60.3967893635452,35.9507937296707,
12.));
#150263=CARTESIAN_POINT('Ctrl Pts',(-60.4107226875714,35.9654832299601,
12.));
#150264=CARTESIAN_POINT('Ctrl Pts',(-60.4246762854926,35.9802253773515,
12.));
#150265=CARTESIAN_POINT('Ctrl Pts',(-60.4386499629481,35.995020096217,12.));
#150266=CARTESIAN_POINT('Ctrl Pts',(-60.4526435269662,36.009867311357,12.));
#150267=CARTESIAN_POINT('Ctrl Pts',(-60.4666567908093,36.0247669500891,
12.));
#150268=CARTESIAN_POINT('Ctrl Pts',(-60.4806895737686,36.0397189421644,
12.));
#150269=CARTESIAN_POINT('Ctrl Pts',(-60.4947416988422,36.0547232187698,
12.));
#150270=CARTESIAN_POINT('Ctrl Pts',(-60.5088129911354,36.0697797118376,
12.));
#150271=CARTESIAN_POINT('Ctrl Pts',(-60.5229032758974,36.0848883531952,
12.));
#150272=CARTESIAN_POINT('Ctrl Pts',(-60.5370123768804,36.100049073851,12.));
#150273=CARTESIAN_POINT('Ctrl Pts',(-60.5511401171984,36.1152618043739,
12.));
#150274=CARTESIAN_POINT('Ctrl Pts',(-60.565286320072,36.1305264752188,12.));
#150275=CARTESIAN_POINT('Ctrl Pts',(-60.5794508095565,36.1458430170431,
12.));
#150276=CARTESIAN_POINT('Ctrl Pts',(-60.5936334114108,36.1612113610773,
12.));
#150277=CARTESIAN_POINT('Ctrl Pts',(-60.6078339534181,36.1766314392641,
12.));
#150278=CARTESIAN_POINT('Ctrl Pts',(-60.6220522649149,36.192103184063,12.));
#150279=CARTESIAN_POINT('Ctrl Pts',(-60.6362881765019,36.2076265283264,
12.));
#150280=CARTESIAN_POINT('Ctrl Pts',(-60.6505415197042,36.2232014051541,
12.));
#150281=CARTESIAN_POINT('Ctrl Pts',(-60.6648121265885,36.2388277477212,
12.));
#150282=CARTESIAN_POINT('Ctrl Pts',(-60.67909982978,36.2545054892897,12.));
#150283=CARTESIAN_POINT('Ctrl Pts',(-60.6934044626291,36.2702345632875,
12.));
#150284=CARTESIAN_POINT('Ctrl Pts',(-60.7077258593268,36.2860149033587,
12.));
#150285=CARTESIAN_POINT('Ctrl Pts',(-60.722063855041,36.3018464434213,12.));
#150286=CARTESIAN_POINT('Ctrl Pts',(-60.7364182860412,36.3177291177163,
12.));
#150287=CARTESIAN_POINT('Ctrl Pts',(-60.7507889896308,36.3336628607859,
12.));
#150288=CARTESIAN_POINT('Ctrl Pts',(-60.7651758040803,36.3496476074488,
12.));
#150289=CARTESIAN_POINT('Ctrl Pts',(-60.7795785685625,36.365683292773,12.));
#150290=CARTESIAN_POINT('Ctrl Pts',(-60.793997123076,36.3817698520388,12.));
#150291=CARTESIAN_POINT('Ctrl Pts',(-60.8084313083984,36.397907220716,12.));
#150292=CARTESIAN_POINT('Ctrl Pts',(-60.822880966116,36.4140953344858,12.));
#150293=CARTESIAN_POINT('Ctrl Pts',(-60.8373459386392,36.4303341292494,
12.));
#150294=CARTESIAN_POINT('Ctrl Pts',(-60.8518260692188,36.4466235411358,
12.));
#150295=CARTESIAN_POINT('Ctrl Pts',(-60.8663212019657,36.4629635065045,
12.));
#150296=CARTESIAN_POINT('Ctrl Pts',(-60.8808311818499,36.4793539619466,
12.));
#150297=CARTESIAN_POINT('Ctrl Pts',(-60.8953558546795,36.4957948442835,
12.));
#150298=CARTESIAN_POINT('Ctrl Pts',(-60.9098950670847,36.5122860905612,
12.));
#150299=CARTESIAN_POINT('Ctrl Pts',(-60.9244486664988,36.5288276380416,
12.));
#150300=CARTESIAN_POINT('Ctrl Pts',(-60.9390165011355,36.5454194241865,
12.));
#150301=CARTESIAN_POINT('Ctrl Pts',(-60.9535984199873,36.5620613866615,
12.));
#150302=CARTESIAN_POINT('Ctrl Pts',(-60.9681942728236,36.5787534633416,
12.));
#150303=CARTESIAN_POINT('Ctrl Pts',(-60.9828039101887,36.5954955923109,
12.));
#150304=CARTESIAN_POINT('Ctrl Pts',(-60.9974271833981,36.61228771186,12.));
#150305=CARTESIAN_POINT('Ctrl Pts',(-61.0120639445349,36.6291297604776,
12.));
#150306=CARTESIAN_POINT('Ctrl Pts',(-61.0267140464432,36.6460216768553,
12.));
#150307=CARTESIAN_POINT('Ctrl Pts',(-61.0413773427203,36.6629633998886,
12.));
#150308=CARTESIAN_POINT('Ctrl Pts',(-61.0560536877083,36.679954868674,12.));
#150309=CARTESIAN_POINT('Ctrl Pts',(-61.0707429364847,36.6969960225022,
12.));
#150310=CARTESIAN_POINT('Ctrl Pts',(-61.0854449448524,36.7140868008486,
12.));
#150311=CARTESIAN_POINT('Ctrl Pts',(-61.100159569337,36.7312271433807,12.));
#150312=CARTESIAN_POINT('Ctrl Pts',(-61.1148866671829,36.7484169899596,
12.));
#150313=CARTESIAN_POINT('Ctrl Pts',(-61.1296260963466,36.765656280638,12.));
#150314=CARTESIAN_POINT('Ctrl Pts',(-61.1443777154911,36.7829449556532,
12.));
#150315=CARTESIAN_POINT('Ctrl Pts',(-61.1591413839787,36.8002829554209,
12.));
#150316=CARTESIAN_POINT('Ctrl Pts',(-61.1739169618666,36.8176702205423,
12.));
#150317=CARTESIAN_POINT('Ctrl Pts',(-61.1887043099014,36.8351066918036,
12.));
#150318=CARTESIAN_POINT('Ctrl Pts',(-61.2035032895127,36.852592310174,12.));
#150319=CARTESIAN_POINT('Ctrl Pts',(-61.2183137628056,36.8701270167969,
12.));
#150320=CARTESIAN_POINT('Ctrl Pts',(-61.2331355925547,36.8877107529865,
12.));
#150321=CARTESIAN_POINT('Ctrl Pts',(-61.247968642201,36.9053434602343,12.));
#150322=CARTESIAN_POINT('Ctrl Pts',(-61.2628127758457,36.9230250802087,
12.));
#150323=CARTESIAN_POINT('Ctrl Pts',(-61.2776678582461,36.9407555547535,
12.));
#150324=CARTESIAN_POINT('Ctrl Pts',(-61.2925337548077,36.9585348258776,
12.));
#150325=CARTESIAN_POINT('Ctrl Pts',(-61.3074103315792,36.9763628357544,
12.));
#150326=CARTESIAN_POINT('Ctrl Pts',(-61.3222974552487,36.994239526727,12.));
#150327=CARTESIAN_POINT('Ctrl Pts',(-61.3371949931387,37.0121648413082,
12.));
#150328=CARTESIAN_POINT('Ctrl Pts',(-61.3521028132003,37.0301387221774,
12.));
#150329=CARTESIAN_POINT('Ctrl Pts',(-61.3670207840069,37.0481611121717,
12.));
#150330=CARTESIAN_POINT('Ctrl Pts',(-61.381948774749,37.0662319542849,12.));
#150331=CARTESIAN_POINT('Ctrl Pts',(-61.3968866552317,37.0843511916745,
12.));
#150332=CARTESIAN_POINT('Ctrl Pts',(-61.4118342958697,37.1025187676602,
12.));
#150333=CARTESIAN_POINT('Ctrl Pts',(-61.4267915676822,37.1207346257222,
12.));
#150334=CARTESIAN_POINT('Ctrl Pts',(-61.4417583422863,37.1389987094905,
12.));
#150335=CARTESIAN_POINT('Ctrl Pts',(-61.4567344918919,37.1573109627454,
12.));
#150336=CARTESIAN_POINT('Ctrl Pts',(-61.4717198892994,37.175671329424,12.));
#150337=CARTESIAN_POINT('Ctrl Pts',(-61.4867144078936,37.1940797536181,
12.));
#150338=CARTESIAN_POINT('Ctrl Pts',(-61.501717921641,37.2125361795731,12.));
#150339=CARTESIAN_POINT('Ctrl Pts',(-61.5167303050832,37.2310405516781,
12.));
#150340=CARTESIAN_POINT('Ctrl Pts',(-61.5317514333328,37.2495928144667,
12.));
#150341=CARTESIAN_POINT('Ctrl Pts',(-61.5467811820691,37.2681929126221,
12.));
#150342=CARTESIAN_POINT('Ctrl Pts',(-61.5618194275348,37.286840790977,12.));
#150343=CARTESIAN_POINT('Ctrl Pts',(-61.5768660465311,37.3055363945107,
12.));
#150344=CARTESIAN_POINT('Ctrl Pts',(-61.591920916412,37.3242796683395,12.));
#150345=CARTESIAN_POINT('Ctrl Pts',(-61.6069839150807,37.343070557718,12.));
#150346=CARTESIAN_POINT('Ctrl Pts',(-61.6220549209866,37.361909008045,12.));
#150347=CARTESIAN_POINT('Ctrl Pts',(-61.637133813121,37.3807949648624,12.));
#150348=CARTESIAN_POINT('Ctrl Pts',(-61.6522204710131,37.3997283738533,
12.));
#150349=CARTESIAN_POINT('Ctrl Pts',(-61.6673147747242,37.4187091808321,
12.));
#150350=CARTESIAN_POINT('Ctrl Pts',(-61.6824166048444,37.4377373317451,
12.));
#150351=CARTESIAN_POINT('Ctrl Pts',(-61.6975258424894,37.4568127726773,
12.));
#150352=CARTESIAN_POINT('Ctrl Pts',(-61.7126423692963,37.4759354498509,
12.));
#150353=CARTESIAN_POINT('Ctrl Pts',(-61.7277660674205,37.4951053096237,
12.));
#150354=CARTESIAN_POINT('Ctrl Pts',(-61.7428968195299,37.5143222984796,
12.));
#150355=CARTESIAN_POINT('Ctrl Pts',(-61.7580345088016,37.5335863630287,
12.));
#150356=CARTESIAN_POINT('Ctrl Pts',(-61.7731790189191,37.5528974500142,
12.));
#150357=CARTESIAN_POINT('Ctrl Pts',(-61.7883302340687,37.5722555063111,
12.));
#150358=CARTESIAN_POINT('Ctrl Pts',(-61.8034880389362,37.5916604789253,
12.));
#150359=CARTESIAN_POINT('Ctrl Pts',(-61.8186523187015,37.6111123149839,
12.));
#150360=CARTESIAN_POINT('Ctrl Pts',(-61.8338229590353,37.6306109617346,
12.));
#150361=CARTESIAN_POINT('Ctrl Pts',(-61.8489998460957,37.6501563665523,
12.));
#150362=CARTESIAN_POINT('Ctrl Pts',(-61.8641828665261,37.6697484769392,
12.));
#150363=CARTESIAN_POINT('Ctrl Pts',(-61.8793719074507,37.6893872405228,
12.));
#150364=CARTESIAN_POINT('Ctrl Pts',(-61.8945668564704,37.7090726050482,
12.));
#150365=CARTESIAN_POINT('Ctrl Pts',(-61.9097676016601,37.7288045183756,
12.));
#150366=CARTESIAN_POINT('Ctrl Pts',(-61.9249740315649,37.7485829284871,
12.));
#150367=CARTESIAN_POINT('Ctrl Pts',(-61.9401860351972,37.7684077834872,
12.));
#150368=CARTESIAN_POINT('Ctrl Pts',(-61.9554035020338,37.7882790316014,
12.));
#150369=CARTESIAN_POINT('Ctrl Pts',(-61.9706263220114,37.8081966211689,
12.));
#150370=CARTESIAN_POINT('Ctrl Pts',(-61.9858543855236,37.828160500638,12.));
#150371=CARTESIAN_POINT('Ctrl Pts',(-62.0010875834187,37.8481706185749,
12.));
#150372=CARTESIAN_POINT('Ctrl Pts',(-62.0163258069957,37.868226923663,12.));
#150373=CARTESIAN_POINT('Ctrl Pts',(-62.031568948002,37.8883293647029,12.));
#150374=CARTESIAN_POINT('Ctrl Pts',(-62.0468168986288,37.9084778906053,
12.));
#150375=CARTESIAN_POINT('Ctrl Pts',(-62.0620695515074,37.9286724503851,
12.));
#150376=CARTESIAN_POINT('Ctrl Pts',(-62.0773267997079,37.9489129931689,
12.));
#150377=CARTESIAN_POINT('Ctrl Pts',(-62.0925885367352,37.9691994681966,
12.));
#150378=CARTESIAN_POINT('Ctrl Pts',(-62.107854656528,37.9895318248212,12.));
#150379=CARTESIAN_POINT('Ctrl Pts',(-62.123125053455,38.0099100125037,12.));
#150380=CARTESIAN_POINT('Ctrl Pts',(-62.1383996223125,38.0303339808053,
12.));
#150381=CARTESIAN_POINT('Ctrl Pts',(-62.1536782583199,38.0508036793939,
12.));
#150382=CARTESIAN_POINT('Ctrl Pts',(-62.1689608571176,38.0713190580463,
12.));
#150383=CARTESIAN_POINT('Ctrl Pts',(-62.1842473147626,38.0918800666479,
12.));
#150384=CARTESIAN_POINT('Ctrl Pts',(-62.1995375277257,38.1124866551886,
12.));
#150385=CARTESIAN_POINT('Ctrl Pts',(-62.2148313928863,38.133138773753,12.));
#150386=CARTESIAN_POINT('Ctrl Pts',(-62.2301288075321,38.1538363725264,
12.));
#150387=CARTESIAN_POINT('Ctrl Pts',(-62.245429669358,38.1745794017996,12.));
#150388=CARTESIAN_POINT('Ctrl Pts',(-62.2607338764654,38.1953678119691,
12.));
#150389=CARTESIAN_POINT('Ctrl Pts',(-62.2760413273602,38.2162015535353,
12.));
#150390=CARTESIAN_POINT('Ctrl Pts',(-62.2913519209521,38.2370805770935,
12.));
#150391=CARTESIAN_POINT('Ctrl Pts',(-62.3066655565503,38.2580048333361,
12.));
#150392=CARTESIAN_POINT('Ctrl Pts',(-62.3219821338569,38.2789742730564,
12.));
#150393=CARTESIAN_POINT('Ctrl Pts',(-62.3373015529613,38.2999888471476,
12.));
#150394=CARTESIAN_POINT('Ctrl Pts',(-62.3526237143336,38.3210485066001,
12.));
#150395=CARTESIAN_POINT('Ctrl Pts',(-62.3679485188172,38.342153202491,12.));
#150396=CARTESIAN_POINT('Ctrl Pts',(-62.3832758676271,38.3633028859828,
12.));
#150397=CARTESIAN_POINT('Ctrl Pts',(-62.3986056623577,38.3844975083343,
12.));
#150398=CARTESIAN_POINT('Ctrl Pts',(-62.4139378049885,38.405737020905,12.));
#150399=CARTESIAN_POINT('Ctrl Pts',(-62.4292721978901,38.4270213751568,
12.));
#150400=CARTESIAN_POINT('Ctrl Pts',(-62.4446087438312,38.4483505226518,
12.));
#150401=CARTESIAN_POINT('Ctrl Pts',(-62.4599473459811,38.4697244150482,
12.));
#150402=CARTESIAN_POINT('Ctrl Pts',(-62.4752879078854,38.4911430040997,
12.));
#150403=CARTESIAN_POINT('Ctrl Pts',(-62.4906303334443,38.5126062416502,
12.));
#150404=CARTESIAN_POINT('Ctrl Pts',(-62.5059745268901,38.5341140796248,
12.));
#150405=CARTESIAN_POINT('Ctrl Pts',(-62.5213203927663,38.5556664700195,
12.));
#150406=CARTESIAN_POINT('Ctrl Pts',(-62.5366678359023,38.5772633648832,
12.));
#150407=CARTESIAN_POINT('Ctrl Pts',(-62.5520167614516,38.5989047163393,
12.));
#150408=CARTESIAN_POINT('Ctrl Pts',(-62.5673670749361,38.6205904766073,
12.));
#150409=CARTESIAN_POINT('Ctrl Pts',(-62.5827186822921,38.6423205980213,
12.));
#150410=CARTESIAN_POINT('Ctrl Pts',(-62.5980714899052,38.6640950330421,
12.));
#150411=CARTESIAN_POINT('Ctrl Pts',(-62.6134254046739,38.6859137342731,
12.));
#150412=CARTESIAN_POINT('Ctrl Pts',(-62.6287803339542,38.7077766544416,
12.));
#150413=CARTESIAN_POINT('Ctrl Pts',(-62.6441361854411,38.7296837463609,
12.));
#150414=CARTESIAN_POINT('Ctrl Pts',(-62.6594928670628,38.7516349628904,
12.));
#150415=CARTESIAN_POINT('Ctrl Pts',(-62.6748502868835,38.7736302568982,
12.));
#150416=CARTESIAN_POINT('Ctrl Pts',(-62.6902083529694,38.795669581203,12.));
#150417=CARTESIAN_POINT('Ctrl Pts',(-62.7055669733802,38.8177528885681,
12.));
#150418=CARTESIAN_POINT('Ctrl Pts',(-62.7209260564493,38.8398801318177,
12.));
#150419=CARTESIAN_POINT('Ctrl Pts',(-62.7362855110042,38.8620512639232,
12.));
#150420=CARTESIAN_POINT('Ctrl Pts',(-62.7516452466128,38.8842662380984,
12.));
#150421=CARTESIAN_POINT('Ctrl Pts',(-62.7670051738143,38.9065250078832,
12.));
#150422=CARTESIAN_POINT('Ctrl Pts',(-62.78236520437,38.9288275272335,12.));
#150423=CARTESIAN_POINT('Ctrl Pts',(-62.7977252507118,38.9511737503165,
12.));
#150424=CARTESIAN_POINT('Ctrl Pts',(-62.8130852254027,38.9735636313089,
12.));
#150425=CARTESIAN_POINT('Ctrl Pts',(-62.8284450405459,38.9959971241701,
12.));
#150426=CARTESIAN_POINT('Ctrl Pts',(-62.8438046073224,39.0184741824641,
12.));
#150427=CARTESIAN_POINT('Ctrl Pts',(-62.8591638352056,39.0409947590497,
12.));
#150428=CARTESIAN_POINT('Ctrl Pts',(-62.8745226325998,39.0635588063276,
12.));
#150429=CARTESIAN_POINT('Ctrl Pts',(-62.8898809082612,39.0861662767932,
12.));
#150430=CARTESIAN_POINT('Ctrl Pts',(-62.9052385725387,39.1088171235125,
12.));
#150431=CARTESIAN_POINT('Ctrl Pts',(-62.9205955385558,39.131511300575,12.));
#150432=CARTESIAN_POINT('Ctrl Pts',(-62.9359517237404,39.1542487636744,
12.));
#150433=CARTESIAN_POINT('Ctrl Pts',(-62.9513070501867,39.1770294702428,
12.));
#150434=CARTESIAN_POINT('Ctrl Pts',(-62.9644687386836,39.1965939820933,
12.));
#150435=CARTESIAN_POINT('Ctrl Pts',(-62.9745590018672,39.2116170128461,
12.));
#150436=CARTESIAN_POINT('Ctrl Pts',(-62.9815782721325,39.2220794388806,
12.));
#150437=CARTESIAN_POINT('Ctrl Pts',(-62.9855268616127,39.2279686275006,
12.));
#150438=CARTESIAN_POINT('Ctrl Pts',(-62.9864049293894,39.2292784191812,
12.));
#150439=CARTESIAN_POINT('',(-60.1903555511633,35.736831121751,0.));
#150440=CARTESIAN_POINT('',(-60.1903555511633,35.7368311217509,0.));
#150441=CARTESIAN_POINT('Ctrl Pts',(-62.9864049293893,39.2292784191812,
0.));
#150442=CARTESIAN_POINT('Ctrl Pts',(-62.9855268616127,39.2279686275006,
0.));
#150443=CARTESIAN_POINT('Ctrl Pts',(-62.9815782721325,39.2220794388806,
0.));
#150444=CARTESIAN_POINT('Ctrl Pts',(-62.9745590018672,39.211617012846,0.));
#150445=CARTESIAN_POINT('Ctrl Pts',(-62.9644687386836,39.1965939820933,
0.));
#150446=CARTESIAN_POINT('Ctrl Pts',(-62.9513070501867,39.1770294702428,
0.));
#150447=CARTESIAN_POINT('Ctrl Pts',(-62.9359517237404,39.1542487636744,
0.));
#150448=CARTESIAN_POINT('Ctrl Pts',(-62.9205955385558,39.131511300575,0.));
#150449=CARTESIAN_POINT('Ctrl Pts',(-62.9052385725387,39.1088171235125,
0.));
#150450=CARTESIAN_POINT('Ctrl Pts',(-62.8898809082612,39.0861662767932,
0.));
#150451=CARTESIAN_POINT('Ctrl Pts',(-62.8745226325998,39.0635588063276,
0.));
#150452=CARTESIAN_POINT('Ctrl Pts',(-62.8591638352056,39.0409947590497,
0.));
#150453=CARTESIAN_POINT('Ctrl Pts',(-62.8438046073224,39.0184741824641,
0.));
#150454=CARTESIAN_POINT('Ctrl Pts',(-62.8284450405459,38.9959971241701,
0.));
#150455=CARTESIAN_POINT('Ctrl Pts',(-62.8130852254027,38.9735636313089,
0.));
#150456=CARTESIAN_POINT('Ctrl Pts',(-62.7977252507118,38.9511737503165,
0.));
#150457=CARTESIAN_POINT('Ctrl Pts',(-62.78236520437,38.9288275272335,0.));
#150458=CARTESIAN_POINT('Ctrl Pts',(-62.7670051738143,38.9065250078832,
0.));
#150459=CARTESIAN_POINT('Ctrl Pts',(-62.7516452466128,38.8842662380984,
0.));
#150460=CARTESIAN_POINT('Ctrl Pts',(-62.7362855110042,38.8620512639232,
0.));
#150461=CARTESIAN_POINT('Ctrl Pts',(-62.7209260564493,38.8398801318177,
0.));
#150462=CARTESIAN_POINT('Ctrl Pts',(-62.7055669733802,38.8177528885681,
0.));
#150463=CARTESIAN_POINT('Ctrl Pts',(-62.6902083529694,38.795669581203,0.));
#150464=CARTESIAN_POINT('Ctrl Pts',(-62.6748502868835,38.7736302568982,
0.));
#150465=CARTESIAN_POINT('Ctrl Pts',(-62.6594928670628,38.7516349628904,
0.));
#150466=CARTESIAN_POINT('Ctrl Pts',(-62.6441361854411,38.7296837463609,
0.));
#150467=CARTESIAN_POINT('Ctrl Pts',(-62.6287803339542,38.7077766544416,
0.));
#150468=CARTESIAN_POINT('Ctrl Pts',(-62.6134254046739,38.6859137342731,
0.));
#150469=CARTESIAN_POINT('Ctrl Pts',(-62.5980714899052,38.6640950330421,
0.));
#150470=CARTESIAN_POINT('Ctrl Pts',(-62.5827186822921,38.6423205980213,
0.));
#150471=CARTESIAN_POINT('Ctrl Pts',(-62.5673670749361,38.6205904766073,
0.));
#150472=CARTESIAN_POINT('Ctrl Pts',(-62.5520167614516,38.5989047163393,
0.));
#150473=CARTESIAN_POINT('Ctrl Pts',(-62.5366678359023,38.5772633648832,
0.));
#150474=CARTESIAN_POINT('Ctrl Pts',(-62.5213203927663,38.5556664700195,
0.));
#150475=CARTESIAN_POINT('Ctrl Pts',(-62.5059745268901,38.5341140796248,
0.));
#150476=CARTESIAN_POINT('Ctrl Pts',(-62.4906303334443,38.5126062416502,
0.));
#150477=CARTESIAN_POINT('Ctrl Pts',(-62.4752879078854,38.4911430040997,
0.));
#150478=CARTESIAN_POINT('Ctrl Pts',(-62.4599473459811,38.4697244150482,
0.));
#150479=CARTESIAN_POINT('Ctrl Pts',(-62.4446087438312,38.4483505226518,
0.));
#150480=CARTESIAN_POINT('Ctrl Pts',(-62.4292721978901,38.4270213751568,
0.));
#150481=CARTESIAN_POINT('Ctrl Pts',(-62.4139378049885,38.405737020905,0.));
#150482=CARTESIAN_POINT('Ctrl Pts',(-62.3986056623577,38.3844975083343,
0.));
#150483=CARTESIAN_POINT('Ctrl Pts',(-62.3832758676271,38.3633028859828,
0.));
#150484=CARTESIAN_POINT('Ctrl Pts',(-62.3679485188172,38.342153202491,0.));
#150485=CARTESIAN_POINT('Ctrl Pts',(-62.3526237143336,38.3210485066001,
0.));
#150486=CARTESIAN_POINT('Ctrl Pts',(-62.3373015529613,38.2999888471476,
0.));
#150487=CARTESIAN_POINT('Ctrl Pts',(-62.3219821338569,38.2789742730564,
0.));
#150488=CARTESIAN_POINT('Ctrl Pts',(-62.3066655565503,38.2580048333361,
0.));
#150489=CARTESIAN_POINT('Ctrl Pts',(-62.2913519209521,38.2370805770935,
0.));
#150490=CARTESIAN_POINT('Ctrl Pts',(-62.2760413273602,38.2162015535353,
0.));
#150491=CARTESIAN_POINT('Ctrl Pts',(-62.2607338764654,38.1953678119691,
0.));
#150492=CARTESIAN_POINT('Ctrl Pts',(-62.245429669358,38.1745794017996,0.));
#150493=CARTESIAN_POINT('Ctrl Pts',(-62.2301288075321,38.1538363725264,
0.));
#150494=CARTESIAN_POINT('Ctrl Pts',(-62.2148313928863,38.133138773753,0.));
#150495=CARTESIAN_POINT('Ctrl Pts',(-62.1995375277257,38.1124866551886,
0.));
#150496=CARTESIAN_POINT('Ctrl Pts',(-62.1842473147626,38.0918800666479,
0.));
#150497=CARTESIAN_POINT('Ctrl Pts',(-62.1689608571176,38.0713190580463,
0.));
#150498=CARTESIAN_POINT('Ctrl Pts',(-62.1536782583199,38.0508036793939,
0.));
#150499=CARTESIAN_POINT('Ctrl Pts',(-62.1383996223125,38.0303339808053,
0.));
#150500=CARTESIAN_POINT('Ctrl Pts',(-62.123125053455,38.0099100125037,0.));
#150501=CARTESIAN_POINT('Ctrl Pts',(-62.107854656528,37.9895318248212,0.));
#150502=CARTESIAN_POINT('Ctrl Pts',(-62.0925885367352,37.9691994681966,
0.));
#150503=CARTESIAN_POINT('Ctrl Pts',(-62.0773267997079,37.9489129931689,
0.));
#150504=CARTESIAN_POINT('Ctrl Pts',(-62.0620695515074,37.9286724503851,
0.));
#150505=CARTESIAN_POINT('Ctrl Pts',(-62.0468168986288,37.9084778906053,
0.));
#150506=CARTESIAN_POINT('Ctrl Pts',(-62.031568948002,37.8883293647029,0.));
#150507=CARTESIAN_POINT('Ctrl Pts',(-62.0163258069957,37.868226923663,0.));
#150508=CARTESIAN_POINT('Ctrl Pts',(-62.0010875834187,37.8481706185749,
0.));
#150509=CARTESIAN_POINT('Ctrl Pts',(-61.9858543855236,37.828160500638,0.));
#150510=CARTESIAN_POINT('Ctrl Pts',(-61.9706263220114,37.8081966211689,
0.));
#150511=CARTESIAN_POINT('Ctrl Pts',(-61.9554035020338,37.7882790316014,
0.));
#150512=CARTESIAN_POINT('Ctrl Pts',(-61.9401860351972,37.7684077834872,
0.));
#150513=CARTESIAN_POINT('Ctrl Pts',(-61.9249740315649,37.7485829284871,
0.));
#150514=CARTESIAN_POINT('Ctrl Pts',(-61.9097676016601,37.7288045183756,
0.));
#150515=CARTESIAN_POINT('Ctrl Pts',(-61.8945668564704,37.7090726050482,
0.));
#150516=CARTESIAN_POINT('Ctrl Pts',(-61.8793719074507,37.6893872405228,
0.));
#150517=CARTESIAN_POINT('Ctrl Pts',(-61.8641828665261,37.6697484769392,
0.));
#150518=CARTESIAN_POINT('Ctrl Pts',(-61.8489998460957,37.6501563665523,
0.));
#150519=CARTESIAN_POINT('Ctrl Pts',(-61.8338229590353,37.6306109617346,
0.));
#150520=CARTESIAN_POINT('Ctrl Pts',(-61.8186523187015,37.6111123149839,
0.));
#150521=CARTESIAN_POINT('Ctrl Pts',(-61.8034880389362,37.5916604789253,
0.));
#150522=CARTESIAN_POINT('Ctrl Pts',(-61.7883302340687,37.5722555063111,
0.));
#150523=CARTESIAN_POINT('Ctrl Pts',(-61.7731790189191,37.5528974500142,
0.));
#150524=CARTESIAN_POINT('Ctrl Pts',(-61.7580345088016,37.5335863630287,
0.));
#150525=CARTESIAN_POINT('Ctrl Pts',(-61.7428968195299,37.5143222984796,
0.));
#150526=CARTESIAN_POINT('Ctrl Pts',(-61.7277660674205,37.4951053096237,
0.));
#150527=CARTESIAN_POINT('Ctrl Pts',(-61.7126423692963,37.4759354498509,
0.));
#150528=CARTESIAN_POINT('Ctrl Pts',(-61.6975258424894,37.4568127726773,
0.));
#150529=CARTESIAN_POINT('Ctrl Pts',(-61.6824166048444,37.4377373317451,
0.));
#150530=CARTESIAN_POINT('Ctrl Pts',(-61.6673147747242,37.4187091808321,
0.));
#150531=CARTESIAN_POINT('Ctrl Pts',(-61.6522204710131,37.3997283738533,
0.));
#150532=CARTESIAN_POINT('Ctrl Pts',(-61.637133813121,37.3807949648624,0.));
#150533=CARTESIAN_POINT('Ctrl Pts',(-61.6220549209866,37.361909008045,0.));
#150534=CARTESIAN_POINT('Ctrl Pts',(-61.6069839150807,37.343070557718,0.));
#150535=CARTESIAN_POINT('Ctrl Pts',(-61.591920916412,37.3242796683395,0.));
#150536=CARTESIAN_POINT('Ctrl Pts',(-61.5768660465311,37.3055363945107,
0.));
#150537=CARTESIAN_POINT('Ctrl Pts',(-61.5618194275348,37.286840790977,0.));
#150538=CARTESIAN_POINT('Ctrl Pts',(-61.5467811820691,37.2681929126221,
0.));
#150539=CARTESIAN_POINT('Ctrl Pts',(-61.5317514333328,37.2495928144667,
0.));
#150540=CARTESIAN_POINT('Ctrl Pts',(-61.5167303050832,37.2310405516781,
0.));
#150541=CARTESIAN_POINT('Ctrl Pts',(-61.501717921641,37.2125361795731,0.));
#150542=CARTESIAN_POINT('Ctrl Pts',(-61.4867144078936,37.1940797536181,
0.));
#150543=CARTESIAN_POINT('Ctrl Pts',(-61.4717198892994,37.175671329424,0.));
#150544=CARTESIAN_POINT('Ctrl Pts',(-61.4567344918919,37.1573109627454,
0.));
#150545=CARTESIAN_POINT('Ctrl Pts',(-61.4417583422863,37.1389987094905,
0.));
#150546=CARTESIAN_POINT('Ctrl Pts',(-61.4267915676822,37.1207346257222,
0.));
#150547=CARTESIAN_POINT('Ctrl Pts',(-61.4118342958697,37.1025187676602,
0.));
#150548=CARTESIAN_POINT('Ctrl Pts',(-61.3968866552317,37.0843511916745,
0.));
#150549=CARTESIAN_POINT('Ctrl Pts',(-61.381948774749,37.0662319542849,0.));
#150550=CARTESIAN_POINT('Ctrl Pts',(-61.3670207840069,37.0481611121717,
0.));
#150551=CARTESIAN_POINT('Ctrl Pts',(-61.3521028132003,37.0301387221774,
0.));
#150552=CARTESIAN_POINT('Ctrl Pts',(-61.3371949931387,37.0121648413082,
0.));
#150553=CARTESIAN_POINT('Ctrl Pts',(-61.3222974552487,36.994239526727,0.));
#150554=CARTESIAN_POINT('Ctrl Pts',(-61.3074103315792,36.9763628357544,
0.));
#150555=CARTESIAN_POINT('Ctrl Pts',(-61.2925337548077,36.9585348258776,
0.));
#150556=CARTESIAN_POINT('Ctrl Pts',(-61.2776678582461,36.9407555547535,
0.));
#150557=CARTESIAN_POINT('Ctrl Pts',(-61.2628127758457,36.9230250802087,
0.));
#150558=CARTESIAN_POINT('Ctrl Pts',(-61.247968642201,36.9053434602343,0.));
#150559=CARTESIAN_POINT('Ctrl Pts',(-61.2331355925547,36.8877107529865,
0.));
#150560=CARTESIAN_POINT('Ctrl Pts',(-61.2183137628056,36.8701270167969,
0.));
#150561=CARTESIAN_POINT('Ctrl Pts',(-61.2035032895127,36.852592310174,0.));
#150562=CARTESIAN_POINT('Ctrl Pts',(-61.1887043099014,36.8351066918036,
0.));
#150563=CARTESIAN_POINT('Ctrl Pts',(-61.1739169618666,36.8176702205423,
0.));
#150564=CARTESIAN_POINT('Ctrl Pts',(-61.1591413839787,36.8002829554209,
0.));
#150565=CARTESIAN_POINT('Ctrl Pts',(-61.1443777154911,36.7829449556532,
0.));
#150566=CARTESIAN_POINT('Ctrl Pts',(-61.1296260963466,36.765656280638,0.));
#150567=CARTESIAN_POINT('Ctrl Pts',(-61.1148866671829,36.7484169899596,
0.));
#150568=CARTESIAN_POINT('Ctrl Pts',(-61.100159569337,36.7312271433807,0.));
#150569=CARTESIAN_POINT('Ctrl Pts',(-61.0854449448524,36.7140868008486,
0.));
#150570=CARTESIAN_POINT('Ctrl Pts',(-61.0707429364847,36.6969960225022,
0.));
#150571=CARTESIAN_POINT('Ctrl Pts',(-61.0560536877083,36.679954868674,0.));
#150572=CARTESIAN_POINT('Ctrl Pts',(-61.0413773427203,36.6629633998886,
0.));
#150573=CARTESIAN_POINT('Ctrl Pts',(-61.0267140464432,36.6460216768553,
0.));
#150574=CARTESIAN_POINT('Ctrl Pts',(-61.0120639445349,36.6291297604776,
0.));
#150575=CARTESIAN_POINT('Ctrl Pts',(-60.9974271833981,36.61228771186,0.));
#150576=CARTESIAN_POINT('Ctrl Pts',(-60.9828039101887,36.5954955923109,
0.));
#150577=CARTESIAN_POINT('Ctrl Pts',(-60.9681942728236,36.5787534633416,
0.));
#150578=CARTESIAN_POINT('Ctrl Pts',(-60.9535984199873,36.5620613866615,
0.));
#150579=CARTESIAN_POINT('Ctrl Pts',(-60.9390165011355,36.5454194241865,
0.));
#150580=CARTESIAN_POINT('Ctrl Pts',(-60.9244486664988,36.5288276380416,
0.));
#150581=CARTESIAN_POINT('Ctrl Pts',(-60.9098950670847,36.5122860905612,
0.));
#150582=CARTESIAN_POINT('Ctrl Pts',(-60.8953558546795,36.4957948442835,
0.));
#150583=CARTESIAN_POINT('Ctrl Pts',(-60.8808311818499,36.4793539619466,
0.));
#150584=CARTESIAN_POINT('Ctrl Pts',(-60.8663212019657,36.4629635065045,
0.));
#150585=CARTESIAN_POINT('Ctrl Pts',(-60.8518260692188,36.4466235411358,
0.));
#150586=CARTESIAN_POINT('Ctrl Pts',(-60.8373459386392,36.4303341292494,
0.));
#150587=CARTESIAN_POINT('Ctrl Pts',(-60.822880966116,36.4140953344858,0.));
#150588=CARTESIAN_POINT('Ctrl Pts',(-60.8084313083984,36.397907220716,0.));
#150589=CARTESIAN_POINT('Ctrl Pts',(-60.793997123076,36.3817698520388,0.));
#150590=CARTESIAN_POINT('Ctrl Pts',(-60.7795785685625,36.365683292773,0.));
#150591=CARTESIAN_POINT('Ctrl Pts',(-60.7651758040803,36.3496476074488,
0.));
#150592=CARTESIAN_POINT('Ctrl Pts',(-60.7507889896308,36.3336628607859,
0.));
#150593=CARTESIAN_POINT('Ctrl Pts',(-60.7364182860412,36.3177291177163,
0.));
#150594=CARTESIAN_POINT('Ctrl Pts',(-60.722063855041,36.3018464434213,0.));
#150595=CARTESIAN_POINT('Ctrl Pts',(-60.7077258593268,36.2860149033587,
0.));
#150596=CARTESIAN_POINT('Ctrl Pts',(-60.6934044626291,36.2702345632875,
0.));
#150597=CARTESIAN_POINT('Ctrl Pts',(-60.67909982978,36.2545054892897,0.));
#150598=CARTESIAN_POINT('Ctrl Pts',(-60.6648121265885,36.2388277477212,
0.));
#150599=CARTESIAN_POINT('Ctrl Pts',(-60.6505415197042,36.2232014051541,
0.));
#150600=CARTESIAN_POINT('Ctrl Pts',(-60.6362881765019,36.2076265283264,
0.));
#150601=CARTESIAN_POINT('Ctrl Pts',(-60.6220522649149,36.192103184063,0.));
#150602=CARTESIAN_POINT('Ctrl Pts',(-60.6078339534181,36.1766314392641,
0.));
#150603=CARTESIAN_POINT('Ctrl Pts',(-60.5936334114108,36.1612113610773,
0.));
#150604=CARTESIAN_POINT('Ctrl Pts',(-60.5794508095565,36.1458430170431,
0.));
#150605=CARTESIAN_POINT('Ctrl Pts',(-60.565286320072,36.1305264752188,0.));
#150606=CARTESIAN_POINT('Ctrl Pts',(-60.5511401171984,36.1152618043739,
0.));
#150607=CARTESIAN_POINT('Ctrl Pts',(-60.5370123768804,36.100049073851,0.));
#150608=CARTESIAN_POINT('Ctrl Pts',(-60.5229032758974,36.0848883531952,
0.));
#150609=CARTESIAN_POINT('Ctrl Pts',(-60.5088129911354,36.0697797118376,
0.));
#150610=CARTESIAN_POINT('Ctrl Pts',(-60.4947416988422,36.0547232187698,
0.));
#150611=CARTESIAN_POINT('Ctrl Pts',(-60.4806895737686,36.0397189421644,
0.));
#150612=CARTESIAN_POINT('Ctrl Pts',(-60.4666567908093,36.0247669500891,
0.));
#150613=CARTESIAN_POINT('Ctrl Pts',(-60.4526435269662,36.009867311357,0.));
#150614=CARTESIAN_POINT('Ctrl Pts',(-60.4386499629481,35.995020096217,0.));
#150615=CARTESIAN_POINT('Ctrl Pts',(-60.4246762854926,35.9802253773515,
0.));
#150616=CARTESIAN_POINT('Ctrl Pts',(-60.4107226875714,35.9654832299601,
0.));
#150617=CARTESIAN_POINT('Ctrl Pts',(-60.3967893635452,35.9507937296707,
0.));
#150618=CARTESIAN_POINT('Ctrl Pts',(-60.3828765049019,35.936156950695,0.));
#150619=CARTESIAN_POINT('Ctrl Pts',(-60.3689842965481,35.9215729642231,
0.));
#150620=CARTESIAN_POINT('Ctrl Pts',(-60.3551129108845,35.907041835853,0.));
#150621=CARTESIAN_POINT('Ctrl Pts',(-60.3412625135287,35.8925636280668,
0.));
#150622=CARTESIAN_POINT('Ctrl Pts',(-60.327433274683,35.8781384051537,0.));
#150623=CARTESIAN_POINT('Ctrl Pts',(-60.313625378281,35.8637662371635,0.));
#150624=CARTESIAN_POINT('Ctrl Pts',(-60.2998390330102,35.8494472046745,
0.));
#150625=CARTESIAN_POINT('Ctrl Pts',(-60.2860744798436,35.8351814020357,
0.));
#150626=CARTESIAN_POINT('Ctrl Pts',(-60.2723319687369,35.8209689272501,
0.));
#150627=CARTESIAN_POINT('Ctrl Pts',(-60.2586117365205,35.8068098723347,
0.));
#150628=CARTESIAN_POINT('Ctrl Pts',(-60.2449139865275,35.7927043145201,
0.));
#150629=CARTESIAN_POINT('Ctrl Pts',(-60.2312388621529,35.7786523045912,
0.));
#150630=CARTESIAN_POINT('Ctrl Pts',(-60.2175864450043,35.7646538667493,
0.));
#150631=CARTESIAN_POINT('Ctrl Pts',(-60.206682708692,35.7534979802053,0.));
#150632=CARTESIAN_POINT('Ctrl Pts',(-60.1985151474623,35.7451551752572,
0.));
#150633=CARTESIAN_POINT('Ctrl Pts',(-60.193074658032,35.7396040204017,0.));
#150634=CARTESIAN_POINT('Ctrl Pts',(-60.1903555511633,35.736831121751,0.));
#150635=CARTESIAN_POINT('Ctrl Pts',(-59.483083043136,44.8554660179045,0.));
#150636=CARTESIAN_POINT('Ctrl Pts',(-59.483083043136,44.8554660179045,12.));
#150637=CARTESIAN_POINT('Ctrl Pts',(-59.4804358983083,44.8505359826461,
0.));
#150638=CARTESIAN_POINT('Ctrl Pts',(-59.4804358983083,44.8505359826461,
12.));
#150639=CARTESIAN_POINT('Ctrl Pts',(-59.4751410547732,44.8406801497742,
0.));
#150640=CARTESIAN_POINT('Ctrl Pts',(-59.4751410547732,44.8406801497742,
12.));
#150641=CARTESIAN_POINT('Ctrl Pts',(-59.4671971278321,44.8259091134016,
0.));
#150642=CARTESIAN_POINT('Ctrl Pts',(-59.4671971278321,44.8259091134016,
12.));
#150643=CARTESIAN_POINT('Ctrl Pts',(-59.4566019018254,44.8062398251406,
0.));
#150644=CARTESIAN_POINT('Ctrl Pts',(-59.4566019018254,44.8062398251406,
12.));
#150645=CARTESIAN_POINT('Ctrl Pts',(-59.4433523335147,44.7816956017528,
0.));
#150646=CARTESIAN_POINT('Ctrl Pts',(-59.4433523335147,44.7816956017528,
12.));
#150647=CARTESIAN_POINT('Ctrl Pts',(-59.430097240324,44.7571937812113,0.));
#150648=CARTESIAN_POINT('Ctrl Pts',(-59.430097240324,44.7571937812113,12.));
#150649=CARTESIAN_POINT('Ctrl Pts',(-59.4168366453118,44.7327343876391,
0.));
#150650=CARTESIAN_POINT('Ctrl Pts',(-59.4168366453118,44.7327343876391,
12.));
#150651=CARTESIAN_POINT('Ctrl Pts',(-59.4035705873811,44.7083174541702,
0.));
#150652=CARTESIAN_POINT('Ctrl Pts',(-59.4035705873811,44.7083174541702,
12.));
#150653=CARTESIAN_POINT('Ctrl Pts',(-59.3902991267889,44.683943024421,0.));
#150654=CARTESIAN_POINT('Ctrl Pts',(-59.3902991267889,44.683943024421,12.));
#150655=CARTESIAN_POINT('Ctrl Pts',(-59.377022343519,44.6596111512687,0.));
#150656=CARTESIAN_POINT('Ctrl Pts',(-59.377022343519,44.6596111512687,12.));
#150657=CARTESIAN_POINT('Ctrl Pts',(-59.3637403301801,44.6353218935685,
0.));
#150658=CARTESIAN_POINT('Ctrl Pts',(-59.3637403301801,44.6353218935685,
12.));
#150659=CARTESIAN_POINT('Ctrl Pts',(-59.3504531864154,44.6110753134277,
0.));
#150660=CARTESIAN_POINT('Ctrl Pts',(-59.3504531864154,44.6110753134277,
12.));
#150661=CARTESIAN_POINT('Ctrl Pts',(-59.3371610128511,44.5868714733234,
0.));
#150662=CARTESIAN_POINT('Ctrl Pts',(-59.3371610128511,44.5868714733234,
12.));
#150663=CARTESIAN_POINT('Ctrl Pts',(-59.3238639048694,44.5627104331017,
0.));
#150664=CARTESIAN_POINT('Ctrl Pts',(-59.3238639048694,44.5627104331017,
12.));
#150665=CARTESIAN_POINT('Ctrl Pts',(-59.3105619475609,44.5385922475573,
0.));
#150666=CARTESIAN_POINT('Ctrl Pts',(-59.3105619475609,44.5385922475573,
12.));
#150667=CARTESIAN_POINT('Ctrl Pts',(-59.2972552192156,44.5145169681349,
0.));
#150668=CARTESIAN_POINT('Ctrl Pts',(-59.2972552192156,44.5145169681349,
12.));
#150669=CARTESIAN_POINT('Ctrl Pts',(-59.2839437938237,44.490484644151,0.));
#150670=CARTESIAN_POINT('Ctrl Pts',(-59.2839437938237,44.490484644151,12.));
#150671=CARTESIAN_POINT('Ctrl Pts',(-59.2706277440445,44.4664953242379,
0.));
#150672=CARTESIAN_POINT('Ctrl Pts',(-59.2706277440445,44.4664953242379,
12.));
#150673=CARTESIAN_POINT('Ctrl Pts',(-59.2573071437774,44.4425490575911,
0.));
#150674=CARTESIAN_POINT('Ctrl Pts',(-59.2573071437774,44.4425490575911,
12.));
#150675=CARTESIAN_POINT('Ctrl Pts',(-59.2439820714187,44.4186458955451,
0.));
#150676=CARTESIAN_POINT('Ctrl Pts',(-59.2439820714187,44.4186458955451,
12.));
#150677=CARTESIAN_POINT('Ctrl Pts',(-59.2306526095131,44.3947858914074,
0.));
#150678=CARTESIAN_POINT('Ctrl Pts',(-59.2306526095131,44.3947858914074,
12.));
#150679=CARTESIAN_POINT('Ctrl Pts',(-59.2173188432798,44.3709690997469,
0.));
#150680=CARTESIAN_POINT('Ctrl Pts',(-59.2173188432798,44.3709690997469,
12.));
#150681=CARTESIAN_POINT('Ctrl Pts',(-59.2039808594752,44.3471955758403,
0.));
#150682=CARTESIAN_POINT('Ctrl Pts',(-59.2039808594752,44.3471955758403,
12.));
#150683=CARTESIAN_POINT('Ctrl Pts',(-59.1906387451979,44.3234653750884,
0.));
#150684=CARTESIAN_POINT('Ctrl Pts',(-59.1906387451979,44.3234653750884,
12.));
#150685=CARTESIAN_POINT('Ctrl Pts',(-59.1772925865213,44.2997785523431,
0.));
#150686=CARTESIAN_POINT('Ctrl Pts',(-59.1772925865213,44.2997785523431,
12.));
#150687=CARTESIAN_POINT('Ctrl Pts',(-59.1639424678793,44.2761351616048,
0.));
#150688=CARTESIAN_POINT('Ctrl Pts',(-59.1639424678793,44.2761351616048,
12.));
#150689=CARTESIAN_POINT('Ctrl Pts',(-59.1505884728215,44.2525352563996,
0.));
#150690=CARTESIAN_POINT('Ctrl Pts',(-59.1505884728215,44.2525352563996,
12.));
#150691=CARTESIAN_POINT('Ctrl Pts',(-59.1372306844586,44.228978889997,0.));
#150692=CARTESIAN_POINT('Ctrl Pts',(-59.1372306844586,44.228978889997,12.));
#150693=CARTESIAN_POINT('Ctrl Pts',(-59.1238691860306,44.2054661156875,
0.));
#150694=CARTESIAN_POINT('Ctrl Pts',(-59.1238691860306,44.2054661156875,
12.));
#150695=CARTESIAN_POINT('Ctrl Pts',(-59.1105040614276,44.1819969870307,
0.));
#150696=CARTESIAN_POINT('Ctrl Pts',(-59.1105040614276,44.1819969870307,
12.));
#150697=CARTESIAN_POINT('Ctrl Pts',(-59.0971353957206,44.1585715581064,
0.));
#150698=CARTESIAN_POINT('Ctrl Pts',(-59.0971353957206,44.1585715581064,
12.));
#150699=CARTESIAN_POINT('Ctrl Pts',(-59.08376327492,44.1351898834051,0.));
#150700=CARTESIAN_POINT('Ctrl Pts',(-59.08376327492,44.1351898834051,12.));
#150701=CARTESIAN_POINT('Ctrl Pts',(-59.0703877857526,44.1118520177221,
0.));
#150702=CARTESIAN_POINT('Ctrl Pts',(-59.0703877857526,44.1118520177221,
12.));
#150703=CARTESIAN_POINT('Ctrl Pts',(-59.0570090154243,44.0885580160432,
0.));
#150704=CARTESIAN_POINT('Ctrl Pts',(-59.0570090154243,44.0885580160432,
12.));
#150705=CARTESIAN_POINT('Ctrl Pts',(-59.0436270514087,44.0653079334385,
0.));
#150706=CARTESIAN_POINT('Ctrl Pts',(-59.0436270514087,44.0653079334385,
12.));
#150707=CARTESIAN_POINT('Ctrl Pts',(-59.0302419811777,44.0421018249223,
0.));
#150708=CARTESIAN_POINT('Ctrl Pts',(-59.0302419811777,44.0421018249223,
12.));
#150709=CARTESIAN_POINT('Ctrl Pts',(-59.0168538922095,44.0189397454599,
0.));
#150710=CARTESIAN_POINT('Ctrl Pts',(-59.0168538922095,44.0189397454599,
12.));
#150711=CARTESIAN_POINT('Ctrl Pts',(-59.0034628721168,43.9958217500369,
0.));
#150712=CARTESIAN_POINT('Ctrl Pts',(-59.0034628721168,43.9958217500369,
12.));
#150713=CARTESIAN_POINT('Ctrl Pts',(-58.9900690087408,43.9727478937056,
0.));
#150714=CARTESIAN_POINT('Ctrl Pts',(-58.9900690087408,43.9727478937056,
12.));
#150715=CARTESIAN_POINT('Ctrl Pts',(-58.9766723902529,43.9497182316331,
0.));
#150716=CARTESIAN_POINT('Ctrl Pts',(-58.9766723902529,43.9497182316331,
12.));
#150717=CARTESIAN_POINT('Ctrl Pts',(-58.9632731052696,43.9267328191501,
0.));
#150718=CARTESIAN_POINT('Ctrl Pts',(-58.9632731052696,43.9267328191501,
12.));
#150719=CARTESIAN_POINT('Ctrl Pts',(-58.9498712429054,43.9037917117739,
0.));
#150720=CARTESIAN_POINT('Ctrl Pts',(-58.9498712429054,43.9037917117739,
12.));
#150721=CARTESIAN_POINT('Ctrl Pts',(-58.936466892712,43.8808949651873,0.));
#150722=CARTESIAN_POINT('Ctrl Pts',(-58.936466892712,43.8808949651873,12.));
#150723=CARTESIAN_POINT('Ctrl Pts',(-58.9230601446436,43.858042635223,0.));
#150724=CARTESIAN_POINT('Ctrl Pts',(-58.9230601446436,43.858042635223,12.));
#150725=CARTESIAN_POINT('Ctrl Pts',(-58.9096510890129,43.835234777842,0.));
#150726=CARTESIAN_POINT('Ctrl Pts',(-58.9096510890129,43.835234777842,12.));
#150727=CARTESIAN_POINT('Ctrl Pts',(-58.8962398164493,43.8124714491076,
0.));
#150728=CARTESIAN_POINT('Ctrl Pts',(-58.8962398164493,43.8124714491076,
12.));
#150729=CARTESIAN_POINT('Ctrl Pts',(-58.8828264178621,43.7897527051609,
0.));
#150730=CARTESIAN_POINT('Ctrl Pts',(-58.8828264178621,43.7897527051609,
12.));
#150731=CARTESIAN_POINT('Ctrl Pts',(-58.8694109844648,43.7670786022402,
0.));
#150732=CARTESIAN_POINT('Ctrl Pts',(-58.8694109844648,43.7670786022402,
12.));
#150733=CARTESIAN_POINT('Ctrl Pts',(-58.855993607794,43.7444491966942,0.));
#150734=CARTESIAN_POINT('Ctrl Pts',(-58.855993607794,43.7444491966942,12.));
#150735=CARTESIAN_POINT('Ctrl Pts',(-58.8425743797326,43.7218645449922,
0.));
#150736=CARTESIAN_POINT('Ctrl Pts',(-58.8425743797326,43.7218645449922,
12.));
#150737=CARTESIAN_POINT('Ctrl Pts',(-58.8291533925293,43.6993247037314,
0.));
#150738=CARTESIAN_POINT('Ctrl Pts',(-58.8291533925293,43.6993247037314,
12.));
#150739=CARTESIAN_POINT('Ctrl Pts',(-58.8157307388238,43.6768297296395,
0.));
#150740=CARTESIAN_POINT('Ctrl Pts',(-58.8157307388238,43.6768297296395,
12.));
#150741=CARTESIAN_POINT('Ctrl Pts',(-58.8023065116436,43.6543796795789,
0.));
#150742=CARTESIAN_POINT('Ctrl Pts',(-58.8023065116436,43.6543796795789,
12.));
#150743=CARTESIAN_POINT('Ctrl Pts',(-58.788880804397,43.6319746105482,0.));
#150744=CARTESIAN_POINT('Ctrl Pts',(-58.788880804397,43.6319746105482,12.));
#150745=CARTESIAN_POINT('Ctrl Pts',(-58.775453710867,43.6096145796797,0.));
#150746=CARTESIAN_POINT('Ctrl Pts',(-58.775453710867,43.6096145796797,12.));
#150747=CARTESIAN_POINT('Ctrl Pts',(-58.7620253252062,43.5872996442345,
0.));
#150748=CARTESIAN_POINT('Ctrl Pts',(-58.7620253252062,43.5872996442345,
12.));
#150749=CARTESIAN_POINT('Ctrl Pts',(-58.74859574193,43.5650298615917,0.));
#150750=CARTESIAN_POINT('Ctrl Pts',(-58.74859574193,43.5650298615917,12.));
#150751=CARTESIAN_POINT('Ctrl Pts',(-58.735165055918,43.5428052892488,0.));
#150752=CARTESIAN_POINT('Ctrl Pts',(-58.735165055918,43.5428052892488,12.));
#150753=CARTESIAN_POINT('Ctrl Pts',(-58.7217333624209,43.5206259848337,
0.));
#150754=CARTESIAN_POINT('Ctrl Pts',(-58.7217333624209,43.5206259848337,
12.));
#150755=CARTESIAN_POINT('Ctrl Pts',(-58.7083007570661,43.4984920061073,
0.));
#150756=CARTESIAN_POINT('Ctrl Pts',(-58.7083007570661,43.4984920061073,
12.));
#150757=CARTESIAN_POINT('Ctrl Pts',(-58.6948673358638,43.4764034109654,
0.));
#150758=CARTESIAN_POINT('Ctrl Pts',(-58.6948673358638,43.4764034109654,
12.));
#150759=CARTESIAN_POINT('Ctrl Pts',(-58.6814331952138,43.4543602574351,
0.));
#150760=CARTESIAN_POINT('Ctrl Pts',(-58.6814331952138,43.4543602574351,
12.));
#150761=CARTESIAN_POINT('Ctrl Pts',(-58.6679984319097,43.4323626036737,
0.));
#150762=CARTESIAN_POINT('Ctrl Pts',(-58.6679984319097,43.4323626036737,
12.));
#150763=CARTESIAN_POINT('Ctrl Pts',(-58.6545631431393,43.4104105079768,
0.));
#150764=CARTESIAN_POINT('Ctrl Pts',(-58.6545631431393,43.4104105079768,
12.));
#150765=CARTESIAN_POINT('Ctrl Pts',(-58.6411274264857,43.388504028781,0.));
#150766=CARTESIAN_POINT('Ctrl Pts',(-58.6411274264857,43.388504028781,12.));
#150767=CARTESIAN_POINT('Ctrl Pts',(-58.627691379929,43.3666432246635,0.));
#150768=CARTESIAN_POINT('Ctrl Pts',(-58.627691379929,43.3666432246635,12.));
#150769=CARTESIAN_POINT('Ctrl Pts',(-58.6142551018467,43.3448281543371,
0.));
#150770=CARTESIAN_POINT('Ctrl Pts',(-58.6142551018467,43.3448281543371,
12.));
#150771=CARTESIAN_POINT('Ctrl Pts',(-58.6008186910156,43.3230588766449,
0.));
#150772=CARTESIAN_POINT('Ctrl Pts',(-58.6008186910156,43.3230588766449,
12.));
#150773=CARTESIAN_POINT('Ctrl Pts',(-58.5873822466152,43.3013354505701,
0.));
#150774=CARTESIAN_POINT('Ctrl Pts',(-58.5873822466152,43.3013354505701,
12.));
#150775=CARTESIAN_POINT('Ctrl Pts',(-58.573945868231,43.27965793524,0.));
#150776=CARTESIAN_POINT('Ctrl Pts',(-58.573945868231,43.27965793524,12.));
#150777=CARTESIAN_POINT('Ctrl Pts',(-58.5605096558578,43.2580263899278,
0.));
#150778=CARTESIAN_POINT('Ctrl Pts',(-58.5605096558578,43.2580263899278,
12.));
#150779=CARTESIAN_POINT('Ctrl Pts',(-58.5470737099032,43.2364408740493,
0.));
#150780=CARTESIAN_POINT('Ctrl Pts',(-58.5470737099032,43.2364408740493,
12.));
#150781=CARTESIAN_POINT('Ctrl Pts',(-58.5336381311917,43.2149014471574,
0.));
#150782=CARTESIAN_POINT('Ctrl Pts',(-58.5336381311917,43.2149014471574,
12.));
#150783=CARTESIAN_POINT('Ctrl Pts',(-58.5202030209669,43.1934081689505,
0.));
#150784=CARTESIAN_POINT('Ctrl Pts',(-58.5202030209669,43.1934081689505,
12.));
#150785=CARTESIAN_POINT('Ctrl Pts',(-58.5067684808944,43.1719610992771,
0.));
#150786=CARTESIAN_POINT('Ctrl Pts',(-58.5067684808944,43.1719610992771,
12.));
#150787=CARTESIAN_POINT('Ctrl Pts',(-58.4933346130636,43.1505602981365,
0.));
#150788=CARTESIAN_POINT('Ctrl Pts',(-58.4933346130636,43.1505602981365,
12.));
#150789=CARTESIAN_POINT('Ctrl Pts',(-58.4799015199907,43.1292058256777,
0.));
#150790=CARTESIAN_POINT('Ctrl Pts',(-58.4799015199907,43.1292058256777,
12.));
#150791=CARTESIAN_POINT('Ctrl Pts',(-58.4664693046217,43.1078977421916,
0.));
#150792=CARTESIAN_POINT('Ctrl Pts',(-58.4664693046217,43.1078977421916,
12.));
#150793=CARTESIAN_POINT('Ctrl Pts',(-58.4530380703348,43.0866361081177,
0.));
#150794=CARTESIAN_POINT('Ctrl Pts',(-58.4530380703348,43.0866361081177,
12.));
#150795=CARTESIAN_POINT('Ctrl Pts',(-58.439607920945,43.0654209840511,0.));
#150796=CARTESIAN_POINT('Ctrl Pts',(-58.439607920945,43.0654209840511,12.));
#150797=CARTESIAN_POINT('Ctrl Pts',(-58.4261789607058,43.0442524307434,
0.));
#150798=CARTESIAN_POINT('Ctrl Pts',(-58.4261789607058,43.0442524307434,
12.));
#150799=CARTESIAN_POINT('Ctrl Pts',(-58.4127512943136,43.0231305091027,
0.));
#150800=CARTESIAN_POINT('Ctrl Pts',(-58.4127512943136,43.0231305091027,
12.));
#150801=CARTESIAN_POINT('Ctrl Pts',(-58.3993250269101,43.0020552801859,
0.));
#150802=CARTESIAN_POINT('Ctrl Pts',(-58.3993250269101,43.0020552801859,
12.));
#150803=CARTESIAN_POINT('Ctrl Pts',(-58.3859002640856,42.9810268052032,
0.));
#150804=CARTESIAN_POINT('Ctrl Pts',(-58.3859002640856,42.9810268052032,
12.));
#150805=CARTESIAN_POINT('Ctrl Pts',(-58.3724771118826,42.960045145526,0.));
#150806=CARTESIAN_POINT('Ctrl Pts',(-58.3724771118826,42.960045145526,12.));
#150807=CARTESIAN_POINT('Ctrl Pts',(-58.3590556767978,42.9391103626879,
0.));
#150808=CARTESIAN_POINT('Ctrl Pts',(-58.3590556767978,42.9391103626879,
12.));
#150809=CARTESIAN_POINT('Ctrl Pts',(-58.3456360657865,42.9182225183855,
0.));
#150810=CARTESIAN_POINT('Ctrl Pts',(-58.3456360657865,42.9182225183855,
12.));
#150811=CARTESIAN_POINT('Ctrl Pts',(-58.3322183862654,42.8973816744709,
0.));
#150812=CARTESIAN_POINT('Ctrl Pts',(-58.3322183862654,42.8973816744709,
12.));
#150813=CARTESIAN_POINT('Ctrl Pts',(-58.3188027461164,42.8765878929551,
0.));
#150814=CARTESIAN_POINT('Ctrl Pts',(-58.3188027461164,42.8765878929551,
12.));
#150815=CARTESIAN_POINT('Ctrl Pts',(-58.3053892536894,42.8558412360158,
0.));
#150816=CARTESIAN_POINT('Ctrl Pts',(-58.3053892536894,42.8558412360158,
12.));
#150817=CARTESIAN_POINT('Ctrl Pts',(-58.2919780178064,42.8351417659999,
0.));
#150818=CARTESIAN_POINT('Ctrl Pts',(-58.2919780178064,42.8351417659999,
12.));
#150819=CARTESIAN_POINT('Ctrl Pts',(-58.2785691477638,42.8144895454233,
0.));
#150820=CARTESIAN_POINT('Ctrl Pts',(-58.2785691477638,42.8144895454233,
12.));
#150821=CARTESIAN_POINT('Ctrl Pts',(-58.2651627533368,42.7938846369651,
0.));
#150822=CARTESIAN_POINT('Ctrl Pts',(-58.2651627533368,42.7938846369651,
12.));
#150823=CARTESIAN_POINT('Ctrl Pts',(-58.251758944782,42.7733271034679,0.));
#150824=CARTESIAN_POINT('Ctrl Pts',(-58.251758944782,42.7733271034679,12.));
#150825=CARTESIAN_POINT('Ctrl Pts',(-58.2383578328424,42.7528170079484,
0.));
#150826=CARTESIAN_POINT('Ctrl Pts',(-58.2383578328424,42.7528170079484,
12.));
#150827=CARTESIAN_POINT('Ctrl Pts',(-58.22495952875,42.7323544135985,0.));
#150828=CARTESIAN_POINT('Ctrl Pts',(-58.22495952875,42.7323544135985,12.));
#150829=CARTESIAN_POINT('Ctrl Pts',(-58.21156414423,42.7119393837866,0.));
#150830=CARTESIAN_POINT('Ctrl Pts',(-58.21156414423,42.7119393837866,12.));
#150831=CARTESIAN_POINT('Ctrl Pts',(-58.1981717915037,42.6915719820513,
0.));
#150832=CARTESIAN_POINT('Ctrl Pts',(-58.1981717915037,42.6915719820513,
12.));
#150833=CARTESIAN_POINT('Ctrl Pts',(-58.1847825832923,42.6712522721016,
0.));
#150834=CARTESIAN_POINT('Ctrl Pts',(-58.1847825832923,42.6712522721016,
12.));
#150835=CARTESIAN_POINT('Ctrl Pts',(-58.171396632821,42.6509803178265,0.));
#150836=CARTESIAN_POINT('Ctrl Pts',(-58.171396632821,42.6509803178265,12.));
#150837=CARTESIAN_POINT('Ctrl Pts',(-58.1580140538228,42.6307561832976,
0.));
#150838=CARTESIAN_POINT('Ctrl Pts',(-58.1580140538228,42.6307561832976,
12.));
#150839=CARTESIAN_POINT('Ctrl Pts',(-58.1446349605421,42.6105799327699,
0.));
#150840=CARTESIAN_POINT('Ctrl Pts',(-58.1446349605421,42.6105799327699,
12.));
#150841=CARTESIAN_POINT('Ctrl Pts',(-58.1312594677386,42.5904516306762,
0.));
#150842=CARTESIAN_POINT('Ctrl Pts',(-58.1312594677386,42.5904516306762,
12.));
#150843=CARTESIAN_POINT('Ctrl Pts',(-58.1178876906907,42.5703713416265,
0.));
#150844=CARTESIAN_POINT('Ctrl Pts',(-58.1178876906907,42.5703713416265,
12.));
#150845=CARTESIAN_POINT('Ctrl Pts',(-58.1045197452002,42.5503391304183,
0.));
#150846=CARTESIAN_POINT('Ctrl Pts',(-58.1045197452002,42.5503391304183,
12.));
#150847=CARTESIAN_POINT('Ctrl Pts',(-58.0911557475965,42.5303550620387,
0.));
#150848=CARTESIAN_POINT('Ctrl Pts',(-58.0911557475965,42.5303550620387,
12.));
#150849=CARTESIAN_POINT('Ctrl Pts',(-58.0777958147403,42.5104192016664,
0.));
#150850=CARTESIAN_POINT('Ctrl Pts',(-58.0777958147403,42.5104192016664,
12.));
#150851=CARTESIAN_POINT('Ctrl Pts',(-58.0644400640275,42.4905316146653,
0.));
#150852=CARTESIAN_POINT('Ctrl Pts',(-58.0644400640275,42.4905316146653,
12.));
#150853=CARTESIAN_POINT('Ctrl Pts',(-58.0510886133926,42.4706923665845,
0.));
#150854=CARTESIAN_POINT('Ctrl Pts',(-58.0510886133926,42.4706923665845,
12.));
#150855=CARTESIAN_POINT('Ctrl Pts',(-58.037741581314,42.4509015231674,0.));
#150856=CARTESIAN_POINT('Ctrl Pts',(-58.037741581314,42.4509015231674,12.));
#150857=CARTESIAN_POINT('Ctrl Pts',(-58.0243990868181,42.4311591503555,
0.));
#150858=CARTESIAN_POINT('Ctrl Pts',(-58.0243990868181,42.4311591503555,
12.));
#150859=CARTESIAN_POINT('Ctrl Pts',(-58.0110612494828,42.411465314289,0.));
#150860=CARTESIAN_POINT('Ctrl Pts',(-58.0110612494828,42.411465314289,12.));
#150861=CARTESIAN_POINT('Ctrl Pts',(-57.9977281894422,42.3918200813014,
0.));
#150862=CARTESIAN_POINT('Ctrl Pts',(-57.9977281894422,42.3918200813014,
12.));
#150863=CARTESIAN_POINT('Ctrl Pts',(-57.9844000273911,42.3722235179197,
0.));
#150864=CARTESIAN_POINT('Ctrl Pts',(-57.9844000273911,42.3722235179197,
12.));
#150865=CARTESIAN_POINT('Ctrl Pts',(-57.9710768845899,42.3526756908746,
0.));
#150866=CARTESIAN_POINT('Ctrl Pts',(-57.9710768845899,42.3526756908746,
12.));
#150867=CARTESIAN_POINT('Ctrl Pts',(-57.9577588828682,42.333176667102,0.));
#150868=CARTESIAN_POINT('Ctrl Pts',(-57.9577588828682,42.333176667102,12.));
#150869=CARTESIAN_POINT('Ctrl Pts',(-57.9444461446299,42.3137265137452,
0.));
#150870=CARTESIAN_POINT('Ctrl Pts',(-57.9444461446299,42.3137265137452,
12.));
#150871=CARTESIAN_POINT('Ctrl Pts',(-57.9311387928563,42.2943252981489,
0.));
#150872=CARTESIAN_POINT('Ctrl Pts',(-57.9311387928563,42.2943252981489,
12.));
#150873=CARTESIAN_POINT('Ctrl Pts',(-57.9178369511114,42.2749730878594,
0.));
#150874=CARTESIAN_POINT('Ctrl Pts',(-57.9178369511114,42.2749730878594,
12.));
#150875=CARTESIAN_POINT('Ctrl Pts',(-57.9045407435474,42.2556699506353,
0.));
#150876=CARTESIAN_POINT('Ctrl Pts',(-57.9045407435474,42.2556699506353,
12.));
#150877=CARTESIAN_POINT('Ctrl Pts',(-57.8912502949096,42.2364159544501,
0.));
#150878=CARTESIAN_POINT('Ctrl Pts',(-57.8912502949096,42.2364159544501,
12.));
#150879=CARTESIAN_POINT('Ctrl Pts',(-57.8779657305413,42.2172111674938,
0.));
#150880=CARTESIAN_POINT('Ctrl Pts',(-57.8779657305413,42.2172111674938,
12.));
#150881=CARTESIAN_POINT('Ctrl Pts',(-57.864687176387,42.1980556581665,0.));
#150882=CARTESIAN_POINT('Ctrl Pts',(-57.864687176387,42.1980556581665,12.));
#150883=CARTESIAN_POINT('Ctrl Pts',(-57.8514147589972,42.1789494950794,
0.));
#150884=CARTESIAN_POINT('Ctrl Pts',(-57.8514147589972,42.1789494950794,
12.));
#150885=CARTESIAN_POINT('Ctrl Pts',(-57.8381486055342,42.1598927470646,
0.));
#150886=CARTESIAN_POINT('Ctrl Pts',(-57.8381486055342,42.1598927470646,
12.));
#150887=CARTESIAN_POINT('Ctrl Pts',(-57.8248888437775,42.1408854831783,
0.));
#150888=CARTESIAN_POINT('Ctrl Pts',(-57.8248888437775,42.1408854831783,
12.));
#150889=CARTESIAN_POINT('Ctrl Pts',(-57.8116356021288,42.1219277727021,
0.));
#150890=CARTESIAN_POINT('Ctrl Pts',(-57.8116356021288,42.1219277727021,
12.));
#150891=CARTESIAN_POINT('Ctrl Pts',(-57.798389009616,42.1030196851366,0.));
#150892=CARTESIAN_POINT('Ctrl Pts',(-57.798389009616,42.1030196851366,12.));
#150893=CARTESIAN_POINT('Ctrl Pts',(-57.7851491958987,42.0841612902042,
0.));
#150894=CARTESIAN_POINT('Ctrl Pts',(-57.7851491958987,42.0841612902042,
12.));
#150895=CARTESIAN_POINT('Ctrl Pts',(-57.7719162912744,42.0653526578588,
0.));
#150896=CARTESIAN_POINT('Ctrl Pts',(-57.7719162912744,42.0653526578588,
12.));
#150897=CARTESIAN_POINT('Ctrl Pts',(-57.7586904266834,42.0465938582882,
0.));
#150898=CARTESIAN_POINT('Ctrl Pts',(-57.7586904266834,42.0465938582882,
12.));
#150899=CARTESIAN_POINT('Ctrl Pts',(-57.745471733714,42.0278849619148,0.));
#150900=CARTESIAN_POINT('Ctrl Pts',(-57.745471733714,42.0278849619148,12.));
#150901=CARTESIAN_POINT('Ctrl Pts',(-57.7322603446066,42.0092260393897,
0.));
#150902=CARTESIAN_POINT('Ctrl Pts',(-57.7322603446066,42.0092260393897,
12.));
#150903=CARTESIAN_POINT('Ctrl Pts',(-57.7190563922593,41.990617161596,0.));
#150904=CARTESIAN_POINT('Ctrl Pts',(-57.7190563922593,41.990617161596,12.));
#150905=CARTESIAN_POINT('Ctrl Pts',(-57.7058600102351,41.9720583996592,
0.));
#150906=CARTESIAN_POINT('Ctrl Pts',(-57.7058600102351,41.9720583996592,
12.));
#150907=CARTESIAN_POINT('Ctrl Pts',(-57.6926713327672,41.9535498249488,
0.));
#150908=CARTESIAN_POINT('Ctrl Pts',(-57.6926713327672,41.9535498249488,
12.));
#150909=CARTESIAN_POINT('Ctrl Pts',(-57.6794904947649,41.9350915090796,
0.));
#150910=CARTESIAN_POINT('Ctrl Pts',(-57.6794904947649,41.9350915090796,
12.));
#150911=CARTESIAN_POINT('Ctrl Pts',(-57.6663176318189,41.9166835239054,
0.));
#150912=CARTESIAN_POINT('Ctrl Pts',(-57.6663176318189,41.9166835239054,
12.));
#150913=CARTESIAN_POINT('Ctrl Pts',(-57.6531528802072,41.8983259415253,
0.));
#150914=CARTESIAN_POINT('Ctrl Pts',(-57.6531528802072,41.8983259415253,
12.));
#150915=CARTESIAN_POINT('Ctrl Pts',(-57.6399963769009,41.8800188342912,
0.));
#150916=CARTESIAN_POINT('Ctrl Pts',(-57.6399963769009,41.8800188342912,
12.));
#150917=CARTESIAN_POINT('Ctrl Pts',(-57.6268482595701,41.8617622748107,
0.));
#150918=CARTESIAN_POINT('Ctrl Pts',(-57.6268482595701,41.8617622748107,
12.));
#150919=CARTESIAN_POINT('Ctrl Pts',(-57.613708666588,41.8435563359456,0.));
#150920=CARTESIAN_POINT('Ctrl Pts',(-57.613708666588,41.8435563359456,12.));
#150921=CARTESIAN_POINT('Ctrl Pts',(-57.6005777370347,41.8254010908051,
0.));
#150922=CARTESIAN_POINT('Ctrl Pts',(-57.6005777370347,41.8254010908051,
12.));
#150923=CARTESIAN_POINT('Ctrl Pts',(-57.5874556107054,41.8072966127559,
0.));
#150924=CARTESIAN_POINT('Ctrl Pts',(-57.5874556107054,41.8072966127559,
12.));
#150925=CARTESIAN_POINT('Ctrl Pts',(-57.5743424281204,41.7892429754298,
0.));
#150926=CARTESIAN_POINT('Ctrl Pts',(-57.5743424281204,41.7892429754298,
12.));
#150927=CARTESIAN_POINT('Ctrl Pts',(-57.561238330532,41.7712402527273,0.));
#150928=CARTESIAN_POINT('Ctrl Pts',(-57.561238330532,41.7712402527273,12.));
#150929=CARTESIAN_POINT('Ctrl Pts',(-57.5481434599334,41.7532885188174,
0.));
#150930=CARTESIAN_POINT('Ctrl Pts',(-57.5481434599334,41.7532885188174,
12.));
#150931=CARTESIAN_POINT('Ctrl Pts',(-57.5350579590648,41.7353878481336,
0.));
#150932=CARTESIAN_POINT('Ctrl Pts',(-57.5350579590648,41.7353878481336,
12.));
#150933=CARTESIAN_POINT('Ctrl Pts',(-57.5219819714169,41.7175383153819,
0.));
#150934=CARTESIAN_POINT('Ctrl Pts',(-57.5219819714169,41.7175383153819,
12.));
#150935=CARTESIAN_POINT('Ctrl Pts',(-57.5089156412341,41.6997399955445,
0.));
#150936=CARTESIAN_POINT('Ctrl Pts',(-57.5089156412341,41.6997399955445,
12.));
#150937=CARTESIAN_POINT('Ctrl Pts',(-57.4958591135165,41.6819929638797,
0.));
#150938=CARTESIAN_POINT('Ctrl Pts',(-57.4958591135165,41.6819929638797,
12.));
#150939=CARTESIAN_POINT('Ctrl Pts',(-57.4828125340222,41.6642972959168,
0.));
#150940=CARTESIAN_POINT('Ctrl Pts',(-57.4828125340222,41.6642972959168,
12.));
#150941=CARTESIAN_POINT('Ctrl Pts',(-57.4697760492693,41.6466530674522,
0.));
#150942=CARTESIAN_POINT('Ctrl Pts',(-57.4697760492693,41.6466530674522,
12.));
#150943=CARTESIAN_POINT('Ctrl Pts',(-57.4567498065573,41.6290603545674,
0.));
#150944=CARTESIAN_POINT('Ctrl Pts',(-57.4567498065573,41.6290603545674,
12.));
#150945=CARTESIAN_POINT('Ctrl Pts',(-57.4437339539848,41.6115192336393,
0.));
#150946=CARTESIAN_POINT('Ctrl Pts',(-57.4437339539848,41.6115192336393,
12.));
#150947=CARTESIAN_POINT('Ctrl Pts',(-57.4307286404656,41.5940297813474,
0.));
#150948=CARTESIAN_POINT('Ctrl Pts',(-57.4307286404656,41.5940297813474,
12.));
#150949=CARTESIAN_POINT('Ctrl Pts',(-57.417734015749,41.5765920746764,0.));
#150950=CARTESIAN_POINT('Ctrl Pts',(-57.417734015749,41.5765920746764,12.));
#150951=CARTESIAN_POINT('Ctrl Pts',(-57.4047502304207,41.5592061909159,
0.));
#150952=CARTESIAN_POINT('Ctrl Pts',(-57.4047502304207,41.5592061909159,
12.));
#150953=CARTESIAN_POINT('Ctrl Pts',(-57.3917774358844,41.5418722076558,
0.));
#150954=CARTESIAN_POINT('Ctrl Pts',(-57.3917774358844,41.5418722076558,
12.));
#150955=CARTESIAN_POINT('Ctrl Pts',(-57.378815784345,41.5245902027767,0.));
#150956=CARTESIAN_POINT('Ctrl Pts',(-57.378815784345,41.5245902027767,12.));
#150957=CARTESIAN_POINT('Ctrl Pts',(-57.3658654287948,41.5073602544404,
0.));
#150958=CARTESIAN_POINT('Ctrl Pts',(-57.3658654287948,41.5073602544404,
12.));
#150959=CARTESIAN_POINT('Ctrl Pts',(-57.3529265229858,41.4901824410654,
0.));
#150960=CARTESIAN_POINT('Ctrl Pts',(-57.3529265229858,41.4901824410654,
12.));
#150961=CARTESIAN_POINT('Ctrl Pts',(-57.339999221474,41.4730568413535,0.));
#150962=CARTESIAN_POINT('Ctrl Pts',(-57.339999221474,41.4730568413535,12.));
#150963=CARTESIAN_POINT('Ctrl Pts',(-57.3270836796925,41.4559835343338,
0.));
#150964=CARTESIAN_POINT('Ctrl Pts',(-57.3270836796925,41.4559835343338,
12.));
#150965=CARTESIAN_POINT('Ctrl Pts',(-57.3141800540137,41.4389625993948,
0.));
#150966=CARTESIAN_POINT('Ctrl Pts',(-57.3141800540137,41.4389625993948,
12.));
#150967=CARTESIAN_POINT('Ctrl Pts',(-57.3012885018139,41.4219941163154,
0.));
#150968=CARTESIAN_POINT('Ctrl Pts',(-57.3012885018139,41.4219941163154,
12.));
#150969=CARTESIAN_POINT('Ctrl Pts',(-57.2884091815385,41.4050781652923,
0.));
#150970=CARTESIAN_POINT('Ctrl Pts',(-57.2884091815385,41.4050781652923,
12.));
#150971=CARTESIAN_POINT('Ctrl Pts',(-57.2755422525822,41.3882148268798,
0.));
#150972=CARTESIAN_POINT('Ctrl Pts',(-57.2755422525822,41.3882148268798,
12.));
#150973=CARTESIAN_POINT('Ctrl Pts',(-57.2626878751584,41.3714041819215,
0.));
#150974=CARTESIAN_POINT('Ctrl Pts',(-57.2626878751584,41.3714041819215,
12.));
#150975=CARTESIAN_POINT('Ctrl Pts',(-57.2498462101883,41.3546463114889,
0.));
#150976=CARTESIAN_POINT('Ctrl Pts',(-57.2498462101883,41.3546463114889,
12.));
#150977=CARTESIAN_POINT('Ctrl Pts',(-57.237017419142,41.3379412967889,0.));
#150978=CARTESIAN_POINT('Ctrl Pts',(-57.237017419142,41.3379412967889,12.));
#150979=CARTESIAN_POINT('Ctrl Pts',(-57.2242016640226,41.321289219151,0.));
#150980=CARTESIAN_POINT('Ctrl Pts',(-57.2242016640226,41.321289219151,12.));
#150981=CARTESIAN_POINT('Ctrl Pts',(-57.2113991077325,41.304690160231,0.));
#150982=CARTESIAN_POINT('Ctrl Pts',(-57.2113991077325,41.304690160231,12.));
#150983=CARTESIAN_POINT('Ctrl Pts',(-57.1986099143992,41.2881442021869,
0.));
#150984=CARTESIAN_POINT('Ctrl Pts',(-57.1986099143992,41.2881442021869,
12.));
#150985=CARTESIAN_POINT('Ctrl Pts',(-57.1858342496526,41.2716514278268,
0.));
#150986=CARTESIAN_POINT('Ctrl Pts',(-57.1858342496526,41.2716514278268,
12.));
#150987=CARTESIAN_POINT('Ctrl Pts',(-57.1730722810771,41.2552119208445,
0.));
#150988=CARTESIAN_POINT('Ctrl Pts',(-57.1730722810771,41.2552119208445,
12.));
#150989=CARTESIAN_POINT('Ctrl Pts',(-57.1603241779042,41.2388257656534,
0.));
#150990=CARTESIAN_POINT('Ctrl Pts',(-57.1603241779042,41.2388257656534,
12.));
#150991=CARTESIAN_POINT('Ctrl Pts',(-57.1475901101795,41.2224930469412,
0.));
#150992=CARTESIAN_POINT('Ctrl Pts',(-57.1475901101795,41.2224930469412,
12.));
#150993=CARTESIAN_POINT('Ctrl Pts',(-57.1348702480644,41.2062138492913,
0.));
#150994=CARTESIAN_POINT('Ctrl Pts',(-57.1348702480644,41.2062138492913,
12.));
#150995=CARTESIAN_POINT('Ctrl Pts',(-57.1221647611231,41.1899882567941,
0.));
#150996=CARTESIAN_POINT('Ctrl Pts',(-57.1221647611231,41.1899882567941,
12.));
#150997=CARTESIAN_POINT('Ctrl Pts',(-57.1094738174998,41.1738163525931,
0.));
#150998=CARTESIAN_POINT('Ctrl Pts',(-57.1094738174998,41.1738163525931,
12.));
#150999=CARTESIAN_POINT('Ctrl Pts',(-57.0967975854912,41.1576982197402,
0.));
#151000=CARTESIAN_POINT('Ctrl Pts',(-57.0967975854912,41.1576982197402,
12.));
#151001=CARTESIAN_POINT('Ctrl Pts',(-57.0841362354281,41.1416339422132,
0.));
#151002=CARTESIAN_POINT('Ctrl Pts',(-57.0841362354281,41.1416339422132,
12.));
#151003=CARTESIAN_POINT('Ctrl Pts',(-57.0714899412091,41.1256236057436,
0.));
#151004=CARTESIAN_POINT('Ctrl Pts',(-57.0714899412091,41.1256236057436,
12.));
#151005=CARTESIAN_POINT('Ctrl Pts',(-57.0588588825266,41.1096672990125,
0.));
#151006=CARTESIAN_POINT('Ctrl Pts',(-57.0588588825266,41.1096672990125,
12.));
#151007=CARTESIAN_POINT('Ctrl Pts',(-57.0462432450637,41.0937651137519,
0.));
#151008=CARTESIAN_POINT('Ctrl Pts',(-57.0462432450637,41.0937651137519,
12.));
#151009=CARTESIAN_POINT('Ctrl Pts',(-57.0336432158503,41.0779171422415,
0.));
#151010=CARTESIAN_POINT('Ctrl Pts',(-57.0336432158503,41.0779171422415,
12.));
#151011=CARTESIAN_POINT('Ctrl Pts',(-57.0210589791777,41.0621234751,0.));
#151012=CARTESIAN_POINT('Ctrl Pts',(-57.0210589791777,41.0621234751,12.));
#151013=CARTESIAN_POINT('Ctrl Pts',(-57.008490713044,41.0463841993622,0.));
#151014=CARTESIAN_POINT('Ctrl Pts',(-57.008490713044,41.0463841993622,12.));
#151015=CARTESIAN_POINT('Ctrl Pts',(-56.9959385834768,41.0306993954021,
0.));
#151016=CARTESIAN_POINT('Ctrl Pts',(-56.9959385834768,41.0306993954021,
12.));
#151017=CARTESIAN_POINT('Ctrl Pts',(-56.9834027500178,41.0150691398988,
0.));
#151018=CARTESIAN_POINT('Ctrl Pts',(-56.9834027500178,41.0150691398988,
12.));
#151019=CARTESIAN_POINT('Ctrl Pts',(-56.9708833766183,40.9994935117307,
0.));
#151020=CARTESIAN_POINT('Ctrl Pts',(-56.9708833766183,40.9994935117307,
12.));
#151021=CARTESIAN_POINT('Ctrl Pts',(-56.9583806404069,40.9839725967121,
0.));
#151022=CARTESIAN_POINT('Ctrl Pts',(-56.9583806404069,40.9839725967121,
12.));
#151023=CARTESIAN_POINT('Ctrl Pts',(-56.9458947422541,40.968506493303,0.));
#151024=CARTESIAN_POINT('Ctrl Pts',(-56.9458947422541,40.968506493303,12.));
#151025=CARTESIAN_POINT('Ctrl Pts',(-56.9334259139928,40.9530953164952,
0.));
#151026=CARTESIAN_POINT('Ctrl Pts',(-56.9334259139928,40.9530953164952,
12.));
#151027=CARTESIAN_POINT('Ctrl Pts',(-56.9209743960861,40.9377391857044,
0.));
#151028=CARTESIAN_POINT('Ctrl Pts',(-56.9209743960861,40.9377391857044,
12.));
#151029=CARTESIAN_POINT('Ctrl Pts',(-56.9085404164432,40.9224382132382,
0.));
#151030=CARTESIAN_POINT('Ctrl Pts',(-56.9085404164432,40.9224382132382,
12.));
#151031=CARTESIAN_POINT('Ctrl Pts',(-56.8961241708926,40.9071924937551,
0.));
#151032=CARTESIAN_POINT('Ctrl Pts',(-56.8961241708926,40.9071924937551,
12.));
#151033=CARTESIAN_POINT('Ctrl Pts',(-56.8837257978574,40.8920020903443,
0.));
#151034=CARTESIAN_POINT('Ctrl Pts',(-56.8837257978574,40.8920020903443,
12.));
#151035=CARTESIAN_POINT('Ctrl Pts',(-56.8713453765252,40.8768670342278,
0.));
#151036=CARTESIAN_POINT('Ctrl Pts',(-56.8713453765252,40.8768670342278,
12.));
#151037=CARTESIAN_POINT('Ctrl Pts',(-56.8614554317993,40.8648032759631,
0.));
#151038=CARTESIAN_POINT('Ctrl Pts',(-56.8614554317993,40.8648032759631,
12.));
#151039=CARTESIAN_POINT('Ctrl Pts',(-56.8540460739677,40.8557803680411,
0.));
#151040=CARTESIAN_POINT('Ctrl Pts',(-56.8540460739677,40.8557803680411,
12.));
#151041=CARTESIAN_POINT('Ctrl Pts',(-56.8491101022668,40.8497761671086,
0.));
#151042=CARTESIAN_POINT('Ctrl Pts',(-56.8491101022668,40.8497761671086,
12.));
#151043=CARTESIAN_POINT('Ctrl Pts',(-56.8466430164621,40.8467768343956,
0.));
#151044=CARTESIAN_POINT('Ctrl Pts',(-56.8466430164621,40.8467768343956,
12.));
#151045=CARTESIAN_POINT('',(-56.8466430164621,40.8467768343956,12.));
#151046=CARTESIAN_POINT('Ctrl Pts',(-56.8466430164621,40.8467768343956,
12.));
#151047=CARTESIAN_POINT('Ctrl Pts',(-56.8491101022668,40.8497761671086,
12.));
#151048=CARTESIAN_POINT('Ctrl Pts',(-56.8540460739677,40.8557803680411,
12.));
#151049=CARTESIAN_POINT('Ctrl Pts',(-56.8614554317993,40.8648032759631,
12.));
#151050=CARTESIAN_POINT('Ctrl Pts',(-56.8713453765252,40.8768670342278,
12.));
#151051=CARTESIAN_POINT('Ctrl Pts',(-56.8837257978574,40.8920020903443,
12.));
#151052=CARTESIAN_POINT('Ctrl Pts',(-56.8961241708926,40.9071924937551,
12.));
#151053=CARTESIAN_POINT('Ctrl Pts',(-56.9085404164432,40.9224382132382,
12.));
#151054=CARTESIAN_POINT('Ctrl Pts',(-56.9209743960861,40.9377391857044,
12.));
#151055=CARTESIAN_POINT('Ctrl Pts',(-56.9334259139928,40.9530953164952,
12.));
#151056=CARTESIAN_POINT('Ctrl Pts',(-56.9458947422541,40.968506493303,12.));
#151057=CARTESIAN_POINT('Ctrl Pts',(-56.9583806404069,40.9839725967121,
12.));
#151058=CARTESIAN_POINT('Ctrl Pts',(-56.9708833766183,40.9994935117307,
12.));
#151059=CARTESIAN_POINT('Ctrl Pts',(-56.9834027500178,41.0150691398988,
12.));
#151060=CARTESIAN_POINT('Ctrl Pts',(-56.9959385834768,41.0306993954021,
12.));
#151061=CARTESIAN_POINT('Ctrl Pts',(-57.008490713044,41.0463841993622,12.));
#151062=CARTESIAN_POINT('Ctrl Pts',(-57.0210589791777,41.0621234751,12.));
#151063=CARTESIAN_POINT('Ctrl Pts',(-57.0336432158503,41.0779171422415,
12.));
#151064=CARTESIAN_POINT('Ctrl Pts',(-57.0462432450637,41.0937651137519,
12.));
#151065=CARTESIAN_POINT('Ctrl Pts',(-57.0588588825266,41.1096672990125,
12.));
#151066=CARTESIAN_POINT('Ctrl Pts',(-57.0714899412091,41.1256236057436,
12.));
#151067=CARTESIAN_POINT('Ctrl Pts',(-57.0841362354281,41.1416339422132,
12.));
#151068=CARTESIAN_POINT('Ctrl Pts',(-57.0967975854912,41.1576982197402,
12.));
#151069=CARTESIAN_POINT('Ctrl Pts',(-57.1094738174998,41.1738163525931,
12.));
#151070=CARTESIAN_POINT('Ctrl Pts',(-57.1221647611231,41.1899882567941,
12.));
#151071=CARTESIAN_POINT('Ctrl Pts',(-57.1348702480644,41.2062138492913,
12.));
#151072=CARTESIAN_POINT('Ctrl Pts',(-57.1475901101795,41.2224930469412,
12.));
#151073=CARTESIAN_POINT('Ctrl Pts',(-57.1603241779042,41.2388257656534,
12.));
#151074=CARTESIAN_POINT('Ctrl Pts',(-57.1730722810771,41.2552119208445,
12.));
#151075=CARTESIAN_POINT('Ctrl Pts',(-57.1858342496526,41.2716514278268,
12.));
#151076=CARTESIAN_POINT('Ctrl Pts',(-57.1986099143992,41.2881442021869,
12.));
#151077=CARTESIAN_POINT('Ctrl Pts',(-57.2113991077325,41.304690160231,12.));
#151078=CARTESIAN_POINT('Ctrl Pts',(-57.2242016640226,41.321289219151,12.));
#151079=CARTESIAN_POINT('Ctrl Pts',(-57.237017419142,41.3379412967889,12.));
#151080=CARTESIAN_POINT('Ctrl Pts',(-57.2498462101883,41.3546463114889,
12.));
#151081=CARTESIAN_POINT('Ctrl Pts',(-57.2626878751584,41.3714041819215,
12.));
#151082=CARTESIAN_POINT('Ctrl Pts',(-57.2755422525822,41.3882148268798,
12.));
#151083=CARTESIAN_POINT('Ctrl Pts',(-57.2884091815385,41.4050781652923,
12.));
#151084=CARTESIAN_POINT('Ctrl Pts',(-57.3012885018139,41.4219941163154,
12.));
#151085=CARTESIAN_POINT('Ctrl Pts',(-57.3141800540137,41.4389625993948,
12.));
#151086=CARTESIAN_POINT('Ctrl Pts',(-57.3270836796925,41.4559835343338,
12.));
#151087=CARTESIAN_POINT('Ctrl Pts',(-57.339999221474,41.4730568413535,12.));
#151088=CARTESIAN_POINT('Ctrl Pts',(-57.3529265229858,41.4901824410654,
12.));
#151089=CARTESIAN_POINT('Ctrl Pts',(-57.3658654287948,41.5073602544404,
12.));
#151090=CARTESIAN_POINT('Ctrl Pts',(-57.378815784345,41.5245902027767,12.));
#151091=CARTESIAN_POINT('Ctrl Pts',(-57.3917774358844,41.5418722076558,
12.));
#151092=CARTESIAN_POINT('Ctrl Pts',(-57.4047502304207,41.5592061909159,
12.));
#151093=CARTESIAN_POINT('Ctrl Pts',(-57.417734015749,41.5765920746764,12.));
#151094=CARTESIAN_POINT('Ctrl Pts',(-57.4307286404656,41.5940297813474,
12.));
#151095=CARTESIAN_POINT('Ctrl Pts',(-57.4437339539848,41.6115192336393,
12.));
#151096=CARTESIAN_POINT('Ctrl Pts',(-57.4567498065573,41.6290603545674,
12.));
#151097=CARTESIAN_POINT('Ctrl Pts',(-57.4697760492693,41.6466530674522,
12.));
#151098=CARTESIAN_POINT('Ctrl Pts',(-57.4828125340222,41.6642972959168,
12.));
#151099=CARTESIAN_POINT('Ctrl Pts',(-57.4958591135165,41.6819929638797,
12.));
#151100=CARTESIAN_POINT('Ctrl Pts',(-57.5089156412341,41.6997399955445,
12.));
#151101=CARTESIAN_POINT('Ctrl Pts',(-57.5219819714169,41.7175383153819,
12.));
#151102=CARTESIAN_POINT('Ctrl Pts',(-57.5350579590648,41.7353878481336,
12.));
#151103=CARTESIAN_POINT('Ctrl Pts',(-57.5481434599334,41.7532885188174,
12.));
#151104=CARTESIAN_POINT('Ctrl Pts',(-57.561238330532,41.7712402527273,12.));
#151105=CARTESIAN_POINT('Ctrl Pts',(-57.5743424281204,41.7892429754298,
12.));
#151106=CARTESIAN_POINT('Ctrl Pts',(-57.5874556107054,41.8072966127559,
12.));
#151107=CARTESIAN_POINT('Ctrl Pts',(-57.6005777370347,41.8254010908051,
12.));
#151108=CARTESIAN_POINT('Ctrl Pts',(-57.613708666588,41.8435563359456,12.));
#151109=CARTESIAN_POINT('Ctrl Pts',(-57.6268482595701,41.8617622748107,
12.));
#151110=CARTESIAN_POINT('Ctrl Pts',(-57.6399963769009,41.8800188342912,
12.));
#151111=CARTESIAN_POINT('Ctrl Pts',(-57.6531528802072,41.8983259415253,
12.));
#151112=CARTESIAN_POINT('Ctrl Pts',(-57.6663176318189,41.9166835239054,
12.));
#151113=CARTESIAN_POINT('Ctrl Pts',(-57.6794904947649,41.9350915090796,
12.));
#151114=CARTESIAN_POINT('Ctrl Pts',(-57.6926713327672,41.9535498249488,
12.));
#151115=CARTESIAN_POINT('Ctrl Pts',(-57.7058600102351,41.9720583996592,
12.));
#151116=CARTESIAN_POINT('Ctrl Pts',(-57.7190563922593,41.990617161596,12.));
#151117=CARTESIAN_POINT('Ctrl Pts',(-57.7322603446066,42.0092260393897,
12.));
#151118=CARTESIAN_POINT('Ctrl Pts',(-57.745471733714,42.0278849619148,12.));
#151119=CARTESIAN_POINT('Ctrl Pts',(-57.7586904266834,42.0465938582882,
12.));
#151120=CARTESIAN_POINT('Ctrl Pts',(-57.7719162912744,42.0653526578588,
12.));
#151121=CARTESIAN_POINT('Ctrl Pts',(-57.7851491958987,42.0841612902042,
12.));
#151122=CARTESIAN_POINT('Ctrl Pts',(-57.798389009616,42.1030196851366,12.));
#151123=CARTESIAN_POINT('Ctrl Pts',(-57.8116356021288,42.1219277727021,
12.));
#151124=CARTESIAN_POINT('Ctrl Pts',(-57.8248888437775,42.1408854831783,
12.));
#151125=CARTESIAN_POINT('Ctrl Pts',(-57.8381486055342,42.1598927470646,
12.));
#151126=CARTESIAN_POINT('Ctrl Pts',(-57.8514147589972,42.1789494950794,
12.));
#151127=CARTESIAN_POINT('Ctrl Pts',(-57.864687176387,42.1980556581665,12.));
#151128=CARTESIAN_POINT('Ctrl Pts',(-57.8779657305413,42.2172111674938,
12.));
#151129=CARTESIAN_POINT('Ctrl Pts',(-57.8912502949096,42.2364159544501,
12.));
#151130=CARTESIAN_POINT('Ctrl Pts',(-57.9045407435474,42.2556699506353,
12.));
#151131=CARTESIAN_POINT('Ctrl Pts',(-57.9178369511114,42.2749730878594,
12.));
#151132=CARTESIAN_POINT('Ctrl Pts',(-57.9311387928563,42.2943252981489,
12.));
#151133=CARTESIAN_POINT('Ctrl Pts',(-57.9444461446299,42.3137265137452,
12.));
#151134=CARTESIAN_POINT('Ctrl Pts',(-57.9577588828682,42.333176667102,12.));
#151135=CARTESIAN_POINT('Ctrl Pts',(-57.9710768845899,42.3526756908746,
12.));
#151136=CARTESIAN_POINT('Ctrl Pts',(-57.9844000273911,42.3722235179197,
12.));
#151137=CARTESIAN_POINT('Ctrl Pts',(-57.9977281894422,42.3918200813014,
12.));
#151138=CARTESIAN_POINT('Ctrl Pts',(-58.0110612494828,42.411465314289,12.));
#151139=CARTESIAN_POINT('Ctrl Pts',(-58.0243990868181,42.4311591503555,
12.));
#151140=CARTESIAN_POINT('Ctrl Pts',(-58.037741581314,42.4509015231674,12.));
#151141=CARTESIAN_POINT('Ctrl Pts',(-58.0510886133926,42.4706923665845,
12.));
#151142=CARTESIAN_POINT('Ctrl Pts',(-58.0644400640275,42.4905316146653,
12.));
#151143=CARTESIAN_POINT('Ctrl Pts',(-58.0777958147403,42.5104192016664,
12.));
#151144=CARTESIAN_POINT('Ctrl Pts',(-58.0911557475965,42.5303550620387,
12.));
#151145=CARTESIAN_POINT('Ctrl Pts',(-58.1045197452002,42.5503391304183,
12.));
#151146=CARTESIAN_POINT('Ctrl Pts',(-58.1178876906907,42.5703713416265,
12.));
#151147=CARTESIAN_POINT('Ctrl Pts',(-58.1312594677386,42.5904516306762,
12.));
#151148=CARTESIAN_POINT('Ctrl Pts',(-58.1446349605421,42.6105799327699,
12.));
#151149=CARTESIAN_POINT('Ctrl Pts',(-58.1580140538228,42.6307561832976,
12.));
#151150=CARTESIAN_POINT('Ctrl Pts',(-58.171396632821,42.6509803178265,12.));
#151151=CARTESIAN_POINT('Ctrl Pts',(-58.1847825832923,42.6712522721016,
12.));
#151152=CARTESIAN_POINT('Ctrl Pts',(-58.1981717915037,42.6915719820513,
12.));
#151153=CARTESIAN_POINT('Ctrl Pts',(-58.21156414423,42.7119393837866,12.));
#151154=CARTESIAN_POINT('Ctrl Pts',(-58.22495952875,42.7323544135985,12.));
#151155=CARTESIAN_POINT('Ctrl Pts',(-58.2383578328424,42.7528170079484,
12.));
#151156=CARTESIAN_POINT('Ctrl Pts',(-58.251758944782,42.7733271034679,12.));
#151157=CARTESIAN_POINT('Ctrl Pts',(-58.2651627533368,42.7938846369651,
12.));
#151158=CARTESIAN_POINT('Ctrl Pts',(-58.2785691477638,42.8144895454233,
12.));
#151159=CARTESIAN_POINT('Ctrl Pts',(-58.2919780178064,42.8351417659999,
12.));
#151160=CARTESIAN_POINT('Ctrl Pts',(-58.3053892536894,42.8558412360158,
12.));
#151161=CARTESIAN_POINT('Ctrl Pts',(-58.3188027461164,42.8765878929551,
12.));
#151162=CARTESIAN_POINT('Ctrl Pts',(-58.3322183862654,42.8973816744709,
12.));
#151163=CARTESIAN_POINT('Ctrl Pts',(-58.3456360657865,42.9182225183855,
12.));
#151164=CARTESIAN_POINT('Ctrl Pts',(-58.3590556767978,42.9391103626879,
12.));
#151165=CARTESIAN_POINT('Ctrl Pts',(-58.3724771118826,42.960045145526,12.));
#151166=CARTESIAN_POINT('Ctrl Pts',(-58.3859002640856,42.9810268052032,
12.));
#151167=CARTESIAN_POINT('Ctrl Pts',(-58.3993250269101,43.0020552801859,
12.));
#151168=CARTESIAN_POINT('Ctrl Pts',(-58.4127512943136,43.0231305091027,
12.));
#151169=CARTESIAN_POINT('Ctrl Pts',(-58.4261789607058,43.0442524307434,
12.));
#151170=CARTESIAN_POINT('Ctrl Pts',(-58.439607920945,43.0654209840511,12.));
#151171=CARTESIAN_POINT('Ctrl Pts',(-58.4530380703348,43.0866361081177,
12.));
#151172=CARTESIAN_POINT('Ctrl Pts',(-58.4664693046217,43.1078977421916,
12.));
#151173=CARTESIAN_POINT('Ctrl Pts',(-58.4799015199907,43.1292058256777,
12.));
#151174=CARTESIAN_POINT('Ctrl Pts',(-58.4933346130636,43.1505602981365,
12.));
#151175=CARTESIAN_POINT('Ctrl Pts',(-58.5067684808944,43.1719610992771,
12.));
#151176=CARTESIAN_POINT('Ctrl Pts',(-58.5202030209669,43.1934081689505,
12.));
#151177=CARTESIAN_POINT('Ctrl Pts',(-58.5336381311917,43.2149014471574,
12.));
#151178=CARTESIAN_POINT('Ctrl Pts',(-58.5470737099032,43.2364408740493,
12.));
#151179=CARTESIAN_POINT('Ctrl Pts',(-58.5605096558578,43.2580263899278,
12.));
#151180=CARTESIAN_POINT('Ctrl Pts',(-58.573945868231,43.27965793524,12.));
#151181=CARTESIAN_POINT('Ctrl Pts',(-58.5873822466152,43.3013354505701,
12.));
#151182=CARTESIAN_POINT('Ctrl Pts',(-58.6008186910156,43.3230588766449,
12.));
#151183=CARTESIAN_POINT('Ctrl Pts',(-58.6142551018467,43.3448281543371,
12.));
#151184=CARTESIAN_POINT('Ctrl Pts',(-58.627691379929,43.3666432246635,12.));
#151185=CARTESIAN_POINT('Ctrl Pts',(-58.6411274264857,43.388504028781,12.));
#151186=CARTESIAN_POINT('Ctrl Pts',(-58.6545631431393,43.4104105079768,
12.));
#151187=CARTESIAN_POINT('Ctrl Pts',(-58.6679984319097,43.4323626036737,
12.));
#151188=CARTESIAN_POINT('Ctrl Pts',(-58.6814331952138,43.4543602574351,
12.));
#151189=CARTESIAN_POINT('Ctrl Pts',(-58.6948673358638,43.4764034109654,
12.));
#151190=CARTESIAN_POINT('Ctrl Pts',(-58.7083007570661,43.4984920061073,
12.));
#151191=CARTESIAN_POINT('Ctrl Pts',(-58.7217333624209,43.5206259848337,
12.));
#151192=CARTESIAN_POINT('Ctrl Pts',(-58.735165055918,43.5428052892488,12.));
#151193=CARTESIAN_POINT('Ctrl Pts',(-58.74859574193,43.5650298615917,12.));
#151194=CARTESIAN_POINT('Ctrl Pts',(-58.7620253252062,43.5872996442345,
12.));
#151195=CARTESIAN_POINT('Ctrl Pts',(-58.775453710867,43.6096145796797,12.));
#151196=CARTESIAN_POINT('Ctrl Pts',(-58.788880804397,43.6319746105482,12.));
#151197=CARTESIAN_POINT('Ctrl Pts',(-58.8023065116436,43.6543796795789,
12.));
#151198=CARTESIAN_POINT('Ctrl Pts',(-58.8157307388238,43.6768297296395,
12.));
#151199=CARTESIAN_POINT('Ctrl Pts',(-58.8291533925293,43.6993247037314,
12.));
#151200=CARTESIAN_POINT('Ctrl Pts',(-58.8425743797326,43.7218645449922,
12.));
#151201=CARTESIAN_POINT('Ctrl Pts',(-58.855993607794,43.7444491966942,12.));
#151202=CARTESIAN_POINT('Ctrl Pts',(-58.8694109844648,43.7670786022402,
12.));
#151203=CARTESIAN_POINT('Ctrl Pts',(-58.8828264178621,43.7897527051609,
12.));
#151204=CARTESIAN_POINT('Ctrl Pts',(-58.8962398164493,43.8124714491076,
12.));
#151205=CARTESIAN_POINT('Ctrl Pts',(-58.9096510890129,43.835234777842,12.));
#151206=CARTESIAN_POINT('Ctrl Pts',(-58.9230601446436,43.858042635223,12.));
#151207=CARTESIAN_POINT('Ctrl Pts',(-58.936466892712,43.8808949651873,12.));
#151208=CARTESIAN_POINT('Ctrl Pts',(-58.9498712429054,43.9037917117739,
12.));
#151209=CARTESIAN_POINT('Ctrl Pts',(-58.9632731052696,43.9267328191501,
12.));
#151210=CARTESIAN_POINT('Ctrl Pts',(-58.9766723902529,43.9497182316331,
12.));
#151211=CARTESIAN_POINT('Ctrl Pts',(-58.9900690087408,43.9727478937056,
12.));
#151212=CARTESIAN_POINT('Ctrl Pts',(-59.0034628721168,43.9958217500369,
12.));
#151213=CARTESIAN_POINT('Ctrl Pts',(-59.0168538922095,44.0189397454599,
12.));
#151214=CARTESIAN_POINT('Ctrl Pts',(-59.0302419811777,44.0421018249223,
12.));
#151215=CARTESIAN_POINT('Ctrl Pts',(-59.0436270514087,44.0653079334385,
12.));
#151216=CARTESIAN_POINT('Ctrl Pts',(-59.0570090154243,44.0885580160432,
12.));
#151217=CARTESIAN_POINT('Ctrl Pts',(-59.0703877857526,44.1118520177221,
12.));
#151218=CARTESIAN_POINT('Ctrl Pts',(-59.08376327492,44.1351898834051,12.));
#151219=CARTESIAN_POINT('Ctrl Pts',(-59.0971353957206,44.1585715581064,
12.));
#151220=CARTESIAN_POINT('Ctrl Pts',(-59.1105040614276,44.1819969870307,
12.));
#151221=CARTESIAN_POINT('Ctrl Pts',(-59.1238691860306,44.2054661156875,
12.));
#151222=CARTESIAN_POINT('Ctrl Pts',(-59.1372306844586,44.228978889997,12.));
#151223=CARTESIAN_POINT('Ctrl Pts',(-59.1505884728215,44.2525352563996,
12.));
#151224=CARTESIAN_POINT('Ctrl Pts',(-59.1639424678793,44.2761351616048,
12.));
#151225=CARTESIAN_POINT('Ctrl Pts',(-59.1772925865213,44.2997785523431,
12.));
#151226=CARTESIAN_POINT('Ctrl Pts',(-59.1906387451979,44.3234653750884,
12.));
#151227=CARTESIAN_POINT('Ctrl Pts',(-59.2039808594752,44.3471955758403,
12.));
#151228=CARTESIAN_POINT('Ctrl Pts',(-59.2173188432798,44.3709690997469,
12.));
#151229=CARTESIAN_POINT('Ctrl Pts',(-59.2306526095131,44.3947858914074,
12.));
#151230=CARTESIAN_POINT('Ctrl Pts',(-59.2439820714187,44.4186458955451,
12.));
#151231=CARTESIAN_POINT('Ctrl Pts',(-59.2573071437774,44.4425490575911,
12.));
#151232=CARTESIAN_POINT('Ctrl Pts',(-59.2706277440445,44.4664953242379,
12.));
#151233=CARTESIAN_POINT('Ctrl Pts',(-59.2839437938237,44.490484644151,12.));
#151234=CARTESIAN_POINT('Ctrl Pts',(-59.2972552192156,44.5145169681349,
12.));
#151235=CARTESIAN_POINT('Ctrl Pts',(-59.3086616639523,44.5351541478479,
12.));
#151236=CARTESIAN_POINT('Ctrl Pts',(-59.3174041872347,44.5509994358154,
12.));
#151237=CARTESIAN_POINT('Ctrl Pts',(-59.3234848865455,44.5620338188738,
12.));
#151238=CARTESIAN_POINT('Ctrl Pts',(-59.3269051738423,44.5682447396021,
12.));
#151239=CARTESIAN_POINT('Ctrl Pts',(-59.3276657444392,44.5696260757792,
12.));
#151240=CARTESIAN_POINT('',(-56.8466430164621,40.8467768343956,0.));
#151241=CARTESIAN_POINT('',(-56.8466430164621,40.8467768343956,0.));
#151242=CARTESIAN_POINT('Ctrl Pts',(-59.3276657444392,44.5696260757791,
0.));
#151243=CARTESIAN_POINT('Ctrl Pts',(-59.3269051738423,44.5682447396021,
0.));
#151244=CARTESIAN_POINT('Ctrl Pts',(-59.3234848865455,44.5620338188738,
0.));
#151245=CARTESIAN_POINT('Ctrl Pts',(-59.3174041872347,44.5509994358154,
0.));
#151246=CARTESIAN_POINT('Ctrl Pts',(-59.3086616639523,44.5351541478479,
0.));
#151247=CARTESIAN_POINT('Ctrl Pts',(-59.2972552192156,44.5145169681349,
0.));
#151248=CARTESIAN_POINT('Ctrl Pts',(-59.2839437938237,44.490484644151,0.));
#151249=CARTESIAN_POINT('Ctrl Pts',(-59.2706277440445,44.4664953242379,
0.));
#151250=CARTESIAN_POINT('Ctrl Pts',(-59.2573071437774,44.4425490575911,
0.));
#151251=CARTESIAN_POINT('Ctrl Pts',(-59.2439820714187,44.4186458955451,
0.));
#151252=CARTESIAN_POINT('Ctrl Pts',(-59.2306526095131,44.3947858914074,
0.));
#151253=CARTESIAN_POINT('Ctrl Pts',(-59.2173188432798,44.3709690997469,
0.));
#151254=CARTESIAN_POINT('Ctrl Pts',(-59.2039808594752,44.3471955758403,
0.));
#151255=CARTESIAN_POINT('Ctrl Pts',(-59.1906387451979,44.3234653750884,
0.));
#151256=CARTESIAN_POINT('Ctrl Pts',(-59.1772925865213,44.2997785523431,
0.));
#151257=CARTESIAN_POINT('Ctrl Pts',(-59.1639424678793,44.2761351616048,
0.));
#151258=CARTESIAN_POINT('Ctrl Pts',(-59.1505884728215,44.2525352563996,
0.));
#151259=CARTESIAN_POINT('Ctrl Pts',(-59.1372306844586,44.228978889997,0.));
#151260=CARTESIAN_POINT('Ctrl Pts',(-59.1238691860306,44.2054661156875,
0.));
#151261=CARTESIAN_POINT('Ctrl Pts',(-59.1105040614276,44.1819969870307,
0.));
#151262=CARTESIAN_POINT('Ctrl Pts',(-59.0971353957206,44.1585715581064,
0.));
#151263=CARTESIAN_POINT('Ctrl Pts',(-59.08376327492,44.1351898834051,0.));
#151264=CARTESIAN_POINT('Ctrl Pts',(-59.0703877857526,44.1118520177221,
0.));
#151265=CARTESIAN_POINT('Ctrl Pts',(-59.0570090154243,44.0885580160432,
0.));
#151266=CARTESIAN_POINT('Ctrl Pts',(-59.0436270514087,44.0653079334385,
0.));
#151267=CARTESIAN_POINT('Ctrl Pts',(-59.0302419811777,44.0421018249223,
0.));
#151268=CARTESIAN_POINT('Ctrl Pts',(-59.0168538922095,44.0189397454599,
0.));
#151269=CARTESIAN_POINT('Ctrl Pts',(-59.0034628721168,43.9958217500369,
0.));
#151270=CARTESIAN_POINT('Ctrl Pts',(-58.9900690087408,43.9727478937056,
0.));
#151271=CARTESIAN_POINT('Ctrl Pts',(-58.9766723902529,43.9497182316331,
0.));
#151272=CARTESIAN_POINT('Ctrl Pts',(-58.9632731052696,43.9267328191501,
0.));
#151273=CARTESIAN_POINT('Ctrl Pts',(-58.9498712429054,43.9037917117739,
0.));
#151274=CARTESIAN_POINT('Ctrl Pts',(-58.936466892712,43.8808949651873,0.));
#151275=CARTESIAN_POINT('Ctrl Pts',(-58.9230601446436,43.858042635223,0.));
#151276=CARTESIAN_POINT('Ctrl Pts',(-58.9096510890129,43.835234777842,0.));
#151277=CARTESIAN_POINT('Ctrl Pts',(-58.8962398164493,43.8124714491076,
0.));
#151278=CARTESIAN_POINT('Ctrl Pts',(-58.8828264178621,43.7897527051609,
0.));
#151279=CARTESIAN_POINT('Ctrl Pts',(-58.8694109844648,43.7670786022402,
0.));
#151280=CARTESIAN_POINT('Ctrl Pts',(-58.855993607794,43.7444491966942,0.));
#151281=CARTESIAN_POINT('Ctrl Pts',(-58.8425743797326,43.7218645449922,
0.));
#151282=CARTESIAN_POINT('Ctrl Pts',(-58.8291533925293,43.6993247037314,
0.));
#151283=CARTESIAN_POINT('Ctrl Pts',(-58.8157307388238,43.6768297296395,
0.));
#151284=CARTESIAN_POINT('Ctrl Pts',(-58.8023065116436,43.6543796795789,
0.));
#151285=CARTESIAN_POINT('Ctrl Pts',(-58.788880804397,43.6319746105482,0.));
#151286=CARTESIAN_POINT('Ctrl Pts',(-58.775453710867,43.6096145796797,0.));
#151287=CARTESIAN_POINT('Ctrl Pts',(-58.7620253252062,43.5872996442345,
0.));
#151288=CARTESIAN_POINT('Ctrl Pts',(-58.74859574193,43.5650298615917,0.));
#151289=CARTESIAN_POINT('Ctrl Pts',(-58.735165055918,43.5428052892488,0.));
#151290=CARTESIAN_POINT('Ctrl Pts',(-58.7217333624209,43.5206259848337,
0.));
#151291=CARTESIAN_POINT('Ctrl Pts',(-58.7083007570661,43.4984920061073,
0.));
#151292=CARTESIAN_POINT('Ctrl Pts',(-58.6948673358638,43.4764034109654,
0.));
#151293=CARTESIAN_POINT('Ctrl Pts',(-58.6814331952138,43.4543602574351,
0.));
#151294=CARTESIAN_POINT('Ctrl Pts',(-58.6679984319097,43.4323626036737,
0.));
#151295=CARTESIAN_POINT('Ctrl Pts',(-58.6545631431393,43.4104105079768,
0.));
#151296=CARTESIAN_POINT('Ctrl Pts',(-58.6411274264857,43.388504028781,0.));
#151297=CARTESIAN_POINT('Ctrl Pts',(-58.627691379929,43.3666432246635,0.));
#151298=CARTESIAN_POINT('Ctrl Pts',(-58.6142551018467,43.3448281543371,
0.));
#151299=CARTESIAN_POINT('Ctrl Pts',(-58.6008186910156,43.3230588766449,
0.));
#151300=CARTESIAN_POINT('Ctrl Pts',(-58.5873822466152,43.3013354505701,
0.));
#151301=CARTESIAN_POINT('Ctrl Pts',(-58.573945868231,43.27965793524,0.));
#151302=CARTESIAN_POINT('Ctrl Pts',(-58.5605096558578,43.2580263899278,
0.));
#151303=CARTESIAN_POINT('Ctrl Pts',(-58.5470737099032,43.2364408740493,
0.));
#151304=CARTESIAN_POINT('Ctrl Pts',(-58.5336381311917,43.2149014471574,
0.));
#151305=CARTESIAN_POINT('Ctrl Pts',(-58.5202030209669,43.1934081689505,
0.));
#151306=CARTESIAN_POINT('Ctrl Pts',(-58.5067684808944,43.1719610992771,
0.));
#151307=CARTESIAN_POINT('Ctrl Pts',(-58.4933346130636,43.1505602981365,
0.));
#151308=CARTESIAN_POINT('Ctrl Pts',(-58.4799015199907,43.1292058256777,
0.));
#151309=CARTESIAN_POINT('Ctrl Pts',(-58.4664693046217,43.1078977421916,
0.));
#151310=CARTESIAN_POINT('Ctrl Pts',(-58.4530380703348,43.0866361081177,
0.));
#151311=CARTESIAN_POINT('Ctrl Pts',(-58.439607920945,43.0654209840511,0.));
#151312=CARTESIAN_POINT('Ctrl Pts',(-58.4261789607058,43.0442524307434,
0.));
#151313=CARTESIAN_POINT('Ctrl Pts',(-58.4127512943136,43.0231305091027,
0.));
#151314=CARTESIAN_POINT('Ctrl Pts',(-58.3993250269101,43.0020552801859,
0.));
#151315=CARTESIAN_POINT('Ctrl Pts',(-58.3859002640856,42.9810268052032,
0.));
#151316=CARTESIAN_POINT('Ctrl Pts',(-58.3724771118826,42.960045145526,0.));
#151317=CARTESIAN_POINT('Ctrl Pts',(-58.3590556767978,42.9391103626879,
0.));
#151318=CARTESIAN_POINT('Ctrl Pts',(-58.3456360657865,42.9182225183855,
0.));
#151319=CARTESIAN_POINT('Ctrl Pts',(-58.3322183862654,42.8973816744709,
0.));
#151320=CARTESIAN_POINT('Ctrl Pts',(-58.3188027461164,42.8765878929551,
0.));
#151321=CARTESIAN_POINT('Ctrl Pts',(-58.3053892536894,42.8558412360158,
0.));
#151322=CARTESIAN_POINT('Ctrl Pts',(-58.2919780178064,42.8351417659999,
0.));
#151323=CARTESIAN_POINT('Ctrl Pts',(-58.2785691477638,42.8144895454233,
0.));
#151324=CARTESIAN_POINT('Ctrl Pts',(-58.2651627533368,42.7938846369651,
0.));
#151325=CARTESIAN_POINT('Ctrl Pts',(-58.251758944782,42.7733271034679,0.));
#151326=CARTESIAN_POINT('Ctrl Pts',(-58.2383578328424,42.7528170079484,
0.));
#151327=CARTESIAN_POINT('Ctrl Pts',(-58.22495952875,42.7323544135985,0.));
#151328=CARTESIAN_POINT('Ctrl Pts',(-58.21156414423,42.7119393837866,0.));
#151329=CARTESIAN_POINT('Ctrl Pts',(-58.1981717915037,42.6915719820513,
0.));
#151330=CARTESIAN_POINT('Ctrl Pts',(-58.1847825832923,42.6712522721016,
0.));
#151331=CARTESIAN_POINT('Ctrl Pts',(-58.171396632821,42.6509803178265,0.));
#151332=CARTESIAN_POINT('Ctrl Pts',(-58.1580140538228,42.6307561832976,
0.));
#151333=CARTESIAN_POINT('Ctrl Pts',(-58.1446349605421,42.6105799327699,
0.));
#151334=CARTESIAN_POINT('Ctrl Pts',(-58.1312594677386,42.5904516306762,
0.));
#151335=CARTESIAN_POINT('Ctrl Pts',(-58.1178876906907,42.5703713416265,
0.));
#151336=CARTESIAN_POINT('Ctrl Pts',(-58.1045197452002,42.5503391304183,
0.));
#151337=CARTESIAN_POINT('Ctrl Pts',(-58.0911557475965,42.5303550620387,
0.));
#151338=CARTESIAN_POINT('Ctrl Pts',(-58.0777958147403,42.5104192016664,
0.));
#151339=CARTESIAN_POINT('Ctrl Pts',(-58.0644400640275,42.4905316146653,
0.));
#151340=CARTESIAN_POINT('Ctrl Pts',(-58.0510886133926,42.4706923665845,
0.));
#151341=CARTESIAN_POINT('Ctrl Pts',(-58.037741581314,42.4509015231674,0.));
#151342=CARTESIAN_POINT('Ctrl Pts',(-58.0243990868181,42.4311591503555,
0.));
#151343=CARTESIAN_POINT('Ctrl Pts',(-58.0110612494828,42.411465314289,0.));
#151344=CARTESIAN_POINT('Ctrl Pts',(-57.9977281894422,42.3918200813014,
0.));
#151345=CARTESIAN_POINT('Ctrl Pts',(-57.9844000273911,42.3722235179197,
0.));
#151346=CARTESIAN_POINT('Ctrl Pts',(-57.9710768845899,42.3526756908746,
0.));
#151347=CARTESIAN_POINT('Ctrl Pts',(-57.9577588828682,42.333176667102,0.));
#151348=CARTESIAN_POINT('Ctrl Pts',(-57.9444461446299,42.3137265137452,
0.));
#151349=CARTESIAN_POINT('Ctrl Pts',(-57.9311387928563,42.2943252981489,
0.));
#151350=CARTESIAN_POINT('Ctrl Pts',(-57.9178369511114,42.2749730878594,
0.));
#151351=CARTESIAN_POINT('Ctrl Pts',(-57.9045407435474,42.2556699506353,
0.));
#151352=CARTESIAN_POINT('Ctrl Pts',(-57.8912502949096,42.2364159544501,
0.));
#151353=CARTESIAN_POINT('Ctrl Pts',(-57.8779657305413,42.2172111674938,
0.));
#151354=CARTESIAN_POINT('Ctrl Pts',(-57.864687176387,42.1980556581665,0.));
#151355=CARTESIAN_POINT('Ctrl Pts',(-57.8514147589972,42.1789494950794,
0.));
#151356=CARTESIAN_POINT('Ctrl Pts',(-57.8381486055342,42.1598927470646,
0.));
#151357=CARTESIAN_POINT('Ctrl Pts',(-57.8248888437775,42.1408854831783,
0.));
#151358=CARTESIAN_POINT('Ctrl Pts',(-57.8116356021288,42.1219277727021,
0.));
#151359=CARTESIAN_POINT('Ctrl Pts',(-57.798389009616,42.1030196851366,0.));
#151360=CARTESIAN_POINT('Ctrl Pts',(-57.7851491958987,42.0841612902042,
0.));
#151361=CARTESIAN_POINT('Ctrl Pts',(-57.7719162912744,42.0653526578588,
0.));
#151362=CARTESIAN_POINT('Ctrl Pts',(-57.7586904266834,42.0465938582882,
0.));
#151363=CARTESIAN_POINT('Ctrl Pts',(-57.745471733714,42.0278849619148,0.));
#151364=CARTESIAN_POINT('Ctrl Pts',(-57.7322603446066,42.0092260393897,
0.));
#151365=CARTESIAN_POINT('Ctrl Pts',(-57.7190563922593,41.990617161596,0.));
#151366=CARTESIAN_POINT('Ctrl Pts',(-57.7058600102351,41.9720583996592,
0.));
#151367=CARTESIAN_POINT('Ctrl Pts',(-57.6926713327672,41.9535498249488,
0.));
#151368=CARTESIAN_POINT('Ctrl Pts',(-57.6794904947649,41.9350915090796,
0.));
#151369=CARTESIAN_POINT('Ctrl Pts',(-57.6663176318189,41.9166835239054,
0.));
#151370=CARTESIAN_POINT('Ctrl Pts',(-57.6531528802072,41.8983259415253,
0.));
#151371=CARTESIAN_POINT('Ctrl Pts',(-57.6399963769009,41.8800188342912,
0.));
#151372=CARTESIAN_POINT('Ctrl Pts',(-57.6268482595701,41.8617622748107,
0.));
#151373=CARTESIAN_POINT('Ctrl Pts',(-57.613708666588,41.8435563359456,0.));
#151374=CARTESIAN_POINT('Ctrl Pts',(-57.6005777370347,41.8254010908051,
0.));
#151375=CARTESIAN_POINT('Ctrl Pts',(-57.5874556107054,41.8072966127559,
0.));
#151376=CARTESIAN_POINT('Ctrl Pts',(-57.5743424281204,41.7892429754298,
0.));
#151377=CARTESIAN_POINT('Ctrl Pts',(-57.561238330532,41.7712402527273,0.));
#151378=CARTESIAN_POINT('Ctrl Pts',(-57.5481434599334,41.7532885188174,
0.));
#151379=CARTESIAN_POINT('Ctrl Pts',(-57.5350579590648,41.7353878481336,
0.));
#151380=CARTESIAN_POINT('Ctrl Pts',(-57.5219819714169,41.7175383153819,
0.));
#151381=CARTESIAN_POINT('Ctrl Pts',(-57.5089156412341,41.6997399955445,
0.));
#151382=CARTESIAN_POINT('Ctrl Pts',(-57.4958591135165,41.6819929638797,
0.));
#151383=CARTESIAN_POINT('Ctrl Pts',(-57.4828125340222,41.6642972959168,
0.));
#151384=CARTESIAN_POINT('Ctrl Pts',(-57.4697760492693,41.6466530674522,
0.));
#151385=CARTESIAN_POINT('Ctrl Pts',(-57.4567498065573,41.6290603545674,
0.));
#151386=CARTESIAN_POINT('Ctrl Pts',(-57.4437339539848,41.6115192336393,
0.));
#151387=CARTESIAN_POINT('Ctrl Pts',(-57.4307286404656,41.5940297813474,
0.));
#151388=CARTESIAN_POINT('Ctrl Pts',(-57.417734015749,41.5765920746764,0.));
#151389=CARTESIAN_POINT('Ctrl Pts',(-57.4047502304207,41.5592061909159,
0.));
#151390=CARTESIAN_POINT('Ctrl Pts',(-57.3917774358844,41.5418722076558,
0.));
#151391=CARTESIAN_POINT('Ctrl Pts',(-57.378815784345,41.5245902027767,0.));
#151392=CARTESIAN_POINT('Ctrl Pts',(-57.3658654287948,41.5073602544404,
0.));
#151393=CARTESIAN_POINT('Ctrl Pts',(-57.3529265229858,41.4901824410654,
0.));
#151394=CARTESIAN_POINT('Ctrl Pts',(-57.339999221474,41.4730568413535,0.));
#151395=CARTESIAN_POINT('Ctrl Pts',(-57.3270836796925,41.4559835343338,
0.));
#151396=CARTESIAN_POINT('Ctrl Pts',(-57.3141800540137,41.4389625993948,
0.));
#151397=CARTESIAN_POINT('Ctrl Pts',(-57.3012885018139,41.4219941163154,
0.));
#151398=CARTESIAN_POINT('Ctrl Pts',(-57.2884091815385,41.4050781652923,
0.));
#151399=CARTESIAN_POINT('Ctrl Pts',(-57.2755422525822,41.3882148268798,
0.));
#151400=CARTESIAN_POINT('Ctrl Pts',(-57.2626878751584,41.3714041819215,
0.));
#151401=CARTESIAN_POINT('Ctrl Pts',(-57.2498462101883,41.3546463114889,
0.));
#151402=CARTESIAN_POINT('Ctrl Pts',(-57.237017419142,41.3379412967889,0.));
#151403=CARTESIAN_POINT('Ctrl Pts',(-57.2242016640226,41.321289219151,0.));
#151404=CARTESIAN_POINT('Ctrl Pts',(-57.2113991077325,41.304690160231,0.));
#151405=CARTESIAN_POINT('Ctrl Pts',(-57.1986099143992,41.2881442021869,
0.));
#151406=CARTESIAN_POINT('Ctrl Pts',(-57.1858342496526,41.2716514278268,
0.));
#151407=CARTESIAN_POINT('Ctrl Pts',(-57.1730722810771,41.2552119208445,
0.));
#151408=CARTESIAN_POINT('Ctrl Pts',(-57.1603241779042,41.2388257656534,
0.));
#151409=CARTESIAN_POINT('Ctrl Pts',(-57.1475901101795,41.2224930469412,
0.));
#151410=CARTESIAN_POINT('Ctrl Pts',(-57.1348702480644,41.2062138492913,
0.));
#151411=CARTESIAN_POINT('Ctrl Pts',(-57.1221647611231,41.1899882567941,
0.));
#151412=CARTESIAN_POINT('Ctrl Pts',(-57.1094738174998,41.1738163525931,
0.));
#151413=CARTESIAN_POINT('Ctrl Pts',(-57.0967975854912,41.1576982197402,
0.));
#151414=CARTESIAN_POINT('Ctrl Pts',(-57.0841362354281,41.1416339422132,
0.));
#151415=CARTESIAN_POINT('Ctrl Pts',(-57.0714899412091,41.1256236057436,
0.));
#151416=CARTESIAN_POINT('Ctrl Pts',(-57.0588588825266,41.1096672990125,
0.));
#151417=CARTESIAN_POINT('Ctrl Pts',(-57.0462432450637,41.0937651137519,
0.));
#151418=CARTESIAN_POINT('Ctrl Pts',(-57.0336432158503,41.0779171422415,
0.));
#151419=CARTESIAN_POINT('Ctrl Pts',(-57.0210589791777,41.0621234751,0.));
#151420=CARTESIAN_POINT('Ctrl Pts',(-57.008490713044,41.0463841993622,0.));
#151421=CARTESIAN_POINT('Ctrl Pts',(-56.9959385834768,41.0306993954021,
0.));
#151422=CARTESIAN_POINT('Ctrl Pts',(-56.9834027500178,41.0150691398988,
0.));
#151423=CARTESIAN_POINT('Ctrl Pts',(-56.9708833766183,40.9994935117307,
0.));
#151424=CARTESIAN_POINT('Ctrl Pts',(-56.9583806404069,40.9839725967121,
0.));
#151425=CARTESIAN_POINT('Ctrl Pts',(-56.9458947422541,40.968506493303,0.));
#151426=CARTESIAN_POINT('Ctrl Pts',(-56.9334259139928,40.9530953164952,
0.));
#151427=CARTESIAN_POINT('Ctrl Pts',(-56.9209743960861,40.9377391857044,
0.));
#151428=CARTESIAN_POINT('Ctrl Pts',(-56.9085404164432,40.9224382132382,
0.));
#151429=CARTESIAN_POINT('Ctrl Pts',(-56.8961241708926,40.9071924937551,
0.));
#151430=CARTESIAN_POINT('Ctrl Pts',(-56.8837257978574,40.8920020903443,
0.));
#151431=CARTESIAN_POINT('Ctrl Pts',(-56.8713453765252,40.8768670342278,
0.));
#151432=CARTESIAN_POINT('Ctrl Pts',(-56.8614554317993,40.8648032759631,
0.));
#151433=CARTESIAN_POINT('Ctrl Pts',(-56.8540460739677,40.8557803680411,
0.));
#151434=CARTESIAN_POINT('Ctrl Pts',(-56.8491101022668,40.8497761671086,
0.));
#151435=CARTESIAN_POINT('Ctrl Pts',(-56.8466430164621,40.8467768343956,
0.));
#151436=CARTESIAN_POINT('Ctrl Pts',(-55.3473204966403,49.8690697110161,
0.));
#151437=CARTESIAN_POINT('Ctrl Pts',(-55.3473204966403,49.8690697110161,
12.));
#151438=CARTESIAN_POINT('Ctrl Pts',(-55.3451131058826,49.8639277221566,
0.));
#151439=CARTESIAN_POINT('Ctrl Pts',(-55.3451131058826,49.8639277221566,
12.));
#151440=CARTESIAN_POINT('Ctrl Pts',(-55.34069740326,49.8536479176833,0.));
#151441=CARTESIAN_POINT('Ctrl Pts',(-55.34069740326,49.8536479176833,12.));
#151442=CARTESIAN_POINT('Ctrl Pts',(-55.3340710860055,49.8382407307107,
0.));
#151443=CARTESIAN_POINT('Ctrl Pts',(-55.3340710860055,49.8382407307107,
12.));
#151444=CARTESIAN_POINT('Ctrl Pts',(-55.3252304694602,49.8177228552376,
0.));
#151445=CARTESIAN_POINT('Ctrl Pts',(-55.3252304694602,49.8177228552376,
12.));
#151446=CARTESIAN_POINT('Ctrl Pts',(-55.3141704897766,49.7921172540628,
0.));
#151447=CARTESIAN_POINT('Ctrl Pts',(-55.3141704897766,49.7921172540628,
12.));
#151448=CARTESIAN_POINT('Ctrl Pts',(-55.3031013105853,49.7665534128535,
0.));
#151449=CARTESIAN_POINT('Ctrl Pts',(-55.3031013105853,49.7665534128535,
12.));
#151450=CARTESIAN_POINT('Ctrl Pts',(-55.2920229527546,49.7410313576508,
0.));
#151451=CARTESIAN_POINT('Ctrl Pts',(-55.2920229527546,49.7410313576508,
12.));
#151452=CARTESIAN_POINT('Ctrl Pts',(-55.2809354521515,49.7155511248531,
0.));
#151453=CARTESIAN_POINT('Ctrl Pts',(-55.2809354521515,49.7155511248531,
12.));
#151454=CARTESIAN_POINT('Ctrl Pts',(-55.2698388650025,49.6901127631627,
0.));
#151455=CARTESIAN_POINT('Ctrl Pts',(-55.2698388650025,49.6901127631627,
12.));
#151456=CARTESIAN_POINT('Ctrl Pts',(-55.2587332663783,49.6647163322266,
0.));
#151457=CARTESIAN_POINT('Ctrl Pts',(-55.2587332663783,49.6647163322266,
12.));
#151458=CARTESIAN_POINT('Ctrl Pts',(-55.2476187434057,49.6393618987473,
0.));
#151459=CARTESIAN_POINT('Ctrl Pts',(-55.2476187434057,49.6393618987473,
12.));
#151460=CARTESIAN_POINT('Ctrl Pts',(-55.2364953899358,49.6140495332803,
0.));
#151461=CARTESIAN_POINT('Ctrl Pts',(-55.2364953899358,49.6140495332803,
12.));
#151462=CARTESIAN_POINT('Ctrl Pts',(-55.2253633007666,49.5887793068352,
0.));
#151463=CARTESIAN_POINT('Ctrl Pts',(-55.2253633007666,49.5887793068352,
12.));
#151464=CARTESIAN_POINT('Ctrl Pts',(-55.2142225657013,49.5635512873435,
0.));
#151465=CARTESIAN_POINT('Ctrl Pts',(-55.2142225657013,49.5635512873435,
12.));
#151466=CARTESIAN_POINT('Ctrl Pts',(-55.2030732647312,49.5383655368073,
0.));
#151467=CARTESIAN_POINT('Ctrl Pts',(-55.2030732647312,49.5383655368073,
12.));
#151468=CARTESIAN_POINT('Ctrl Pts',(-55.1919154713647,49.5132221132992,
0.));
#151469=CARTESIAN_POINT('Ctrl Pts',(-55.1919154713647,49.5132221132992,
12.));
#151470=CARTESIAN_POINT('Ctrl Pts',(-55.1807492550119,49.4881210723966,
0.));
#151471=CARTESIAN_POINT('Ctrl Pts',(-55.1807492550119,49.4881210723966,
12.));
#151472=CARTESIAN_POINT('Ctrl Pts',(-55.1695746838174,49.4630624688793,
0.));
#151473=CARTESIAN_POINT('Ctrl Pts',(-55.1695746838174,49.4630624688793,
12.));
#151474=CARTESIAN_POINT('Ctrl Pts',(-55.1583918271116,49.4380463581965,
0.));
#151475=CARTESIAN_POINT('Ctrl Pts',(-55.1583918271116,49.4380463581965,
12.));
#151476=CARTESIAN_POINT('Ctrl Pts',(-55.1472007585183,49.4130727983201,
0.));
#151477=CARTESIAN_POINT('Ctrl Pts',(-55.1472007585183,49.4130727983201,
12.));
#151478=CARTESIAN_POINT('Ctrl Pts',(-55.1360015556221,49.3881418495489,
0.));
#151479=CARTESIAN_POINT('Ctrl Pts',(-55.1360015556221,49.3881418495489,
12.));
#151480=CARTESIAN_POINT('Ctrl Pts',(-55.1247942985619,49.3632535736715,
0.));
#151481=CARTESIAN_POINT('Ctrl Pts',(-55.1247942985619,49.3632535736715,
12.));
#151482=CARTESIAN_POINT('Ctrl Pts',(-55.1135790689464,49.3384080333155,
0.));
#151483=CARTESIAN_POINT('Ctrl Pts',(-55.1135790689464,49.3384080333155,
12.));
#151484=CARTESIAN_POINT('Ctrl Pts',(-55.102355948714,49.3136052912621,0.));
#151485=CARTESIAN_POINT('Ctrl Pts',(-55.102355948714,49.3136052912621,12.));
#151486=CARTESIAN_POINT('Ctrl Pts',(-55.0911250188302,49.2888454096563,
0.));
#151487=CARTESIAN_POINT('Ctrl Pts',(-55.0911250188302,49.2888454096563,
12.));
#151488=CARTESIAN_POINT('Ctrl Pts',(-55.079886358701,49.264128449652,0.));
#151489=CARTESIAN_POINT('Ctrl Pts',(-55.079886358701,49.264128449652,12.));
#151490=CARTESIAN_POINT('Ctrl Pts',(-55.0686400468931,49.2394544718531,
0.));
#151491=CARTESIAN_POINT('Ctrl Pts',(-55.0686400468931,49.2394544718531,
12.));
#151492=CARTESIAN_POINT('Ctrl Pts',(-55.0573861615579,49.2148235365703,
0.));
#151493=CARTESIAN_POINT('Ctrl Pts',(-55.0573861615579,49.2148235365703,
12.));
#151494=CARTESIAN_POINT('Ctrl Pts',(-55.0461247809744,49.1902357041461,
0.));
#151495=CARTESIAN_POINT('Ctrl Pts',(-55.0461247809744,49.1902357041461,
12.));
#151496=CARTESIAN_POINT('Ctrl Pts',(-55.0348559840453,49.1656910352476,
0.));
#151497=CARTESIAN_POINT('Ctrl Pts',(-55.0348559840453,49.1656910352476,
12.));
#151498=CARTESIAN_POINT('Ctrl Pts',(-55.0235798508045,49.1411895911635,
0.));
#151499=CARTESIAN_POINT('Ctrl Pts',(-55.0235798508045,49.1411895911635,
12.));
#151500=CARTESIAN_POINT('Ctrl Pts',(-55.012296462186,49.116731433673,0.));
#151501=CARTESIAN_POINT('Ctrl Pts',(-55.012296462186,49.116731433673,12.));
#151502=CARTESIAN_POINT('Ctrl Pts',(-55.0010058998107,49.0923166249219,
0.));
#151503=CARTESIAN_POINT('Ctrl Pts',(-55.0010058998107,49.0923166249219,
12.));
#151504=CARTESIAN_POINT('Ctrl Pts',(-54.9897082457606,49.067945227287,0.));
#151505=CARTESIAN_POINT('Ctrl Pts',(-54.9897082457606,49.067945227287,12.));
#151506=CARTESIAN_POINT('Ctrl Pts',(-54.9784035823766,49.0436173032528,
0.));
#151507=CARTESIAN_POINT('Ctrl Pts',(-54.9784035823766,49.0436173032528,
12.));
#151508=CARTESIAN_POINT('Ctrl Pts',(-54.9670919920029,49.0193329152479,
0.));
#151509=CARTESIAN_POINT('Ctrl Pts',(-54.9670919920029,49.0193329152479,
12.));
#151510=CARTESIAN_POINT('Ctrl Pts',(-54.9557735569943,48.9950921256526,
0.));
#151511=CARTESIAN_POINT('Ctrl Pts',(-54.9557735569943,48.9950921256526,
12.));
#151512=CARTESIAN_POINT('Ctrl Pts',(-54.9444483598378,48.9708949968795,
0.));
#151513=CARTESIAN_POINT('Ctrl Pts',(-54.9444483598378,48.9708949968795,
12.));
#151514=CARTESIAN_POINT('Ctrl Pts',(-54.9331164832424,48.9467415914269,
0.));
#151515=CARTESIAN_POINT('Ctrl Pts',(-54.9331164832424,48.9467415914269,
12.));
#151516=CARTESIAN_POINT('Ctrl Pts',(-54.9217780102355,48.9226319719368,
0.));
#151517=CARTESIAN_POINT('Ctrl Pts',(-54.9217780102355,48.9226319719368,
12.));
#151518=CARTESIAN_POINT('Ctrl Pts',(-54.9104330242742,48.8985662012528,
0.));
#151519=CARTESIAN_POINT('Ctrl Pts',(-54.9104330242742,48.8985662012528,
12.));
#151520=CARTESIAN_POINT('Ctrl Pts',(-54.8990816092953,48.8745443424477,
0.));
#151521=CARTESIAN_POINT('Ctrl Pts',(-54.8990816092953,48.8745443424477,
12.));
#151522=CARTESIAN_POINT('Ctrl Pts',(-54.8877238496566,48.8505664587974,
0.));
#151523=CARTESIAN_POINT('Ctrl Pts',(-54.8877238496566,48.8505664587974,
12.));
#151524=CARTESIAN_POINT('Ctrl Pts',(-54.8763598301037,48.8266326137622,
0.));
#151525=CARTESIAN_POINT('Ctrl Pts',(-54.8763598301037,48.8266326137622,
12.));
#151526=CARTESIAN_POINT('Ctrl Pts',(-54.8649896357285,48.8027428709614,
0.));
#151527=CARTESIAN_POINT('Ctrl Pts',(-54.8649896357285,48.8027428709614,
12.));
#151528=CARTESIAN_POINT('Ctrl Pts',(-54.8536133519292,48.7788972941438,
0.));
#151529=CARTESIAN_POINT('Ctrl Pts',(-54.8536133519292,48.7788972941438,
12.));
#151530=CARTESIAN_POINT('Ctrl Pts',(-54.8422310643763,48.7550959471601,
0.));
#151531=CARTESIAN_POINT('Ctrl Pts',(-54.8422310643763,48.7550959471601,
12.));
#151532=CARTESIAN_POINT('Ctrl Pts',(-54.8308428590344,48.7313388939845,
0.));
#151533=CARTESIAN_POINT('Ctrl Pts',(-54.8308428590344,48.7313388939845,
12.));
#151534=CARTESIAN_POINT('Ctrl Pts',(-54.819448822181,48.7076261987292,0.));
#151535=CARTESIAN_POINT('Ctrl Pts',(-54.819448822181,48.7076261987292,12.));
#151536=CARTESIAN_POINT('Ctrl Pts',(-54.8080490404275,48.6839579256566,
0.));
#151537=CARTESIAN_POINT('Ctrl Pts',(-54.8080490404275,48.6839579256566,
12.));
#151538=CARTESIAN_POINT('Ctrl Pts',(-54.796643600739,48.6603341391886,0.));
#151539=CARTESIAN_POINT('Ctrl Pts',(-54.796643600739,48.6603341391886,12.));
#151540=CARTESIAN_POINT('Ctrl Pts',(-54.7852325904583,48.6367549039112,
0.));
#151541=CARTESIAN_POINT('Ctrl Pts',(-54.7852325904583,48.6367549039112,
12.));
#151542=CARTESIAN_POINT('Ctrl Pts',(-54.7738160973031,48.6132202845783,
0.));
#151543=CARTESIAN_POINT('Ctrl Pts',(-54.7738160973031,48.6132202845783,
12.));
#151544=CARTESIAN_POINT('Ctrl Pts',(-54.7623942093586,48.5897303461125,
0.));
#151545=CARTESIAN_POINT('Ctrl Pts',(-54.7623942093586,48.5897303461125,
12.));
#151546=CARTESIAN_POINT('Ctrl Pts',(-54.7509670150714,48.5662851536026,
0.));
#151547=CARTESIAN_POINT('Ctrl Pts',(-54.7509670150714,48.5662851536026,
12.));
#151548=CARTESIAN_POINT('Ctrl Pts',(-54.7395346032453,48.5428847722977,
0.));
#151549=CARTESIAN_POINT('Ctrl Pts',(-54.7395346032453,48.5428847722977,
12.));
#151550=CARTESIAN_POINT('Ctrl Pts',(-54.7280970630351,48.519529267596,0.));
#151551=CARTESIAN_POINT('Ctrl Pts',(-54.7280970630351,48.519529267596,12.));
#151552=CARTESIAN_POINT('Ctrl Pts',(-54.716654483948,48.4962187050457,0.));
#151553=CARTESIAN_POINT('Ctrl Pts',(-54.716654483948,48.4962187050457,12.));
#151554=CARTESIAN_POINT('Ctrl Pts',(-54.7052069558497,48.472953150357,0.));
#151555=CARTESIAN_POINT('Ctrl Pts',(-54.7052069558497,48.472953150357,12.));
#151556=CARTESIAN_POINT('Ctrl Pts',(-54.6937545689695,48.4497326694052,
0.));
#151557=CARTESIAN_POINT('Ctrl Pts',(-54.6937545689695,48.4497326694052,
12.));
#151558=CARTESIAN_POINT('Ctrl Pts',(-54.6822974139064,48.426557328234,0.));
#151559=CARTESIAN_POINT('Ctrl Pts',(-54.6822974139064,48.426557328234,12.));
#151560=CARTESIAN_POINT('Ctrl Pts',(-54.6708355816358,48.4034271930514,
0.));
#151561=CARTESIAN_POINT('Ctrl Pts',(-54.6708355816358,48.4034271930514,
12.));
#151562=CARTESIAN_POINT('Ctrl Pts',(-54.6593691635145,48.3803423302294,
0.));
#151563=CARTESIAN_POINT('Ctrl Pts',(-54.6593691635145,48.3803423302294,
12.));
#151564=CARTESIAN_POINT('Ctrl Pts',(-54.6478982512794,48.3573028063124,
0.));
#151565=CARTESIAN_POINT('Ctrl Pts',(-54.6478982512794,48.3573028063124,
12.));
#151566=CARTESIAN_POINT('Ctrl Pts',(-54.6364229370494,48.3343086880194,
0.));
#151567=CARTESIAN_POINT('Ctrl Pts',(-54.6364229370494,48.3343086880194,
12.));
#151568=CARTESIAN_POINT('Ctrl Pts',(-54.6249433133261,48.3113600422443,
0.));
#151569=CARTESIAN_POINT('Ctrl Pts',(-54.6249433133261,48.3113600422443,
12.));
#151570=CARTESIAN_POINT('Ctrl Pts',(-54.6134594729959,48.2884569360506,
0.));
#151571=CARTESIAN_POINT('Ctrl Pts',(-54.6134594729959,48.2884569360506,
12.));
#151572=CARTESIAN_POINT('Ctrl Pts',(-54.6019715093309,48.2655994366665,
0.));
#151573=CARTESIAN_POINT('Ctrl Pts',(-54.6019715093309,48.2655994366665,
12.));
#151574=CARTESIAN_POINT('Ctrl Pts',(-54.5904795159926,48.2427876114947,
0.));
#151575=CARTESIAN_POINT('Ctrl Pts',(-54.5904795159926,48.2427876114947,
12.));
#151576=CARTESIAN_POINT('Ctrl Pts',(-54.5789835870342,48.2200215281173,
0.));
#151577=CARTESIAN_POINT('Ctrl Pts',(-54.5789835870342,48.2200215281173,
12.));
#151578=CARTESIAN_POINT('Ctrl Pts',(-54.5674838169041,48.1973012542966,
0.));
#151579=CARTESIAN_POINT('Ctrl Pts',(-54.5674838169041,48.1973012542966,
12.));
#151580=CARTESIAN_POINT('Ctrl Pts',(-54.5559803004492,48.1746268579736,
0.));
#151581=CARTESIAN_POINT('Ctrl Pts',(-54.5559803004492,48.1746268579736,
12.));
#151582=CARTESIAN_POINT('Ctrl Pts',(-54.5444731329201,48.1519984072622,
0.));
#151583=CARTESIAN_POINT('Ctrl Pts',(-54.5444731329201,48.1519984072622,
12.));
#151584=CARTESIAN_POINT('Ctrl Pts',(-54.5329624099721,48.1294159704573,
0.));
#151585=CARTESIAN_POINT('Ctrl Pts',(-54.5329624099721,48.1294159704573,
12.));
#151586=CARTESIAN_POINT('Ctrl Pts',(-54.5214482276678,48.1068796160405,
0.));
#151587=CARTESIAN_POINT('Ctrl Pts',(-54.5214482276678,48.1068796160405,
12.));
#151588=CARTESIAN_POINT('Ctrl Pts',(-54.5099306824786,48.0843894126806,
0.));
#151589=CARTESIAN_POINT('Ctrl Pts',(-54.5099306824786,48.0843894126806,
12.));
#151590=CARTESIAN_POINT('Ctrl Pts',(-54.4984098712886,48.0619454292324,
0.));
#151591=CARTESIAN_POINT('Ctrl Pts',(-54.4984098712886,48.0619454292324,
12.));
#151592=CARTESIAN_POINT('Ctrl Pts',(-54.4868858913971,48.0395477347298,
0.));
#151593=CARTESIAN_POINT('Ctrl Pts',(-54.4868858913971,48.0395477347298,
12.));
#151594=CARTESIAN_POINT('Ctrl Pts',(-54.4753588405215,48.0171963983924,
0.));
#151595=CARTESIAN_POINT('Ctrl Pts',(-54.4753588405215,48.0171963983924,
12.));
#151596=CARTESIAN_POINT('Ctrl Pts',(-54.4638288168003,47.9948914896326,
0.));
#151597=CARTESIAN_POINT('Ctrl Pts',(-54.4638288168003,47.9948914896326,
12.));
#151598=CARTESIAN_POINT('Ctrl Pts',(-54.4522959187955,47.9726330780572,
0.));
#151599=CARTESIAN_POINT('Ctrl Pts',(-54.4522959187955,47.9726330780572,
12.));
#151600=CARTESIAN_POINT('Ctrl Pts',(-54.4407602454967,47.9504212334675,
0.));
#151601=CARTESIAN_POINT('Ctrl Pts',(-54.4407602454967,47.9504212334675,
12.));
#151602=CARTESIAN_POINT('Ctrl Pts',(-54.429221896324,47.9282560258516,0.));
#151603=CARTESIAN_POINT('Ctrl Pts',(-54.429221896324,47.9282560258516,12.));
#151604=CARTESIAN_POINT('Ctrl Pts',(-54.4176809711311,47.9061375253897,
0.));
#151605=CARTESIAN_POINT('Ctrl Pts',(-54.4176809711311,47.9061375253897,
12.));
#151606=CARTESIAN_POINT('Ctrl Pts',(-54.4061375702079,47.8840658024618,
0.));
#151607=CARTESIAN_POINT('Ctrl Pts',(-54.4061375702079,47.8840658024618,
12.));
#151608=CARTESIAN_POINT('Ctrl Pts',(-54.3945917942832,47.8620409276493,
0.));
#151609=CARTESIAN_POINT('Ctrl Pts',(-54.3945917942832,47.8620409276493,
12.));
#151610=CARTESIAN_POINT('Ctrl Pts',(-54.3830437445279,47.8400629717355,
0.));
#151611=CARTESIAN_POINT('Ctrl Pts',(-54.3830437445279,47.8400629717355,
12.));
#151612=CARTESIAN_POINT('Ctrl Pts',(-54.3714935225591,47.8181320056995,
0.));
#151613=CARTESIAN_POINT('Ctrl Pts',(-54.3714935225591,47.8181320056995,
12.));
#151614=CARTESIAN_POINT('Ctrl Pts',(-54.3599412304437,47.7962481007185,
0.));
#151615=CARTESIAN_POINT('Ctrl Pts',(-54.3599412304437,47.7962481007185,
12.));
#151616=CARTESIAN_POINT('Ctrl Pts',(-54.3483869707002,47.7744113281771,
0.));
#151617=CARTESIAN_POINT('Ctrl Pts',(-54.3483869707002,47.7744113281771,
12.));
#151618=CARTESIAN_POINT('Ctrl Pts',(-54.3368308463023,47.7526217596694,
0.));
#151619=CARTESIAN_POINT('Ctrl Pts',(-54.3368308463023,47.7526217596694,
12.));
#151620=CARTESIAN_POINT('Ctrl Pts',(-54.3252729606823,47.7308794669993,
0.));
#151621=CARTESIAN_POINT('Ctrl Pts',(-54.3252729606823,47.7308794669993,
12.));
#151622=CARTESIAN_POINT('Ctrl Pts',(-54.3137134177345,47.7091845221747,
0.));
#151623=CARTESIAN_POINT('Ctrl Pts',(-54.3137134177345,47.7091845221747,
12.));
#151624=CARTESIAN_POINT('Ctrl Pts',(-54.302152321819,47.6875369974087,0.));
#151625=CARTESIAN_POINT('Ctrl Pts',(-54.302152321819,47.6875369974087,12.));
#151626=CARTESIAN_POINT('Ctrl Pts',(-54.290589777765,47.6659369651301,0.));
#151627=CARTESIAN_POINT('Ctrl Pts',(-54.290589777765,47.6659369651301,12.));
#151628=CARTESIAN_POINT('Ctrl Pts',(-54.2790258908738,47.6443844979847,
0.));
#151629=CARTESIAN_POINT('Ctrl Pts',(-54.2790258908738,47.6443844979847,
12.));
#151630=CARTESIAN_POINT('Ctrl Pts',(-54.2674607669226,47.6228796688375,
0.));
#151631=CARTESIAN_POINT('Ctrl Pts',(-54.2674607669226,47.6228796688375,
12.));
#151632=CARTESIAN_POINT('Ctrl Pts',(-54.2558945121678,47.6014225507659,
0.));
#151633=CARTESIAN_POINT('Ctrl Pts',(-54.2558945121678,47.6014225507659,
12.));
#151634=CARTESIAN_POINT('Ctrl Pts',(-54.244327233349,47.5800132170608,0.));
#151635=CARTESIAN_POINT('Ctrl Pts',(-54.244327233349,47.5800132170608,12.));
#151636=CARTESIAN_POINT('Ctrl Pts',(-54.2327590376924,47.5586517412363,
0.));
#151637=CARTESIAN_POINT('Ctrl Pts',(-54.2327590376924,47.5586517412363,
12.));
#151638=CARTESIAN_POINT('Ctrl Pts',(-54.2211900329138,47.5373381970326,
0.));
#151639=CARTESIAN_POINT('Ctrl Pts',(-54.2211900329138,47.5373381970326,
12.));
#151640=CARTESIAN_POINT('Ctrl Pts',(-54.209620327223,47.5160726584174,0.));
#151641=CARTESIAN_POINT('Ctrl Pts',(-54.209620327223,47.5160726584174,12.));
#151642=CARTESIAN_POINT('Ctrl Pts',(-54.198050029327,47.4948551995801,0.));
#151643=CARTESIAN_POINT('Ctrl Pts',(-54.198050029327,47.4948551995801,12.));
#151644=CARTESIAN_POINT('Ctrl Pts',(-54.1864792484345,47.4736858949322,
0.));
#151645=CARTESIAN_POINT('Ctrl Pts',(-54.1864792484345,47.4736858949322,
12.));
#151646=CARTESIAN_POINT('Ctrl Pts',(-54.1749080942593,47.4525648191173,
0.));
#151647=CARTESIAN_POINT('Ctrl Pts',(-54.1749080942593,47.4525648191173,
12.));
#151648=CARTESIAN_POINT('Ctrl Pts',(-54.1633366770239,47.4314920470141,
0.));
#151649=CARTESIAN_POINT('Ctrl Pts',(-54.1633366770239,47.4314920470141,
12.));
#151650=CARTESIAN_POINT('Ctrl Pts',(-54.1517651074637,47.4104676537381,
0.));
#151651=CARTESIAN_POINT('Ctrl Pts',(-54.1517651074637,47.4104676537381,
12.));
#151652=CARTESIAN_POINT('Ctrl Pts',(-54.1401934968311,47.3894917146365,
0.));
#151653=CARTESIAN_POINT('Ctrl Pts',(-54.1401934968311,47.3894917146365,
12.));
#151654=CARTESIAN_POINT('Ctrl Pts',(-54.1286219568989,47.3685643052874,
0.));
#151655=CARTESIAN_POINT('Ctrl Pts',(-54.1286219568989,47.3685643052874,
12.));
#151656=CARTESIAN_POINT('Ctrl Pts',(-54.1170505999645,47.3476855015102,
0.));
#151657=CARTESIAN_POINT('Ctrl Pts',(-54.1170505999645,47.3476855015102,
12.));
#151658=CARTESIAN_POINT('Ctrl Pts',(-54.1054795388543,47.3268553793694,
0.));
#151659=CARTESIAN_POINT('Ctrl Pts',(-54.1054795388543,47.3268553793694,
12.));
#151660=CARTESIAN_POINT('Ctrl Pts',(-54.0939088869269,47.3060740151752,
0.));
#151661=CARTESIAN_POINT('Ctrl Pts',(-54.0939088869269,47.3060740151752,
12.));
#151662=CARTESIAN_POINT('Ctrl Pts',(-54.0823387580776,47.2853414854793,
0.));
#151663=CARTESIAN_POINT('Ctrl Pts',(-54.0823387580776,47.2853414854793,
12.));
#151664=CARTESIAN_POINT('Ctrl Pts',(-54.0707692667438,47.2646578670746,
0.));
#151665=CARTESIAN_POINT('Ctrl Pts',(-54.0707692667438,47.2646578670746,
12.));
#151666=CARTESIAN_POINT('Ctrl Pts',(-54.0592005279086,47.2440232370065,
0.));
#151667=CARTESIAN_POINT('Ctrl Pts',(-54.0592005279086,47.2440232370065,
12.));
#151668=CARTESIAN_POINT('Ctrl Pts',(-54.047632657104,47.2234376725743,0.));
#151669=CARTESIAN_POINT('Ctrl Pts',(-54.047632657104,47.2234376725743,12.));
#151670=CARTESIAN_POINT('Ctrl Pts',(-54.0360657704163,47.202901251334,0.));
#151671=CARTESIAN_POINT('Ctrl Pts',(-54.0360657704163,47.202901251334,12.));
#151672=CARTESIAN_POINT('Ctrl Pts',(-54.0244999844893,47.1824140510926,
0.));
#151673=CARTESIAN_POINT('Ctrl Pts',(-54.0244999844893,47.1824140510926,
12.));
#151674=CARTESIAN_POINT('Ctrl Pts',(-54.0129354165297,47.1619761499087,
0.));
#151675=CARTESIAN_POINT('Ctrl Pts',(-54.0129354165297,47.1619761499087,
12.));
#151676=CARTESIAN_POINT('Ctrl Pts',(-54.0013721843118,47.1415876261035,
0.));
#151677=CARTESIAN_POINT('Ctrl Pts',(-54.0013721843118,47.1415876261035,
12.));
#151678=CARTESIAN_POINT('Ctrl Pts',(-53.989810406182,47.1212485582643,0.));
#151679=CARTESIAN_POINT('Ctrl Pts',(-53.989810406182,47.1212485582643,12.));
#151680=CARTESIAN_POINT('Ctrl Pts',(-53.9782502010634,47.1009590252458,
0.));
#151681=CARTESIAN_POINT('Ctrl Pts',(-53.9782502010634,47.1009590252458,
12.));
#151682=CARTESIAN_POINT('Ctrl Pts',(-53.9666916884596,47.0807191061648,
0.));
#151683=CARTESIAN_POINT('Ctrl Pts',(-53.9666916884596,47.0807191061648,
12.));
#151684=CARTESIAN_POINT('Ctrl Pts',(-53.95513498846,47.0605288804008,0.));
#151685=CARTESIAN_POINT('Ctrl Pts',(-53.95513498846,47.0605288804008,12.));
#151686=CARTESIAN_POINT('Ctrl Pts',(-53.9435802217436,47.0403884276071,
0.));
#151687=CARTESIAN_POINT('Ctrl Pts',(-53.9435802217436,47.0403884276071,
12.));
#151688=CARTESIAN_POINT('Ctrl Pts',(-53.9320275095853,47.0202978277138,
0.));
#151689=CARTESIAN_POINT('Ctrl Pts',(-53.9320275095853,47.0202978277138,
12.));
#151690=CARTESIAN_POINT('Ctrl Pts',(-53.9204769738596,47.0002571609297,
0.));
#151691=CARTESIAN_POINT('Ctrl Pts',(-53.9204769738596,47.0002571609297,
12.));
#151692=CARTESIAN_POINT('Ctrl Pts',(-53.9089287370463,46.9802665077366,
0.));
#151693=CARTESIAN_POINT('Ctrl Pts',(-53.9089287370463,46.9802665077366,
12.));
#151694=CARTESIAN_POINT('Ctrl Pts',(-53.8973829222348,46.960325948892,0.));
#151695=CARTESIAN_POINT('Ctrl Pts',(-53.8973829222348,46.960325948892,12.));
#151696=CARTESIAN_POINT('Ctrl Pts',(-53.8858396531298,46.94043556544,0.));
#151697=CARTESIAN_POINT('Ctrl Pts',(-53.8858396531298,46.94043556544,12.));
#151698=CARTESIAN_POINT('Ctrl Pts',(-53.8742990540563,46.9205954387133,
0.));
#151699=CARTESIAN_POINT('Ctrl Pts',(-53.8742990540563,46.9205954387133,
12.));
#151700=CARTESIAN_POINT('Ctrl Pts',(-53.8627612499638,46.9008056503351,
0.));
#151701=CARTESIAN_POINT('Ctrl Pts',(-53.8627612499638,46.9008056503351,
12.));
#151702=CARTESIAN_POINT('Ctrl Pts',(-53.8512263664321,46.881066282213,0.));
#151703=CARTESIAN_POINT('Ctrl Pts',(-53.8512263664321,46.881066282213,12.));
#151704=CARTESIAN_POINT('Ctrl Pts',(-53.8396945296757,46.8613774165435,
0.));
#151705=CARTESIAN_POINT('Ctrl Pts',(-53.8396945296757,46.8613774165435,
12.));
#151706=CARTESIAN_POINT('Ctrl Pts',(-53.8281658665503,46.841739135822,0.));
#151707=CARTESIAN_POINT('Ctrl Pts',(-53.8281658665503,46.841739135822,12.));
#151708=CARTESIAN_POINT('Ctrl Pts',(-53.816640504558,46.8221515228457,0.));
#151709=CARTESIAN_POINT('Ctrl Pts',(-53.816640504558,46.8221515228457,12.));
#151710=CARTESIAN_POINT('Ctrl Pts',(-53.8051185718532,46.802614660715,0.));
#151711=CARTESIAN_POINT('Ctrl Pts',(-53.8051185718532,46.802614660715,12.));
#151712=CARTESIAN_POINT('Ctrl Pts',(-53.793600197248,46.7831286328278,0.));
#151713=CARTESIAN_POINT('Ctrl Pts',(-53.793600197248,46.7831286328278,12.));
#151714=CARTESIAN_POINT('Ctrl Pts',(-53.7820855102182,46.763693522886,0.));
#151715=CARTESIAN_POINT('Ctrl Pts',(-53.7820855102182,46.763693522886,12.));
#151716=CARTESIAN_POINT('Ctrl Pts',(-53.7705746409076,46.7443094149045,
0.));
#151717=CARTESIAN_POINT('Ctrl Pts',(-53.7705746409076,46.7443094149045,
12.));
#151718=CARTESIAN_POINT('Ctrl Pts',(-53.7590677201342,46.7249763932129,
0.));
#151719=CARTESIAN_POINT('Ctrl Pts',(-53.7590677201342,46.7249763932129,
12.));
#151720=CARTESIAN_POINT('Ctrl Pts',(-53.7475648793946,46.7056945424559,
0.));
#151721=CARTESIAN_POINT('Ctrl Pts',(-53.7475648793946,46.7056945424559,
12.));
#151722=CARTESIAN_POINT('Ctrl Pts',(-53.7360662508675,46.6864639475862,
0.));
#151723=CARTESIAN_POINT('Ctrl Pts',(-53.7360662508675,46.6864639475862,
12.));
#151724=CARTESIAN_POINT('Ctrl Pts',(-53.7245719674221,46.6672846938752,
0.));
#151725=CARTESIAN_POINT('Ctrl Pts',(-53.7245719674221,46.6672846938752,
12.));
#151726=CARTESIAN_POINT('Ctrl Pts',(-53.7130821626262,46.6481568669217,
0.));
#151727=CARTESIAN_POINT('Ctrl Pts',(-53.7130821626262,46.6481568669217,
12.));
#151728=CARTESIAN_POINT('Ctrl Pts',(-53.7015969707541,46.6290805526559,
0.));
#151729=CARTESIAN_POINT('Ctrl Pts',(-53.7015969707541,46.6290805526559,
12.));
#151730=CARTESIAN_POINT('Ctrl Pts',(-53.690116526794,46.6100558373401,0.));
#151731=CARTESIAN_POINT('Ctrl Pts',(-53.690116526794,46.6100558373401,12.));
#151732=CARTESIAN_POINT('Ctrl Pts',(-53.678640966456,46.5910828075652,0.));
#151733=CARTESIAN_POINT('Ctrl Pts',(-53.678640966456,46.5910828075652,12.));
#151734=CARTESIAN_POINT('Ctrl Pts',(-53.6671704261735,46.5721615502589,
0.));
#151735=CARTESIAN_POINT('Ctrl Pts',(-53.6671704261735,46.5721615502589,
12.));
#151736=CARTESIAN_POINT('Ctrl Pts',(-53.6557050431069,46.5532921526899,
0.));
#151737=CARTESIAN_POINT('Ctrl Pts',(-53.6557050431069,46.5532921526899,
12.));
#151738=CARTESIAN_POINT('Ctrl Pts',(-53.6442449551455,46.5344747024677,
0.));
#151739=CARTESIAN_POINT('Ctrl Pts',(-53.6442449551455,46.5344747024677,
12.));
#151740=CARTESIAN_POINT('Ctrl Pts',(-53.6327903009098,46.5157092875377,
0.));
#151741=CARTESIAN_POINT('Ctrl Pts',(-53.6327903009098,46.5157092875377,
12.));
#151742=CARTESIAN_POINT('Ctrl Pts',(-53.6213412197542,46.4969959961779,
0.));
#151743=CARTESIAN_POINT('Ctrl Pts',(-53.6213412197542,46.4969959961779,
12.));
#151744=CARTESIAN_POINT('Ctrl Pts',(-53.6098978517869,46.4783349170182,
0.));
#151745=CARTESIAN_POINT('Ctrl Pts',(-53.6098978517869,46.4783349170182,
12.));
#151746=CARTESIAN_POINT('Ctrl Pts',(-53.5984603378862,46.4597261390526,
0.));
#151747=CARTESIAN_POINT('Ctrl Pts',(-53.5984603378862,46.4597261390526,
12.));
#151748=CARTESIAN_POINT('Ctrl Pts',(-53.5870288197161,46.4411697516474,
0.));
#151749=CARTESIAN_POINT('Ctrl Pts',(-53.5870288197161,46.4411697516474,
12.));
#151750=CARTESIAN_POINT('Ctrl Pts',(-53.5756034397464,46.422665844546,0.));
#151751=CARTESIAN_POINT('Ctrl Pts',(-53.5756034397464,46.422665844546,12.));
#151752=CARTESIAN_POINT('Ctrl Pts',(-53.5641843412537,46.4042145078682,
0.));
#151753=CARTESIAN_POINT('Ctrl Pts',(-53.5641843412537,46.4042145078682,
12.));
#151754=CARTESIAN_POINT('Ctrl Pts',(-53.552771668303,46.3858158321044,0.));
#151755=CARTESIAN_POINT('Ctrl Pts',(-53.552771668303,46.3858158321044,12.));
#151756=CARTESIAN_POINT('Ctrl Pts',(-53.5413655657323,46.3674699081043,
0.));
#151757=CARTESIAN_POINT('Ctrl Pts',(-53.5413655657323,46.3674699081043,
12.));
#151758=CARTESIAN_POINT('Ctrl Pts',(-53.5299661791396,46.3491768270664,
0.));
#151759=CARTESIAN_POINT('Ctrl Pts',(-53.5299661791396,46.3491768270664,
12.));
#151760=CARTESIAN_POINT('Ctrl Pts',(-53.518573654857,46.3309366805112,0.));
#151761=CARTESIAN_POINT('Ctrl Pts',(-53.518573654857,46.3309366805112,12.));
#151762=CARTESIAN_POINT('Ctrl Pts',(-53.5071881399932,46.3127495603117,
0.));
#151763=CARTESIAN_POINT('Ctrl Pts',(-53.5071881399932,46.3127495603117,
12.));
#151764=CARTESIAN_POINT('Ctrl Pts',(-53.4958097825019,46.2946155587428,
0.));
#151765=CARTESIAN_POINT('Ctrl Pts',(-53.4958097825019,46.2946155587428,
12.));
#151766=CARTESIAN_POINT('Ctrl Pts',(-53.4844387312414,46.2765347685198,
0.));
#151767=CARTESIAN_POINT('Ctrl Pts',(-53.4844387312414,46.2765347685198,
12.));
#151768=CARTESIAN_POINT('Ctrl Pts',(-53.4730751360359,46.2585072828343,
0.));
#151769=CARTESIAN_POINT('Ctrl Pts',(-53.4730751360359,46.2585072828343,
12.));
#151770=CARTESIAN_POINT('Ctrl Pts',(-53.4617191477382,46.2405331953872,
0.));
#151771=CARTESIAN_POINT('Ctrl Pts',(-53.4617191477382,46.2405331953872,
12.));
#151772=CARTESIAN_POINT('Ctrl Pts',(-53.4503709181158,46.2226126003185,
0.));
#151773=CARTESIAN_POINT('Ctrl Pts',(-53.4503709181158,46.2226126003185,
12.));
#151774=CARTESIAN_POINT('Ctrl Pts',(-53.4390305997263,46.2047455921276,
0.));
#151775=CARTESIAN_POINT('Ctrl Pts',(-53.4390305997263,46.2047455921276,
12.));
#151776=CARTESIAN_POINT('Ctrl Pts',(-53.4276983458129,46.1869322656027,
0.));
#151777=CARTESIAN_POINT('Ctrl Pts',(-53.4276983458129,46.1869322656027,
12.));
#151778=CARTESIAN_POINT('Ctrl Pts',(-53.4163743101535,46.1691727157149,
0.));
#151779=CARTESIAN_POINT('Ctrl Pts',(-53.4163743101535,46.1691727157149,
12.));
#151780=CARTESIAN_POINT('Ctrl Pts',(-53.4050586470463,46.1514670376035,
0.));
#151781=CARTESIAN_POINT('Ctrl Pts',(-53.4050586470463,46.1514670376035,
12.));
#151782=CARTESIAN_POINT('Ctrl Pts',(-53.3937515116572,46.1338153268116,
0.));
#151783=CARTESIAN_POINT('Ctrl Pts',(-53.3937515116572,46.1338153268116,
12.));
#151784=CARTESIAN_POINT('Ctrl Pts',(-53.3824530603284,46.1162176794891,
0.));
#151785=CARTESIAN_POINT('Ctrl Pts',(-53.3824530603284,46.1162176794891,
12.));
#151786=CARTESIAN_POINT('Ctrl Pts',(-53.3711634508426,46.0986741925646,
0.));
#151787=CARTESIAN_POINT('Ctrl Pts',(-53.3711634508426,46.0986741925646,
12.));
#151788=CARTESIAN_POINT('Ctrl Pts',(-53.3598828428519,46.0811849640195,
0.));
#151789=CARTESIAN_POINT('Ctrl Pts',(-53.3598828428519,46.0811849640195,
12.));
#151790=CARTESIAN_POINT('Ctrl Pts',(-53.3486113975868,46.0637500926954,
0.));
#151791=CARTESIAN_POINT('Ctrl Pts',(-53.3486113975868,46.0637500926954,
12.));
#151792=CARTESIAN_POINT('Ctrl Pts',(-53.3373492770647,46.046369677778,0.));
#151793=CARTESIAN_POINT('Ctrl Pts',(-53.3373492770647,46.046369677778,12.));
#151794=CARTESIAN_POINT('Ctrl Pts',(-53.3260966434277,46.0290438183598,
0.));
#151795=CARTESIAN_POINT('Ctrl Pts',(-53.3260966434277,46.0290438183598,
12.));
#151796=CARTESIAN_POINT('Ctrl Pts',(-53.3148536582658,46.0117726129893,
0.));
#151797=CARTESIAN_POINT('Ctrl Pts',(-53.3148536582658,46.0117726129893,
12.));
#151798=CARTESIAN_POINT('Ctrl Pts',(-53.3036204818367,45.9945561591486,
0.));
#151799=CARTESIAN_POINT('Ctrl Pts',(-53.3036204818367,45.9945561591486,
12.));
#151800=CARTESIAN_POINT('Ctrl Pts',(-53.2923972745585,45.9773945542415,
0.));
#151801=CARTESIAN_POINT('Ctrl Pts',(-53.2923972745585,45.9773945542415,
12.));
#151802=CARTESIAN_POINT('Ctrl Pts',(-53.2811841987945,45.9602878967714,
0.));
#151803=CARTESIAN_POINT('Ctrl Pts',(-53.2811841987945,45.9602878967714,
12.));
#151804=CARTESIAN_POINT('Ctrl Pts',(-53.2699814203097,45.9432362873001,
0.));
#151805=CARTESIAN_POINT('Ctrl Pts',(-53.2699814203097,45.9432362873001,
12.));
#151806=CARTESIAN_POINT('Ctrl Pts',(-53.2587891103835,45.9262398298323,
0.));
#151807=CARTESIAN_POINT('Ctrl Pts',(-53.2587891103835,45.9262398298323,
12.));
#151808=CARTESIAN_POINT('Ctrl Pts',(-53.2476074459977,45.9092986319343,
0.));
#151809=CARTESIAN_POINT('Ctrl Pts',(-53.2476074459977,45.9092986319343,
12.));
#151810=CARTESIAN_POINT('Ctrl Pts',(-53.2364366054276,45.8924128018354,
0.));
#151811=CARTESIAN_POINT('Ctrl Pts',(-53.2364366054276,45.8924128018354,
12.));
#151812=CARTESIAN_POINT('Ctrl Pts',(-53.2252767643652,45.8755824458715,
0.));
#151813=CARTESIAN_POINT('Ctrl Pts',(-53.2252767643652,45.8755824458715,
12.));
#151814=CARTESIAN_POINT('Ctrl Pts',(-53.2141280925458,45.8588076662598,
0.));
#151815=CARTESIAN_POINT('Ctrl Pts',(-53.2141280925458,45.8588076662598,
12.));
#151816=CARTESIAN_POINT('Ctrl Pts',(-53.2029907483602,45.8420885575386,
0.));
#151817=CARTESIAN_POINT('Ctrl Pts',(-53.2029907483602,45.8420885575386,
12.));
#151818=CARTESIAN_POINT('Ctrl Pts',(-53.1918648840598,45.8254252100003,
0.));
#151819=CARTESIAN_POINT('Ctrl Pts',(-53.1918648840598,45.8254252100003,
12.));
#151820=CARTESIAN_POINT('Ctrl Pts',(-53.1807506560977,45.8088177165124,
0.));
#151821=CARTESIAN_POINT('Ctrl Pts',(-53.1807506560977,45.8088177165124,
12.));
#151822=CARTESIAN_POINT('Ctrl Pts',(-53.1696482334487,45.7922661780005,
0.));
#151823=CARTESIAN_POINT('Ctrl Pts',(-53.1696482334487,45.7922661780005,
12.));
#151824=CARTESIAN_POINT('Ctrl Pts',(-53.158557807638,45.7757707100568,0.));
#151825=CARTESIAN_POINT('Ctrl Pts',(-53.158557807638,45.7757707100568,12.));
#151826=CARTESIAN_POINT('Ctrl Pts',(-53.147479599594,45.7593314474412,0.));
#151827=CARTESIAN_POINT('Ctrl Pts',(-53.147479599594,45.7593314474412,12.));
#151828=CARTESIAN_POINT('Ctrl Pts',(-53.136413838457,45.7429485300727,0.));
#151829=CARTESIAN_POINT('Ctrl Pts',(-53.136413838457,45.7429485300727,12.));
#151830=CARTESIAN_POINT('Ctrl Pts',(-53.1253607414806,45.7266220896951,
0.));
#151831=CARTESIAN_POINT('Ctrl Pts',(-53.1253607414806,45.7266220896951,
12.));
#151832=CARTESIAN_POINT('Ctrl Pts',(-53.1143204954981,45.7103522376744,
0.));
#151833=CARTESIAN_POINT('Ctrl Pts',(-53.1143204954981,45.7103522376744,
12.));
#151834=CARTESIAN_POINT('Ctrl Pts',(-53.1032932329074,45.6941390489239,
0.));
#151835=CARTESIAN_POINT('Ctrl Pts',(-53.1032932329074,45.6941390489239,
12.));
#151836=CARTESIAN_POINT('Ctrl Pts',(-53.0922790298736,45.6779825614486,
0.));
#151837=CARTESIAN_POINT('Ctrl Pts',(-53.0922790298736,45.6779825614486,
12.));
#151838=CARTESIAN_POINT('Ctrl Pts',(-53.083478145185,45.6651027439479,0.));
#151839=CARTESIAN_POINT('Ctrl Pts',(-53.083478145185,45.6651027439479,12.));
#151840=CARTESIAN_POINT('Ctrl Pts',(-53.0768833804386,45.6554684028296,
0.));
#151841=CARTESIAN_POINT('Ctrl Pts',(-53.0768833804386,45.6554684028296,
12.));
#151842=CARTESIAN_POINT('Ctrl Pts',(-53.0724894921921,45.6490568514146,
0.));
#151843=CARTESIAN_POINT('Ctrl Pts',(-53.0724894921921,45.6490568514146,
12.));
#151844=CARTESIAN_POINT('Ctrl Pts',(-53.0702932034641,45.6458539113724,
0.));
#151845=CARTESIAN_POINT('Ctrl Pts',(-53.0702932034641,45.6458539113724,
12.));
#151846=CARTESIAN_POINT('',(-53.0702932034641,45.6458539113724,12.));
#151847=CARTESIAN_POINT('Ctrl Pts',(-53.0702932034641,45.6458539113724,
12.));
#151848=CARTESIAN_POINT('Ctrl Pts',(-53.0724894921921,45.6490568514146,
12.));
#151849=CARTESIAN_POINT('Ctrl Pts',(-53.0768833804386,45.6554684028296,
12.));
#151850=CARTESIAN_POINT('Ctrl Pts',(-53.083478145185,45.6651027439479,12.));
#151851=CARTESIAN_POINT('Ctrl Pts',(-53.0922790298736,45.6779825614486,
12.));
#151852=CARTESIAN_POINT('Ctrl Pts',(-53.1032932329074,45.6941390489239,
12.));
#151853=CARTESIAN_POINT('Ctrl Pts',(-53.1143204954981,45.7103522376744,
12.));
#151854=CARTESIAN_POINT('Ctrl Pts',(-53.1253607414806,45.7266220896951,
12.));
#151855=CARTESIAN_POINT('Ctrl Pts',(-53.136413838457,45.7429485300727,12.));
#151856=CARTESIAN_POINT('Ctrl Pts',(-53.147479599594,45.7593314474412,12.));
#151857=CARTESIAN_POINT('Ctrl Pts',(-53.158557807638,45.7757707100568,12.));
#151858=CARTESIAN_POINT('Ctrl Pts',(-53.1696482334487,45.7922661780005,
12.));
#151859=CARTESIAN_POINT('Ctrl Pts',(-53.1807506560977,45.8088177165124,
12.));
#151860=CARTESIAN_POINT('Ctrl Pts',(-53.1918648840598,45.8254252100003,
12.));
#151861=CARTESIAN_POINT('Ctrl Pts',(-53.2029907483602,45.8420885575386,
12.));
#151862=CARTESIAN_POINT('Ctrl Pts',(-53.2141280925458,45.8588076662598,
12.));
#151863=CARTESIAN_POINT('Ctrl Pts',(-53.2252767643652,45.8755824458715,
12.));
#151864=CARTESIAN_POINT('Ctrl Pts',(-53.2364366054276,45.8924128018354,
12.));
#151865=CARTESIAN_POINT('Ctrl Pts',(-53.2476074459977,45.9092986319343,
12.));
#151866=CARTESIAN_POINT('Ctrl Pts',(-53.2587891103835,45.9262398298323,
12.));
#151867=CARTESIAN_POINT('Ctrl Pts',(-53.2699814203097,45.9432362873001,
12.));
#151868=CARTESIAN_POINT('Ctrl Pts',(-53.2811841987945,45.9602878967714,
12.));
#151869=CARTESIAN_POINT('Ctrl Pts',(-53.2923972745585,45.9773945542415,
12.));
#151870=CARTESIAN_POINT('Ctrl Pts',(-53.3036204818367,45.9945561591486,
12.));
#151871=CARTESIAN_POINT('Ctrl Pts',(-53.3148536582658,46.0117726129893,
12.));
#151872=CARTESIAN_POINT('Ctrl Pts',(-53.3260966434277,46.0290438183598,
12.));
#151873=CARTESIAN_POINT('Ctrl Pts',(-53.3373492770647,46.046369677778,12.));
#151874=CARTESIAN_POINT('Ctrl Pts',(-53.3486113975868,46.0637500926954,
12.));
#151875=CARTESIAN_POINT('Ctrl Pts',(-53.3598828428519,46.0811849640195,
12.));
#151876=CARTESIAN_POINT('Ctrl Pts',(-53.3711634508426,46.0986741925646,
12.));
#151877=CARTESIAN_POINT('Ctrl Pts',(-53.3824530603284,46.1162176794891,
12.));
#151878=CARTESIAN_POINT('Ctrl Pts',(-53.3937515116572,46.1338153268116,
12.));
#151879=CARTESIAN_POINT('Ctrl Pts',(-53.4050586470463,46.1514670376035,
12.));
#151880=CARTESIAN_POINT('Ctrl Pts',(-53.4163743101535,46.1691727157149,
12.));
#151881=CARTESIAN_POINT('Ctrl Pts',(-53.4276983458129,46.1869322656027,
12.));
#151882=CARTESIAN_POINT('Ctrl Pts',(-53.4390305997263,46.2047455921276,
12.));
#151883=CARTESIAN_POINT('Ctrl Pts',(-53.4503709181158,46.2226126003185,
12.));
#151884=CARTESIAN_POINT('Ctrl Pts',(-53.4617191477382,46.2405331953872,
12.));
#151885=CARTESIAN_POINT('Ctrl Pts',(-53.4730751360359,46.2585072828343,
12.));
#151886=CARTESIAN_POINT('Ctrl Pts',(-53.4844387312414,46.2765347685198,
12.));
#151887=CARTESIAN_POINT('Ctrl Pts',(-53.4958097825019,46.2946155587428,
12.));
#151888=CARTESIAN_POINT('Ctrl Pts',(-53.5071881399932,46.3127495603117,
12.));
#151889=CARTESIAN_POINT('Ctrl Pts',(-53.518573654857,46.3309366805112,12.));
#151890=CARTESIAN_POINT('Ctrl Pts',(-53.5299661791396,46.3491768270664,
12.));
#151891=CARTESIAN_POINT('Ctrl Pts',(-53.5413655657323,46.3674699081043,
12.));
#151892=CARTESIAN_POINT('Ctrl Pts',(-53.552771668303,46.3858158321044,12.));
#151893=CARTESIAN_POINT('Ctrl Pts',(-53.5641843412537,46.4042145078682,
12.));
#151894=CARTESIAN_POINT('Ctrl Pts',(-53.5756034397464,46.422665844546,12.));
#151895=CARTESIAN_POINT('Ctrl Pts',(-53.5870288197161,46.4411697516474,
12.));
#151896=CARTESIAN_POINT('Ctrl Pts',(-53.5984603378862,46.4597261390526,
12.));
#151897=CARTESIAN_POINT('Ctrl Pts',(-53.6098978517869,46.4783349170182,
12.));
#151898=CARTESIAN_POINT('Ctrl Pts',(-53.6213412197542,46.4969959961779,
12.));
#151899=CARTESIAN_POINT('Ctrl Pts',(-53.6327903009098,46.5157092875377,
12.));
#151900=CARTESIAN_POINT('Ctrl Pts',(-53.6442449551455,46.5344747024677,
12.));
#151901=CARTESIAN_POINT('Ctrl Pts',(-53.6557050431069,46.5532921526899,
12.));
#151902=CARTESIAN_POINT('Ctrl Pts',(-53.6671704261735,46.5721615502589,
12.));
#151903=CARTESIAN_POINT('Ctrl Pts',(-53.678640966456,46.5910828075652,12.));
#151904=CARTESIAN_POINT('Ctrl Pts',(-53.690116526794,46.6100558373401,12.));
#151905=CARTESIAN_POINT('Ctrl Pts',(-53.7015969707541,46.6290805526559,
12.));
#151906=CARTESIAN_POINT('Ctrl Pts',(-53.7130821626262,46.6481568669217,
12.));
#151907=CARTESIAN_POINT('Ctrl Pts',(-53.7245719674221,46.6672846938752,
12.));
#151908=CARTESIAN_POINT('Ctrl Pts',(-53.7360662508675,46.6864639475862,
12.));
#151909=CARTESIAN_POINT('Ctrl Pts',(-53.7475648793946,46.7056945424559,
12.));
#151910=CARTESIAN_POINT('Ctrl Pts',(-53.7590677201342,46.7249763932129,
12.));
#151911=CARTESIAN_POINT('Ctrl Pts',(-53.7705746409076,46.7443094149045,
12.));
#151912=CARTESIAN_POINT('Ctrl Pts',(-53.7820855102182,46.763693522886,12.));
#151913=CARTESIAN_POINT('Ctrl Pts',(-53.793600197248,46.7831286328278,12.));
#151914=CARTESIAN_POINT('Ctrl Pts',(-53.8051185718532,46.802614660715,12.));
#151915=CARTESIAN_POINT('Ctrl Pts',(-53.816640504558,46.8221515228457,12.));
#151916=CARTESIAN_POINT('Ctrl Pts',(-53.8281658665503,46.841739135822,12.));
#151917=CARTESIAN_POINT('Ctrl Pts',(-53.8396945296757,46.8613774165435,
12.));
#151918=CARTESIAN_POINT('Ctrl Pts',(-53.8512263664321,46.881066282213,12.));
#151919=CARTESIAN_POINT('Ctrl Pts',(-53.8627612499638,46.9008056503351,
12.));
#151920=CARTESIAN_POINT('Ctrl Pts',(-53.8742990540563,46.9205954387133,
12.));
#151921=CARTESIAN_POINT('Ctrl Pts',(-53.8858396531298,46.94043556544,12.));
#151922=CARTESIAN_POINT('Ctrl Pts',(-53.8973829222348,46.960325948892,12.));
#151923=CARTESIAN_POINT('Ctrl Pts',(-53.9089287370463,46.9802665077366,
12.));
#151924=CARTESIAN_POINT('Ctrl Pts',(-53.9204769738596,47.0002571609297,
12.));
#151925=CARTESIAN_POINT('Ctrl Pts',(-53.9320275095853,47.0202978277138,
12.));
#151926=CARTESIAN_POINT('Ctrl Pts',(-53.9435802217436,47.0403884276071,
12.));
#151927=CARTESIAN_POINT('Ctrl Pts',(-53.95513498846,47.0605288804008,12.));
#151928=CARTESIAN_POINT('Ctrl Pts',(-53.9666916884596,47.0807191061648,
12.));
#151929=CARTESIAN_POINT('Ctrl Pts',(-53.9782502010634,47.1009590252458,
12.));
#151930=CARTESIAN_POINT('Ctrl Pts',(-53.989810406182,47.1212485582643,12.));
#151931=CARTESIAN_POINT('Ctrl Pts',(-54.0013721843118,47.1415876261035,
12.));
#151932=CARTESIAN_POINT('Ctrl Pts',(-54.0129354165297,47.1619761499087,
12.));
#151933=CARTESIAN_POINT('Ctrl Pts',(-54.0244999844893,47.1824140510926,
12.));
#151934=CARTESIAN_POINT('Ctrl Pts',(-54.0360657704163,47.202901251334,12.));
#151935=CARTESIAN_POINT('Ctrl Pts',(-54.047632657104,47.2234376725743,12.));
#151936=CARTESIAN_POINT('Ctrl Pts',(-54.0592005279086,47.2440232370065,
12.));
#151937=CARTESIAN_POINT('Ctrl Pts',(-54.0707692667438,47.2646578670746,
12.));
#151938=CARTESIAN_POINT('Ctrl Pts',(-54.0823387580776,47.2853414854793,
12.));
#151939=CARTESIAN_POINT('Ctrl Pts',(-54.0939088869269,47.3060740151752,
12.));
#151940=CARTESIAN_POINT('Ctrl Pts',(-54.1054795388543,47.3268553793694,
12.));
#151941=CARTESIAN_POINT('Ctrl Pts',(-54.1170505999645,47.3476855015102,
12.));
#151942=CARTESIAN_POINT('Ctrl Pts',(-54.1286219568989,47.3685643052874,
12.));
#151943=CARTESIAN_POINT('Ctrl Pts',(-54.1401934968311,47.3894917146365,
12.));
#151944=CARTESIAN_POINT('Ctrl Pts',(-54.1517651074637,47.4104676537381,
12.));
#151945=CARTESIAN_POINT('Ctrl Pts',(-54.1633366770239,47.4314920470141,
12.));
#151946=CARTESIAN_POINT('Ctrl Pts',(-54.1749080942593,47.4525648191173,
12.));
#151947=CARTESIAN_POINT('Ctrl Pts',(-54.1864792484345,47.4736858949322,
12.));
#151948=CARTESIAN_POINT('Ctrl Pts',(-54.198050029327,47.4948551995801,12.));
#151949=CARTESIAN_POINT('Ctrl Pts',(-54.209620327223,47.5160726584174,12.));
#151950=CARTESIAN_POINT('Ctrl Pts',(-54.2211900329138,47.5373381970326,
12.));
#151951=CARTESIAN_POINT('Ctrl Pts',(-54.2327590376924,47.5586517412363,
12.));
#151952=CARTESIAN_POINT('Ctrl Pts',(-54.244327233349,47.5800132170608,12.));
#151953=CARTESIAN_POINT('Ctrl Pts',(-54.2558945121678,47.6014225507659,
12.));
#151954=CARTESIAN_POINT('Ctrl Pts',(-54.2674607669226,47.6228796688375,
12.));
#151955=CARTESIAN_POINT('Ctrl Pts',(-54.2790258908738,47.6443844979847,
12.));
#151956=CARTESIAN_POINT('Ctrl Pts',(-54.290589777765,47.6659369651301,12.));
#151957=CARTESIAN_POINT('Ctrl Pts',(-54.302152321819,47.6875369974087,12.));
#151958=CARTESIAN_POINT('Ctrl Pts',(-54.3137134177345,47.7091845221747,
12.));
#151959=CARTESIAN_POINT('Ctrl Pts',(-54.3252729606823,47.7308794669993,
12.));
#151960=CARTESIAN_POINT('Ctrl Pts',(-54.3368308463023,47.7526217596694,
12.));
#151961=CARTESIAN_POINT('Ctrl Pts',(-54.3483869707002,47.7744113281771,
12.));
#151962=CARTESIAN_POINT('Ctrl Pts',(-54.3599412304437,47.7962481007185,
12.));
#151963=CARTESIAN_POINT('Ctrl Pts',(-54.3714935225591,47.8181320056995,
12.));
#151964=CARTESIAN_POINT('Ctrl Pts',(-54.3830437445279,47.8400629717355,
12.));
#151965=CARTESIAN_POINT('Ctrl Pts',(-54.3945917942832,47.8620409276493,
12.));
#151966=CARTESIAN_POINT('Ctrl Pts',(-54.4061375702079,47.8840658024618,
12.));
#151967=CARTESIAN_POINT('Ctrl Pts',(-54.4176809711311,47.9061375253897,
12.));
#151968=CARTESIAN_POINT('Ctrl Pts',(-54.429221896324,47.9282560258516,12.));
#151969=CARTESIAN_POINT('Ctrl Pts',(-54.4407602454967,47.9504212334675,
12.));
#151970=CARTESIAN_POINT('Ctrl Pts',(-54.4522959187955,47.9726330780572,
12.));
#151971=CARTESIAN_POINT('Ctrl Pts',(-54.4638288168003,47.9948914896326,
12.));
#151972=CARTESIAN_POINT('Ctrl Pts',(-54.4753588405215,48.0171963983924,
12.));
#151973=CARTESIAN_POINT('Ctrl Pts',(-54.4868858913971,48.0395477347298,
12.));
#151974=CARTESIAN_POINT('Ctrl Pts',(-54.4984098712886,48.0619454292324,
12.));
#151975=CARTESIAN_POINT('Ctrl Pts',(-54.5099306824786,48.0843894126806,
12.));
#151976=CARTESIAN_POINT('Ctrl Pts',(-54.5214482276678,48.1068796160405,
12.));
#151977=CARTESIAN_POINT('Ctrl Pts',(-54.5329624099721,48.1294159704573,
12.));
#151978=CARTESIAN_POINT('Ctrl Pts',(-54.5444731329201,48.1519984072622,
12.));
#151979=CARTESIAN_POINT('Ctrl Pts',(-54.5559803004492,48.1746268579736,
12.));
#151980=CARTESIAN_POINT('Ctrl Pts',(-54.5674838169041,48.1973012542966,
12.));
#151981=CARTESIAN_POINT('Ctrl Pts',(-54.5789835870342,48.2200215281173,
12.));
#151982=CARTESIAN_POINT('Ctrl Pts',(-54.5904795159926,48.2427876114947,
12.));
#151983=CARTESIAN_POINT('Ctrl Pts',(-54.6019715093309,48.2655994366665,
12.));
#151984=CARTESIAN_POINT('Ctrl Pts',(-54.6134594729959,48.2884569360506,
12.));
#151985=CARTESIAN_POINT('Ctrl Pts',(-54.6249433133261,48.3113600422443,
12.));
#151986=CARTESIAN_POINT('Ctrl Pts',(-54.6364229370494,48.3343086880194,
12.));
#151987=CARTESIAN_POINT('Ctrl Pts',(-54.6478982512794,48.3573028063124,
12.));
#151988=CARTESIAN_POINT('Ctrl Pts',(-54.6593691635145,48.3803423302294,
12.));
#151989=CARTESIAN_POINT('Ctrl Pts',(-54.6708355816358,48.4034271930514,
12.));
#151990=CARTESIAN_POINT('Ctrl Pts',(-54.6822974139064,48.426557328234,12.));
#151991=CARTESIAN_POINT('Ctrl Pts',(-54.6937545689695,48.4497326694052,
12.));
#151992=CARTESIAN_POINT('Ctrl Pts',(-54.7052069558497,48.472953150357,12.));
#151993=CARTESIAN_POINT('Ctrl Pts',(-54.716654483948,48.4962187050457,12.));
#151994=CARTESIAN_POINT('Ctrl Pts',(-54.7280970630351,48.519529267596,12.));
#151995=CARTESIAN_POINT('Ctrl Pts',(-54.7395346032453,48.5428847722977,
12.));
#151996=CARTESIAN_POINT('Ctrl Pts',(-54.7509670150714,48.5662851536026,
12.));
#151997=CARTESIAN_POINT('Ctrl Pts',(-54.7623942093586,48.5897303461125,
12.));
#151998=CARTESIAN_POINT('Ctrl Pts',(-54.7738160973031,48.6132202845783,
12.));
#151999=CARTESIAN_POINT('Ctrl Pts',(-54.7852325904583,48.6367549039112,
12.));
#152000=CARTESIAN_POINT('Ctrl Pts',(-54.796643600739,48.6603341391886,12.));
#152001=CARTESIAN_POINT('Ctrl Pts',(-54.8080490404275,48.6839579256566,
12.));
#152002=CARTESIAN_POINT('Ctrl Pts',(-54.819448822181,48.7076261987292,12.));
#152003=CARTESIAN_POINT('Ctrl Pts',(-54.8308428590344,48.7313388939845,
12.));
#152004=CARTESIAN_POINT('Ctrl Pts',(-54.8422310643763,48.7550959471601,
12.));
#152005=CARTESIAN_POINT('Ctrl Pts',(-54.8536133519292,48.7788972941438,
12.));
#152006=CARTESIAN_POINT('Ctrl Pts',(-54.8649896357285,48.8027428709614,
12.));
#152007=CARTESIAN_POINT('Ctrl Pts',(-54.8763598301037,48.8266326137622,
12.));
#152008=CARTESIAN_POINT('Ctrl Pts',(-54.8877238496566,48.8505664587974,
12.));
#152009=CARTESIAN_POINT('Ctrl Pts',(-54.8990816092953,48.8745443424477,
12.));
#152010=CARTESIAN_POINT('Ctrl Pts',(-54.9104330242742,48.8985662012528,
12.));
#152011=CARTESIAN_POINT('Ctrl Pts',(-54.9217780102355,48.9226319719368,
12.));
#152012=CARTESIAN_POINT('Ctrl Pts',(-54.9331164832424,48.9467415914269,
12.));
#152013=CARTESIAN_POINT('Ctrl Pts',(-54.9444483598378,48.9708949968795,
12.));
#152014=CARTESIAN_POINT('Ctrl Pts',(-54.9557735569943,48.9950921256526,
12.));
#152015=CARTESIAN_POINT('Ctrl Pts',(-54.9670919920029,49.0193329152479,
12.));
#152016=CARTESIAN_POINT('Ctrl Pts',(-54.9784035823766,49.0436173032528,
12.));
#152017=CARTESIAN_POINT('Ctrl Pts',(-54.9897082457606,49.067945227287,12.));
#152018=CARTESIAN_POINT('Ctrl Pts',(-55.0010058998107,49.0923166249219,
12.));
#152019=CARTESIAN_POINT('Ctrl Pts',(-55.012296462186,49.116731433673,12.));
#152020=CARTESIAN_POINT('Ctrl Pts',(-55.0235798508045,49.1411895911635,
12.));
#152021=CARTESIAN_POINT('Ctrl Pts',(-55.0348559840453,49.1656910352476,
12.));
#152022=CARTESIAN_POINT('Ctrl Pts',(-55.0461247809744,49.1902357041461,
12.));
#152023=CARTESIAN_POINT('Ctrl Pts',(-55.0573861615579,49.2148235365703,
12.));
#152024=CARTESIAN_POINT('Ctrl Pts',(-55.0686400468931,49.2394544718531,
12.));
#152025=CARTESIAN_POINT('Ctrl Pts',(-55.079886358701,49.264128449652,12.));
#152026=CARTESIAN_POINT('Ctrl Pts',(-55.0911250188302,49.2888454096563,
12.));
#152027=CARTESIAN_POINT('Ctrl Pts',(-55.102355948714,49.3136052912621,12.));
#152028=CARTESIAN_POINT('Ctrl Pts',(-55.1135790689464,49.3384080333155,
12.));
#152029=CARTESIAN_POINT('Ctrl Pts',(-55.1247942985619,49.3632535736715,
12.));
#152030=CARTESIAN_POINT('Ctrl Pts',(-55.1360015556221,49.3881418495489,
12.));
#152031=CARTESIAN_POINT('Ctrl Pts',(-55.1472007585183,49.4130727983201,
12.));
#152032=CARTESIAN_POINT('Ctrl Pts',(-55.1583918271116,49.4380463581965,
12.));
#152033=CARTESIAN_POINT('Ctrl Pts',(-55.1695746838174,49.4630624688793,
12.));
#152034=CARTESIAN_POINT('Ctrl Pts',(-55.1807492550119,49.4881210723966,
12.));
#152035=CARTESIAN_POINT('Ctrl Pts',(-55.1919154713647,49.5132221132992,
12.));
#152036=CARTESIAN_POINT('Ctrl Pts',(-55.2014798624093,49.5347748994759,
12.));
#152037=CARTESIAN_POINT('Ctrl Pts',(-55.2088081099093,49.551321852449,12.));
#152038=CARTESIAN_POINT('Ctrl Pts',(-55.2139039604722,49.5628442142133,
12.));
#152039=CARTESIAN_POINT('Ctrl Pts',(-55.2167699151339,49.5693295981928,
12.));
#152040=CARTESIAN_POINT('Ctrl Pts',(-55.2174072001495,49.5707719660639,
12.));
#152041=CARTESIAN_POINT('',(-53.0702932034641,45.6458539113724,0.));
#152042=CARTESIAN_POINT('',(-53.0702932034641,45.6458539113724,0.));
#152043=CARTESIAN_POINT('Ctrl Pts',(-55.2174072001495,49.5707719660639,
0.));
#152044=CARTESIAN_POINT('Ctrl Pts',(-55.2167699151339,49.5693295981928,
0.));
#152045=CARTESIAN_POINT('Ctrl Pts',(-55.2139039604722,49.5628442142133,
0.));
#152046=CARTESIAN_POINT('Ctrl Pts',(-55.2088081099093,49.551321852449,0.));
#152047=CARTESIAN_POINT('Ctrl Pts',(-55.2014798624093,49.5347748994759,
0.));
#152048=CARTESIAN_POINT('Ctrl Pts',(-55.1919154713647,49.5132221132992,
0.));
#152049=CARTESIAN_POINT('Ctrl Pts',(-55.1807492550119,49.4881210723966,
0.));
#152050=CARTESIAN_POINT('Ctrl Pts',(-55.1695746838174,49.4630624688793,
0.));
#152051=CARTESIAN_POINT('Ctrl Pts',(-55.1583918271116,49.4380463581965,
0.));
#152052=CARTESIAN_POINT('Ctrl Pts',(-55.1472007585183,49.4130727983201,
0.));
#152053=CARTESIAN_POINT('Ctrl Pts',(-55.1360015556221,49.3881418495489,
0.));
#152054=CARTESIAN_POINT('Ctrl Pts',(-55.1247942985619,49.3632535736715,
0.));
#152055=CARTESIAN_POINT('Ctrl Pts',(-55.1135790689464,49.3384080333155,
0.));
#152056=CARTESIAN_POINT('Ctrl Pts',(-55.102355948714,49.3136052912621,0.));
#152057=CARTESIAN_POINT('Ctrl Pts',(-55.0911250188302,49.2888454096563,
0.));
#152058=CARTESIAN_POINT('Ctrl Pts',(-55.079886358701,49.264128449652,0.));
#152059=CARTESIAN_POINT('Ctrl Pts',(-55.0686400468931,49.2394544718531,
0.));
#152060=CARTESIAN_POINT('Ctrl Pts',(-55.0573861615579,49.2148235365703,
0.));
#152061=CARTESIAN_POINT('Ctrl Pts',(-55.0461247809744,49.1902357041461,
0.));
#152062=CARTESIAN_POINT('Ctrl Pts',(-55.0348559840453,49.1656910352476,
0.));
#152063=CARTESIAN_POINT('Ctrl Pts',(-55.0235798508045,49.1411895911635,
0.));
#152064=CARTESIAN_POINT('Ctrl Pts',(-55.012296462186,49.116731433673,0.));
#152065=CARTESIAN_POINT('Ctrl Pts',(-55.0010058998107,49.0923166249219,
0.));
#152066=CARTESIAN_POINT('Ctrl Pts',(-54.9897082457606,49.067945227287,0.));
#152067=CARTESIAN_POINT('Ctrl Pts',(-54.9784035823766,49.0436173032528,
0.));
#152068=CARTESIAN_POINT('Ctrl Pts',(-54.9670919920029,49.0193329152479,
0.));
#152069=CARTESIAN_POINT('Ctrl Pts',(-54.9557735569943,48.9950921256526,
0.));
#152070=CARTESIAN_POINT('Ctrl Pts',(-54.9444483598378,48.9708949968795,
0.));
#152071=CARTESIAN_POINT('Ctrl Pts',(-54.9331164832424,48.9467415914269,
0.));
#152072=CARTESIAN_POINT('Ctrl Pts',(-54.9217780102355,48.9226319719368,
0.));
#152073=CARTESIAN_POINT('Ctrl Pts',(-54.9104330242742,48.8985662012528,
0.));
#152074=CARTESIAN_POINT('Ctrl Pts',(-54.8990816092953,48.8745443424477,
0.));
#152075=CARTESIAN_POINT('Ctrl Pts',(-54.8877238496566,48.8505664587974,
0.));
#152076=CARTESIAN_POINT('Ctrl Pts',(-54.8763598301037,48.8266326137622,
0.));
#152077=CARTESIAN_POINT('Ctrl Pts',(-54.8649896357285,48.8027428709614,
0.));
#152078=CARTESIAN_POINT('Ctrl Pts',(-54.8536133519292,48.7788972941438,
0.));
#152079=CARTESIAN_POINT('Ctrl Pts',(-54.8422310643763,48.7550959471601,
0.));
#152080=CARTESIAN_POINT('Ctrl Pts',(-54.8308428590344,48.7313388939845,
0.));
#152081=CARTESIAN_POINT('Ctrl Pts',(-54.819448822181,48.7076261987292,0.));
#152082=CARTESIAN_POINT('Ctrl Pts',(-54.8080490404275,48.6839579256566,
0.));
#152083=CARTESIAN_POINT('Ctrl Pts',(-54.796643600739,48.6603341391886,0.));
#152084=CARTESIAN_POINT('Ctrl Pts',(-54.7852325904583,48.6367549039112,
0.));
#152085=CARTESIAN_POINT('Ctrl Pts',(-54.7738160973031,48.6132202845783,
0.));
#152086=CARTESIAN_POINT('Ctrl Pts',(-54.7623942093586,48.5897303461125,
0.));
#152087=CARTESIAN_POINT('Ctrl Pts',(-54.7509670150714,48.5662851536026,
0.));
#152088=CARTESIAN_POINT('Ctrl Pts',(-54.7395346032453,48.5428847722977,
0.));
#152089=CARTESIAN_POINT('Ctrl Pts',(-54.7280970630351,48.519529267596,0.));
#152090=CARTESIAN_POINT('Ctrl Pts',(-54.716654483948,48.4962187050457,0.));
#152091=CARTESIAN_POINT('Ctrl Pts',(-54.7052069558497,48.472953150357,0.));
#152092=CARTESIAN_POINT('Ctrl Pts',(-54.6937545689695,48.4497326694052,
0.));
#152093=CARTESIAN_POINT('Ctrl Pts',(-54.6822974139064,48.426557328234,0.));
#152094=CARTESIAN_POINT('Ctrl Pts',(-54.6708355816358,48.4034271930514,
0.));
#152095=CARTESIAN_POINT('Ctrl Pts',(-54.6593691635145,48.3803423302294,
0.));
#152096=CARTESIAN_POINT('Ctrl Pts',(-54.6478982512794,48.3573028063124,
0.));
#152097=CARTESIAN_POINT('Ctrl Pts',(-54.6364229370494,48.3343086880194,
0.));
#152098=CARTESIAN_POINT('Ctrl Pts',(-54.6249433133261,48.3113600422443,
0.));
#152099=CARTESIAN_POINT('Ctrl Pts',(-54.6134594729959,48.2884569360506,
0.));
#152100=CARTESIAN_POINT('Ctrl Pts',(-54.6019715093309,48.2655994366665,
0.));
#152101=CARTESIAN_POINT('Ctrl Pts',(-54.5904795159926,48.2427876114947,
0.));
#152102=CARTESIAN_POINT('Ctrl Pts',(-54.5789835870342,48.2200215281173,
0.));
#152103=CARTESIAN_POINT('Ctrl Pts',(-54.5674838169041,48.1973012542966,
0.));
#152104=CARTESIAN_POINT('Ctrl Pts',(-54.5559803004492,48.1746268579736,
0.));
#152105=CARTESIAN_POINT('Ctrl Pts',(-54.5444731329201,48.1519984072622,
0.));
#152106=CARTESIAN_POINT('Ctrl Pts',(-54.5329624099721,48.1294159704573,
0.));
#152107=CARTESIAN_POINT('Ctrl Pts',(-54.5214482276678,48.1068796160405,
0.));
#152108=CARTESIAN_POINT('Ctrl Pts',(-54.5099306824786,48.0843894126806,
0.));
#152109=CARTESIAN_POINT('Ctrl Pts',(-54.4984098712886,48.0619454292324,
0.));
#152110=CARTESIAN_POINT('Ctrl Pts',(-54.4868858913971,48.0395477347298,
0.));
#152111=CARTESIAN_POINT('Ctrl Pts',(-54.4753588405215,48.0171963983924,
0.));
#152112=CARTESIAN_POINT('Ctrl Pts',(-54.4638288168003,47.9948914896326,
0.));
#152113=CARTESIAN_POINT('Ctrl Pts',(-54.4522959187955,47.9726330780572,
0.));
#152114=CARTESIAN_POINT('Ctrl Pts',(-54.4407602454967,47.9504212334675,
0.));
#152115=CARTESIAN_POINT('Ctrl Pts',(-54.429221896324,47.9282560258516,0.));
#152116=CARTESIAN_POINT('Ctrl Pts',(-54.4176809711311,47.9061375253897,
0.));
#152117=CARTESIAN_POINT('Ctrl Pts',(-54.4061375702079,47.8840658024618,
0.));
#152118=CARTESIAN_POINT('Ctrl Pts',(-54.3945917942832,47.8620409276493,
0.));
#152119=CARTESIAN_POINT('Ctrl Pts',(-54.3830437445279,47.8400629717355,
0.));
#152120=CARTESIAN_POINT('Ctrl Pts',(-54.3714935225591,47.8181320056995,
0.));
#152121=CARTESIAN_POINT('Ctrl Pts',(-54.3599412304437,47.7962481007185,
0.));
#152122=CARTESIAN_POINT('Ctrl Pts',(-54.3483869707002,47.7744113281771,
0.));
#152123=CARTESIAN_POINT('Ctrl Pts',(-54.3368308463023,47.7526217596694,
0.));
#152124=CARTESIAN_POINT('Ctrl Pts',(-54.3252729606823,47.7308794669993,
0.));
#152125=CARTESIAN_POINT('Ctrl Pts',(-54.3137134177345,47.7091845221747,
0.));
#152126=CARTESIAN_POINT('Ctrl Pts',(-54.302152321819,47.6875369974087,0.));
#152127=CARTESIAN_POINT('Ctrl Pts',(-54.290589777765,47.6659369651301,0.));
#152128=CARTESIAN_POINT('Ctrl Pts',(-54.2790258908738,47.6443844979847,
0.));
#152129=CARTESIAN_POINT('Ctrl Pts',(-54.2674607669226,47.6228796688375,
0.));
#152130=CARTESIAN_POINT('Ctrl Pts',(-54.2558945121678,47.6014225507659,
0.));
#152131=CARTESIAN_POINT('Ctrl Pts',(-54.244327233349,47.5800132170608,0.));
#152132=CARTESIAN_POINT('Ctrl Pts',(-54.2327590376924,47.5586517412363,
0.));
#152133=CARTESIAN_POINT('Ctrl Pts',(-54.2211900329138,47.5373381970326,
0.));
#152134=CARTESIAN_POINT('Ctrl Pts',(-54.209620327223,47.5160726584174,0.));
#152135=CARTESIAN_POINT('Ctrl Pts',(-54.198050029327,47.4948551995801,0.));
#152136=CARTESIAN_POINT('Ctrl Pts',(-54.1864792484345,47.4736858949322,
0.));
#152137=CARTESIAN_POINT('Ctrl Pts',(-54.1749080942593,47.4525648191173,
0.));
#152138=CARTESIAN_POINT('Ctrl Pts',(-54.1633366770239,47.4314920470141,
0.));
#152139=CARTESIAN_POINT('Ctrl Pts',(-54.1517651074637,47.4104676537381,
0.));
#152140=CARTESIAN_POINT('Ctrl Pts',(-54.1401934968311,47.3894917146365,
0.));
#152141=CARTESIAN_POINT('Ctrl Pts',(-54.1286219568989,47.3685643052874,
0.));
#152142=CARTESIAN_POINT('Ctrl Pts',(-54.1170505999645,47.3476855015102,
0.));
#152143=CARTESIAN_POINT('Ctrl Pts',(-54.1054795388543,47.3268553793694,
0.));
#152144=CARTESIAN_POINT('Ctrl Pts',(-54.0939088869269,47.3060740151752,
0.));
#152145=CARTESIAN_POINT('Ctrl Pts',(-54.0823387580776,47.2853414854793,
0.));
#152146=CARTESIAN_POINT('Ctrl Pts',(-54.0707692667438,47.2646578670746,
0.));
#152147=CARTESIAN_POINT('Ctrl Pts',(-54.0592005279086,47.2440232370065,
0.));
#152148=CARTESIAN_POINT('Ctrl Pts',(-54.047632657104,47.2234376725743,0.));
#152149=CARTESIAN_POINT('Ctrl Pts',(-54.0360657704163,47.202901251334,0.));
#152150=CARTESIAN_POINT('Ctrl Pts',(-54.0244999844893,47.1824140510926,
0.));
#152151=CARTESIAN_POINT('Ctrl Pts',(-54.0129354165297,47.1619761499087,
0.));
#152152=CARTESIAN_POINT('Ctrl Pts',(-54.0013721843118,47.1415876261035,
0.));
#152153=CARTESIAN_POINT('Ctrl Pts',(-53.989810406182,47.1212485582643,0.));
#152154=CARTESIAN_POINT('Ctrl Pts',(-53.9782502010634,47.1009590252458,
0.));
#152155=CARTESIAN_POINT('Ctrl Pts',(-53.9666916884596,47.0807191061648,
0.));
#152156=CARTESIAN_POINT('Ctrl Pts',(-53.95513498846,47.0605288804008,0.));
#152157=CARTESIAN_POINT('Ctrl Pts',(-53.9435802217436,47.0403884276071,
0.));
#152158=CARTESIAN_POINT('Ctrl Pts',(-53.9320275095853,47.0202978277138,
0.));
#152159=CARTESIAN_POINT('Ctrl Pts',(-53.9204769738596,47.0002571609297,
0.));
#152160=CARTESIAN_POINT('Ctrl Pts',(-53.9089287370463,46.9802665077366,
0.));
#152161=CARTESIAN_POINT('Ctrl Pts',(-53.8973829222348,46.960325948892,0.));
#152162=CARTESIAN_POINT('Ctrl Pts',(-53.8858396531298,46.94043556544,0.));
#152163=CARTESIAN_POINT('Ctrl Pts',(-53.8742990540563,46.9205954387133,
0.));
#152164=CARTESIAN_POINT('Ctrl Pts',(-53.8627612499638,46.9008056503351,
0.));
#152165=CARTESIAN_POINT('Ctrl Pts',(-53.8512263664321,46.881066282213,0.));
#152166=CARTESIAN_POINT('Ctrl Pts',(-53.8396945296757,46.8613774165435,
0.));
#152167=CARTESIAN_POINT('Ctrl Pts',(-53.8281658665503,46.841739135822,0.));
#152168=CARTESIAN_POINT('Ctrl Pts',(-53.816640504558,46.8221515228457,0.));
#152169=CARTESIAN_POINT('Ctrl Pts',(-53.8051185718532,46.802614660715,0.));
#152170=CARTESIAN_POINT('Ctrl Pts',(-53.793600197248,46.7831286328278,0.));
#152171=CARTESIAN_POINT('Ctrl Pts',(-53.7820855102182,46.763693522886,0.));
#152172=CARTESIAN_POINT('Ctrl Pts',(-53.7705746409076,46.7443094149045,
0.));
#152173=CARTESIAN_POINT('Ctrl Pts',(-53.7590677201342,46.7249763932129,
0.));
#152174=CARTESIAN_POINT('Ctrl Pts',(-53.7475648793946,46.7056945424559,
0.));
#152175=CARTESIAN_POINT('Ctrl Pts',(-53.7360662508675,46.6864639475862,
0.));
#152176=CARTESIAN_POINT('Ctrl Pts',(-53.7245719674221,46.6672846938752,
0.));
#152177=CARTESIAN_POINT('Ctrl Pts',(-53.7130821626262,46.6481568669217,
0.));
#152178=CARTESIAN_POINT('Ctrl Pts',(-53.7015969707541,46.6290805526559,
0.));
#152179=CARTESIAN_POINT('Ctrl Pts',(-53.690116526794,46.6100558373401,0.));
#152180=CARTESIAN_POINT('Ctrl Pts',(-53.678640966456,46.5910828075652,0.));
#152181=CARTESIAN_POINT('Ctrl Pts',(-53.6671704261735,46.5721615502589,
0.));
#152182=CARTESIAN_POINT('Ctrl Pts',(-53.6557050431069,46.5532921526899,
0.));
#152183=CARTESIAN_POINT('Ctrl Pts',(-53.6442449551455,46.5344747024677,
0.));
#152184=CARTESIAN_POINT('Ctrl Pts',(-53.6327903009098,46.5157092875377,
0.));
#152185=CARTESIAN_POINT('Ctrl Pts',(-53.6213412197542,46.4969959961779,
0.));
#152186=CARTESIAN_POINT('Ctrl Pts',(-53.6098978517869,46.4783349170182,
0.));
#152187=CARTESIAN_POINT('Ctrl Pts',(-53.5984603378862,46.4597261390526,
0.));
#152188=CARTESIAN_POINT('Ctrl Pts',(-53.5870288197161,46.4411697516474,
0.));
#152189=CARTESIAN_POINT('Ctrl Pts',(-53.5756034397464,46.422665844546,0.));
#152190=CARTESIAN_POINT('Ctrl Pts',(-53.5641843412537,46.4042145078682,
0.));
#152191=CARTESIAN_POINT('Ctrl Pts',(-53.552771668303,46.3858158321044,0.));
#152192=CARTESIAN_POINT('Ctrl Pts',(-53.5413655657323,46.3674699081043,
0.));
#152193=CARTESIAN_POINT('Ctrl Pts',(-53.5299661791396,46.3491768270664,
0.));
#152194=CARTESIAN_POINT('Ctrl Pts',(-53.518573654857,46.3309366805112,0.));
#152195=CARTESIAN_POINT('Ctrl Pts',(-53.5071881399932,46.3127495603117,
0.));
#152196=CARTESIAN_POINT('Ctrl Pts',(-53.4958097825019,46.2946155587428,
0.));
#152197=CARTESIAN_POINT('Ctrl Pts',(-53.4844387312414,46.2765347685198,
0.));
#152198=CARTESIAN_POINT('Ctrl Pts',(-53.4730751360359,46.2585072828343,
0.));
#152199=CARTESIAN_POINT('Ctrl Pts',(-53.4617191477382,46.2405331953872,
0.));
#152200=CARTESIAN_POINT('Ctrl Pts',(-53.4503709181158,46.2226126003185,
0.));
#152201=CARTESIAN_POINT('Ctrl Pts',(-53.4390305997263,46.2047455921276,
0.));
#152202=CARTESIAN_POINT('Ctrl Pts',(-53.4276983458129,46.1869322656027,
0.));
#152203=CARTESIAN_POINT('Ctrl Pts',(-53.4163743101535,46.1691727157149,
0.));
#152204=CARTESIAN_POINT('Ctrl Pts',(-53.4050586470463,46.1514670376035,
0.));
#152205=CARTESIAN_POINT('Ctrl Pts',(-53.3937515116572,46.1338153268116,
0.));
#152206=CARTESIAN_POINT('Ctrl Pts',(-53.3824530603284,46.1162176794891,
0.));
#152207=CARTESIAN_POINT('Ctrl Pts',(-53.3711634508426,46.0986741925646,
0.));
#152208=CARTESIAN_POINT('Ctrl Pts',(-53.3598828428519,46.0811849640195,
0.));
#152209=CARTESIAN_POINT('Ctrl Pts',(-53.3486113975868,46.0637500926954,
0.));
#152210=CARTESIAN_POINT('Ctrl Pts',(-53.3373492770647,46.046369677778,0.));
#152211=CARTESIAN_POINT('Ctrl Pts',(-53.3260966434277,46.0290438183598,
0.));
#152212=CARTESIAN_POINT('Ctrl Pts',(-53.3148536582658,46.0117726129893,
0.));
#152213=CARTESIAN_POINT('Ctrl Pts',(-53.3036204818367,45.9945561591486,
0.));
#152214=CARTESIAN_POINT('Ctrl Pts',(-53.2923972745585,45.9773945542415,
0.));
#152215=CARTESIAN_POINT('Ctrl Pts',(-53.2811841987945,45.9602878967714,
0.));
#152216=CARTESIAN_POINT('Ctrl Pts',(-53.2699814203097,45.9432362873001,
0.));
#152217=CARTESIAN_POINT('Ctrl Pts',(-53.2587891103835,45.9262398298323,
0.));
#152218=CARTESIAN_POINT('Ctrl Pts',(-53.2476074459977,45.9092986319343,
0.));
#152219=CARTESIAN_POINT('Ctrl Pts',(-53.2364366054276,45.8924128018354,
0.));
#152220=CARTESIAN_POINT('Ctrl Pts',(-53.2252767643652,45.8755824458715,
0.));
#152221=CARTESIAN_POINT('Ctrl Pts',(-53.2141280925458,45.8588076662598,
0.));
#152222=CARTESIAN_POINT('Ctrl Pts',(-53.2029907483602,45.8420885575386,
0.));
#152223=CARTESIAN_POINT('Ctrl Pts',(-53.1918648840598,45.8254252100003,
0.));
#152224=CARTESIAN_POINT('Ctrl Pts',(-53.1807506560977,45.8088177165124,
0.));
#152225=CARTESIAN_POINT('Ctrl Pts',(-53.1696482334487,45.7922661780005,
0.));
#152226=CARTESIAN_POINT('Ctrl Pts',(-53.158557807638,45.7757707100568,0.));
#152227=CARTESIAN_POINT('Ctrl Pts',(-53.147479599594,45.7593314474412,0.));
#152228=CARTESIAN_POINT('Ctrl Pts',(-53.136413838457,45.7429485300727,0.));
#152229=CARTESIAN_POINT('Ctrl Pts',(-53.1253607414806,45.7266220896951,
0.));
#152230=CARTESIAN_POINT('Ctrl Pts',(-53.1143204954981,45.7103522376744,
0.));
#152231=CARTESIAN_POINT('Ctrl Pts',(-53.1032932329074,45.6941390489239,
0.));
#152232=CARTESIAN_POINT('Ctrl Pts',(-53.0922790298736,45.6779825614486,
0.));
#152233=CARTESIAN_POINT('Ctrl Pts',(-53.083478145185,45.6651027439479,0.));
#152234=CARTESIAN_POINT('Ctrl Pts',(-53.0768833804386,45.6554684028296,
0.));
#152235=CARTESIAN_POINT('Ctrl Pts',(-53.0724894921921,45.6490568514146,
0.));
#152236=CARTESIAN_POINT('Ctrl Pts',(-53.0702932034641,45.6458539113724,
0.));
#152237=CARTESIAN_POINT('Ctrl Pts',(-50.7903314215393,54.5031396718592,
0.));
#152238=CARTESIAN_POINT('Ctrl Pts',(-50.7903314215393,54.5031396718592,
12.));
#152239=CARTESIAN_POINT('Ctrl Pts',(-50.7885805844281,54.4978248630387,
0.));
#152240=CARTESIAN_POINT('Ctrl Pts',(-50.7885805844281,54.4978248630387,
12.));
#152241=CARTESIAN_POINT('Ctrl Pts',(-50.7850776288814,54.4871993224832,
0.));
#152242=CARTESIAN_POINT('Ctrl Pts',(-50.7850776288814,54.4871993224832,
12.));
#152243=CARTESIAN_POINT('Ctrl Pts',(-50.7798193515888,54.4712732429066,
0.));
#152244=CARTESIAN_POINT('Ctrl Pts',(-50.7798193515888,54.4712732429066,
12.));
#152245=CARTESIAN_POINT('Ctrl Pts',(-50.7728006269349,54.4500629336429,
0.));
#152246=CARTESIAN_POINT('Ctrl Pts',(-50.7728006269349,54.4500629336429,
12.));
#152247=CARTESIAN_POINT('Ctrl Pts',(-50.764014409002,54.423590828767,0.));
#152248=CARTESIAN_POINT('Ctrl Pts',(-50.764014409002,54.423590828767,12.));
#152249=CARTESIAN_POINT('Ctrl Pts',(-50.7552153869475,54.3971595231574,
0.));
#152250=CARTESIAN_POINT('Ctrl Pts',(-50.7552153869475,54.3971595231574,
12.));
#152251=CARTESIAN_POINT('Ctrl Pts',(-50.7464035792906,54.3707690445748,
0.));
#152252=CARTESIAN_POINT('Ctrl Pts',(-50.7464035792906,54.3707690445748,
12.));
#152253=CARTESIAN_POINT('Ctrl Pts',(-50.7375790185896,54.3444194324054,
0.));
#152254=CARTESIAN_POINT('Ctrl Pts',(-50.7375790185896,54.3444194324054,
12.));
#152255=CARTESIAN_POINT('Ctrl Pts',(-50.7287417566123,54.3181107400663,
0.));
#152256=CARTESIAN_POINT('Ctrl Pts',(-50.7287417566123,54.3181107400663,
12.));
#152257=CARTESIAN_POINT('Ctrl Pts',(-50.7198918629451,54.2918430335206,
0.));
#152258=CARTESIAN_POINT('Ctrl Pts',(-50.7198918629451,54.2918430335206,
12.));
#152259=CARTESIAN_POINT('Ctrl Pts',(-50.7110294185698,54.2656163868104,
0.));
#152260=CARTESIAN_POINT('Ctrl Pts',(-50.7110294185698,54.2656163868104,
12.));
#152261=CARTESIAN_POINT('Ctrl Pts',(-50.7021545108311,54.2394308784026,
0.));
#152262=CARTESIAN_POINT('Ctrl Pts',(-50.7021545108311,54.2394308784026,
12.));
#152263=CARTESIAN_POINT('Ctrl Pts',(-50.6932672279772,54.2132865872985,
0.));
#152264=CARTESIAN_POINT('Ctrl Pts',(-50.6932672279772,54.2132865872985,
12.));
#152265=CARTESIAN_POINT('Ctrl Pts',(-50.6843676535492,54.1871835889981,
0.));
#152266=CARTESIAN_POINT('Ctrl Pts',(-50.6843676535492,54.1871835889981,
12.));
#152267=CARTESIAN_POINT('Ctrl Pts',(-50.67545586183,54.1611219522394,0.));
#152268=CARTESIAN_POINT('Ctrl Pts',(-50.67545586183,54.1611219522394,12.));
#152269=CARTESIAN_POINT('Ctrl Pts',(-50.6665319209869,54.1351017412804,
0.));
#152270=CARTESIAN_POINT('Ctrl Pts',(-50.6665319209869,54.1351017412804,
12.));
#152271=CARTESIAN_POINT('Ctrl Pts',(-50.6575958953221,54.1091230175367,
0.));
#152272=CARTESIAN_POINT('Ctrl Pts',(-50.6575958953221,54.1091230175367,
12.));
#152273=CARTESIAN_POINT('Ctrl Pts',(-50.6486478479465,54.0831858415189,
0.));
#152274=CARTESIAN_POINT('Ctrl Pts',(-50.6486478479465,54.0831858415189,
12.));
#152275=CARTESIAN_POINT('Ctrl Pts',(-50.6396878430939,54.0572902745076,
0.));
#152276=CARTESIAN_POINT('Ctrl Pts',(-50.6396878430939,54.0572902745076,
12.));
#152277=CARTESIAN_POINT('Ctrl Pts',(-50.6307159490553,54.0314363806708,
0.));
#152278=CARTESIAN_POINT('Ctrl Pts',(-50.6307159490553,54.0314363806708,
12.));
#152279=CARTESIAN_POINT('Ctrl Pts',(-50.6217322378648,54.0056242268399,
0.));
#152280=CARTESIAN_POINT('Ctrl Pts',(-50.6217322378648,54.0056242268399,
12.));
#152281=CARTESIAN_POINT('Ctrl Pts',(-50.6127367839711,53.979853881553,0.));
#152282=CARTESIAN_POINT('Ctrl Pts',(-50.6127367839711,53.979853881553,12.));
#152283=CARTESIAN_POINT('Ctrl Pts',(-50.603729663214,53.9541254143119,0.));
#152284=CARTESIAN_POINT('Ctrl Pts',(-50.603729663214,53.9541254143119,12.));
#152285=CARTESIAN_POINT('Ctrl Pts',(-50.5947109517483,53.9284388948004,
0.));
#152286=CARTESIAN_POINT('Ctrl Pts',(-50.5947109517483,53.9284388948004,
12.));
#152287=CARTESIAN_POINT('Ctrl Pts',(-50.5856807248151,53.9027943919836,
0.));
#152288=CARTESIAN_POINT('Ctrl Pts',(-50.5856807248151,53.9027943919836,
12.));
#152289=CARTESIAN_POINT('Ctrl Pts',(-50.5766390561884,53.8771919737032,
0.));
#152290=CARTESIAN_POINT('Ctrl Pts',(-50.5766390561884,53.8771919737032,
12.));
#152291=CARTESIAN_POINT('Ctrl Pts',(-50.5675860188538,53.8516317071804,
0.));
#152292=CARTESIAN_POINT('Ctrl Pts',(-50.5675860188538,53.8516317071804,
12.));
#152293=CARTESIAN_POINT('Ctrl Pts',(-50.5585216854091,53.8261136593075,
0.));
#152294=CARTESIAN_POINT('Ctrl Pts',(-50.5585216854091,53.8261136593075,
12.));
#152295=CARTESIAN_POINT('Ctrl Pts',(-50.5494461285761,53.8006378970197,
0.));
#152296=CARTESIAN_POINT('Ctrl Pts',(-50.5494461285761,53.8006378970197,
12.));
#152297=CARTESIAN_POINT('Ctrl Pts',(-50.5403594216698,53.7752044876304,
0.));
#152298=CARTESIAN_POINT('Ctrl Pts',(-50.5403594216698,53.7752044876304,
12.));
#152299=CARTESIAN_POINT('Ctrl Pts',(-50.5312616390779,53.7498134991703,
0.));
#152300=CARTESIAN_POINT('Ctrl Pts',(-50.5312616390779,53.7498134991703,
12.));
#152301=CARTESIAN_POINT('Ctrl Pts',(-50.522152856042,53.7244650002374,0.));
#152302=CARTESIAN_POINT('Ctrl Pts',(-50.522152856042,53.7244650002374,12.));
#152303=CARTESIAN_POINT('Ctrl Pts',(-50.513033148456,53.6991590598548,0.));
#152304=CARTESIAN_POINT('Ctrl Pts',(-50.513033148456,53.6991590598548,12.));
#152305=CARTESIAN_POINT('Ctrl Pts',(-50.503902592653,53.6738957473158,0.));
#152306=CARTESIAN_POINT('Ctrl Pts',(-50.503902592653,53.6738957473158,12.));
#152307=CARTESIAN_POINT('Ctrl Pts',(-50.4947612652148,53.6486751320436,
0.));
#152308=CARTESIAN_POINT('Ctrl Pts',(-50.4947612652148,53.6486751320436,
12.));
#152309=CARTESIAN_POINT('Ctrl Pts',(-50.4856092427314,53.623497283406,0.));
#152310=CARTESIAN_POINT('Ctrl Pts',(-50.4856092427314,53.623497283406,12.));
#152311=CARTESIAN_POINT('Ctrl Pts',(-50.4764466018071,53.5983622707238,
0.));
#152312=CARTESIAN_POINT('Ctrl Pts',(-50.4764466018071,53.5983622707238,
12.));
#152313=CARTESIAN_POINT('Ctrl Pts',(-50.4672734191756,53.5732701633609,
0.));
#152314=CARTESIAN_POINT('Ctrl Pts',(-50.4672734191756,53.5732701633609,
12.));
#152315=CARTESIAN_POINT('Ctrl Pts',(-50.4580897717838,53.5482210307868,
0.));
#152316=CARTESIAN_POINT('Ctrl Pts',(-50.4580897717838,53.5482210307868,
12.));
#152317=CARTESIAN_POINT('Ctrl Pts',(-50.4488957368839,53.5232149426413,
0.));
#152318=CARTESIAN_POINT('Ctrl Pts',(-50.4488957368839,53.5232149426413,
12.));
#152319=CARTESIAN_POINT('Ctrl Pts',(-50.4396913921382,53.4982519688024,
0.));
#152320=CARTESIAN_POINT('Ctrl Pts',(-50.4396913921382,53.4982519688024,
12.));
#152321=CARTESIAN_POINT('Ctrl Pts',(-50.4304768156667,53.4733321794188,
0.));
#152322=CARTESIAN_POINT('Ctrl Pts',(-50.4304768156667,53.4733321794188,
12.));
#152323=CARTESIAN_POINT('Ctrl Pts',(-50.4212520859914,53.4484556448776,
0.));
#152324=CARTESIAN_POINT('Ctrl Pts',(-50.4212520859914,53.4484556448776,
12.));
#152325=CARTESIAN_POINT('Ctrl Pts',(-50.4120172820047,53.4236224357838,
0.));
#152326=CARTESIAN_POINT('Ctrl Pts',(-50.4120172820047,53.4236224357838,
12.));
#152327=CARTESIAN_POINT('Ctrl Pts',(-50.4027724829297,53.398832622931,0.));
#152328=CARTESIAN_POINT('Ctrl Pts',(-50.4027724829297,53.398832622931,12.));
#152329=CARTESIAN_POINT('Ctrl Pts',(-50.3935177682837,53.3740862772681,
0.));
#152330=CARTESIAN_POINT('Ctrl Pts',(-50.3935177682837,53.3740862772681,
12.));
#152331=CARTESIAN_POINT('Ctrl Pts',(-50.384253217846,53.3493834698697,0.));
#152332=CARTESIAN_POINT('Ctrl Pts',(-50.384253217846,53.3493834698697,12.));
#152333=CARTESIAN_POINT('Ctrl Pts',(-50.3749789116786,53.3247242719587,
0.));
#152334=CARTESIAN_POINT('Ctrl Pts',(-50.3749789116786,53.3247242719587,
12.));
#152335=CARTESIAN_POINT('Ctrl Pts',(-50.365694930143,53.300108754923,0.));
#152336=CARTESIAN_POINT('Ctrl Pts',(-50.365694930143,53.300108754923,12.));
#152337=CARTESIAN_POINT('Ctrl Pts',(-50.3564013539199,53.2755369903293,
0.));
#152338=CARTESIAN_POINT('Ctrl Pts',(-50.3564013539199,53.2755369903293,
12.));
#152339=CARTESIAN_POINT('Ctrl Pts',(-50.3470982640289,53.2510090499336,
0.));
#152340=CARTESIAN_POINT('Ctrl Pts',(-50.3470982640289,53.2510090499336,
12.));
#152341=CARTESIAN_POINT('Ctrl Pts',(-50.3377857418514,53.2265250056887,
0.));
#152342=CARTESIAN_POINT('Ctrl Pts',(-50.3377857418514,53.2265250056887,
12.));
#152343=CARTESIAN_POINT('Ctrl Pts',(-50.3284638691278,53.2020849297471,
0.));
#152344=CARTESIAN_POINT('Ctrl Pts',(-50.3284638691278,53.2020849297471,
12.));
#152345=CARTESIAN_POINT('Ctrl Pts',(-50.3191327279493,53.1776888944616,
0.));
#152346=CARTESIAN_POINT('Ctrl Pts',(-50.3191327279493,53.1776888944616,
12.));
#152347=CARTESIAN_POINT('Ctrl Pts',(-50.3097924007534,53.1533369723818,
0.));
#152348=CARTESIAN_POINT('Ctrl Pts',(-50.3097924007534,53.1533369723818,
12.));
#152349=CARTESIAN_POINT('Ctrl Pts',(-50.300442970319,53.1290292362485,0.));
#152350=CARTESIAN_POINT('Ctrl Pts',(-50.300442970319,53.1290292362485,12.));
#152351=CARTESIAN_POINT('Ctrl Pts',(-50.2910845197619,53.1047657589812,
0.));
#152352=CARTESIAN_POINT('Ctrl Pts',(-50.2910845197619,53.1047657589812,
12.));
#152353=CARTESIAN_POINT('Ctrl Pts',(-50.2817171325358,53.0805466136797,
0.));
#152354=CARTESIAN_POINT('Ctrl Pts',(-50.2817171325358,53.0805466136797,
12.));
#152355=CARTESIAN_POINT('Ctrl Pts',(-50.2723408924373,53.0563718736366,
0.));
#152356=CARTESIAN_POINT('Ctrl Pts',(-50.2723408924373,53.0563718736366,
12.));
#152357=CARTESIAN_POINT('Ctrl Pts',(-50.2629558836111,53.0322416123406,
0.));
#152358=CARTESIAN_POINT('Ctrl Pts',(-50.2629558836111,53.0322416123406,
12.));
#152359=CARTESIAN_POINT('Ctrl Pts',(-50.2535621905552,53.0081559034801,
0.));
#152360=CARTESIAN_POINT('Ctrl Pts',(-50.2535621905552,53.0081559034801,
12.));
#152361=CARTESIAN_POINT('Ctrl Pts',(-50.2441598981286,52.9841148209402,
0.));
#152362=CARTESIAN_POINT('Ctrl Pts',(-50.2441598981286,52.9841148209402,
12.));
#152363=CARTESIAN_POINT('Ctrl Pts',(-50.2347490915555,52.9601184388027,
0.));
#152364=CARTESIAN_POINT('Ctrl Pts',(-50.2347490915555,52.9601184388027,
12.));
#152365=CARTESIAN_POINT('Ctrl Pts',(-50.2253298564241,52.9361668313542,
0.));
#152366=CARTESIAN_POINT('Ctrl Pts',(-50.2253298564241,52.9361668313542,
12.));
#152367=CARTESIAN_POINT('Ctrl Pts',(-50.2159022786879,52.9122600730884,
0.));
#152368=CARTESIAN_POINT('Ctrl Pts',(-50.2159022786879,52.9122600730884,
12.));
#152369=CARTESIAN_POINT('Ctrl Pts',(-50.2064664446663,52.8883982387068,
0.));
#152370=CARTESIAN_POINT('Ctrl Pts',(-50.2064664446663,52.8883982387068,
12.));
#152371=CARTESIAN_POINT('Ctrl Pts',(-50.1970224410471,52.8645814031133,
0.));
#152372=CARTESIAN_POINT('Ctrl Pts',(-50.1970224410471,52.8645814031133,
12.));
#152373=CARTESIAN_POINT('Ctrl Pts',(-50.1875703548884,52.8408096414093,
0.));
#152374=CARTESIAN_POINT('Ctrl Pts',(-50.1875703548884,52.8408096414093,
12.));
#152375=CARTESIAN_POINT('Ctrl Pts',(-50.1781102736205,52.8170830289044,
0.));
#152376=CARTESIAN_POINT('Ctrl Pts',(-50.1781102736205,52.8170830289044,
12.));
#152377=CARTESIAN_POINT('Ctrl Pts',(-50.1686422850488,52.7934016411205,
0.));
#152378=CARTESIAN_POINT('Ctrl Pts',(-50.1686422850488,52.7934016411205,
12.));
#152379=CARTESIAN_POINT('Ctrl Pts',(-50.1591664773561,52.769765553794,0.));
#152380=CARTESIAN_POINT('Ctrl Pts',(-50.1591664773561,52.769765553794,12.));
#152381=CARTESIAN_POINT('Ctrl Pts',(-50.1496829391073,52.7461748428738,
0.));
#152382=CARTESIAN_POINT('Ctrl Pts',(-50.1496829391073,52.7461748428738,
12.));
#152383=CARTESIAN_POINT('Ctrl Pts',(-50.1401917592537,52.7226295845161,
0.));
#152384=CARTESIAN_POINT('Ctrl Pts',(-50.1401917592537,52.7226295845161,
12.));
#152385=CARTESIAN_POINT('Ctrl Pts',(-50.1306930271345,52.699129855093,0.));
#152386=CARTESIAN_POINT('Ctrl Pts',(-50.1306930271345,52.699129855093,12.));
#152387=CARTESIAN_POINT('Ctrl Pts',(-50.1211868324781,52.6756757311978,
0.));
#152388=CARTESIAN_POINT('Ctrl Pts',(-50.1211868324781,52.6756757311978,
12.));
#152389=CARTESIAN_POINT('Ctrl Pts',(-50.111673265404,52.652267289646,0.));
#152390=CARTESIAN_POINT('Ctrl Pts',(-50.111673265404,52.652267289646,12.));
#152391=CARTESIAN_POINT('Ctrl Pts',(-50.1021524164264,52.6289046074746,
0.));
#152392=CARTESIAN_POINT('Ctrl Pts',(-50.1021524164264,52.6289046074746,
12.));
#152393=CARTESIAN_POINT('Ctrl Pts',(-50.0926243764578,52.6055877619348,
0.));
#152394=CARTESIAN_POINT('Ctrl Pts',(-50.0926243764578,52.6055877619348,
12.));
#152395=CARTESIAN_POINT('Ctrl Pts',(-50.0830892368107,52.5823168304994,
0.));
#152396=CARTESIAN_POINT('Ctrl Pts',(-50.0830892368107,52.5823168304994,
12.));
#152397=CARTESIAN_POINT('Ctrl Pts',(-50.0735470892007,52.5590918908702,
0.));
#152398=CARTESIAN_POINT('Ctrl Pts',(-50.0735470892007,52.5590918908702,
12.));
#152399=CARTESIAN_POINT('Ctrl Pts',(-50.0639980257479,52.5359130209792,
0.));
#152400=CARTESIAN_POINT('Ctrl Pts',(-50.0639980257479,52.5359130209792,
12.));
#152401=CARTESIAN_POINT('Ctrl Pts',(-50.0544421389818,52.5127802989896,
0.));
#152402=CARTESIAN_POINT('Ctrl Pts',(-50.0544421389818,52.5127802989896,
12.));
#152403=CARTESIAN_POINT('Ctrl Pts',(-50.0448795218441,52.4896938032884,
0.));
#152404=CARTESIAN_POINT('Ctrl Pts',(-50.0448795218441,52.4896938032884,
12.));
#152405=CARTESIAN_POINT('Ctrl Pts',(-50.0353102676921,52.4666536124913,
0.));
#152406=CARTESIAN_POINT('Ctrl Pts',(-50.0353102676921,52.4666536124913,
12.));
#152407=CARTESIAN_POINT('Ctrl Pts',(-50.0257344703,52.4436598054515,0.));
#152408=CARTESIAN_POINT('Ctrl Pts',(-50.0257344703,52.4436598054515,12.));
#152409=CARTESIAN_POINT('Ctrl Pts',(-50.0161522238616,52.4207124612608,
0.));
#152410=CARTESIAN_POINT('Ctrl Pts',(-50.0161522238616,52.4207124612608,
12.));
#152411=CARTESIAN_POINT('Ctrl Pts',(-50.0065636229938,52.3978116592509,
0.));
#152412=CARTESIAN_POINT('Ctrl Pts',(-50.0065636229938,52.3978116592509,
12.));
#152413=CARTESIAN_POINT('Ctrl Pts',(-49.9969687627408,52.3749574789871,
0.));
#152414=CARTESIAN_POINT('Ctrl Pts',(-49.9969687627408,52.3749574789871,
12.));
#152415=CARTESIAN_POINT('Ctrl Pts',(-49.9873677385775,52.3521500002718,
0.));
#152416=CARTESIAN_POINT('Ctrl Pts',(-49.9873677385775,52.3521500002718,
12.));
#152417=CARTESIAN_POINT('Ctrl Pts',(-49.9777606464106,52.3293893031528,
0.));
#152418=CARTESIAN_POINT('Ctrl Pts',(-49.9777606464106,52.3293893031528,
12.));
#152419=CARTESIAN_POINT('Ctrl Pts',(-49.9681475825824,52.3066754679265,
0.));
#152420=CARTESIAN_POINT('Ctrl Pts',(-49.9681475825824,52.3066754679265,
12.));
#152421=CARTESIAN_POINT('Ctrl Pts',(-49.9585286438733,52.2840085751384,
0.));
#152422=CARTESIAN_POINT('Ctrl Pts',(-49.9585286438733,52.2840085751384,
12.));
#152423=CARTESIAN_POINT('Ctrl Pts',(-49.9489039275064,52.2613887055773,
0.));
#152424=CARTESIAN_POINT('Ctrl Pts',(-49.9489039275064,52.2613887055773,
12.));
#152425=CARTESIAN_POINT('Ctrl Pts',(-49.9392735311509,52.2388159402771,
0.));
#152426=CARTESIAN_POINT('Ctrl Pts',(-49.9392735311509,52.2388159402771,
12.));
#152427=CARTESIAN_POINT('Ctrl Pts',(-49.9296375529245,52.2162903605275,
0.));
#152428=CARTESIAN_POINT('Ctrl Pts',(-49.9296375529245,52.2162903605275,
12.));
#152429=CARTESIAN_POINT('Ctrl Pts',(-49.9199960913962,52.1938120478754,
0.));
#152430=CARTESIAN_POINT('Ctrl Pts',(-49.9199960913962,52.1938120478754,
12.));
#152431=CARTESIAN_POINT('Ctrl Pts',(-49.9103492455902,52.1713810841276,
0.));
#152432=CARTESIAN_POINT('Ctrl Pts',(-49.9103492455902,52.1713810841276,
12.));
#152433=CARTESIAN_POINT('Ctrl Pts',(-49.9006971149895,52.1489975513444,
0.));
#152434=CARTESIAN_POINT('Ctrl Pts',(-49.9006971149895,52.1489975513444,
12.));
#152435=CARTESIAN_POINT('Ctrl Pts',(-49.8910397995397,52.1266615318407,
0.));
#152436=CARTESIAN_POINT('Ctrl Pts',(-49.8910397995397,52.1266615318407,
12.));
#152437=CARTESIAN_POINT('Ctrl Pts',(-49.8813773996517,52.1043731081962,
0.));
#152438=CARTESIAN_POINT('Ctrl Pts',(-49.8813773996517,52.1043731081962,
12.));
#152439=CARTESIAN_POINT('Ctrl Pts',(-49.8717100162048,52.0821323632587,
0.));
#152440=CARTESIAN_POINT('Ctrl Pts',(-49.8717100162048,52.0821323632587,
12.));
#152441=CARTESIAN_POINT('Ctrl Pts',(-49.86203775055,52.0599393801452,0.));
#152442=CARTESIAN_POINT('Ctrl Pts',(-49.86203775055,52.0599393801452,12.));
#152443=CARTESIAN_POINT('Ctrl Pts',(-49.8523607045149,52.0377942422376,
0.));
#152444=CARTESIAN_POINT('Ctrl Pts',(-49.8523607045149,52.0377942422376,
12.));
#152445=CARTESIAN_POINT('Ctrl Pts',(-49.8426789804071,52.0156970331822,
0.));
#152446=CARTESIAN_POINT('Ctrl Pts',(-49.8426789804071,52.0156970331822,
12.));
#152447=CARTESIAN_POINT('Ctrl Pts',(-49.8329926810172,51.9936478369008,
0.));
#152448=CARTESIAN_POINT('Ctrl Pts',(-49.8329926810172,51.9936478369008,
12.));
#152449=CARTESIAN_POINT('Ctrl Pts',(-49.8233019096222,51.9716467375937,
0.));
#152450=CARTESIAN_POINT('Ctrl Pts',(-49.8233019096222,51.9716467375937,
12.));
#152451=CARTESIAN_POINT('Ctrl Pts',(-49.8136067699896,51.9496938197418,
0.));
#152452=CARTESIAN_POINT('Ctrl Pts',(-49.8136067699896,51.9496938197418,
12.));
#152453=CARTESIAN_POINT('Ctrl Pts',(-49.8039073663812,51.9277891681018,
0.));
#152454=CARTESIAN_POINT('Ctrl Pts',(-49.8039073663812,51.9277891681018,
12.));
#152455=CARTESIAN_POINT('Ctrl Pts',(-49.7942038035576,51.9059328677059,
0.));
#152456=CARTESIAN_POINT('Ctrl Pts',(-49.7942038035576,51.9059328677059,
12.));
#152457=CARTESIAN_POINT('Ctrl Pts',(-49.7844961867807,51.8841250038724,
0.));
#152458=CARTESIAN_POINT('Ctrl Pts',(-49.7844961867807,51.8841250038724,
12.));
#152459=CARTESIAN_POINT('Ctrl Pts',(-49.7747846218182,51.8623656622097,
0.));
#152460=CARTESIAN_POINT('Ctrl Pts',(-49.7747846218182,51.8623656622097,
12.));
#152461=CARTESIAN_POINT('Ctrl Pts',(-49.7650692149462,51.8406549286175,
0.));
#152462=CARTESIAN_POINT('Ctrl Pts',(-49.7650692149462,51.8406549286175,
12.));
#152463=CARTESIAN_POINT('Ctrl Pts',(-49.755350072955,51.8189928892828,0.));
#152464=CARTESIAN_POINT('Ctrl Pts',(-49.755350072955,51.8189928892828,12.));
#152465=CARTESIAN_POINT('Ctrl Pts',(-49.7456273031534,51.7973796306803,
0.));
#152466=CARTESIAN_POINT('Ctrl Pts',(-49.7456273031534,51.7973796306803,
12.));
#152467=CARTESIAN_POINT('Ctrl Pts',(-49.7359010133721,51.7758152395836,
0.));
#152468=CARTESIAN_POINT('Ctrl Pts',(-49.7359010133721,51.7758152395836,
12.));
#152469=CARTESIAN_POINT('Ctrl Pts',(-49.7261713119663,51.754299803067,0.));
#152470=CARTESIAN_POINT('Ctrl Pts',(-49.7261713119663,51.754299803067,12.));
#152471=CARTESIAN_POINT('Ctrl Pts',(-49.7164383078212,51.7328334085091,
0.));
#152472=CARTESIAN_POINT('Ctrl Pts',(-49.7164383078212,51.7328334085091,
12.));
#152473=CARTESIAN_POINT('Ctrl Pts',(-49.7067021103553,51.7114161435869,
0.));
#152474=CARTESIAN_POINT('Ctrl Pts',(-49.7067021103553,51.7114161435869,
12.));
#152475=CARTESIAN_POINT('Ctrl Pts',(-49.6969628295262,51.6900480962773,
0.));
#152476=CARTESIAN_POINT('Ctrl Pts',(-49.6969628295262,51.6900480962773,
12.));
#152477=CARTESIAN_POINT('Ctrl Pts',(-49.6872205758336,51.6687293548682,
0.));
#152478=CARTESIAN_POINT('Ctrl Pts',(-49.6872205758336,51.6687293548682,
12.));
#152479=CARTESIAN_POINT('Ctrl Pts',(-49.6774754603245,51.6474600079622,
0.));
#152480=CARTESIAN_POINT('Ctrl Pts',(-49.6774754603245,51.6474600079622,
12.));
#152481=CARTESIAN_POINT('Ctrl Pts',(-49.6677275945967,51.626240144479,0.));
#152482=CARTESIAN_POINT('Ctrl Pts',(-49.6677275945967,51.626240144479,12.));
#152483=CARTESIAN_POINT('Ctrl Pts',(-49.6579770908037,51.6050698536496,
0.));
#152484=CARTESIAN_POINT('Ctrl Pts',(-49.6579770908037,51.6050698536496,
12.));
#152485=CARTESIAN_POINT('Ctrl Pts',(-49.6482240616593,51.5839492250181,
0.));
#152486=CARTESIAN_POINT('Ctrl Pts',(-49.6482240616593,51.5839492250181,
12.));
#152487=CARTESIAN_POINT('Ctrl Pts',(-49.6384686204413,51.5628783484525,
0.));
#152488=CARTESIAN_POINT('Ctrl Pts',(-49.6384686204413,51.5628783484525,
12.));
#152489=CARTESIAN_POINT('Ctrl Pts',(-49.6287108809966,51.5418573141484,
0.));
#152490=CARTESIAN_POINT('Ctrl Pts',(-49.6287108809966,51.5418573141484,
12.));
#152491=CARTESIAN_POINT('Ctrl Pts',(-49.6189509577452,51.5208862126315,
0.));
#152492=CARTESIAN_POINT('Ctrl Pts',(-49.6189509577452,51.5208862126315,
12.));
#152493=CARTESIAN_POINT('Ctrl Pts',(-49.6091889656866,51.4999651347522,
0.));
#152494=CARTESIAN_POINT('Ctrl Pts',(-49.6091889656866,51.4999651347522,
12.));
#152495=CARTESIAN_POINT('Ctrl Pts',(-49.5994250204031,51.4790941716888,
0.));
#152496=CARTESIAN_POINT('Ctrl Pts',(-49.5994250204031,51.4790941716888,
12.));
#152497=CARTESIAN_POINT('Ctrl Pts',(-49.5896592380654,51.4582734149583,
0.));
#152498=CARTESIAN_POINT('Ctrl Pts',(-49.5896592380654,51.4582734149583,
12.));
#152499=CARTESIAN_POINT('Ctrl Pts',(-49.5798917354366,51.4375029564197,
0.));
#152500=CARTESIAN_POINT('Ctrl Pts',(-49.5798917354366,51.4375029564197,
12.));
#152501=CARTESIAN_POINT('Ctrl Pts',(-49.5701226298769,51.4167828882756,
0.));
#152502=CARTESIAN_POINT('Ctrl Pts',(-49.5701226298769,51.4167828882756,
12.));
#152503=CARTESIAN_POINT('Ctrl Pts',(-49.5603520393496,51.396113303067,0.));
#152504=CARTESIAN_POINT('Ctrl Pts',(-49.5603520393496,51.396113303067,12.));
#152505=CARTESIAN_POINT('Ctrl Pts',(-49.550580082425,51.3754942936778,0.));
#152506=CARTESIAN_POINT('Ctrl Pts',(-49.550580082425,51.3754942936778,12.));
#152507=CARTESIAN_POINT('Ctrl Pts',(-49.5408068782859,51.3549259533458,
0.));
#152508=CARTESIAN_POINT('Ctrl Pts',(-49.5408068782859,51.3549259533458,
12.));
#152509=CARTESIAN_POINT('Ctrl Pts',(-49.5310325467332,51.3344083756657,
0.));
#152510=CARTESIAN_POINT('Ctrl Pts',(-49.5310325467332,51.3344083756657,
12.));
#152511=CARTESIAN_POINT('Ctrl Pts',(-49.5212572081908,51.313941654591,0.));
#152512=CARTESIAN_POINT('Ctrl Pts',(-49.5212572081908,51.313941654591,12.));
#152513=CARTESIAN_POINT('Ctrl Pts',(-49.5114809837122,51.2935258844289,
0.));
#152514=CARTESIAN_POINT('Ctrl Pts',(-49.5114809837122,51.2935258844289,
12.));
#152515=CARTESIAN_POINT('Ctrl Pts',(-49.5017039949852,51.2731611598475,
0.));
#152516=CARTESIAN_POINT('Ctrl Pts',(-49.5017039949852,51.2731611598475,
12.));
#152517=CARTESIAN_POINT('Ctrl Pts',(-49.4919263643362,51.2528475758846,
0.));
#152518=CARTESIAN_POINT('Ctrl Pts',(-49.4919263643362,51.2528475758846,
12.));
#152519=CARTESIAN_POINT('Ctrl Pts',(-49.4821482147356,51.2325852279506,
0.));
#152520=CARTESIAN_POINT('Ctrl Pts',(-49.4821482147356,51.2325852279506,
12.));
#152521=CARTESIAN_POINT('Ctrl Pts',(-49.4723696698021,51.2123742118287,
0.));
#152522=CARTESIAN_POINT('Ctrl Pts',(-49.4723696698021,51.2123742118287,
12.));
#152523=CARTESIAN_POINT('Ctrl Pts',(-49.4625908538074,51.1922146236686,
0.));
#152524=CARTESIAN_POINT('Ctrl Pts',(-49.4625908538074,51.1922146236686,
12.));
#152525=CARTESIAN_POINT('Ctrl Pts',(-49.4528118916832,51.1721065599972,
0.));
#152526=CARTESIAN_POINT('Ctrl Pts',(-49.4528118916832,51.1721065599972,
12.));
#152527=CARTESIAN_POINT('Ctrl Pts',(-49.4430329090287,51.1520501177291,
0.));
#152528=CARTESIAN_POINT('Ctrl Pts',(-49.4430329090287,51.1520501177291,
12.));
#152529=CARTESIAN_POINT('Ctrl Pts',(-49.4332540321178,51.1320453941702,
0.));
#152530=CARTESIAN_POINT('Ctrl Pts',(-49.4332540321178,51.1320453941702,
12.));
#152531=CARTESIAN_POINT('Ctrl Pts',(-49.423475387907,51.1120924870195,0.));
#152532=CARTESIAN_POINT('Ctrl Pts',(-49.423475387907,51.1120924870195,12.));
#152533=CARTESIAN_POINT('Ctrl Pts',(-49.4136971040428,51.0921914943662,
0.));
#152534=CARTESIAN_POINT('Ctrl Pts',(-49.4136971040428,51.0921914943662,
12.));
#152535=CARTESIAN_POINT('Ctrl Pts',(-49.4039193088634,51.0723425146985,
0.));
#152536=CARTESIAN_POINT('Ctrl Pts',(-49.4039193088634,51.0723425146985,
12.));
#152537=CARTESIAN_POINT('Ctrl Pts',(-49.3941421314013,51.052545646907,0.));
#152538=CARTESIAN_POINT('Ctrl Pts',(-49.3941421314013,51.052545646907,12.));
#152539=CARTESIAN_POINT('Ctrl Pts',(-49.3843657013852,51.0328009902858,
0.));
#152540=CARTESIAN_POINT('Ctrl Pts',(-49.3843657013852,51.0328009902858,
12.));
#152541=CARTESIAN_POINT('Ctrl Pts',(-49.3745901492432,51.0131086445272,
0.));
#152542=CARTESIAN_POINT('Ctrl Pts',(-49.3745901492432,51.0131086445272,
12.));
#152543=CARTESIAN_POINT('Ctrl Pts',(-49.3648156061058,50.9934687097188,
0.));
#152544=CARTESIAN_POINT('Ctrl Pts',(-49.3648156061058,50.9934687097188,
12.));
#152545=CARTESIAN_POINT('Ctrl Pts',(-49.355042203823,50.9738812863646,0.));
#152546=CARTESIAN_POINT('Ctrl Pts',(-49.355042203823,50.9738812863646,12.));
#152547=CARTESIAN_POINT('Ctrl Pts',(-49.345270074981,50.9543464753981,0.));
#152548=CARTESIAN_POINT('Ctrl Pts',(-49.345270074981,50.9543464753981,12.));
#152549=CARTESIAN_POINT('Ctrl Pts',(-49.3354993529158,50.9348643781924,
0.));
#152550=CARTESIAN_POINT('Ctrl Pts',(-49.3354993529158,50.9348643781924,
12.));
#152551=CARTESIAN_POINT('Ctrl Pts',(-49.3257301717335,50.9154350965666,
0.));
#152552=CARTESIAN_POINT('Ctrl Pts',(-49.3257301717335,50.9154350965666,
12.));
#152553=CARTESIAN_POINT('Ctrl Pts',(-49.3159626663109,50.8960587327848,
0.));
#152554=CARTESIAN_POINT('Ctrl Pts',(-49.3159626663109,50.8960587327848,
12.));
#152555=CARTESIAN_POINT('Ctrl Pts',(-49.3061969722781,50.8767353895492,
0.));
#152556=CARTESIAN_POINT('Ctrl Pts',(-49.3061969722781,50.8767353895492,
12.));
#152557=CARTESIAN_POINT('Ctrl Pts',(-49.2964332260039,50.8574651699873,
0.));
#152558=CARTESIAN_POINT('Ctrl Pts',(-49.2964332260039,50.8574651699873,
12.));
#152559=CARTESIAN_POINT('Ctrl Pts',(-49.2866715645838,50.8382481776403,
0.));
#152560=CARTESIAN_POINT('Ctrl Pts',(-49.2866715645838,50.8382481776403,
12.));
#152561=CARTESIAN_POINT('Ctrl Pts',(-49.2769121258164,50.819084516434,0.));
#152562=CARTESIAN_POINT('Ctrl Pts',(-49.2769121258164,50.819084516434,12.));
#152563=CARTESIAN_POINT('Ctrl Pts',(-49.2671550482435,50.7999742907131,
0.));
#152564=CARTESIAN_POINT('Ctrl Pts',(-49.2671550482435,50.7999742907131,
12.));
#152565=CARTESIAN_POINT('Ctrl Pts',(-49.2574004712134,50.7809176052966,
0.));
#152566=CARTESIAN_POINT('Ctrl Pts',(-49.2574004712134,50.7809176052966,
12.));
#152567=CARTESIAN_POINT('Ctrl Pts',(-49.2476485349373,50.7619145655207,
0.));
#152568=CARTESIAN_POINT('Ctrl Pts',(-49.2476485349373,50.7619145655207,
12.));
#152569=CARTESIAN_POINT('Ctrl Pts',(-49.2378993805471,50.7429652772805,
0.));
#152570=CARTESIAN_POINT('Ctrl Pts',(-49.2378993805471,50.7429652772805,
12.));
#152571=CARTESIAN_POINT('Ctrl Pts',(-49.228153150155,50.7240698470679,0.));
#152572=CARTESIAN_POINT('Ctrl Pts',(-49.228153150155,50.7240698470679,12.));
#152573=CARTESIAN_POINT('Ctrl Pts',(-49.2184099867461,50.7052283818922,
0.));
#152574=CARTESIAN_POINT('Ctrl Pts',(-49.2184099867461,50.7052283818922,
12.));
#152575=CARTESIAN_POINT('Ctrl Pts',(-49.2086700340614,50.6864409891895,
0.));
#152576=CARTESIAN_POINT('Ctrl Pts',(-49.2086700340614,50.6864409891895,
12.));
#152577=CARTESIAN_POINT('Ctrl Pts',(-49.1989334364996,50.6677077767432,
0.));
#152578=CARTESIAN_POINT('Ctrl Pts',(-49.1989334364996,50.6677077767432,
12.));
#152579=CARTESIAN_POINT('Ctrl Pts',(-49.189200338976,50.6490288525656,0.));
#152580=CARTESIAN_POINT('Ctrl Pts',(-49.189200338976,50.6490288525656,12.));
#152581=CARTESIAN_POINT('Ctrl Pts',(-49.1794708869099,50.6304043248821,
0.));
#152582=CARTESIAN_POINT('Ctrl Pts',(-49.1794708869099,50.6304043248821,
12.));
#152583=CARTESIAN_POINT('Ctrl Pts',(-49.1697452265494,50.6118343023957,
0.));
#152584=CARTESIAN_POINT('Ctrl Pts',(-49.1697452265494,50.6118343023957,
12.));
#152585=CARTESIAN_POINT('Ctrl Pts',(-49.1600235052621,50.5933188945168,
0.));
#152586=CARTESIAN_POINT('Ctrl Pts',(-49.1600235052621,50.5933188945168,
12.));
#152587=CARTESIAN_POINT('Ctrl Pts',(-49.1503058717821,50.5748582115565,
0.));
#152588=CARTESIAN_POINT('Ctrl Pts',(-49.1503058717821,50.5748582115565,
12.));
#152589=CARTESIAN_POINT('Ctrl Pts',(-49.1405924766144,50.556452365038,0.));
#152590=CARTESIAN_POINT('Ctrl Pts',(-49.1405924766144,50.556452365038,12.));
#152591=CARTESIAN_POINT('Ctrl Pts',(-49.1308834717615,50.5381014674791,
0.));
#152592=CARTESIAN_POINT('Ctrl Pts',(-49.1308834717615,50.5381014674791,
12.));
#152593=CARTESIAN_POINT('Ctrl Pts',(-49.1211790099795,50.5198056318088,
0.));
#152594=CARTESIAN_POINT('Ctrl Pts',(-49.1211790099795,50.5198056318088,
12.));
#152595=CARTESIAN_POINT('Ctrl Pts',(-49.1114792441571,50.501564970874,0.));
#152596=CARTESIAN_POINT('Ctrl Pts',(-49.1114792441571,50.501564970874,12.));
#152597=CARTESIAN_POINT('Ctrl Pts',(-49.1017843266803,50.4833795969318,
0.));
#152598=CARTESIAN_POINT('Ctrl Pts',(-49.1017843266803,50.4833795969318,
12.));
#152599=CARTESIAN_POINT('Ctrl Pts',(-49.0920944087008,50.4652496210607,
0.));
#152600=CARTESIAN_POINT('Ctrl Pts',(-49.0920944087008,50.4652496210607,
12.));
#152601=CARTESIAN_POINT('Ctrl Pts',(-49.0824096415371,50.4471751542751,
0.));
#152602=CARTESIAN_POINT('Ctrl Pts',(-49.0824096415371,50.4471751542751,
12.));
#152603=CARTESIAN_POINT('Ctrl Pts',(-49.0727301783494,50.4291563088547,
0.));
#152604=CARTESIAN_POINT('Ctrl Pts',(-49.0727301783494,50.4291563088547,
12.));
#152605=CARTESIAN_POINT('Ctrl Pts',(-49.0630561755075,50.4111931994257,
0.));
#152606=CARTESIAN_POINT('Ctrl Pts',(-49.0630561755075,50.4111931994257,
12.));
#152607=CARTESIAN_POINT('Ctrl Pts',(-49.0533877945744,50.3932859445252,
0.));
#152608=CARTESIAN_POINT('Ctrl Pts',(-49.0533877945744,50.3932859445252,
12.));
#152609=CARTESIAN_POINT('Ctrl Pts',(-49.0437252024832,50.3754346667353,
0.));
#152610=CARTESIAN_POINT('Ctrl Pts',(-49.0437252024832,50.3754346667353,
12.));
#152611=CARTESIAN_POINT('Ctrl Pts',(-49.0340685673982,50.3576394894108,
0.));
#152612=CARTESIAN_POINT('Ctrl Pts',(-49.0340685673982,50.3576394894108,
12.));
#152613=CARTESIAN_POINT('Ctrl Pts',(-49.024418055075,50.3399005337958,0.));
#152614=CARTESIAN_POINT('Ctrl Pts',(-49.024418055075,50.3399005337958,12.));
#152615=CARTESIAN_POINT('Ctrl Pts',(-49.0147738256942,50.3222179165119,
0.));
#152616=CARTESIAN_POINT('Ctrl Pts',(-49.0147738256942,50.3222179165119,
12.));
#152617=CARTESIAN_POINT('Ctrl Pts',(-49.0051360288044,50.3045917455424,
0.));
#152618=CARTESIAN_POINT('Ctrl Pts',(-49.0051360288044,50.3045917455424,
12.));
#152619=CARTESIAN_POINT('Ctrl Pts',(-48.9955048082081,50.2870221241054,
0.));
#152620=CARTESIAN_POINT('Ctrl Pts',(-48.9955048082081,50.2870221241054,
12.));
#152621=CARTESIAN_POINT('Ctrl Pts',(-48.9858803116689,50.2695091583511,
0.));
#152622=CARTESIAN_POINT('Ctrl Pts',(-48.9858803116689,50.2695091583511,
12.));
#152623=CARTESIAN_POINT('Ctrl Pts',(-48.9762626987227,50.252052963548,0.));
#152624=CARTESIAN_POINT('Ctrl Pts',(-48.9762626987227,50.252052963548,12.));
#152625=CARTESIAN_POINT('Ctrl Pts',(-48.9666521500911,50.234653671541,0.));
#152626=CARTESIAN_POINT('Ctrl Pts',(-48.9666521500911,50.234653671541,12.));
#152627=CARTESIAN_POINT('Ctrl Pts',(-48.9570488741167,50.2173114358325,
0.));
#152628=CARTESIAN_POINT('Ctrl Pts',(-48.9570488741167,50.2173114358325,
12.));
#152629=CARTESIAN_POINT('Ctrl Pts',(-48.9474530868733,50.2000264157797,
0.));
#152630=CARTESIAN_POINT('Ctrl Pts',(-48.9474530868733,50.2000264157797,
12.));
#152631=CARTESIAN_POINT('Ctrl Pts',(-48.9378649933055,50.1827987615602,
0.));
#152632=CARTESIAN_POINT('Ctrl Pts',(-48.9378649933055,50.1827987615602,
12.));
#152633=CARTESIAN_POINT('Ctrl Pts',(-48.9282847698294,50.1656286003997,
0.));
#152634=CARTESIAN_POINT('Ctrl Pts',(-48.9282847698294,50.1656286003997,
12.));
#152635=CARTESIAN_POINT('Ctrl Pts',(-48.9187125418099,50.1485160184657,
0.));
#152636=CARTESIAN_POINT('Ctrl Pts',(-48.9187125418099,50.1485160184657,
12.));
#152637=CARTESIAN_POINT('Ctrl Pts',(-48.90914838181,50.1314610602569,0.));
#152638=CARTESIAN_POINT('Ctrl Pts',(-48.90914838181,50.1314610602569,12.));
#152639=CARTESIAN_POINT('Ctrl Pts',(-48.9015035372055,50.1178632067084,
0.));
#152640=CARTESIAN_POINT('Ctrl Pts',(-48.9015035372055,50.1178632067084,
12.));
#152641=CARTESIAN_POINT('Ctrl Pts',(-48.895773555686,50.1076907555471,0.));
#152642=CARTESIAN_POINT('Ctrl Pts',(-48.895773555686,50.1076907555471,12.));
#152643=CARTESIAN_POINT('Ctrl Pts',(-48.8919551910366,50.1009206494272,
0.));
#152644=CARTESIAN_POINT('Ctrl Pts',(-48.8919551910366,50.1009206494272,
12.));
#152645=CARTESIAN_POINT('Ctrl Pts',(-48.8900464144686,50.0975384783635,
0.));
#152646=CARTESIAN_POINT('Ctrl Pts',(-48.8900464144686,50.0975384783635,
12.));
#152647=CARTESIAN_POINT('',(-48.8900464144686,50.0975384783635,12.));
#152648=CARTESIAN_POINT('Ctrl Pts',(-48.8900464144686,50.0975384783635,
12.));
#152649=CARTESIAN_POINT('Ctrl Pts',(-48.8919551910366,50.1009206494272,
12.));
#152650=CARTESIAN_POINT('Ctrl Pts',(-48.895773555686,50.1076907555471,12.));
#152651=CARTESIAN_POINT('Ctrl Pts',(-48.9015035372055,50.1178632067084,
12.));
#152652=CARTESIAN_POINT('Ctrl Pts',(-48.90914838181,50.1314610602569,12.));
#152653=CARTESIAN_POINT('Ctrl Pts',(-48.9187125418099,50.1485160184657,
12.));
#152654=CARTESIAN_POINT('Ctrl Pts',(-48.9282847698294,50.1656286003997,
12.));
#152655=CARTESIAN_POINT('Ctrl Pts',(-48.9378649933055,50.1827987615602,
12.));
#152656=CARTESIAN_POINT('Ctrl Pts',(-48.9474530868733,50.2000264157797,
12.));
#152657=CARTESIAN_POINT('Ctrl Pts',(-48.9570488741167,50.2173114358325,
12.));
#152658=CARTESIAN_POINT('Ctrl Pts',(-48.9666521500911,50.234653671541,12.));
#152659=CARTESIAN_POINT('Ctrl Pts',(-48.9762626987227,50.252052963548,12.));
#152660=CARTESIAN_POINT('Ctrl Pts',(-48.9858803116689,50.2695091583511,
12.));
#152661=CARTESIAN_POINT('Ctrl Pts',(-48.9955048082081,50.2870221241054,
12.));
#152662=CARTESIAN_POINT('Ctrl Pts',(-49.0051360288044,50.3045917455424,
12.));
#152663=CARTESIAN_POINT('Ctrl Pts',(-49.0147738256942,50.3222179165119,
12.));
#152664=CARTESIAN_POINT('Ctrl Pts',(-49.024418055075,50.3399005337958,12.));
#152665=CARTESIAN_POINT('Ctrl Pts',(-49.0340685673982,50.3576394894108,
12.));
#152666=CARTESIAN_POINT('Ctrl Pts',(-49.0437252024832,50.3754346667353,
12.));
#152667=CARTESIAN_POINT('Ctrl Pts',(-49.0533877945744,50.3932859445252,
12.));
#152668=CARTESIAN_POINT('Ctrl Pts',(-49.0630561755075,50.4111931994257,
12.));
#152669=CARTESIAN_POINT('Ctrl Pts',(-49.0727301783494,50.4291563088547,
12.));
#152670=CARTESIAN_POINT('Ctrl Pts',(-49.0824096415371,50.4471751542751,
12.));
#152671=CARTESIAN_POINT('Ctrl Pts',(-49.0920944087008,50.4652496210607,
12.));
#152672=CARTESIAN_POINT('Ctrl Pts',(-49.1017843266803,50.4833795969318,
12.));
#152673=CARTESIAN_POINT('Ctrl Pts',(-49.1114792441571,50.501564970874,12.));
#152674=CARTESIAN_POINT('Ctrl Pts',(-49.1211790099795,50.5198056318088,
12.));
#152675=CARTESIAN_POINT('Ctrl Pts',(-49.1308834717615,50.5381014674791,
12.));
#152676=CARTESIAN_POINT('Ctrl Pts',(-49.1405924766144,50.556452365038,12.));
#152677=CARTESIAN_POINT('Ctrl Pts',(-49.1503058717821,50.5748582115565,
12.));
#152678=CARTESIAN_POINT('Ctrl Pts',(-49.1600235052621,50.5933188945168,
12.));
#152679=CARTESIAN_POINT('Ctrl Pts',(-49.1697452265494,50.6118343023957,
12.));
#152680=CARTESIAN_POINT('Ctrl Pts',(-49.1794708869099,50.6304043248821,
12.));
#152681=CARTESIAN_POINT('Ctrl Pts',(-49.189200338976,50.6490288525656,12.));
#152682=CARTESIAN_POINT('Ctrl Pts',(-49.1989334364996,50.6677077767432,
12.));
#152683=CARTESIAN_POINT('Ctrl Pts',(-49.2086700340614,50.6864409891895,
12.));
#152684=CARTESIAN_POINT('Ctrl Pts',(-49.2184099867461,50.7052283818922,
12.));
#152685=CARTESIAN_POINT('Ctrl Pts',(-49.228153150155,50.7240698470679,12.));
#152686=CARTESIAN_POINT('Ctrl Pts',(-49.2378993805471,50.7429652772805,
12.));
#152687=CARTESIAN_POINT('Ctrl Pts',(-49.2476485349373,50.7619145655207,
12.));
#152688=CARTESIAN_POINT('Ctrl Pts',(-49.2574004712134,50.7809176052966,
12.));
#152689=CARTESIAN_POINT('Ctrl Pts',(-49.2671550482435,50.7999742907131,
12.));
#152690=CARTESIAN_POINT('Ctrl Pts',(-49.2769121258164,50.819084516434,12.));
#152691=CARTESIAN_POINT('Ctrl Pts',(-49.2866715645838,50.8382481776403,
12.));
#152692=CARTESIAN_POINT('Ctrl Pts',(-49.2964332260039,50.8574651699873,
12.));
#152693=CARTESIAN_POINT('Ctrl Pts',(-49.3061969722781,50.8767353895492,
12.));
#152694=CARTESIAN_POINT('Ctrl Pts',(-49.3159626663109,50.8960587327848,
12.));
#152695=CARTESIAN_POINT('Ctrl Pts',(-49.3257301717335,50.9154350965666,
12.));
#152696=CARTESIAN_POINT('Ctrl Pts',(-49.3354993529158,50.9348643781924,
12.));
#152697=CARTESIAN_POINT('Ctrl Pts',(-49.345270074981,50.9543464753981,12.));
#152698=CARTESIAN_POINT('Ctrl Pts',(-49.355042203823,50.9738812863646,12.));
#152699=CARTESIAN_POINT('Ctrl Pts',(-49.3648156061058,50.9934687097188,
12.));
#152700=CARTESIAN_POINT('Ctrl Pts',(-49.3745901492432,51.0131086445272,
12.));
#152701=CARTESIAN_POINT('Ctrl Pts',(-49.3843657013852,51.0328009902858,
12.));
#152702=CARTESIAN_POINT('Ctrl Pts',(-49.3941421314013,51.052545646907,12.));
#152703=CARTESIAN_POINT('Ctrl Pts',(-49.4039193088634,51.0723425146985,
12.));
#152704=CARTESIAN_POINT('Ctrl Pts',(-49.4136971040428,51.0921914943662,
12.));
#152705=CARTESIAN_POINT('Ctrl Pts',(-49.423475387907,51.1120924870195,12.));
#152706=CARTESIAN_POINT('Ctrl Pts',(-49.4332540321178,51.1320453941702,
12.));
#152707=CARTESIAN_POINT('Ctrl Pts',(-49.4430329090287,51.1520501177291,
12.));
#152708=CARTESIAN_POINT('Ctrl Pts',(-49.4528118916832,51.1721065599972,
12.));
#152709=CARTESIAN_POINT('Ctrl Pts',(-49.4625908538074,51.1922146236686,
12.));
#152710=CARTESIAN_POINT('Ctrl Pts',(-49.4723696698021,51.2123742118287,
12.));
#152711=CARTESIAN_POINT('Ctrl Pts',(-49.4821482147356,51.2325852279506,
12.));
#152712=CARTESIAN_POINT('Ctrl Pts',(-49.4919263643362,51.2528475758846,
12.));
#152713=CARTESIAN_POINT('Ctrl Pts',(-49.5017039949852,51.2731611598475,
12.));
#152714=CARTESIAN_POINT('Ctrl Pts',(-49.5114809837122,51.2935258844289,
12.));
#152715=CARTESIAN_POINT('Ctrl Pts',(-49.5212572081908,51.313941654591,12.));
#152716=CARTESIAN_POINT('Ctrl Pts',(-49.5310325467332,51.3344083756657,
12.));
#152717=CARTESIAN_POINT('Ctrl Pts',(-49.5408068782859,51.3549259533458,
12.));
#152718=CARTESIAN_POINT('Ctrl Pts',(-49.550580082425,51.3754942936778,12.));
#152719=CARTESIAN_POINT('Ctrl Pts',(-49.5603520393496,51.396113303067,12.));
#152720=CARTESIAN_POINT('Ctrl Pts',(-49.5701226298769,51.4167828882756,
12.));
#152721=CARTESIAN_POINT('Ctrl Pts',(-49.5798917354366,51.4375029564197,
12.));
#152722=CARTESIAN_POINT('Ctrl Pts',(-49.5896592380654,51.4582734149583,
12.));
#152723=CARTESIAN_POINT('Ctrl Pts',(-49.5994250204031,51.4790941716888,
12.));
#152724=CARTESIAN_POINT('Ctrl Pts',(-49.6091889656866,51.4999651347522,
12.));
#152725=CARTESIAN_POINT('Ctrl Pts',(-49.6189509577452,51.5208862126315,
12.));
#152726=CARTESIAN_POINT('Ctrl Pts',(-49.6287108809966,51.5418573141484,
12.));
#152727=CARTESIAN_POINT('Ctrl Pts',(-49.6384686204413,51.5628783484525,
12.));
#152728=CARTESIAN_POINT('Ctrl Pts',(-49.6482240616593,51.5839492250181,
12.));
#152729=CARTESIAN_POINT('Ctrl Pts',(-49.6579770908037,51.6050698536496,
12.));
#152730=CARTESIAN_POINT('Ctrl Pts',(-49.6677275945967,51.626240144479,12.));
#152731=CARTESIAN_POINT('Ctrl Pts',(-49.6774754603245,51.6474600079622,
12.));
#152732=CARTESIAN_POINT('Ctrl Pts',(-49.6872205758336,51.6687293548682,
12.));
#152733=CARTESIAN_POINT('Ctrl Pts',(-49.6969628295262,51.6900480962773,
12.));
#152734=CARTESIAN_POINT('Ctrl Pts',(-49.7067021103553,51.7114161435869,
12.));
#152735=CARTESIAN_POINT('Ctrl Pts',(-49.7164383078212,51.7328334085091,
12.));
#152736=CARTESIAN_POINT('Ctrl Pts',(-49.7261713119663,51.754299803067,12.));
#152737=CARTESIAN_POINT('Ctrl Pts',(-49.7359010133721,51.7758152395836,
12.));
#152738=CARTESIAN_POINT('Ctrl Pts',(-49.7456273031534,51.7973796306803,
12.));
#152739=CARTESIAN_POINT('Ctrl Pts',(-49.755350072955,51.8189928892828,12.));
#152740=CARTESIAN_POINT('Ctrl Pts',(-49.7650692149462,51.8406549286175,
12.));
#152741=CARTESIAN_POINT('Ctrl Pts',(-49.7747846218182,51.8623656622097,
12.));
#152742=CARTESIAN_POINT('Ctrl Pts',(-49.7844961867807,51.8841250038724,
12.));
#152743=CARTESIAN_POINT('Ctrl Pts',(-49.7942038035576,51.9059328677059,
12.));
#152744=CARTESIAN_POINT('Ctrl Pts',(-49.8039073663812,51.9277891681018,
12.));
#152745=CARTESIAN_POINT('Ctrl Pts',(-49.8136067699896,51.9496938197418,
12.));
#152746=CARTESIAN_POINT('Ctrl Pts',(-49.8233019096222,51.9716467375937,
12.));
#152747=CARTESIAN_POINT('Ctrl Pts',(-49.8329926810172,51.9936478369008,
12.));
#152748=CARTESIAN_POINT('Ctrl Pts',(-49.8426789804071,52.0156970331822,
12.));
#152749=CARTESIAN_POINT('Ctrl Pts',(-49.8523607045149,52.0377942422376,
12.));
#152750=CARTESIAN_POINT('Ctrl Pts',(-49.86203775055,52.0599393801452,12.));
#152751=CARTESIAN_POINT('Ctrl Pts',(-49.8717100162048,52.0821323632587,
12.));
#152752=CARTESIAN_POINT('Ctrl Pts',(-49.8813773996517,52.1043731081962,
12.));
#152753=CARTESIAN_POINT('Ctrl Pts',(-49.8910397995397,52.1266615318407,
12.));
#152754=CARTESIAN_POINT('Ctrl Pts',(-49.9006971149895,52.1489975513444,
12.));
#152755=CARTESIAN_POINT('Ctrl Pts',(-49.9103492455902,52.1713810841276,
12.));
#152756=CARTESIAN_POINT('Ctrl Pts',(-49.9199960913962,52.1938120478754,
12.));
#152757=CARTESIAN_POINT('Ctrl Pts',(-49.9296375529245,52.2162903605275,
12.));
#152758=CARTESIAN_POINT('Ctrl Pts',(-49.9392735311509,52.2388159402771,
12.));
#152759=CARTESIAN_POINT('Ctrl Pts',(-49.9489039275064,52.2613887055773,
12.));
#152760=CARTESIAN_POINT('Ctrl Pts',(-49.9585286438733,52.2840085751384,
12.));
#152761=CARTESIAN_POINT('Ctrl Pts',(-49.9681475825824,52.3066754679265,
12.));
#152762=CARTESIAN_POINT('Ctrl Pts',(-49.9777606464106,52.3293893031528,
12.));
#152763=CARTESIAN_POINT('Ctrl Pts',(-49.9873677385775,52.3521500002718,
12.));
#152764=CARTESIAN_POINT('Ctrl Pts',(-49.9969687627408,52.3749574789871,
12.));
#152765=CARTESIAN_POINT('Ctrl Pts',(-50.0065636229938,52.3978116592509,
12.));
#152766=CARTESIAN_POINT('Ctrl Pts',(-50.0161522238616,52.4207124612608,
12.));
#152767=CARTESIAN_POINT('Ctrl Pts',(-50.0257344703,52.4436598054515,12.));
#152768=CARTESIAN_POINT('Ctrl Pts',(-50.0353102676921,52.4666536124913,
12.));
#152769=CARTESIAN_POINT('Ctrl Pts',(-50.0448795218441,52.4896938032884,
12.));
#152770=CARTESIAN_POINT('Ctrl Pts',(-50.0544421389818,52.5127802989896,
12.));
#152771=CARTESIAN_POINT('Ctrl Pts',(-50.0639980257479,52.5359130209792,
12.));
#152772=CARTESIAN_POINT('Ctrl Pts',(-50.0735470892007,52.5590918908702,
12.));
#152773=CARTESIAN_POINT('Ctrl Pts',(-50.0830892368107,52.5823168304994,
12.));
#152774=CARTESIAN_POINT('Ctrl Pts',(-50.0926243764578,52.6055877619348,
12.));
#152775=CARTESIAN_POINT('Ctrl Pts',(-50.1021524164264,52.6289046074746,
12.));
#152776=CARTESIAN_POINT('Ctrl Pts',(-50.111673265404,52.652267289646,12.));
#152777=CARTESIAN_POINT('Ctrl Pts',(-50.1211868324781,52.6756757311978,
12.));
#152778=CARTESIAN_POINT('Ctrl Pts',(-50.1306930271345,52.699129855093,12.));
#152779=CARTESIAN_POINT('Ctrl Pts',(-50.1401917592537,52.7226295845161,
12.));
#152780=CARTESIAN_POINT('Ctrl Pts',(-50.1496829391073,52.7461748428738,
12.));
#152781=CARTESIAN_POINT('Ctrl Pts',(-50.1591664773561,52.769765553794,12.));
#152782=CARTESIAN_POINT('Ctrl Pts',(-50.1686422850488,52.7934016411205,
12.));
#152783=CARTESIAN_POINT('Ctrl Pts',(-50.1781102736205,52.8170830289044,
12.));
#152784=CARTESIAN_POINT('Ctrl Pts',(-50.1875703548884,52.8408096414093,
12.));
#152785=CARTESIAN_POINT('Ctrl Pts',(-50.1970224410471,52.8645814031133,
12.));
#152786=CARTESIAN_POINT('Ctrl Pts',(-50.2064664446663,52.8883982387068,
12.));
#152787=CARTESIAN_POINT('Ctrl Pts',(-50.2159022786879,52.9122600730884,
12.));
#152788=CARTESIAN_POINT('Ctrl Pts',(-50.2253298564241,52.9361668313542,
12.));
#152789=CARTESIAN_POINT('Ctrl Pts',(-50.2347490915555,52.9601184388027,
12.));
#152790=CARTESIAN_POINT('Ctrl Pts',(-50.2441598981286,52.9841148209402,
12.));
#152791=CARTESIAN_POINT('Ctrl Pts',(-50.2535621905552,53.0081559034801,
12.));
#152792=CARTESIAN_POINT('Ctrl Pts',(-50.2629558836111,53.0322416123406,
12.));
#152793=CARTESIAN_POINT('Ctrl Pts',(-50.2723408924373,53.0563718736366,
12.));
#152794=CARTESIAN_POINT('Ctrl Pts',(-50.2817171325358,53.0805466136797,
12.));
#152795=CARTESIAN_POINT('Ctrl Pts',(-50.2910845197619,53.1047657589812,
12.));
#152796=CARTESIAN_POINT('Ctrl Pts',(-50.300442970319,53.1290292362485,12.));
#152797=CARTESIAN_POINT('Ctrl Pts',(-50.3097924007534,53.1533369723818,
12.));
#152798=CARTESIAN_POINT('Ctrl Pts',(-50.3191327279493,53.1776888944616,
12.));
#152799=CARTESIAN_POINT('Ctrl Pts',(-50.3284638691278,53.2020849297471,
12.));
#152800=CARTESIAN_POINT('Ctrl Pts',(-50.3377857418514,53.2265250056887,
12.));
#152801=CARTESIAN_POINT('Ctrl Pts',(-50.3470982640289,53.2510090499336,
12.));
#152802=CARTESIAN_POINT('Ctrl Pts',(-50.3564013539199,53.2755369903293,
12.));
#152803=CARTESIAN_POINT('Ctrl Pts',(-50.365694930143,53.300108754923,12.));
#152804=CARTESIAN_POINT('Ctrl Pts',(-50.3749789116786,53.3247242719587,
12.));
#152805=CARTESIAN_POINT('Ctrl Pts',(-50.384253217846,53.3493834698697,12.));
#152806=CARTESIAN_POINT('Ctrl Pts',(-50.3935177682837,53.3740862772681,
12.));
#152807=CARTESIAN_POINT('Ctrl Pts',(-50.4027724829297,53.398832622931,12.));
#152808=CARTESIAN_POINT('Ctrl Pts',(-50.4120172820047,53.4236224357838,
12.));
#152809=CARTESIAN_POINT('Ctrl Pts',(-50.4212520859914,53.4484556448776,
12.));
#152810=CARTESIAN_POINT('Ctrl Pts',(-50.4304768156667,53.4733321794188,
12.));
#152811=CARTESIAN_POINT('Ctrl Pts',(-50.4396913921382,53.4982519688024,
12.));
#152812=CARTESIAN_POINT('Ctrl Pts',(-50.4488957368839,53.5232149426413,
12.));
#152813=CARTESIAN_POINT('Ctrl Pts',(-50.4580897717838,53.5482210307868,
12.));
#152814=CARTESIAN_POINT('Ctrl Pts',(-50.4672734191756,53.5732701633609,
12.));
#152815=CARTESIAN_POINT('Ctrl Pts',(-50.4764466018071,53.5983622707238,
12.));
#152816=CARTESIAN_POINT('Ctrl Pts',(-50.4856092427314,53.623497283406,12.));
#152817=CARTESIAN_POINT('Ctrl Pts',(-50.4947612652148,53.6486751320436,
12.));
#152818=CARTESIAN_POINT('Ctrl Pts',(-50.503902592653,53.6738957473158,12.));
#152819=CARTESIAN_POINT('Ctrl Pts',(-50.513033148456,53.6991590598548,12.));
#152820=CARTESIAN_POINT('Ctrl Pts',(-50.522152856042,53.7244650002374,12.));
#152821=CARTESIAN_POINT('Ctrl Pts',(-50.5312616390779,53.7498134991703,
12.));
#152822=CARTESIAN_POINT('Ctrl Pts',(-50.5403594216698,53.7752044876304,
12.));
#152823=CARTESIAN_POINT('Ctrl Pts',(-50.5494461285761,53.8006378970197,
12.));
#152824=CARTESIAN_POINT('Ctrl Pts',(-50.5585216854091,53.8261136593075,
12.));
#152825=CARTESIAN_POINT('Ctrl Pts',(-50.5675860188538,53.8516317071804,
12.));
#152826=CARTESIAN_POINT('Ctrl Pts',(-50.5766390561884,53.8771919737032,
12.));
#152827=CARTESIAN_POINT('Ctrl Pts',(-50.5856807248151,53.9027943919836,
12.));
#152828=CARTESIAN_POINT('Ctrl Pts',(-50.5947109517483,53.9284388948004,
12.));
#152829=CARTESIAN_POINT('Ctrl Pts',(-50.603729663214,53.9541254143119,12.));
#152830=CARTESIAN_POINT('Ctrl Pts',(-50.6127367839711,53.979853881553,12.));
#152831=CARTESIAN_POINT('Ctrl Pts',(-50.6217322378648,54.0056242268399,
12.));
#152832=CARTESIAN_POINT('Ctrl Pts',(-50.6307159490553,54.0314363806708,
12.));
#152833=CARTESIAN_POINT('Ctrl Pts',(-50.6396878430939,54.0572902745076,
12.));
#152834=CARTESIAN_POINT('Ctrl Pts',(-50.6486478479465,54.0831858415189,
12.));
#152835=CARTESIAN_POINT('Ctrl Pts',(-50.6575958953221,54.1091230175367,
12.));
#152836=CARTESIAN_POINT('Ctrl Pts',(-50.6665319209869,54.1351017412804,
12.));
#152837=CARTESIAN_POINT('Ctrl Pts',(-50.6741814675486,54.1574061042042,
12.));
#152838=CARTESIAN_POINT('Ctrl Pts',(-50.6800396668778,54.1745287898795,
12.));
#152839=CARTESIAN_POINT('Ctrl Pts',(-50.684111886193,54.1864514382194,12.));
#152840=CARTESIAN_POINT('Ctrl Pts',(-50.6864016965743,54.1931619277621,
12.));
#152841=CARTESIAN_POINT('Ctrl Pts',(-50.6869108458849,54.194654350037,12.));
#152842=CARTESIAN_POINT('',(-48.8900464144686,50.0975384783635,0.));
#152843=CARTESIAN_POINT('',(-48.8900464144686,50.0975384783634,0.));
#152844=CARTESIAN_POINT('Ctrl Pts',(-50.6869108458849,54.1946543500369,
0.));
#152845=CARTESIAN_POINT('Ctrl Pts',(-50.6864016965743,54.1931619277621,
0.));
#152846=CARTESIAN_POINT('Ctrl Pts',(-50.684111886193,54.1864514382194,0.));
#152847=CARTESIAN_POINT('Ctrl Pts',(-50.6800396668778,54.1745287898795,
0.));
#152848=CARTESIAN_POINT('Ctrl Pts',(-50.6741814675486,54.1574061042042,
0.));
#152849=CARTESIAN_POINT('Ctrl Pts',(-50.6665319209869,54.1351017412804,
0.));
#152850=CARTESIAN_POINT('Ctrl Pts',(-50.6575958953221,54.1091230175367,
0.));
#152851=CARTESIAN_POINT('Ctrl Pts',(-50.6486478479465,54.0831858415189,
0.));
#152852=CARTESIAN_POINT('Ctrl Pts',(-50.6396878430939,54.0572902745076,
0.));
#152853=CARTESIAN_POINT('Ctrl Pts',(-50.6307159490553,54.0314363806708,
0.));
#152854=CARTESIAN_POINT('Ctrl Pts',(-50.6217322378648,54.0056242268399,
0.));
#152855=CARTESIAN_POINT('Ctrl Pts',(-50.6127367839711,53.979853881553,0.));
#152856=CARTESIAN_POINT('Ctrl Pts',(-50.603729663214,53.9541254143119,0.));
#152857=CARTESIAN_POINT('Ctrl Pts',(-50.5947109517483,53.9284388948004,
0.));
#152858=CARTESIAN_POINT('Ctrl Pts',(-50.5856807248151,53.9027943919836,
0.));
#152859=CARTESIAN_POINT('Ctrl Pts',(-50.5766390561884,53.8771919737032,
0.));
#152860=CARTESIAN_POINT('Ctrl Pts',(-50.5675860188538,53.8516317071804,
0.));
#152861=CARTESIAN_POINT('Ctrl Pts',(-50.5585216854091,53.8261136593075,
0.));
#152862=CARTESIAN_POINT('Ctrl Pts',(-50.5494461285761,53.8006378970197,
0.));
#152863=CARTESIAN_POINT('Ctrl Pts',(-50.5403594216698,53.7752044876304,
0.));
#152864=CARTESIAN_POINT('Ctrl Pts',(-50.5312616390779,53.7498134991703,
0.));
#152865=CARTESIAN_POINT('Ctrl Pts',(-50.522152856042,53.7244650002374,0.));
#152866=CARTESIAN_POINT('Ctrl Pts',(-50.513033148456,53.6991590598548,0.));
#152867=CARTESIAN_POINT('Ctrl Pts',(-50.503902592653,53.6738957473158,0.));
#152868=CARTESIAN_POINT('Ctrl Pts',(-50.4947612652148,53.6486751320436,
0.));
#152869=CARTESIAN_POINT('Ctrl Pts',(-50.4856092427314,53.623497283406,0.));
#152870=CARTESIAN_POINT('Ctrl Pts',(-50.4764466018071,53.5983622707238,
0.));
#152871=CARTESIAN_POINT('Ctrl Pts',(-50.4672734191756,53.5732701633609,
0.));
#152872=CARTESIAN_POINT('Ctrl Pts',(-50.4580897717838,53.5482210307868,
0.));
#152873=CARTESIAN_POINT('Ctrl Pts',(-50.4488957368839,53.5232149426413,
0.));
#152874=CARTESIAN_POINT('Ctrl Pts',(-50.4396913921382,53.4982519688024,
0.));
#152875=CARTESIAN_POINT('Ctrl Pts',(-50.4304768156667,53.4733321794188,
0.));
#152876=CARTESIAN_POINT('Ctrl Pts',(-50.4212520859914,53.4484556448776,
0.));
#152877=CARTESIAN_POINT('Ctrl Pts',(-50.4120172820047,53.4236224357838,
0.));
#152878=CARTESIAN_POINT('Ctrl Pts',(-50.4027724829297,53.398832622931,0.));
#152879=CARTESIAN_POINT('Ctrl Pts',(-50.3935177682837,53.3740862772681,
0.));
#152880=CARTESIAN_POINT('Ctrl Pts',(-50.384253217846,53.3493834698697,0.));
#152881=CARTESIAN_POINT('Ctrl Pts',(-50.3749789116786,53.3247242719587,
0.));
#152882=CARTESIAN_POINT('Ctrl Pts',(-50.365694930143,53.300108754923,0.));
#152883=CARTESIAN_POINT('Ctrl Pts',(-50.3564013539199,53.2755369903293,
0.));
#152884=CARTESIAN_POINT('Ctrl Pts',(-50.3470982640289,53.2510090499336,
0.));
#152885=CARTESIAN_POINT('Ctrl Pts',(-50.3377857418514,53.2265250056887,
0.));
#152886=CARTESIAN_POINT('Ctrl Pts',(-50.3284638691278,53.2020849297471,
0.));
#152887=CARTESIAN_POINT('Ctrl Pts',(-50.3191327279493,53.1776888944616,
0.));
#152888=CARTESIAN_POINT('Ctrl Pts',(-50.3097924007534,53.1533369723818,
0.));
#152889=CARTESIAN_POINT('Ctrl Pts',(-50.300442970319,53.1290292362485,0.));
#152890=CARTESIAN_POINT('Ctrl Pts',(-50.2910845197619,53.1047657589812,
0.));
#152891=CARTESIAN_POINT('Ctrl Pts',(-50.2817171325358,53.0805466136797,
0.));
#152892=CARTESIAN_POINT('Ctrl Pts',(-50.2723408924373,53.0563718736366,
0.));
#152893=CARTESIAN_POINT('Ctrl Pts',(-50.2629558836111,53.0322416123406,
0.));
#152894=CARTESIAN_POINT('Ctrl Pts',(-50.2535621905552,53.0081559034801,
0.));
#152895=CARTESIAN_POINT('Ctrl Pts',(-50.2441598981286,52.9841148209402,
0.));
#152896=CARTESIAN_POINT('Ctrl Pts',(-50.2347490915555,52.9601184388027,
0.));
#152897=CARTESIAN_POINT('Ctrl Pts',(-50.2253298564241,52.9361668313542,
0.));
#152898=CARTESIAN_POINT('Ctrl Pts',(-50.2159022786879,52.9122600730884,
0.));
#152899=CARTESIAN_POINT('Ctrl Pts',(-50.2064664446663,52.8883982387068,
0.));
#152900=CARTESIAN_POINT('Ctrl Pts',(-50.1970224410471,52.8645814031133,
0.));
#152901=CARTESIAN_POINT('Ctrl Pts',(-50.1875703548884,52.8408096414093,
0.));
#152902=CARTESIAN_POINT('Ctrl Pts',(-50.1781102736205,52.8170830289044,
0.));
#152903=CARTESIAN_POINT('Ctrl Pts',(-50.1686422850488,52.7934016411205,
0.));
#152904=CARTESIAN_POINT('Ctrl Pts',(-50.1591664773561,52.769765553794,0.));
#152905=CARTESIAN_POINT('Ctrl Pts',(-50.1496829391073,52.7461748428738,
0.));
#152906=CARTESIAN_POINT('Ctrl Pts',(-50.1401917592537,52.7226295845161,
0.));
#152907=CARTESIAN_POINT('Ctrl Pts',(-50.1306930271345,52.699129855093,0.));
#152908=CARTESIAN_POINT('Ctrl Pts',(-50.1211868324781,52.6756757311978,
0.));
#152909=CARTESIAN_POINT('Ctrl Pts',(-50.111673265404,52.652267289646,0.));
#152910=CARTESIAN_POINT('Ctrl Pts',(-50.1021524164264,52.6289046074746,
0.));
#152911=CARTESIAN_POINT('Ctrl Pts',(-50.0926243764578,52.6055877619348,
0.));
#152912=CARTESIAN_POINT('Ctrl Pts',(-50.0830892368107,52.5823168304994,
0.));
#152913=CARTESIAN_POINT('Ctrl Pts',(-50.0735470892007,52.5590918908702,
0.));
#152914=CARTESIAN_POINT('Ctrl Pts',(-50.0639980257479,52.5359130209792,
0.));
#152915=CARTESIAN_POINT('Ctrl Pts',(-50.0544421389818,52.5127802989896,
0.));
#152916=CARTESIAN_POINT('Ctrl Pts',(-50.0448795218441,52.4896938032884,
0.));
#152917=CARTESIAN_POINT('Ctrl Pts',(-50.0353102676921,52.4666536124913,
0.));
#152918=CARTESIAN_POINT('Ctrl Pts',(-50.0257344703,52.4436598054515,0.));
#152919=CARTESIAN_POINT('Ctrl Pts',(-50.0161522238616,52.4207124612608,
0.));
#152920=CARTESIAN_POINT('Ctrl Pts',(-50.0065636229938,52.3978116592509,
0.));
#152921=CARTESIAN_POINT('Ctrl Pts',(-49.9969687627408,52.3749574789871,
0.));
#152922=CARTESIAN_POINT('Ctrl Pts',(-49.9873677385775,52.3521500002718,
0.));
#152923=CARTESIAN_POINT('Ctrl Pts',(-49.9777606464106,52.3293893031528,
0.));
#152924=CARTESIAN_POINT('Ctrl Pts',(-49.9681475825824,52.3066754679265,
0.));
#152925=CARTESIAN_POINT('Ctrl Pts',(-49.9585286438733,52.2840085751384,
0.));
#152926=CARTESIAN_POINT('Ctrl Pts',(-49.9489039275064,52.2613887055773,
0.));
#152927=CARTESIAN_POINT('Ctrl Pts',(-49.9392735311509,52.2388159402771,
0.));
#152928=CARTESIAN_POINT('Ctrl Pts',(-49.9296375529245,52.2162903605275,
0.));
#152929=CARTESIAN_POINT('Ctrl Pts',(-49.9199960913962,52.1938120478754,
0.));
#152930=CARTESIAN_POINT('Ctrl Pts',(-49.9103492455902,52.1713810841276,
0.));
#152931=CARTESIAN_POINT('Ctrl Pts',(-49.9006971149895,52.1489975513444,
0.));
#152932=CARTESIAN_POINT('Ctrl Pts',(-49.8910397995397,52.1266615318407,
0.));
#152933=CARTESIAN_POINT('Ctrl Pts',(-49.8813773996517,52.1043731081962,
0.));
#152934=CARTESIAN_POINT('Ctrl Pts',(-49.8717100162048,52.0821323632587,
0.));
#152935=CARTESIAN_POINT('Ctrl Pts',(-49.86203775055,52.0599393801452,0.));
#152936=CARTESIAN_POINT('Ctrl Pts',(-49.8523607045149,52.0377942422376,
0.));
#152937=CARTESIAN_POINT('Ctrl Pts',(-49.8426789804071,52.0156970331822,
0.));
#152938=CARTESIAN_POINT('Ctrl Pts',(-49.8329926810172,51.9936478369008,
0.));
#152939=CARTESIAN_POINT('Ctrl Pts',(-49.8233019096222,51.9716467375937,
0.));
#152940=CARTESIAN_POINT('Ctrl Pts',(-49.8136067699896,51.9496938197418,
0.));
#152941=CARTESIAN_POINT('Ctrl Pts',(-49.8039073663812,51.9277891681018,
0.));
#152942=CARTESIAN_POINT('Ctrl Pts',(-49.7942038035576,51.9059328677059,
0.));
#152943=CARTESIAN_POINT('Ctrl Pts',(-49.7844961867807,51.8841250038724,
0.));
#152944=CARTESIAN_POINT('Ctrl Pts',(-49.7747846218182,51.8623656622097,
0.));
#152945=CARTESIAN_POINT('Ctrl Pts',(-49.7650692149462,51.8406549286175,
0.));
#152946=CARTESIAN_POINT('Ctrl Pts',(-49.755350072955,51.8189928892828,0.));
#152947=CARTESIAN_POINT('Ctrl Pts',(-49.7456273031534,51.7973796306803,
0.));
#152948=CARTESIAN_POINT('Ctrl Pts',(-49.7359010133721,51.7758152395836,
0.));
#152949=CARTESIAN_POINT('Ctrl Pts',(-49.7261713119663,51.754299803067,0.));
#152950=CARTESIAN_POINT('Ctrl Pts',(-49.7164383078212,51.7328334085091,
0.));
#152951=CARTESIAN_POINT('Ctrl Pts',(-49.7067021103553,51.7114161435869,
0.));
#152952=CARTESIAN_POINT('Ctrl Pts',(-49.6969628295262,51.6900480962773,
0.));
#152953=CARTESIAN_POINT('Ctrl Pts',(-49.6872205758336,51.6687293548682,
0.));
#152954=CARTESIAN_POINT('Ctrl Pts',(-49.6774754603245,51.6474600079622,
0.));
#152955=CARTESIAN_POINT('Ctrl Pts',(-49.6677275945967,51.626240144479,0.));
#152956=CARTESIAN_POINT('Ctrl Pts',(-49.6579770908037,51.6050698536496,
0.));
#152957=CARTESIAN_POINT('Ctrl Pts',(-49.6482240616593,51.5839492250181,
0.));
#152958=CARTESIAN_POINT('Ctrl Pts',(-49.6384686204413,51.5628783484525,
0.));
#152959=CARTESIAN_POINT('Ctrl Pts',(-49.6287108809966,51.5418573141484,
0.));
#152960=CARTESIAN_POINT('Ctrl Pts',(-49.6189509577452,51.5208862126315,
0.));
#152961=CARTESIAN_POINT('Ctrl Pts',(-49.6091889656866,51.4999651347522,
0.));
#152962=CARTESIAN_POINT('Ctrl Pts',(-49.5994250204031,51.4790941716888,
0.));
#152963=CARTESIAN_POINT('Ctrl Pts',(-49.5896592380654,51.4582734149583,
0.));
#152964=CARTESIAN_POINT('Ctrl Pts',(-49.5798917354366,51.4375029564197,
0.));
#152965=CARTESIAN_POINT('Ctrl Pts',(-49.5701226298769,51.4167828882756,
0.));
#152966=CARTESIAN_POINT('Ctrl Pts',(-49.5603520393496,51.396113303067,0.));
#152967=CARTESIAN_POINT('Ctrl Pts',(-49.550580082425,51.3754942936778,0.));
#152968=CARTESIAN_POINT('Ctrl Pts',(-49.5408068782859,51.3549259533458,
0.));
#152969=CARTESIAN_POINT('Ctrl Pts',(-49.5310325467332,51.3344083756657,
0.));
#152970=CARTESIAN_POINT('Ctrl Pts',(-49.5212572081908,51.313941654591,0.));
#152971=CARTESIAN_POINT('Ctrl Pts',(-49.5114809837122,51.2935258844289,
0.));
#152972=CARTESIAN_POINT('Ctrl Pts',(-49.5017039949852,51.2731611598475,
0.));
#152973=CARTESIAN_POINT('Ctrl Pts',(-49.4919263643362,51.2528475758846,
0.));
#152974=CARTESIAN_POINT('Ctrl Pts',(-49.4821482147356,51.2325852279506,
0.));
#152975=CARTESIAN_POINT('Ctrl Pts',(-49.4723696698021,51.2123742118287,
0.));
#152976=CARTESIAN_POINT('Ctrl Pts',(-49.4625908538074,51.1922146236686,
0.));
#152977=CARTESIAN_POINT('Ctrl Pts',(-49.4528118916832,51.1721065599972,
0.));
#152978=CARTESIAN_POINT('Ctrl Pts',(-49.4430329090287,51.1520501177291,
0.));
#152979=CARTESIAN_POINT('Ctrl Pts',(-49.4332540321178,51.1320453941702,
0.));
#152980=CARTESIAN_POINT('Ctrl Pts',(-49.423475387907,51.1120924870195,0.));
#152981=CARTESIAN_POINT('Ctrl Pts',(-49.4136971040428,51.0921914943662,
0.));
#152982=CARTESIAN_POINT('Ctrl Pts',(-49.4039193088634,51.0723425146985,
0.));
#152983=CARTESIAN_POINT('Ctrl Pts',(-49.3941421314013,51.052545646907,0.));
#152984=CARTESIAN_POINT('Ctrl Pts',(-49.3843657013852,51.0328009902858,
0.));
#152985=CARTESIAN_POINT('Ctrl Pts',(-49.3745901492432,51.0131086445272,
0.));
#152986=CARTESIAN_POINT('Ctrl Pts',(-49.3648156061058,50.9934687097188,
0.));
#152987=CARTESIAN_POINT('Ctrl Pts',(-49.355042203823,50.9738812863646,0.));
#152988=CARTESIAN_POINT('Ctrl Pts',(-49.345270074981,50.9543464753981,0.));
#152989=CARTESIAN_POINT('Ctrl Pts',(-49.3354993529158,50.9348643781924,
0.));
#152990=CARTESIAN_POINT('Ctrl Pts',(-49.3257301717335,50.9154350965666,
0.));
#152991=CARTESIAN_POINT('Ctrl Pts',(-49.3159626663109,50.8960587327848,
0.));
#152992=CARTESIAN_POINT('Ctrl Pts',(-49.3061969722781,50.8767353895492,
0.));
#152993=CARTESIAN_POINT('Ctrl Pts',(-49.2964332260039,50.8574651699873,
0.));
#152994=CARTESIAN_POINT('Ctrl Pts',(-49.2866715645838,50.8382481776403,
0.));
#152995=CARTESIAN_POINT('Ctrl Pts',(-49.2769121258164,50.819084516434,0.));
#152996=CARTESIAN_POINT('Ctrl Pts',(-49.2671550482435,50.7999742907131,
0.));
#152997=CARTESIAN_POINT('Ctrl Pts',(-49.2574004712134,50.7809176052966,
0.));
#152998=CARTESIAN_POINT('Ctrl Pts',(-49.2476485349373,50.7619145655207,
0.));
#152999=CARTESIAN_POINT('Ctrl Pts',(-49.2378993805471,50.7429652772805,
0.));
#153000=CARTESIAN_POINT('Ctrl Pts',(-49.228153150155,50.7240698470679,0.));
#153001=CARTESIAN_POINT('Ctrl Pts',(-49.2184099867461,50.7052283818922,
0.));
#153002=CARTESIAN_POINT('Ctrl Pts',(-49.2086700340614,50.6864409891895,
0.));
#153003=CARTESIAN_POINT('Ctrl Pts',(-49.1989334364996,50.6677077767432,
0.));
#153004=CARTESIAN_POINT('Ctrl Pts',(-49.189200338976,50.6490288525656,0.));
#153005=CARTESIAN_POINT('Ctrl Pts',(-49.1794708869099,50.6304043248821,
0.));
#153006=CARTESIAN_POINT('Ctrl Pts',(-49.1697452265494,50.6118343023957,
0.));
#153007=CARTESIAN_POINT('Ctrl Pts',(-49.1600235052621,50.5933188945168,
0.));
#153008=CARTESIAN_POINT('Ctrl Pts',(-49.1503058717821,50.5748582115565,
0.));
#153009=CARTESIAN_POINT('Ctrl Pts',(-49.1405924766144,50.556452365038,0.));
#153010=CARTESIAN_POINT('Ctrl Pts',(-49.1308834717615,50.5381014674791,
0.));
#153011=CARTESIAN_POINT('Ctrl Pts',(-49.1211790099795,50.5198056318088,
0.));
#153012=CARTESIAN_POINT('Ctrl Pts',(-49.1114792441571,50.501564970874,0.));
#153013=CARTESIAN_POINT('Ctrl Pts',(-49.1017843266803,50.4833795969318,
0.));
#153014=CARTESIAN_POINT('Ctrl Pts',(-49.0920944087008,50.4652496210607,
0.));
#153015=CARTESIAN_POINT('Ctrl Pts',(-49.0824096415371,50.4471751542751,
0.));
#153016=CARTESIAN_POINT('Ctrl Pts',(-49.0727301783494,50.4291563088547,
0.));
#153017=CARTESIAN_POINT('Ctrl Pts',(-49.0630561755075,50.4111931994257,
0.));
#153018=CARTESIAN_POINT('Ctrl Pts',(-49.0533877945744,50.3932859445252,
0.));
#153019=CARTESIAN_POINT('Ctrl Pts',(-49.0437252024832,50.3754346667353,
0.));
#153020=CARTESIAN_POINT('Ctrl Pts',(-49.0340685673982,50.3576394894108,
0.));
#153021=CARTESIAN_POINT('Ctrl Pts',(-49.024418055075,50.3399005337958,0.));
#153022=CARTESIAN_POINT('Ctrl Pts',(-49.0147738256942,50.3222179165119,
0.));
#153023=CARTESIAN_POINT('Ctrl Pts',(-49.0051360288044,50.3045917455424,
0.));
#153024=CARTESIAN_POINT('Ctrl Pts',(-48.9955048082081,50.2870221241054,
0.));
#153025=CARTESIAN_POINT('Ctrl Pts',(-48.9858803116689,50.2695091583511,
0.));
#153026=CARTESIAN_POINT('Ctrl Pts',(-48.9762626987227,50.252052963548,0.));
#153027=CARTESIAN_POINT('Ctrl Pts',(-48.9666521500911,50.234653671541,0.));
#153028=CARTESIAN_POINT('Ctrl Pts',(-48.9570488741167,50.2173114358325,
0.));
#153029=CARTESIAN_POINT('Ctrl Pts',(-48.9474530868733,50.2000264157797,
0.));
#153030=CARTESIAN_POINT('Ctrl Pts',(-48.9378649933055,50.1827987615602,
0.));
#153031=CARTESIAN_POINT('Ctrl Pts',(-48.9282847698294,50.1656286003997,
0.));
#153032=CARTESIAN_POINT('Ctrl Pts',(-48.9187125418099,50.1485160184657,
0.));
#153033=CARTESIAN_POINT('Ctrl Pts',(-48.90914838181,50.1314610602569,0.));
#153034=CARTESIAN_POINT('Ctrl Pts',(-48.9015035372055,50.1178632067084,
0.));
#153035=CARTESIAN_POINT('Ctrl Pts',(-48.895773555686,50.1076907555471,0.));
#153036=CARTESIAN_POINT('Ctrl Pts',(-48.8919551910366,50.1009206494272,
0.));
#153037=CARTESIAN_POINT('Ctrl Pts',(-48.8900464144686,50.0975384783635,
0.));
#153038=CARTESIAN_POINT('Ctrl Pts',(-45.8467972562798,58.722407829904,0.));
#153039=CARTESIAN_POINT('Ctrl Pts',(-45.8467972562798,58.722407829904,12.));
#153040=CARTESIAN_POINT('Ctrl Pts',(-45.8455162977427,58.7169606500268,
0.));
#153041=CARTESIAN_POINT('Ctrl Pts',(-45.8455162977427,58.7169606500268,
12.));
#153042=CARTESIAN_POINT('Ctrl Pts',(-45.8429527488786,58.7060702401686,
0.));
#153043=CARTESIAN_POINT('Ctrl Pts',(-45.8429527488786,58.7060702401686,
12.));
#153044=CARTESIAN_POINT('Ctrl Pts',(-45.8391025302132,58.68974647507,0.));
#153045=CARTESIAN_POINT('Ctrl Pts',(-45.8391025302132,58.68974647507,12.));
#153046=CARTESIAN_POINT('Ctrl Pts',(-45.8339591141834,58.6680051552762,
0.));
#153047=CARTESIAN_POINT('Ctrl Pts',(-45.8339591141834,58.6680051552762,
12.));
#153048=CARTESIAN_POINT('Ctrl Pts',(-45.8275135264249,58.6408680154016,
0.));
#153049=CARTESIAN_POINT('Ctrl Pts',(-45.8275135264249,58.6408680154016,
12.));
#153050=CARTESIAN_POINT('Ctrl Pts',(-45.8210516273781,58.6137704035871,
0.));
#153051=CARTESIAN_POINT('Ctrl Pts',(-45.8210516273781,58.6137704035871,
12.));
#153052=CARTESIAN_POINT('Ctrl Pts',(-45.814573433072,58.5867123491018,0.));
#153053=CARTESIAN_POINT('Ctrl Pts',(-45.814573433072,58.5867123491018,12.));
#153054=CARTESIAN_POINT('Ctrl Pts',(-45.8080789725084,58.5596938940195,
0.));
#153055=CARTESIAN_POINT('Ctrl Pts',(-45.8080789725084,58.5596938940195,
12.));
#153056=CARTESIAN_POINT('Ctrl Pts',(-45.8015682926024,58.5327150960661,
0.));
#153057=CARTESIAN_POINT('Ctrl Pts',(-45.8015682926024,58.5327150960661,
12.));
#153058=CARTESIAN_POINT('Ctrl Pts',(-45.7950414569268,58.5057760270184,
0.));
#153059=CARTESIAN_POINT('Ctrl Pts',(-45.7950414569268,58.5057760270184,
12.));
#153060=CARTESIAN_POINT('Ctrl Pts',(-45.7884985397018,58.4788767676949,
0.));
#153061=CARTESIAN_POINT('Ctrl Pts',(-45.7884985397018,58.4788767676949,
12.));
#153062=CARTESIAN_POINT('Ctrl Pts',(-45.7819396211009,58.4520174038764,
0.));
#153063=CARTESIAN_POINT('Ctrl Pts',(-45.7819396211009,58.4520174038764,
12.));
#153064=CARTESIAN_POINT('Ctrl Pts',(-45.7753647821513,58.425198021955,0.));
#153065=CARTESIAN_POINT('Ctrl Pts',(-45.7753647821513,58.425198021955,12.));
#153066=CARTESIAN_POINT('Ctrl Pts',(-45.7687740994956,58.3984187044245,
0.));
#153067=CARTESIAN_POINT('Ctrl Pts',(-45.7687740994956,58.3984187044245,
12.));
#153068=CARTESIAN_POINT('Ctrl Pts',(-45.7621676411434,58.3716795262353,
0.));
#153069=CARTESIAN_POINT('Ctrl Pts',(-45.7621676411434,58.3716795262353,
12.));
#153070=CARTESIAN_POINT('Ctrl Pts',(-45.755545469402,58.3449805573423,0.));
#153071=CARTESIAN_POINT('Ctrl Pts',(-45.755545469402,58.3449805573423,12.));
#153072=CARTESIAN_POINT('Ctrl Pts',(-45.7489076429763,58.3183218645317,
0.));
#153073=CARTESIAN_POINT('Ctrl Pts',(-45.7489076429763,58.3183218645317,
12.));
#153074=CARTESIAN_POINT('Ctrl Pts',(-45.742254219463,58.291703513584,0.));
#153075=CARTESIAN_POINT('Ctrl Pts',(-45.742254219463,58.291703513584,12.));
#153076=CARTESIAN_POINT('Ctrl Pts',(-45.7355852575106,58.2651255711453,
0.));
#153077=CARTESIAN_POINT('Ctrl Pts',(-45.7355852575106,58.2651255711453,
12.));
#153078=CARTESIAN_POINT('Ctrl Pts',(-45.7289008195578,58.2385881070913,
0.));
#153079=CARTESIAN_POINT('Ctrl Pts',(-45.7289008195578,58.2385881070913,
12.));
#153080=CARTESIAN_POINT('Ctrl Pts',(-45.7222009715397,58.2120911942772,
0.));
#153081=CARTESIAN_POINT('Ctrl Pts',(-45.7222009715397,58.2120911942772,
12.));
#153082=CARTESIAN_POINT('Ctrl Pts',(-45.7154857816483,58.185634907469,0.));
#153083=CARTESIAN_POINT('Ctrl Pts',(-45.7154857816483,58.185634907469,12.));
#153084=CARTESIAN_POINT('Ctrl Pts',(-45.7087553193771,58.1592193225137,
0.));
#153085=CARTESIAN_POINT('Ctrl Pts',(-45.7087553193771,58.1592193225137,
12.));
#153086=CARTESIAN_POINT('Ctrl Pts',(-45.702009654518,58.1328445154676,0.));
#153087=CARTESIAN_POINT('Ctrl Pts',(-45.702009654518,58.1328445154676,12.));
#153088=CARTESIAN_POINT('Ctrl Pts',(-45.695248856015,58.1065105615907,0.));
#153089=CARTESIAN_POINT('Ctrl Pts',(-45.695248856015,58.1065105615907,12.));
#153090=CARTESIAN_POINT('Ctrl Pts',(-45.6884729914485,58.0802175348966,
0.));
#153091=CARTESIAN_POINT('Ctrl Pts',(-45.6884729914485,58.0802175348966,
12.));
#153092=CARTESIAN_POINT('Ctrl Pts',(-45.6816821276678,58.0539655087117,
0.));
#153093=CARTESIAN_POINT('Ctrl Pts',(-45.6816821276678,58.0539655087117,
12.));
#153094=CARTESIAN_POINT('Ctrl Pts',(-45.6748763311643,58.0277545560012,
0.));
#153095=CARTESIAN_POINT('Ctrl Pts',(-45.6748763311643,58.0277545560012,
12.));
#153096=CARTESIAN_POINT('Ctrl Pts',(-45.6680556685493,58.0015847497837,
0.));
#153097=CARTESIAN_POINT('Ctrl Pts',(-45.6680556685493,58.0015847497837,
12.));
#153098=CARTESIAN_POINT('Ctrl Pts',(-45.661220206992,57.9754561635061,0.));
#153099=CARTESIAN_POINT('Ctrl Pts',(-45.661220206992,57.9754561635061,12.));
#153100=CARTESIAN_POINT('Ctrl Pts',(-45.6543700146679,57.9493688714237,
0.));
#153101=CARTESIAN_POINT('Ctrl Pts',(-45.6543700146679,57.9493688714237,
12.));
#153102=CARTESIAN_POINT('Ctrl Pts',(-45.6475051605535,57.9233229484311,
0.));
#153103=CARTESIAN_POINT('Ctrl Pts',(-45.6475051605535,57.9233229484311,
12.));
#153104=CARTESIAN_POINT('Ctrl Pts',(-45.6406257142381,57.8973184699034,
0.));
#153105=CARTESIAN_POINT('Ctrl Pts',(-45.6406257142381,57.8973184699034,
12.));
#153106=CARTESIAN_POINT('Ctrl Pts',(-45.6337317457252,57.8713555115232,
0.));
#153107=CARTESIAN_POINT('Ctrl Pts',(-45.6337317457252,57.8713555115232,
12.));
#153108=CARTESIAN_POINT('Ctrl Pts',(-45.6268233252544,57.8454341491238,
0.));
#153109=CARTESIAN_POINT('Ctrl Pts',(-45.6268233252544,57.8454341491238,
12.));
#153110=CARTESIAN_POINT('Ctrl Pts',(-45.6199005230783,57.8195544584845,
0.));
#153111=CARTESIAN_POINT('Ctrl Pts',(-45.6199005230783,57.8195544584845,
12.));
#153112=CARTESIAN_POINT('Ctrl Pts',(-45.6129634094683,57.7937165153387,
0.));
#153113=CARTESIAN_POINT('Ctrl Pts',(-45.6129634094683,57.7937165153387,
12.));
#153114=CARTESIAN_POINT('Ctrl Pts',(-45.6060120548205,57.7679203954742,
0.));
#153115=CARTESIAN_POINT('Ctrl Pts',(-45.6060120548205,57.7679203954742,
12.));
#153116=CARTESIAN_POINT('Ctrl Pts',(-45.5990465297343,57.7421661748026,
0.));
#153117=CARTESIAN_POINT('Ctrl Pts',(-45.5990465297343,57.7421661748026,
12.));
#153118=CARTESIAN_POINT('Ctrl Pts',(-45.5920669050986,57.7164539294314,
0.));
#153119=CARTESIAN_POINT('Ctrl Pts',(-45.5920669050986,57.7164539294314,
12.));
#153120=CARTESIAN_POINT('Ctrl Pts',(-45.5850732521895,57.6907837357418,
0.));
#153121=CARTESIAN_POINT('Ctrl Pts',(-45.5850732521895,57.6907837357418,
12.));
#153122=CARTESIAN_POINT('Ctrl Pts',(-45.5780656427163,57.6651556704237,
0.));
#153123=CARTESIAN_POINT('Ctrl Pts',(-45.5780656427163,57.6651556704237,
12.));
#153124=CARTESIAN_POINT('Ctrl Pts',(-45.5710441487674,57.6395698104404,
0.));
#153125=CARTESIAN_POINT('Ctrl Pts',(-45.5710441487674,57.6395698104404,
12.));
#153126=CARTESIAN_POINT('Ctrl Pts',(-45.5640088427813,57.614026233004,0.));
#153127=CARTESIAN_POINT('Ctrl Pts',(-45.5640088427813,57.614026233004,12.));
#153128=CARTESIAN_POINT('Ctrl Pts',(-45.5569597975096,57.5885250155433,
0.));
#153129=CARTESIAN_POINT('Ctrl Pts',(-45.5569597975096,57.5885250155433,
12.));
#153130=CARTESIAN_POINT('Ctrl Pts',(-45.5498970859834,57.563066235668,0.));
#153131=CARTESIAN_POINT('Ctrl Pts',(-45.5498970859834,57.563066235668,12.));
#153132=CARTESIAN_POINT('Ctrl Pts',(-45.542820781484,57.537649971135,0.));
#153133=CARTESIAN_POINT('Ctrl Pts',(-45.542820781484,57.537649971135,12.));
#153134=CARTESIAN_POINT('Ctrl Pts',(-45.5357309575611,57.5122762998745,
0.));
#153135=CARTESIAN_POINT('Ctrl Pts',(-45.5357309575611,57.5122762998745,
12.));
#153136=CARTESIAN_POINT('Ctrl Pts',(-45.5286276880484,57.4869453000063,
0.));
#153137=CARTESIAN_POINT('Ctrl Pts',(-45.5286276880484,57.4869453000063,
12.));
#153138=CARTESIAN_POINT('Ctrl Pts',(-45.5215110470825,57.4616570498568,
0.));
#153139=CARTESIAN_POINT('Ctrl Pts',(-45.5215110470825,57.4616570498568,
12.));
#153140=CARTESIAN_POINT('Ctrl Pts',(-45.5143811091205,57.4364116279702,
0.));
#153141=CARTESIAN_POINT('Ctrl Pts',(-45.5143811091205,57.4364116279702,
12.));
#153142=CARTESIAN_POINT('Ctrl Pts',(-45.5072379489631,57.4112091131183,
0.));
#153143=CARTESIAN_POINT('Ctrl Pts',(-45.5072379489631,57.4112091131183,
12.));
#153144=CARTESIAN_POINT('Ctrl Pts',(-45.5000816417509,57.3860495843033,
0.));
#153145=CARTESIAN_POINT('Ctrl Pts',(-45.5000816417509,57.3860495843033,
12.));
#153146=CARTESIAN_POINT('Ctrl Pts',(-45.4929122629572,57.3609331207574,
0.));
#153147=CARTESIAN_POINT('Ctrl Pts',(-45.4929122629572,57.3609331207574,
12.));
#153148=CARTESIAN_POINT('Ctrl Pts',(-45.4857298883824,57.3358598019389,
0.));
#153149=CARTESIAN_POINT('Ctrl Pts',(-45.4857298883824,57.3358598019389,
12.));
#153150=CARTESIAN_POINT('Ctrl Pts',(-45.4785345941507,57.3108297075265,
0.));
#153151=CARTESIAN_POINT('Ctrl Pts',(-45.4785345941507,57.3108297075265,
12.));
#153152=CARTESIAN_POINT('Ctrl Pts',(-45.4713264567063,57.2858429174062,
0.));
#153153=CARTESIAN_POINT('Ctrl Pts',(-45.4713264567063,57.2858429174062,
12.));
#153154=CARTESIAN_POINT('Ctrl Pts',(-45.4641055528141,57.2608995116733,
0.));
#153155=CARTESIAN_POINT('Ctrl Pts',(-45.4641055528141,57.2608995116733,
12.));
#153156=CARTESIAN_POINT('Ctrl Pts',(-45.4568719595641,57.2359995706447,
0.));
#153157=CARTESIAN_POINT('Ctrl Pts',(-45.4568719595641,57.2359995706447,
12.));
#153158=CARTESIAN_POINT('Ctrl Pts',(-45.4496257543759,57.2111431748631,
0.));
#153159=CARTESIAN_POINT('Ctrl Pts',(-45.4496257543759,57.2111431748631,
12.));
#153160=CARTESIAN_POINT('Ctrl Pts',(-45.4423670150034,57.186330405101,0.));
#153161=CARTESIAN_POINT('Ctrl Pts',(-45.4423670150034,57.186330405101,12.));
#153162=CARTESIAN_POINT('Ctrl Pts',(-45.4350958195433,57.1615613423584,
0.));
#153163=CARTESIAN_POINT('Ctrl Pts',(-45.4350958195433,57.1615613423584,
12.));
#153164=CARTESIAN_POINT('Ctrl Pts',(-45.4278122464389,57.136836067863,0.));
#153165=CARTESIAN_POINT('Ctrl Pts',(-45.4278122464389,57.136836067863,12.));
#153166=CARTESIAN_POINT('Ctrl Pts',(-45.4205163744781,57.112154663078,0.));
#153167=CARTESIAN_POINT('Ctrl Pts',(-45.4205163744781,57.112154663078,12.));
#153168=CARTESIAN_POINT('Ctrl Pts',(-45.4132082827948,57.0875172097051,
0.));
#153169=CARTESIAN_POINT('Ctrl Pts',(-45.4132082827948,57.0875172097051,
12.));
#153170=CARTESIAN_POINT('Ctrl Pts',(-45.4058880508693,57.0629237896848,
0.));
#153171=CARTESIAN_POINT('Ctrl Pts',(-45.4058880508693,57.0629237896848,
12.));
#153172=CARTESIAN_POINT('Ctrl Pts',(-45.3985557585311,57.0383744851913,
0.));
#153173=CARTESIAN_POINT('Ctrl Pts',(-45.3985557585311,57.0383744851913,
12.));
#153174=CARTESIAN_POINT('Ctrl Pts',(-45.3912114859616,57.0138693786278,
0.));
#153175=CARTESIAN_POINT('Ctrl Pts',(-45.3912114859616,57.0138693786278,
12.));
#153176=CARTESIAN_POINT('Ctrl Pts',(-45.3838553136948,56.9894085526373,
0.));
#153177=CARTESIAN_POINT('Ctrl Pts',(-45.3838553136948,56.9894085526373,
12.));
#153178=CARTESIAN_POINT('Ctrl Pts',(-45.3764873226196,56.9649920901073,
0.));
#153179=CARTESIAN_POINT('Ctrl Pts',(-45.3764873226196,56.9649920901073,
12.));
#153180=CARTESIAN_POINT('Ctrl Pts',(-45.3691075939826,56.9406200741714,
0.));
#153181=CARTESIAN_POINT('Ctrl Pts',(-45.3691075939826,56.9406200741714,
12.));
#153182=CARTESIAN_POINT('Ctrl Pts',(-45.3617162093922,56.9162925882085,
0.));
#153183=CARTESIAN_POINT('Ctrl Pts',(-45.3617162093922,56.9162925882085,
12.));
#153184=CARTESIAN_POINT('Ctrl Pts',(-45.3543132508238,56.8920097158377,
0.));
#153185=CARTESIAN_POINT('Ctrl Pts',(-45.3543132508238,56.8920097158377,
12.));
#153186=CARTESIAN_POINT('Ctrl Pts',(-45.3468988006203,56.8677715409268,
0.));
#153187=CARTESIAN_POINT('Ctrl Pts',(-45.3468988006203,56.8677715409268,
12.));
#153188=CARTESIAN_POINT('Ctrl Pts',(-45.3394729414931,56.8435781475981,
0.));
#153189=CARTESIAN_POINT('Ctrl Pts',(-45.3394729414931,56.8435781475981,
12.));
#153190=CARTESIAN_POINT('Ctrl Pts',(-45.332035756524,56.8194296202291,0.));
#153191=CARTESIAN_POINT('Ctrl Pts',(-45.332035756524,56.8194296202291,12.));
#153192=CARTESIAN_POINT('Ctrl Pts',(-45.3245873291684,56.7953260434524,
0.));
#153193=CARTESIAN_POINT('Ctrl Pts',(-45.3245873291684,56.7953260434524,
12.));
#153194=CARTESIAN_POINT('Ctrl Pts',(-45.31712774326,56.7712675021491,0.));
#153195=CARTESIAN_POINT('Ctrl Pts',(-45.31712774326,56.7712675021491,12.));
#153196=CARTESIAN_POINT('Ctrl Pts',(-45.3096570830117,56.7472540814554,
0.));
#153197=CARTESIAN_POINT('Ctrl Pts',(-45.3096570830117,56.7472540814554,
12.));
#153198=CARTESIAN_POINT('Ctrl Pts',(-45.3021754330178,56.7232858667709,
0.));
#153199=CARTESIAN_POINT('Ctrl Pts',(-45.3021754330178,56.7232858667709,
12.));
#153200=CARTESIAN_POINT('Ctrl Pts',(-45.2946828782559,56.69936294376,0.));
#153201=CARTESIAN_POINT('Ctrl Pts',(-45.2946828782559,56.69936294376,12.));
#153202=CARTESIAN_POINT('Ctrl Pts',(-45.2871795040906,56.6754853983528,
0.));
#153203=CARTESIAN_POINT('Ctrl Pts',(-45.2871795040906,56.6754853983528,
12.));
#153204=CARTESIAN_POINT('Ctrl Pts',(-45.2796653962785,56.6516533167384,
0.));
#153205=CARTESIAN_POINT('Ctrl Pts',(-45.2796653962785,56.6516533167384,
12.));
#153206=CARTESIAN_POINT('Ctrl Pts',(-45.2721406409695,56.6278667853702,
0.));
#153207=CARTESIAN_POINT('Ctrl Pts',(-45.2721406409695,56.6278667853702,
12.));
#153208=CARTESIAN_POINT('Ctrl Pts',(-45.2646053247087,56.6041258909741,
0.));
#153209=CARTESIAN_POINT('Ctrl Pts',(-45.2646053247087,56.6041258909741,
12.));
#153210=CARTESIAN_POINT('Ctrl Pts',(-45.257059534438,56.5804307205505,0.));
#153211=CARTESIAN_POINT('Ctrl Pts',(-45.257059534438,56.5804307205505,12.));
#153212=CARTESIAN_POINT('Ctrl Pts',(-45.2495033575,56.5567813613756,0.));
#153213=CARTESIAN_POINT('Ctrl Pts',(-45.2495033575,56.5567813613756,12.));
#153214=CARTESIAN_POINT('Ctrl Pts',(-45.2419368816428,56.5331779009958,
0.));
#153215=CARTESIAN_POINT('Ctrl Pts',(-45.2419368816428,56.5331779009958,
12.));
#153216=CARTESIAN_POINT('Ctrl Pts',(-45.2343601950227,56.5096204272306,
0.));
#153217=CARTESIAN_POINT('Ctrl Pts',(-45.2343601950227,56.5096204272306,
12.));
#153218=CARTESIAN_POINT('Ctrl Pts',(-45.2267733862049,56.4861090281823,
0.));
#153219=CARTESIAN_POINT('Ctrl Pts',(-45.2267733862049,56.4861090281823,
12.));
#153220=CARTESIAN_POINT('Ctrl Pts',(-45.2191765441666,56.4626437922386,
0.));
#153221=CARTESIAN_POINT('Ctrl Pts',(-45.2191765441666,56.4626437922386,
12.));
#153222=CARTESIAN_POINT('Ctrl Pts',(-45.2115697583,56.4392248080732,0.));
#153223=CARTESIAN_POINT('Ctrl Pts',(-45.2115697583,56.4392248080732,12.));
#153224=CARTESIAN_POINT('Ctrl Pts',(-45.2039531184171,56.4158521646411,
0.));
#153225=CARTESIAN_POINT('Ctrl Pts',(-45.2039531184171,56.4158521646411,
12.));
#153226=CARTESIAN_POINT('Ctrl Pts',(-45.1963267147529,56.3925259511806,
0.));
#153227=CARTESIAN_POINT('Ctrl Pts',(-45.1963267147529,56.3925259511806,
12.));
#153228=CARTESIAN_POINT('Ctrl Pts',(-45.1886906379667,56.3692462572231,
0.));
#153229=CARTESIAN_POINT('Ctrl Pts',(-45.1886906379667,56.3692462572231,
12.));
#153230=CARTESIAN_POINT('Ctrl Pts',(-45.1810449791453,56.3460131725964,
0.));
#153231=CARTESIAN_POINT('Ctrl Pts',(-45.1810449791453,56.3460131725964,
12.));
#153232=CARTESIAN_POINT('Ctrl Pts',(-45.173389829806,56.3228267874264,0.));
#153233=CARTESIAN_POINT('Ctrl Pts',(-45.173389829806,56.3228267874264,12.));
#153234=CARTESIAN_POINT('Ctrl Pts',(-45.1657252819013,56.2996871921316,
0.));
#153235=CARTESIAN_POINT('Ctrl Pts',(-45.1657252819013,56.2996871921316,
12.));
#153236=CARTESIAN_POINT('Ctrl Pts',(-45.1580514278223,56.2765944774245,
0.));
#153237=CARTESIAN_POINT('Ctrl Pts',(-45.1580514278223,56.2765944774245,
12.));
#153238=CARTESIAN_POINT('Ctrl Pts',(-45.1503683604005,56.2535487343221,
0.));
#153239=CARTESIAN_POINT('Ctrl Pts',(-45.1503683604005,56.2535487343221,
12.));
#153240=CARTESIAN_POINT('Ctrl Pts',(-45.1426761729105,56.230550054149,0.));
#153241=CARTESIAN_POINT('Ctrl Pts',(-45.1426761729105,56.230550054149,12.));
#153242=CARTESIAN_POINT('Ctrl Pts',(-45.1349749590737,56.2075985285393,
0.));
#153243=CARTESIAN_POINT('Ctrl Pts',(-45.1349749590737,56.2075985285393,
12.));
#153244=CARTESIAN_POINT('Ctrl Pts',(-45.127264813063,56.1846942494325,0.));
#153245=CARTESIAN_POINT('Ctrl Pts',(-45.127264813063,56.1846942494325,12.));
#153246=CARTESIAN_POINT('Ctrl Pts',(-45.1195458295062,56.1618373090732,
0.));
#153247=CARTESIAN_POINT('Ctrl Pts',(-45.1195458295062,56.1618373090732,
12.));
#153248=CARTESIAN_POINT('Ctrl Pts',(-45.1118181034888,56.1390278000226,
0.));
#153249=CARTESIAN_POINT('Ctrl Pts',(-45.1118181034888,56.1390278000226,
12.));
#153250=CARTESIAN_POINT('Ctrl Pts',(-45.1040817305561,56.116265815162,0.));
#153251=CARTESIAN_POINT('Ctrl Pts',(-45.1040817305561,56.116265815162,12.));
#153252=CARTESIAN_POINT('Ctrl Pts',(-45.0963368067177,56.0935514476945,
0.));
#153253=CARTESIAN_POINT('Ctrl Pts',(-45.0963368067177,56.0935514476945,
12.));
#153254=CARTESIAN_POINT('Ctrl Pts',(-45.0885834284517,56.0708847911416,
0.));
#153255=CARTESIAN_POINT('Ctrl Pts',(-45.0885834284517,56.0708847911416,
12.));
#153256=CARTESIAN_POINT('Ctrl Pts',(-45.0808216927089,56.048265939342,0.));
#153257=CARTESIAN_POINT('Ctrl Pts',(-45.0808216927089,56.048265939342,12.));
#153258=CARTESIAN_POINT('Ctrl Pts',(-45.0730516969148,56.0256949864639,
0.));
#153259=CARTESIAN_POINT('Ctrl Pts',(-45.0730516969148,56.0256949864639,
12.));
#153260=CARTESIAN_POINT('Ctrl Pts',(-45.0652735389733,56.003172027008,0.));
#153261=CARTESIAN_POINT('Ctrl Pts',(-45.0652735389733,56.003172027008,12.));
#153262=CARTESIAN_POINT('Ctrl Pts',(-45.0574873172694,55.9806971558097,
0.));
#153263=CARTESIAN_POINT('Ctrl Pts',(-45.0574873172694,55.9806971558097,
12.));
#153264=CARTESIAN_POINT('Ctrl Pts',(-45.0496931306755,55.9582704680356,
0.));
#153265=CARTESIAN_POINT('Ctrl Pts',(-45.0496931306755,55.9582704680356,
12.));
#153266=CARTESIAN_POINT('Ctrl Pts',(-45.041891078555,55.9358920591837,0.));
#153267=CARTESIAN_POINT('Ctrl Pts',(-45.041891078555,55.9358920591837,12.));
#153268=CARTESIAN_POINT('Ctrl Pts',(-45.0340812607657,55.9135620250954,
0.));
#153269=CARTESIAN_POINT('Ctrl Pts',(-45.0340812607657,55.9135620250954,
12.));
#153270=CARTESIAN_POINT('Ctrl Pts',(-45.0262637776614,55.8912804619577,
0.));
#153271=CARTESIAN_POINT('Ctrl Pts',(-45.0262637776614,55.8912804619577,
12.));
#153272=CARTESIAN_POINT('Ctrl Pts',(-45.0184387300973,55.8690474663065,
0.));
#153273=CARTESIAN_POINT('Ctrl Pts',(-45.0184387300973,55.8690474663065,
12.));
#153274=CARTESIAN_POINT('Ctrl Pts',(-45.0106062194342,55.8468631350218,
0.));
#153275=CARTESIAN_POINT('Ctrl Pts',(-45.0106062194342,55.8468631350218,
12.));
#153276=CARTESIAN_POINT('Ctrl Pts',(-45.0027663475433,55.8247275653289,
0.));
#153277=CARTESIAN_POINT('Ctrl Pts',(-45.0027663475433,55.8247275653289,
12.));
#153278=CARTESIAN_POINT('Ctrl Pts',(-44.9949192168093,55.8026408548105,
0.));
#153279=CARTESIAN_POINT('Ctrl Pts',(-44.9949192168093,55.8026408548105,
12.));
#153280=CARTESIAN_POINT('Ctrl Pts',(-44.9870649301342,55.7806031014106,
0.));
#153281=CARTESIAN_POINT('Ctrl Pts',(-44.9870649301342,55.7806031014106,
12.));
#153282=CARTESIAN_POINT('Ctrl Pts',(-44.9792035909413,55.7586144034367,
0.));
#153283=CARTESIAN_POINT('Ctrl Pts',(-44.9792035909413,55.7586144034367,
12.));
#153284=CARTESIAN_POINT('Ctrl Pts',(-44.9713353031804,55.7366748595552,
0.));
#153285=CARTESIAN_POINT('Ctrl Pts',(-44.9713353031804,55.7366748595552,
12.));
#153286=CARTESIAN_POINT('Ctrl Pts',(-44.9634601713321,55.714784568793,0.));
#153287=CARTESIAN_POINT('Ctrl Pts',(-44.9634601713321,55.714784568793,12.));
#153288=CARTESIAN_POINT('Ctrl Pts',(-44.9555783004106,55.6929436305489,
0.));
#153289=CARTESIAN_POINT('Ctrl Pts',(-44.9555783004106,55.6929436305489,
12.));
#153290=CARTESIAN_POINT('Ctrl Pts',(-44.9476897959684,55.6711521445979,
0.));
#153291=CARTESIAN_POINT('Ctrl Pts',(-44.9476897959684,55.6711521445979,
12.));
#153292=CARTESIAN_POINT('Ctrl Pts',(-44.9397947641006,55.6494102110935,
0.));
#153293=CARTESIAN_POINT('Ctrl Pts',(-44.9397947641006,55.6494102110935,
12.));
#153294=CARTESIAN_POINT('Ctrl Pts',(-44.9318933114506,55.6277179305633,
0.));
#153295=CARTESIAN_POINT('Ctrl Pts',(-44.9318933114506,55.6277179305633,
12.));
#153296=CARTESIAN_POINT('Ctrl Pts',(-44.9239855452144,55.6060754039121,
0.));
#153297=CARTESIAN_POINT('Ctrl Pts',(-44.9239855452144,55.6060754039121,
12.));
#153298=CARTESIAN_POINT('Ctrl Pts',(-44.9160715731443,55.5844827324338,
0.));
#153299=CARTESIAN_POINT('Ctrl Pts',(-44.9160715731443,55.5844827324338,
12.));
#153300=CARTESIAN_POINT('Ctrl Pts',(-44.908151503553,55.5629400178142,0.));
#153301=CARTESIAN_POINT('Ctrl Pts',(-44.908151503553,55.5629400178142,12.));
#153302=CARTESIAN_POINT('Ctrl Pts',(-44.9002254453183,55.541447362134,0.));
#153303=CARTESIAN_POINT('Ctrl Pts',(-44.9002254453183,55.541447362134,12.));
#153304=CARTESIAN_POINT('Ctrl Pts',(-44.8922935078889,55.5200048678629,
0.));
#153305=CARTESIAN_POINT('Ctrl Pts',(-44.8922935078889,55.5200048678629,
12.));
#153306=CARTESIAN_POINT('Ctrl Pts',(-44.8843558012886,55.4986126378656,
0.));
#153307=CARTESIAN_POINT('Ctrl Pts',(-44.8843558012886,55.4986126378656,
12.));
#153308=CARTESIAN_POINT('Ctrl Pts',(-44.8764124361206,55.4772707754126,
0.));
#153309=CARTESIAN_POINT('Ctrl Pts',(-44.8764124361206,55.4772707754126,
12.));
#153310=CARTESIAN_POINT('Ctrl Pts',(-44.8684635235725,55.4559793841836,
0.));
#153311=CARTESIAN_POINT('Ctrl Pts',(-44.8684635235725,55.4559793841836,
12.));
#153312=CARTESIAN_POINT('Ctrl Pts',(-44.8605091754214,55.4347385682704,
0.));
#153313=CARTESIAN_POINT('Ctrl Pts',(-44.8605091754214,55.4347385682704,
12.));
#153314=CARTESIAN_POINT('Ctrl Pts',(-44.8525495040408,55.4135484321718,
0.));
#153315=CARTESIAN_POINT('Ctrl Pts',(-44.8525495040408,55.4135484321718,
12.));
#153316=CARTESIAN_POINT('Ctrl Pts',(-44.8445846224044,55.3924090808014,
0.));
#153317=CARTESIAN_POINT('Ctrl Pts',(-44.8445846224044,55.3924090808014,
12.));
#153318=CARTESIAN_POINT('Ctrl Pts',(-44.8366146440901,55.3713206194967,
0.));
#153319=CARTESIAN_POINT('Ctrl Pts',(-44.8366146440901,55.3713206194967,
12.));
#153320=CARTESIAN_POINT('Ctrl Pts',(-44.8286396832847,55.3502831540228,
0.));
#153321=CARTESIAN_POINT('Ctrl Pts',(-44.8286396832847,55.3502831540228,
12.));
#153322=CARTESIAN_POINT('Ctrl Pts',(-44.8206598547887,55.3292967905725,
0.));
#153323=CARTESIAN_POINT('Ctrl Pts',(-44.8206598547887,55.3292967905725,
12.));
#153324=CARTESIAN_POINT('Ctrl Pts',(-44.8126752740208,55.3083616357605,
0.));
#153325=CARTESIAN_POINT('Ctrl Pts',(-44.8126752740208,55.3083616357605,
12.));
#153326=CARTESIAN_POINT('Ctrl Pts',(-44.8046860570244,55.287477796635,0.));
#153327=CARTESIAN_POINT('Ctrl Pts',(-44.8046860570244,55.287477796635,12.));
#153328=CARTESIAN_POINT('Ctrl Pts',(-44.796692320474,55.2666453806883,0.));
#153329=CARTESIAN_POINT('Ctrl Pts',(-44.796692320474,55.2666453806883,12.));
#153330=CARTESIAN_POINT('Ctrl Pts',(-44.7886941816823,55.2458644958617,
0.));
#153331=CARTESIAN_POINT('Ctrl Pts',(-44.7886941816823,55.2458644958617,
12.));
#153332=CARTESIAN_POINT('Ctrl Pts',(-44.7806917586077,55.2251352505474,
0.));
#153333=CARTESIAN_POINT('Ctrl Pts',(-44.7806917586077,55.2251352505474,
12.));
#153334=CARTESIAN_POINT('Ctrl Pts',(-44.7726851698618,55.2044577535865,
0.));
#153335=CARTESIAN_POINT('Ctrl Pts',(-44.7726851698618,55.2044577535865,
12.));
#153336=CARTESIAN_POINT('Ctrl Pts',(-44.7646745347108,55.1838321142777,
0.));
#153337=CARTESIAN_POINT('Ctrl Pts',(-44.7646745347108,55.1838321142777,
12.));
#153338=CARTESIAN_POINT('Ctrl Pts',(-44.7566599730771,55.1632584423813,
0.));
#153339=CARTESIAN_POINT('Ctrl Pts',(-44.7566599730771,55.1632584423813,
12.));
#153340=CARTESIAN_POINT('Ctrl Pts',(-44.7486416055419,55.1427368481201,
0.));
#153341=CARTESIAN_POINT('Ctrl Pts',(-44.7486416055419,55.1427368481201,
12.));
#153342=CARTESIAN_POINT('Ctrl Pts',(-44.7406195533482,55.1222674421747,
0.));
#153343=CARTESIAN_POINT('Ctrl Pts',(-44.7406195533482,55.1222674421747,
12.));
#153344=CARTESIAN_POINT('Ctrl Pts',(-44.7325939384042,55.1018503356806,
0.));
#153345=CARTESIAN_POINT('Ctrl Pts',(-44.7325939384042,55.1018503356806,
12.));
#153346=CARTESIAN_POINT('Ctrl Pts',(-44.7245648832988,55.0814856402507,
0.));
#153347=CARTESIAN_POINT('Ctrl Pts',(-44.7245648832988,55.0814856402507,
12.));
#153348=CARTESIAN_POINT('Ctrl Pts',(-44.7165325113165,55.0611734679902,
0.));
#153349=CARTESIAN_POINT('Ctrl Pts',(-44.7165325113165,55.0611734679902,
12.));
#153350=CARTESIAN_POINT('Ctrl Pts',(-44.7084969464509,55.0409139315074,
0.));
#153351=CARTESIAN_POINT('Ctrl Pts',(-44.7084969464509,55.0409139315074,
12.));
#153352=CARTESIAN_POINT('Ctrl Pts',(-44.7004583134235,55.020707143922,0.));
#153353=CARTESIAN_POINT('Ctrl Pts',(-44.7004583134235,55.020707143922,12.));
#153354=CARTESIAN_POINT('Ctrl Pts',(-44.6924167376851,55.0005532188644,
0.));
#153355=CARTESIAN_POINT('Ctrl Pts',(-44.6924167376851,55.0005532188644,
12.));
#153356=CARTESIAN_POINT('Ctrl Pts',(-44.6843723453985,54.9804522704668,
0.));
#153357=CARTESIAN_POINT('Ctrl Pts',(-44.6843723453985,54.9804522704668,
12.));
#153358=CARTESIAN_POINT('Ctrl Pts',(-44.6763252634255,54.9604044133497,
0.));
#153359=CARTESIAN_POINT('Ctrl Pts',(-44.6763252634255,54.9604044133497,
12.));
#153360=CARTESIAN_POINT('Ctrl Pts',(-44.6682756193155,54.9404097626088,
0.));
#153361=CARTESIAN_POINT('Ctrl Pts',(-44.6682756193155,54.9404097626088,
12.));
#153362=CARTESIAN_POINT('Ctrl Pts',(-44.6602235412853,54.9204684337845,
0.));
#153363=CARTESIAN_POINT('Ctrl Pts',(-44.6602235412853,54.9204684337845,
12.));
#153364=CARTESIAN_POINT('Ctrl Pts',(-44.6521691582551,54.9005805428991,
0.));
#153365=CARTESIAN_POINT('Ctrl Pts',(-44.6521691582551,54.9005805428991,
12.));
#153366=CARTESIAN_POINT('Ctrl Pts',(-44.6441125999074,54.8807462065177,
0.));
#153367=CARTESIAN_POINT('Ctrl Pts',(-44.6441125999074,54.8807462065177,
12.));
#153368=CARTESIAN_POINT('Ctrl Pts',(-44.6360539967392,54.860965541796,0.));
#153369=CARTESIAN_POINT('Ctrl Pts',(-44.6360539967392,54.860965541796,12.));
#153370=CARTESIAN_POINT('Ctrl Pts',(-44.6279934801159,54.8412386665264,
0.));
#153371=CARTESIAN_POINT('Ctrl Pts',(-44.6279934801159,54.8412386665264,
12.));
#153372=CARTESIAN_POINT('Ctrl Pts',(-44.6199311823276,54.8215656991817,
0.));
#153373=CARTESIAN_POINT('Ctrl Pts',(-44.6199311823276,54.8215656991817,
12.));
#153374=CARTESIAN_POINT('Ctrl Pts',(-44.6118672364889,54.8019467588258,
0.));
#153375=CARTESIAN_POINT('Ctrl Pts',(-44.6118672364889,54.8019467588258,
12.));
#153376=CARTESIAN_POINT('Ctrl Pts',(-44.60380177643,54.7823819650137,0.));
#153377=CARTESIAN_POINT('Ctrl Pts',(-44.60380177643,54.7823819650137,12.));
#153378=CARTESIAN_POINT('Ctrl Pts',(-44.5957349366062,54.7628714377042,
0.));
#153379=CARTESIAN_POINT('Ctrl Pts',(-44.5957349366062,54.7628714377042,
12.));
#153380=CARTESIAN_POINT('Ctrl Pts',(-44.5876668519676,54.7434152971285,
0.));
#153381=CARTESIAN_POINT('Ctrl Pts',(-44.5876668519676,54.7434152971285,
12.));
#153382=CARTESIAN_POINT('Ctrl Pts',(-44.5795976579476,54.7240136637744,
0.));
#153383=CARTESIAN_POINT('Ctrl Pts',(-44.5795976579476,54.7240136637744,
12.));
#153384=CARTESIAN_POINT('Ctrl Pts',(-44.5715274907637,54.7046666586777,
0.));
#153385=CARTESIAN_POINT('Ctrl Pts',(-44.5715274907637,54.7046666586777,
12.));
#153386=CARTESIAN_POINT('Ctrl Pts',(-44.5634564876869,54.685374403676,0.));
#153387=CARTESIAN_POINT('Ctrl Pts',(-44.5634564876869,54.685374403676,12.));
#153388=CARTESIAN_POINT('Ctrl Pts',(-44.5553847872712,54.6661370216242,
0.));
#153389=CARTESIAN_POINT('Ctrl Pts',(-44.5553847872712,54.6661370216242,
12.));
#153390=CARTESIAN_POINT('Ctrl Pts',(-44.5473125297289,54.6469546367381,
0.));
#153391=CARTESIAN_POINT('Ctrl Pts',(-44.5473125297289,54.6469546367381,
12.));
#153392=CARTESIAN_POINT('Ctrl Pts',(-44.5392398566775,54.6278273743554,
0.));
#153393=CARTESIAN_POINT('Ctrl Pts',(-44.5392398566775,54.6278273743554,
12.));
#153394=CARTESIAN_POINT('Ctrl Pts',(-44.5311669104494,54.6087553602889,
0.));
#153395=CARTESIAN_POINT('Ctrl Pts',(-44.5311669104494,54.6087553602889,
12.));
#153396=CARTESIAN_POINT('Ctrl Pts',(-44.5230938335165,54.5897387202812,
0.));
#153397=CARTESIAN_POINT('Ctrl Pts',(-44.5230938335165,54.5897387202812,
12.));
#153398=CARTESIAN_POINT('Ctrl Pts',(-44.5150207679007,54.5707775794436,
0.));
#153399=CARTESIAN_POINT('Ctrl Pts',(-44.5150207679007,54.5707775794436,
12.));
#153400=CARTESIAN_POINT('Ctrl Pts',(-44.5069478544977,54.5518720616056,
0.));
#153401=CARTESIAN_POINT('Ctrl Pts',(-44.5069478544977,54.5518720616056,
12.));
#153402=CARTESIAN_POINT('Ctrl Pts',(-44.4988752343744,54.5330222905475,
0.));
#153403=CARTESIAN_POINT('Ctrl Pts',(-44.4988752343744,54.5330222905475,
12.));
#153404=CARTESIAN_POINT('Ctrl Pts',(-44.4908030503225,54.5142283914704,
0.));
#153405=CARTESIAN_POINT('Ctrl Pts',(-44.4908030503225,54.5142283914704,
12.));
#153406=CARTESIAN_POINT('Ctrl Pts',(-44.4827314481264,54.495490492193,0.));
#153407=CARTESIAN_POINT('Ctrl Pts',(-44.4827314481264,54.495490492193,12.));
#153408=CARTESIAN_POINT('Ctrl Pts',(-44.4746605784031,54.4768087248824,
0.));
#153409=CARTESIAN_POINT('Ctrl Pts',(-44.4746605784031,54.4768087248824,
12.));
#153410=CARTESIAN_POINT('Ctrl Pts',(-44.4665905967668,54.4581832262033,
0.));
#153411=CARTESIAN_POINT('Ctrl Pts',(-44.4665905967668,54.4581832262033,
12.));
#153412=CARTESIAN_POINT('Ctrl Pts',(-44.4585216599907,54.4396141336978,
0.));
#153413=CARTESIAN_POINT('Ctrl Pts',(-44.4585216599907,54.4396141336978,
12.));
#153414=CARTESIAN_POINT('Ctrl Pts',(-44.4504539226327,54.421101582595,0.));
#153415=CARTESIAN_POINT('Ctrl Pts',(-44.4504539226327,54.421101582595,12.));
#153416=CARTESIAN_POINT('Ctrl Pts',(-44.4423875340995,54.4026457030335,
0.));
#153417=CARTESIAN_POINT('Ctrl Pts',(-44.4423875340995,54.4026457030335,
12.));
#153418=CARTESIAN_POINT('Ctrl Pts',(-44.4343226339592,54.3842466156196,
0.));
#153419=CARTESIAN_POINT('Ctrl Pts',(-44.4343226339592,54.3842466156196,
12.));
#153420=CARTESIAN_POINT('Ctrl Pts',(-44.4262593564712,54.3659044357119,
0.));
#153421=CARTESIAN_POINT('Ctrl Pts',(-44.4262593564712,54.3659044357119,
12.));
#153422=CARTESIAN_POINT('Ctrl Pts',(-44.4181978395851,54.3476192819352,
0.));
#153423=CARTESIAN_POINT('Ctrl Pts',(-44.4181978395851,54.3476192819352,
12.));
#153424=CARTESIAN_POINT('Ctrl Pts',(-44.4101382321834,54.3293912830237,
0.));
#153425=CARTESIAN_POINT('Ctrl Pts',(-44.4101382321834,54.3293912830237,
12.));
#153426=CARTESIAN_POINT('Ctrl Pts',(-44.402080702809,54.3112205860716,0.));
#153427=CARTESIAN_POINT('Ctrl Pts',(-44.402080702809,54.3112205860716,12.));
#153428=CARTESIAN_POINT('Ctrl Pts',(-44.3940254456331,54.2931073621553,
0.));
#153429=CARTESIAN_POINT('Ctrl Pts',(-44.3940254456331,54.2931073621553,
12.));
#153430=CARTESIAN_POINT('Ctrl Pts',(-44.3859726620183,54.2750517888579,
0.));
#153431=CARTESIAN_POINT('Ctrl Pts',(-44.3859726620183,54.2750517888579,
12.));
#153432=CARTESIAN_POINT('Ctrl Pts',(-44.3779225430405,54.2570540336475,
0.));
#153433=CARTESIAN_POINT('Ctrl Pts',(-44.3779225430405,54.2570540336475,
12.));
#153434=CARTESIAN_POINT('Ctrl Pts',(-44.3698752533561,54.2391142386412,
0.));
#153435=CARTESIAN_POINT('Ctrl Pts',(-44.3698752533561,54.2391142386412,
12.));
#153436=CARTESIAN_POINT('Ctrl Pts',(-44.361830910343,54.2212325006052,0.));
#153437=CARTESIAN_POINT('Ctrl Pts',(-44.361830910343,54.2212325006052,12.));
#153438=CARTESIAN_POINT('Ctrl Pts',(-44.3537895824096,54.2034088701928,
0.));
#153439=CARTESIAN_POINT('Ctrl Pts',(-44.3537895824096,54.2034088701928,
12.));
#153440=CARTESIAN_POINT('Ctrl Pts',(-44.3473589597726,54.1891964684727,
0.));
#153441=CARTESIAN_POINT('Ctrl Pts',(-44.3473589597726,54.1891964684727,
12.));
#153442=CARTESIAN_POINT('Ctrl Pts',(-44.3425373700993,54.1785633257639,
0.));
#153443=CARTESIAN_POINT('Ctrl Pts',(-44.3425373700993,54.1785633257639,
12.));
#153444=CARTESIAN_POINT('Ctrl Pts',(-44.3393235891075,54.1714861895346,
0.));
#153445=CARTESIAN_POINT('Ctrl Pts',(-44.3393235891075,54.1714861895346,
12.));
#153446=CARTESIAN_POINT('Ctrl Pts',(-44.3377168516418,54.1679505278134,
0.));
#153447=CARTESIAN_POINT('Ctrl Pts',(-44.3377168516418,54.1679505278134,
12.));
#153448=CARTESIAN_POINT('',(-44.3377168516418,54.1679505278134,12.));
#153449=CARTESIAN_POINT('Ctrl Pts',(-44.3377168516418,54.1679505278134,
12.));
#153450=CARTESIAN_POINT('Ctrl Pts',(-44.3393235891075,54.1714861895346,
12.));
#153451=CARTESIAN_POINT('Ctrl Pts',(-44.3425373700993,54.1785633257639,
12.));
#153452=CARTESIAN_POINT('Ctrl Pts',(-44.3473589597726,54.1891964684727,
12.));
#153453=CARTESIAN_POINT('Ctrl Pts',(-44.3537895824096,54.2034088701928,
12.));
#153454=CARTESIAN_POINT('Ctrl Pts',(-44.361830910343,54.2212325006052,12.));
#153455=CARTESIAN_POINT('Ctrl Pts',(-44.3698752533561,54.2391142386412,
12.));
#153456=CARTESIAN_POINT('Ctrl Pts',(-44.3779225430405,54.2570540336475,
12.));
#153457=CARTESIAN_POINT('Ctrl Pts',(-44.3859726620183,54.2750517888579,
12.));
#153458=CARTESIAN_POINT('Ctrl Pts',(-44.3940254456331,54.2931073621553,
12.));
#153459=CARTESIAN_POINT('Ctrl Pts',(-44.402080702809,54.3112205860716,12.));
#153460=CARTESIAN_POINT('Ctrl Pts',(-44.4101382321834,54.3293912830237,
12.));
#153461=CARTESIAN_POINT('Ctrl Pts',(-44.4181978395851,54.3476192819352,
12.));
#153462=CARTESIAN_POINT('Ctrl Pts',(-44.4262593564712,54.3659044357119,
12.));
#153463=CARTESIAN_POINT('Ctrl Pts',(-44.4343226339592,54.3842466156196,
12.));
#153464=CARTESIAN_POINT('Ctrl Pts',(-44.4423875340995,54.4026457030335,
12.));
#153465=CARTESIAN_POINT('Ctrl Pts',(-44.4504539226327,54.421101582595,12.));
#153466=CARTESIAN_POINT('Ctrl Pts',(-44.4585216599907,54.4396141336978,
12.));
#153467=CARTESIAN_POINT('Ctrl Pts',(-44.4665905967668,54.4581832262033,
12.));
#153468=CARTESIAN_POINT('Ctrl Pts',(-44.4746605784031,54.4768087248824,
12.));
#153469=CARTESIAN_POINT('Ctrl Pts',(-44.4827314481264,54.495490492193,12.));
#153470=CARTESIAN_POINT('Ctrl Pts',(-44.4908030503225,54.5142283914704,
12.));
#153471=CARTESIAN_POINT('Ctrl Pts',(-44.4988752343744,54.5330222905475,
12.));
#153472=CARTESIAN_POINT('Ctrl Pts',(-44.5069478544977,54.5518720616056,
12.));
#153473=CARTESIAN_POINT('Ctrl Pts',(-44.5150207679007,54.5707775794436,
12.));
#153474=CARTESIAN_POINT('Ctrl Pts',(-44.5230938335165,54.5897387202812,
12.));
#153475=CARTESIAN_POINT('Ctrl Pts',(-44.5311669104494,54.6087553602889,
12.));
#153476=CARTESIAN_POINT('Ctrl Pts',(-44.5392398566775,54.6278273743554,
12.));
#153477=CARTESIAN_POINT('Ctrl Pts',(-44.5473125297289,54.6469546367381,
12.));
#153478=CARTESIAN_POINT('Ctrl Pts',(-44.5553847872712,54.6661370216242,
12.));
#153479=CARTESIAN_POINT('Ctrl Pts',(-44.5634564876869,54.685374403676,12.));
#153480=CARTESIAN_POINT('Ctrl Pts',(-44.5715274907637,54.7046666586777,
12.));
#153481=CARTESIAN_POINT('Ctrl Pts',(-44.5795976579476,54.7240136637744,
12.));
#153482=CARTESIAN_POINT('Ctrl Pts',(-44.5876668519676,54.7434152971285,
12.));
#153483=CARTESIAN_POINT('Ctrl Pts',(-44.5957349366062,54.7628714377042,
12.));
#153484=CARTESIAN_POINT('Ctrl Pts',(-44.60380177643,54.7823819650137,12.));
#153485=CARTESIAN_POINT('Ctrl Pts',(-44.6118672364889,54.8019467588258,
12.));
#153486=CARTESIAN_POINT('Ctrl Pts',(-44.6199311823276,54.8215656991817,
12.));
#153487=CARTESIAN_POINT('Ctrl Pts',(-44.6279934801159,54.8412386665264,
12.));
#153488=CARTESIAN_POINT('Ctrl Pts',(-44.6360539967392,54.860965541796,12.));
#153489=CARTESIAN_POINT('Ctrl Pts',(-44.6441125999074,54.8807462065177,
12.));
#153490=CARTESIAN_POINT('Ctrl Pts',(-44.6521691582551,54.9005805428991,
12.));
#153491=CARTESIAN_POINT('Ctrl Pts',(-44.6602235412853,54.9204684337845,
12.));
#153492=CARTESIAN_POINT('Ctrl Pts',(-44.6682756193155,54.9404097626088,
12.));
#153493=CARTESIAN_POINT('Ctrl Pts',(-44.6763252634255,54.9604044133497,
12.));
#153494=CARTESIAN_POINT('Ctrl Pts',(-44.6843723453985,54.9804522704668,
12.));
#153495=CARTESIAN_POINT('Ctrl Pts',(-44.6924167376851,55.0005532188644,
12.));
#153496=CARTESIAN_POINT('Ctrl Pts',(-44.7004583134235,55.020707143922,12.));
#153497=CARTESIAN_POINT('Ctrl Pts',(-44.7084969464509,55.0409139315074,
12.));
#153498=CARTESIAN_POINT('Ctrl Pts',(-44.7165325113165,55.0611734679902,
12.));
#153499=CARTESIAN_POINT('Ctrl Pts',(-44.7245648832988,55.0814856402507,
12.));
#153500=CARTESIAN_POINT('Ctrl Pts',(-44.7325939384042,55.1018503356806,
12.));
#153501=CARTESIAN_POINT('Ctrl Pts',(-44.7406195533482,55.1222674421747,
12.));
#153502=CARTESIAN_POINT('Ctrl Pts',(-44.7486416055419,55.1427368481201,
12.));
#153503=CARTESIAN_POINT('Ctrl Pts',(-44.7566599730771,55.1632584423813,
12.));
#153504=CARTESIAN_POINT('Ctrl Pts',(-44.7646745347108,55.1838321142777,
12.));
#153505=CARTESIAN_POINT('Ctrl Pts',(-44.7726851698618,55.2044577535865,
12.));
#153506=CARTESIAN_POINT('Ctrl Pts',(-44.7806917586077,55.2251352505474,
12.));
#153507=CARTESIAN_POINT('Ctrl Pts',(-44.7886941816823,55.2458644958617,
12.));
#153508=CARTESIAN_POINT('Ctrl Pts',(-44.796692320474,55.2666453806883,12.));
#153509=CARTESIAN_POINT('Ctrl Pts',(-44.8046860570244,55.287477796635,12.));
#153510=CARTESIAN_POINT('Ctrl Pts',(-44.8126752740208,55.3083616357605,
12.));
#153511=CARTESIAN_POINT('Ctrl Pts',(-44.8206598547887,55.3292967905725,
12.));
#153512=CARTESIAN_POINT('Ctrl Pts',(-44.8286396832847,55.3502831540228,
12.));
#153513=CARTESIAN_POINT('Ctrl Pts',(-44.8366146440901,55.3713206194967,
12.));
#153514=CARTESIAN_POINT('Ctrl Pts',(-44.8445846224044,55.3924090808014,
12.));
#153515=CARTESIAN_POINT('Ctrl Pts',(-44.8525495040408,55.4135484321718,
12.));
#153516=CARTESIAN_POINT('Ctrl Pts',(-44.8605091754214,55.4347385682704,
12.));
#153517=CARTESIAN_POINT('Ctrl Pts',(-44.8684635235725,55.4559793841836,
12.));
#153518=CARTESIAN_POINT('Ctrl Pts',(-44.8764124361206,55.4772707754126,
12.));
#153519=CARTESIAN_POINT('Ctrl Pts',(-44.8843558012886,55.4986126378656,
12.));
#153520=CARTESIAN_POINT('Ctrl Pts',(-44.8922935078889,55.5200048678629,
12.));
#153521=CARTESIAN_POINT('Ctrl Pts',(-44.9002254453183,55.541447362134,12.));
#153522=CARTESIAN_POINT('Ctrl Pts',(-44.908151503553,55.5629400178142,12.));
#153523=CARTESIAN_POINT('Ctrl Pts',(-44.9160715731443,55.5844827324338,
12.));
#153524=CARTESIAN_POINT('Ctrl Pts',(-44.9239855452144,55.6060754039121,
12.));
#153525=CARTESIAN_POINT('Ctrl Pts',(-44.9318933114506,55.6277179305633,
12.));
#153526=CARTESIAN_POINT('Ctrl Pts',(-44.9397947641006,55.6494102110935,
12.));
#153527=CARTESIAN_POINT('Ctrl Pts',(-44.9476897959684,55.6711521445979,
12.));
#153528=CARTESIAN_POINT('Ctrl Pts',(-44.9555783004106,55.6929436305489,
12.));
#153529=CARTESIAN_POINT('Ctrl Pts',(-44.9634601713321,55.714784568793,12.));
#153530=CARTESIAN_POINT('Ctrl Pts',(-44.9713353031804,55.7366748595552,
12.));
#153531=CARTESIAN_POINT('Ctrl Pts',(-44.9792035909413,55.7586144034367,
12.));
#153532=CARTESIAN_POINT('Ctrl Pts',(-44.9870649301342,55.7806031014106,
12.));
#153533=CARTESIAN_POINT('Ctrl Pts',(-44.9949192168093,55.8026408548105,
12.));
#153534=CARTESIAN_POINT('Ctrl Pts',(-45.0027663475433,55.8247275653289,
12.));
#153535=CARTESIAN_POINT('Ctrl Pts',(-45.0106062194342,55.8468631350218,
12.));
#153536=CARTESIAN_POINT('Ctrl Pts',(-45.0184387300973,55.8690474663065,
12.));
#153537=CARTESIAN_POINT('Ctrl Pts',(-45.0262637776614,55.8912804619577,
12.));
#153538=CARTESIAN_POINT('Ctrl Pts',(-45.0340812607657,55.9135620250954,
12.));
#153539=CARTESIAN_POINT('Ctrl Pts',(-45.041891078555,55.9358920591837,12.));
#153540=CARTESIAN_POINT('Ctrl Pts',(-45.0496931306755,55.9582704680356,
12.));
#153541=CARTESIAN_POINT('Ctrl Pts',(-45.0574873172694,55.9806971558097,
12.));
#153542=CARTESIAN_POINT('Ctrl Pts',(-45.0652735389733,56.003172027008,12.));
#153543=CARTESIAN_POINT('Ctrl Pts',(-45.0730516969148,56.0256949864639,
12.));
#153544=CARTESIAN_POINT('Ctrl Pts',(-45.0808216927089,56.048265939342,12.));
#153545=CARTESIAN_POINT('Ctrl Pts',(-45.0885834284517,56.0708847911416,
12.));
#153546=CARTESIAN_POINT('Ctrl Pts',(-45.0963368067177,56.0935514476945,
12.));
#153547=CARTESIAN_POINT('Ctrl Pts',(-45.1040817305561,56.116265815162,12.));
#153548=CARTESIAN_POINT('Ctrl Pts',(-45.1118181034888,56.1390278000226,
12.));
#153549=CARTESIAN_POINT('Ctrl Pts',(-45.1195458295062,56.1618373090732,
12.));
#153550=CARTESIAN_POINT('Ctrl Pts',(-45.127264813063,56.1846942494325,12.));
#153551=CARTESIAN_POINT('Ctrl Pts',(-45.1349749590737,56.2075985285393,
12.));
#153552=CARTESIAN_POINT('Ctrl Pts',(-45.1426761729105,56.230550054149,12.));
#153553=CARTESIAN_POINT('Ctrl Pts',(-45.1503683604005,56.2535487343221,
12.));
#153554=CARTESIAN_POINT('Ctrl Pts',(-45.1580514278223,56.2765944774245,
12.));
#153555=CARTESIAN_POINT('Ctrl Pts',(-45.1657252819013,56.2996871921316,
12.));
#153556=CARTESIAN_POINT('Ctrl Pts',(-45.173389829806,56.3228267874264,12.));
#153557=CARTESIAN_POINT('Ctrl Pts',(-45.1810449791453,56.3460131725964,
12.));
#153558=CARTESIAN_POINT('Ctrl Pts',(-45.1886906379667,56.3692462572231,
12.));
#153559=CARTESIAN_POINT('Ctrl Pts',(-45.1963267147529,56.3925259511806,
12.));
#153560=CARTESIAN_POINT('Ctrl Pts',(-45.2039531184171,56.4158521646411,
12.));
#153561=CARTESIAN_POINT('Ctrl Pts',(-45.2115697583,56.4392248080732,12.));
#153562=CARTESIAN_POINT('Ctrl Pts',(-45.2191765441666,56.4626437922386,
12.));
#153563=CARTESIAN_POINT('Ctrl Pts',(-45.2267733862049,56.4861090281823,
12.));
#153564=CARTESIAN_POINT('Ctrl Pts',(-45.2343601950227,56.5096204272306,
12.));
#153565=CARTESIAN_POINT('Ctrl Pts',(-45.2419368816428,56.5331779009958,
12.));
#153566=CARTESIAN_POINT('Ctrl Pts',(-45.2495033575,56.5567813613756,12.));
#153567=CARTESIAN_POINT('Ctrl Pts',(-45.257059534438,56.5804307205505,12.));
#153568=CARTESIAN_POINT('Ctrl Pts',(-45.2646053247087,56.6041258909741,
12.));
#153569=CARTESIAN_POINT('Ctrl Pts',(-45.2721406409695,56.6278667853702,
12.));
#153570=CARTESIAN_POINT('Ctrl Pts',(-45.2796653962785,56.6516533167384,
12.));
#153571=CARTESIAN_POINT('Ctrl Pts',(-45.2871795040906,56.6754853983528,
12.));
#153572=CARTESIAN_POINT('Ctrl Pts',(-45.2946828782559,56.69936294376,12.));
#153573=CARTESIAN_POINT('Ctrl Pts',(-45.3021754330178,56.7232858667709,
12.));
#153574=CARTESIAN_POINT('Ctrl Pts',(-45.3096570830117,56.7472540814554,
12.));
#153575=CARTESIAN_POINT('Ctrl Pts',(-45.31712774326,56.7712675021491,12.));
#153576=CARTESIAN_POINT('Ctrl Pts',(-45.3245873291684,56.7953260434524,
12.));
#153577=CARTESIAN_POINT('Ctrl Pts',(-45.332035756524,56.8194296202291,12.));
#153578=CARTESIAN_POINT('Ctrl Pts',(-45.3394729414931,56.8435781475981,
12.));
#153579=CARTESIAN_POINT('Ctrl Pts',(-45.3468988006203,56.8677715409268,
12.));
#153580=CARTESIAN_POINT('Ctrl Pts',(-45.3543132508238,56.8920097158377,
12.));
#153581=CARTESIAN_POINT('Ctrl Pts',(-45.3617162093922,56.9162925882085,
12.));
#153582=CARTESIAN_POINT('Ctrl Pts',(-45.3691075939826,56.9406200741714,
12.));
#153583=CARTESIAN_POINT('Ctrl Pts',(-45.3764873226196,56.9649920901073,
12.));
#153584=CARTESIAN_POINT('Ctrl Pts',(-45.3838553136948,56.9894085526373,
12.));
#153585=CARTESIAN_POINT('Ctrl Pts',(-45.3912114859616,57.0138693786278,
12.));
#153586=CARTESIAN_POINT('Ctrl Pts',(-45.3985557585311,57.0383744851913,
12.));
#153587=CARTESIAN_POINT('Ctrl Pts',(-45.4058880508693,57.0629237896848,
12.));
#153588=CARTESIAN_POINT('Ctrl Pts',(-45.4132082827948,57.0875172097051,
12.));
#153589=CARTESIAN_POINT('Ctrl Pts',(-45.4205163744781,57.112154663078,12.));
#153590=CARTESIAN_POINT('Ctrl Pts',(-45.4278122464389,57.136836067863,12.));
#153591=CARTESIAN_POINT('Ctrl Pts',(-45.4350958195433,57.1615613423584,
12.));
#153592=CARTESIAN_POINT('Ctrl Pts',(-45.4423670150034,57.186330405101,12.));
#153593=CARTESIAN_POINT('Ctrl Pts',(-45.4496257543759,57.2111431748631,
12.));
#153594=CARTESIAN_POINT('Ctrl Pts',(-45.4568719595641,57.2359995706447,
12.));
#153595=CARTESIAN_POINT('Ctrl Pts',(-45.4641055528141,57.2608995116733,
12.));
#153596=CARTESIAN_POINT('Ctrl Pts',(-45.4713264567063,57.2858429174062,
12.));
#153597=CARTESIAN_POINT('Ctrl Pts',(-45.4785345941507,57.3108297075265,
12.));
#153598=CARTESIAN_POINT('Ctrl Pts',(-45.4857298883824,57.3358598019389,
12.));
#153599=CARTESIAN_POINT('Ctrl Pts',(-45.4929122629572,57.3609331207574,
12.));
#153600=CARTESIAN_POINT('Ctrl Pts',(-45.5000816417509,57.3860495843033,
12.));
#153601=CARTESIAN_POINT('Ctrl Pts',(-45.5072379489631,57.4112091131183,
12.));
#153602=CARTESIAN_POINT('Ctrl Pts',(-45.5143811091205,57.4364116279702,
12.));
#153603=CARTESIAN_POINT('Ctrl Pts',(-45.5215110470825,57.4616570498568,
12.));
#153604=CARTESIAN_POINT('Ctrl Pts',(-45.5286276880484,57.4869453000063,
12.));
#153605=CARTESIAN_POINT('Ctrl Pts',(-45.5357309575611,57.5122762998745,
12.));
#153606=CARTESIAN_POINT('Ctrl Pts',(-45.542820781484,57.537649971135,12.));
#153607=CARTESIAN_POINT('Ctrl Pts',(-45.5498970859834,57.563066235668,12.));
#153608=CARTESIAN_POINT('Ctrl Pts',(-45.5569597975096,57.5885250155433,
12.));
#153609=CARTESIAN_POINT('Ctrl Pts',(-45.5640088427813,57.614026233004,12.));
#153610=CARTESIAN_POINT('Ctrl Pts',(-45.5710441487674,57.6395698104404,
12.));
#153611=CARTESIAN_POINT('Ctrl Pts',(-45.5780656427163,57.6651556704237,
12.));
#153612=CARTESIAN_POINT('Ctrl Pts',(-45.5850732521895,57.6907837357418,
12.));
#153613=CARTESIAN_POINT('Ctrl Pts',(-45.5920669050986,57.7164539294314,
12.));
#153614=CARTESIAN_POINT('Ctrl Pts',(-45.5990465297343,57.7421661748026,
12.));
#153615=CARTESIAN_POINT('Ctrl Pts',(-45.6060120548205,57.7679203954742,
12.));
#153616=CARTESIAN_POINT('Ctrl Pts',(-45.6129634094683,57.7937165153387,
12.));
#153617=CARTESIAN_POINT('Ctrl Pts',(-45.6199005230783,57.8195544584845,
12.));
#153618=CARTESIAN_POINT('Ctrl Pts',(-45.6268233252544,57.8454341491238,
12.));
#153619=CARTESIAN_POINT('Ctrl Pts',(-45.6337317457252,57.8713555115232,
12.));
#153620=CARTESIAN_POINT('Ctrl Pts',(-45.6406257142381,57.8973184699034,
12.));
#153621=CARTESIAN_POINT('Ctrl Pts',(-45.6475051605535,57.9233229484311,
12.));
#153622=CARTESIAN_POINT('Ctrl Pts',(-45.6543700146679,57.9493688714237,
12.));
#153623=CARTESIAN_POINT('Ctrl Pts',(-45.661220206992,57.9754561635061,12.));
#153624=CARTESIAN_POINT('Ctrl Pts',(-45.6680556685493,58.0015847497837,
12.));
#153625=CARTESIAN_POINT('Ctrl Pts',(-45.6748763311643,58.0277545560012,
12.));
#153626=CARTESIAN_POINT('Ctrl Pts',(-45.6816821276678,58.0539655087117,
12.));
#153627=CARTESIAN_POINT('Ctrl Pts',(-45.6884729914485,58.0802175348966,
12.));
#153628=CARTESIAN_POINT('Ctrl Pts',(-45.695248856015,58.1065105615907,12.));
#153629=CARTESIAN_POINT('Ctrl Pts',(-45.702009654518,58.1328445154676,12.));
#153630=CARTESIAN_POINT('Ctrl Pts',(-45.7087553193771,58.1592193225137,
12.));
#153631=CARTESIAN_POINT('Ctrl Pts',(-45.7154857816483,58.185634907469,12.));
#153632=CARTESIAN_POINT('Ctrl Pts',(-45.7222009715397,58.2120911942772,
12.));
#153633=CARTESIAN_POINT('Ctrl Pts',(-45.7289008195578,58.2385881070913,
12.));
#153634=CARTESIAN_POINT('Ctrl Pts',(-45.7355852575106,58.2651255711453,
12.));
#153635=CARTESIAN_POINT('Ctrl Pts',(-45.742254219463,58.291703513584,12.));
#153636=CARTESIAN_POINT('Ctrl Pts',(-45.7489076429763,58.3183218645317,
12.));
#153637=CARTESIAN_POINT('Ctrl Pts',(-45.755545469402,58.3449805573423,12.));
#153638=CARTESIAN_POINT('Ctrl Pts',(-45.7612219538124,58.3678667473438,
12.));
#153639=CARTESIAN_POINT('Ctrl Pts',(-45.7655655205367,58.3854348517444,
12.));
#153640=CARTESIAN_POINT('Ctrl Pts',(-45.7685831165565,58.397667048107,12.));
#153641=CARTESIAN_POINT('Ctrl Pts',(-45.7702793558177,58.4045515723357,
12.));
#153642=CARTESIAN_POINT('Ctrl Pts',(-45.7706564944896,58.4060826907797,
12.));
#153643=CARTESIAN_POINT('',(-44.3377168516418,54.1679505278134,0.));
#153644=CARTESIAN_POINT('',(-44.3377168516418,54.1679505278134,0.));
#153645=CARTESIAN_POINT('Ctrl Pts',(-45.7706564944896,58.4060826907797,
0.));
#153646=CARTESIAN_POINT('Ctrl Pts',(-45.7702793558177,58.4045515723357,
0.));
#153647=CARTESIAN_POINT('Ctrl Pts',(-45.7685831165565,58.397667048107,0.));
#153648=CARTESIAN_POINT('Ctrl Pts',(-45.7655655205367,58.3854348517444,
0.));
#153649=CARTESIAN_POINT('Ctrl Pts',(-45.7612219538124,58.3678667473437,
0.));
#153650=CARTESIAN_POINT('Ctrl Pts',(-45.755545469402,58.3449805573423,0.));
#153651=CARTESIAN_POINT('Ctrl Pts',(-45.7489076429763,58.3183218645317,
0.));
#153652=CARTESIAN_POINT('Ctrl Pts',(-45.742254219463,58.291703513584,0.));
#153653=CARTESIAN_POINT('Ctrl Pts',(-45.7355852575106,58.2651255711453,
0.));
#153654=CARTESIAN_POINT('Ctrl Pts',(-45.7289008195578,58.2385881070913,
0.));
#153655=CARTESIAN_POINT('Ctrl Pts',(-45.7222009715397,58.2120911942772,
0.));
#153656=CARTESIAN_POINT('Ctrl Pts',(-45.7154857816483,58.185634907469,0.));
#153657=CARTESIAN_POINT('Ctrl Pts',(-45.7087553193771,58.1592193225137,
0.));
#153658=CARTESIAN_POINT('Ctrl Pts',(-45.702009654518,58.1328445154676,0.));
#153659=CARTESIAN_POINT('Ctrl Pts',(-45.695248856015,58.1065105615907,0.));
#153660=CARTESIAN_POINT('Ctrl Pts',(-45.6884729914485,58.0802175348966,
0.));
#153661=CARTESIAN_POINT('Ctrl Pts',(-45.6816821276678,58.0539655087117,
0.));
#153662=CARTESIAN_POINT('Ctrl Pts',(-45.6748763311643,58.0277545560012,
0.));
#153663=CARTESIAN_POINT('Ctrl Pts',(-45.6680556685493,58.0015847497837,
0.));
#153664=CARTESIAN_POINT('Ctrl Pts',(-45.661220206992,57.9754561635061,0.));
#153665=CARTESIAN_POINT('Ctrl Pts',(-45.6543700146679,57.9493688714237,
0.));
#153666=CARTESIAN_POINT('Ctrl Pts',(-45.6475051605535,57.9233229484311,
0.));
#153667=CARTESIAN_POINT('Ctrl Pts',(-45.6406257142381,57.8973184699034,
0.));
#153668=CARTESIAN_POINT('Ctrl Pts',(-45.6337317457252,57.8713555115232,
0.));
#153669=CARTESIAN_POINT('Ctrl Pts',(-45.6268233252544,57.8454341491238,
0.));
#153670=CARTESIAN_POINT('Ctrl Pts',(-45.6199005230783,57.8195544584845,
0.));
#153671=CARTESIAN_POINT('Ctrl Pts',(-45.6129634094683,57.7937165153387,
0.));
#153672=CARTESIAN_POINT('Ctrl Pts',(-45.6060120548205,57.7679203954742,
0.));
#153673=CARTESIAN_POINT('Ctrl Pts',(-45.5990465297343,57.7421661748026,
0.));
#153674=CARTESIAN_POINT('Ctrl Pts',(-45.5920669050986,57.7164539294314,
0.));
#153675=CARTESIAN_POINT('Ctrl Pts',(-45.5850732521895,57.6907837357418,
0.));
#153676=CARTESIAN_POINT('Ctrl Pts',(-45.5780656427163,57.6651556704237,
0.));
#153677=CARTESIAN_POINT('Ctrl Pts',(-45.5710441487674,57.6395698104404,
0.));
#153678=CARTESIAN_POINT('Ctrl Pts',(-45.5640088427813,57.614026233004,0.));
#153679=CARTESIAN_POINT('Ctrl Pts',(-45.5569597975096,57.5885250155433,
0.));
#153680=CARTESIAN_POINT('Ctrl Pts',(-45.5498970859834,57.563066235668,0.));
#153681=CARTESIAN_POINT('Ctrl Pts',(-45.542820781484,57.537649971135,0.));
#153682=CARTESIAN_POINT('Ctrl Pts',(-45.5357309575611,57.5122762998745,
0.));
#153683=CARTESIAN_POINT('Ctrl Pts',(-45.5286276880484,57.4869453000063,
0.));
#153684=CARTESIAN_POINT('Ctrl Pts',(-45.5215110470825,57.4616570498568,
0.));
#153685=CARTESIAN_POINT('Ctrl Pts',(-45.5143811091205,57.4364116279702,
0.));
#153686=CARTESIAN_POINT('Ctrl Pts',(-45.5072379489631,57.4112091131183,
0.));
#153687=CARTESIAN_POINT('Ctrl Pts',(-45.5000816417509,57.3860495843033,
0.));
#153688=CARTESIAN_POINT('Ctrl Pts',(-45.4929122629572,57.3609331207574,
0.));
#153689=CARTESIAN_POINT('Ctrl Pts',(-45.4857298883824,57.3358598019389,
0.));
#153690=CARTESIAN_POINT('Ctrl Pts',(-45.4785345941507,57.3108297075265,
0.));
#153691=CARTESIAN_POINT('Ctrl Pts',(-45.4713264567063,57.2858429174062,
0.));
#153692=CARTESIAN_POINT('Ctrl Pts',(-45.4641055528141,57.2608995116733,
0.));
#153693=CARTESIAN_POINT('Ctrl Pts',(-45.4568719595641,57.2359995706447,
0.));
#153694=CARTESIAN_POINT('Ctrl Pts',(-45.4496257543759,57.2111431748631,
0.));
#153695=CARTESIAN_POINT('Ctrl Pts',(-45.4423670150034,57.186330405101,0.));
#153696=CARTESIAN_POINT('Ctrl Pts',(-45.4350958195433,57.1615613423584,
0.));
#153697=CARTESIAN_POINT('Ctrl Pts',(-45.4278122464389,57.136836067863,0.));
#153698=CARTESIAN_POINT('Ctrl Pts',(-45.4205163744781,57.112154663078,0.));
#153699=CARTESIAN_POINT('Ctrl Pts',(-45.4132082827948,57.0875172097051,
0.));
#153700=CARTESIAN_POINT('Ctrl Pts',(-45.4058880508693,57.0629237896848,
0.));
#153701=CARTESIAN_POINT('Ctrl Pts',(-45.3985557585311,57.0383744851913,
0.));
#153702=CARTESIAN_POINT('Ctrl Pts',(-45.3912114859616,57.0138693786278,
0.));
#153703=CARTESIAN_POINT('Ctrl Pts',(-45.3838553136948,56.9894085526373,
0.));
#153704=CARTESIAN_POINT('Ctrl Pts',(-45.3764873226196,56.9649920901073,
0.));
#153705=CARTESIAN_POINT('Ctrl Pts',(-45.3691075939826,56.9406200741714,
0.));
#153706=CARTESIAN_POINT('Ctrl Pts',(-45.3617162093922,56.9162925882085,
0.));
#153707=CARTESIAN_POINT('Ctrl Pts',(-45.3543132508238,56.8920097158377,
0.));
#153708=CARTESIAN_POINT('Ctrl Pts',(-45.3468988006203,56.8677715409268,
0.));
#153709=CARTESIAN_POINT('Ctrl Pts',(-45.3394729414931,56.8435781475981,
0.));
#153710=CARTESIAN_POINT('Ctrl Pts',(-45.332035756524,56.8194296202291,0.));
#153711=CARTESIAN_POINT('Ctrl Pts',(-45.3245873291684,56.7953260434524,
0.));
#153712=CARTESIAN_POINT('Ctrl Pts',(-45.31712774326,56.7712675021491,0.));
#153713=CARTESIAN_POINT('Ctrl Pts',(-45.3096570830117,56.7472540814554,
0.));
#153714=CARTESIAN_POINT('Ctrl Pts',(-45.3021754330178,56.7232858667709,
0.));
#153715=CARTESIAN_POINT('Ctrl Pts',(-45.2946828782559,56.69936294376,0.));
#153716=CARTESIAN_POINT('Ctrl Pts',(-45.2871795040906,56.6754853983528,
0.));
#153717=CARTESIAN_POINT('Ctrl Pts',(-45.2796653962785,56.6516533167384,
0.));
#153718=CARTESIAN_POINT('Ctrl Pts',(-45.2721406409695,56.6278667853702,
0.));
#153719=CARTESIAN_POINT('Ctrl Pts',(-45.2646053247087,56.6041258909741,
0.));
#153720=CARTESIAN_POINT('Ctrl Pts',(-45.257059534438,56.5804307205505,0.));
#153721=CARTESIAN_POINT('Ctrl Pts',(-45.2495033575,56.5567813613756,0.));
#153722=CARTESIAN_POINT('Ctrl Pts',(-45.2419368816428,56.5331779009958,
0.));
#153723=CARTESIAN_POINT('Ctrl Pts',(-45.2343601950227,56.5096204272306,
0.));
#153724=CARTESIAN_POINT('Ctrl Pts',(-45.2267733862049,56.4861090281823,
0.));
#153725=CARTESIAN_POINT('Ctrl Pts',(-45.2191765441666,56.4626437922386,
0.));
#153726=CARTESIAN_POINT('Ctrl Pts',(-45.2115697583,56.4392248080732,0.));
#153727=CARTESIAN_POINT('Ctrl Pts',(-45.2039531184171,56.4158521646411,
0.));
#153728=CARTESIAN_POINT('Ctrl Pts',(-45.1963267147529,56.3925259511806,
0.));
#153729=CARTESIAN_POINT('Ctrl Pts',(-45.1886906379667,56.3692462572231,
0.));
#153730=CARTESIAN_POINT('Ctrl Pts',(-45.1810449791453,56.3460131725964,
0.));
#153731=CARTESIAN_POINT('Ctrl Pts',(-45.173389829806,56.3228267874264,0.));
#153732=CARTESIAN_POINT('Ctrl Pts',(-45.1657252819013,56.2996871921316,
0.));
#153733=CARTESIAN_POINT('Ctrl Pts',(-45.1580514278223,56.2765944774245,
0.));
#153734=CARTESIAN_POINT('Ctrl Pts',(-45.1503683604005,56.2535487343221,
0.));
#153735=CARTESIAN_POINT('Ctrl Pts',(-45.1426761729105,56.230550054149,0.));
#153736=CARTESIAN_POINT('Ctrl Pts',(-45.1349749590737,56.2075985285393,
0.));
#153737=CARTESIAN_POINT('Ctrl Pts',(-45.127264813063,56.1846942494325,0.));
#153738=CARTESIAN_POINT('Ctrl Pts',(-45.1195458295062,56.1618373090732,
0.));
#153739=CARTESIAN_POINT('Ctrl Pts',(-45.1118181034888,56.1390278000226,
0.));
#153740=CARTESIAN_POINT('Ctrl Pts',(-45.1040817305561,56.116265815162,0.));
#153741=CARTESIAN_POINT('Ctrl Pts',(-45.0963368067177,56.0935514476945,
0.));
#153742=CARTESIAN_POINT('Ctrl Pts',(-45.0885834284517,56.0708847911416,
0.));
#153743=CARTESIAN_POINT('Ctrl Pts',(-45.0808216927089,56.048265939342,0.));
#153744=CARTESIAN_POINT('Ctrl Pts',(-45.0730516969148,56.0256949864639,
0.));
#153745=CARTESIAN_POINT('Ctrl Pts',(-45.0652735389733,56.003172027008,0.));
#153746=CARTESIAN_POINT('Ctrl Pts',(-45.0574873172694,55.9806971558097,
0.));
#153747=CARTESIAN_POINT('Ctrl Pts',(-45.0496931306755,55.9582704680356,
0.));
#153748=CARTESIAN_POINT('Ctrl Pts',(-45.041891078555,55.9358920591837,0.));
#153749=CARTESIAN_POINT('Ctrl Pts',(-45.0340812607657,55.9135620250954,
0.));
#153750=CARTESIAN_POINT('Ctrl Pts',(-45.0262637776614,55.8912804619577,
0.));
#153751=CARTESIAN_POINT('Ctrl Pts',(-45.0184387300973,55.8690474663065,
0.));
#153752=CARTESIAN_POINT('Ctrl Pts',(-45.0106062194342,55.8468631350218,
0.));
#153753=CARTESIAN_POINT('Ctrl Pts',(-45.0027663475433,55.8247275653289,
0.));
#153754=CARTESIAN_POINT('Ctrl Pts',(-44.9949192168093,55.8026408548105,
0.));
#153755=CARTESIAN_POINT('Ctrl Pts',(-44.9870649301342,55.7806031014106,
0.));
#153756=CARTESIAN_POINT('Ctrl Pts',(-44.9792035909413,55.7586144034367,
0.));
#153757=CARTESIAN_POINT('Ctrl Pts',(-44.9713353031804,55.7366748595552,
0.));
#153758=CARTESIAN_POINT('Ctrl Pts',(-44.9634601713321,55.714784568793,0.));
#153759=CARTESIAN_POINT('Ctrl Pts',(-44.9555783004106,55.6929436305489,
0.));
#153760=CARTESIAN_POINT('Ctrl Pts',(-44.9476897959684,55.6711521445979,
0.));
#153761=CARTESIAN_POINT('Ctrl Pts',(-44.9397947641006,55.6494102110935,
0.));
#153762=CARTESIAN_POINT('Ctrl Pts',(-44.9318933114506,55.6277179305633,
0.));
#153763=CARTESIAN_POINT('Ctrl Pts',(-44.9239855452144,55.6060754039121,
0.));
#153764=CARTESIAN_POINT('Ctrl Pts',(-44.9160715731443,55.5844827324338,
0.));
#153765=CARTESIAN_POINT('Ctrl Pts',(-44.908151503553,55.5629400178142,0.));
#153766=CARTESIAN_POINT('Ctrl Pts',(-44.9002254453183,55.541447362134,0.));
#153767=CARTESIAN_POINT('Ctrl Pts',(-44.8922935078889,55.5200048678629,
0.));
#153768=CARTESIAN_POINT('Ctrl Pts',(-44.8843558012886,55.4986126378656,
0.));
#153769=CARTESIAN_POINT('Ctrl Pts',(-44.8764124361206,55.4772707754126,
0.));
#153770=CARTESIAN_POINT('Ctrl Pts',(-44.8684635235725,55.4559793841836,
0.));
#153771=CARTESIAN_POINT('Ctrl Pts',(-44.8605091754214,55.4347385682704,
0.));
#153772=CARTESIAN_POINT('Ctrl Pts',(-44.8525495040408,55.4135484321718,
0.));
#153773=CARTESIAN_POINT('Ctrl Pts',(-44.8445846224044,55.3924090808014,
0.));
#153774=CARTESIAN_POINT('Ctrl Pts',(-44.8366146440901,55.3713206194967,
0.));
#153775=CARTESIAN_POINT('Ctrl Pts',(-44.8286396832847,55.3502831540228,
0.));
#153776=CARTESIAN_POINT('Ctrl Pts',(-44.8206598547887,55.3292967905725,
0.));
#153777=CARTESIAN_POINT('Ctrl Pts',(-44.8126752740208,55.3083616357605,
0.));
#153778=CARTESIAN_POINT('Ctrl Pts',(-44.8046860570244,55.287477796635,0.));
#153779=CARTESIAN_POINT('Ctrl Pts',(-44.796692320474,55.2666453806883,0.));
#153780=CARTESIAN_POINT('Ctrl Pts',(-44.7886941816823,55.2458644958617,
0.));
#153781=CARTESIAN_POINT('Ctrl Pts',(-44.7806917586077,55.2251352505474,
0.));
#153782=CARTESIAN_POINT('Ctrl Pts',(-44.7726851698618,55.2044577535865,
0.));
#153783=CARTESIAN_POINT('Ctrl Pts',(-44.7646745347108,55.1838321142777,
0.));
#153784=CARTESIAN_POINT('Ctrl Pts',(-44.7566599730771,55.1632584423813,
0.));
#153785=CARTESIAN_POINT('Ctrl Pts',(-44.7486416055419,55.1427368481201,
0.));
#153786=CARTESIAN_POINT('Ctrl Pts',(-44.7406195533482,55.1222674421747,
0.));
#153787=CARTESIAN_POINT('Ctrl Pts',(-44.7325939384042,55.1018503356806,
0.));
#153788=CARTESIAN_POINT('Ctrl Pts',(-44.7245648832988,55.0814856402507,
0.));
#153789=CARTESIAN_POINT('Ctrl Pts',(-44.7165325113165,55.0611734679902,
0.));
#153790=CARTESIAN_POINT('Ctrl Pts',(-44.7084969464509,55.0409139315074,
0.));
#153791=CARTESIAN_POINT('Ctrl Pts',(-44.7004583134235,55.020707143922,0.));
#153792=CARTESIAN_POINT('Ctrl Pts',(-44.6924167376851,55.0005532188644,
0.));
#153793=CARTESIAN_POINT('Ctrl Pts',(-44.6843723453985,54.9804522704668,
0.));
#153794=CARTESIAN_POINT('Ctrl Pts',(-44.6763252634255,54.9604044133497,
0.));
#153795=CARTESIAN_POINT('Ctrl Pts',(-44.6682756193155,54.9404097626088,
0.));
#153796=CARTESIAN_POINT('Ctrl Pts',(-44.6602235412853,54.9204684337845,
0.));
#153797=CARTESIAN_POINT('Ctrl Pts',(-44.6521691582551,54.9005805428991,
0.));
#153798=CARTESIAN_POINT('Ctrl Pts',(-44.6441125999074,54.8807462065177,
0.));
#153799=CARTESIAN_POINT('Ctrl Pts',(-44.6360539967392,54.860965541796,0.));
#153800=CARTESIAN_POINT('Ctrl Pts',(-44.6279934801159,54.8412386665264,
0.));
#153801=CARTESIAN_POINT('Ctrl Pts',(-44.6199311823276,54.8215656991817,
0.));
#153802=CARTESIAN_POINT('Ctrl Pts',(-44.6118672364889,54.8019467588258,
0.));
#153803=CARTESIAN_POINT('Ctrl Pts',(-44.60380177643,54.7823819650137,0.));
#153804=CARTESIAN_POINT('Ctrl Pts',(-44.5957349366062,54.7628714377042,
0.));
#153805=CARTESIAN_POINT('Ctrl Pts',(-44.5876668519676,54.7434152971285,
0.));
#153806=CARTESIAN_POINT('Ctrl Pts',(-44.5795976579476,54.7240136637744,
0.));
#153807=CARTESIAN_POINT('Ctrl Pts',(-44.5715274907637,54.7046666586777,
0.));
#153808=CARTESIAN_POINT('Ctrl Pts',(-44.5634564876869,54.685374403676,0.));
#153809=CARTESIAN_POINT('Ctrl Pts',(-44.5553847872712,54.6661370216242,
0.));
#153810=CARTESIAN_POINT('Ctrl Pts',(-44.5473125297289,54.6469546367381,
0.));
#153811=CARTESIAN_POINT('Ctrl Pts',(-44.5392398566775,54.6278273743554,
0.));
#153812=CARTESIAN_POINT('Ctrl Pts',(-44.5311669104494,54.6087553602889,
0.));
#153813=CARTESIAN_POINT('Ctrl Pts',(-44.5230938335165,54.5897387202812,
0.));
#153814=CARTESIAN_POINT('Ctrl Pts',(-44.5150207679007,54.5707775794436,
0.));
#153815=CARTESIAN_POINT('Ctrl Pts',(-44.5069478544977,54.5518720616056,
0.));
#153816=CARTESIAN_POINT('Ctrl Pts',(-44.4988752343744,54.5330222905475,
0.));
#153817=CARTESIAN_POINT('Ctrl Pts',(-44.4908030503225,54.5142283914704,
0.));
#153818=CARTESIAN_POINT('Ctrl Pts',(-44.4827314481264,54.495490492193,0.));
#153819=CARTESIAN_POINT('Ctrl Pts',(-44.4746605784031,54.4768087248824,
0.));
#153820=CARTESIAN_POINT('Ctrl Pts',(-44.4665905967668,54.4581832262033,
0.));
#153821=CARTESIAN_POINT('Ctrl Pts',(-44.4585216599907,54.4396141336978,
0.));
#153822=CARTESIAN_POINT('Ctrl Pts',(-44.4504539226327,54.421101582595,0.));
#153823=CARTESIAN_POINT('Ctrl Pts',(-44.4423875340995,54.4026457030335,
0.));
#153824=CARTESIAN_POINT('Ctrl Pts',(-44.4343226339592,54.3842466156196,
0.));
#153825=CARTESIAN_POINT('Ctrl Pts',(-44.4262593564712,54.3659044357119,
0.));
#153826=CARTESIAN_POINT('Ctrl Pts',(-44.4181978395851,54.3476192819352,
0.));
#153827=CARTESIAN_POINT('Ctrl Pts',(-44.4101382321834,54.3293912830237,
0.));
#153828=CARTESIAN_POINT('Ctrl Pts',(-44.402080702809,54.3112205860716,0.));
#153829=CARTESIAN_POINT('Ctrl Pts',(-44.3940254456331,54.2931073621553,
0.));
#153830=CARTESIAN_POINT('Ctrl Pts',(-44.3859726620183,54.2750517888579,
0.));
#153831=CARTESIAN_POINT('Ctrl Pts',(-44.3779225430405,54.2570540336475,
0.));
#153832=CARTESIAN_POINT('Ctrl Pts',(-44.3698752533561,54.2391142386412,
0.));
#153833=CARTESIAN_POINT('Ctrl Pts',(-44.361830910343,54.2212325006052,0.));
#153834=CARTESIAN_POINT('Ctrl Pts',(-44.3537895824096,54.2034088701928,
0.));
#153835=CARTESIAN_POINT('Ctrl Pts',(-44.3473589597726,54.1891964684727,
0.));
#153836=CARTESIAN_POINT('Ctrl Pts',(-44.3425373700993,54.1785633257639,
0.));
#153837=CARTESIAN_POINT('Ctrl Pts',(-44.3393235891075,54.1714861895346,
0.));
#153838=CARTESIAN_POINT('Ctrl Pts',(-44.3377168516418,54.1679505278134,
0.));
#153839=CARTESIAN_POINT('Ctrl Pts',(-40.5543412808469,62.494763006804,0.));
#153840=CARTESIAN_POINT('Ctrl Pts',(-40.5543412808469,62.494763006804,12.));
#153841=CARTESIAN_POINT('Ctrl Pts',(-40.5535399497519,62.489224912198,0.));
#153842=CARTESIAN_POINT('Ctrl Pts',(-40.5535399497519,62.489224912198,12.));
#153843=CARTESIAN_POINT('Ctrl Pts',(-40.5519353177252,62.4781525156318,
0.));
#153844=CARTESIAN_POINT('Ctrl Pts',(-40.5519353177252,62.4781525156318,
12.));
#153845=CARTESIAN_POINT('Ctrl Pts',(-40.5495224601758,62.4615552987202,
0.));
#153846=CARTESIAN_POINT('Ctrl Pts',(-40.5495224601758,62.4615552987202,
12.));
#153847=CARTESIAN_POINT('Ctrl Pts',(-40.5462934972718,62.4394484329678,
0.));
#153848=CARTESIAN_POINT('Ctrl Pts',(-40.5462934972718,62.4394484329678,
12.));
#153849=CARTESIAN_POINT('Ctrl Pts',(-40.5422375945026,62.4118527881148,
0.));
#153850=CARTESIAN_POINT('Ctrl Pts',(-40.5422375945026,62.4118527881148,
12.));
#153851=CARTESIAN_POINT('Ctrl Pts',(-40.5381619974169,62.3842950992833,
0.));
#153852=CARTESIAN_POINT('Ctrl Pts',(-40.5381619974169,62.3842950992833,
12.));
#153853=CARTESIAN_POINT('Ctrl Pts',(-40.5340667194319,62.3567753970279,
0.));
#153854=CARTESIAN_POINT('Ctrl Pts',(-40.5340667194319,62.3567753970279,
12.));
#153855=CARTESIAN_POINT('Ctrl Pts',(-40.5299517857721,62.3292937257901,
0.));
#153856=CARTESIAN_POINT('Ctrl Pts',(-40.5299517857721,62.3292937257901,
12.));
#153857=CARTESIAN_POINT('Ctrl Pts',(-40.5258172381428,62.301850147165,0.));
#153858=CARTESIAN_POINT('Ctrl Pts',(-40.5258172381428,62.301850147165,12.));
#153859=CARTESIAN_POINT('Ctrl Pts',(-40.5216631336193,62.2744447381971,
0.));
#153860=CARTESIAN_POINT('Ctrl Pts',(-40.5216631336193,62.2744447381971,
12.));
#153861=CARTESIAN_POINT('Ctrl Pts',(-40.5174895390954,62.247077585866,0.));
#153862=CARTESIAN_POINT('Ctrl Pts',(-40.5174895390954,62.247077585866,12.));
#153863=CARTESIAN_POINT('Ctrl Pts',(-40.5132965269633,62.2197487826136,
0.));
#153864=CARTESIAN_POINT('Ctrl Pts',(-40.5132965269633,62.2197487826136,
12.));
#153865=CARTESIAN_POINT('Ctrl Pts',(-40.5090841704122,62.1924584215653,
0.));
#153866=CARTESIAN_POINT('Ctrl Pts',(-40.5090841704122,62.1924584215653,
12.));
#153867=CARTESIAN_POINT('Ctrl Pts',(-40.5048525386035,62.1652065915808,
0.));
#153868=CARTESIAN_POINT('Ctrl Pts',(-40.5048525386035,62.1652065915808,
12.));
#153869=CARTESIAN_POINT('Ctrl Pts',(-40.5006016927554,62.1379933732528,
0.));
#153870=CARTESIAN_POINT('Ctrl Pts',(-40.5006016927554,62.1379933732528,
12.));
#153871=CARTESIAN_POINT('Ctrl Pts',(-40.4963316888412,62.1108188417003,
0.));
#153872=CARTESIAN_POINT('Ctrl Pts',(-40.4963316888412,62.1108188417003,
12.));
#153873=CARTESIAN_POINT('Ctrl Pts',(-40.4920425795216,62.0836830685719,
0.));
#153874=CARTESIAN_POINT('Ctrl Pts',(-40.4920425795216,62.0836830685719,
12.));
#153875=CARTESIAN_POINT('Ctrl Pts',(-40.4877344164411,62.0565861244179,
0.));
#153876=CARTESIAN_POINT('Ctrl Pts',(-40.4877344164411,62.0565861244179,
12.));
#153877=CARTESIAN_POINT('Ctrl Pts',(-40.4834072522164,62.029528080742,0.));
#153878=CARTESIAN_POINT('Ctrl Pts',(-40.4834072522164,62.029528080742,12.));
#153879=CARTESIAN_POINT('Ctrl Pts',(-40.4790611429583,62.0025090125959,
0.));
#153880=CARTESIAN_POINT('Ctrl Pts',(-40.4790611429583,62.0025090125959,
12.));
#153881=CARTESIAN_POINT('Ctrl Pts',(-40.4746961480015,61.9755289983044,
0.));
#153882=CARTESIAN_POINT('Ctrl Pts',(-40.4746961480015,61.9755289983044,
12.));
#153883=CARTESIAN_POINT('Ctrl Pts',(-40.470312328762,61.9485881182921,0.));
#153884=CARTESIAN_POINT('Ctrl Pts',(-40.470312328762,61.9485881182921,12.));
#153885=CARTESIAN_POINT('Ctrl Pts',(-40.4659097478587,61.9216864541744,
0.));
#153886=CARTESIAN_POINT('Ctrl Pts',(-40.4659097478587,61.9216864541744,
12.));
#153887=CARTESIAN_POINT('Ctrl Pts',(-40.4614884681889,61.8948240878008,
0.));
#153888=CARTESIAN_POINT('Ctrl Pts',(-40.4614884681889,61.8948240878008,
12.));
#153889=CARTESIAN_POINT('Ctrl Pts',(-40.4570485518749,61.8680011001537,
0.));
#153890=CARTESIAN_POINT('Ctrl Pts',(-40.4570485518749,61.8680011001537,
12.));
#153891=CARTESIAN_POINT('Ctrl Pts',(-40.4525900597894,61.8412175708552,
0.));
#153892=CARTESIAN_POINT('Ctrl Pts',(-40.4525900597894,61.8412175708552,
12.));
#153893=CARTESIAN_POINT('Ctrl Pts',(-40.4481130521364,61.814473578779,0.));
#153894=CARTESIAN_POINT('Ctrl Pts',(-40.4481130521364,61.814473578779,12.));
#153895=CARTESIAN_POINT('Ctrl Pts',(-40.4436175887949,61.7877692024076,
0.));
#153896=CARTESIAN_POINT('Ctrl Pts',(-40.4436175887949,61.7877692024076,
12.));
#153897=CARTESIAN_POINT('Ctrl Pts',(-40.4391037297588,61.7611045202874,
0.));
#153898=CARTESIAN_POINT('Ctrl Pts',(-40.4391037297588,61.7611045202874,
12.));
#153899=CARTESIAN_POINT('Ctrl Pts',(-40.4345715355404,61.7344796114399,
0.));
#153900=CARTESIAN_POINT('Ctrl Pts',(-40.4345715355404,61.7344796114399,
12.));
#153901=CARTESIAN_POINT('Ctrl Pts',(-40.430021067584,61.7078945557799,0.));
#153902=CARTESIAN_POINT('Ctrl Pts',(-40.430021067584,61.7078945557799,12.));
#153903=CARTESIAN_POINT('Ctrl Pts',(-40.425452388076,61.6813494339286,0.));
#153904=CARTESIAN_POINT('Ctrl Pts',(-40.425452388076,61.6813494339286,12.));
#153905=CARTESIAN_POINT('Ctrl Pts',(-40.4208655597717,61.6548443270394,
0.));
#153906=CARTESIAN_POINT('Ctrl Pts',(-40.4208655597717,61.6548443270394,
12.));
#153907=CARTESIAN_POINT('Ctrl Pts',(-40.4162606458119,61.628379316608,0.));
#153908=CARTESIAN_POINT('Ctrl Pts',(-40.4162606458119,61.628379316608,12.));
#153909=CARTESIAN_POINT('Ctrl Pts',(-40.4116377095596,61.601954484301,0.));
#153910=CARTESIAN_POINT('Ctrl Pts',(-40.4116377095596,61.601954484301,12.));
#153911=CARTESIAN_POINT('Ctrl Pts',(-40.4069968143956,61.5755699117324,
0.));
#153912=CARTESIAN_POINT('Ctrl Pts',(-40.4069968143956,61.5755699117324,
12.));
#153913=CARTESIAN_POINT('Ctrl Pts',(-40.4023380237232,61.5492256804717,
0.));
#153914=CARTESIAN_POINT('Ctrl Pts',(-40.4023380237232,61.5492256804717,
12.));
#153915=CARTESIAN_POINT('Ctrl Pts',(-40.3976614010652,61.522921872154,0.));
#153916=CARTESIAN_POINT('Ctrl Pts',(-40.3976614010652,61.522921872154,12.));
#153917=CARTESIAN_POINT('Ctrl Pts',(-40.3929670101366,61.4966585685549,
0.));
#153918=CARTESIAN_POINT('Ctrl Pts',(-40.3929670101366,61.4966585685549,
12.));
#153919=CARTESIAN_POINT('Ctrl Pts',(-40.3882549149227,61.4704358516709,
0.));
#153920=CARTESIAN_POINT('Ctrl Pts',(-40.3882549149227,61.4704358516709,
12.));
#153921=CARTESIAN_POINT('Ctrl Pts',(-40.383525179772,61.4442538038044,0.));
#153922=CARTESIAN_POINT('Ctrl Pts',(-40.383525179772,61.4442538038044,12.));
#153923=CARTESIAN_POINT('Ctrl Pts',(-40.3787778694364,61.4181125076037,
0.));
#153924=CARTESIAN_POINT('Ctrl Pts',(-40.3787778694364,61.4181125076037,
12.));
#153925=CARTESIAN_POINT('Ctrl Pts',(-40.3740130490225,61.3920120460219,
0.));
#153926=CARTESIAN_POINT('Ctrl Pts',(-40.3740130490225,61.3920120460219,
12.));
#153927=CARTESIAN_POINT('Ctrl Pts',(-40.3692307839636,61.3659525022908,
0.));
#153928=CARTESIAN_POINT('Ctrl Pts',(-40.3692307839636,61.3659525022908,
12.));
#153929=CARTESIAN_POINT('Ctrl Pts',(-40.3644311399861,61.3399339598853,
0.));
#153930=CARTESIAN_POINT('Ctrl Pts',(-40.3644311399861,61.3399339598853,
12.));
#153931=CARTESIAN_POINT('Ctrl Pts',(-40.3596141830791,61.3139565024847,
0.));
#153932=CARTESIAN_POINT('Ctrl Pts',(-40.3596141830791,61.3139565024847,
12.));
#153933=CARTESIAN_POINT('Ctrl Pts',(-40.3547799794679,61.2880202139371,
0.));
#153934=CARTESIAN_POINT('Ctrl Pts',(-40.3547799794679,61.2880202139371,
12.));
#153935=CARTESIAN_POINT('Ctrl Pts',(-40.3499285956304,61.2621251782863,
0.));
#153936=CARTESIAN_POINT('Ctrl Pts',(-40.3499285956304,61.2621251782863,
12.));
#153937=CARTESIAN_POINT('Ctrl Pts',(-40.3450600983109,61.23627147979,0.));
#153938=CARTESIAN_POINT('Ctrl Pts',(-40.3450600983109,61.23627147979,12.));
#153939=CARTESIAN_POINT('Ctrl Pts',(-40.340174554537,61.2104592029377,0.));
#153940=CARTESIAN_POINT('Ctrl Pts',(-40.340174554537,61.2104592029377,12.));
#153941=CARTESIAN_POINT('Ctrl Pts',(-40.335272031637,61.1846884324644,0.));
#153942=CARTESIAN_POINT('Ctrl Pts',(-40.335272031637,61.1846884324644,12.));
#153943=CARTESIAN_POINT('Ctrl Pts',(-40.3303525972615,61.1589592533613,
0.));
#153944=CARTESIAN_POINT('Ctrl Pts',(-40.3303525972615,61.1589592533613,
12.));
#153945=CARTESIAN_POINT('Ctrl Pts',(-40.32541631938,61.1332717508789,0.));
#153946=CARTESIAN_POINT('Ctrl Pts',(-40.32541631938,61.1332717508789,12.));
#153947=CARTESIAN_POINT('Ctrl Pts',(-40.3204632662725,61.1076260105258,
0.));
#153948=CARTESIAN_POINT('Ctrl Pts',(-40.3204632662725,61.1076260105258,
12.));
#153949=CARTESIAN_POINT('Ctrl Pts',(-40.3154935065262,61.0820221180645,
0.));
#153950=CARTESIAN_POINT('Ctrl Pts',(-40.3154935065262,61.0820221180645,
12.));
#153951=CARTESIAN_POINT('Ctrl Pts',(-40.3105071090309,61.056460159505,0.));
#153952=CARTESIAN_POINT('Ctrl Pts',(-40.3105071090309,61.056460159505,12.));
#153953=CARTESIAN_POINT('Ctrl Pts',(-40.3055041429775,61.0309402210921,
0.));
#153954=CARTESIAN_POINT('Ctrl Pts',(-40.3055041429775,61.0309402210921,
12.));
#153955=CARTESIAN_POINT('Ctrl Pts',(-40.300484677858,61.0054623893066,0.));
#153956=CARTESIAN_POINT('Ctrl Pts',(-40.300484677858,61.0054623893066,12.));
#153957=CARTESIAN_POINT('Ctrl Pts',(-40.295448783469,60.9800267508786,0.));
#153958=CARTESIAN_POINT('Ctrl Pts',(-40.295448783469,60.9800267508786,12.));
#153959=CARTESIAN_POINT('Ctrl Pts',(-40.2903965299155,60.9546333927921,
0.));
#153960=CARTESIAN_POINT('Ctrl Pts',(-40.2903965299155,60.9546333927921,
12.));
#153961=CARTESIAN_POINT('Ctrl Pts',(-40.2853279876161,60.9292824022887,
0.));
#153962=CARTESIAN_POINT('Ctrl Pts',(-40.2853279876161,60.9292824022887,
12.));
#153963=CARTESIAN_POINT('Ctrl Pts',(-40.2802432273104,60.9039738668669,
0.));
#153964=CARTESIAN_POINT('Ctrl Pts',(-40.2802432273104,60.9039738668669,
12.));
#153965=CARTESIAN_POINT('Ctrl Pts',(-40.2751423200639,60.8787078742818,
0.));
#153966=CARTESIAN_POINT('Ctrl Pts',(-40.2751423200639,60.8787078742818,
12.));
#153967=CARTESIAN_POINT('Ctrl Pts',(-40.2700253372647,60.8534845125538,
0.));
#153968=CARTESIAN_POINT('Ctrl Pts',(-40.2700253372647,60.8534845125538,
12.));
#153969=CARTESIAN_POINT('Ctrl Pts',(-40.2648923506248,60.8283038699706,
0.));
#153970=CARTESIAN_POINT('Ctrl Pts',(-40.2648923506248,60.8283038699706,
12.));
#153971=CARTESIAN_POINT('Ctrl Pts',(-40.2597434321803,60.8031660350879,
0.));
#153972=CARTESIAN_POINT('Ctrl Pts',(-40.2597434321803,60.8031660350879,
12.));
#153973=CARTESIAN_POINT('Ctrl Pts',(-40.2545786542953,60.7780710967248,
0.));
#153974=CARTESIAN_POINT('Ctrl Pts',(-40.2545786542953,60.7780710967248,
12.));
#153975=CARTESIAN_POINT('Ctrl Pts',(-40.2493980896638,60.7530191439593,
0.));
#153976=CARTESIAN_POINT('Ctrl Pts',(-40.2493980896638,60.7530191439593,
12.));
#153977=CARTESIAN_POINT('Ctrl Pts',(-40.2442018113108,60.728010266139,0.));
#153978=CARTESIAN_POINT('Ctrl Pts',(-40.2442018113108,60.728010266139,12.));
#153979=CARTESIAN_POINT('Ctrl Pts',(-40.2389898925932,60.7030445528857,
0.));
#153980=CARTESIAN_POINT('Ctrl Pts',(-40.2389898925932,60.7030445528857,
12.));
#153981=CARTESIAN_POINT('Ctrl Pts',(-40.2337624072029,60.678122094098,0.));
#153982=CARTESIAN_POINT('Ctrl Pts',(-40.2337624072029,60.678122094098,12.));
#153983=CARTESIAN_POINT('Ctrl Pts',(-40.2285194291706,60.6532429799499,
0.));
#153984=CARTESIAN_POINT('Ctrl Pts',(-40.2285194291706,60.6532429799499,
12.));
#153985=CARTESIAN_POINT('Ctrl Pts',(-40.2232610328721,60.6284073008871,
0.));
#153986=CARTESIAN_POINT('Ctrl Pts',(-40.2232610328721,60.6284073008871,
12.));
#153987=CARTESIAN_POINT('Ctrl Pts',(-40.2179872930273,60.6036151476349,
0.));
#153988=CARTESIAN_POINT('Ctrl Pts',(-40.2179872930273,60.6036151476349,
12.));
#153989=CARTESIAN_POINT('Ctrl Pts',(-40.2126982847011,60.5788666112042,
0.));
#153990=CARTESIAN_POINT('Ctrl Pts',(-40.2126982847011,60.5788666112042,
12.));
#153991=CARTESIAN_POINT('Ctrl Pts',(-40.2073940833052,60.5541617828925,
0.));
#153992=CARTESIAN_POINT('Ctrl Pts',(-40.2073940833052,60.5541617828925,
12.));
#153993=CARTESIAN_POINT('Ctrl Pts',(-40.2020747646014,60.5295007542841,
0.));
#153994=CARTESIAN_POINT('Ctrl Pts',(-40.2020747646014,60.5295007542841,
12.));
#153995=CARTESIAN_POINT('Ctrl Pts',(-40.1967404047062,60.5048836172435,
0.));
#153996=CARTESIAN_POINT('Ctrl Pts',(-40.1967404047062,60.5048836172435,
12.));
#153997=CARTESIAN_POINT('Ctrl Pts',(-40.1913910800921,60.4803104639226,
0.));
#153998=CARTESIAN_POINT('Ctrl Pts',(-40.1913910800921,60.4803104639226,
12.));
#153999=CARTESIAN_POINT('Ctrl Pts',(-40.1860268675883,60.455781386769,0.));
#154000=CARTESIAN_POINT('Ctrl Pts',(-40.1860268675883,60.455781386769,12.));
#154001=CARTESIAN_POINT('Ctrl Pts',(-40.180647844383,60.4312964785273,0.));
#154002=CARTESIAN_POINT('Ctrl Pts',(-40.180647844383,60.4312964785273,12.));
#154003=CARTESIAN_POINT('Ctrl Pts',(-40.1752540880268,60.4068558322407,
0.));
#154004=CARTESIAN_POINT('Ctrl Pts',(-40.1752540880268,60.4068558322407,
12.));
#154005=CARTESIAN_POINT('Ctrl Pts',(-40.1698456764377,60.3824595412445,
0.));
#154006=CARTESIAN_POINT('Ctrl Pts',(-40.1698456764377,60.3824595412445,
12.));
#154007=CARTESIAN_POINT('Ctrl Pts',(-40.1644226879033,60.3581076991716,
0.));
#154008=CARTESIAN_POINT('Ctrl Pts',(-40.1644226879033,60.3581076991716,
12.));
#154009=CARTESIAN_POINT('Ctrl Pts',(-40.1589852010804,60.3338003999607,
0.));
#154010=CARTESIAN_POINT('Ctrl Pts',(-40.1589852010804,60.3338003999607,
12.));
#154011=CARTESIAN_POINT('Ctrl Pts',(-40.1535332949976,60.3095377378586,
0.));
#154012=CARTESIAN_POINT('Ctrl Pts',(-40.1535332949976,60.3095377378586,
12.));
#154013=CARTESIAN_POINT('Ctrl Pts',(-40.1480670490586,60.285319807422,0.));
#154014=CARTESIAN_POINT('Ctrl Pts',(-40.1480670490586,60.285319807422,12.));
#154015=CARTESIAN_POINT('Ctrl Pts',(-40.1425865430472,60.2611467035117,
0.));
#154016=CARTESIAN_POINT('Ctrl Pts',(-40.1425865430472,60.2611467035117,
12.));
#154017=CARTESIAN_POINT('Ctrl Pts',(-40.1370918571304,60.2370185212964,
0.));
#154018=CARTESIAN_POINT('Ctrl Pts',(-40.1370918571304,60.2370185212964,
12.));
#154019=CARTESIAN_POINT('Ctrl Pts',(-40.1315830718577,60.2129353562622,
0.));
#154020=CARTESIAN_POINT('Ctrl Pts',(-40.1315830718577,60.2129353562622,
12.));
#154021=CARTESIAN_POINT('Ctrl Pts',(-40.1260602681644,60.1888973042152,
0.));
#154022=CARTESIAN_POINT('Ctrl Pts',(-40.1260602681644,60.1888973042152,
12.));
#154023=CARTESIAN_POINT('Ctrl Pts',(-40.1205235273739,60.1649044612828,
0.));
#154024=CARTESIAN_POINT('Ctrl Pts',(-40.1205235273739,60.1649044612828,
12.));
#154025=CARTESIAN_POINT('Ctrl Pts',(-40.1149729312036,60.1409569239092,
0.));
#154026=CARTESIAN_POINT('Ctrl Pts',(-40.1149729312036,60.1409569239092,
12.));
#154027=CARTESIAN_POINT('Ctrl Pts',(-40.1094085617674,60.1170547888574,
0.));
#154028=CARTESIAN_POINT('Ctrl Pts',(-40.1094085617674,60.1170547888574,
12.));
#154029=CARTESIAN_POINT('Ctrl Pts',(-40.1038305015766,60.0931981532198,
0.));
#154030=CARTESIAN_POINT('Ctrl Pts',(-40.1038305015766,60.0931981532198,
12.));
#154031=CARTESIAN_POINT('Ctrl Pts',(-40.0982388335423,60.069387114421,0.));
#154032=CARTESIAN_POINT('Ctrl Pts',(-40.0982388335423,60.069387114421,12.));
#154033=CARTESIAN_POINT('Ctrl Pts',(-40.0926336409785,60.0456217702202,
0.));
#154034=CARTESIAN_POINT('Ctrl Pts',(-40.0926336409785,60.0456217702202,
12.));
#154035=CARTESIAN_POINT('Ctrl Pts',(-40.0870150076074,60.021902218706,0.));
#154036=CARTESIAN_POINT('Ctrl Pts',(-40.0870150076074,60.021902218706,12.));
#154037=CARTESIAN_POINT('Ctrl Pts',(-40.0813830175623,59.9982285582983,
0.));
#154038=CARTESIAN_POINT('Ctrl Pts',(-40.0813830175623,59.9982285582983,
12.));
#154039=CARTESIAN_POINT('Ctrl Pts',(-40.0757377553888,59.9746008877584,
0.));
#154040=CARTESIAN_POINT('Ctrl Pts',(-40.0757377553888,59.9746008877584,
12.));
#154041=CARTESIAN_POINT('Ctrl Pts',(-40.0700793060473,59.9510193061927,
0.));
#154042=CARTESIAN_POINT('Ctrl Pts',(-40.0700793060473,59.9510193061927,
12.));
#154043=CARTESIAN_POINT('Ctrl Pts',(-40.0644077549159,59.9274839130553,
0.));
#154044=CARTESIAN_POINT('Ctrl Pts',(-40.0644077549159,59.9274839130553,
12.));
#154045=CARTESIAN_POINT('Ctrl Pts',(-40.0587231877961,59.9039948081432,
0.));
#154046=CARTESIAN_POINT('Ctrl Pts',(-40.0587231877961,59.9039948081432,
12.));
#154047=CARTESIAN_POINT('Ctrl Pts',(-40.0530256909162,59.8805520915975,
0.));
#154048=CARTESIAN_POINT('Ctrl Pts',(-40.0530256909162,59.8805520915975,
12.));
#154049=CARTESIAN_POINT('Ctrl Pts',(-40.0473153509323,59.8571558639145,
0.));
#154050=CARTESIAN_POINT('Ctrl Pts',(-40.0473153509323,59.8571558639145,
12.));
#154051=CARTESIAN_POINT('Ctrl Pts',(-40.0415922549313,59.8338062259491,
0.));
#154052=CARTESIAN_POINT('Ctrl Pts',(-40.0415922549313,59.8338062259491,
12.));
#154053=CARTESIAN_POINT('Ctrl Pts',(-40.035856490434,59.8105032789179,0.));
#154054=CARTESIAN_POINT('Ctrl Pts',(-40.035856490434,59.8105032789179,12.));
#154055=CARTESIAN_POINT('Ctrl Pts',(-40.0301081454006,59.7872471243948,
0.));
#154056=CARTESIAN_POINT('Ctrl Pts',(-40.0301081454006,59.7872471243948,
12.));
#154057=CARTESIAN_POINT('Ctrl Pts',(-40.0243473082343,59.7640378643115,
0.));
#154058=CARTESIAN_POINT('Ctrl Pts',(-40.0243473082343,59.7640378643115,
12.));
#154059=CARTESIAN_POINT('Ctrl Pts',(-40.0185740677827,59.7408756009688,
0.));
#154060=CARTESIAN_POINT('Ctrl Pts',(-40.0185740677827,59.7408756009688,
12.));
#154061=CARTESIAN_POINT('Ctrl Pts',(-40.0127885133407,59.7177604370409,
0.));
#154062=CARTESIAN_POINT('Ctrl Pts',(-40.0127885133407,59.7177604370409,
12.));
#154063=CARTESIAN_POINT('Ctrl Pts',(-40.0069907346536,59.6946924755771,
0.));
#154064=CARTESIAN_POINT('Ctrl Pts',(-40.0069907346536,59.6946924755771,
12.));
#154065=CARTESIAN_POINT('Ctrl Pts',(-40.001180821923,59.671671819999,0.));
#154066=CARTESIAN_POINT('Ctrl Pts',(-40.001180821923,59.671671819999,12.));
#154067=CARTESIAN_POINT('Ctrl Pts',(-39.9953588658114,59.6486985741015,
0.));
#154068=CARTESIAN_POINT('Ctrl Pts',(-39.9953588658114,59.6486985741015,
12.));
#154069=CARTESIAN_POINT('Ctrl Pts',(-39.9895249574432,59.6257728420644,
0.));
#154070=CARTESIAN_POINT('Ctrl Pts',(-39.9895249574432,59.6257728420644,
12.));
#154071=CARTESIAN_POINT('Ctrl Pts',(-39.9836791884071,59.6028947284551,
0.));
#154072=CARTESIAN_POINT('Ctrl Pts',(-39.9836791884071,59.6028947284551,
12.));
#154073=CARTESIAN_POINT('Ctrl Pts',(-39.9778216507609,59.5800643382322,
0.));
#154074=CARTESIAN_POINT('Ctrl Pts',(-39.9778216507609,59.5800643382322,
12.));
#154075=CARTESIAN_POINT('Ctrl Pts',(-39.971952437036,59.5572817767412,0.));
#154076=CARTESIAN_POINT('Ctrl Pts',(-39.971952437036,59.5572817767412,12.));
#154077=CARTESIAN_POINT('Ctrl Pts',(-39.9660716402423,59.5345471497162,
0.));
#154078=CARTESIAN_POINT('Ctrl Pts',(-39.9660716402423,59.5345471497162,
12.));
#154079=CARTESIAN_POINT('Ctrl Pts',(-39.96017935387,59.511860563292,0.));
#154080=CARTESIAN_POINT('Ctrl Pts',(-39.96017935387,59.511860563292,12.));
#154081=CARTESIAN_POINT('Ctrl Pts',(-39.954275671893,59.4892221240081,0.));
#154082=CARTESIAN_POINT('Ctrl Pts',(-39.954275671893,59.4892221240081,12.));
#154083=CARTESIAN_POINT('Ctrl Pts',(-39.9483606887731,59.4666319388123,
0.));
#154084=CARTESIAN_POINT('Ctrl Pts',(-39.9483606887731,59.4666319388123,
12.));
#154085=CARTESIAN_POINT('Ctrl Pts',(-39.9424344994652,59.444090115055,0.));
#154086=CARTESIAN_POINT('Ctrl Pts',(-39.9424344994652,59.444090115055,12.));
#154087=CARTESIAN_POINT('Ctrl Pts',(-39.9364971994215,59.4215967604925,
0.));
#154088=CARTESIAN_POINT('Ctrl Pts',(-39.9364971994215,59.4215967604925,
12.));
#154089=CARTESIAN_POINT('Ctrl Pts',(-39.9305488845934,59.3991519832981,
0.));
#154090=CARTESIAN_POINT('Ctrl Pts',(-39.9305488845934,59.3991519832981,
12.));
#154091=CARTESIAN_POINT('Ctrl Pts',(-39.9245896514359,59.3767558920663,
0.));
#154092=CARTESIAN_POINT('Ctrl Pts',(-39.9245896514359,59.3767558920663,
12.));
#154093=CARTESIAN_POINT('Ctrl Pts',(-39.9186195969113,59.3544085958165,
0.));
#154094=CARTESIAN_POINT('Ctrl Pts',(-39.9186195969113,59.3544085958165,
12.));
#154095=CARTESIAN_POINT('Ctrl Pts',(-39.9126388184956,59.3321102039883,
0.));
#154096=CARTESIAN_POINT('Ctrl Pts',(-39.9126388184956,59.3321102039883,
12.));
#154097=CARTESIAN_POINT('Ctrl Pts',(-39.9066474141826,59.3098608264452,
0.));
#154098=CARTESIAN_POINT('Ctrl Pts',(-39.9066474141826,59.3098608264452,
12.));
#154099=CARTESIAN_POINT('Ctrl Pts',(-39.9006454824861,59.2876605734871,
0.));
#154100=CARTESIAN_POINT('Ctrl Pts',(-39.9006454824861,59.2876605734871,
12.));
#154101=CARTESIAN_POINT('Ctrl Pts',(-39.8946331224442,59.2655095558527,
0.));
#154102=CARTESIAN_POINT('Ctrl Pts',(-39.8946331224442,59.2655095558527,
12.));
#154103=CARTESIAN_POINT('Ctrl Pts',(-39.8886104336234,59.2434078847236,
0.));
#154104=CARTESIAN_POINT('Ctrl Pts',(-39.8886104336234,59.2434078847236,
12.));
#154105=CARTESIAN_POINT('Ctrl Pts',(-39.8825775161252,59.2213556717189,
0.));
#154106=CARTESIAN_POINT('Ctrl Pts',(-39.8825775161252,59.2213556717189,
12.));
#154107=CARTESIAN_POINT('Ctrl Pts',(-39.8765344705894,59.1993530289008,
0.));
#154108=CARTESIAN_POINT('Ctrl Pts',(-39.8765344705894,59.1993530289008,
12.));
#154109=CARTESIAN_POINT('Ctrl Pts',(-39.8704813981978,59.1774000687865,
0.));
#154110=CARTESIAN_POINT('Ctrl Pts',(-39.8704813981978,59.1774000687865,
12.));
#154111=CARTESIAN_POINT('Ctrl Pts',(-39.8644184006785,59.155496904352,0.));
#154112=CARTESIAN_POINT('Ctrl Pts',(-39.8644184006785,59.155496904352,12.));
#154113=CARTESIAN_POINT('Ctrl Pts',(-39.8583455803111,59.133643649035,0.));
#154114=CARTESIAN_POINT('Ctrl Pts',(-39.8583455803111,59.133643649035,12.));
#154115=CARTESIAN_POINT('Ctrl Pts',(-39.8522630399337,59.1118404167304,
0.));
#154116=CARTESIAN_POINT('Ctrl Pts',(-39.8522630399337,59.1118404167304,
12.));
#154117=CARTESIAN_POINT('Ctrl Pts',(-39.8461708829465,59.0900873217992,
0.));
#154118=CARTESIAN_POINT('Ctrl Pts',(-39.8461708829465,59.0900873217992,
12.));
#154119=CARTESIAN_POINT('Ctrl Pts',(-39.8400692133143,59.068384479077,0.));
#154120=CARTESIAN_POINT('Ctrl Pts',(-39.8400692133143,59.068384479077,12.));
#154121=CARTESIAN_POINT('Ctrl Pts',(-39.8339581355714,59.0467320038782,
0.));
#154122=CARTESIAN_POINT('Ctrl Pts',(-39.8339581355714,59.0467320038782,
12.));
#154123=CARTESIAN_POINT('Ctrl Pts',(-39.8278377548261,59.0251300119973,
0.));
#154124=CARTESIAN_POINT('Ctrl Pts',(-39.8278377548261,59.0251300119973,
12.));
#154125=CARTESIAN_POINT('Ctrl Pts',(-39.8217081767658,59.0035786197024,
0.));
#154126=CARTESIAN_POINT('Ctrl Pts',(-39.8217081767658,59.0035786197024,
12.));
#154127=CARTESIAN_POINT('Ctrl Pts',(-39.8155695076625,58.9820779437485,
0.));
#154128=CARTESIAN_POINT('Ctrl Pts',(-39.8155695076625,58.9820779437485,
12.));
#154129=CARTESIAN_POINT('Ctrl Pts',(-39.8094218543781,58.9606281013876,
0.));
#154130=CARTESIAN_POINT('Ctrl Pts',(-39.8094218543781,58.9606281013876,
12.));
#154131=CARTESIAN_POINT('Ctrl Pts',(-39.8032653243712,58.9392292103747,
0.));
#154132=CARTESIAN_POINT('Ctrl Pts',(-39.8032653243712,58.9392292103747,
12.));
#154133=CARTESIAN_POINT('Ctrl Pts',(-39.7971000257044,58.9178813889703,
0.));
#154134=CARTESIAN_POINT('Ctrl Pts',(-39.7971000257044,58.9178813889703,
12.));
#154135=CARTESIAN_POINT('Ctrl Pts',(-39.7909260670517,58.896584755939,0.));
#154136=CARTESIAN_POINT('Ctrl Pts',(-39.7909260670517,58.896584755939,12.));
#154137=CARTESIAN_POINT('Ctrl Pts',(-39.7847435576995,58.8753394305583,
0.));
#154138=CARTESIAN_POINT('Ctrl Pts',(-39.7847435576995,58.8753394305583,
12.));
#154139=CARTESIAN_POINT('Ctrl Pts',(-39.7785526075477,58.8541455326229,
0.));
#154140=CARTESIAN_POINT('Ctrl Pts',(-39.7785526075477,58.8541455326229,
12.));
#154141=CARTESIAN_POINT('Ctrl Pts',(-39.772353327112,58.8330031824453,0.));
#154142=CARTESIAN_POINT('Ctrl Pts',(-39.772353327112,58.8330031824453,12.));
#154143=CARTESIAN_POINT('Ctrl Pts',(-39.7661458275276,58.8119125008521,
0.));
#154144=CARTESIAN_POINT('Ctrl Pts',(-39.7661458275276,58.8119125008521,
12.));
#154145=CARTESIAN_POINT('Ctrl Pts',(-39.7599302205527,58.7908736091808,
0.));
#154146=CARTESIAN_POINT('Ctrl Pts',(-39.7599302205527,58.7908736091808,
12.));
#154147=CARTESIAN_POINT('Ctrl Pts',(-39.753706618582,58.7698866293041,0.));
#154148=CARTESIAN_POINT('Ctrl Pts',(-39.753706618582,58.7698866293041,12.));
#154149=CARTESIAN_POINT('Ctrl Pts',(-39.7474751346603,58.7489516836453,
0.));
#154150=CARTESIAN_POINT('Ctrl Pts',(-39.7474751346603,58.7489516836453,
12.));
#154151=CARTESIAN_POINT('Ctrl Pts',(-39.7412358824949,58.7280688951911,
0.));
#154152=CARTESIAN_POINT('Ctrl Pts',(-39.7412358824949,58.7280688951911,
12.));
#154153=CARTESIAN_POINT('Ctrl Pts',(-39.7349889764737,58.7072383875009,
0.));
#154154=CARTESIAN_POINT('Ctrl Pts',(-39.7349889764737,58.7072383875009,
12.));
#154155=CARTESIAN_POINT('Ctrl Pts',(-39.7287345316664,58.6864602847064,
0.));
#154156=CARTESIAN_POINT('Ctrl Pts',(-39.7287345316664,58.6864602847064,
12.));
#154157=CARTESIAN_POINT('Ctrl Pts',(-39.7224726638087,58.6657347115014,
0.));
#154158=CARTESIAN_POINT('Ctrl Pts',(-39.7224726638087,58.6657347115014,
12.));
#154159=CARTESIAN_POINT('Ctrl Pts',(-39.7162034892896,58.6450617931269,
0.));
#154160=CARTESIAN_POINT('Ctrl Pts',(-39.7162034892896,58.6450617931269,
12.));
#154161=CARTESIAN_POINT('Ctrl Pts',(-39.7099271251421,58.6244416553574,
0.));
#154162=CARTESIAN_POINT('Ctrl Pts',(-39.7099271251421,58.6244416553574,
12.));
#154163=CARTESIAN_POINT('Ctrl Pts',(-39.7036436890248,58.6038744244683,
0.));
#154164=CARTESIAN_POINT('Ctrl Pts',(-39.7036436890248,58.6038744244683,
12.));
#154165=CARTESIAN_POINT('Ctrl Pts',(-39.6973532992555,58.5833602272767,
0.));
#154166=CARTESIAN_POINT('Ctrl Pts',(-39.6973532992555,58.5833602272767,
12.));
#154167=CARTESIAN_POINT('Ctrl Pts',(-39.6910560748639,58.5628991912067,
0.));
#154168=CARTESIAN_POINT('Ctrl Pts',(-39.6910560748639,58.5628991912067,
12.));
#154169=CARTESIAN_POINT('Ctrl Pts',(-39.6847521356395,58.5424914443415,
0.));
#154170=CARTESIAN_POINT('Ctrl Pts',(-39.6847521356395,58.5424914443415,
12.));
#154171=CARTESIAN_POINT('Ctrl Pts',(-39.6784416021817,58.5221371154748,
0.));
#154172=CARTESIAN_POINT('Ctrl Pts',(-39.6784416021817,58.5221371154748,
12.));
#154173=CARTESIAN_POINT('Ctrl Pts',(-39.6721245959516,58.5018363341582,
0.));
#154174=CARTESIAN_POINT('Ctrl Pts',(-39.6721245959516,58.5018363341582,
12.));
#154175=CARTESIAN_POINT('Ctrl Pts',(-39.66580123918,58.4815892306044,0.));
#154176=CARTESIAN_POINT('Ctrl Pts',(-39.66580123918,58.4815892306044,12.));
#154177=CARTESIAN_POINT('Ctrl Pts',(-39.659471654768,58.4613959355776,0.));
#154178=CARTESIAN_POINT('Ctrl Pts',(-39.659471654768,58.4613959355776,12.));
#154179=CARTESIAN_POINT('Ctrl Pts',(-39.6531359662043,58.4412565802984,
0.));
#154180=CARTESIAN_POINT('Ctrl Pts',(-39.6531359662043,58.4412565802984,
12.));
#154181=CARTESIAN_POINT('Ctrl Pts',(-39.6467942974464,58.4211712963024,
0.));
#154182=CARTESIAN_POINT('Ctrl Pts',(-39.6467942974464,58.4211712963024,
12.));
#154183=CARTESIAN_POINT('Ctrl Pts',(-39.6404467729113,58.4011402154225,
0.));
#154184=CARTESIAN_POINT('Ctrl Pts',(-39.6404467729113,58.4011402154225,
12.));
#154185=CARTESIAN_POINT('Ctrl Pts',(-39.6340935177492,58.3811634701061,
0.));
#154186=CARTESIAN_POINT('Ctrl Pts',(-39.6340935177492,58.3811634701061,
12.));
#154187=CARTESIAN_POINT('Ctrl Pts',(-39.6277346580898,58.3612411936914,
0.));
#154188=CARTESIAN_POINT('Ctrl Pts',(-39.6277346580898,58.3612411936914,
12.));
#154189=CARTESIAN_POINT('Ctrl Pts',(-39.6213703212523,58.3413735206412,
0.));
#154190=CARTESIAN_POINT('Ctrl Pts',(-39.6213703212523,58.3413735206412,
12.));
#154191=CARTESIAN_POINT('Ctrl Pts',(-39.6150006360894,58.3215605869192,
0.));
#154192=CARTESIAN_POINT('Ctrl Pts',(-39.6150006360894,58.3215605869192,
12.));
#154193=CARTESIAN_POINT('Ctrl Pts',(-39.6086257327559,58.3018025297288,
0.));
#154194=CARTESIAN_POINT('Ctrl Pts',(-39.6086257327559,58.3018025297288,
12.));
#154195=CARTESIAN_POINT('Ctrl Pts',(-39.6022457420772,58.2820994868092,
0.));
#154196=CARTESIAN_POINT('Ctrl Pts',(-39.6022457420772,58.2820994868092,
12.));
#154197=CARTESIAN_POINT('Ctrl Pts',(-39.5958607950237,58.2624515958416,
0.));
#154198=CARTESIAN_POINT('Ctrl Pts',(-39.5958607950237,58.2624515958416,
12.));
#154199=CARTESIAN_POINT('Ctrl Pts',(-39.5894710221729,58.2428589938394,
0.));
#154200=CARTESIAN_POINT('Ctrl Pts',(-39.5894710221729,58.2428589938394,
12.));
#154201=CARTESIAN_POINT('Ctrl Pts',(-39.5830765530919,58.2233218164407,
0.));
#154202=CARTESIAN_POINT('Ctrl Pts',(-39.5830765530919,58.2233218164407,
12.));
#154203=CARTESIAN_POINT('Ctrl Pts',(-39.5766775175226,58.2038401992496,
0.));
#154204=CARTESIAN_POINT('Ctrl Pts',(-39.5766775175226,58.2038401992496,
12.));
#154205=CARTESIAN_POINT('Ctrl Pts',(-39.5702740468013,58.1844142794359,
0.));
#154206=CARTESIAN_POINT('Ctrl Pts',(-39.5702740468013,58.1844142794359,
12.));
#154207=CARTESIAN_POINT('Ctrl Pts',(-39.5638662750174,58.1650441970379,
0.));
#154208=CARTESIAN_POINT('Ctrl Pts',(-39.5638662750174,58.1650441970379,
12.));
#154209=CARTESIAN_POINT('Ctrl Pts',(-39.5574543406959,58.1457300968467,
0.));
#154210=CARTESIAN_POINT('Ctrl Pts',(-39.5574543406959,58.1457300968467,
12.));
#154211=CARTESIAN_POINT('Ctrl Pts',(-39.5510383869476,58.1264721285698,
0.));
#154212=CARTESIAN_POINT('Ctrl Pts',(-39.5510383869476,58.1264721285698,
12.));
#154213=CARTESIAN_POINT('Ctrl Pts',(-39.5446185579615,58.1072704428895,
0.));
#154214=CARTESIAN_POINT('Ctrl Pts',(-39.5446185579615,58.1072704428895,
12.));
#154215=CARTESIAN_POINT('Ctrl Pts',(-39.5381949959214,58.088125187991,0.));
#154216=CARTESIAN_POINT('Ctrl Pts',(-39.5381949959214,58.088125187991,12.));
#154217=CARTESIAN_POINT('Ctrl Pts',(-39.5317678383231,58.0690365065393,
0.));
#154218=CARTESIAN_POINT('Ctrl Pts',(-39.5317678383231,58.0690365065393,
12.));
#154219=CARTESIAN_POINT('Ctrl Pts',(-39.5253372136921,58.050004530846,0.));
#154220=CARTESIAN_POINT('Ctrl Pts',(-39.5253372136921,58.050004530846,12.));
#154221=CARTESIAN_POINT('Ctrl Pts',(-39.5189032457227,58.0310293875321,
0.));
#154222=CARTESIAN_POINT('Ctrl Pts',(-39.5189032457227,58.0310293875321,
12.));
#154223=CARTESIAN_POINT('Ctrl Pts',(-39.5124660615009,58.012111206794,0.));
#154224=CARTESIAN_POINT('Ctrl Pts',(-39.5124660615009,58.012111206794,12.));
#154225=CARTESIAN_POINT('Ctrl Pts',(-39.5060257981225,57.9932501298522,
0.));
#154226=CARTESIAN_POINT('Ctrl Pts',(-39.5060257981225,57.9932501298522,
12.));
#154227=CARTESIAN_POINT('Ctrl Pts',(-39.4995826106691,57.9744463179305,
0.));
#154228=CARTESIAN_POINT('Ctrl Pts',(-39.4995826106691,57.9744463179305,
12.));
#154229=CARTESIAN_POINT('Ctrl Pts',(-39.4931366776627,57.9556999583777,
0.));
#154230=CARTESIAN_POINT('Ctrl Pts',(-39.4931366776627,57.9556999583777,
12.));
#154231=CARTESIAN_POINT('Ctrl Pts',(-39.4866881842223,57.9370112456506,
0.));
#154232=CARTESIAN_POINT('Ctrl Pts',(-39.4866881842223,57.9370112456506,
12.));
#154233=CARTESIAN_POINT('Ctrl Pts',(-39.4802373061008,57.9183803632337,
0.));
#154234=CARTESIAN_POINT('Ctrl Pts',(-39.4802373061008,57.9183803632337,
12.));
#154235=CARTESIAN_POINT('Ctrl Pts',(-39.4737841949417,57.8998074670541,
0.));
#154236=CARTESIAN_POINT('Ctrl Pts',(-39.4737841949417,57.8998074670541,
12.));
#154237=CARTESIAN_POINT('Ctrl Pts',(-39.4673289592425,57.8812926637397,
0.));
#154238=CARTESIAN_POINT('Ctrl Pts',(-39.4673289592425,57.8812926637397,
12.));
#154239=CARTESIAN_POINT('Ctrl Pts',(-39.4608716627367,57.8628360097134,
0.));
#154240=CARTESIAN_POINT('Ctrl Pts',(-39.4608716627367,57.8628360097134,
12.));
#154241=CARTESIAN_POINT('Ctrl Pts',(-39.4557042029884,57.8481172247805,
0.));
#154242=CARTESIAN_POINT('Ctrl Pts',(-39.4557042029884,57.8481172247805,
12.));
#154243=CARTESIAN_POINT('Ctrl Pts',(-39.45182770037,57.8371043151607,0.));
#154244=CARTESIAN_POINT('Ctrl Pts',(-39.45182770037,57.8371043151607,12.));
#154245=CARTESIAN_POINT('Ctrl Pts',(-39.4492429618498,57.829774010102,0.));
#154246=CARTESIAN_POINT('Ctrl Pts',(-39.4492429618498,57.829774010102,12.));
#154247=CARTESIAN_POINT('Ctrl Pts',(-39.4479504917286,57.8261117662439,
0.));
#154248=CARTESIAN_POINT('Ctrl Pts',(-39.4479504917286,57.8261117662439,
12.));
#154249=CARTESIAN_POINT('',(-39.4479504917286,57.8261117662439,12.));
#154250=CARTESIAN_POINT('Ctrl Pts',(-39.4479504917286,57.8261117662439,
12.));
#154251=CARTESIAN_POINT('Ctrl Pts',(-39.4492429618498,57.829774010102,12.));
#154252=CARTESIAN_POINT('Ctrl Pts',(-39.45182770037,57.8371043151607,12.));
#154253=CARTESIAN_POINT('Ctrl Pts',(-39.4557042029884,57.8481172247805,
12.));
#154254=CARTESIAN_POINT('Ctrl Pts',(-39.4608716627367,57.8628360097134,
12.));
#154255=CARTESIAN_POINT('Ctrl Pts',(-39.4673289592425,57.8812926637397,
12.));
#154256=CARTESIAN_POINT('Ctrl Pts',(-39.4737841949417,57.8998074670541,
12.));
#154257=CARTESIAN_POINT('Ctrl Pts',(-39.4802373061008,57.9183803632337,
12.));
#154258=CARTESIAN_POINT('Ctrl Pts',(-39.4866881842223,57.9370112456506,
12.));
#154259=CARTESIAN_POINT('Ctrl Pts',(-39.4931366776627,57.9556999583777,
12.));
#154260=CARTESIAN_POINT('Ctrl Pts',(-39.4995826106691,57.9744463179305,
12.));
#154261=CARTESIAN_POINT('Ctrl Pts',(-39.5060257981225,57.9932501298522,
12.));
#154262=CARTESIAN_POINT('Ctrl Pts',(-39.5124660615009,58.012111206794,12.));
#154263=CARTESIAN_POINT('Ctrl Pts',(-39.5189032457227,58.0310293875321,
12.));
#154264=CARTESIAN_POINT('Ctrl Pts',(-39.5253372136921,58.050004530846,12.));
#154265=CARTESIAN_POINT('Ctrl Pts',(-39.5317678383231,58.0690365065393,
12.));
#154266=CARTESIAN_POINT('Ctrl Pts',(-39.5381949959214,58.088125187991,12.));
#154267=CARTESIAN_POINT('Ctrl Pts',(-39.5446185579615,58.1072704428895,
12.));
#154268=CARTESIAN_POINT('Ctrl Pts',(-39.5510383869476,58.1264721285698,
12.));
#154269=CARTESIAN_POINT('Ctrl Pts',(-39.5574543406959,58.1457300968467,
12.));
#154270=CARTESIAN_POINT('Ctrl Pts',(-39.5638662750174,58.1650441970379,
12.));
#154271=CARTESIAN_POINT('Ctrl Pts',(-39.5702740468013,58.1844142794359,
12.));
#154272=CARTESIAN_POINT('Ctrl Pts',(-39.5766775175226,58.2038401992496,
12.));
#154273=CARTESIAN_POINT('Ctrl Pts',(-39.5830765530919,58.2233218164407,
12.));
#154274=CARTESIAN_POINT('Ctrl Pts',(-39.5894710221729,58.2428589938394,
12.));
#154275=CARTESIAN_POINT('Ctrl Pts',(-39.5958607950237,58.2624515958416,
12.));
#154276=CARTESIAN_POINT('Ctrl Pts',(-39.6022457420772,58.2820994868092,
12.));
#154277=CARTESIAN_POINT('Ctrl Pts',(-39.6086257327559,58.3018025297288,
12.));
#154278=CARTESIAN_POINT('Ctrl Pts',(-39.6150006360894,58.3215605869192,
12.));
#154279=CARTESIAN_POINT('Ctrl Pts',(-39.6213703212523,58.3413735206412,
12.));
#154280=CARTESIAN_POINT('Ctrl Pts',(-39.6277346580898,58.3612411936914,
12.));
#154281=CARTESIAN_POINT('Ctrl Pts',(-39.6340935177492,58.3811634701061,
12.));
#154282=CARTESIAN_POINT('Ctrl Pts',(-39.6404467729113,58.4011402154225,
12.));
#154283=CARTESIAN_POINT('Ctrl Pts',(-39.6467942974464,58.4211712963024,
12.));
#154284=CARTESIAN_POINT('Ctrl Pts',(-39.6531359662043,58.4412565802984,
12.));
#154285=CARTESIAN_POINT('Ctrl Pts',(-39.659471654768,58.4613959355776,12.));
#154286=CARTESIAN_POINT('Ctrl Pts',(-39.66580123918,58.4815892306044,12.));
#154287=CARTESIAN_POINT('Ctrl Pts',(-39.6721245959516,58.5018363341582,
12.));
#154288=CARTESIAN_POINT('Ctrl Pts',(-39.6784416021817,58.5221371154748,
12.));
#154289=CARTESIAN_POINT('Ctrl Pts',(-39.6847521356395,58.5424914443415,
12.));
#154290=CARTESIAN_POINT('Ctrl Pts',(-39.6910560748639,58.5628991912067,
12.));
#154291=CARTESIAN_POINT('Ctrl Pts',(-39.6973532992555,58.5833602272767,
12.));
#154292=CARTESIAN_POINT('Ctrl Pts',(-39.7036436890248,58.6038744244683,
12.));
#154293=CARTESIAN_POINT('Ctrl Pts',(-39.7099271251421,58.6244416553574,
12.));
#154294=CARTESIAN_POINT('Ctrl Pts',(-39.7162034892896,58.6450617931269,
12.));
#154295=CARTESIAN_POINT('Ctrl Pts',(-39.7224726638087,58.6657347115014,
12.));
#154296=CARTESIAN_POINT('Ctrl Pts',(-39.7287345316664,58.6864602847064,
12.));
#154297=CARTESIAN_POINT('Ctrl Pts',(-39.7349889764737,58.7072383875009,
12.));
#154298=CARTESIAN_POINT('Ctrl Pts',(-39.7412358824949,58.7280688951911,
12.));
#154299=CARTESIAN_POINT('Ctrl Pts',(-39.7474751346603,58.7489516836453,
12.));
#154300=CARTESIAN_POINT('Ctrl Pts',(-39.753706618582,58.7698866293041,12.));
#154301=CARTESIAN_POINT('Ctrl Pts',(-39.7599302205527,58.7908736091808,
12.));
#154302=CARTESIAN_POINT('Ctrl Pts',(-39.7661458275276,58.8119125008521,
12.));
#154303=CARTESIAN_POINT('Ctrl Pts',(-39.772353327112,58.8330031824453,12.));
#154304=CARTESIAN_POINT('Ctrl Pts',(-39.7785526075477,58.8541455326229,
12.));
#154305=CARTESIAN_POINT('Ctrl Pts',(-39.7847435576995,58.8753394305583,
12.));
#154306=CARTESIAN_POINT('Ctrl Pts',(-39.7909260670517,58.896584755939,12.));
#154307=CARTESIAN_POINT('Ctrl Pts',(-39.7971000257044,58.9178813889703,
12.));
#154308=CARTESIAN_POINT('Ctrl Pts',(-39.8032653243712,58.9392292103747,
12.));
#154309=CARTESIAN_POINT('Ctrl Pts',(-39.8094218543781,58.9606281013876,
12.));
#154310=CARTESIAN_POINT('Ctrl Pts',(-39.8155695076625,58.9820779437485,
12.));
#154311=CARTESIAN_POINT('Ctrl Pts',(-39.8217081767658,59.0035786197024,
12.));
#154312=CARTESIAN_POINT('Ctrl Pts',(-39.8278377548261,59.0251300119973,
12.));
#154313=CARTESIAN_POINT('Ctrl Pts',(-39.8339581355714,59.0467320038782,
12.));
#154314=CARTESIAN_POINT('Ctrl Pts',(-39.8400692133143,59.068384479077,12.));
#154315=CARTESIAN_POINT('Ctrl Pts',(-39.8461708829465,59.0900873217992,
12.));
#154316=CARTESIAN_POINT('Ctrl Pts',(-39.8522630399337,59.1118404167304,
12.));
#154317=CARTESIAN_POINT('Ctrl Pts',(-39.8583455803111,59.133643649035,12.));
#154318=CARTESIAN_POINT('Ctrl Pts',(-39.8644184006785,59.155496904352,12.));
#154319=CARTESIAN_POINT('Ctrl Pts',(-39.8704813981978,59.1774000687865,
12.));
#154320=CARTESIAN_POINT('Ctrl Pts',(-39.8765344705894,59.1993530289008,
12.));
#154321=CARTESIAN_POINT('Ctrl Pts',(-39.8825775161252,59.2213556717189,
12.));
#154322=CARTESIAN_POINT('Ctrl Pts',(-39.8886104336234,59.2434078847236,
12.));
#154323=CARTESIAN_POINT('Ctrl Pts',(-39.8946331224442,59.2655095558527,
12.));
#154324=CARTESIAN_POINT('Ctrl Pts',(-39.9006454824861,59.2876605734871,
12.));
#154325=CARTESIAN_POINT('Ctrl Pts',(-39.9066474141826,59.3098608264452,
12.));
#154326=CARTESIAN_POINT('Ctrl Pts',(-39.9126388184956,59.3321102039883,
12.));
#154327=CARTESIAN_POINT('Ctrl Pts',(-39.9186195969113,59.3544085958165,
12.));
#154328=CARTESIAN_POINT('Ctrl Pts',(-39.9245896514359,59.3767558920663,
12.));
#154329=CARTESIAN_POINT('Ctrl Pts',(-39.9305488845934,59.3991519832981,
12.));
#154330=CARTESIAN_POINT('Ctrl Pts',(-39.9364971994215,59.4215967604925,
12.));
#154331=CARTESIAN_POINT('Ctrl Pts',(-39.9424344994652,59.444090115055,12.));
#154332=CARTESIAN_POINT('Ctrl Pts',(-39.9483606887731,59.4666319388123,
12.));
#154333=CARTESIAN_POINT('Ctrl Pts',(-39.954275671893,59.4892221240081,12.));
#154334=CARTESIAN_POINT('Ctrl Pts',(-39.96017935387,59.511860563292,12.));
#154335=CARTESIAN_POINT('Ctrl Pts',(-39.9660716402423,59.5345471497162,
12.));
#154336=CARTESIAN_POINT('Ctrl Pts',(-39.971952437036,59.5572817767412,12.));
#154337=CARTESIAN_POINT('Ctrl Pts',(-39.9778216507609,59.5800643382322,
12.));
#154338=CARTESIAN_POINT('Ctrl Pts',(-39.9836791884071,59.6028947284551,
12.));
#154339=CARTESIAN_POINT('Ctrl Pts',(-39.9895249574432,59.6257728420644,
12.));
#154340=CARTESIAN_POINT('Ctrl Pts',(-39.9953588658114,59.6486985741015,
12.));
#154341=CARTESIAN_POINT('Ctrl Pts',(-40.001180821923,59.671671819999,12.));
#154342=CARTESIAN_POINT('Ctrl Pts',(-40.0069907346536,59.6946924755771,
12.));
#154343=CARTESIAN_POINT('Ctrl Pts',(-40.0127885133407,59.7177604370409,
12.));
#154344=CARTESIAN_POINT('Ctrl Pts',(-40.0185740677827,59.7408756009688,
12.));
#154345=CARTESIAN_POINT('Ctrl Pts',(-40.0243473082343,59.7640378643115,
12.));
#154346=CARTESIAN_POINT('Ctrl Pts',(-40.0301081454006,59.7872471243948,
12.));
#154347=CARTESIAN_POINT('Ctrl Pts',(-40.035856490434,59.8105032789179,12.));
#154348=CARTESIAN_POINT('Ctrl Pts',(-40.0415922549313,59.8338062259491,
12.));
#154349=CARTESIAN_POINT('Ctrl Pts',(-40.0473153509323,59.8571558639145,
12.));
#154350=CARTESIAN_POINT('Ctrl Pts',(-40.0530256909162,59.8805520915975,
12.));
#154351=CARTESIAN_POINT('Ctrl Pts',(-40.0587231877961,59.9039948081432,
12.));
#154352=CARTESIAN_POINT('Ctrl Pts',(-40.0644077549159,59.9274839130553,
12.));
#154353=CARTESIAN_POINT('Ctrl Pts',(-40.0700793060473,59.9510193061927,
12.));
#154354=CARTESIAN_POINT('Ctrl Pts',(-40.0757377553888,59.9746008877584,
12.));
#154355=CARTESIAN_POINT('Ctrl Pts',(-40.0813830175623,59.9982285582983,
12.));
#154356=CARTESIAN_POINT('Ctrl Pts',(-40.0870150076074,60.021902218706,12.));
#154357=CARTESIAN_POINT('Ctrl Pts',(-40.0926336409785,60.0456217702202,
12.));
#154358=CARTESIAN_POINT('Ctrl Pts',(-40.0982388335423,60.069387114421,12.));
#154359=CARTESIAN_POINT('Ctrl Pts',(-40.1038305015766,60.0931981532198,
12.));
#154360=CARTESIAN_POINT('Ctrl Pts',(-40.1094085617674,60.1170547888574,
12.));
#154361=CARTESIAN_POINT('Ctrl Pts',(-40.1149729312036,60.1409569239092,
12.));
#154362=CARTESIAN_POINT('Ctrl Pts',(-40.1205235273739,60.1649044612828,
12.));
#154363=CARTESIAN_POINT('Ctrl Pts',(-40.1260602681644,60.1888973042152,
12.));
#154364=CARTESIAN_POINT('Ctrl Pts',(-40.1315830718577,60.2129353562622,
12.));
#154365=CARTESIAN_POINT('Ctrl Pts',(-40.1370918571304,60.2370185212964,
12.));
#154366=CARTESIAN_POINT('Ctrl Pts',(-40.1425865430472,60.2611467035117,
12.));
#154367=CARTESIAN_POINT('Ctrl Pts',(-40.1480670490586,60.285319807422,12.));
#154368=CARTESIAN_POINT('Ctrl Pts',(-40.1535332949976,60.3095377378586,
12.));
#154369=CARTESIAN_POINT('Ctrl Pts',(-40.1589852010804,60.3338003999607,
12.));
#154370=CARTESIAN_POINT('Ctrl Pts',(-40.1644226879033,60.3581076991716,
12.));
#154371=CARTESIAN_POINT('Ctrl Pts',(-40.1698456764377,60.3824595412445,
12.));
#154372=CARTESIAN_POINT('Ctrl Pts',(-40.1752540880268,60.4068558322407,
12.));
#154373=CARTESIAN_POINT('Ctrl Pts',(-40.180647844383,60.4312964785273,12.));
#154374=CARTESIAN_POINT('Ctrl Pts',(-40.1860268675883,60.455781386769,12.));
#154375=CARTESIAN_POINT('Ctrl Pts',(-40.1913910800921,60.4803104639226,
12.));
#154376=CARTESIAN_POINT('Ctrl Pts',(-40.1967404047062,60.5048836172435,
12.));
#154377=CARTESIAN_POINT('Ctrl Pts',(-40.2020747646014,60.5295007542841,
12.));
#154378=CARTESIAN_POINT('Ctrl Pts',(-40.2073940833052,60.5541617828925,
12.));
#154379=CARTESIAN_POINT('Ctrl Pts',(-40.2126982847011,60.5788666112042,
12.));
#154380=CARTESIAN_POINT('Ctrl Pts',(-40.2179872930273,60.6036151476349,
12.));
#154381=CARTESIAN_POINT('Ctrl Pts',(-40.2232610328721,60.6284073008871,
12.));
#154382=CARTESIAN_POINT('Ctrl Pts',(-40.2285194291706,60.6532429799499,
12.));
#154383=CARTESIAN_POINT('Ctrl Pts',(-40.2337624072029,60.678122094098,12.));
#154384=CARTESIAN_POINT('Ctrl Pts',(-40.2389898925932,60.7030445528857,
12.));
#154385=CARTESIAN_POINT('Ctrl Pts',(-40.2442018113108,60.728010266139,12.));
#154386=CARTESIAN_POINT('Ctrl Pts',(-40.2493980896638,60.7530191439593,
12.));
#154387=CARTESIAN_POINT('Ctrl Pts',(-40.2545786542953,60.7780710967248,
12.));
#154388=CARTESIAN_POINT('Ctrl Pts',(-40.2597434321803,60.8031660350879,
12.));
#154389=CARTESIAN_POINT('Ctrl Pts',(-40.2648923506248,60.8283038699706,
12.));
#154390=CARTESIAN_POINT('Ctrl Pts',(-40.2700253372647,60.8534845125538,
12.));
#154391=CARTESIAN_POINT('Ctrl Pts',(-40.2751423200639,60.8787078742818,
12.));
#154392=CARTESIAN_POINT('Ctrl Pts',(-40.2802432273104,60.9039738668669,
12.));
#154393=CARTESIAN_POINT('Ctrl Pts',(-40.2853279876161,60.9292824022887,
12.));
#154394=CARTESIAN_POINT('Ctrl Pts',(-40.2903965299155,60.9546333927921,
12.));
#154395=CARTESIAN_POINT('Ctrl Pts',(-40.295448783469,60.9800267508786,12.));
#154396=CARTESIAN_POINT('Ctrl Pts',(-40.300484677858,61.0054623893066,12.));
#154397=CARTESIAN_POINT('Ctrl Pts',(-40.3055041429775,61.0309402210921,
12.));
#154398=CARTESIAN_POINT('Ctrl Pts',(-40.3105071090309,61.056460159505,12.));
#154399=CARTESIAN_POINT('Ctrl Pts',(-40.3154935065262,61.0820221180645,
12.));
#154400=CARTESIAN_POINT('Ctrl Pts',(-40.3204632662725,61.1076260105258,
12.));
#154401=CARTESIAN_POINT('Ctrl Pts',(-40.32541631938,61.1332717508789,12.));
#154402=CARTESIAN_POINT('Ctrl Pts',(-40.3303525972615,61.1589592533613,
12.));
#154403=CARTESIAN_POINT('Ctrl Pts',(-40.335272031637,61.1846884324644,12.));
#154404=CARTESIAN_POINT('Ctrl Pts',(-40.340174554537,61.2104592029377,12.));
#154405=CARTESIAN_POINT('Ctrl Pts',(-40.3450600983109,61.23627147979,12.));
#154406=CARTESIAN_POINT('Ctrl Pts',(-40.3499285956304,61.2621251782863,
12.));
#154407=CARTESIAN_POINT('Ctrl Pts',(-40.3547799794679,61.2880202139371,
12.));
#154408=CARTESIAN_POINT('Ctrl Pts',(-40.3596141830791,61.3139565024847,
12.));
#154409=CARTESIAN_POINT('Ctrl Pts',(-40.3644311399861,61.3399339598853,
12.));
#154410=CARTESIAN_POINT('Ctrl Pts',(-40.3692307839636,61.3659525022908,
12.));
#154411=CARTESIAN_POINT('Ctrl Pts',(-40.3740130490225,61.3920120460219,
12.));
#154412=CARTESIAN_POINT('Ctrl Pts',(-40.3787778694364,61.4181125076037,
12.));
#154413=CARTESIAN_POINT('Ctrl Pts',(-40.383525179772,61.4442538038044,12.));
#154414=CARTESIAN_POINT('Ctrl Pts',(-40.3882549149227,61.4704358516709,
12.));
#154415=CARTESIAN_POINT('Ctrl Pts',(-40.3929670101366,61.4966585685549,
12.));
#154416=CARTESIAN_POINT('Ctrl Pts',(-40.3976614010652,61.522921872154,12.));
#154417=CARTESIAN_POINT('Ctrl Pts',(-40.4023380237232,61.5492256804717,
12.));
#154418=CARTESIAN_POINT('Ctrl Pts',(-40.4069968143956,61.5755699117324,
12.));
#154419=CARTESIAN_POINT('Ctrl Pts',(-40.4116377095596,61.601954484301,12.));
#154420=CARTESIAN_POINT('Ctrl Pts',(-40.4162606458119,61.628379316608,12.));
#154421=CARTESIAN_POINT('Ctrl Pts',(-40.4208655597717,61.6548443270394,
12.));
#154422=CARTESIAN_POINT('Ctrl Pts',(-40.425452388076,61.6813494339286,12.));
#154423=CARTESIAN_POINT('Ctrl Pts',(-40.430021067584,61.7078945557799,12.));
#154424=CARTESIAN_POINT('Ctrl Pts',(-40.4345715355404,61.7344796114399,
12.));
#154425=CARTESIAN_POINT('Ctrl Pts',(-40.4391037297588,61.7611045202874,
12.));
#154426=CARTESIAN_POINT('Ctrl Pts',(-40.4436175887949,61.7877692024076,
12.));
#154427=CARTESIAN_POINT('Ctrl Pts',(-40.4481130521364,61.814473578779,12.));
#154428=CARTESIAN_POINT('Ctrl Pts',(-40.4525900597894,61.8412175708552,
12.));
#154429=CARTESIAN_POINT('Ctrl Pts',(-40.4570485518749,61.8680011001537,
12.));
#154430=CARTESIAN_POINT('Ctrl Pts',(-40.4614884681889,61.8948240878008,
12.));
#154431=CARTESIAN_POINT('Ctrl Pts',(-40.4659097478587,61.9216864541744,
12.));
#154432=CARTESIAN_POINT('Ctrl Pts',(-40.470312328762,61.9485881182921,12.));
#154433=CARTESIAN_POINT('Ctrl Pts',(-40.4746961480015,61.9755289983044,
12.));
#154434=CARTESIAN_POINT('Ctrl Pts',(-40.4790611429583,62.0025090125959,
12.));
#154435=CARTESIAN_POINT('Ctrl Pts',(-40.4834072522164,62.029528080742,12.));
#154436=CARTESIAN_POINT('Ctrl Pts',(-40.4877344164411,62.0565861244179,
12.));
#154437=CARTESIAN_POINT('Ctrl Pts',(-40.4920425795216,62.0836830685719,
12.));
#154438=CARTESIAN_POINT('Ctrl Pts',(-40.4963316888412,62.1108188417003,
12.));
#154439=CARTESIAN_POINT('Ctrl Pts',(-40.4999919096264,62.1341126810541,
12.));
#154440=CARTESIAN_POINT('Ctrl Pts',(-40.5027877865802,62.1519925002973,
12.));
#154441=CARTESIAN_POINT('Ctrl Pts',(-40.5047277935766,62.164441150282,12.));
#154442=CARTESIAN_POINT('Ctrl Pts',(-40.5058175523127,62.17144731381,12.));
#154443=CARTESIAN_POINT('Ctrl Pts',(-40.5060598100929,62.1730054756869,
12.));
#154444=CARTESIAN_POINT('',(-39.4479504917286,57.8261117662439,0.));
#154445=CARTESIAN_POINT('',(-39.4479504917286,57.8261117662439,0.));
#154446=CARTESIAN_POINT('Ctrl Pts',(-40.5060598100929,62.1730054756869,
0.));
#154447=CARTESIAN_POINT('Ctrl Pts',(-40.5058175523127,62.17144731381,0.));
#154448=CARTESIAN_POINT('Ctrl Pts',(-40.5047277935766,62.164441150282,0.));
#154449=CARTESIAN_POINT('Ctrl Pts',(-40.5027877865802,62.1519925002973,
0.));
#154450=CARTESIAN_POINT('Ctrl Pts',(-40.4999919096264,62.1341126810541,
0.));
#154451=CARTESIAN_POINT('Ctrl Pts',(-40.4963316888412,62.1108188417003,
0.));
#154452=CARTESIAN_POINT('Ctrl Pts',(-40.4920425795216,62.0836830685719,
0.));
#154453=CARTESIAN_POINT('Ctrl Pts',(-40.4877344164411,62.0565861244179,
0.));
#154454=CARTESIAN_POINT('Ctrl Pts',(-40.4834072522164,62.029528080742,0.));
#154455=CARTESIAN_POINT('Ctrl Pts',(-40.4790611429583,62.0025090125959,
0.));
#154456=CARTESIAN_POINT('Ctrl Pts',(-40.4746961480015,61.9755289983044,
0.));
#154457=CARTESIAN_POINT('Ctrl Pts',(-40.470312328762,61.9485881182921,0.));
#154458=CARTESIAN_POINT('Ctrl Pts',(-40.4659097478587,61.9216864541744,
0.));
#154459=CARTESIAN_POINT('Ctrl Pts',(-40.4614884681889,61.8948240878008,
0.));
#154460=CARTESIAN_POINT('Ctrl Pts',(-40.4570485518749,61.8680011001537,
0.));
#154461=CARTESIAN_POINT('Ctrl Pts',(-40.4525900597894,61.8412175708552,
0.));
#154462=CARTESIAN_POINT('Ctrl Pts',(-40.4481130521364,61.814473578779,0.));
#154463=CARTESIAN_POINT('Ctrl Pts',(-40.4436175887949,61.7877692024076,
0.));
#154464=CARTESIAN_POINT('Ctrl Pts',(-40.4391037297588,61.7611045202874,
0.));
#154465=CARTESIAN_POINT('Ctrl Pts',(-40.4345715355404,61.7344796114399,
0.));
#154466=CARTESIAN_POINT('Ctrl Pts',(-40.430021067584,61.7078945557799,0.));
#154467=CARTESIAN_POINT('Ctrl Pts',(-40.425452388076,61.6813494339286,0.));
#154468=CARTESIAN_POINT('Ctrl Pts',(-40.4208655597717,61.6548443270394,
0.));
#154469=CARTESIAN_POINT('Ctrl Pts',(-40.4162606458119,61.628379316608,0.));
#154470=CARTESIAN_POINT('Ctrl Pts',(-40.4116377095596,61.601954484301,0.));
#154471=CARTESIAN_POINT('Ctrl Pts',(-40.4069968143956,61.5755699117324,
0.));
#154472=CARTESIAN_POINT('Ctrl Pts',(-40.4023380237232,61.5492256804717,
0.));
#154473=CARTESIAN_POINT('Ctrl Pts',(-40.3976614010652,61.522921872154,0.));
#154474=CARTESIAN_POINT('Ctrl Pts',(-40.3929670101366,61.4966585685549,
0.));
#154475=CARTESIAN_POINT('Ctrl Pts',(-40.3882549149227,61.4704358516709,
0.));
#154476=CARTESIAN_POINT('Ctrl Pts',(-40.383525179772,61.4442538038044,0.));
#154477=CARTESIAN_POINT('Ctrl Pts',(-40.3787778694364,61.4181125076037,
0.));
#154478=CARTESIAN_POINT('Ctrl Pts',(-40.3740130490225,61.3920120460219,
0.));
#154479=CARTESIAN_POINT('Ctrl Pts',(-40.3692307839636,61.3659525022908,
0.));
#154480=CARTESIAN_POINT('Ctrl Pts',(-40.3644311399861,61.3399339598853,
0.));
#154481=CARTESIAN_POINT('Ctrl Pts',(-40.3596141830791,61.3139565024847,
0.));
#154482=CARTESIAN_POINT('Ctrl Pts',(-40.3547799794679,61.2880202139371,
0.));
#154483=CARTESIAN_POINT('Ctrl Pts',(-40.3499285956304,61.2621251782863,
0.));
#154484=CARTESIAN_POINT('Ctrl Pts',(-40.3450600983109,61.23627147979,0.));
#154485=CARTESIAN_POINT('Ctrl Pts',(-40.340174554537,61.2104592029377,0.));
#154486=CARTESIAN_POINT('Ctrl Pts',(-40.335272031637,61.1846884324644,0.));
#154487=CARTESIAN_POINT('Ctrl Pts',(-40.3303525972615,61.1589592533613,
0.));
#154488=CARTESIAN_POINT('Ctrl Pts',(-40.32541631938,61.1332717508789,0.));
#154489=CARTESIAN_POINT('Ctrl Pts',(-40.3204632662725,61.1076260105258,
0.));
#154490=CARTESIAN_POINT('Ctrl Pts',(-40.3154935065262,61.0820221180645,
0.));
#154491=CARTESIAN_POINT('Ctrl Pts',(-40.3105071090309,61.056460159505,0.));
#154492=CARTESIAN_POINT('Ctrl Pts',(-40.3055041429775,61.0309402210921,
0.));
#154493=CARTESIAN_POINT('Ctrl Pts',(-40.300484677858,61.0054623893066,0.));
#154494=CARTESIAN_POINT('Ctrl Pts',(-40.295448783469,60.9800267508786,0.));
#154495=CARTESIAN_POINT('Ctrl Pts',(-40.2903965299155,60.9546333927921,
0.));
#154496=CARTESIAN_POINT('Ctrl Pts',(-40.2853279876161,60.9292824022887,
0.));
#154497=CARTESIAN_POINT('Ctrl Pts',(-40.2802432273104,60.9039738668669,
0.));
#154498=CARTESIAN_POINT('Ctrl Pts',(-40.2751423200639,60.8787078742818,
0.));
#154499=CARTESIAN_POINT('Ctrl Pts',(-40.2700253372647,60.8534845125538,
0.));
#154500=CARTESIAN_POINT('Ctrl Pts',(-40.2648923506248,60.8283038699706,
0.));
#154501=CARTESIAN_POINT('Ctrl Pts',(-40.2597434321803,60.8031660350879,
0.));
#154502=CARTESIAN_POINT('Ctrl Pts',(-40.2545786542953,60.7780710967248,
0.));
#154503=CARTESIAN_POINT('Ctrl Pts',(-40.2493980896638,60.7530191439593,
0.));
#154504=CARTESIAN_POINT('Ctrl Pts',(-40.2442018113108,60.728010266139,0.));
#154505=CARTESIAN_POINT('Ctrl Pts',(-40.2389898925932,60.7030445528857,
0.));
#154506=CARTESIAN_POINT('Ctrl Pts',(-40.2337624072029,60.678122094098,0.));
#154507=CARTESIAN_POINT('Ctrl Pts',(-40.2285194291706,60.6532429799499,
0.));
#154508=CARTESIAN_POINT('Ctrl Pts',(-40.2232610328721,60.6284073008871,
0.));
#154509=CARTESIAN_POINT('Ctrl Pts',(-40.2179872930273,60.6036151476349,
0.));
#154510=CARTESIAN_POINT('Ctrl Pts',(-40.2126982847011,60.5788666112042,
0.));
#154511=CARTESIAN_POINT('Ctrl Pts',(-40.2073940833052,60.5541617828925,
0.));
#154512=CARTESIAN_POINT('Ctrl Pts',(-40.2020747646014,60.5295007542841,
0.));
#154513=CARTESIAN_POINT('Ctrl Pts',(-40.1967404047062,60.5048836172435,
0.));
#154514=CARTESIAN_POINT('Ctrl Pts',(-40.1913910800921,60.4803104639226,
0.));
#154515=CARTESIAN_POINT('Ctrl Pts',(-40.1860268675883,60.455781386769,0.));
#154516=CARTESIAN_POINT('Ctrl Pts',(-40.180647844383,60.4312964785273,0.));
#154517=CARTESIAN_POINT('Ctrl Pts',(-40.1752540880268,60.4068558322407,
0.));
#154518=CARTESIAN_POINT('Ctrl Pts',(-40.1698456764377,60.3824595412445,
0.));
#154519=CARTESIAN_POINT('Ctrl Pts',(-40.1644226879033,60.3581076991716,
0.));
#154520=CARTESIAN_POINT('Ctrl Pts',(-40.1589852010804,60.3338003999607,
0.));
#154521=CARTESIAN_POINT('Ctrl Pts',(-40.1535332949976,60.3095377378586,
0.));
#154522=CARTESIAN_POINT('Ctrl Pts',(-40.1480670490586,60.285319807422,0.));
#154523=CARTESIAN_POINT('Ctrl Pts',(-40.1425865430472,60.2611467035117,
0.));
#154524=CARTESIAN_POINT('Ctrl Pts',(-40.1370918571304,60.2370185212964,
0.));
#154525=CARTESIAN_POINT('Ctrl Pts',(-40.1315830718577,60.2129353562622,
0.));
#154526=CARTESIAN_POINT('Ctrl Pts',(-40.1260602681644,60.1888973042152,
0.));
#154527=CARTESIAN_POINT('Ctrl Pts',(-40.1205235273739,60.1649044612828,
0.));
#154528=CARTESIAN_POINT('Ctrl Pts',(-40.1149729312036,60.1409569239092,
0.));
#154529=CARTESIAN_POINT('Ctrl Pts',(-40.1094085617674,60.1170547888574,
0.));
#154530=CARTESIAN_POINT('Ctrl Pts',(-40.1038305015766,60.0931981532198,
0.));
#154531=CARTESIAN_POINT('Ctrl Pts',(-40.0982388335423,60.069387114421,0.));
#154532=CARTESIAN_POINT('Ctrl Pts',(-40.0926336409785,60.0456217702202,
0.));
#154533=CARTESIAN_POINT('Ctrl Pts',(-40.0870150076074,60.021902218706,0.));
#154534=CARTESIAN_POINT('Ctrl Pts',(-40.0813830175623,59.9982285582983,
0.));
#154535=CARTESIAN_POINT('Ctrl Pts',(-40.0757377553888,59.9746008877584,
0.));
#154536=CARTESIAN_POINT('Ctrl Pts',(-40.0700793060473,59.9510193061927,
0.));
#154537=CARTESIAN_POINT('Ctrl Pts',(-40.0644077549159,59.9274839130553,
0.));
#154538=CARTESIAN_POINT('Ctrl Pts',(-40.0587231877961,59.9039948081432,
0.));
#154539=CARTESIAN_POINT('Ctrl Pts',(-40.0530256909162,59.8805520915975,
0.));
#154540=CARTESIAN_POINT('Ctrl Pts',(-40.0473153509323,59.8571558639145,
0.));
#154541=CARTESIAN_POINT('Ctrl Pts',(-40.0415922549313,59.8338062259491,
0.));
#154542=CARTESIAN_POINT('Ctrl Pts',(-40.035856490434,59.8105032789179,0.));
#154543=CARTESIAN_POINT('Ctrl Pts',(-40.0301081454006,59.7872471243948,
0.));
#154544=CARTESIAN_POINT('Ctrl Pts',(-40.0243473082343,59.7640378643115,
0.));
#154545=CARTESIAN_POINT('Ctrl Pts',(-40.0185740677827,59.7408756009688,
0.));
#154546=CARTESIAN_POINT('Ctrl Pts',(-40.0127885133407,59.7177604370409,
0.));
#154547=CARTESIAN_POINT('Ctrl Pts',(-40.0069907346536,59.6946924755771,
0.));
#154548=CARTESIAN_POINT('Ctrl Pts',(-40.001180821923,59.671671819999,0.));
#154549=CARTESIAN_POINT('Ctrl Pts',(-39.9953588658114,59.6486985741015,
0.));
#154550=CARTESIAN_POINT('Ctrl Pts',(-39.9895249574432,59.6257728420644,
0.));
#154551=CARTESIAN_POINT('Ctrl Pts',(-39.9836791884071,59.6028947284551,
0.));
#154552=CARTESIAN_POINT('Ctrl Pts',(-39.9778216507609,59.5800643382322,
0.));
#154553=CARTESIAN_POINT('Ctrl Pts',(-39.971952437036,59.5572817767412,0.));
#154554=CARTESIAN_POINT('Ctrl Pts',(-39.9660716402423,59.5345471497162,
0.));
#154555=CARTESIAN_POINT('Ctrl Pts',(-39.96017935387,59.511860563292,0.));
#154556=CARTESIAN_POINT('Ctrl Pts',(-39.954275671893,59.4892221240081,0.));
#154557=CARTESIAN_POINT('Ctrl Pts',(-39.9483606887731,59.4666319388123,
0.));
#154558=CARTESIAN_POINT('Ctrl Pts',(-39.9424344994652,59.444090115055,0.));
#154559=CARTESIAN_POINT('Ctrl Pts',(-39.9364971994215,59.4215967604925,
0.));
#154560=CARTESIAN_POINT('Ctrl Pts',(-39.9305488845934,59.3991519832981,
0.));
#154561=CARTESIAN_POINT('Ctrl Pts',(-39.9245896514359,59.3767558920663,
0.));
#154562=CARTESIAN_POINT('Ctrl Pts',(-39.9186195969113,59.3544085958165,
0.));
#154563=CARTESIAN_POINT('Ctrl Pts',(-39.9126388184956,59.3321102039883,
0.));
#154564=CARTESIAN_POINT('Ctrl Pts',(-39.9066474141826,59.3098608264452,
0.));
#154565=CARTESIAN_POINT('Ctrl Pts',(-39.9006454824861,59.2876605734871,
0.));
#154566=CARTESIAN_POINT('Ctrl Pts',(-39.8946331224442,59.2655095558527,
0.));
#154567=CARTESIAN_POINT('Ctrl Pts',(-39.8886104336234,59.2434078847236,
0.));
#154568=CARTESIAN_POINT('Ctrl Pts',(-39.8825775161252,59.2213556717189,
0.));
#154569=CARTESIAN_POINT('Ctrl Pts',(-39.8765344705894,59.1993530289008,
0.));
#154570=CARTESIAN_POINT('Ctrl Pts',(-39.8704813981978,59.1774000687865,
0.));
#154571=CARTESIAN_POINT('Ctrl Pts',(-39.8644184006785,59.155496904352,0.));
#154572=CARTESIAN_POINT('Ctrl Pts',(-39.8583455803111,59.133643649035,0.));
#154573=CARTESIAN_POINT('Ctrl Pts',(-39.8522630399337,59.1118404167304,
0.));
#154574=CARTESIAN_POINT('Ctrl Pts',(-39.8461708829465,59.0900873217992,
0.));
#154575=CARTESIAN_POINT('Ctrl Pts',(-39.8400692133143,59.068384479077,0.));
#154576=CARTESIAN_POINT('Ctrl Pts',(-39.8339581355714,59.0467320038782,
0.));
#154577=CARTESIAN_POINT('Ctrl Pts',(-39.8278377548261,59.0251300119973,
0.));
#154578=CARTESIAN_POINT('Ctrl Pts',(-39.8217081767658,59.0035786197024,
0.));
#154579=CARTESIAN_POINT('Ctrl Pts',(-39.8155695076625,58.9820779437485,
0.));
#154580=CARTESIAN_POINT('Ctrl Pts',(-39.8094218543781,58.9606281013876,
0.));
#154581=CARTESIAN_POINT('Ctrl Pts',(-39.8032653243712,58.9392292103747,
0.));
#154582=CARTESIAN_POINT('Ctrl Pts',(-39.7971000257044,58.9178813889703,
0.));
#154583=CARTESIAN_POINT('Ctrl Pts',(-39.7909260670517,58.896584755939,0.));
#154584=CARTESIAN_POINT('Ctrl Pts',(-39.7847435576995,58.8753394305583,
0.));
#154585=CARTESIAN_POINT('Ctrl Pts',(-39.7785526075477,58.8541455326229,
0.));
#154586=CARTESIAN_POINT('Ctrl Pts',(-39.772353327112,58.8330031824453,0.));
#154587=CARTESIAN_POINT('Ctrl Pts',(-39.7661458275276,58.8119125008521,
0.));
#154588=CARTESIAN_POINT('Ctrl Pts',(-39.7599302205527,58.7908736091808,
0.));
#154589=CARTESIAN_POINT('Ctrl Pts',(-39.753706618582,58.7698866293041,0.));
#154590=CARTESIAN_POINT('Ctrl Pts',(-39.7474751346603,58.7489516836453,
0.));
#154591=CARTESIAN_POINT('Ctrl Pts',(-39.7412358824949,58.7280688951911,
0.));
#154592=CARTESIAN_POINT('Ctrl Pts',(-39.7349889764737,58.7072383875009,
0.));
#154593=CARTESIAN_POINT('Ctrl Pts',(-39.7287345316664,58.6864602847064,
0.));
#154594=CARTESIAN_POINT('Ctrl Pts',(-39.7224726638087,58.6657347115014,
0.));
#154595=CARTESIAN_POINT('Ctrl Pts',(-39.7162034892896,58.6450617931269,
0.));
#154596=CARTESIAN_POINT('Ctrl Pts',(-39.7099271251421,58.6244416553574,
0.));
#154597=CARTESIAN_POINT('Ctrl Pts',(-39.7036436890248,58.6038744244683,
0.));
#154598=CARTESIAN_POINT('Ctrl Pts',(-39.6973532992555,58.5833602272767,
0.));
#154599=CARTESIAN_POINT('Ctrl Pts',(-39.6910560748639,58.5628991912067,
0.));
#154600=CARTESIAN_POINT('Ctrl Pts',(-39.6847521356395,58.5424914443415,
0.));
#154601=CARTESIAN_POINT('Ctrl Pts',(-39.6784416021817,58.5221371154748,
0.));
#154602=CARTESIAN_POINT('Ctrl Pts',(-39.6721245959516,58.5018363341582,
0.));
#154603=CARTESIAN_POINT('Ctrl Pts',(-39.66580123918,58.4815892306044,0.));
#154604=CARTESIAN_POINT('Ctrl Pts',(-39.659471654768,58.4613959355776,0.));
#154605=CARTESIAN_POINT('Ctrl Pts',(-39.6531359662043,58.4412565802984,
0.));
#154606=CARTESIAN_POINT('Ctrl Pts',(-39.6467942974464,58.4211712963024,
0.));
#154607=CARTESIAN_POINT('Ctrl Pts',(-39.6404467729113,58.4011402154225,
0.));
#154608=CARTESIAN_POINT('Ctrl Pts',(-39.6340935177492,58.3811634701061,
0.));
#154609=CARTESIAN_POINT('Ctrl Pts',(-39.6277346580898,58.3612411936914,
0.));
#154610=CARTESIAN_POINT('Ctrl Pts',(-39.6213703212523,58.3413735206412,
0.));
#154611=CARTESIAN_POINT('Ctrl Pts',(-39.6150006360894,58.3215605869192,
0.));
#154612=CARTESIAN_POINT('Ctrl Pts',(-39.6086257327559,58.3018025297288,
0.));
#154613=CARTESIAN_POINT('Ctrl Pts',(-39.6022457420772,58.2820994868092,
0.));
#154614=CARTESIAN_POINT('Ctrl Pts',(-39.5958607950237,58.2624515958416,
0.));
#154615=CARTESIAN_POINT('Ctrl Pts',(-39.5894710221729,58.2428589938394,
0.));
#154616=CARTESIAN_POINT('Ctrl Pts',(-39.5830765530919,58.2233218164407,
0.));
#154617=CARTESIAN_POINT('Ctrl Pts',(-39.5766775175226,58.2038401992496,
0.));
#154618=CARTESIAN_POINT('Ctrl Pts',(-39.5702740468013,58.1844142794359,
0.));
#154619=CARTESIAN_POINT('Ctrl Pts',(-39.5638662750174,58.1650441970379,
0.));
#154620=CARTESIAN_POINT('Ctrl Pts',(-39.5574543406959,58.1457300968467,
0.));
#154621=CARTESIAN_POINT('Ctrl Pts',(-39.5510383869476,58.1264721285698,
0.));
#154622=CARTESIAN_POINT('Ctrl Pts',(-39.5446185579615,58.1072704428895,
0.));
#154623=CARTESIAN_POINT('Ctrl Pts',(-39.5381949959214,58.088125187991,0.));
#154624=CARTESIAN_POINT('Ctrl Pts',(-39.5317678383231,58.0690365065393,
0.));
#154625=CARTESIAN_POINT('Ctrl Pts',(-39.5253372136921,58.050004530846,0.));
#154626=CARTESIAN_POINT('Ctrl Pts',(-39.5189032457227,58.0310293875321,
0.));
#154627=CARTESIAN_POINT('Ctrl Pts',(-39.5124660615009,58.012111206794,0.));
#154628=CARTESIAN_POINT('Ctrl Pts',(-39.5060257981225,57.9932501298522,
0.));
#154629=CARTESIAN_POINT('Ctrl Pts',(-39.4995826106691,57.9744463179305,
0.));
#154630=CARTESIAN_POINT('Ctrl Pts',(-39.4931366776627,57.9556999583777,
0.));
#154631=CARTESIAN_POINT('Ctrl Pts',(-39.4866881842223,57.9370112456506,
0.));
#154632=CARTESIAN_POINT('Ctrl Pts',(-39.4802373061008,57.9183803632337,
0.));
#154633=CARTESIAN_POINT('Ctrl Pts',(-39.4737841949417,57.8998074670541,
0.));
#154634=CARTESIAN_POINT('Ctrl Pts',(-39.4673289592425,57.8812926637397,
0.));
#154635=CARTESIAN_POINT('Ctrl Pts',(-39.4608716627367,57.8628360097134,
0.));
#154636=CARTESIAN_POINT('Ctrl Pts',(-39.4557042029884,57.8481172247805,
0.));
#154637=CARTESIAN_POINT('Ctrl Pts',(-39.45182770037,57.8371043151607,0.));
#154638=CARTESIAN_POINT('Ctrl Pts',(-39.4492429618498,57.829774010102,0.));
#154639=CARTESIAN_POINT('Ctrl Pts',(-39.4479504917286,57.8261117662439,
0.));
#154640=CARTESIAN_POINT('Ctrl Pts',(-34.9532422808861,65.7914953018525,
0.));
#154641=CARTESIAN_POINT('Ctrl Pts',(-34.9532422808861,65.7914953018525,
12.));
#154642=CARTESIAN_POINT('Ctrl Pts',(-34.9529266758466,65.7859084407617,
0.));
#154643=CARTESIAN_POINT('Ctrl Pts',(-34.9529266758466,65.7859084407617,
12.));
#154644=CARTESIAN_POINT('Ctrl Pts',(-34.9522931728759,65.7747383251112,
0.));
#154645=CARTESIAN_POINT('Ctrl Pts',(-34.9522931728759,65.7747383251112,
12.));
#154646=CARTESIAN_POINT('Ctrl Pts',(-34.9513360397454,65.7579939712289,
0.));
#154647=CARTESIAN_POINT('Ctrl Pts',(-34.9513360397454,65.7579939712289,
12.));
#154648=CARTESIAN_POINT('Ctrl Pts',(-34.9500461043246,65.7356898061147,
0.));
#154649=CARTESIAN_POINT('Ctrl Pts',(-34.9500461043246,65.7356898061147,
12.));
#154650=CARTESIAN_POINT('Ctrl Pts',(-34.9484107544137,65.7078456758034,
0.));
#154651=CARTESIAN_POINT('Ctrl Pts',(-34.9484107544137,65.7078456758034,
12.));
#154652=CARTESIAN_POINT('Ctrl Pts',(-34.9467524770439,65.6800376406066,
0.));
#154653=CARTESIAN_POINT('Ctrl Pts',(-34.9467524770439,65.6800376406066,
12.));
#154654=CARTESIAN_POINT('Ctrl Pts',(-34.9450712829183,65.6522657321322,
0.));
#154655=CARTESIAN_POINT('Ctrl Pts',(-34.9450712829183,65.6522657321322,
12.));
#154656=CARTESIAN_POINT('Ctrl Pts',(-34.943367193292,65.624529996851,0.));
#154657=CARTESIAN_POINT('Ctrl Pts',(-34.943367193292,65.624529996851,12.));
#154658=CARTESIAN_POINT('Ctrl Pts',(-34.9416402443435,65.5968304997584,
0.));
#154659=CARTESIAN_POINT('Ctrl Pts',(-34.9416402443435,65.5968304997584,
12.));
#154660=CARTESIAN_POINT('Ctrl Pts',(-34.9398904862157,65.5691673225803,
0.));
#154661=CARTESIAN_POINT('Ctrl Pts',(-34.9398904862157,65.5691673225803,
12.));
#154662=CARTESIAN_POINT('Ctrl Pts',(-34.9381179779673,65.5415405577955,
0.));
#154663=CARTESIAN_POINT('Ctrl Pts',(-34.9381179779673,65.5415405577955,
12.));
#154664=CARTESIAN_POINT('Ctrl Pts',(-34.9363227836582,65.5139503038036,
0.));
#154665=CARTESIAN_POINT('Ctrl Pts',(-34.9363227836582,65.5139503038036,
12.));
#154666=CARTESIAN_POINT('Ctrl Pts',(-34.9345049680825,65.4863966597544,
0.));
#154667=CARTESIAN_POINT('Ctrl Pts',(-34.9345049680825,65.4863966597544,
12.));
#154668=CARTESIAN_POINT('Ctrl Pts',(-34.932664592394,65.4588797201972,0.));
#154669=CARTESIAN_POINT('Ctrl Pts',(-34.932664592394,65.4588797201972,12.));
#154670=CARTESIAN_POINT('Ctrl Pts',(-34.9308017105536,65.4313995707536,
0.));
#154671=CARTESIAN_POINT('Ctrl Pts',(-34.9308017105536,65.4313995707536,
12.));
#154672=CARTESIAN_POINT('Ctrl Pts',(-34.9289163717747,65.4039562911352,
0.));
#154673=CARTESIAN_POINT('Ctrl Pts',(-34.9289163717747,65.4039562911352,
12.));
#154674=CARTESIAN_POINT('Ctrl Pts',(-34.9270086222731,65.3765499573077,
0.));
#154675=CARTESIAN_POINT('Ctrl Pts',(-34.9270086222731,65.3765499573077,
12.));
#154676=CARTESIAN_POINT('Ctrl Pts',(-34.9250785073477,65.3491806440537,
0.));
#154677=CARTESIAN_POINT('Ctrl Pts',(-34.9250785073477,65.3491806440537,
12.));
#154678=CARTESIAN_POINT('Ctrl Pts',(-34.9231260731831,65.321848427191,0.));
#154679=CARTESIAN_POINT('Ctrl Pts',(-34.9231260731831,65.321848427191,12.));
#154680=CARTESIAN_POINT('Ctrl Pts',(-34.9211513691355,65.2945533863761,
0.));
#154681=CARTESIAN_POINT('Ctrl Pts',(-34.9211513691355,65.2945533863761,
12.));
#154682=CARTESIAN_POINT('Ctrl Pts',(-34.9191544474872,65.2672956048069,
0.));
#154683=CARTESIAN_POINT('Ctrl Pts',(-34.9191544474872,65.2672956048069,
12.));
#154684=CARTESIAN_POINT('Ctrl Pts',(-34.9171353624113,65.2400751679549,
0.));
#154685=CARTESIAN_POINT('Ctrl Pts',(-34.9171353624113,65.2400751679549,
12.));
#154686=CARTESIAN_POINT('Ctrl Pts',(-34.9150941691747,65.2128921625823,
0.));
#154687=CARTESIAN_POINT('Ctrl Pts',(-34.9150941691747,65.2128921625823,
12.));
#154688=CARTESIAN_POINT('Ctrl Pts',(-34.9130309233022,65.1857466757092,
0.));
#154689=CARTESIAN_POINT('Ctrl Pts',(-34.9130309233022,65.1857466757092,
12.));
#154690=CARTESIAN_POINT('Ctrl Pts',(-34.9109456796213,65.1586387934241,
0.));
#154691=CARTESIAN_POINT('Ctrl Pts',(-34.9109456796213,65.1586387934241,
12.));
#154692=CARTESIAN_POINT('Ctrl Pts',(-34.9088384918336,65.1315686003516,
0.));
#154693=CARTESIAN_POINT('Ctrl Pts',(-34.9088384918336,65.1315686003516,
12.));
#154694=CARTESIAN_POINT('Ctrl Pts',(-34.9067094130399,65.1045361803121,
0.));
#154695=CARTESIAN_POINT('Ctrl Pts',(-34.9067094130399,65.1045361803121,
12.));
#154696=CARTESIAN_POINT('Ctrl Pts',(-34.9045584960509,65.0775416167085,
0.));
#154697=CARTESIAN_POINT('Ctrl Pts',(-34.9045584960509,65.0775416167085,
12.));
#154698=CARTESIAN_POINT('Ctrl Pts',(-34.9023857937865,65.0505849930171,
0.));
#154699=CARTESIAN_POINT('Ctrl Pts',(-34.9023857937865,65.0505849930171,
12.));
#154700=CARTESIAN_POINT('Ctrl Pts',(-34.9001913596416,65.0236663932328,
0.));
#154701=CARTESIAN_POINT('Ctrl Pts',(-34.9001913596416,65.0236663932328,
12.));
#154702=CARTESIAN_POINT('Ctrl Pts',(-34.8979752478616,64.9967859023212,
0.));
#154703=CARTESIAN_POINT('Ctrl Pts',(-34.8979752478616,64.9967859023212,
12.));
#154704=CARTESIAN_POINT('Ctrl Pts',(-34.8957375133697,64.9699436060169,
0.));
#154705=CARTESIAN_POINT('Ctrl Pts',(-34.8957375133697,64.9699436060169,
12.));
#154706=CARTESIAN_POINT('Ctrl Pts',(-34.8934782116095,64.9431395906337,
0.));
#154707=CARTESIAN_POINT('Ctrl Pts',(-34.8934782116095,64.9431395906337,
12.));
#154708=CARTESIAN_POINT('Ctrl Pts',(-34.8911973983785,64.9163739428605,
0.));
#154709=CARTESIAN_POINT('Ctrl Pts',(-34.8911973983785,64.9163739428605,
12.));
#154710=CARTESIAN_POINT('Ctrl Pts',(-34.888895129681,64.8896467495757,0.));
#154711=CARTESIAN_POINT('Ctrl Pts',(-34.888895129681,64.8896467495757,12.));
#154712=CARTESIAN_POINT('Ctrl Pts',(-34.8865714615436,64.8629580976063,
0.));
#154713=CARTESIAN_POINT('Ctrl Pts',(-34.8865714615436,64.8629580976063,
12.));
#154714=CARTESIAN_POINT('Ctrl Pts',(-34.8842264500188,64.8363080737377,
0.));
#154715=CARTESIAN_POINT('Ctrl Pts',(-34.8842264500188,64.8363080737377,
12.));
#154716=CARTESIAN_POINT('Ctrl Pts',(-34.881860151273,64.8096967648307,0.));
#154717=CARTESIAN_POINT('Ctrl Pts',(-34.881860151273,64.8096967648307,12.));
#154718=CARTESIAN_POINT('Ctrl Pts',(-34.8794726216513,64.7831242579028,
0.));
#154719=CARTESIAN_POINT('Ctrl Pts',(-34.8794726216513,64.7831242579028,
12.));
#154720=CARTESIAN_POINT('Ctrl Pts',(-34.8770639177493,64.7565906402151,
0.));
#154721=CARTESIAN_POINT('Ctrl Pts',(-34.8770639177493,64.7565906402151,
12.));
#154722=CARTESIAN_POINT('Ctrl Pts',(-34.8746340964971,64.7300959993653,
0.));
#154723=CARTESIAN_POINT('Ctrl Pts',(-34.8746340964971,64.7300959993653,
12.));
#154724=CARTESIAN_POINT('Ctrl Pts',(-34.8721832151974,64.7036404233306,
0.));
#154725=CARTESIAN_POINT('Ctrl Pts',(-34.8721832151974,64.7036404233306,
12.));
#154726=CARTESIAN_POINT('Ctrl Pts',(-34.869711331479,64.6772240004228,0.));
#154727=CARTESIAN_POINT('Ctrl Pts',(-34.869711331479,64.6772240004228,12.));
#154728=CARTESIAN_POINT('Ctrl Pts',(-34.867218503272,64.6508468192599,0.));
#154729=CARTESIAN_POINT('Ctrl Pts',(-34.867218503272,64.6508468192599,12.));
#154730=CARTESIAN_POINT('Ctrl Pts',(-34.8647047887774,64.6245089687277,
0.));
#154731=CARTESIAN_POINT('Ctrl Pts',(-34.8647047887774,64.6245089687277,
12.));
#154732=CARTESIAN_POINT('Ctrl Pts',(-34.8621702464401,64.5982105379383,
0.));
#154733=CARTESIAN_POINT('Ctrl Pts',(-34.8621702464401,64.5982105379383,
12.));
#154734=CARTESIAN_POINT('Ctrl Pts',(-34.8596149349257,64.5719516161927,
0.));
#154735=CARTESIAN_POINT('Ctrl Pts',(-34.8596149349257,64.5719516161927,
12.));
#154736=CARTESIAN_POINT('Ctrl Pts',(-34.857038913134,64.5457322930088,0.));
#154737=CARTESIAN_POINT('Ctrl Pts',(-34.857038913134,64.5457322930088,12.));
#154738=CARTESIAN_POINT('Ctrl Pts',(-34.8544422402118,64.5195526581407,
0.));
#154739=CARTESIAN_POINT('Ctrl Pts',(-34.8544422402118,64.5195526581407,
12.));
#154740=CARTESIAN_POINT('Ctrl Pts',(-34.851824975568,64.4934128015985,0.));
#154741=CARTESIAN_POINT('Ctrl Pts',(-34.851824975568,64.4934128015985,12.));
#154742=CARTESIAN_POINT('Ctrl Pts',(-34.8491871788895,64.4673128136625,
0.));
#154743=CARTESIAN_POINT('Ctrl Pts',(-34.8491871788895,64.4673128136625,
12.));
#154744=CARTESIAN_POINT('Ctrl Pts',(-34.8465289101621,64.4412527848969,
0.));
#154745=CARTESIAN_POINT('Ctrl Pts',(-34.8465289101621,64.4412527848969,
12.));
#154746=CARTESIAN_POINT('Ctrl Pts',(-34.8438502296664,64.4152328061515,
0.));
#154747=CARTESIAN_POINT('Ctrl Pts',(-34.8438502296664,64.4152328061515,
12.));
#154748=CARTESIAN_POINT('Ctrl Pts',(-34.8411511979702,64.3892529685607,
0.));
#154749=CARTESIAN_POINT('Ctrl Pts',(-34.8411511979702,64.3892529685607,
12.));
#154750=CARTESIAN_POINT('Ctrl Pts',(-34.8384318759248,64.3633133635382,
0.));
#154751=CARTESIAN_POINT('Ctrl Pts',(-34.8384318759248,64.3633133635382,
12.));
#154752=CARTESIAN_POINT('Ctrl Pts',(-34.8356923246618,64.3374140827711,
0.));
#154753=CARTESIAN_POINT('Ctrl Pts',(-34.8356923246618,64.3374140827711,
12.));
#154754=CARTESIAN_POINT('Ctrl Pts',(-34.8329326055919,64.3115552182062,
0.));
#154755=CARTESIAN_POINT('Ctrl Pts',(-34.8329326055919,64.3115552182062,
12.));
#154756=CARTESIAN_POINT('Ctrl Pts',(-34.8301527804054,64.285736862052,0.));
#154757=CARTESIAN_POINT('Ctrl Pts',(-34.8301527804054,64.285736862052,12.));
#154758=CARTESIAN_POINT('Ctrl Pts',(-34.8273529110744,64.2599591067916,
0.));
#154759=CARTESIAN_POINT('Ctrl Pts',(-34.8273529110744,64.2599591067916,
12.));
#154760=CARTESIAN_POINT('Ctrl Pts',(-34.8245330598559,64.234222045188,0.));
#154761=CARTESIAN_POINT('Ctrl Pts',(-34.8245330598559,64.234222045188,12.));
#154762=CARTESIAN_POINT('Ctrl Pts',(-34.8216932892968,64.2085257702884,
0.));
#154763=CARTESIAN_POINT('Ctrl Pts',(-34.8216932892968,64.2085257702884,
12.));
#154764=CARTESIAN_POINT('Ctrl Pts',(-34.8188336622419,64.1828703754236,
0.));
#154765=CARTESIAN_POINT('Ctrl Pts',(-34.8188336622419,64.1828703754236,
12.));
#154766=CARTESIAN_POINT('Ctrl Pts',(-34.8159542418374,64.1572559542086,
0.));
#154767=CARTESIAN_POINT('Ctrl Pts',(-34.8159542418374,64.1572559542086,
12.));
#154768=CARTESIAN_POINT('Ctrl Pts',(-34.8130550915287,64.1316826005506,
0.));
#154769=CARTESIAN_POINT('Ctrl Pts',(-34.8130550915287,64.1316826005506,
12.));
#154770=CARTESIAN_POINT('Ctrl Pts',(-34.8101362750597,64.1061504086515,
0.));
#154771=CARTESIAN_POINT('Ctrl Pts',(-34.8101362750597,64.1061504086515,
12.));
#154772=CARTESIAN_POINT('Ctrl Pts',(-34.8071978564747,64.0806594730085,
0.));
#154773=CARTESIAN_POINT('Ctrl Pts',(-34.8071978564747,64.0806594730085,
12.));
#154774=CARTESIAN_POINT('Ctrl Pts',(-34.8042399001211,64.0552098884095,
0.));
#154775=CARTESIAN_POINT('Ctrl Pts',(-34.8042399001211,64.0552098884095,
12.));
#154776=CARTESIAN_POINT('Ctrl Pts',(-34.8012624706526,64.0298017499294,
0.));
#154777=CARTESIAN_POINT('Ctrl Pts',(-34.8012624706526,64.0298017499294,
12.));
#154778=CARTESIAN_POINT('Ctrl Pts',(-34.7982656330293,64.0044351529402,
0.));
#154779=CARTESIAN_POINT('Ctrl Pts',(-34.7982656330293,64.0044351529402,
12.));
#154780=CARTESIAN_POINT('Ctrl Pts',(-34.7952494525177,63.9791101931162,
0.));
#154781=CARTESIAN_POINT('Ctrl Pts',(-34.7952494525177,63.9791101931162,
12.));
#154782=CARTESIAN_POINT('Ctrl Pts',(-34.7922139946943,63.9538269664366,
0.));
#154783=CARTESIAN_POINT('Ctrl Pts',(-34.7922139946943,63.9538269664366,
12.));
#154784=CARTESIAN_POINT('Ctrl Pts',(-34.7891593254488,63.9285855691845,
0.));
#154785=CARTESIAN_POINT('Ctrl Pts',(-34.7891593254488,63.9285855691845,
12.));
#154786=CARTESIAN_POINT('Ctrl Pts',(-34.7860855109911,63.9033860979435,
0.));
#154787=CARTESIAN_POINT('Ctrl Pts',(-34.7860855109911,63.9033860979435,
12.));
#154788=CARTESIAN_POINT('Ctrl Pts',(-34.7829926178496,63.8782286496062,
0.));
#154789=CARTESIAN_POINT('Ctrl Pts',(-34.7829926178496,63.8782286496062,
12.));
#154790=CARTESIAN_POINT('Ctrl Pts',(-34.7798807128715,63.8531133213793,
0.));
#154791=CARTESIAN_POINT('Ctrl Pts',(-34.7798807128715,63.8531133213793,
12.));
#154792=CARTESIAN_POINT('Ctrl Pts',(-34.7767498632243,63.8280402107856,
0.));
#154793=CARTESIAN_POINT('Ctrl Pts',(-34.7767498632243,63.8280402107856,
12.));
#154794=CARTESIAN_POINT('Ctrl Pts',(-34.7736001363993,63.8030094156639,
0.));
#154795=CARTESIAN_POINT('Ctrl Pts',(-34.7736001363993,63.8030094156639,
12.));
#154796=CARTESIAN_POINT('Ctrl Pts',(-34.7704316002171,63.778021034163,0.));
#154797=CARTESIAN_POINT('Ctrl Pts',(-34.7704316002171,63.778021034163,12.));
#154798=CARTESIAN_POINT('Ctrl Pts',(-34.7672443228275,63.7530751647494,
0.));
#154799=CARTESIAN_POINT('Ctrl Pts',(-34.7672443228275,63.7530751647494,
12.));
#154800=CARTESIAN_POINT('Ctrl Pts',(-34.7640383727101,63.7281719062149,
0.));
#154801=CARTESIAN_POINT('Ctrl Pts',(-34.7640383727101,63.7281719062149,
12.));
#154802=CARTESIAN_POINT('Ctrl Pts',(-34.7608138186759,63.7033113576785,
0.));
#154803=CARTESIAN_POINT('Ctrl Pts',(-34.7608138186759,63.7033113576785,
12.));
#154804=CARTESIAN_POINT('Ctrl Pts',(-34.7575707298713,63.6784936185885,
0.));
#154805=CARTESIAN_POINT('Ctrl Pts',(-34.7575707298713,63.6784936185885,
12.));
#154806=CARTESIAN_POINT('Ctrl Pts',(-34.7543091757833,63.6537187887159,
0.));
#154807=CARTESIAN_POINT('Ctrl Pts',(-34.7543091757833,63.6537187887159,
12.));
#154808=CARTESIAN_POINT('Ctrl Pts',(-34.7510292262406,63.6289869681604,
0.));
#154809=CARTESIAN_POINT('Ctrl Pts',(-34.7510292262406,63.6289869681604,
12.));
#154810=CARTESIAN_POINT('Ctrl Pts',(-34.7477309514136,63.6042982573588,
0.));
#154811=CARTESIAN_POINT('Ctrl Pts',(-34.7477309514136,63.6042982573588,
12.));
#154812=CARTESIAN_POINT('Ctrl Pts',(-34.744414421816,63.5796527570871,0.));
#154813=CARTESIAN_POINT('Ctrl Pts',(-34.744414421816,63.5796527570871,12.));
#154814=CARTESIAN_POINT('Ctrl Pts',(-34.7410797083081,63.5550505684626,
0.));
#154815=CARTESIAN_POINT('Ctrl Pts',(-34.7410797083081,63.5550505684626,
12.));
#154816=CARTESIAN_POINT('Ctrl Pts',(-34.7377268821025,63.5304917929386,
0.));
#154817=CARTESIAN_POINT('Ctrl Pts',(-34.7377268821025,63.5304917929386,
12.));
#154818=CARTESIAN_POINT('Ctrl Pts',(-34.7343560147667,63.505976532309,0.));
#154819=CARTESIAN_POINT('Ctrl Pts',(-34.7343560147667,63.505976532309,12.));
#154820=CARTESIAN_POINT('Ctrl Pts',(-34.7309671782214,63.4815048887165,
0.));
#154821=CARTESIAN_POINT('Ctrl Pts',(-34.7309671782214,63.4815048887165,
12.));
#154822=CARTESIAN_POINT('Ctrl Pts',(-34.7275604447439,63.4570769646569,
0.));
#154823=CARTESIAN_POINT('Ctrl Pts',(-34.7275604447439,63.4570769646569,
12.));
#154824=CARTESIAN_POINT('Ctrl Pts',(-34.7241358869701,63.4326928629795,
0.));
#154825=CARTESIAN_POINT('Ctrl Pts',(-34.7241358869701,63.4326928629795,
12.));
#154826=CARTESIAN_POINT('Ctrl Pts',(-34.7206935779007,63.4083526868836,
0.));
#154827=CARTESIAN_POINT('Ctrl Pts',(-34.7206935779007,63.4083526868836,
12.));
#154828=CARTESIAN_POINT('Ctrl Pts',(-34.7172335909038,63.3840565399208,
0.));
#154829=CARTESIAN_POINT('Ctrl Pts',(-34.7172335909038,63.3840565399208,
12.));
#154830=CARTESIAN_POINT('Ctrl Pts',(-34.7137559997146,63.3598045260053,
0.));
#154831=CARTESIAN_POINT('Ctrl Pts',(-34.7137559997146,63.3598045260053,
12.));
#154832=CARTESIAN_POINT('Ctrl Pts',(-34.7102608784374,63.3355967494171,
0.));
#154833=CARTESIAN_POINT('Ctrl Pts',(-34.7102608784374,63.3355967494171,
12.));
#154834=CARTESIAN_POINT('Ctrl Pts',(-34.7067483015491,63.3114333148048,
0.));
#154835=CARTESIAN_POINT('Ctrl Pts',(-34.7067483015491,63.3114333148048,
12.));
#154836=CARTESIAN_POINT('Ctrl Pts',(-34.703218343904,63.2873143271807,0.));
#154837=CARTESIAN_POINT('Ctrl Pts',(-34.703218343904,63.2873143271807,12.));
#154838=CARTESIAN_POINT('Ctrl Pts',(-34.6996710807378,63.2632398919225,
0.));
#154839=CARTESIAN_POINT('Ctrl Pts',(-34.6996710807378,63.2632398919225,
12.));
#154840=CARTESIAN_POINT('Ctrl Pts',(-34.6961065876666,63.2392101147847,
0.));
#154841=CARTESIAN_POINT('Ctrl Pts',(-34.6961065876666,63.2392101147847,
12.));
#154842=CARTESIAN_POINT('Ctrl Pts',(-34.6925249406897,63.2152251019012,
0.));
#154843=CARTESIAN_POINT('Ctrl Pts',(-34.6925249406897,63.2152251019012,
12.));
#154844=CARTESIAN_POINT('Ctrl Pts',(-34.6889262161924,63.1912849597887,
0.));
#154845=CARTESIAN_POINT('Ctrl Pts',(-34.6889262161924,63.1912849597887,
12.));
#154846=CARTESIAN_POINT('Ctrl Pts',(-34.6853104909518,63.1673897953429,
0.));
#154847=CARTESIAN_POINT('Ctrl Pts',(-34.6853104909518,63.1673897953429,
12.));
#154848=CARTESIAN_POINT('Ctrl Pts',(-34.6816778421402,63.1435397158388,
0.));
#154849=CARTESIAN_POINT('Ctrl Pts',(-34.6816778421402,63.1435397158388,
12.));
#154850=CARTESIAN_POINT('Ctrl Pts',(-34.6780283473252,63.119734828943,0.));
#154851=CARTESIAN_POINT('Ctrl Pts',(-34.6780283473252,63.119734828943,12.));
#154852=CARTESIAN_POINT('Ctrl Pts',(-34.674362084472,63.0959752427168,0.));
#154853=CARTESIAN_POINT('Ctrl Pts',(-34.674362084472,63.0959752427168,12.));
#154854=CARTESIAN_POINT('Ctrl Pts',(-34.670679131947,63.0722610656194,0.));
#154855=CARTESIAN_POINT('Ctrl Pts',(-34.670679131947,63.0722610656194,12.));
#154856=CARTESIAN_POINT('Ctrl Pts',(-34.6669795685228,63.0485924065045,
0.));
#154857=CARTESIAN_POINT('Ctrl Pts',(-34.6669795685228,63.0485924065045,
12.));
#154858=CARTESIAN_POINT('Ctrl Pts',(-34.6632634733824,63.0249693746208,
0.));
#154859=CARTESIAN_POINT('Ctrl Pts',(-34.6632634733824,63.0249693746208,
12.));
#154860=CARTESIAN_POINT('Ctrl Pts',(-34.6595309261191,63.0013920796235,
0.));
#154861=CARTESIAN_POINT('Ctrl Pts',(-34.6595309261191,63.0013920796235,
12.));
#154862=CARTESIAN_POINT('Ctrl Pts',(-34.6557820067393,62.9778606315783,
0.));
#154863=CARTESIAN_POINT('Ctrl Pts',(-34.6557820067393,62.9778606315783,
12.));
#154864=CARTESIAN_POINT('Ctrl Pts',(-34.6520167956655,62.9543751409645,
0.));
#154865=CARTESIAN_POINT('Ctrl Pts',(-34.6520167956655,62.9543751409645,
12.));
#154866=CARTESIAN_POINT('Ctrl Pts',(-34.6482353737424,62.9309357186717,
0.));
#154867=CARTESIAN_POINT('Ctrl Pts',(-34.6482353737424,62.9309357186717,
12.));
#154868=CARTESIAN_POINT('Ctrl Pts',(-34.6444378222411,62.9075424760015,
0.));
#154869=CARTESIAN_POINT('Ctrl Pts',(-34.6444378222411,62.9075424760015,
12.));
#154870=CARTESIAN_POINT('Ctrl Pts',(-34.6406242228592,62.8841955246794,
0.));
#154871=CARTESIAN_POINT('Ctrl Pts',(-34.6406242228592,62.8841955246794,
12.));
#154872=CARTESIAN_POINT('Ctrl Pts',(-34.6367946577235,62.8608949768571,
0.));
#154873=CARTESIAN_POINT('Ctrl Pts',(-34.6367946577235,62.8608949768571,
12.));
#154874=CARTESIAN_POINT('Ctrl Pts',(-34.6329492093935,62.8376409451175,
0.));
#154875=CARTESIAN_POINT('Ctrl Pts',(-34.6329492093935,62.8376409451175,
12.));
#154876=CARTESIAN_POINT('Ctrl Pts',(-34.6290879608673,62.8144335424697,
0.));
#154877=CARTESIAN_POINT('Ctrl Pts',(-34.6290879608673,62.8144335424697,
12.));
#154878=CARTESIAN_POINT('Ctrl Pts',(-34.6252109955853,62.7912728823518,
0.));
#154879=CARTESIAN_POINT('Ctrl Pts',(-34.6252109955853,62.7912728823518,
12.));
#154880=CARTESIAN_POINT('Ctrl Pts',(-34.6213183974317,62.7681590786429,
0.));
#154881=CARTESIAN_POINT('Ctrl Pts',(-34.6213183974317,62.7681590786429,
12.));
#154882=CARTESIAN_POINT('Ctrl Pts',(-34.6174102507375,62.7450922456676,
0.));
#154883=CARTESIAN_POINT('Ctrl Pts',(-34.6174102507375,62.7450922456676,
12.));
#154884=CARTESIAN_POINT('Ctrl Pts',(-34.6134866402837,62.7220724981994,
0.));
#154885=CARTESIAN_POINT('Ctrl Pts',(-34.6134866402837,62.7220724981994,
12.));
#154886=CARTESIAN_POINT('Ctrl Pts',(-34.6095476513077,62.6990999514563,
0.));
#154887=CARTESIAN_POINT('Ctrl Pts',(-34.6095476513077,62.6990999514563,
12.));
#154888=CARTESIAN_POINT('Ctrl Pts',(-34.6055933695069,62.6761747211037,
0.));
#154889=CARTESIAN_POINT('Ctrl Pts',(-34.6055933695069,62.6761747211037,
12.));
#154890=CARTESIAN_POINT('Ctrl Pts',(-34.6016238810399,62.6532969232657,
0.));
#154891=CARTESIAN_POINT('Ctrl Pts',(-34.6016238810399,62.6532969232657,
12.));
#154892=CARTESIAN_POINT('Ctrl Pts',(-34.5976392725296,62.6304666745306,
0.));
#154893=CARTESIAN_POINT('Ctrl Pts',(-34.5976392725296,62.6304666745306,
12.));
#154894=CARTESIAN_POINT('Ctrl Pts',(-34.5936396310679,62.6076840919536,
0.));
#154895=CARTESIAN_POINT('Ctrl Pts',(-34.5936396310679,62.6076840919536,
12.));
#154896=CARTESIAN_POINT('Ctrl Pts',(-34.5896250442216,62.5849492930533,
0.));
#154897=CARTESIAN_POINT('Ctrl Pts',(-34.5896250442216,62.5849492930533,
12.));
#154898=CARTESIAN_POINT('Ctrl Pts',(-34.5855956000363,62.562262395816,0.));
#154899=CARTESIAN_POINT('Ctrl Pts',(-34.5855956000363,62.562262395816,12.));
#154900=CARTESIAN_POINT('Ctrl Pts',(-34.5815513870377,62.5396235187079,
0.));
#154901=CARTESIAN_POINT('Ctrl Pts',(-34.5815513870377,62.5396235187079,
12.));
#154902=CARTESIAN_POINT('Ctrl Pts',(-34.5774924942355,62.5170327806781,
0.));
#154903=CARTESIAN_POINT('Ctrl Pts',(-34.5774924942355,62.5170327806781,
12.));
#154904=CARTESIAN_POINT('Ctrl Pts',(-34.5734190111272,62.4944903011628,
0.));
#154905=CARTESIAN_POINT('Ctrl Pts',(-34.5734190111272,62.4944903011628,
12.));
#154906=CARTESIAN_POINT('Ctrl Pts',(-34.5693310277051,62.4719962000808,
0.));
#154907=CARTESIAN_POINT('Ctrl Pts',(-34.5693310277051,62.4719962000808,
12.));
#154908=CARTESIAN_POINT('Ctrl Pts',(-34.5652286344593,62.4495505978393,
0.));
#154909=CARTESIAN_POINT('Ctrl Pts',(-34.5652286344593,62.4495505978393,
12.));
#154910=CARTESIAN_POINT('Ctrl Pts',(-34.5611119223798,62.4271536153459,
0.));
#154911=CARTESIAN_POINT('Ctrl Pts',(-34.5611119223798,62.4271536153459,
12.));
#154912=CARTESIAN_POINT('Ctrl Pts',(-34.5569809829613,62.4048053740127,
0.));
#154913=CARTESIAN_POINT('Ctrl Pts',(-34.5569809829613,62.4048053740127,
12.));
#154914=CARTESIAN_POINT('Ctrl Pts',(-34.5528359082075,62.3825059957601,
0.));
#154915=CARTESIAN_POINT('Ctrl Pts',(-34.5528359082075,62.3825059957601,
12.));
#154916=CARTESIAN_POINT('Ctrl Pts',(-34.5486767906384,62.3602556030127,
0.));
#154917=CARTESIAN_POINT('Ctrl Pts',(-34.5486767906384,62.3602556030127,
12.));
#154918=CARTESIAN_POINT('Ctrl Pts',(-34.5445037232936,62.338054318708,0.));
#154919=CARTESIAN_POINT('Ctrl Pts',(-34.5445037232936,62.338054318708,12.));
#154920=CARTESIAN_POINT('Ctrl Pts',(-34.5403167997337,62.3159022663058,
0.));
#154921=CARTESIAN_POINT('Ctrl Pts',(-34.5403167997337,62.3159022663058,
12.));
#154922=CARTESIAN_POINT('Ctrl Pts',(-34.5361161140449,62.2937995697925,
0.));
#154923=CARTESIAN_POINT('Ctrl Pts',(-34.5361161140449,62.2937995697925,
12.));
#154924=CARTESIAN_POINT('Ctrl Pts',(-34.5319017608433,62.2717463536827,
0.));
#154925=CARTESIAN_POINT('Ctrl Pts',(-34.5319017608433,62.2717463536827,
12.));
#154926=CARTESIAN_POINT('Ctrl Pts',(-34.5276738352808,62.2497427430135,
0.));
#154927=CARTESIAN_POINT('Ctrl Pts',(-34.5276738352808,62.2497427430135,
12.));
#154928=CARTESIAN_POINT('Ctrl Pts',(-34.523432433049,62.2277888633576,0.));
#154929=CARTESIAN_POINT('Ctrl Pts',(-34.523432433049,62.2277888633576,12.));
#154930=CARTESIAN_POINT('Ctrl Pts',(-34.5191776503842,62.2058848408347,
0.));
#154931=CARTESIAN_POINT('Ctrl Pts',(-34.5191776503842,62.2058848408347,
12.));
#154932=CARTESIAN_POINT('Ctrl Pts',(-34.514909584073,62.1840308021171,0.));
#154933=CARTESIAN_POINT('Ctrl Pts',(-34.514909584073,62.1840308021171,12.));
#154934=CARTESIAN_POINT('Ctrl Pts',(-34.5106283314594,62.1622268744336,
0.));
#154935=CARTESIAN_POINT('Ctrl Pts',(-34.5106283314594,62.1622268744336,
12.));
#154936=CARTESIAN_POINT('Ctrl Pts',(-34.5063339904533,62.1404731855686,
0.));
#154937=CARTESIAN_POINT('Ctrl Pts',(-34.5063339904533,62.1404731855686,
12.));
#154938=CARTESIAN_POINT('Ctrl Pts',(-34.5020266595292,62.1187698638705,
0.));
#154939=CARTESIAN_POINT('Ctrl Pts',(-34.5020266595292,62.1187698638705,
12.));
#154940=CARTESIAN_POINT('Ctrl Pts',(-34.4977064377281,62.0971170382565,
0.));
#154941=CARTESIAN_POINT('Ctrl Pts',(-34.4977064377281,62.0971170382565,
12.));
#154942=CARTESIAN_POINT('Ctrl Pts',(-34.4933734246592,62.0755148382136,
0.));
#154943=CARTESIAN_POINT('Ctrl Pts',(-34.4933734246592,62.0755148382136,
12.));
#154944=CARTESIAN_POINT('Ctrl Pts',(-34.4890277205042,62.0539633937944,
0.));
#154945=CARTESIAN_POINT('Ctrl Pts',(-34.4890277205042,62.0539633937944,
12.));
#154946=CARTESIAN_POINT('Ctrl Pts',(-34.4846694260205,62.0324628356152,
0.));
#154947=CARTESIAN_POINT('Ctrl Pts',(-34.4846694260205,62.0324628356152,
12.));
#154948=CARTESIAN_POINT('Ctrl Pts',(-34.4802986425535,62.0110132948807,
0.));
#154949=CARTESIAN_POINT('Ctrl Pts',(-34.4802986425535,62.0110132948807,
12.));
#154950=CARTESIAN_POINT('Ctrl Pts',(-34.4759154720477,61.9896149034009,
0.));
#154951=CARTESIAN_POINT('Ctrl Pts',(-34.4759154720477,61.9896149034009,
12.));
#154952=CARTESIAN_POINT('Ctrl Pts',(-34.4715200170589,61.9682677936048,
0.));
#154953=CARTESIAN_POINT('Ctrl Pts',(-34.4715200170589,61.9682677936048,
12.));
#154954=CARTESIAN_POINT('Ctrl Pts',(-34.4671123807706,61.9469720985512,
0.));
#154955=CARTESIAN_POINT('Ctrl Pts',(-34.4671123807706,61.9469720985512,
12.));
#154956=CARTESIAN_POINT('Ctrl Pts',(-34.462692666996,61.9257279519283,0.));
#154957=CARTESIAN_POINT('Ctrl Pts',(-34.462692666996,61.9257279519283,12.));
#154958=CARTESIAN_POINT('Ctrl Pts',(-34.4582609801625,61.9045354880424,
0.));
#154959=CARTESIAN_POINT('Ctrl Pts',(-34.4582609801625,61.9045354880424,
12.));
#154960=CARTESIAN_POINT('Ctrl Pts',(-34.4538174253009,61.883394841802,0.));
#154961=CARTESIAN_POINT('Ctrl Pts',(-34.4538174253009,61.883394841802,12.));
#154962=CARTESIAN_POINT('Ctrl Pts',(-34.4493621080367,61.862306148703,0.));
#154963=CARTESIAN_POINT('Ctrl Pts',(-34.4493621080367,61.862306148703,12.));
#154964=CARTESIAN_POINT('Ctrl Pts',(-34.4448951345753,61.8412695447951,
0.));
#154965=CARTESIAN_POINT('Ctrl Pts',(-34.4448951345753,61.8412695447951,
12.));
#154966=CARTESIAN_POINT('Ctrl Pts',(-34.4404166117313,61.8202851667247,
0.));
#154967=CARTESIAN_POINT('Ctrl Pts',(-34.4404166117313,61.8202851667247,
12.));
#154968=CARTESIAN_POINT('Ctrl Pts',(-34.4359266469757,61.7993531518052,
0.));
#154969=CARTESIAN_POINT('Ctrl Pts',(-34.4359266469757,61.7993531518052,
12.));
#154970=CARTESIAN_POINT('Ctrl Pts',(-34.4314253484791,61.7784736380727,
0.));
#154971=CARTESIAN_POINT('Ctrl Pts',(-34.4314253484791,61.7784736380727,
12.));
#154972=CARTESIAN_POINT('Ctrl Pts',(-34.4269128251569,61.7576467643419,
0.));
#154973=CARTESIAN_POINT('Ctrl Pts',(-34.4269128251569,61.7576467643419,
12.));
#154974=CARTESIAN_POINT('Ctrl Pts',(-34.4223891867166,61.7368726702573,
0.));
#154975=CARTESIAN_POINT('Ctrl Pts',(-34.4223891867166,61.7368726702573,
12.));
#154976=CARTESIAN_POINT('Ctrl Pts',(-34.4178545435753,61.7161514961892,
0.));
#154977=CARTESIAN_POINT('Ctrl Pts',(-34.4178545435753,61.7161514961892,
12.));
#154978=CARTESIAN_POINT('Ctrl Pts',(-34.4133090067696,61.6954833831157,
0.));
#154979=CARTESIAN_POINT('Ctrl Pts',(-34.4133090067696,61.6954833831157,
12.));
#154980=CARTESIAN_POINT('Ctrl Pts',(-34.4087526878815,61.674868472521,0.));
#154981=CARTESIAN_POINT('Ctrl Pts',(-34.4087526878815,61.674868472521,12.));
#154982=CARTESIAN_POINT('Ctrl Pts',(-34.4041856989328,61.6543069062436,
0.));
#154983=CARTESIAN_POINT('Ctrl Pts',(-34.4041856989328,61.6543069062436,
12.));
#154984=CARTESIAN_POINT('Ctrl Pts',(-34.399608152377,61.6337988264586,0.));
#154985=CARTESIAN_POINT('Ctrl Pts',(-34.399608152377,61.6337988264586,12.));
#154986=CARTESIAN_POINT('Ctrl Pts',(-34.3950201613446,61.6133443760168,
0.));
#154987=CARTESIAN_POINT('Ctrl Pts',(-34.3950201613446,61.6133443760168,
12.));
#154988=CARTESIAN_POINT('Ctrl Pts',(-34.3904218398642,61.5929436987419,
0.));
#154989=CARTESIAN_POINT('Ctrl Pts',(-34.3904218398642,61.5929436987419,
12.));
#154990=CARTESIAN_POINT('Ctrl Pts',(-34.3858133030511,61.5725969396817,
0.));
#154991=CARTESIAN_POINT('Ctrl Pts',(-34.3858133030511,61.5725969396817,
12.));
#154992=CARTESIAN_POINT('Ctrl Pts',(-34.3811946674179,61.5523042455127,
0.));
#154993=CARTESIAN_POINT('Ctrl Pts',(-34.3811946674179,61.5523042455127,
12.));
#154994=CARTESIAN_POINT('Ctrl Pts',(-34.3765660506659,61.5320657642601,
0.));
#154995=CARTESIAN_POINT('Ctrl Pts',(-34.3765660506659,61.5320657642601,
12.));
#154996=CARTESIAN_POINT('Ctrl Pts',(-34.3719275711179,61.511881644541,0.));
#154997=CARTESIAN_POINT('Ctrl Pts',(-34.3719275711179,61.511881644541,12.));
#154998=CARTESIAN_POINT('Ctrl Pts',(-34.3672793472464,61.4917520349276,
0.));
#154999=CARTESIAN_POINT('Ctrl Pts',(-34.3672793472464,61.4917520349276,
12.));
#155000=CARTESIAN_POINT('Ctrl Pts',(-34.3626214971903,61.4716770832924,
0.));
#155001=CARTESIAN_POINT('Ctrl Pts',(-34.3626214971903,61.4716770832924,
12.));
#155002=CARTESIAN_POINT('Ctrl Pts',(-34.357954138202,61.4516569360499,0.));
#155003=CARTESIAN_POINT('Ctrl Pts',(-34.357954138202,61.4516569360499,12.));
#155004=CARTESIAN_POINT('Ctrl Pts',(-34.3532773877112,61.4316917395959,
0.));
#155005=CARTESIAN_POINT('Ctrl Pts',(-34.3532773877112,61.4316917395959,
12.));
#155006=CARTESIAN_POINT('Ctrl Pts',(-34.3485913645991,61.4117816420251,
0.));
#155007=CARTESIAN_POINT('Ctrl Pts',(-34.3485913645991,61.4117816420251,
12.));
#155008=CARTESIAN_POINT('Ctrl Pts',(-34.34389619024,61.3919267945293,0.));
#155009=CARTESIAN_POINT('Ctrl Pts',(-34.34389619024,61.3919267945293,12.));
#155010=CARTESIAN_POINT('Ctrl Pts',(-34.339191990012,61.3721273534222,0.));
#155011=CARTESIAN_POINT('Ctrl Pts',(-34.339191990012,61.3721273534222,12.));
#155012=CARTESIAN_POINT('Ctrl Pts',(-34.3344788934337,61.3523834803144,
0.));
#155013=CARTESIAN_POINT('Ctrl Pts',(-34.3344788934337,61.3523834803144,
12.));
#155014=CARTESIAN_POINT('Ctrl Pts',(-34.3297570310126,61.3326953378817,
0.));
#155015=CARTESIAN_POINT('Ctrl Pts',(-34.3297570310126,61.3326953378817,
12.));
#155016=CARTESIAN_POINT('Ctrl Pts',(-34.3250265314761,61.3130630861375,
0.));
#155017=CARTESIAN_POINT('Ctrl Pts',(-34.3250265314761,61.3130630861375,
12.));
#155018=CARTESIAN_POINT('Ctrl Pts',(-34.3202875193629,61.2934868791875,
0.));
#155019=CARTESIAN_POINT('Ctrl Pts',(-34.3202875193629,61.2934868791875,
12.));
#155020=CARTESIAN_POINT('Ctrl Pts',(-34.3155401111776,61.2739668600415,
0.));
#155021=CARTESIAN_POINT('Ctrl Pts',(-34.3155401111776,61.2739668600415,
12.));
#155022=CARTESIAN_POINT('Ctrl Pts',(-34.3107844191081,61.2545031656196,
0.));
#155023=CARTESIAN_POINT('Ctrl Pts',(-34.3107844191081,61.2545031656196,
12.));
#155024=CARTESIAN_POINT('Ctrl Pts',(-34.3060205584093,61.2350959366987,
0.));
#155025=CARTESIAN_POINT('Ctrl Pts',(-34.3060205584093,61.2350959366987,
12.));
#155026=CARTESIAN_POINT('Ctrl Pts',(-34.3012486533474,61.2157453259107,
0.));
#155027=CARTESIAN_POINT('Ctrl Pts',(-34.3012486533474,61.2157453259107,
12.));
#155028=CARTESIAN_POINT('Ctrl Pts',(-34.296468844362,61.1964515073823,0.));
#155029=CARTESIAN_POINT('Ctrl Pts',(-34.296468844362,61.1964515073823,12.));
#155030=CARTESIAN_POINT('Ctrl Pts',(-34.2916812929675,61.1772146833083,
0.));
#155031=CARTESIAN_POINT('Ctrl Pts',(-34.2916812929675,61.1772146833083,
12.));
#155032=CARTESIAN_POINT('Ctrl Pts',(-34.2868861666301,61.15803506354,0.));
#155033=CARTESIAN_POINT('Ctrl Pts',(-34.2868861666301,61.15803506354,12.));
#155034=CARTESIAN_POINT('Ctrl Pts',(-34.2820836244425,61.1389128461815,
0.));
#155035=CARTESIAN_POINT('Ctrl Pts',(-34.2820836244425,61.1389128461815,
12.));
#155036=CARTESIAN_POINT('Ctrl Pts',(-34.2772738038812,61.119848199783,0.));
#155037=CARTESIAN_POINT('Ctrl Pts',(-34.2772738038812,61.119848199783,12.));
#155038=CARTESIAN_POINT('Ctrl Pts',(-34.2724568037374,61.100841240023,0.));
#155039=CARTESIAN_POINT('Ctrl Pts',(-34.2724568037374,61.100841240023,12.));
#155040=CARTESIAN_POINT('Ctrl Pts',(-34.2676326825846,61.0818920286644,
0.));
#155041=CARTESIAN_POINT('Ctrl Pts',(-34.2676326825846,61.0818920286644,
12.));
#155042=CARTESIAN_POINT('Ctrl Pts',(-34.2637677132139,61.0667788793594,
0.));
#155043=CARTESIAN_POINT('Ctrl Pts',(-34.2637677132139,61.0667788793594,
12.));
#155044=CARTESIAN_POINT('Ctrl Pts',(-34.2608658001761,61.0554700177206,
0.));
#155045=CARTESIAN_POINT('Ctrl Pts',(-34.2608658001761,61.0554700177206,
12.));
#155046=CARTESIAN_POINT('Ctrl Pts',(-34.2589297755482,61.0479423318803,
0.));
#155047=CARTESIAN_POINT('Ctrl Pts',(-34.2589297755482,61.0479423318803,
12.));
#155048=CARTESIAN_POINT('Ctrl Pts',(-34.2579614092497,61.0441813777723,
0.));
#155049=CARTESIAN_POINT('Ctrl Pts',(-34.2579614092497,61.0441813777723,
12.));
#155050=CARTESIAN_POINT('',(-34.2579614092497,61.0441813777723,12.));
#155051=CARTESIAN_POINT('Ctrl Pts',(-34.2579614092497,61.0441813777723,
12.));
#155052=CARTESIAN_POINT('Ctrl Pts',(-34.2589297755482,61.0479423318803,
12.));
#155053=CARTESIAN_POINT('Ctrl Pts',(-34.2608658001761,61.0554700177206,
12.));
#155054=CARTESIAN_POINT('Ctrl Pts',(-34.2637677132139,61.0667788793594,
12.));
#155055=CARTESIAN_POINT('Ctrl Pts',(-34.2676326825846,61.0818920286644,
12.));
#155056=CARTESIAN_POINT('Ctrl Pts',(-34.2724568037374,61.100841240023,12.));
#155057=CARTESIAN_POINT('Ctrl Pts',(-34.2772738038812,61.119848199783,12.));
#155058=CARTESIAN_POINT('Ctrl Pts',(-34.2820836244425,61.1389128461815,
12.));
#155059=CARTESIAN_POINT('Ctrl Pts',(-34.2868861666301,61.15803506354,12.));
#155060=CARTESIAN_POINT('Ctrl Pts',(-34.2916812929675,61.1772146833083,
12.));
#155061=CARTESIAN_POINT('Ctrl Pts',(-34.296468844362,61.1964515073823,12.));
#155062=CARTESIAN_POINT('Ctrl Pts',(-34.3012486533474,61.2157453259107,
12.));
#155063=CARTESIAN_POINT('Ctrl Pts',(-34.3060205584093,61.2350959366987,
12.));
#155064=CARTESIAN_POINT('Ctrl Pts',(-34.3107844191081,61.2545031656196,
12.));
#155065=CARTESIAN_POINT('Ctrl Pts',(-34.3155401111776,61.2739668600415,
12.));
#155066=CARTESIAN_POINT('Ctrl Pts',(-34.3202875193629,61.2934868791875,
12.));
#155067=CARTESIAN_POINT('Ctrl Pts',(-34.3250265314761,61.3130630861375,
12.));
#155068=CARTESIAN_POINT('Ctrl Pts',(-34.3297570310126,61.3326953378817,
12.));
#155069=CARTESIAN_POINT('Ctrl Pts',(-34.3344788934337,61.3523834803144,
12.));
#155070=CARTESIAN_POINT('Ctrl Pts',(-34.339191990012,61.3721273534222,12.));
#155071=CARTESIAN_POINT('Ctrl Pts',(-34.34389619024,61.3919267945293,12.));
#155072=CARTESIAN_POINT('Ctrl Pts',(-34.3485913645991,61.4117816420251,
12.));
#155073=CARTESIAN_POINT('Ctrl Pts',(-34.3532773877112,61.4316917395959,
12.));
#155074=CARTESIAN_POINT('Ctrl Pts',(-34.357954138202,61.4516569360499,12.));
#155075=CARTESIAN_POINT('Ctrl Pts',(-34.3626214971903,61.4716770832924,
12.));
#155076=CARTESIAN_POINT('Ctrl Pts',(-34.3672793472464,61.4917520349276,
12.));
#155077=CARTESIAN_POINT('Ctrl Pts',(-34.3719275711179,61.511881644541,12.));
#155078=CARTESIAN_POINT('Ctrl Pts',(-34.3765660506659,61.5320657642601,
12.));
#155079=CARTESIAN_POINT('Ctrl Pts',(-34.3811946674179,61.5523042455127,
12.));
#155080=CARTESIAN_POINT('Ctrl Pts',(-34.3858133030511,61.5725969396817,
12.));
#155081=CARTESIAN_POINT('Ctrl Pts',(-34.3904218398642,61.5929436987419,
12.));
#155082=CARTESIAN_POINT('Ctrl Pts',(-34.3950201613446,61.6133443760168,
12.));
#155083=CARTESIAN_POINT('Ctrl Pts',(-34.399608152377,61.6337988264586,12.));
#155084=CARTESIAN_POINT('Ctrl Pts',(-34.4041856989328,61.6543069062436,
12.));
#155085=CARTESIAN_POINT('Ctrl Pts',(-34.4087526878815,61.674868472521,12.));
#155086=CARTESIAN_POINT('Ctrl Pts',(-34.4133090067696,61.6954833831157,
12.));
#155087=CARTESIAN_POINT('Ctrl Pts',(-34.4178545435753,61.7161514961892,
12.));
#155088=CARTESIAN_POINT('Ctrl Pts',(-34.4223891867166,61.7368726702573,
12.));
#155089=CARTESIAN_POINT('Ctrl Pts',(-34.4269128251569,61.7576467643419,
12.));
#155090=CARTESIAN_POINT('Ctrl Pts',(-34.4314253484791,61.7784736380727,
12.));
#155091=CARTESIAN_POINT('Ctrl Pts',(-34.4359266469757,61.7993531518052,
12.));
#155092=CARTESIAN_POINT('Ctrl Pts',(-34.4404166117313,61.8202851667247,
12.));
#155093=CARTESIAN_POINT('Ctrl Pts',(-34.4448951345753,61.8412695447951,
12.));
#155094=CARTESIAN_POINT('Ctrl Pts',(-34.4493621080367,61.862306148703,12.));
#155095=CARTESIAN_POINT('Ctrl Pts',(-34.4538174253009,61.883394841802,12.));
#155096=CARTESIAN_POINT('Ctrl Pts',(-34.4582609801625,61.9045354880424,
12.));
#155097=CARTESIAN_POINT('Ctrl Pts',(-34.462692666996,61.9257279519283,12.));
#155098=CARTESIAN_POINT('Ctrl Pts',(-34.4671123807706,61.9469720985512,
12.));
#155099=CARTESIAN_POINT('Ctrl Pts',(-34.4715200170589,61.9682677936048,
12.));
#155100=CARTESIAN_POINT('Ctrl Pts',(-34.4759154720477,61.9896149034009,
12.));
#155101=CARTESIAN_POINT('Ctrl Pts',(-34.4802986425535,62.0110132948807,
12.));
#155102=CARTESIAN_POINT('Ctrl Pts',(-34.4846694260205,62.0324628356152,
12.));
#155103=CARTESIAN_POINT('Ctrl Pts',(-34.4890277205042,62.0539633937944,
12.));
#155104=CARTESIAN_POINT('Ctrl Pts',(-34.4933734246592,62.0755148382136,
12.));
#155105=CARTESIAN_POINT('Ctrl Pts',(-34.4977064377281,62.0971170382565,
12.));
#155106=CARTESIAN_POINT('Ctrl Pts',(-34.5020266595292,62.1187698638705,
12.));
#155107=CARTESIAN_POINT('Ctrl Pts',(-34.5063339904533,62.1404731855686,
12.));
#155108=CARTESIAN_POINT('Ctrl Pts',(-34.5106283314594,62.1622268744336,
12.));
#155109=CARTESIAN_POINT('Ctrl Pts',(-34.514909584073,62.1840308021171,12.));
#155110=CARTESIAN_POINT('Ctrl Pts',(-34.5191776503842,62.2058848408347,
12.));
#155111=CARTESIAN_POINT('Ctrl Pts',(-34.523432433049,62.2277888633576,12.));
#155112=CARTESIAN_POINT('Ctrl Pts',(-34.5276738352808,62.2497427430135,
12.));
#155113=CARTESIAN_POINT('Ctrl Pts',(-34.5319017608433,62.2717463536827,
12.));
#155114=CARTESIAN_POINT('Ctrl Pts',(-34.5361161140449,62.2937995697925,
12.));
#155115=CARTESIAN_POINT('Ctrl Pts',(-34.5403167997337,62.3159022663058,
12.));
#155116=CARTESIAN_POINT('Ctrl Pts',(-34.5445037232936,62.338054318708,12.));
#155117=CARTESIAN_POINT('Ctrl Pts',(-34.5486767906384,62.3602556030127,
12.));
#155118=CARTESIAN_POINT('Ctrl Pts',(-34.5528359082075,62.3825059957601,
12.));
#155119=CARTESIAN_POINT('Ctrl Pts',(-34.5569809829613,62.4048053740127,
12.));
#155120=CARTESIAN_POINT('Ctrl Pts',(-34.5611119223798,62.4271536153459,
12.));
#155121=CARTESIAN_POINT('Ctrl Pts',(-34.5652286344593,62.4495505978393,
12.));
#155122=CARTESIAN_POINT('Ctrl Pts',(-34.5693310277051,62.4719962000808,
12.));
#155123=CARTESIAN_POINT('Ctrl Pts',(-34.5734190111272,62.4944903011628,
12.));
#155124=CARTESIAN_POINT('Ctrl Pts',(-34.5774924942355,62.5170327806781,
12.));
#155125=CARTESIAN_POINT('Ctrl Pts',(-34.5815513870377,62.5396235187079,
12.));
#155126=CARTESIAN_POINT('Ctrl Pts',(-34.5855956000363,62.562262395816,12.));
#155127=CARTESIAN_POINT('Ctrl Pts',(-34.5896250442216,62.5849492930533,
12.));
#155128=CARTESIAN_POINT('Ctrl Pts',(-34.5936396310679,62.6076840919536,
12.));
#155129=CARTESIAN_POINT('Ctrl Pts',(-34.5976392725296,62.6304666745306,
12.));
#155130=CARTESIAN_POINT('Ctrl Pts',(-34.6016238810399,62.6532969232657,
12.));
#155131=CARTESIAN_POINT('Ctrl Pts',(-34.6055933695069,62.6761747211037,
12.));
#155132=CARTESIAN_POINT('Ctrl Pts',(-34.6095476513077,62.6990999514563,
12.));
#155133=CARTESIAN_POINT('Ctrl Pts',(-34.6134866402837,62.7220724981994,
12.));
#155134=CARTESIAN_POINT('Ctrl Pts',(-34.6174102507375,62.7450922456676,
12.));
#155135=CARTESIAN_POINT('Ctrl Pts',(-34.6213183974317,62.7681590786429,
12.));
#155136=CARTESIAN_POINT('Ctrl Pts',(-34.6252109955853,62.7912728823518,
12.));
#155137=CARTESIAN_POINT('Ctrl Pts',(-34.6290879608673,62.8144335424697,
12.));
#155138=CARTESIAN_POINT('Ctrl Pts',(-34.6329492093935,62.8376409451175,
12.));
#155139=CARTESIAN_POINT('Ctrl Pts',(-34.6367946577235,62.8608949768571,
12.));
#155140=CARTESIAN_POINT('Ctrl Pts',(-34.6406242228592,62.8841955246794,
12.));
#155141=CARTESIAN_POINT('Ctrl Pts',(-34.6444378222411,62.9075424760015,
12.));
#155142=CARTESIAN_POINT('Ctrl Pts',(-34.6482353737424,62.9309357186717,
12.));
#155143=CARTESIAN_POINT('Ctrl Pts',(-34.6520167956655,62.9543751409645,
12.));
#155144=CARTESIAN_POINT('Ctrl Pts',(-34.6557820067393,62.9778606315783,
12.));
#155145=CARTESIAN_POINT('Ctrl Pts',(-34.6595309261191,63.0013920796235,
12.));
#155146=CARTESIAN_POINT('Ctrl Pts',(-34.6632634733824,63.0249693746208,
12.));
#155147=CARTESIAN_POINT('Ctrl Pts',(-34.6669795685228,63.0485924065045,
12.));
#155148=CARTESIAN_POINT('Ctrl Pts',(-34.670679131947,63.0722610656194,12.));
#155149=CARTESIAN_POINT('Ctrl Pts',(-34.674362084472,63.0959752427168,12.));
#155150=CARTESIAN_POINT('Ctrl Pts',(-34.6780283473252,63.119734828943,12.));
#155151=CARTESIAN_POINT('Ctrl Pts',(-34.6816778421402,63.1435397158388,
12.));
#155152=CARTESIAN_POINT('Ctrl Pts',(-34.6853104909518,63.1673897953429,
12.));
#155153=CARTESIAN_POINT('Ctrl Pts',(-34.6889262161924,63.1912849597887,
12.));
#155154=CARTESIAN_POINT('Ctrl Pts',(-34.6925249406897,63.2152251019012,
12.));
#155155=CARTESIAN_POINT('Ctrl Pts',(-34.6961065876666,63.2392101147847,
12.));
#155156=CARTESIAN_POINT('Ctrl Pts',(-34.6996710807378,63.2632398919225,
12.));
#155157=CARTESIAN_POINT('Ctrl Pts',(-34.703218343904,63.2873143271807,12.));
#155158=CARTESIAN_POINT('Ctrl Pts',(-34.7067483015491,63.3114333148048,
12.));
#155159=CARTESIAN_POINT('Ctrl Pts',(-34.7102608784374,63.3355967494171,
12.));
#155160=CARTESIAN_POINT('Ctrl Pts',(-34.7137559997146,63.3598045260053,
12.));
#155161=CARTESIAN_POINT('Ctrl Pts',(-34.7172335909038,63.3840565399208,
12.));
#155162=CARTESIAN_POINT('Ctrl Pts',(-34.7206935779007,63.4083526868836,
12.));
#155163=CARTESIAN_POINT('Ctrl Pts',(-34.7241358869701,63.4326928629795,
12.));
#155164=CARTESIAN_POINT('Ctrl Pts',(-34.7275604447439,63.4570769646569,
12.));
#155165=CARTESIAN_POINT('Ctrl Pts',(-34.7309671782214,63.4815048887165,
12.));
#155166=CARTESIAN_POINT('Ctrl Pts',(-34.7343560147667,63.505976532309,12.));
#155167=CARTESIAN_POINT('Ctrl Pts',(-34.7377268821025,63.5304917929386,
12.));
#155168=CARTESIAN_POINT('Ctrl Pts',(-34.7410797083081,63.5550505684626,
12.));
#155169=CARTESIAN_POINT('Ctrl Pts',(-34.744414421816,63.5796527570871,12.));
#155170=CARTESIAN_POINT('Ctrl Pts',(-34.7477309514136,63.6042982573588,
12.));
#155171=CARTESIAN_POINT('Ctrl Pts',(-34.7510292262406,63.6289869681604,
12.));
#155172=CARTESIAN_POINT('Ctrl Pts',(-34.7543091757833,63.6537187887159,
12.));
#155173=CARTESIAN_POINT('Ctrl Pts',(-34.7575707298713,63.6784936185885,
12.));
#155174=CARTESIAN_POINT('Ctrl Pts',(-34.7608138186759,63.7033113576785,
12.));
#155175=CARTESIAN_POINT('Ctrl Pts',(-34.7640383727101,63.7281719062149,
12.));
#155176=CARTESIAN_POINT('Ctrl Pts',(-34.7672443228275,63.7530751647494,
12.));
#155177=CARTESIAN_POINT('Ctrl Pts',(-34.7704316002171,63.778021034163,12.));
#155178=CARTESIAN_POINT('Ctrl Pts',(-34.7736001363993,63.8030094156639,
12.));
#155179=CARTESIAN_POINT('Ctrl Pts',(-34.7767498632243,63.8280402107856,
12.));
#155180=CARTESIAN_POINT('Ctrl Pts',(-34.7798807128715,63.8531133213793,
12.));
#155181=CARTESIAN_POINT('Ctrl Pts',(-34.7829926178496,63.8782286496062,
12.));
#155182=CARTESIAN_POINT('Ctrl Pts',(-34.7860855109911,63.9033860979435,
12.));
#155183=CARTESIAN_POINT('Ctrl Pts',(-34.7891593254488,63.9285855691845,
12.));
#155184=CARTESIAN_POINT('Ctrl Pts',(-34.7922139946943,63.9538269664366,
12.));
#155185=CARTESIAN_POINT('Ctrl Pts',(-34.7952494525177,63.9791101931162,
12.));
#155186=CARTESIAN_POINT('Ctrl Pts',(-34.7982656330293,64.0044351529402,
12.));
#155187=CARTESIAN_POINT('Ctrl Pts',(-34.8012624706526,64.0298017499294,
12.));
#155188=CARTESIAN_POINT('Ctrl Pts',(-34.8042399001211,64.0552098884095,
12.));
#155189=CARTESIAN_POINT('Ctrl Pts',(-34.8071978564747,64.0806594730085,
12.));
#155190=CARTESIAN_POINT('Ctrl Pts',(-34.8101362750597,64.1061504086515,
12.));
#155191=CARTESIAN_POINT('Ctrl Pts',(-34.8130550915287,64.1316826005506,
12.));
#155192=CARTESIAN_POINT('Ctrl Pts',(-34.8159542418374,64.1572559542086,
12.));
#155193=CARTESIAN_POINT('Ctrl Pts',(-34.8188336622419,64.1828703754236,
12.));
#155194=CARTESIAN_POINT('Ctrl Pts',(-34.8216932892968,64.2085257702884,
12.));
#155195=CARTESIAN_POINT('Ctrl Pts',(-34.8245330598559,64.234222045188,12.));
#155196=CARTESIAN_POINT('Ctrl Pts',(-34.8273529110744,64.2599591067916,
12.));
#155197=CARTESIAN_POINT('Ctrl Pts',(-34.8301527804054,64.285736862052,12.));
#155198=CARTESIAN_POINT('Ctrl Pts',(-34.8329326055919,64.3115552182062,
12.));
#155199=CARTESIAN_POINT('Ctrl Pts',(-34.8356923246618,64.3374140827711,
12.));
#155200=CARTESIAN_POINT('Ctrl Pts',(-34.8384318759248,64.3633133635382,
12.));
#155201=CARTESIAN_POINT('Ctrl Pts',(-34.8411511979702,64.3892529685607,
12.));
#155202=CARTESIAN_POINT('Ctrl Pts',(-34.8438502296664,64.4152328061515,
12.));
#155203=CARTESIAN_POINT('Ctrl Pts',(-34.8465289101621,64.4412527848969,
12.));
#155204=CARTESIAN_POINT('Ctrl Pts',(-34.8491871788895,64.4673128136625,
12.));
#155205=CARTESIAN_POINT('Ctrl Pts',(-34.851824975568,64.4934128015985,12.));
#155206=CARTESIAN_POINT('Ctrl Pts',(-34.8544422402118,64.5195526581407,
12.));
#155207=CARTESIAN_POINT('Ctrl Pts',(-34.857038913134,64.5457322930088,12.));
#155208=CARTESIAN_POINT('Ctrl Pts',(-34.8596149349257,64.5719516161927,
12.));
#155209=CARTESIAN_POINT('Ctrl Pts',(-34.8621702464401,64.5982105379383,
12.));
#155210=CARTESIAN_POINT('Ctrl Pts',(-34.8647047887774,64.6245089687277,
12.));
#155211=CARTESIAN_POINT('Ctrl Pts',(-34.867218503272,64.6508468192599,12.));
#155212=CARTESIAN_POINT('Ctrl Pts',(-34.869711331479,64.6772240004228,12.));
#155213=CARTESIAN_POINT('Ctrl Pts',(-34.8721832151974,64.7036404233306,
12.));
#155214=CARTESIAN_POINT('Ctrl Pts',(-34.8746340964971,64.7300959993653,
12.));
#155215=CARTESIAN_POINT('Ctrl Pts',(-34.8770639177493,64.7565906402151,
12.));
#155216=CARTESIAN_POINT('Ctrl Pts',(-34.8794726216513,64.7831242579028,
12.));
#155217=CARTESIAN_POINT('Ctrl Pts',(-34.881860151273,64.8096967648307,12.));
#155218=CARTESIAN_POINT('Ctrl Pts',(-34.8842264500188,64.8363080737377,
12.));
#155219=CARTESIAN_POINT('Ctrl Pts',(-34.8865714615436,64.8629580976063,
12.));
#155220=CARTESIAN_POINT('Ctrl Pts',(-34.888895129681,64.8896467495757,12.));
#155221=CARTESIAN_POINT('Ctrl Pts',(-34.8911973983785,64.9163739428605,
12.));
#155222=CARTESIAN_POINT('Ctrl Pts',(-34.8934782116095,64.9431395906337,
12.));
#155223=CARTESIAN_POINT('Ctrl Pts',(-34.8957375133697,64.9699436060169,
12.));
#155224=CARTESIAN_POINT('Ctrl Pts',(-34.8979752478616,64.9967859023212,
12.));
#155225=CARTESIAN_POINT('Ctrl Pts',(-34.9001913596416,65.0236663932328,
12.));
#155226=CARTESIAN_POINT('Ctrl Pts',(-34.9023857937865,65.0505849930171,
12.));
#155227=CARTESIAN_POINT('Ctrl Pts',(-34.9045584960509,65.0775416167085,
12.));
#155228=CARTESIAN_POINT('Ctrl Pts',(-34.9067094130399,65.1045361803121,
12.));
#155229=CARTESIAN_POINT('Ctrl Pts',(-34.9088384918336,65.1315686003516,
12.));
#155230=CARTESIAN_POINT('Ctrl Pts',(-34.9109456796213,65.1586387934241,
12.));
#155231=CARTESIAN_POINT('Ctrl Pts',(-34.9130309233022,65.1857466757092,
12.));
#155232=CARTESIAN_POINT('Ctrl Pts',(-34.9150941691747,65.2128921625823,
12.));
#155233=CARTESIAN_POINT('Ctrl Pts',(-34.9171353624113,65.2400751679549,
12.));
#155234=CARTESIAN_POINT('Ctrl Pts',(-34.9191544474872,65.2672956048069,
12.));
#155235=CARTESIAN_POINT('Ctrl Pts',(-34.9211513691355,65.2945533863761,
12.));
#155236=CARTESIAN_POINT('Ctrl Pts',(-34.9231260731831,65.321848427191,12.));
#155237=CARTESIAN_POINT('Ctrl Pts',(-34.9250785073477,65.3491806440537,
12.));
#155238=CARTESIAN_POINT('Ctrl Pts',(-34.9270086222731,65.3765499573077,
12.));
#155239=CARTESIAN_POINT('Ctrl Pts',(-34.9289163717747,65.4039562911352,
12.));
#155240=CARTESIAN_POINT('Ctrl Pts',(-34.9305324724445,65.4274804996589,
12.));
#155241=CARTESIAN_POINT('Ctrl Pts',(-34.931759381316,65.4455359575244,12.));
#155242=CARTESIAN_POINT('Ctrl Pts',(-34.9326070346645,65.4581063193883,
12.));
#155243=CARTESIAN_POINT('Ctrl Pts',(-34.9330820191535,65.465180801081,12.));
#155244=CARTESIAN_POINT('Ctrl Pts',(-34.933187552314,65.4667541478384,12.));
#155245=CARTESIAN_POINT('',(-34.2579614092497,61.0441813777723,0.));
#155246=CARTESIAN_POINT('',(-34.2579614092497,61.0441813777723,0.));
#155247=CARTESIAN_POINT('Ctrl Pts',(-34.933187552314,65.4667541478384,0.));
#155248=CARTESIAN_POINT('Ctrl Pts',(-34.9330820191535,65.465180801081,0.));
#155249=CARTESIAN_POINT('Ctrl Pts',(-34.9326070346645,65.4581063193883,
0.));
#155250=CARTESIAN_POINT('Ctrl Pts',(-34.931759381316,65.4455359575244,0.));
#155251=CARTESIAN_POINT('Ctrl Pts',(-34.9305324724445,65.4274804996589,
0.));
#155252=CARTESIAN_POINT('Ctrl Pts',(-34.9289163717747,65.4039562911352,
0.));
#155253=CARTESIAN_POINT('Ctrl Pts',(-34.9270086222731,65.3765499573077,
0.));
#155254=CARTESIAN_POINT('Ctrl Pts',(-34.9250785073477,65.3491806440537,
0.));
#155255=CARTESIAN_POINT('Ctrl Pts',(-34.9231260731831,65.321848427191,0.));
#155256=CARTESIAN_POINT('Ctrl Pts',(-34.9211513691355,65.2945533863761,
0.));
#155257=CARTESIAN_POINT('Ctrl Pts',(-34.9191544474872,65.2672956048069,
0.));
#155258=CARTESIAN_POINT('Ctrl Pts',(-34.9171353624113,65.2400751679549,
0.));
#155259=CARTESIAN_POINT('Ctrl Pts',(-34.9150941691747,65.2128921625823,
0.));
#155260=CARTESIAN_POINT('Ctrl Pts',(-34.9130309233022,65.1857466757092,
0.));
#155261=CARTESIAN_POINT('Ctrl Pts',(-34.9109456796213,65.1586387934241,
0.));
#155262=CARTESIAN_POINT('Ctrl Pts',(-34.9088384918336,65.1315686003516,
0.));
#155263=CARTESIAN_POINT('Ctrl Pts',(-34.9067094130399,65.1045361803121,
0.));
#155264=CARTESIAN_POINT('Ctrl Pts',(-34.9045584960509,65.0775416167085,
0.));
#155265=CARTESIAN_POINT('Ctrl Pts',(-34.9023857937865,65.0505849930171,
0.));
#155266=CARTESIAN_POINT('Ctrl Pts',(-34.9001913596416,65.0236663932328,
0.));
#155267=CARTESIAN_POINT('Ctrl Pts',(-34.8979752478616,64.9967859023212,
0.));
#155268=CARTESIAN_POINT('Ctrl Pts',(-34.8957375133697,64.9699436060169,
0.));
#155269=CARTESIAN_POINT('Ctrl Pts',(-34.8934782116095,64.9431395906337,
0.));
#155270=CARTESIAN_POINT('Ctrl Pts',(-34.8911973983785,64.9163739428605,
0.));
#155271=CARTESIAN_POINT('Ctrl Pts',(-34.888895129681,64.8896467495757,0.));
#155272=CARTESIAN_POINT('Ctrl Pts',(-34.8865714615436,64.8629580976063,
0.));
#155273=CARTESIAN_POINT('Ctrl Pts',(-34.8842264500188,64.8363080737377,
0.));
#155274=CARTESIAN_POINT('Ctrl Pts',(-34.881860151273,64.8096967648307,0.));
#155275=CARTESIAN_POINT('Ctrl Pts',(-34.8794726216513,64.7831242579028,
0.));
#155276=CARTESIAN_POINT('Ctrl Pts',(-34.8770639177493,64.7565906402151,
0.));
#155277=CARTESIAN_POINT('Ctrl Pts',(-34.8746340964971,64.7300959993653,
0.));
#155278=CARTESIAN_POINT('Ctrl Pts',(-34.8721832151974,64.7036404233306,
0.));
#155279=CARTESIAN_POINT('Ctrl Pts',(-34.869711331479,64.6772240004228,0.));
#155280=CARTESIAN_POINT('Ctrl Pts',(-34.867218503272,64.6508468192599,0.));
#155281=CARTESIAN_POINT('Ctrl Pts',(-34.8647047887774,64.6245089687277,
0.));
#155282=CARTESIAN_POINT('Ctrl Pts',(-34.8621702464401,64.5982105379383,
0.));
#155283=CARTESIAN_POINT('Ctrl Pts',(-34.8596149349257,64.5719516161927,
0.));
#155284=CARTESIAN_POINT('Ctrl Pts',(-34.857038913134,64.5457322930088,0.));
#155285=CARTESIAN_POINT('Ctrl Pts',(-34.8544422402118,64.5195526581407,
0.));
#155286=CARTESIAN_POINT('Ctrl Pts',(-34.851824975568,64.4934128015985,0.));
#155287=CARTESIAN_POINT('Ctrl Pts',(-34.8491871788895,64.4673128136625,
0.));
#155288=CARTESIAN_POINT('Ctrl Pts',(-34.8465289101621,64.4412527848969,
0.));
#155289=CARTESIAN_POINT('Ctrl Pts',(-34.8438502296664,64.4152328061515,
0.));
#155290=CARTESIAN_POINT('Ctrl Pts',(-34.8411511979702,64.3892529685607,
0.));
#155291=CARTESIAN_POINT('Ctrl Pts',(-34.8384318759248,64.3633133635382,
0.));
#155292=CARTESIAN_POINT('Ctrl Pts',(-34.8356923246618,64.3374140827711,
0.));
#155293=CARTESIAN_POINT('Ctrl Pts',(-34.8329326055919,64.3115552182062,
0.));
#155294=CARTESIAN_POINT('Ctrl Pts',(-34.8301527804054,64.285736862052,0.));
#155295=CARTESIAN_POINT('Ctrl Pts',(-34.8273529110744,64.2599591067916,
0.));
#155296=CARTESIAN_POINT('Ctrl Pts',(-34.8245330598559,64.234222045188,0.));
#155297=CARTESIAN_POINT('Ctrl Pts',(-34.8216932892968,64.2085257702884,
0.));
#155298=CARTESIAN_POINT('Ctrl Pts',(-34.8188336622419,64.1828703754236,
0.));
#155299=CARTESIAN_POINT('Ctrl Pts',(-34.8159542418374,64.1572559542086,
0.));
#155300=CARTESIAN_POINT('Ctrl Pts',(-34.8130550915287,64.1316826005506,
0.));
#155301=CARTESIAN_POINT('Ctrl Pts',(-34.8101362750597,64.1061504086515,
0.));
#155302=CARTESIAN_POINT('Ctrl Pts',(-34.8071978564747,64.0806594730085,
0.));
#155303=CARTESIAN_POINT('Ctrl Pts',(-34.8042399001211,64.0552098884095,
0.));
#155304=CARTESIAN_POINT('Ctrl Pts',(-34.8012624706526,64.0298017499294,
0.));
#155305=CARTESIAN_POINT('Ctrl Pts',(-34.7982656330293,64.0044351529402,
0.));
#155306=CARTESIAN_POINT('Ctrl Pts',(-34.7952494525177,63.9791101931162,
0.));
#155307=CARTESIAN_POINT('Ctrl Pts',(-34.7922139946943,63.9538269664366,
0.));
#155308=CARTESIAN_POINT('Ctrl Pts',(-34.7891593254488,63.9285855691845,
0.));
#155309=CARTESIAN_POINT('Ctrl Pts',(-34.7860855109911,63.9033860979435,
0.));
#155310=CARTESIAN_POINT('Ctrl Pts',(-34.7829926178496,63.8782286496062,
0.));
#155311=CARTESIAN_POINT('Ctrl Pts',(-34.7798807128715,63.8531133213793,
0.));
#155312=CARTESIAN_POINT('Ctrl Pts',(-34.7767498632243,63.8280402107856,
0.));
#155313=CARTESIAN_POINT('Ctrl Pts',(-34.7736001363993,63.8030094156639,
0.));
#155314=CARTESIAN_POINT('Ctrl Pts',(-34.7704316002171,63.778021034163,0.));
#155315=CARTESIAN_POINT('Ctrl Pts',(-34.7672443228275,63.7530751647494,
0.));
#155316=CARTESIAN_POINT('Ctrl Pts',(-34.7640383727101,63.7281719062149,
0.));
#155317=CARTESIAN_POINT('Ctrl Pts',(-34.7608138186759,63.7033113576785,
0.));
#155318=CARTESIAN_POINT('Ctrl Pts',(-34.7575707298713,63.6784936185885,
0.));
#155319=CARTESIAN_POINT('Ctrl Pts',(-34.7543091757833,63.6537187887159,
0.));
#155320=CARTESIAN_POINT('Ctrl Pts',(-34.7510292262406,63.6289869681604,
0.));
#155321=CARTESIAN_POINT('Ctrl Pts',(-34.7477309514136,63.6042982573588,
0.));
#155322=CARTESIAN_POINT('Ctrl Pts',(-34.744414421816,63.5796527570871,0.));
#155323=CARTESIAN_POINT('Ctrl Pts',(-34.7410797083081,63.5550505684626,
0.));
#155324=CARTESIAN_POINT('Ctrl Pts',(-34.7377268821025,63.5304917929386,
0.));
#155325=CARTESIAN_POINT('Ctrl Pts',(-34.7343560147667,63.505976532309,0.));
#155326=CARTESIAN_POINT('Ctrl Pts',(-34.7309671782214,63.4815048887165,
0.));
#155327=CARTESIAN_POINT('Ctrl Pts',(-34.7275604447439,63.4570769646569,
0.));
#155328=CARTESIAN_POINT('Ctrl Pts',(-34.7241358869701,63.4326928629795,
0.));
#155329=CARTESIAN_POINT('Ctrl Pts',(-34.7206935779007,63.4083526868836,
0.));
#155330=CARTESIAN_POINT('Ctrl Pts',(-34.7172335909038,63.3840565399208,
0.));
#155331=CARTESIAN_POINT('Ctrl Pts',(-34.7137559997146,63.3598045260053,
0.));
#155332=CARTESIAN_POINT('Ctrl Pts',(-34.7102608784374,63.3355967494171,
0.));
#155333=CARTESIAN_POINT('Ctrl Pts',(-34.7067483015491,63.3114333148048,
0.));
#155334=CARTESIAN_POINT('Ctrl Pts',(-34.703218343904,63.2873143271807,0.));
#155335=CARTESIAN_POINT('Ctrl Pts',(-34.6996710807378,63.2632398919225,
0.));
#155336=CARTESIAN_POINT('Ctrl Pts',(-34.6961065876666,63.2392101147847,
0.));
#155337=CARTESIAN_POINT('Ctrl Pts',(-34.6925249406897,63.2152251019012,
0.));
#155338=CARTESIAN_POINT('Ctrl Pts',(-34.6889262161924,63.1912849597887,
0.));
#155339=CARTESIAN_POINT('Ctrl Pts',(-34.6853104909518,63.1673897953429,
0.));
#155340=CARTESIAN_POINT('Ctrl Pts',(-34.6816778421402,63.1435397158388,
0.));
#155341=CARTESIAN_POINT('Ctrl Pts',(-34.6780283473252,63.119734828943,0.));
#155342=CARTESIAN_POINT('Ctrl Pts',(-34.674362084472,63.0959752427168,0.));
#155343=CARTESIAN_POINT('Ctrl Pts',(-34.670679131947,63.0722610656194,0.));
#155344=CARTESIAN_POINT('Ctrl Pts',(-34.6669795685228,63.0485924065045,
0.));
#155345=CARTESIAN_POINT('Ctrl Pts',(-34.6632634733824,63.0249693746208,
0.));
#155346=CARTESIAN_POINT('Ctrl Pts',(-34.6595309261191,63.0013920796235,
0.));
#155347=CARTESIAN_POINT('Ctrl Pts',(-34.6557820067393,62.9778606315783,
0.));
#155348=CARTESIAN_POINT('Ctrl Pts',(-34.6520167956655,62.9543751409645,
0.));
#155349=CARTESIAN_POINT('Ctrl Pts',(-34.6482353737424,62.9309357186717,
0.));
#155350=CARTESIAN_POINT('Ctrl Pts',(-34.6444378222411,62.9075424760015,
0.));
#155351=CARTESIAN_POINT('Ctrl Pts',(-34.6406242228592,62.8841955246794,
0.));
#155352=CARTESIAN_POINT('Ctrl Pts',(-34.6367946577235,62.8608949768571,
0.));
#155353=CARTESIAN_POINT('Ctrl Pts',(-34.6329492093935,62.8376409451175,
0.));
#155354=CARTESIAN_POINT('Ctrl Pts',(-34.6290879608673,62.8144335424697,
0.));
#155355=CARTESIAN_POINT('Ctrl Pts',(-34.6252109955853,62.7912728823518,
0.));
#155356=CARTESIAN_POINT('Ctrl Pts',(-34.6213183974317,62.7681590786429,
0.));
#155357=CARTESIAN_POINT('Ctrl Pts',(-34.6174102507375,62.7450922456676,
0.));
#155358=CARTESIAN_POINT('Ctrl Pts',(-34.6134866402837,62.7220724981994,
0.));
#155359=CARTESIAN_POINT('Ctrl Pts',(-34.6095476513077,62.6990999514563,
0.));
#155360=CARTESIAN_POINT('Ctrl Pts',(-34.6055933695069,62.6761747211037,
0.));
#155361=CARTESIAN_POINT('Ctrl Pts',(-34.6016238810399,62.6532969232657,
0.));
#155362=CARTESIAN_POINT('Ctrl Pts',(-34.5976392725296,62.6304666745306,
0.));
#155363=CARTESIAN_POINT('Ctrl Pts',(-34.5936396310679,62.6076840919536,
0.));
#155364=CARTESIAN_POINT('Ctrl Pts',(-34.5896250442216,62.5849492930533,
0.));
#155365=CARTESIAN_POINT('Ctrl Pts',(-34.5855956000363,62.562262395816,0.));
#155366=CARTESIAN_POINT('Ctrl Pts',(-34.5815513870377,62.5396235187079,
0.));
#155367=CARTESIAN_POINT('Ctrl Pts',(-34.5774924942355,62.5170327806781,
0.));
#155368=CARTESIAN_POINT('Ctrl Pts',(-34.5734190111272,62.4944903011628,
0.));
#155369=CARTESIAN_POINT('Ctrl Pts',(-34.5693310277051,62.4719962000808,
0.));
#155370=CARTESIAN_POINT('Ctrl Pts',(-34.5652286344593,62.4495505978393,
0.));
#155371=CARTESIAN_POINT('Ctrl Pts',(-34.5611119223798,62.4271536153459,
0.));
#155372=CARTESIAN_POINT('Ctrl Pts',(-34.5569809829613,62.4048053740127,
0.));
#155373=CARTESIAN_POINT('Ctrl Pts',(-34.5528359082075,62.3825059957601,
0.));
#155374=CARTESIAN_POINT('Ctrl Pts',(-34.5486767906384,62.3602556030127,
0.));
#155375=CARTESIAN_POINT('Ctrl Pts',(-34.5445037232936,62.338054318708,0.));
#155376=CARTESIAN_POINT('Ctrl Pts',(-34.5403167997337,62.3159022663058,
0.));
#155377=CARTESIAN_POINT('Ctrl Pts',(-34.5361161140449,62.2937995697925,
0.));
#155378=CARTESIAN_POINT('Ctrl Pts',(-34.5319017608433,62.2717463536827,
0.));
#155379=CARTESIAN_POINT('Ctrl Pts',(-34.5276738352808,62.2497427430135,
0.));
#155380=CARTESIAN_POINT('Ctrl Pts',(-34.523432433049,62.2277888633576,0.));
#155381=CARTESIAN_POINT('Ctrl Pts',(-34.5191776503842,62.2058848408347,
0.));
#155382=CARTESIAN_POINT('Ctrl Pts',(-34.514909584073,62.1840308021171,0.));
#155383=CARTESIAN_POINT('Ctrl Pts',(-34.5106283314594,62.1622268744336,
0.));
#155384=CARTESIAN_POINT('Ctrl Pts',(-34.5063339904533,62.1404731855686,
0.));
#155385=CARTESIAN_POINT('Ctrl Pts',(-34.5020266595292,62.1187698638705,
0.));
#155386=CARTESIAN_POINT('Ctrl Pts',(-34.4977064377281,62.0971170382565,
0.));
#155387=CARTESIAN_POINT('Ctrl Pts',(-34.4933734246592,62.0755148382136,
0.));
#155388=CARTESIAN_POINT('Ctrl Pts',(-34.4890277205042,62.0539633937944,
0.));
#155389=CARTESIAN_POINT('Ctrl Pts',(-34.4846694260205,62.0324628356152,
0.));
#155390=CARTESIAN_POINT('Ctrl Pts',(-34.4802986425535,62.0110132948807,
0.));
#155391=CARTESIAN_POINT('Ctrl Pts',(-34.4759154720477,61.9896149034009,
0.));
#155392=CARTESIAN_POINT('Ctrl Pts',(-34.4715200170589,61.9682677936048,
0.));
#155393=CARTESIAN_POINT('Ctrl Pts',(-34.4671123807706,61.9469720985512,
0.));
#155394=CARTESIAN_POINT('Ctrl Pts',(-34.462692666996,61.9257279519283,0.));
#155395=CARTESIAN_POINT('Ctrl Pts',(-34.4582609801625,61.9045354880424,
0.));
#155396=CARTESIAN_POINT('Ctrl Pts',(-34.4538174253009,61.883394841802,0.));
#155397=CARTESIAN_POINT('Ctrl Pts',(-34.4493621080367,61.862306148703,0.));
#155398=CARTESIAN_POINT('Ctrl Pts',(-34.4448951345753,61.8412695447951,
0.));
#155399=CARTESIAN_POINT('Ctrl Pts',(-34.4404166117313,61.8202851667247,
0.));
#155400=CARTESIAN_POINT('Ctrl Pts',(-34.4359266469757,61.7993531518052,
0.));
#155401=CARTESIAN_POINT('Ctrl Pts',(-34.4314253484791,61.7784736380727,
0.));
#155402=CARTESIAN_POINT('Ctrl Pts',(-34.4269128251569,61.7576467643419,
0.));
#155403=CARTESIAN_POINT('Ctrl Pts',(-34.4223891867166,61.7368726702573,
0.));
#155404=CARTESIAN_POINT('Ctrl Pts',(-34.4178545435753,61.7161514961892,
0.));
#155405=CARTESIAN_POINT('Ctrl Pts',(-34.4133090067696,61.6954833831157,
0.));
#155406=CARTESIAN_POINT('Ctrl Pts',(-34.4087526878815,61.674868472521,0.));
#155407=CARTESIAN_POINT('Ctrl Pts',(-34.4041856989328,61.6543069062436,
0.));
#155408=CARTESIAN_POINT('Ctrl Pts',(-34.399608152377,61.6337988264586,0.));
#155409=CARTESIAN_POINT('Ctrl Pts',(-34.3950201613446,61.6133443760168,
0.));
#155410=CARTESIAN_POINT('Ctrl Pts',(-34.3904218398642,61.5929436987419,
0.));
#155411=CARTESIAN_POINT('Ctrl Pts',(-34.3858133030511,61.5725969396817,
0.));
#155412=CARTESIAN_POINT('Ctrl Pts',(-34.3811946674179,61.5523042455127,
0.));
#155413=CARTESIAN_POINT('Ctrl Pts',(-34.3765660506659,61.5320657642601,
0.));
#155414=CARTESIAN_POINT('Ctrl Pts',(-34.3719275711179,61.511881644541,0.));
#155415=CARTESIAN_POINT('Ctrl Pts',(-34.3672793472464,61.4917520349276,
0.));
#155416=CARTESIAN_POINT('Ctrl Pts',(-34.3626214971903,61.4716770832924,
0.));
#155417=CARTESIAN_POINT('Ctrl Pts',(-34.357954138202,61.4516569360499,0.));
#155418=CARTESIAN_POINT('Ctrl Pts',(-34.3532773877112,61.4316917395959,
0.));
#155419=CARTESIAN_POINT('Ctrl Pts',(-34.3485913645991,61.4117816420251,
0.));
#155420=CARTESIAN_POINT('Ctrl Pts',(-34.34389619024,61.3919267945293,0.));
#155421=CARTESIAN_POINT('Ctrl Pts',(-34.339191990012,61.3721273534222,0.));
#155422=CARTESIAN_POINT('Ctrl Pts',(-34.3344788934337,61.3523834803144,
0.));
#155423=CARTESIAN_POINT('Ctrl Pts',(-34.3297570310126,61.3326953378817,
0.));
#155424=CARTESIAN_POINT('Ctrl Pts',(-34.3250265314761,61.3130630861375,
0.));
#155425=CARTESIAN_POINT('Ctrl Pts',(-34.3202875193629,61.2934868791875,
0.));
#155426=CARTESIAN_POINT('Ctrl Pts',(-34.3155401111776,61.2739668600415,
0.));
#155427=CARTESIAN_POINT('Ctrl Pts',(-34.3107844191081,61.2545031656196,
0.));
#155428=CARTESIAN_POINT('Ctrl Pts',(-34.3060205584093,61.2350959366987,
0.));
#155429=CARTESIAN_POINT('Ctrl Pts',(-34.3012486533474,61.2157453259107,
0.));
#155430=CARTESIAN_POINT('Ctrl Pts',(-34.296468844362,61.1964515073823,0.));
#155431=CARTESIAN_POINT('Ctrl Pts',(-34.2916812929675,61.1772146833083,
0.));
#155432=CARTESIAN_POINT('Ctrl Pts',(-34.2868861666301,61.15803506354,0.));
#155433=CARTESIAN_POINT('Ctrl Pts',(-34.2820836244425,61.1389128461815,
0.));
#155434=CARTESIAN_POINT('Ctrl Pts',(-34.2772738038812,61.119848199783,0.));
#155435=CARTESIAN_POINT('Ctrl Pts',(-34.2724568037374,61.100841240023,0.));
#155436=CARTESIAN_POINT('Ctrl Pts',(-34.2676326825846,61.0818920286644,
0.));
#155437=CARTESIAN_POINT('Ctrl Pts',(-34.2637677132139,61.0667788793594,
0.));
#155438=CARTESIAN_POINT('Ctrl Pts',(-34.2608658001761,61.0554700177206,
0.));
#155439=CARTESIAN_POINT('Ctrl Pts',(-34.2589297755482,61.0479423318803,
0.));
#155440=CARTESIAN_POINT('Ctrl Pts',(-34.2579614092497,61.0441813777723,
0.));
#155441=CARTESIAN_POINT('Ctrl Pts',(-29.0861280018229,68.5875145916629,
0.));
#155442=CARTESIAN_POINT('Ctrl Pts',(-29.0861280018229,68.5875145916629,
12.));
#155443=CARTESIAN_POINT('Ctrl Pts',(-29.0863005247839,68.5819214834737,
0.));
#155444=CARTESIAN_POINT('Ctrl Pts',(-29.0863005247839,68.5819214834737,
12.));
#155445=CARTESIAN_POINT('Ctrl Pts',(-29.0866429722093,68.5707386600636,
0.));
#155446=CARTESIAN_POINT('Ctrl Pts',(-29.0866429722093,68.5707386600636,
12.));
#155447=CARTESIAN_POINT('Ctrl Pts',(-29.0871488478589,68.5539746038542,
0.));
#155448=CARTESIAN_POINT('Ctrl Pts',(-29.0871488478589,68.5539746038542,
12.));
#155449=CARTESIAN_POINT('Ctrl Pts',(-29.0878077571086,68.5316428875424,
0.));
#155450=CARTESIAN_POINT('Ctrl Pts',(-29.0878077571086,68.5316428875424,
12.));
#155451=CARTESIAN_POINT('Ctrl Pts',(-29.0886054060563,68.5037621824171,
0.));
#155452=CARTESIAN_POINT('Ctrl Pts',(-29.0886054060563,68.5037621824171,
12.));
#155453=CARTESIAN_POINT('Ctrl Pts',(-29.0893770688944,68.4759154367939,
0.));
#155454=CARTESIAN_POINT('Ctrl Pts',(-29.0893770688944,68.4759154367939,
12.));
#155455=CARTESIAN_POINT('Ctrl Pts',(-29.0901227535307,68.4481026830931,
0.));
#155456=CARTESIAN_POINT('Ctrl Pts',(-29.0901227535307,68.4481026830931,
12.));
#155457=CARTESIAN_POINT('Ctrl Pts',(-29.090842477089,68.4203239694612,0.));
#155458=CARTESIAN_POINT('Ctrl Pts',(-29.090842477089,68.4203239694612,12.));
#155459=CARTESIAN_POINT('Ctrl Pts',(-29.0915362699455,68.3925793637995,
0.));
#155460=CARTESIAN_POINT('Ctrl Pts',(-29.0915362699455,68.3925793637995,
12.));
#155461=CARTESIAN_POINT('Ctrl Pts',(-29.0922041749294,68.364868951893,0.));
#155462=CARTESIAN_POINT('Ctrl Pts',(-29.0922041749294,68.364868951893,12.));
#155463=CARTESIAN_POINT('Ctrl Pts',(-29.0928462428145,68.3371928310161,
0.));
#155464=CARTESIAN_POINT('Ctrl Pts',(-29.0928462428145,68.3371928310161,
12.));
#155465=CARTESIAN_POINT('Ctrl Pts',(-29.0934625288409,68.3095511047769,
0.));
#155466=CARTESIAN_POINT('Ctrl Pts',(-29.0934625288409,68.3095511047769,
12.));
#155467=CARTESIAN_POINT('Ctrl Pts',(-29.0940530889149,68.2819438775953,
0.));
#155468=CARTESIAN_POINT('Ctrl Pts',(-29.0940530889149,68.2819438775953,
12.));
#155469=CARTESIAN_POINT('Ctrl Pts',(-29.0946179757167,68.2543712489906,
0.));
#155470=CARTESIAN_POINT('Ctrl Pts',(-29.0946179757167,68.2543712489906,
12.));
#155471=CARTESIAN_POINT('Ctrl Pts',(-29.0951572355397,68.2268333089617,
0.));
#155472=CARTESIAN_POINT('Ctrl Pts',(-29.0951572355397,68.2268333089617,
12.));
#155473=CARTESIAN_POINT('Ctrl Pts',(-29.0956709104627,68.1993301412061,
0.));
#155474=CARTESIAN_POINT('Ctrl Pts',(-29.0956709104627,68.1993301412061,
12.));
#155475=CARTESIAN_POINT('Ctrl Pts',(-29.0961590399046,68.1718618254281,
0.));
#155476=CARTESIAN_POINT('Ctrl Pts',(-29.0961590399046,68.1718618254281,
12.));
#155477=CARTESIAN_POINT('Ctrl Pts',(-29.0966216624743,68.1444284400742,
0.));
#155478=CARTESIAN_POINT('Ctrl Pts',(-29.0966216624743,68.1444284400742,
12.));
#155479=CARTESIAN_POINT('Ctrl Pts',(-29.0970588175728,68.1170300646987,
0.));
#155480=CARTESIAN_POINT('Ctrl Pts',(-29.0970588175728,68.1170300646987,
12.));
#155481=CARTESIAN_POINT('Ctrl Pts',(-29.0974705474259,68.0896667829567,
0.));
#155482=CARTESIAN_POINT('Ctrl Pts',(-29.0974705474259,68.0896667829567,
12.));
#155483=CARTESIAN_POINT('Ctrl Pts',(-29.0978568968657,68.0623386822863,
0.));
#155484=CARTESIAN_POINT('Ctrl Pts',(-29.0978568968657,68.0623386822863,
12.));
#155485=CARTESIAN_POINT('Ctrl Pts',(-29.0982179124097,68.0350458525551,
0.));
#155486=CARTESIAN_POINT('Ctrl Pts',(-29.0982179124097,68.0350458525551,
12.));
#155487=CARTESIAN_POINT('Ctrl Pts',(-29.0985536415531,68.0077883850121,
0.));
#155488=CARTESIAN_POINT('Ctrl Pts',(-29.0985536415531,68.0077883850121,
12.));
#155489=CARTESIAN_POINT('Ctrl Pts',(-29.0988641320247,67.9805663711855,
0.));
#155490=CARTESIAN_POINT('Ctrl Pts',(-29.0988641320247,67.9805663711855,
12.));
#155491=CARTESIAN_POINT('Ctrl Pts',(-29.0991494309404,67.9533799016148,
0.));
#155492=CARTESIAN_POINT('Ctrl Pts',(-29.0991494309404,67.9533799016148,
12.));
#155493=CARTESIAN_POINT('Ctrl Pts',(-29.099409584422,67.9262290652829,0.));
#155494=CARTESIAN_POINT('Ctrl Pts',(-29.099409584422,67.9262290652829,12.));
#155495=CARTESIAN_POINT('Ctrl Pts',(-29.0996446380626,67.8991139503193,
0.));
#155496=CARTESIAN_POINT('Ctrl Pts',(-29.0996446380626,67.8991139503193,
12.));
#155497=CARTESIAN_POINT('Ctrl Pts',(-29.0998546372032,67.8720346444124,
0.));
#155498=CARTESIAN_POINT('Ctrl Pts',(-29.0998546372032,67.8720346444124,
12.));
#155499=CARTESIAN_POINT('Ctrl Pts',(-29.1000396272867,67.8449912353329,
0.));
#155500=CARTESIAN_POINT('Ctrl Pts',(-29.1000396272867,67.8449912353329,
12.));
#155501=CARTESIAN_POINT('Ctrl Pts',(-29.1001996541842,67.8179838114099,
0.));
#155502=CARTESIAN_POINT('Ctrl Pts',(-29.1001996541842,67.8179838114099,
12.));
#155503=CARTESIAN_POINT('Ctrl Pts',(-29.1003347645294,67.7910124620135,
0.));
#155504=CARTESIAN_POINT('Ctrl Pts',(-29.1003347645294,67.7910124620135,
12.));
#155505=CARTESIAN_POINT('Ctrl Pts',(-29.1004450055643,67.7640772773387,
0.));
#155506=CARTESIAN_POINT('Ctrl Pts',(-29.1004450055643,67.7640772773387,
12.));
#155507=CARTESIAN_POINT('Ctrl Pts',(-29.1005304249987,67.7371783482035,
0.));
#155508=CARTESIAN_POINT('Ctrl Pts',(-29.1005304249987,67.7371783482035,
12.));
#155509=CARTESIAN_POINT('Ctrl Pts',(-29.1005910708624,67.7103157658296,
0.));
#155510=CARTESIAN_POINT('Ctrl Pts',(-29.1005910708624,67.7103157658296,
12.));
#155511=CARTESIAN_POINT('Ctrl Pts',(-29.1006269913747,67.6834896216461,
0.));
#155512=CARTESIAN_POINT('Ctrl Pts',(-29.1006269913747,67.6834896216461,
12.));
#155513=CARTESIAN_POINT('Ctrl Pts',(-29.1006382347814,67.6567000070326,
0.));
#155514=CARTESIAN_POINT('Ctrl Pts',(-29.1006382347814,67.6567000070326,
12.));
#155515=CARTESIAN_POINT('Ctrl Pts',(-29.100624849358,67.6299470133295,0.));
#155516=CARTESIAN_POINT('Ctrl Pts',(-29.100624849358,67.6299470133295,12.));
#155517=CARTESIAN_POINT('Ctrl Pts',(-29.1005868834866,67.6032307319623,
0.));
#155518=CARTESIAN_POINT('Ctrl Pts',(-29.1005868834866,67.6032307319623,
12.));
#155519=CARTESIAN_POINT('Ctrl Pts',(-29.1005243857139,67.5765512545281,
0.));
#155520=CARTESIAN_POINT('Ctrl Pts',(-29.1005243857139,67.5765512545281,
12.));
#155521=CARTESIAN_POINT('Ctrl Pts',(-29.1004374048148,67.5499086728888,
0.));
#155522=CARTESIAN_POINT('Ctrl Pts',(-29.1004374048148,67.5499086728888,
12.));
#155523=CARTESIAN_POINT('Ctrl Pts',(-29.1003259898682,67.5233030792704,
0.));
#155524=CARTESIAN_POINT('Ctrl Pts',(-29.1003259898682,67.5233030792704,
12.));
#155525=CARTESIAN_POINT('Ctrl Pts',(-29.1001901902909,67.4967345663096,
0.));
#155526=CARTESIAN_POINT('Ctrl Pts',(-29.1001901902909,67.4967345663096,
12.));
#155527=CARTESIAN_POINT('Ctrl Pts',(-29.1000300557955,67.4702032270048,
0.));
#155528=CARTESIAN_POINT('Ctrl Pts',(-29.1000300557955,67.4702032270048,
12.));
#155529=CARTESIAN_POINT('Ctrl Pts',(-29.0998456363683,67.4437091546859,
0.));
#155530=CARTESIAN_POINT('Ctrl Pts',(-29.0998456363683,67.4437091546859,
12.));
#155531=CARTESIAN_POINT('Ctrl Pts',(-29.0996369822418,67.4172524429727,
0.));
#155532=CARTESIAN_POINT('Ctrl Pts',(-29.0996369822418,67.4172524429727,
12.));
#155533=CARTESIAN_POINT('Ctrl Pts',(-29.0994041438719,67.3908331857323,
0.));
#155534=CARTESIAN_POINT('Ctrl Pts',(-29.0994041438719,67.3908331857323,
12.));
#155535=CARTESIAN_POINT('Ctrl Pts',(-29.0991471719176,67.3644514770387,
0.));
#155536=CARTESIAN_POINT('Ctrl Pts',(-29.0991471719176,67.3644514770387,
12.));
#155537=CARTESIAN_POINT('Ctrl Pts',(-29.0988661172531,67.3381074112027,
0.));
#155538=CARTESIAN_POINT('Ctrl Pts',(-29.0988661172531,67.3381074112027,
12.));
#155539=CARTESIAN_POINT('Ctrl Pts',(-29.0985610309771,67.311801082792,0.));
#155540=CARTESIAN_POINT('Ctrl Pts',(-29.0985610309771,67.311801082792,12.));
#155541=CARTESIAN_POINT('Ctrl Pts',(-29.0982319644277,67.2855325866517,
0.));
#155542=CARTESIAN_POINT('Ctrl Pts',(-29.0982319644277,67.2855325866517,
12.));
#155543=CARTESIAN_POINT('Ctrl Pts',(-29.0978789691962,67.2593020179209,
0.));
#155544=CARTESIAN_POINT('Ctrl Pts',(-29.0978789691962,67.2593020179209,
12.));
#155545=CARTESIAN_POINT('Ctrl Pts',(-29.097502097147,67.2331094720471,0.));
#155546=CARTESIAN_POINT('Ctrl Pts',(-29.097502097147,67.2331094720471,12.));
#155547=CARTESIAN_POINT('Ctrl Pts',(-29.0971014004131,67.2069550447883,
0.));
#155548=CARTESIAN_POINT('Ctrl Pts',(-29.0971014004131,67.2069550447883,
12.));
#155549=CARTESIAN_POINT('Ctrl Pts',(-29.096676931389,67.1808388322109,0.));
#155550=CARTESIAN_POINT('Ctrl Pts',(-29.096676931389,67.1808388322109,12.));
#155551=CARTESIAN_POINT('Ctrl Pts',(-29.0962287427273,67.1547609306843,
0.));
#155552=CARTESIAN_POINT('Ctrl Pts',(-29.0962287427273,67.1547609306843,
12.));
#155553=CARTESIAN_POINT('Ctrl Pts',(-29.0957568873358,67.1287214368746,
0.));
#155554=CARTESIAN_POINT('Ctrl Pts',(-29.0957568873358,67.1287214368746,
12.));
#155555=CARTESIAN_POINT('Ctrl Pts',(-29.0952614183779,67.1027204477311,
0.));
#155556=CARTESIAN_POINT('Ctrl Pts',(-29.0952614183779,67.1027204477311,
12.));
#155557=CARTESIAN_POINT('Ctrl Pts',(-29.0947423892727,67.0767580604879,
0.));
#155558=CARTESIAN_POINT('Ctrl Pts',(-29.0947423892727,67.0767580604879,
12.));
#155559=CARTESIAN_POINT('Ctrl Pts',(-29.0941998536959,67.0508343726776,
0.));
#155560=CARTESIAN_POINT('Ctrl Pts',(-29.0941998536959,67.0508343726776,
12.));
#155561=CARTESIAN_POINT('Ctrl Pts',(-29.0936338655828,67.0249494821363,
0.));
#155562=CARTESIAN_POINT('Ctrl Pts',(-29.0936338655828,67.0249494821363,
12.));
#155563=CARTESIAN_POINT('Ctrl Pts',(-29.0930444791328,66.9991034870083,
0.));
#155564=CARTESIAN_POINT('Ctrl Pts',(-29.0930444791328,66.9991034870083,
12.));
#155565=CARTESIAN_POINT('Ctrl Pts',(-29.092431748817,66.9732964857466,0.));
#155566=CARTESIAN_POINT('Ctrl Pts',(-29.092431748817,66.9732964857466,12.));
#155567=CARTESIAN_POINT('Ctrl Pts',(-29.0917957293826,66.9475285771135,
0.));
#155568=CARTESIAN_POINT('Ctrl Pts',(-29.0917957293826,66.9475285771135,
12.));
#155569=CARTESIAN_POINT('Ctrl Pts',(-29.0911364758487,66.9217998601885,
0.));
#155570=CARTESIAN_POINT('Ctrl Pts',(-29.0911364758487,66.9217998601885,
12.));
#155571=CARTESIAN_POINT('Ctrl Pts',(-29.0904540435065,66.8961104343707,
0.));
#155572=CARTESIAN_POINT('Ctrl Pts',(-29.0904540435065,66.8961104343707,
12.));
#155573=CARTESIAN_POINT('Ctrl Pts',(-29.0897484879207,66.8704603993794,
0.));
#155574=CARTESIAN_POINT('Ctrl Pts',(-29.0897484879207,66.8704603993794,
12.));
#155575=CARTESIAN_POINT('Ctrl Pts',(-29.0890198649323,66.8448498552503,
0.));
#155576=CARTESIAN_POINT('Ctrl Pts',(-29.0890198649323,66.8448498552503,
12.));
#155577=CARTESIAN_POINT('Ctrl Pts',(-29.088268230663,66.8192789023312,0.));
#155578=CARTESIAN_POINT('Ctrl Pts',(-29.088268230663,66.8192789023312,12.));
#155579=CARTESIAN_POINT('Ctrl Pts',(-29.0874936415132,66.793747641293,0.));
#155580=CARTESIAN_POINT('Ctrl Pts',(-29.0874936415132,66.793747641293,12.));
#155581=CARTESIAN_POINT('Ctrl Pts',(-29.0866961541626,66.7682561731341,
0.));
#155582=CARTESIAN_POINT('Ctrl Pts',(-29.0866961541626,66.7682561731341,
12.));
#155583=CARTESIAN_POINT('Ctrl Pts',(-29.0858758255729,66.7428045991841,
0.));
#155584=CARTESIAN_POINT('Ctrl Pts',(-29.0858758255729,66.7428045991841,
12.));
#155585=CARTESIAN_POINT('Ctrl Pts',(-29.0850327129916,66.7173930211022,
0.));
#155586=CARTESIAN_POINT('Ctrl Pts',(-29.0850327129916,66.7173930211022,
12.));
#155587=CARTESIAN_POINT('Ctrl Pts',(-29.0841668739588,66.6920215408751,
0.));
#155588=CARTESIAN_POINT('Ctrl Pts',(-29.0841668739588,66.6920215408751,
12.));
#155589=CARTESIAN_POINT('Ctrl Pts',(-29.083278366305,66.6666902608249,0.));
#155590=CARTESIAN_POINT('Ctrl Pts',(-29.083278366305,66.6666902608249,12.));
#155591=CARTESIAN_POINT('Ctrl Pts',(-29.0823672481507,66.6413992836147,
0.));
#155592=CARTESIAN_POINT('Ctrl Pts',(-29.0823672481507,66.6413992836147,
12.));
#155593=CARTESIAN_POINT('Ctrl Pts',(-29.0814335779084,66.6161487122502,
0.));
#155594=CARTESIAN_POINT('Ctrl Pts',(-29.0814335779084,66.6161487122502,
12.));
#155595=CARTESIAN_POINT('Ctrl Pts',(-29.0804774142854,66.59093865008,0.));
#155596=CARTESIAN_POINT('Ctrl Pts',(-29.0804774142854,66.59093865008,12.));
#155597=CARTESIAN_POINT('Ctrl Pts',(-29.0794988162897,66.5657692007906,
0.));
#155598=CARTESIAN_POINT('Ctrl Pts',(-29.0794988162897,66.5657692007906,
12.));
#155599=CARTESIAN_POINT('Ctrl Pts',(-29.0784978432301,66.5406404684132,
0.));
#155600=CARTESIAN_POINT('Ctrl Pts',(-29.0784978432301,66.5406404684132,
12.));
#155601=CARTESIAN_POINT('Ctrl Pts',(-29.0774745547152,66.5155525573323,
0.));
#155602=CARTESIAN_POINT('Ctrl Pts',(-29.0774745547152,66.5155525573323,
12.));
#155603=CARTESIAN_POINT('Ctrl Pts',(-29.0764290106554,66.4905055722868,
0.));
#155604=CARTESIAN_POINT('Ctrl Pts',(-29.0764290106554,66.4905055722868,
12.));
#155605=CARTESIAN_POINT('Ctrl Pts',(-29.0753612712666,66.4654996183731,
0.));
#155606=CARTESIAN_POINT('Ctrl Pts',(-29.0753612712666,66.4654996183731,
12.));
#155607=CARTESIAN_POINT('Ctrl Pts',(-29.0742713970755,66.4405348010388,
0.));
#155608=CARTESIAN_POINT('Ctrl Pts',(-29.0742713970755,66.4405348010388,
12.));
#155609=CARTESIAN_POINT('Ctrl Pts',(-29.0731594489211,66.4156112260887,
0.));
#155610=CARTESIAN_POINT('Ctrl Pts',(-29.0731594489211,66.4156112260887,
12.));
#155611=CARTESIAN_POINT('Ctrl Pts',(-29.072025487953,66.3907289996932,0.));
#155612=CARTESIAN_POINT('Ctrl Pts',(-29.072025487953,66.3907289996932,12.));
#155613=CARTESIAN_POINT('Ctrl Pts',(-29.0708695756334,66.3658882283903,
0.));
#155614=CARTESIAN_POINT('Ctrl Pts',(-29.0708695756334,66.3658882283903,
12.));
#155615=CARTESIAN_POINT('Ctrl Pts',(-29.0696917737399,66.3410890190884,
0.));
#155616=CARTESIAN_POINT('Ctrl Pts',(-29.0696917737399,66.3410890190884,
12.));
#155617=CARTESIAN_POINT('Ctrl Pts',(-29.0684921443721,66.3163314790615,
0.));
#155618=CARTESIAN_POINT('Ctrl Pts',(-29.0684921443721,66.3163314790615,
12.));
#155619=CARTESIAN_POINT('Ctrl Pts',(-29.067270749953,66.2916157159536,0.));
#155620=CARTESIAN_POINT('Ctrl Pts',(-29.067270749953,66.2916157159536,12.));
#155621=CARTESIAN_POINT('Ctrl Pts',(-29.0660276532274,66.2669418377871,
0.));
#155622=CARTESIAN_POINT('Ctrl Pts',(-29.0660276532274,66.2669418377871,
12.));
#155623=CARTESIAN_POINT('Ctrl Pts',(-29.0647629172645,66.2423099529669,
0.));
#155624=CARTESIAN_POINT('Ctrl Pts',(-29.0647629172645,66.2423099529669,
12.));
#155625=CARTESIAN_POINT('Ctrl Pts',(-29.0634766054598,66.2177201702818,
0.));
#155626=CARTESIAN_POINT('Ctrl Pts',(-29.0634766054598,66.2177201702818,
12.));
#155627=CARTESIAN_POINT('Ctrl Pts',(-29.062168781542,66.1931725989008,0.));
#155628=CARTESIAN_POINT('Ctrl Pts',(-29.062168781542,66.1931725989008,12.));
#155629=CARTESIAN_POINT('Ctrl Pts',(-29.0608395095747,66.1686673483757,
0.));
#155630=CARTESIAN_POINT('Ctrl Pts',(-29.0608395095747,66.1686673483757,
12.));
#155631=CARTESIAN_POINT('Ctrl Pts',(-29.0594888539558,66.144204528652,0.));
#155632=CARTESIAN_POINT('Ctrl Pts',(-29.0594888539558,66.144204528652,12.));
#155633=CARTESIAN_POINT('Ctrl Pts',(-29.0581168794191,66.1197842500714,
0.));
#155634=CARTESIAN_POINT('Ctrl Pts',(-29.0581168794191,66.1197842500714,
12.));
#155635=CARTESIAN_POINT('Ctrl Pts',(-29.0567236510372,66.0954066233752,
0.));
#155636=CARTESIAN_POINT('Ctrl Pts',(-29.0567236510372,66.0954066233752,
12.));
#155637=CARTESIAN_POINT('Ctrl Pts',(-29.0553092342275,66.0710717597003,
0.));
#155638=CARTESIAN_POINT('Ctrl Pts',(-29.0553092342275,66.0710717597003,
12.));
#155639=CARTESIAN_POINT('Ctrl Pts',(-29.0538736947547,66.0467797705806,
0.));
#155640=CARTESIAN_POINT('Ctrl Pts',(-29.0538736947547,66.0467797705806,
12.));
#155641=CARTESIAN_POINT('Ctrl Pts',(-29.0524170987303,66.0225307679584,
0.));
#155642=CARTESIAN_POINT('Ctrl Pts',(-29.0524170987303,66.0225307679584,
12.));
#155643=CARTESIAN_POINT('Ctrl Pts',(-29.0509395126141,65.9983248641877,
0.));
#155644=CARTESIAN_POINT('Ctrl Pts',(-29.0509395126141,65.9983248641877,
12.));
#155645=CARTESIAN_POINT('Ctrl Pts',(-29.0494410032173,65.9741621720372,
0.));
#155646=CARTESIAN_POINT('Ctrl Pts',(-29.0494410032173,65.9741621720372,
12.));
#155647=CARTESIAN_POINT('Ctrl Pts',(-29.0479216377082,65.9500428046873,
0.));
#155648=CARTESIAN_POINT('Ctrl Pts',(-29.0479216377082,65.9500428046873,
12.));
#155649=CARTESIAN_POINT('Ctrl Pts',(-29.0463814836159,65.9259668757309,
0.));
#155650=CARTESIAN_POINT('Ctrl Pts',(-29.0463814836159,65.9259668757309,
12.));
#155651=CARTESIAN_POINT('Ctrl Pts',(-29.0448206088288,65.9019344991854,
0.));
#155652=CARTESIAN_POINT('Ctrl Pts',(-29.0448206088288,65.9019344991854,
12.));
#155653=CARTESIAN_POINT('Ctrl Pts',(-29.0432390815977,65.8779457894959,
0.));
#155654=CARTESIAN_POINT('Ctrl Pts',(-29.0432390815977,65.8779457894959,
12.));
#155655=CARTESIAN_POINT('Ctrl Pts',(-29.0416369705375,65.854000861539,0.));
#155656=CARTESIAN_POINT('Ctrl Pts',(-29.0416369705375,65.854000861539,12.));
#155657=CARTESIAN_POINT('Ctrl Pts',(-29.0400143446341,65.8300998306198,
0.));
#155658=CARTESIAN_POINT('Ctrl Pts',(-29.0400143446341,65.8300998306198,
12.));
#155659=CARTESIAN_POINT('Ctrl Pts',(-29.0383712732473,65.8062428124723,
0.));
#155660=CARTESIAN_POINT('Ctrl Pts',(-29.0383712732473,65.8062428124723,
12.));
#155661=CARTESIAN_POINT('Ctrl Pts',(-29.0367078261107,65.7824299232715,
0.));
#155662=CARTESIAN_POINT('Ctrl Pts',(-29.0367078261107,65.7824299232715,
12.));
#155663=CARTESIAN_POINT('Ctrl Pts',(-29.0350240733333,65.7586612796375,
0.));
#155664=CARTESIAN_POINT('Ctrl Pts',(-29.0350240733333,65.7586612796375,
12.));
#155665=CARTESIAN_POINT('Ctrl Pts',(-29.0333200854026,65.7349369986382,
0.));
#155666=CARTESIAN_POINT('Ctrl Pts',(-29.0333200854026,65.7349369986382,
12.));
#155667=CARTESIAN_POINT('Ctrl Pts',(-29.0315959331911,65.7112571977874,
0.));
#155668=CARTESIAN_POINT('Ctrl Pts',(-29.0315959331911,65.7112571977874,
12.));
#155669=CARTESIAN_POINT('Ctrl Pts',(-29.0298516879599,65.6876219950465,
0.));
#155670=CARTESIAN_POINT('Ctrl Pts',(-29.0298516879599,65.6876219950465,
12.));
#155671=CARTESIAN_POINT('Ctrl Pts',(-29.0280874213584,65.664031508836,0.));
#155672=CARTESIAN_POINT('Ctrl Pts',(-29.0280874213584,65.664031508836,12.));
#155673=CARTESIAN_POINT('Ctrl Pts',(-29.0263032054261,65.6404858580391,
0.));
#155674=CARTESIAN_POINT('Ctrl Pts',(-29.0263032054261,65.6404858580391,
12.));
#155675=CARTESIAN_POINT('Ctrl Pts',(-29.0244991125962,65.6169851620054,
0.));
#155676=CARTESIAN_POINT('Ctrl Pts',(-29.0244991125962,65.6169851620054,
12.));
#155677=CARTESIAN_POINT('Ctrl Pts',(-29.0226752157013,65.593529540548,0.));
#155678=CARTESIAN_POINT('Ctrl Pts',(-29.0226752157013,65.593529540548,12.));
#155679=CARTESIAN_POINT('Ctrl Pts',(-29.0208315879778,65.5701191139455,
0.));
#155680=CARTESIAN_POINT('Ctrl Pts',(-29.0208315879778,65.5701191139455,
12.));
#155681=CARTESIAN_POINT('Ctrl Pts',(-29.0189683030654,65.5467540029546,
0.));
#155682=CARTESIAN_POINT('Ctrl Pts',(-29.0189683030654,65.5467540029546,
12.));
#155683=CARTESIAN_POINT('Ctrl Pts',(-29.01708543501,65.523434328815,0.));
#155684=CARTESIAN_POINT('Ctrl Pts',(-29.01708543501,65.523434328815,12.));
#155685=CARTESIAN_POINT('Ctrl Pts',(-29.015183058267,65.5001602132524,0.));
#155686=CARTESIAN_POINT('Ctrl Pts',(-29.015183058267,65.5001602132524,12.));
#155687=CARTESIAN_POINT('Ctrl Pts',(-29.0132612477075,65.4769317784754,
0.));
#155688=CARTESIAN_POINT('Ctrl Pts',(-29.0132612477075,65.4769317784754,
12.));
#155689=CARTESIAN_POINT('Ctrl Pts',(-29.0113200786219,65.4537491471782,
0.));
#155690=CARTESIAN_POINT('Ctrl Pts',(-29.0113200786219,65.4537491471782,
12.));
#155691=CARTESIAN_POINT('Ctrl Pts',(-29.0093596267198,65.4306124425524,
0.));
#155692=CARTESIAN_POINT('Ctrl Pts',(-29.0093596267198,65.4306124425524,
12.));
#155693=CARTESIAN_POINT('Ctrl Pts',(-29.0073799681336,65.4075217882921,
0.));
#155694=CARTESIAN_POINT('Ctrl Pts',(-29.0073799681336,65.4075217882921,
12.));
#155695=CARTESIAN_POINT('Ctrl Pts',(-29.0053811794214,65.3844773085976,
0.));
#155696=CARTESIAN_POINT('Ctrl Pts',(-29.0053811794214,65.3844773085976,
12.));
#155697=CARTESIAN_POINT('Ctrl Pts',(-29.0033633375745,65.3614791281725,
0.));
#155698=CARTESIAN_POINT('Ctrl Pts',(-29.0033633375745,65.3614791281725,
12.));
#155699=CARTESIAN_POINT('Ctrl Pts',(-29.0013265200201,65.3385273722278,
0.));
#155700=CARTESIAN_POINT('Ctrl Pts',(-29.0013265200201,65.3385273722278,
12.));
#155701=CARTESIAN_POINT('Ctrl Pts',(-28.9992708046223,65.3156221664942,
0.));
#155702=CARTESIAN_POINT('Ctrl Pts',(-28.9992708046223,65.3156221664942,
12.));
#155703=CARTESIAN_POINT('Ctrl Pts',(-28.9971962696848,65.2927636372261,
0.));
#155704=CARTESIAN_POINT('Ctrl Pts',(-28.9971962696848,65.2927636372261,
12.));
#155705=CARTESIAN_POINT('Ctrl Pts',(-28.9951029939551,65.2699519112052,
0.));
#155706=CARTESIAN_POINT('Ctrl Pts',(-28.9951029939551,65.2699519112052,
12.));
#155707=CARTESIAN_POINT('Ctrl Pts',(-28.9929910566314,65.2471871157375,
0.));
#155708=CARTESIAN_POINT('Ctrl Pts',(-28.9929910566314,65.2471871157375,
12.));
#155709=CARTESIAN_POINT('Ctrl Pts',(-28.9908605373652,65.2244693786586,
0.));
#155710=CARTESIAN_POINT('Ctrl Pts',(-28.9908605373652,65.2244693786586,
12.));
#155711=CARTESIAN_POINT('Ctrl Pts',(-28.9887115162626,65.2017988283465,
0.));
#155712=CARTESIAN_POINT('Ctrl Pts',(-28.9887115162626,65.2017988283465,
12.));
#155713=CARTESIAN_POINT('Ctrl Pts',(-28.9865440738882,65.1791755937254,
0.));
#155714=CARTESIAN_POINT('Ctrl Pts',(-28.9865440738882,65.1791755937254,
12.));
#155715=CARTESIAN_POINT('Ctrl Pts',(-28.9843582912697,65.1565998042705,
0.));
#155716=CARTESIAN_POINT('Ctrl Pts',(-28.9843582912697,65.1565998042705,
12.));
#155717=CARTESIAN_POINT('Ctrl Pts',(-28.9821542499049,65.1340715900042,
0.));
#155718=CARTESIAN_POINT('Ctrl Pts',(-28.9821542499049,65.1340715900042,
12.));
#155719=CARTESIAN_POINT('Ctrl Pts',(-28.9799320317648,65.111591081505,0.));
#155720=CARTESIAN_POINT('Ctrl Pts',(-28.9799320317648,65.111591081505,12.));
#155721=CARTESIAN_POINT('Ctrl Pts',(-28.9776917192936,65.0891584099174,
0.));
#155722=CARTESIAN_POINT('Ctrl Pts',(-28.9776917192936,65.0891584099174,
12.));
#155723=CARTESIAN_POINT('Ctrl Pts',(-28.9754333954134,65.0667737069562,
0.));
#155724=CARTESIAN_POINT('Ctrl Pts',(-28.9754333954134,65.0667737069562,
12.));
#155725=CARTESIAN_POINT('Ctrl Pts',(-28.9731571435281,65.0444371049082,
0.));
#155726=CARTESIAN_POINT('Ctrl Pts',(-28.9731571435281,65.0444371049082,
12.));
#155727=CARTESIAN_POINT('Ctrl Pts',(-28.9708630475298,65.0221487366279,
0.));
#155728=CARTESIAN_POINT('Ctrl Pts',(-28.9708630475298,65.0221487366279,
12.));
#155729=CARTESIAN_POINT('Ctrl Pts',(-28.9685511918017,64.9999087355504,
0.));
#155730=CARTESIAN_POINT('Ctrl Pts',(-28.9685511918017,64.9999087355504,
12.));
#155731=CARTESIAN_POINT('Ctrl Pts',(-28.9662216612216,64.9777172357028,
0.));
#155732=CARTESIAN_POINT('Ctrl Pts',(-28.9662216612216,64.9777172357028,
12.));
#155733=CARTESIAN_POINT('Ctrl Pts',(-28.9638745411677,64.955574371711,0.));
#155734=CARTESIAN_POINT('Ctrl Pts',(-28.9638745411677,64.955574371711,12.));
#155735=CARTESIAN_POINT('Ctrl Pts',(-28.961509917525,64.9334802788037,0.));
#155736=CARTESIAN_POINT('Ctrl Pts',(-28.961509917525,64.9334802788037,12.));
#155737=CARTESIAN_POINT('Ctrl Pts',(-28.9591278766934,64.9114350928124,
0.));
#155738=CARTESIAN_POINT('Ctrl Pts',(-28.9591278766934,64.9114350928124,
12.));
#155739=CARTESIAN_POINT('Ctrl Pts',(-28.9567285055866,64.8894389501799,
0.));
#155740=CARTESIAN_POINT('Ctrl Pts',(-28.9567285055866,64.8894389501799,
12.));
#155741=CARTESIAN_POINT('Ctrl Pts',(-28.9543118916327,64.8674919879646,
0.));
#155742=CARTESIAN_POINT('Ctrl Pts',(-28.9543118916327,64.8674919879646,
12.));
#155743=CARTESIAN_POINT('Ctrl Pts',(-28.9518781227765,64.8455943438423,
0.));
#155744=CARTESIAN_POINT('Ctrl Pts',(-28.9518781227765,64.8455943438423,
12.));
#155745=CARTESIAN_POINT('Ctrl Pts',(-28.9494272874833,64.8237461561024,
0.));
#155746=CARTESIAN_POINT('Ctrl Pts',(-28.9494272874833,64.8237461561024,
12.));
#155747=CARTESIAN_POINT('Ctrl Pts',(-28.9469594747436,64.8019475636454,
0.));
#155748=CARTESIAN_POINT('Ctrl Pts',(-28.9469594747436,64.8019475636454,
12.));
#155749=CARTESIAN_POINT('Ctrl Pts',(-28.9444747740815,64.7801987060097,
0.));
#155750=CARTESIAN_POINT('Ctrl Pts',(-28.9444747740815,64.7801987060097,
12.));
#155751=CARTESIAN_POINT('Ctrl Pts',(-28.9419732755659,64.7584997233889,
0.));
#155752=CARTESIAN_POINT('Ctrl Pts',(-28.9419732755659,64.7584997233889,
12.));
#155753=CARTESIAN_POINT('Ctrl Pts',(-28.9394550698201,64.7368507566461,
0.));
#155754=CARTESIAN_POINT('Ctrl Pts',(-28.9394550698201,64.7368507566461,
12.));
#155755=CARTESIAN_POINT('Ctrl Pts',(-28.9369202480383,64.715251947327,0.));
#155756=CARTESIAN_POINT('Ctrl Pts',(-28.9369202480383,64.715251947327,12.));
#155757=CARTESIAN_POINT('Ctrl Pts',(-28.934368901987,64.6937034376591,0.));
#155758=CARTESIAN_POINT('Ctrl Pts',(-28.934368901987,64.6937034376591,12.));
#155759=CARTESIAN_POINT('Ctrl Pts',(-28.9318011239905,64.6722053705389,
0.));
#155760=CARTESIAN_POINT('Ctrl Pts',(-28.9318011239905,64.6722053705389,
12.));
#155761=CARTESIAN_POINT('Ctrl Pts',(-28.9292170069219,64.6507578895155,
0.));
#155762=CARTESIAN_POINT('Ctrl Pts',(-28.9292170069219,64.6507578895155,
12.));
#155763=CARTESIAN_POINT('Ctrl Pts',(-28.9266166441956,64.6293611387753,
0.));
#155764=CARTESIAN_POINT('Ctrl Pts',(-28.9266166441956,64.6293611387753,
12.));
#155765=CARTESIAN_POINT('Ctrl Pts',(-28.9240001297553,64.6080152631065,
0.));
#155766=CARTESIAN_POINT('Ctrl Pts',(-28.9240001297553,64.6080152631065,
12.));
#155767=CARTESIAN_POINT('Ctrl Pts',(-28.9213675580996,64.5867204079452,
0.));
#155768=CARTESIAN_POINT('Ctrl Pts',(-28.9213675580996,64.5867204079452,
12.));
#155769=CARTESIAN_POINT('Ctrl Pts',(-28.9187190243231,64.5654767194487,
0.));
#155770=CARTESIAN_POINT('Ctrl Pts',(-28.9187190243231,64.5654767194487,
12.));
#155771=CARTESIAN_POINT('Ctrl Pts',(-28.9160546241538,64.544284344556,0.));
#155772=CARTESIAN_POINT('Ctrl Pts',(-28.9160546241538,64.544284344556,12.));
#155773=CARTESIAN_POINT('Ctrl Pts',(-28.9133744539943,64.5231434310457,
0.));
#155774=CARTESIAN_POINT('Ctrl Pts',(-28.9133744539943,64.5231434310457,
12.));
#155775=CARTESIAN_POINT('Ctrl Pts',(-28.9106786109639,64.5020541275927,
0.));
#155776=CARTESIAN_POINT('Ctrl Pts',(-28.9106786109639,64.5020541275927,
12.));
#155777=CARTESIAN_POINT('Ctrl Pts',(-28.9079671928253,64.4810165836568,
0.));
#155778=CARTESIAN_POINT('Ctrl Pts',(-28.9079671928253,64.4810165836568,
12.));
#155779=CARTESIAN_POINT('Ctrl Pts',(-28.9052402979055,64.460030949357,0.));
#155780=CARTESIAN_POINT('Ctrl Pts',(-28.9052402979055,64.460030949357,12.));
#155781=CARTESIAN_POINT('Ctrl Pts',(-28.9024980250309,64.439097375364,0.));
#155782=CARTESIAN_POINT('Ctrl Pts',(-28.9024980250309,64.439097375364,12.));
#155783=CARTESIAN_POINT('Ctrl Pts',(-28.899740473435,64.41821601274,0.));
#155784=CARTESIAN_POINT('Ctrl Pts',(-28.899740473435,64.41821601274,12.));
#155785=CARTESIAN_POINT('Ctrl Pts',(-28.8969677427519,64.3973870129201,
0.));
#155786=CARTESIAN_POINT('Ctrl Pts',(-28.8969677427519,64.3973870129201,
12.));
#155787=CARTESIAN_POINT('Ctrl Pts',(-28.8941799332312,64.3766105280715,
0.));
#155788=CARTESIAN_POINT('Ctrl Pts',(-28.8941799332312,64.3766105280715,
12.));
#155789=CARTESIAN_POINT('Ctrl Pts',(-28.8913771459327,64.3558867114087,
0.));
#155790=CARTESIAN_POINT('Ctrl Pts',(-28.8913771459327,64.3558867114087,
12.));
#155791=CARTESIAN_POINT('Ctrl Pts',(-28.888559482892,64.3352157174606,0.));
#155792=CARTESIAN_POINT('Ctrl Pts',(-28.888559482892,64.3352157174606,12.));
#155793=CARTESIAN_POINT('Ctrl Pts',(-28.8857270473944,64.3145977025005,
0.));
#155794=CARTESIAN_POINT('Ctrl Pts',(-28.8857270473944,64.3145977025005,
12.));
#155795=CARTESIAN_POINT('Ctrl Pts',(-28.8828799437922,64.2940328242482,
0.));
#155796=CARTESIAN_POINT('Ctrl Pts',(-28.8828799437922,64.2940328242482,
12.));
#155797=CARTESIAN_POINT('Ctrl Pts',(-28.8800182770052,64.2735212410682,
0.));
#155798=CARTESIAN_POINT('Ctrl Pts',(-28.8800182770052,64.2735212410682,
12.));
#155799=CARTESIAN_POINT('Ctrl Pts',(-28.8771421521058,64.2530631112926,
0.));
#155800=CARTESIAN_POINT('Ctrl Pts',(-28.8771421521058,64.2530631112926,
12.));
#155801=CARTESIAN_POINT('Ctrl Pts',(-28.8742516738959,64.232658592528,0.));
#155802=CARTESIAN_POINT('Ctrl Pts',(-28.8742516738959,64.232658592528,12.));
#155803=CARTESIAN_POINT('Ctrl Pts',(-28.8713469464205,64.2123078408507,
0.));
#155804=CARTESIAN_POINT('Ctrl Pts',(-28.8713469464205,64.2123078408507,
12.));
#155805=CARTESIAN_POINT('Ctrl Pts',(-28.8684280739033,64.1920110123342,
0.));
#155806=CARTESIAN_POINT('Ctrl Pts',(-28.8684280739033,64.1920110123342,
12.));
#155807=CARTESIAN_POINT('Ctrl Pts',(-28.8654951618659,64.1717682648708,
0.));
#155808=CARTESIAN_POINT('Ctrl Pts',(-28.8654951618659,64.1717682648708,
12.));
#155809=CARTESIAN_POINT('Ctrl Pts',(-28.8625483180433,64.1515797596555,
0.));
#155810=CARTESIAN_POINT('Ctrl Pts',(-28.8625483180433,64.1515797596555,
12.));
#155811=CARTESIAN_POINT('Ctrl Pts',(-28.8595876537132,64.1314456633345,
0.));
#155812=CARTESIAN_POINT('Ctrl Pts',(-28.8595876537132,64.1314456633345,
12.));
#155813=CARTESIAN_POINT('Ctrl Pts',(-28.8566132838157,64.1113661481918,
0.));
#155814=CARTESIAN_POINT('Ctrl Pts',(-28.8566132838157,64.1113661481918,
12.));
#155815=CARTESIAN_POINT('Ctrl Pts',(-28.8536253241837,64.0913413876586,
0.));
#155816=CARTESIAN_POINT('Ctrl Pts',(-28.8536253241837,64.0913413876586,
12.));
#155817=CARTESIAN_POINT('Ctrl Pts',(-28.8506238891087,64.0713715523588,
0.));
#155818=CARTESIAN_POINT('Ctrl Pts',(-28.8506238891087,64.0713715523588,
12.));
#155819=CARTESIAN_POINT('Ctrl Pts',(-28.8476090892242,64.0514568066659,
0.));
#155820=CARTESIAN_POINT('Ctrl Pts',(-28.8476090892242,64.0514568066659,
12.));
#155821=CARTESIAN_POINT('Ctrl Pts',(-28.8445810281275,64.0315973031994,
0.));
#155822=CARTESIAN_POINT('Ctrl Pts',(-28.8445810281275,64.0315973031994,
12.));
#155823=CARTESIAN_POINT('Ctrl Pts',(-28.841539805646,64.0117931881364,0.));
#155824=CARTESIAN_POINT('Ctrl Pts',(-28.841539805646,64.0117931881364,12.));
#155825=CARTESIAN_POINT('Ctrl Pts',(-28.8384855243267,63.9920446117632,
0.));
#155826=CARTESIAN_POINT('Ctrl Pts',(-28.8384855243267,63.9920446117632,
12.));
#155827=CARTESIAN_POINT('Ctrl Pts',(-28.8354182946601,63.9723517369614,
0.));
#155828=CARTESIAN_POINT('Ctrl Pts',(-28.8354182946601,63.9723517369614,
12.));
#155829=CARTESIAN_POINT('Ctrl Pts',(-28.8323382413753,63.9527147494351,
0.));
#155830=CARTESIAN_POINT('Ctrl Pts',(-28.8323382413753,63.9527147494351,
12.));
#155831=CARTESIAN_POINT('Ctrl Pts',(-28.8292455077494,63.9331338646868,
0.));
#155832=CARTESIAN_POINT('Ctrl Pts',(-28.8292455077494,63.9331338646868,
12.));
#155833=CARTESIAN_POINT('Ctrl Pts',(-28.826140242322,63.9136093063647,0.));
#155834=CARTESIAN_POINT('Ctrl Pts',(-28.826140242322,63.9136093063647,12.));
#155835=CARTESIAN_POINT('Ctrl Pts',(-28.8230225863142,63.894141285685,0.));
#155836=CARTESIAN_POINT('Ctrl Pts',(-28.8230225863142,63.894141285685,12.));
#155837=CARTESIAN_POINT('Ctrl Pts',(-28.8198926619893,63.8747299825383,
0.));
#155838=CARTESIAN_POINT('Ctrl Pts',(-28.8198926619893,63.8747299825383,
12.));
#155839=CARTESIAN_POINT('Ctrl Pts',(-28.8167505576806,63.8553755207732,
0.));
#155840=CARTESIAN_POINT('Ctrl Pts',(-28.8167505576806,63.8553755207732,
12.));
#155841=CARTESIAN_POINT('Ctrl Pts',(-28.8135963263557,63.8360779670225,
0.));
#155842=CARTESIAN_POINT('Ctrl Pts',(-28.8135963263557,63.8360779670225,
12.));
#155843=CARTESIAN_POINT('Ctrl Pts',(-28.8110632621133,63.8206854735372,
0.));
#155844=CARTESIAN_POINT('Ctrl Pts',(-28.8110632621133,63.8206854735372,
12.));
#155845=CARTESIAN_POINT('Ctrl Pts',(-28.8091580239664,63.809166727145,0.));
#155846=CARTESIAN_POINT('Ctrl Pts',(-28.8091580239664,63.809166727145,12.));
#155847=CARTESIAN_POINT('Ctrl Pts',(-28.8078854475473,63.8014989507575,
0.));
#155848=CARTESIAN_POINT('Ctrl Pts',(-28.8078854475473,63.8014989507575,
12.));
#155849=CARTESIAN_POINT('Ctrl Pts',(-28.8072485549236,63.7976679095314,
0.));
#155850=CARTESIAN_POINT('Ctrl Pts',(-28.8072485549236,63.7976679095314,
12.));
#155851=CARTESIAN_POINT('',(-28.8072485549236,63.7976679095314,12.));
#155852=CARTESIAN_POINT('Ctrl Pts',(-28.8072485549236,63.7976679095314,
12.));
#155853=CARTESIAN_POINT('Ctrl Pts',(-28.8078854475473,63.8014989507575,
12.));
#155854=CARTESIAN_POINT('Ctrl Pts',(-28.8091580239664,63.809166727145,12.));
#155855=CARTESIAN_POINT('Ctrl Pts',(-28.8110632621133,63.8206854735372,
12.));
#155856=CARTESIAN_POINT('Ctrl Pts',(-28.8135963263557,63.8360779670225,
12.));
#155857=CARTESIAN_POINT('Ctrl Pts',(-28.8167505576806,63.8553755207732,
12.));
#155858=CARTESIAN_POINT('Ctrl Pts',(-28.8198926619893,63.8747299825383,
12.));
#155859=CARTESIAN_POINT('Ctrl Pts',(-28.8230225863142,63.894141285685,12.));
#155860=CARTESIAN_POINT('Ctrl Pts',(-28.826140242322,63.9136093063647,12.));
#155861=CARTESIAN_POINT('Ctrl Pts',(-28.8292455077494,63.9331338646868,
12.));
#155862=CARTESIAN_POINT('Ctrl Pts',(-28.8323382413753,63.9527147494351,
12.));
#155863=CARTESIAN_POINT('Ctrl Pts',(-28.8354182946601,63.9723517369614,
12.));
#155864=CARTESIAN_POINT('Ctrl Pts',(-28.8384855243267,63.9920446117632,
12.));
#155865=CARTESIAN_POINT('Ctrl Pts',(-28.841539805646,64.0117931881364,12.));
#155866=CARTESIAN_POINT('Ctrl Pts',(-28.8445810281275,64.0315973031994,
12.));
#155867=CARTESIAN_POINT('Ctrl Pts',(-28.8476090892242,64.0514568066659,
12.));
#155868=CARTESIAN_POINT('Ctrl Pts',(-28.8506238891087,64.0713715523588,
12.));
#155869=CARTESIAN_POINT('Ctrl Pts',(-28.8536253241837,64.0913413876586,
12.));
#155870=CARTESIAN_POINT('Ctrl Pts',(-28.8566132838157,64.1113661481918,
12.));
#155871=CARTESIAN_POINT('Ctrl Pts',(-28.8595876537132,64.1314456633345,
12.));
#155872=CARTESIAN_POINT('Ctrl Pts',(-28.8625483180433,64.1515797596555,
12.));
#155873=CARTESIAN_POINT('Ctrl Pts',(-28.8654951618659,64.1717682648708,
12.));
#155874=CARTESIAN_POINT('Ctrl Pts',(-28.8684280739033,64.1920110123342,
12.));
#155875=CARTESIAN_POINT('Ctrl Pts',(-28.8713469464205,64.2123078408507,
12.));
#155876=CARTESIAN_POINT('Ctrl Pts',(-28.8742516738959,64.232658592528,12.));
#155877=CARTESIAN_POINT('Ctrl Pts',(-28.8771421521058,64.2530631112926,
12.));
#155878=CARTESIAN_POINT('Ctrl Pts',(-28.8800182770052,64.2735212410682,
12.));
#155879=CARTESIAN_POINT('Ctrl Pts',(-28.8828799437922,64.2940328242482,
12.));
#155880=CARTESIAN_POINT('Ctrl Pts',(-28.8857270473944,64.3145977025005,
12.));
#155881=CARTESIAN_POINT('Ctrl Pts',(-28.888559482892,64.3352157174606,12.));
#155882=CARTESIAN_POINT('Ctrl Pts',(-28.8913771459327,64.3558867114087,
12.));
#155883=CARTESIAN_POINT('Ctrl Pts',(-28.8941799332312,64.3766105280715,
12.));
#155884=CARTESIAN_POINT('Ctrl Pts',(-28.8969677427519,64.3973870129201,
12.));
#155885=CARTESIAN_POINT('Ctrl Pts',(-28.899740473435,64.41821601274,12.));
#155886=CARTESIAN_POINT('Ctrl Pts',(-28.9024980250309,64.439097375364,12.));
#155887=CARTESIAN_POINT('Ctrl Pts',(-28.9052402979055,64.460030949357,12.));
#155888=CARTESIAN_POINT('Ctrl Pts',(-28.9079671928253,64.4810165836568,
12.));
#155889=CARTESIAN_POINT('Ctrl Pts',(-28.9106786109639,64.5020541275927,
12.));
#155890=CARTESIAN_POINT('Ctrl Pts',(-28.9133744539943,64.5231434310457,
12.));
#155891=CARTESIAN_POINT('Ctrl Pts',(-28.9160546241538,64.544284344556,12.));
#155892=CARTESIAN_POINT('Ctrl Pts',(-28.9187190243231,64.5654767194487,
12.));
#155893=CARTESIAN_POINT('Ctrl Pts',(-28.9213675580996,64.5867204079452,
12.));
#155894=CARTESIAN_POINT('Ctrl Pts',(-28.9240001297553,64.6080152631065,
12.));
#155895=CARTESIAN_POINT('Ctrl Pts',(-28.9266166441956,64.6293611387753,
12.));
#155896=CARTESIAN_POINT('Ctrl Pts',(-28.9292170069219,64.6507578895155,
12.));
#155897=CARTESIAN_POINT('Ctrl Pts',(-28.9318011239905,64.6722053705389,
12.));
#155898=CARTESIAN_POINT('Ctrl Pts',(-28.934368901987,64.6937034376591,12.));
#155899=CARTESIAN_POINT('Ctrl Pts',(-28.9369202480383,64.715251947327,12.));
#155900=CARTESIAN_POINT('Ctrl Pts',(-28.9394550698201,64.7368507566461,
12.));
#155901=CARTESIAN_POINT('Ctrl Pts',(-28.9419732755659,64.7584997233889,
12.));
#155902=CARTESIAN_POINT('Ctrl Pts',(-28.9444747740815,64.7801987060097,
12.));
#155903=CARTESIAN_POINT('Ctrl Pts',(-28.9469594747436,64.8019475636454,
12.));
#155904=CARTESIAN_POINT('Ctrl Pts',(-28.9494272874833,64.8237461561024,
12.));
#155905=CARTESIAN_POINT('Ctrl Pts',(-28.9518781227765,64.8455943438423,
12.));
#155906=CARTESIAN_POINT('Ctrl Pts',(-28.9543118916327,64.8674919879646,
12.));
#155907=CARTESIAN_POINT('Ctrl Pts',(-28.9567285055866,64.8894389501799,
12.));
#155908=CARTESIAN_POINT('Ctrl Pts',(-28.9591278766934,64.9114350928124,
12.));
#155909=CARTESIAN_POINT('Ctrl Pts',(-28.961509917525,64.9334802788037,12.));
#155910=CARTESIAN_POINT('Ctrl Pts',(-28.9638745411677,64.955574371711,12.));
#155911=CARTESIAN_POINT('Ctrl Pts',(-28.9662216612216,64.9777172357028,
12.));
#155912=CARTESIAN_POINT('Ctrl Pts',(-28.9685511918017,64.9999087355504,
12.));
#155913=CARTESIAN_POINT('Ctrl Pts',(-28.9708630475298,65.0221487366279,
12.));
#155914=CARTESIAN_POINT('Ctrl Pts',(-28.9731571435281,65.0444371049082,
12.));
#155915=CARTESIAN_POINT('Ctrl Pts',(-28.9754333954134,65.0667737069562,
12.));
#155916=CARTESIAN_POINT('Ctrl Pts',(-28.9776917192936,65.0891584099174,
12.));
#155917=CARTESIAN_POINT('Ctrl Pts',(-28.9799320317648,65.111591081505,12.));
#155918=CARTESIAN_POINT('Ctrl Pts',(-28.9821542499049,65.1340715900042,
12.));
#155919=CARTESIAN_POINT('Ctrl Pts',(-28.9843582912697,65.1565998042705,
12.));
#155920=CARTESIAN_POINT('Ctrl Pts',(-28.9865440738882,65.1791755937254,
12.));
#155921=CARTESIAN_POINT('Ctrl Pts',(-28.9887115162626,65.2017988283465,
12.));
#155922=CARTESIAN_POINT('Ctrl Pts',(-28.9908605373652,65.2244693786586,
12.));
#155923=CARTESIAN_POINT('Ctrl Pts',(-28.9929910566314,65.2471871157375,
12.));
#155924=CARTESIAN_POINT('Ctrl Pts',(-28.9951029939551,65.2699519112052,
12.));
#155925=CARTESIAN_POINT('Ctrl Pts',(-28.9971962696848,65.2927636372261,
12.));
#155926=CARTESIAN_POINT('Ctrl Pts',(-28.9992708046223,65.3156221664942,
12.));
#155927=CARTESIAN_POINT('Ctrl Pts',(-29.0013265200201,65.3385273722278,
12.));
#155928=CARTESIAN_POINT('Ctrl Pts',(-29.0033633375745,65.3614791281725,
12.));
#155929=CARTESIAN_POINT('Ctrl Pts',(-29.0053811794214,65.3844773085976,
12.));
#155930=CARTESIAN_POINT('Ctrl Pts',(-29.0073799681336,65.4075217882921,
12.));
#155931=CARTESIAN_POINT('Ctrl Pts',(-29.0093596267198,65.4306124425524,
12.));
#155932=CARTESIAN_POINT('Ctrl Pts',(-29.0113200786219,65.4537491471782,
12.));
#155933=CARTESIAN_POINT('Ctrl Pts',(-29.0132612477075,65.4769317784754,
12.));
#155934=CARTESIAN_POINT('Ctrl Pts',(-29.015183058267,65.5001602132524,12.));
#155935=CARTESIAN_POINT('Ctrl Pts',(-29.01708543501,65.523434328815,12.));
#155936=CARTESIAN_POINT('Ctrl Pts',(-29.0189683030654,65.5467540029546,
12.));
#155937=CARTESIAN_POINT('Ctrl Pts',(-29.0208315879778,65.5701191139455,
12.));
#155938=CARTESIAN_POINT('Ctrl Pts',(-29.0226752157013,65.593529540548,12.));
#155939=CARTESIAN_POINT('Ctrl Pts',(-29.0244991125962,65.6169851620054,
12.));
#155940=CARTESIAN_POINT('Ctrl Pts',(-29.0263032054261,65.6404858580391,
12.));
#155941=CARTESIAN_POINT('Ctrl Pts',(-29.0280874213584,65.664031508836,12.));
#155942=CARTESIAN_POINT('Ctrl Pts',(-29.0298516879599,65.6876219950465,
12.));
#155943=CARTESIAN_POINT('Ctrl Pts',(-29.0315959331911,65.7112571977874,
12.));
#155944=CARTESIAN_POINT('Ctrl Pts',(-29.0333200854026,65.7349369986382,
12.));
#155945=CARTESIAN_POINT('Ctrl Pts',(-29.0350240733333,65.7586612796375,
12.));
#155946=CARTESIAN_POINT('Ctrl Pts',(-29.0367078261107,65.7824299232715,
12.));
#155947=CARTESIAN_POINT('Ctrl Pts',(-29.0383712732473,65.8062428124723,
12.));
#155948=CARTESIAN_POINT('Ctrl Pts',(-29.0400143446341,65.8300998306198,
12.));
#155949=CARTESIAN_POINT('Ctrl Pts',(-29.0416369705375,65.854000861539,12.));
#155950=CARTESIAN_POINT('Ctrl Pts',(-29.0432390815977,65.8779457894959,
12.));
#155951=CARTESIAN_POINT('Ctrl Pts',(-29.0448206088288,65.9019344991854,
12.));
#155952=CARTESIAN_POINT('Ctrl Pts',(-29.0463814836159,65.9259668757309,
12.));
#155953=CARTESIAN_POINT('Ctrl Pts',(-29.0479216377082,65.9500428046873,
12.));
#155954=CARTESIAN_POINT('Ctrl Pts',(-29.0494410032173,65.9741621720372,
12.));
#155955=CARTESIAN_POINT('Ctrl Pts',(-29.0509395126141,65.9983248641877,
12.));
#155956=CARTESIAN_POINT('Ctrl Pts',(-29.0524170987303,66.0225307679584,
12.));
#155957=CARTESIAN_POINT('Ctrl Pts',(-29.0538736947547,66.0467797705806,
12.));
#155958=CARTESIAN_POINT('Ctrl Pts',(-29.0553092342275,66.0710717597003,
12.));
#155959=CARTESIAN_POINT('Ctrl Pts',(-29.0567236510372,66.0954066233752,
12.));
#155960=CARTESIAN_POINT('Ctrl Pts',(-29.0581168794191,66.1197842500714,
12.));
#155961=CARTESIAN_POINT('Ctrl Pts',(-29.0594888539558,66.144204528652,12.));
#155962=CARTESIAN_POINT('Ctrl Pts',(-29.0608395095747,66.1686673483757,
12.));
#155963=CARTESIAN_POINT('Ctrl Pts',(-29.062168781542,66.1931725989008,12.));
#155964=CARTESIAN_POINT('Ctrl Pts',(-29.0634766054598,66.2177201702818,
12.));
#155965=CARTESIAN_POINT('Ctrl Pts',(-29.0647629172645,66.2423099529669,
12.));
#155966=CARTESIAN_POINT('Ctrl Pts',(-29.0660276532274,66.2669418377871,
12.));
#155967=CARTESIAN_POINT('Ctrl Pts',(-29.067270749953,66.2916157159536,12.));
#155968=CARTESIAN_POINT('Ctrl Pts',(-29.0684921443721,66.3163314790615,
12.));
#155969=CARTESIAN_POINT('Ctrl Pts',(-29.0696917737399,66.3410890190884,
12.));
#155970=CARTESIAN_POINT('Ctrl Pts',(-29.0708695756334,66.3658882283903,
12.));
#155971=CARTESIAN_POINT('Ctrl Pts',(-29.072025487953,66.3907289996932,12.));
#155972=CARTESIAN_POINT('Ctrl Pts',(-29.0731594489211,66.4156112260887,
12.));
#155973=CARTESIAN_POINT('Ctrl Pts',(-29.0742713970755,66.4405348010388,
12.));
#155974=CARTESIAN_POINT('Ctrl Pts',(-29.0753612712666,66.4654996183731,
12.));
#155975=CARTESIAN_POINT('Ctrl Pts',(-29.0764290106554,66.4905055722868,
12.));
#155976=CARTESIAN_POINT('Ctrl Pts',(-29.0774745547152,66.5155525573323,
12.));
#155977=CARTESIAN_POINT('Ctrl Pts',(-29.0784978432301,66.5406404684132,
12.));
#155978=CARTESIAN_POINT('Ctrl Pts',(-29.0794988162897,66.5657692007906,
12.));
#155979=CARTESIAN_POINT('Ctrl Pts',(-29.0804774142854,66.59093865008,12.));
#155980=CARTESIAN_POINT('Ctrl Pts',(-29.0814335779084,66.6161487122502,
12.));
#155981=CARTESIAN_POINT('Ctrl Pts',(-29.0823672481507,66.6413992836147,
12.));
#155982=CARTESIAN_POINT('Ctrl Pts',(-29.083278366305,66.6666902608249,12.));
#155983=CARTESIAN_POINT('Ctrl Pts',(-29.0841668739588,66.6920215408751,
12.));
#155984=CARTESIAN_POINT('Ctrl Pts',(-29.0850327129916,66.7173930211022,
12.));
#155985=CARTESIAN_POINT('Ctrl Pts',(-29.0858758255729,66.7428045991841,
12.));
#155986=CARTESIAN_POINT('Ctrl Pts',(-29.0866961541626,66.7682561731341,
12.));
#155987=CARTESIAN_POINT('Ctrl Pts',(-29.0874936415132,66.793747641293,12.));
#155988=CARTESIAN_POINT('Ctrl Pts',(-29.088268230663,66.8192789023312,12.));
#155989=CARTESIAN_POINT('Ctrl Pts',(-29.0890198649323,66.8448498552503,
12.));
#155990=CARTESIAN_POINT('Ctrl Pts',(-29.0897484879207,66.8704603993794,
12.));
#155991=CARTESIAN_POINT('Ctrl Pts',(-29.0904540435065,66.8961104343707,
12.));
#155992=CARTESIAN_POINT('Ctrl Pts',(-29.0911364758487,66.9217998601885,
12.));
#155993=CARTESIAN_POINT('Ctrl Pts',(-29.0917957293826,66.9475285771135,
12.));
#155994=CARTESIAN_POINT('Ctrl Pts',(-29.092431748817,66.9732964857466,12.));
#155995=CARTESIAN_POINT('Ctrl Pts',(-29.0930444791328,66.9991034870083,
12.));
#155996=CARTESIAN_POINT('Ctrl Pts',(-29.0936338655828,67.0249494821363,
12.));
#155997=CARTESIAN_POINT('Ctrl Pts',(-29.0941998536959,67.0508343726776,
12.));
#155998=CARTESIAN_POINT('Ctrl Pts',(-29.0947423892727,67.0767580604879,
12.));
#155999=CARTESIAN_POINT('Ctrl Pts',(-29.0952614183779,67.1027204477311,
12.));
#156000=CARTESIAN_POINT('Ctrl Pts',(-29.0957568873358,67.1287214368746,
12.));
#156001=CARTESIAN_POINT('Ctrl Pts',(-29.0962287427273,67.1547609306843,
12.));
#156002=CARTESIAN_POINT('Ctrl Pts',(-29.096676931389,67.1808388322109,12.));
#156003=CARTESIAN_POINT('Ctrl Pts',(-29.0971014004131,67.2069550447883,
12.));
#156004=CARTESIAN_POINT('Ctrl Pts',(-29.097502097147,67.2331094720471,12.));
#156005=CARTESIAN_POINT('Ctrl Pts',(-29.0978789691962,67.2593020179209,
12.));
#156006=CARTESIAN_POINT('Ctrl Pts',(-29.0982319644277,67.2855325866517,
12.));
#156007=CARTESIAN_POINT('Ctrl Pts',(-29.0985610309771,67.311801082792,12.));
#156008=CARTESIAN_POINT('Ctrl Pts',(-29.0988661172531,67.3381074112027,
12.));
#156009=CARTESIAN_POINT('Ctrl Pts',(-29.0991471719176,67.3644514770387,
12.));
#156010=CARTESIAN_POINT('Ctrl Pts',(-29.0994041438719,67.3908331857323,
12.));
#156011=CARTESIAN_POINT('Ctrl Pts',(-29.0996369822418,67.4172524429727,
12.));
#156012=CARTESIAN_POINT('Ctrl Pts',(-29.0998456363683,67.4437091546859,
12.));
#156013=CARTESIAN_POINT('Ctrl Pts',(-29.1000300557955,67.4702032270048,
12.));
#156014=CARTESIAN_POINT('Ctrl Pts',(-29.1001901902909,67.4967345663096,
12.));
#156015=CARTESIAN_POINT('Ctrl Pts',(-29.1003259898682,67.5233030792704,
12.));
#156016=CARTESIAN_POINT('Ctrl Pts',(-29.1004374048148,67.5499086728888,
12.));
#156017=CARTESIAN_POINT('Ctrl Pts',(-29.1005243857139,67.5765512545281,
12.));
#156018=CARTESIAN_POINT('Ctrl Pts',(-29.1005868834866,67.6032307319623,
12.));
#156019=CARTESIAN_POINT('Ctrl Pts',(-29.100624849358,67.6299470133295,12.));
#156020=CARTESIAN_POINT('Ctrl Pts',(-29.1006382347814,67.6567000070326,
12.));
#156021=CARTESIAN_POINT('Ctrl Pts',(-29.1006269913747,67.6834896216461,
12.));
#156022=CARTESIAN_POINT('Ctrl Pts',(-29.1005910708624,67.7103157658296,
12.));
#156023=CARTESIAN_POINT('Ctrl Pts',(-29.1005304249987,67.7371783482035,
12.));
#156024=CARTESIAN_POINT('Ctrl Pts',(-29.1004450055643,67.7640772773387,
12.));
#156025=CARTESIAN_POINT('Ctrl Pts',(-29.1003347645294,67.7910124620135,
12.));
#156026=CARTESIAN_POINT('Ctrl Pts',(-29.1001996541842,67.8179838114099,
12.));
#156027=CARTESIAN_POINT('Ctrl Pts',(-29.1000396272867,67.8449912353329,
12.));
#156028=CARTESIAN_POINT('Ctrl Pts',(-29.0998546372032,67.8720346444124,
12.));
#156029=CARTESIAN_POINT('Ctrl Pts',(-29.0996446380626,67.8991139503193,
12.));
#156030=CARTESIAN_POINT('Ctrl Pts',(-29.099409584422,67.9262290652829,12.));
#156031=CARTESIAN_POINT('Ctrl Pts',(-29.0991494309404,67.9533799016148,
12.));
#156032=CARTESIAN_POINT('Ctrl Pts',(-29.0988641320247,67.9805663711855,
12.));
#156033=CARTESIAN_POINT('Ctrl Pts',(-29.0985536415531,68.0077883850121,
12.));
#156034=CARTESIAN_POINT('Ctrl Pts',(-29.0982179124097,68.0350458525551,
12.));
#156035=CARTESIAN_POINT('Ctrl Pts',(-29.0978568968657,68.0623386822863,
12.));
#156036=CARTESIAN_POINT('Ctrl Pts',(-29.0974705474259,68.0896667829567,
12.));
#156037=CARTESIAN_POINT('Ctrl Pts',(-29.0970588175728,68.1170300646987,
12.));
#156038=CARTESIAN_POINT('Ctrl Pts',(-29.0966216624743,68.1444284400742,
12.));
#156039=CARTESIAN_POINT('Ctrl Pts',(-29.0961590399046,68.1718618254281,
12.));
#156040=CARTESIAN_POINT('Ctrl Pts',(-29.0956709104627,68.1993301412061,
12.));
#156041=CARTESIAN_POINT('Ctrl Pts',(-29.095230591515,68.2229056854683,12.));
#156042=CARTESIAN_POINT('Ctrl Pts',(-29.094879194787,68.2409993690197,12.));
#156043=CARTESIAN_POINT('Ctrl Pts',(-29.0946280433337,68.2535957747187,
12.));
#156044=CARTESIAN_POINT('Ctrl Pts',(-29.0944846386568,68.2606847334987,
12.));
#156045=CARTESIAN_POINT('Ctrl Pts',(-29.0944526440266,68.2622612910177,
12.));
#156046=CARTESIAN_POINT('',(-28.8072485549236,63.7976679095314,0.));
#156047=CARTESIAN_POINT('',(-28.8072485549236,63.7976679095314,0.));
#156048=CARTESIAN_POINT('Ctrl Pts',(-29.0944526440266,68.2622612910177,
0.));
#156049=CARTESIAN_POINT('Ctrl Pts',(-29.0944846386568,68.2606847334987,
0.));
#156050=CARTESIAN_POINT('Ctrl Pts',(-29.0946280433337,68.2535957747187,
0.));
#156051=CARTESIAN_POINT('Ctrl Pts',(-29.094879194787,68.2409993690197,0.));
#156052=CARTESIAN_POINT('Ctrl Pts',(-29.095230591515,68.2229056854683,0.));
#156053=CARTESIAN_POINT('Ctrl Pts',(-29.0956709104627,68.1993301412061,
0.));
#156054=CARTESIAN_POINT('Ctrl Pts',(-29.0961590399046,68.1718618254281,
0.));
#156055=CARTESIAN_POINT('Ctrl Pts',(-29.0966216624743,68.1444284400742,
0.));
#156056=CARTESIAN_POINT('Ctrl Pts',(-29.0970588175728,68.1170300646987,
0.));
#156057=CARTESIAN_POINT('Ctrl Pts',(-29.0974705474259,68.0896667829567,
0.));
#156058=CARTESIAN_POINT('Ctrl Pts',(-29.0978568968657,68.0623386822863,
0.));
#156059=CARTESIAN_POINT('Ctrl Pts',(-29.0982179124097,68.0350458525551,
0.));
#156060=CARTESIAN_POINT('Ctrl Pts',(-29.0985536415531,68.0077883850121,
0.));
#156061=CARTESIAN_POINT('Ctrl Pts',(-29.0988641320247,67.9805663711855,
0.));
#156062=CARTESIAN_POINT('Ctrl Pts',(-29.0991494309404,67.9533799016148,
0.));
#156063=CARTESIAN_POINT('Ctrl Pts',(-29.099409584422,67.9262290652829,0.));
#156064=CARTESIAN_POINT('Ctrl Pts',(-29.0996446380626,67.8991139503193,
0.));
#156065=CARTESIAN_POINT('Ctrl Pts',(-29.0998546372032,67.8720346444124,
0.));
#156066=CARTESIAN_POINT('Ctrl Pts',(-29.1000396272867,67.8449912353329,
0.));
#156067=CARTESIAN_POINT('Ctrl Pts',(-29.1001996541842,67.8179838114099,
0.));
#156068=CARTESIAN_POINT('Ctrl Pts',(-29.1003347645294,67.7910124620135,
0.));
#156069=CARTESIAN_POINT('Ctrl Pts',(-29.1004450055643,67.7640772773387,
0.));
#156070=CARTESIAN_POINT('Ctrl Pts',(-29.1005304249987,67.7371783482035,
0.));
#156071=CARTESIAN_POINT('Ctrl Pts',(-29.1005910708624,67.7103157658296,
0.));
#156072=CARTESIAN_POINT('Ctrl Pts',(-29.1006269913747,67.6834896216461,
0.));
#156073=CARTESIAN_POINT('Ctrl Pts',(-29.1006382347814,67.6567000070326,
0.));
#156074=CARTESIAN_POINT('Ctrl Pts',(-29.100624849358,67.6299470133295,0.));
#156075=CARTESIAN_POINT('Ctrl Pts',(-29.1005868834866,67.6032307319623,
0.));
#156076=CARTESIAN_POINT('Ctrl Pts',(-29.1005243857139,67.5765512545281,
0.));
#156077=CARTESIAN_POINT('Ctrl Pts',(-29.1004374048148,67.5499086728888,
0.));
#156078=CARTESIAN_POINT('Ctrl Pts',(-29.1003259898682,67.5233030792704,
0.));
#156079=CARTESIAN_POINT('Ctrl Pts',(-29.1001901902909,67.4967345663096,
0.));
#156080=CARTESIAN_POINT('Ctrl Pts',(-29.1000300557955,67.4702032270048,
0.));
#156081=CARTESIAN_POINT('Ctrl Pts',(-29.0998456363683,67.4437091546859,
0.));
#156082=CARTESIAN_POINT('Ctrl Pts',(-29.0996369822418,67.4172524429727,
0.));
#156083=CARTESIAN_POINT('Ctrl Pts',(-29.0994041438719,67.3908331857323,
0.));
#156084=CARTESIAN_POINT('Ctrl Pts',(-29.0991471719176,67.3644514770387,
0.));
#156085=CARTESIAN_POINT('Ctrl Pts',(-29.0988661172531,67.3381074112027,
0.));
#156086=CARTESIAN_POINT('Ctrl Pts',(-29.0985610309771,67.311801082792,0.));
#156087=CARTESIAN_POINT('Ctrl Pts',(-29.0982319644277,67.2855325866517,
0.));
#156088=CARTESIAN_POINT('Ctrl Pts',(-29.0978789691962,67.2593020179209,
0.));
#156089=CARTESIAN_POINT('Ctrl Pts',(-29.097502097147,67.2331094720471,0.));
#156090=CARTESIAN_POINT('Ctrl Pts',(-29.0971014004131,67.2069550447883,
0.));
#156091=CARTESIAN_POINT('Ctrl Pts',(-29.096676931389,67.1808388322109,0.));
#156092=CARTESIAN_POINT('Ctrl Pts',(-29.0962287427273,67.1547609306843,
0.));
#156093=CARTESIAN_POINT('Ctrl Pts',(-29.0957568873358,67.1287214368746,
0.));
#156094=CARTESIAN_POINT('Ctrl Pts',(-29.0952614183779,67.1027204477311,
0.));
#156095=CARTESIAN_POINT('Ctrl Pts',(-29.0947423892727,67.0767580604879,
0.));
#156096=CARTESIAN_POINT('Ctrl Pts',(-29.0941998536959,67.0508343726776,
0.));
#156097=CARTESIAN_POINT('Ctrl Pts',(-29.0936338655828,67.0249494821363,
0.));
#156098=CARTESIAN_POINT('Ctrl Pts',(-29.0930444791328,66.9991034870083,
0.));
#156099=CARTESIAN_POINT('Ctrl Pts',(-29.092431748817,66.9732964857466,0.));
#156100=CARTESIAN_POINT('Ctrl Pts',(-29.0917957293826,66.9475285771135,
0.));
#156101=CARTESIAN_POINT('Ctrl Pts',(-29.0911364758487,66.9217998601885,
0.));
#156102=CARTESIAN_POINT('Ctrl Pts',(-29.0904540435065,66.8961104343707,
0.));
#156103=CARTESIAN_POINT('Ctrl Pts',(-29.0897484879207,66.8704603993794,
0.));
#156104=CARTESIAN_POINT('Ctrl Pts',(-29.0890198649323,66.8448498552503,
0.));
#156105=CARTESIAN_POINT('Ctrl Pts',(-29.088268230663,66.8192789023312,0.));
#156106=CARTESIAN_POINT('Ctrl Pts',(-29.0874936415132,66.793747641293,0.));
#156107=CARTESIAN_POINT('Ctrl Pts',(-29.0866961541626,66.7682561731341,
0.));
#156108=CARTESIAN_POINT('Ctrl Pts',(-29.0858758255729,66.7428045991841,
0.));
#156109=CARTESIAN_POINT('Ctrl Pts',(-29.0850327129916,66.7173930211022,
0.));
#156110=CARTESIAN_POINT('Ctrl Pts',(-29.0841668739588,66.6920215408751,
0.));
#156111=CARTESIAN_POINT('Ctrl Pts',(-29.083278366305,66.6666902608249,0.));
#156112=CARTESIAN_POINT('Ctrl Pts',(-29.0823672481507,66.6413992836147,
0.));
#156113=CARTESIAN_POINT('Ctrl Pts',(-29.0814335779084,66.6161487122502,
0.));
#156114=CARTESIAN_POINT('Ctrl Pts',(-29.0804774142854,66.59093865008,0.));
#156115=CARTESIAN_POINT('Ctrl Pts',(-29.0794988162897,66.5657692007906,
0.));
#156116=CARTESIAN_POINT('Ctrl Pts',(-29.0784978432301,66.5406404684132,
0.));
#156117=CARTESIAN_POINT('Ctrl Pts',(-29.0774745547152,66.5155525573323,
0.));
#156118=CARTESIAN_POINT('Ctrl Pts',(-29.0764290106554,66.4905055722868,
0.));
#156119=CARTESIAN_POINT('Ctrl Pts',(-29.0753612712666,66.4654996183731,
0.));
#156120=CARTESIAN_POINT('Ctrl Pts',(-29.0742713970755,66.4405348010388,
0.));
#156121=CARTESIAN_POINT('Ctrl Pts',(-29.0731594489211,66.4156112260887,
0.));
#156122=CARTESIAN_POINT('Ctrl Pts',(-29.072025487953,66.3907289996932,0.));
#156123=CARTESIAN_POINT('Ctrl Pts',(-29.0708695756334,66.3658882283903,
0.));
#156124=CARTESIAN_POINT('Ctrl Pts',(-29.0696917737399,66.3410890190884,
0.));
#156125=CARTESIAN_POINT('Ctrl Pts',(-29.0684921443721,66.3163314790615,
0.));
#156126=CARTESIAN_POINT('Ctrl Pts',(-29.067270749953,66.2916157159536,0.));
#156127=CARTESIAN_POINT('Ctrl Pts',(-29.0660276532274,66.2669418377871,
0.));
#156128=CARTESIAN_POINT('Ctrl Pts',(-29.0647629172645,66.2423099529669,
0.));
#156129=CARTESIAN_POINT('Ctrl Pts',(-29.0634766054598,66.2177201702818,
0.));
#156130=CARTESIAN_POINT('Ctrl Pts',(-29.062168781542,66.1931725989008,0.));
#156131=CARTESIAN_POINT('Ctrl Pts',(-29.0608395095747,66.1686673483757,
0.));
#156132=CARTESIAN_POINT('Ctrl Pts',(-29.0594888539558,66.144204528652,0.));
#156133=CARTESIAN_POINT('Ctrl Pts',(-29.0581168794191,66.1197842500714,
0.));
#156134=CARTESIAN_POINT('Ctrl Pts',(-29.0567236510372,66.0954066233752,
0.));
#156135=CARTESIAN_POINT('Ctrl Pts',(-29.0553092342275,66.0710717597003,
0.));
#156136=CARTESIAN_POINT('Ctrl Pts',(-29.0538736947547,66.0467797705806,
0.));
#156137=CARTESIAN_POINT('Ctrl Pts',(-29.0524170987303,66.0225307679584,
0.));
#156138=CARTESIAN_POINT('Ctrl Pts',(-29.0509395126141,65.9983248641877,
0.));
#156139=CARTESIAN_POINT('Ctrl Pts',(-29.0494410032173,65.9741621720372,
0.));
#156140=CARTESIAN_POINT('Ctrl Pts',(-29.0479216377082,65.9500428046873,
0.));
#156141=CARTESIAN_POINT('Ctrl Pts',(-29.0463814836159,65.9259668757309,
0.));
#156142=CARTESIAN_POINT('Ctrl Pts',(-29.0448206088288,65.9019344991854,
0.));
#156143=CARTESIAN_POINT('Ctrl Pts',(-29.0432390815977,65.8779457894959,
0.));
#156144=CARTESIAN_POINT('Ctrl Pts',(-29.0416369705375,65.854000861539,0.));
#156145=CARTESIAN_POINT('Ctrl Pts',(-29.0400143446341,65.8300998306198,
0.));
#156146=CARTESIAN_POINT('Ctrl Pts',(-29.0383712732473,65.8062428124723,
0.));
#156147=CARTESIAN_POINT('Ctrl Pts',(-29.0367078261107,65.7824299232715,
0.));
#156148=CARTESIAN_POINT('Ctrl Pts',(-29.0350240733333,65.7586612796375,
0.));
#156149=CARTESIAN_POINT('Ctrl Pts',(-29.0333200854026,65.7349369986382,
0.));
#156150=CARTESIAN_POINT('Ctrl Pts',(-29.0315959331911,65.7112571977874,
0.));
#156151=CARTESIAN_POINT('Ctrl Pts',(-29.0298516879599,65.6876219950465,
0.));
#156152=CARTESIAN_POINT('Ctrl Pts',(-29.0280874213584,65.664031508836,0.));
#156153=CARTESIAN_POINT('Ctrl Pts',(-29.0263032054261,65.6404858580391,
0.));
#156154=CARTESIAN_POINT('Ctrl Pts',(-29.0244991125962,65.6169851620054,
0.));
#156155=CARTESIAN_POINT('Ctrl Pts',(-29.0226752157013,65.593529540548,0.));
#156156=CARTESIAN_POINT('Ctrl Pts',(-29.0208315879778,65.5701191139455,
0.));
#156157=CARTESIAN_POINT('Ctrl Pts',(-29.0189683030654,65.5467540029546,
0.));
#156158=CARTESIAN_POINT('Ctrl Pts',(-29.01708543501,65.523434328815,0.));
#156159=CARTESIAN_POINT('Ctrl Pts',(-29.015183058267,65.5001602132524,0.));
#156160=CARTESIAN_POINT('Ctrl Pts',(-29.0132612477075,65.4769317784754,
0.));
#156161=CARTESIAN_POINT('Ctrl Pts',(-29.0113200786219,65.4537491471782,
0.));
#156162=CARTESIAN_POINT('Ctrl Pts',(-29.0093596267198,65.4306124425524,
0.));
#156163=CARTESIAN_POINT('Ctrl Pts',(-29.0073799681336,65.4075217882921,
0.));
#156164=CARTESIAN_POINT('Ctrl Pts',(-29.0053811794214,65.3844773085976,
0.));
#156165=CARTESIAN_POINT('Ctrl Pts',(-29.0033633375745,65.3614791281725,
0.));
#156166=CARTESIAN_POINT('Ctrl Pts',(-29.0013265200201,65.3385273722278,
0.));
#156167=CARTESIAN_POINT('Ctrl Pts',(-28.9992708046223,65.3156221664942,
0.));
#156168=CARTESIAN_POINT('Ctrl Pts',(-28.9971962696848,65.2927636372261,
0.));
#156169=CARTESIAN_POINT('Ctrl Pts',(-28.9951029939551,65.2699519112052,
0.));
#156170=CARTESIAN_POINT('Ctrl Pts',(-28.9929910566314,65.2471871157375,
0.));
#156171=CARTESIAN_POINT('Ctrl Pts',(-28.9908605373652,65.2244693786586,
0.));
#156172=CARTESIAN_POINT('Ctrl Pts',(-28.9887115162626,65.2017988283465,
0.));
#156173=CARTESIAN_POINT('Ctrl Pts',(-28.9865440738882,65.1791755937254,
0.));
#156174=CARTESIAN_POINT('Ctrl Pts',(-28.9843582912697,65.1565998042705,
0.));
#156175=CARTESIAN_POINT('Ctrl Pts',(-28.9821542499049,65.1340715900042,
0.));
#156176=CARTESIAN_POINT('Ctrl Pts',(-28.9799320317648,65.111591081505,0.));
#156177=CARTESIAN_POINT('Ctrl Pts',(-28.9776917192936,65.0891584099174,
0.));
#156178=CARTESIAN_POINT('Ctrl Pts',(-28.9754333954134,65.0667737069562,
0.));
#156179=CARTESIAN_POINT('Ctrl Pts',(-28.9731571435281,65.0444371049082,
0.));
#156180=CARTESIAN_POINT('Ctrl Pts',(-28.9708630475298,65.0221487366279,
0.));
#156181=CARTESIAN_POINT('Ctrl Pts',(-28.9685511918017,64.9999087355504,
0.));
#156182=CARTESIAN_POINT('Ctrl Pts',(-28.9662216612216,64.9777172357028,
0.));
#156183=CARTESIAN_POINT('Ctrl Pts',(-28.9638745411677,64.955574371711,0.));
#156184=CARTESIAN_POINT('Ctrl Pts',(-28.961509917525,64.9334802788037,0.));
#156185=CARTESIAN_POINT('Ctrl Pts',(-28.9591278766934,64.9114350928124,
0.));
#156186=CARTESIAN_POINT('Ctrl Pts',(-28.9567285055866,64.8894389501799,
0.));
#156187=CARTESIAN_POINT('Ctrl Pts',(-28.9543118916327,64.8674919879646,
0.));
#156188=CARTESIAN_POINT('Ctrl Pts',(-28.9518781227765,64.8455943438423,
0.));
#156189=CARTESIAN_POINT('Ctrl Pts',(-28.9494272874833,64.8237461561024,
0.));
#156190=CARTESIAN_POINT('Ctrl Pts',(-28.9469594747436,64.8019475636454,
0.));
#156191=CARTESIAN_POINT('Ctrl Pts',(-28.9444747740815,64.7801987060097,
0.));
#156192=CARTESIAN_POINT('Ctrl Pts',(-28.9419732755659,64.7584997233889,
0.));
#156193=CARTESIAN_POINT('Ctrl Pts',(-28.9394550698201,64.7368507566461,
0.));
#156194=CARTESIAN_POINT('Ctrl Pts',(-28.9369202480383,64.715251947327,0.));
#156195=CARTESIAN_POINT('Ctrl Pts',(-28.934368901987,64.6937034376591,0.));
#156196=CARTESIAN_POINT('Ctrl Pts',(-28.9318011239905,64.6722053705389,
0.));
#156197=CARTESIAN_POINT('Ctrl Pts',(-28.9292170069219,64.6507578895155,
0.));
#156198=CARTESIAN_POINT('Ctrl Pts',(-28.9266166441956,64.6293611387753,
0.));
#156199=CARTESIAN_POINT('Ctrl Pts',(-28.9240001297553,64.6080152631065,
0.));
#156200=CARTESIAN_POINT('Ctrl Pts',(-28.9213675580996,64.5867204079452,
0.));
#156201=CARTESIAN_POINT('Ctrl Pts',(-28.9187190243231,64.5654767194487,
0.));
#156202=CARTESIAN_POINT('Ctrl Pts',(-28.9160546241538,64.544284344556,0.));
#156203=CARTESIAN_POINT('Ctrl Pts',(-28.9133744539943,64.5231434310457,
0.));
#156204=CARTESIAN_POINT('Ctrl Pts',(-28.9106786109639,64.5020541275927,
0.));
#156205=CARTESIAN_POINT('Ctrl Pts',(-28.9079671928253,64.4810165836568,
0.));
#156206=CARTESIAN_POINT('Ctrl Pts',(-28.9052402979055,64.460030949357,0.));
#156207=CARTESIAN_POINT('Ctrl Pts',(-28.9024980250309,64.439097375364,0.));
#156208=CARTESIAN_POINT('Ctrl Pts',(-28.899740473435,64.41821601274,0.));
#156209=CARTESIAN_POINT('Ctrl Pts',(-28.8969677427519,64.3973870129201,
0.));
#156210=CARTESIAN_POINT('Ctrl Pts',(-28.8941799332312,64.3766105280715,
0.));
#156211=CARTESIAN_POINT('Ctrl Pts',(-28.8913771459327,64.3558867114087,
0.));
#156212=CARTESIAN_POINT('Ctrl Pts',(-28.888559482892,64.3352157174606,0.));
#156213=CARTESIAN_POINT('Ctrl Pts',(-28.8857270473944,64.3145977025005,
0.));
#156214=CARTESIAN_POINT('Ctrl Pts',(-28.8828799437922,64.2940328242482,
0.));
#156215=CARTESIAN_POINT('Ctrl Pts',(-28.8800182770052,64.2735212410682,
0.));
#156216=CARTESIAN_POINT('Ctrl Pts',(-28.8771421521058,64.2530631112926,
0.));
#156217=CARTESIAN_POINT('Ctrl Pts',(-28.8742516738959,64.232658592528,0.));
#156218=CARTESIAN_POINT('Ctrl Pts',(-28.8713469464205,64.2123078408507,
0.));
#156219=CARTESIAN_POINT('Ctrl Pts',(-28.8684280739033,64.1920110123342,
0.));
#156220=CARTESIAN_POINT('Ctrl Pts',(-28.8654951618659,64.1717682648708,
0.));
#156221=CARTESIAN_POINT('Ctrl Pts',(-28.8625483180433,64.1515797596555,
0.));
#156222=CARTESIAN_POINT('Ctrl Pts',(-28.8595876537132,64.1314456633345,
0.));
#156223=CARTESIAN_POINT('Ctrl Pts',(-28.8566132838157,64.1113661481918,
0.));
#156224=CARTESIAN_POINT('Ctrl Pts',(-28.8536253241837,64.0913413876586,
0.));
#156225=CARTESIAN_POINT('Ctrl Pts',(-28.8506238891087,64.0713715523588,
0.));
#156226=CARTESIAN_POINT('Ctrl Pts',(-28.8476090892242,64.0514568066659,
0.));
#156227=CARTESIAN_POINT('Ctrl Pts',(-28.8445810281275,64.0315973031994,
0.));
#156228=CARTESIAN_POINT('Ctrl Pts',(-28.841539805646,64.0117931881364,0.));
#156229=CARTESIAN_POINT('Ctrl Pts',(-28.8384855243267,63.9920446117632,
0.));
#156230=CARTESIAN_POINT('Ctrl Pts',(-28.8354182946601,63.9723517369614,
0.));
#156231=CARTESIAN_POINT('Ctrl Pts',(-28.8323382413753,63.9527147494351,
0.));
#156232=CARTESIAN_POINT('Ctrl Pts',(-28.8292455077494,63.9331338646868,
0.));
#156233=CARTESIAN_POINT('Ctrl Pts',(-28.826140242322,63.9136093063647,0.));
#156234=CARTESIAN_POINT('Ctrl Pts',(-28.8230225863142,63.894141285685,0.));
#156235=CARTESIAN_POINT('Ctrl Pts',(-28.8198926619893,63.8747299825383,
0.));
#156236=CARTESIAN_POINT('Ctrl Pts',(-28.8167505576806,63.8553755207732,
0.));
#156237=CARTESIAN_POINT('Ctrl Pts',(-28.8135963263557,63.8360779670225,
0.));
#156238=CARTESIAN_POINT('Ctrl Pts',(-28.8110632621133,63.8206854735372,
0.));
#156239=CARTESIAN_POINT('Ctrl Pts',(-28.8091580239664,63.809166727145,0.));
#156240=CARTESIAN_POINT('Ctrl Pts',(-28.8078854475473,63.8014989507575,
0.));
#156241=CARTESIAN_POINT('Ctrl Pts',(-28.8072485549236,63.7976679095314,
0.));
#156242=CARTESIAN_POINT('Ctrl Pts',(-22.9976507259816,70.8615414811572,
0.));
#156243=CARTESIAN_POINT('Ctrl Pts',(-22.9976507259816,70.8615414811572,
12.));
#156244=CARTESIAN_POINT('Ctrl Pts',(-22.9983100639391,70.8559846928,0.));
#156245=CARTESIAN_POINT('Ctrl Pts',(-22.9983100639391,70.8559846928,12.));
#156246=CARTESIAN_POINT('Ctrl Pts',(-22.9996258555291,70.8448742696689,
0.));
#156247=CARTESIAN_POINT('Ctrl Pts',(-22.9996258555291,70.8448742696689,
12.));
#156248=CARTESIAN_POINT('Ctrl Pts',(-23.0015908899394,70.8282180957225,
0.));
#156249=CARTESIAN_POINT('Ctrl Pts',(-23.0015908899394,70.8282180957225,
12.));
#156250=CARTESIAN_POINT('Ctrl Pts',(-23.0041936291625,70.8060287860585,
0.));
#156251=CARTESIAN_POINT('Ctrl Pts',(-23.0041936291625,70.8060287860585,
12.));
#156252=CARTESIAN_POINT('Ctrl Pts',(-23.0074182063786,70.7783236951202,
0.));
#156253=CARTESIAN_POINT('Ctrl Pts',(-23.0074182063786,70.7783236951202,
12.));
#156254=CARTESIAN_POINT('Ctrl Pts',(-23.0106139366046,70.750650169619,0.));
#156255=CARTESIAN_POINT('Ctrl Pts',(-23.0106139366046,70.750650169619,12.));
#156256=CARTESIAN_POINT('Ctrl Pts',(-23.0137808248924,70.7230082425413,
0.));
#156257=CARTESIAN_POINT('Ctrl Pts',(-23.0137808248924,70.7230082425413,
12.));
#156258=CARTESIAN_POINT('Ctrl Pts',(-23.0169188841045,70.6953979633426,
0.));
#156259=CARTESIAN_POINT('Ctrl Pts',(-23.0169188841045,70.6953979633426,
12.));
#156260=CARTESIAN_POINT('Ctrl Pts',(-23.0200281385833,70.6678194023135,
0.));
#156261=CARTESIAN_POINT('Ctrl Pts',(-23.0200281385833,70.6678194023135,
12.));
#156262=CARTESIAN_POINT('Ctrl Pts',(-23.0231086235186,70.6402726486453,
0.));
#156263=CARTESIAN_POINT('Ctrl Pts',(-23.0231086235186,70.6402726486453,
12.));
#156264=CARTESIAN_POINT('Ctrl Pts',(-23.026160381013,70.6127578036673,0.));
#156265=CARTESIAN_POINT('Ctrl Pts',(-23.026160381013,70.6127578036673,12.));
#156266=CARTESIAN_POINT('Ctrl Pts',(-23.0291834570663,70.5852749754082,
0.));
#156267=CARTESIAN_POINT('Ctrl Pts',(-23.0291834570663,70.5852749754082,
12.));
#156268=CARTESIAN_POINT('Ctrl Pts',(-23.0321778982711,70.5578242727627,
0.));
#156269=CARTESIAN_POINT('Ctrl Pts',(-23.0321778982711,70.5578242727627,
12.));
#156270=CARTESIAN_POINT('Ctrl Pts',(-23.0351437484336,70.5304057994631,
0.));
#156271=CARTESIAN_POINT('Ctrl Pts',(-23.0351437484336,70.5304057994631,
12.));
#156272=CARTESIAN_POINT('Ctrl Pts',(-23.0380810458271,70.5030196492003,
0.));
#156273=CARTESIAN_POINT('Ctrl Pts',(-23.0380810458271,70.5030196492003,
12.));
#156274=CARTESIAN_POINT('Ctrl Pts',(-23.0409898250756,70.4756659090209,
0.));
#156275=CARTESIAN_POINT('Ctrl Pts',(-23.0409898250756,70.4756659090209,
12.));
#156276=CARTESIAN_POINT('Ctrl Pts',(-23.0438701185013,70.4483446617614,
0.));
#156277=CARTESIAN_POINT('Ctrl Pts',(-23.0438701185013,70.4483446617614,
12.));
#156278=CARTESIAN_POINT('Ctrl Pts',(-23.0467219577291,70.4210559889348,
0.));
#156279=CARTESIAN_POINT('Ctrl Pts',(-23.0467219577291,70.4210559889348,
12.));
#156280=CARTESIAN_POINT('Ctrl Pts',(-23.0495453750763,70.3937999732267,
0.));
#156281=CARTESIAN_POINT('Ctrl Pts',(-23.0495453750763,70.3937999732267,
12.));
#156282=CARTESIAN_POINT('Ctrl Pts',(-23.0523404053172,70.3665767016542,
0.));
#156283=CARTESIAN_POINT('Ctrl Pts',(-23.0523404053172,70.3665767016542,
12.));
#156284=CARTESIAN_POINT('Ctrl Pts',(-23.0551070854926,70.3393862652297,
0.));
#156285=CARTESIAN_POINT('Ctrl Pts',(-23.0551070854926,70.3393862652297,
12.));
#156286=CARTESIAN_POINT('Ctrl Pts',(-23.0578454541104,70.3122287575335,
0.));
#156287=CARTESIAN_POINT('Ctrl Pts',(-23.0578454541104,70.3122287575335,
12.));
#156288=CARTESIAN_POINT('Ctrl Pts',(-23.0605555505321,70.2851042736066,
0.));
#156289=CARTESIAN_POINT('Ctrl Pts',(-23.0605555505321,70.2851042736066,
12.));
#156290=CARTESIAN_POINT('Ctrl Pts',(-23.0632374143279,70.2580129087888,
0.));
#156291=CARTESIAN_POINT('Ctrl Pts',(-23.0632374143279,70.2580129087888,
12.));
#156292=CARTESIAN_POINT('Ctrl Pts',(-23.0658910845433,70.2309547573815,
0.));
#156293=CARTESIAN_POINT('Ctrl Pts',(-23.0658910845433,70.2309547573815,
12.));
#156294=CARTESIAN_POINT('Ctrl Pts',(-23.0685165993691,70.2039299120488,
0.));
#156295=CARTESIAN_POINT('Ctrl Pts',(-23.0685165993691,70.2039299120488,
12.));
#156296=CARTESIAN_POINT('Ctrl Pts',(-23.0711139965439,70.1769384645586,
0.));
#156297=CARTESIAN_POINT('Ctrl Pts',(-23.0711139965439,70.1769384645586,
12.));
#156298=CARTESIAN_POINT('Ctrl Pts',(-23.0736833135938,70.1499805062172,
0.));
#156299=CARTESIAN_POINT('Ctrl Pts',(-23.0736833135938,70.1499805062172,
12.));
#156300=CARTESIAN_POINT('Ctrl Pts',(-23.0762245881389,70.123056128422,0.));
#156301=CARTESIAN_POINT('Ctrl Pts',(-23.0762245881389,70.123056128422,12.));
#156302=CARTESIAN_POINT('Ctrl Pts',(-23.0787378581774,70.0961654231639,
0.));
#156303=CARTESIAN_POINT('Ctrl Pts',(-23.0787378581774,70.0961654231639,
12.));
#156304=CARTESIAN_POINT('Ctrl Pts',(-23.0812231623765,70.0693084835373,
0.));
#156305=CARTESIAN_POINT('Ctrl Pts',(-23.0812231623765,70.0693084835373,
12.));
#156306=CARTESIAN_POINT('Ctrl Pts',(-23.0836805399374,70.0424854035115,
0.));
#156307=CARTESIAN_POINT('Ctrl Pts',(-23.0836805399374,70.0424854035115,
12.));
#156308=CARTESIAN_POINT('Ctrl Pts',(-23.0861100304729,70.0156962777169,
0.));
#156309=CARTESIAN_POINT('Ctrl Pts',(-23.0861100304729,70.0156962777169,
12.));
#156310=CARTESIAN_POINT('Ctrl Pts',(-23.0885116738798,69.9889412012143,
0.));
#156311=CARTESIAN_POINT('Ctrl Pts',(-23.0885116738798,69.9889412012143,
12.));
#156312=CARTESIAN_POINT('Ctrl Pts',(-23.0908855102251,69.9622202692873,
0.));
#156313=CARTESIAN_POINT('Ctrl Pts',(-23.0908855102251,69.9622202692873,
12.));
#156314=CARTESIAN_POINT('Ctrl Pts',(-23.0932315796067,69.9355335771729,
0.));
#156315=CARTESIAN_POINT('Ctrl Pts',(-23.0932315796067,69.9355335771729,
12.));
#156316=CARTESIAN_POINT('Ctrl Pts',(-23.0955499221558,69.9088812200713,
0.));
#156317=CARTESIAN_POINT('Ctrl Pts',(-23.0955499221558,69.9088812200713,
12.));
#156318=CARTESIAN_POINT('Ctrl Pts',(-23.0978405781021,69.8822632932768,
0.));
#156319=CARTESIAN_POINT('Ctrl Pts',(-23.0978405781021,69.8822632932768,
12.));
#156320=CARTESIAN_POINT('Ctrl Pts',(-23.1001035878241,69.8556798922693,
0.));
#156321=CARTESIAN_POINT('Ctrl Pts',(-23.1001035878241,69.8556798922693,
12.));
#156322=CARTESIAN_POINT('Ctrl Pts',(-23.1023389919051,69.8291311128118,
0.));
#156323=CARTESIAN_POINT('Ctrl Pts',(-23.1023389919051,69.8291311128118,
12.));
#156324=CARTESIAN_POINT('Ctrl Pts',(-23.1045468311991,69.8026170510572,
0.));
#156325=CARTESIAN_POINT('Ctrl Pts',(-23.1045468311991,69.8026170510572,
12.));
#156326=CARTESIAN_POINT('Ctrl Pts',(-23.106727146861,69.7761378035964,0.));
#156327=CARTESIAN_POINT('Ctrl Pts',(-23.106727146861,69.7761378035964,12.));
#156328=CARTESIAN_POINT('Ctrl Pts',(-23.1088799803089,69.7496934674069,
0.));
#156329=CARTESIAN_POINT('Ctrl Pts',(-23.1088799803089,69.7496934674069,
12.));
#156330=CARTESIAN_POINT('Ctrl Pts',(-23.1110053732046,69.7232841398197,
0.));
#156331=CARTESIAN_POINT('Ctrl Pts',(-23.1110053732046,69.7232841398197,
12.));
#156332=CARTESIAN_POINT('Ctrl Pts',(-23.1131033674301,69.6969099184767,
0.));
#156333=CARTESIAN_POINT('Ctrl Pts',(-23.1131033674301,69.6969099184767,
12.));
#156334=CARTESIAN_POINT('Ctrl Pts',(-23.1151740050681,69.6705709012852,
0.));
#156335=CARTESIAN_POINT('Ctrl Pts',(-23.1151740050681,69.6705709012852,
12.));
#156336=CARTESIAN_POINT('Ctrl Pts',(-23.1172173283859,69.6442671863765,
0.));
#156337=CARTESIAN_POINT('Ctrl Pts',(-23.1172173283859,69.6442671863765,
12.));
#156338=CARTESIAN_POINT('Ctrl Pts',(-23.1192333798441,69.6179988721365,
0.));
#156339=CARTESIAN_POINT('Ctrl Pts',(-23.1192333798441,69.6179988721365,
12.));
#156340=CARTESIAN_POINT('Ctrl Pts',(-23.1212222021051,69.5917660572265,
0.));
#156341=CARTESIAN_POINT('Ctrl Pts',(-23.1212222021051,69.5917660572265,
12.));
#156342=CARTESIAN_POINT('Ctrl Pts',(-23.1231838380452,69.5655688406052,
0.));
#156343=CARTESIAN_POINT('Ctrl Pts',(-23.1231838380452,69.5655688406052,
12.));
#156344=CARTESIAN_POINT('Ctrl Pts',(-23.1251183307676,69.539407321546,0.));
#156345=CARTESIAN_POINT('Ctrl Pts',(-23.1251183307676,69.539407321546,12.));
#156346=CARTESIAN_POINT('Ctrl Pts',(-23.1270257236204,69.5132815996537,
0.));
#156347=CARTESIAN_POINT('Ctrl Pts',(-23.1270257236204,69.5132815996537,
12.));
#156348=CARTESIAN_POINT('Ctrl Pts',(-23.1289060601924,69.4871917748654,
0.));
#156349=CARTESIAN_POINT('Ctrl Pts',(-23.1289060601924,69.4871917748654,
12.));
#156350=CARTESIAN_POINT('Ctrl Pts',(-23.1307593843061,69.4611379474484,
0.));
#156351=CARTESIAN_POINT('Ctrl Pts',(-23.1307593843061,69.4611379474484,
12.));
#156352=CARTESIAN_POINT('Ctrl Pts',(-23.1325857400144,69.4351202179946,
0.));
#156353=CARTESIAN_POINT('Ctrl Pts',(-23.1325857400144,69.4351202179946,
12.));
#156354=CARTESIAN_POINT('Ctrl Pts',(-23.1343851715989,69.4091386874132,
0.));
#156355=CARTESIAN_POINT('Ctrl Pts',(-23.1343851715989,69.4091386874132,
12.));
#156356=CARTESIAN_POINT('Ctrl Pts',(-23.1361577235709,69.3831934569183,
0.));
#156357=CARTESIAN_POINT('Ctrl Pts',(-23.1361577235709,69.3831934569183,
12.));
#156358=CARTESIAN_POINT('Ctrl Pts',(-23.1379034406718,69.3572846280297,
0.));
#156359=CARTESIAN_POINT('Ctrl Pts',(-23.1379034406718,69.3572846280297,
12.));
#156360=CARTESIAN_POINT('Ctrl Pts',(-23.1396223678725,69.3314123025869,
0.));
#156361=CARTESIAN_POINT('Ctrl Pts',(-23.1396223678725,69.3314123025869,
12.));
#156362=CARTESIAN_POINT('Ctrl Pts',(-23.1413145503762,69.3055765827546,
0.));
#156363=CARTESIAN_POINT('Ctrl Pts',(-23.1413145503762,69.3055765827546,
12.));
#156364=CARTESIAN_POINT('Ctrl Pts',(-23.142980033622,69.2797775710273,0.));
#156365=CARTESIAN_POINT('Ctrl Pts',(-23.142980033622,69.2797775710273,12.));
#156366=CARTESIAN_POINT('Ctrl Pts',(-23.1446188632931,69.254015370231,0.));
#156367=CARTESIAN_POINT('Ctrl Pts',(-23.1446188632931,69.254015370231,12.));
#156368=CARTESIAN_POINT('Ctrl Pts',(-23.1462310853206,69.2282900835236,
0.));
#156369=CARTESIAN_POINT('Ctrl Pts',(-23.1462310853206,69.2282900835236,
12.));
#156370=CARTESIAN_POINT('Ctrl Pts',(-23.147816745879,69.2026018144028,0.));
#156371=CARTESIAN_POINT('Ctrl Pts',(-23.147816745879,69.2026018144028,12.));
#156372=CARTESIAN_POINT('Ctrl Pts',(-23.1493758913858,69.1769506667084,
0.));
#156373=CARTESIAN_POINT('Ctrl Pts',(-23.1493758913858,69.1769506667084,
12.));
#156374=CARTESIAN_POINT('Ctrl Pts',(-23.1509085685032,69.1513367446231,
0.));
#156375=CARTESIAN_POINT('Ctrl Pts',(-23.1509085685032,69.1513367446231,
12.));
#156376=CARTESIAN_POINT('Ctrl Pts',(-23.152414824141,69.1257601526687,0.));
#156377=CARTESIAN_POINT('Ctrl Pts',(-23.152414824141,69.1257601526687,12.));
#156378=CARTESIAN_POINT('Ctrl Pts',(-23.1538947054614,69.1002209957025,
0.));
#156379=CARTESIAN_POINT('Ctrl Pts',(-23.1538947054614,69.1002209957025,
12.));
#156380=CARTESIAN_POINT('Ctrl Pts',(-23.1553482598762,69.074719378928,0.));
#156381=CARTESIAN_POINT('Ctrl Pts',(-23.1553482598762,69.074719378928,12.));
#156382=CARTESIAN_POINT('Ctrl Pts',(-23.1567755350469,69.0492554078992,
0.));
#156383=CARTESIAN_POINT('Ctrl Pts',(-23.1567755350469,69.0492554078992,
12.));
#156384=CARTESIAN_POINT('Ctrl Pts',(-23.1581765788869,69.0238291885245,
0.));
#156385=CARTESIAN_POINT('Ctrl Pts',(-23.1581765788869,69.0238291885245,
12.));
#156386=CARTESIAN_POINT('Ctrl Pts',(-23.1595514395656,68.9984408270659,
0.));
#156387=CARTESIAN_POINT('Ctrl Pts',(-23.1595514395656,68.9984408270659,
12.));
#156388=CARTESIAN_POINT('Ctrl Pts',(-23.1609001655156,68.9730904301369,
0.));
#156389=CARTESIAN_POINT('Ctrl Pts',(-23.1609001655156,68.9730904301369,
12.));
#156390=CARTESIAN_POINT('Ctrl Pts',(-23.1622228054291,68.9477781047106,
0.));
#156391=CARTESIAN_POINT('Ctrl Pts',(-23.1622228054291,68.9477781047106,
12.));
#156392=CARTESIAN_POINT('Ctrl Pts',(-23.1635194082581,68.9225039581248,
0.));
#156393=CARTESIAN_POINT('Ctrl Pts',(-23.1635194082581,68.9225039581248,
12.));
#156394=CARTESIAN_POINT('Ctrl Pts',(-23.164790023215,68.8972680980842,0.));
#156395=CARTESIAN_POINT('Ctrl Pts',(-23.164790023215,68.8972680980842,12.));
#156396=CARTESIAN_POINT('Ctrl Pts',(-23.1660346997764,68.8720706326609,
0.));
#156397=CARTESIAN_POINT('Ctrl Pts',(-23.1660346997764,68.8720706326609,
12.));
#156398=CARTESIAN_POINT('Ctrl Pts',(-23.1672534876889,68.8469116702898,
0.));
#156399=CARTESIAN_POINT('Ctrl Pts',(-23.1672534876889,68.8469116702898,
12.));
#156400=CARTESIAN_POINT('Ctrl Pts',(-23.1684464369686,68.8217913197752,
0.));
#156401=CARTESIAN_POINT('Ctrl Pts',(-23.1684464369686,68.8217913197752,
12.));
#156402=CARTESIAN_POINT('Ctrl Pts',(-23.1696135978997,68.7967096902996,
0.));
#156403=CARTESIAN_POINT('Ctrl Pts',(-23.1696135978997,68.7967096902996,
12.));
#156404=CARTESIAN_POINT('Ctrl Pts',(-23.170755021036,68.771666891425,0.));
#156405=CARTESIAN_POINT('Ctrl Pts',(-23.170755021036,68.771666891425,12.));
#156406=CARTESIAN_POINT('Ctrl Pts',(-23.1718707572043,68.746663033096,0.));
#156407=CARTESIAN_POINT('Ctrl Pts',(-23.1718707572043,68.746663033096,12.));
#156408=CARTESIAN_POINT('Ctrl Pts',(-23.172960857511,68.7216982256341,0.));
#156409=CARTESIAN_POINT('Ctrl Pts',(-23.172960857511,68.7216982256341,12.));
#156410=CARTESIAN_POINT('Ctrl Pts',(-23.1740253733417,68.696772579744,0.));
#156411=CARTESIAN_POINT('Ctrl Pts',(-23.1740253733417,68.696772579744,12.));
#156412=CARTESIAN_POINT('Ctrl Pts',(-23.1750643563601,68.6718862065216,
0.));
#156413=CARTESIAN_POINT('Ctrl Pts',(-23.1750643563601,68.6718862065216,
12.));
#156414=CARTESIAN_POINT('Ctrl Pts',(-23.1760778585092,68.6470392174564,
0.));
#156415=CARTESIAN_POINT('Ctrl Pts',(-23.1760778585092,68.6470392174564,
12.));
#156416=CARTESIAN_POINT('Ctrl Pts',(-23.1770659320138,68.6222317244341,
0.));
#156417=CARTESIAN_POINT('Ctrl Pts',(-23.1770659320138,68.6222317244341,
12.));
#156418=CARTESIAN_POINT('Ctrl Pts',(-23.1780286293875,68.597463839733,0.));
#156419=CARTESIAN_POINT('Ctrl Pts',(-23.1780286293875,68.597463839733,12.));
#156420=CARTESIAN_POINT('Ctrl Pts',(-23.1789660034342,68.5727356760278,
0.));
#156421=CARTESIAN_POINT('Ctrl Pts',(-23.1789660034342,68.5727356760278,
12.));
#156422=CARTESIAN_POINT('Ctrl Pts',(-23.179878107245,68.5480473463985,0.));
#156423=CARTESIAN_POINT('Ctrl Pts',(-23.179878107245,68.5480473463985,12.));
#156424=CARTESIAN_POINT('Ctrl Pts',(-23.180764994201,68.5233989643345,0.));
#156425=CARTESIAN_POINT('Ctrl Pts',(-23.180764994201,68.5233989643345,12.));
#156426=CARTESIAN_POINT('Ctrl Pts',(-23.1816267179751,68.4987906437356,
0.));
#156427=CARTESIAN_POINT('Ctrl Pts',(-23.1816267179751,68.4987906437356,
12.));
#156428=CARTESIAN_POINT('Ctrl Pts',(-23.1824633325385,68.4742224989099,
0.));
#156429=CARTESIAN_POINT('Ctrl Pts',(-23.1824633325385,68.4742224989099,
12.));
#156430=CARTESIAN_POINT('Ctrl Pts',(-23.183274892163,68.4496946445758,0.));
#156431=CARTESIAN_POINT('Ctrl Pts',(-23.183274892163,68.4496946445758,12.));
#156432=CARTESIAN_POINT('Ctrl Pts',(-23.1840614514192,68.4252071958729,
0.));
#156433=CARTESIAN_POINT('Ctrl Pts',(-23.1840614514192,68.4252071958729,
12.));
#156434=CARTESIAN_POINT('Ctrl Pts',(-23.1848230651776,68.4007602683652,
0.));
#156435=CARTESIAN_POINT('Ctrl Pts',(-23.1848230651776,68.4007602683652,
12.));
#156436=CARTESIAN_POINT('Ctrl Pts',(-23.1855597886116,68.376353978044,0.));
#156437=CARTESIAN_POINT('Ctrl Pts',(-23.1855597886116,68.376353978044,12.));
#156438=CARTESIAN_POINT('Ctrl Pts',(-23.186271677203,68.3519884413246,0.));
#156439=CARTESIAN_POINT('Ctrl Pts',(-23.186271677203,68.3519884413246,12.));
#156440=CARTESIAN_POINT('Ctrl Pts',(-23.1869587867459,68.3276637750485,
0.));
#156441=CARTESIAN_POINT('Ctrl Pts',(-23.1869587867459,68.3276637750485,
12.));
#156442=CARTESIAN_POINT('Ctrl Pts',(-23.1876211733436,68.3033800964939,
0.));
#156443=CARTESIAN_POINT('Ctrl Pts',(-23.1876211733436,68.3033800964939,
12.));
#156444=CARTESIAN_POINT('Ctrl Pts',(-23.1882588934107,68.2791375233795,
0.));
#156445=CARTESIAN_POINT('Ctrl Pts',(-23.1882588934107,68.2791375233795,
12.));
#156446=CARTESIAN_POINT('Ctrl Pts',(-23.1888720036757,68.2549361738681,
0.));
#156447=CARTESIAN_POINT('Ctrl Pts',(-23.1888720036757,68.2549361738681,
12.));
#156448=CARTESIAN_POINT('Ctrl Pts',(-23.1894605611871,68.2307761665633,
0.));
#156449=CARTESIAN_POINT('Ctrl Pts',(-23.1894605611871,68.2307761665633,
12.));
#156450=CARTESIAN_POINT('Ctrl Pts',(-23.1900246233165,68.2066576205116,
0.));
#156451=CARTESIAN_POINT('Ctrl Pts',(-23.1900246233165,68.2066576205116,
12.));
#156452=CARTESIAN_POINT('Ctrl Pts',(-23.1905642477571,68.1825806552129,
0.));
#156453=CARTESIAN_POINT('Ctrl Pts',(-23.1905642477571,68.1825806552129,
12.));
#156454=CARTESIAN_POINT('Ctrl Pts',(-23.1910794925251,68.1585453906257,
0.));
#156455=CARTESIAN_POINT('Ctrl Pts',(-23.1910794925251,68.1585453906257,
12.));
#156456=CARTESIAN_POINT('Ctrl Pts',(-23.1915704159623,68.1345519471695,
0.));
#156457=CARTESIAN_POINT('Ctrl Pts',(-23.1915704159623,68.1345519471695,
12.));
#156458=CARTESIAN_POINT('Ctrl Pts',(-23.1920370767425,68.110600445723,0.));
#156459=CARTESIAN_POINT('Ctrl Pts',(-23.1920370767425,68.110600445723,12.));
#156460=CARTESIAN_POINT('Ctrl Pts',(-23.1924795338749,68.0866910076251,
0.));
#156461=CARTESIAN_POINT('Ctrl Pts',(-23.1924795338749,68.0866910076251,
12.));
#156462=CARTESIAN_POINT('Ctrl Pts',(-23.1928978467021,68.0628237546863,
0.));
#156463=CARTESIAN_POINT('Ctrl Pts',(-23.1928978467021,68.0628237546863,
12.));
#156464=CARTESIAN_POINT('Ctrl Pts',(-23.1932920749023,68.0389988091933,
0.));
#156465=CARTESIAN_POINT('Ctrl Pts',(-23.1932920749023,68.0389988091933,
12.));
#156466=CARTESIAN_POINT('Ctrl Pts',(-23.1936622784919,68.0152162939121,
0.));
#156467=CARTESIAN_POINT('Ctrl Pts',(-23.1936622784919,68.0152162939121,
12.));
#156468=CARTESIAN_POINT('Ctrl Pts',(-23.1940085178313,67.991476332086,0.));
#156469=CARTESIAN_POINT('Ctrl Pts',(-23.1940085178313,67.991476332086,12.));
#156470=CARTESIAN_POINT('Ctrl Pts',(-23.1943308536297,67.9677790474385,
0.));
#156471=CARTESIAN_POINT('Ctrl Pts',(-23.1943308536297,67.9677790474385,
12.));
#156472=CARTESIAN_POINT('Ctrl Pts',(-23.1946293469427,67.9441245641842,
0.));
#156473=CARTESIAN_POINT('Ctrl Pts',(-23.1946293469427,67.9441245641842,
12.));
#156474=CARTESIAN_POINT('Ctrl Pts',(-23.1949040591744,67.9205130070324,
0.));
#156475=CARTESIAN_POINT('Ctrl Pts',(-23.1949040591744,67.9205130070324,
12.));
#156476=CARTESIAN_POINT('Ctrl Pts',(-23.1951550520802,67.8969445011916,
0.));
#156477=CARTESIAN_POINT('Ctrl Pts',(-23.1951550520802,67.8969445011916,
12.));
#156478=CARTESIAN_POINT('Ctrl Pts',(-23.1953823877734,67.8734191723667,
0.));
#156479=CARTESIAN_POINT('Ctrl Pts',(-23.1953823877734,67.8734191723667,
12.));
#156480=CARTESIAN_POINT('Ctrl Pts',(-23.1955861287286,67.8499371467616,
0.));
#156481=CARTESIAN_POINT('Ctrl Pts',(-23.1955861287286,67.8499371467616,
12.));
#156482=CARTESIAN_POINT('Ctrl Pts',(-23.1957663377806,67.8264985510917,
0.));
#156483=CARTESIAN_POINT('Ctrl Pts',(-23.1957663377806,67.8264985510917,
12.));
#156484=CARTESIAN_POINT('Ctrl Pts',(-23.1959230781269,67.8031035125887,
0.));
#156485=CARTESIAN_POINT('Ctrl Pts',(-23.1959230781269,67.8031035125887,
12.));
#156486=CARTESIAN_POINT('Ctrl Pts',(-23.1960564133304,67.7797521590045,
0.));
#156487=CARTESIAN_POINT('Ctrl Pts',(-23.1960564133304,67.7797521590045,
12.));
#156488=CARTESIAN_POINT('Ctrl Pts',(-23.1961664073262,67.7564446186079,
0.));
#156489=CARTESIAN_POINT('Ctrl Pts',(-23.1961664073262,67.7564446186079,
12.));
#156490=CARTESIAN_POINT('Ctrl Pts',(-23.1962531244245,67.7331810201883,
0.));
#156491=CARTESIAN_POINT('Ctrl Pts',(-23.1962531244245,67.7331810201883,
12.));
#156492=CARTESIAN_POINT('Ctrl Pts',(-23.1963166293102,67.7099614930671,
0.));
#156493=CARTESIAN_POINT('Ctrl Pts',(-23.1963166293102,67.7099614930671,
12.));
#156494=CARTESIAN_POINT('Ctrl Pts',(-23.1963569870451,67.6867861671031,
0.));
#156495=CARTESIAN_POINT('Ctrl Pts',(-23.1963569870451,67.6867861671031,
12.));
#156496=CARTESIAN_POINT('Ctrl Pts',(-23.1963742630714,67.6636551726964,
0.));
#156497=CARTESIAN_POINT('Ctrl Pts',(-23.1963742630714,67.6636551726964,
12.));
#156498=CARTESIAN_POINT('Ctrl Pts',(-23.1963685232187,67.6405686407863,
0.));
#156499=CARTESIAN_POINT('Ctrl Pts',(-23.1963685232187,67.6405686407863,
12.));
#156500=CARTESIAN_POINT('Ctrl Pts',(-23.1963398337068,67.6175267028555,
0.));
#156501=CARTESIAN_POINT('Ctrl Pts',(-23.1963398337068,67.6175267028555,
12.));
#156502=CARTESIAN_POINT('Ctrl Pts',(-23.1962882611453,67.5945294909426,
0.));
#156503=CARTESIAN_POINT('Ctrl Pts',(-23.1962882611453,67.5945294909426,
12.));
#156504=CARTESIAN_POINT('Ctrl Pts',(-23.196213872536,67.5715771376461,0.));
#156505=CARTESIAN_POINT('Ctrl Pts',(-23.196213872536,67.5715771376461,12.));
#156506=CARTESIAN_POINT('Ctrl Pts',(-23.1961167352772,67.5486697761288,
0.));
#156507=CARTESIAN_POINT('Ctrl Pts',(-23.1961167352772,67.5486697761288,
12.));
#156508=CARTESIAN_POINT('Ctrl Pts',(-23.1959969171701,67.5258075401146,
0.));
#156509=CARTESIAN_POINT('Ctrl Pts',(-23.1959969171701,67.5258075401146,
12.));
#156510=CARTESIAN_POINT('Ctrl Pts',(-23.1958544864215,67.5029905638949,
0.));
#156511=CARTESIAN_POINT('Ctrl Pts',(-23.1958544864215,67.5029905638949,
12.));
#156512=CARTESIAN_POINT('Ctrl Pts',(-23.195689511644,67.4802189823408,0.));
#156513=CARTESIAN_POINT('Ctrl Pts',(-23.195689511644,67.4802189823408,12.));
#156514=CARTESIAN_POINT('Ctrl Pts',(-23.195502061859,67.4574929309076,0.));
#156515=CARTESIAN_POINT('Ctrl Pts',(-23.195502061859,67.4574929309076,12.));
#156516=CARTESIAN_POINT('Ctrl Pts',(-23.1952922065012,67.4348125456398,
0.));
#156517=CARTESIAN_POINT('Ctrl Pts',(-23.1952922065012,67.4348125456398,
12.));
#156518=CARTESIAN_POINT('Ctrl Pts',(-23.1950600154265,67.412177963168,0.));
#156519=CARTESIAN_POINT('Ctrl Pts',(-23.1950600154265,67.412177963168,12.));
#156520=CARTESIAN_POINT('Ctrl Pts',(-23.1948055589129,67.3895893207182,
0.));
#156521=CARTESIAN_POINT('Ctrl Pts',(-23.1948055589129,67.3895893207182,
12.));
#156522=CARTESIAN_POINT('Ctrl Pts',(-23.194528907661,67.3670467561212,0.));
#156523=CARTESIAN_POINT('Ctrl Pts',(-23.194528907661,67.3670467561212,12.));
#156524=CARTESIAN_POINT('Ctrl Pts',(-23.1942301327978,67.3445504078176,
0.));
#156525=CARTESIAN_POINT('Ctrl Pts',(-23.1942301327978,67.3445504078176,
12.));
#156526=CARTESIAN_POINT('Ctrl Pts',(-23.1939093058801,67.3221004148603,
0.));
#156527=CARTESIAN_POINT('Ctrl Pts',(-23.1939093058801,67.3221004148603,
12.));
#156528=CARTESIAN_POINT('Ctrl Pts',(-23.1935664989018,67.2996969169098,
0.));
#156529=CARTESIAN_POINT('Ctrl Pts',(-23.1935664989018,67.2996969169098,
12.));
#156530=CARTESIAN_POINT('Ctrl Pts',(-23.1932017842953,67.2773400542477,
0.));
#156531=CARTESIAN_POINT('Ctrl Pts',(-23.1932017842953,67.2773400542477,
12.));
#156532=CARTESIAN_POINT('Ctrl Pts',(-23.1928152349343,67.2550299677888,
0.));
#156533=CARTESIAN_POINT('Ctrl Pts',(-23.1928152349343,67.2550299677888,
12.));
#156534=CARTESIAN_POINT('Ctrl Pts',(-23.1924069241385,67.232766799088,0.));
#156535=CARTESIAN_POINT('Ctrl Pts',(-23.1924069241385,67.232766799088,12.));
#156536=CARTESIAN_POINT('Ctrl Pts',(-23.1919769256803,67.2105506903447,
0.));
#156537=CARTESIAN_POINT('Ctrl Pts',(-23.1919769256803,67.2105506903447,
12.));
#156538=CARTESIAN_POINT('Ctrl Pts',(-23.1915253137924,67.1883817844038,
0.));
#156539=CARTESIAN_POINT('Ctrl Pts',(-23.1915253137924,67.1883817844038,
12.));
#156540=CARTESIAN_POINT('Ctrl Pts',(-23.1910521631657,67.1662602247639,
0.));
#156541=CARTESIAN_POINT('Ctrl Pts',(-23.1910521631657,67.1662602247639,
12.));
#156542=CARTESIAN_POINT('Ctrl Pts',(-23.1905575489504,67.1441861555817,
0.));
#156543=CARTESIAN_POINT('Ctrl Pts',(-23.1905575489504,67.1441861555817,
12.));
#156544=CARTESIAN_POINT('Ctrl Pts',(-23.1900415467574,67.1221597216741,
0.));
#156545=CARTESIAN_POINT('Ctrl Pts',(-23.1900415467574,67.1221597216741,
12.));
#156546=CARTESIAN_POINT('Ctrl Pts',(-23.1895042326626,67.1001810685143,
0.));
#156547=CARTESIAN_POINT('Ctrl Pts',(-23.1895042326626,67.1001810685143,
12.));
#156548=CARTESIAN_POINT('Ctrl Pts',(-23.1889456832119,67.0782503422305,
0.));
#156549=CARTESIAN_POINT('Ctrl Pts',(-23.1889456832119,67.0782503422305,
12.));
#156550=CARTESIAN_POINT('Ctrl Pts',(-23.1883659754271,67.0563676896325,
0.));
#156551=CARTESIAN_POINT('Ctrl Pts',(-23.1883659754271,67.0563676896325,
12.));
#156552=CARTESIAN_POINT('Ctrl Pts',(-23.1877651868158,67.0345332582306,
0.));
#156553=CARTESIAN_POINT('Ctrl Pts',(-23.1877651868158,67.0345332582306,
12.));
#156554=CARTESIAN_POINT('Ctrl Pts',(-23.1871433953793,67.0127471962501,
0.));
#156555=CARTESIAN_POINT('Ctrl Pts',(-23.1871433953793,67.0127471962501,
12.));
#156556=CARTESIAN_POINT('Ctrl Pts',(-23.1865006796283,66.9910096526462,
0.));
#156557=CARTESIAN_POINT('Ctrl Pts',(-23.1865006796283,66.9910096526462,
12.));
#156558=CARTESIAN_POINT('Ctrl Pts',(-23.1858371185842,66.9693207771031,
0.));
#156559=CARTESIAN_POINT('Ctrl Pts',(-23.1858371185842,66.9693207771031,
12.));
#156560=CARTESIAN_POINT('Ctrl Pts',(-23.1851527917657,66.9476807200203,
0.));
#156561=CARTESIAN_POINT('Ctrl Pts',(-23.1851527917657,66.9476807200203,
12.));
#156562=CARTESIAN_POINT('Ctrl Pts',(-23.1844477791814,66.9260896324949,
0.));
#156563=CARTESIAN_POINT('Ctrl Pts',(-23.1844477791814,66.9260896324949,
12.));
#156564=CARTESIAN_POINT('Ctrl Pts',(-23.1837221613235,66.9045476663063,
0.));
#156565=CARTESIAN_POINT('Ctrl Pts',(-23.1837221613235,66.9045476663063,
12.));
#156566=CARTESIAN_POINT('Ctrl Pts',(-23.1829760191591,66.8830549738795,
0.));
#156567=CARTESIAN_POINT('Ctrl Pts',(-23.1829760191591,66.8830549738795,
12.));
#156568=CARTESIAN_POINT('Ctrl Pts',(-23.1822094341517,66.8616117083331,
0.));
#156569=CARTESIAN_POINT('Ctrl Pts',(-23.1822094341517,66.8616117083331,
12.));
#156570=CARTESIAN_POINT('Ctrl Pts',(-23.1814224882953,66.8402180235566,
0.));
#156571=CARTESIAN_POINT('Ctrl Pts',(-23.1814224882953,66.8402180235566,
12.));
#156572=CARTESIAN_POINT('Ctrl Pts',(-23.1806152641475,66.8188740742727,
0.));
#156573=CARTESIAN_POINT('Ctrl Pts',(-23.1806152641475,66.8188740742727,
12.));
#156574=CARTESIAN_POINT('Ctrl Pts',(-23.1797878448639,66.7975800161,0.));
#156575=CARTESIAN_POINT('Ctrl Pts',(-23.1797878448639,66.7975800161,12.));
#156576=CARTESIAN_POINT('Ctrl Pts',(-23.1789403142366,66.776336005612,0.));
#156577=CARTESIAN_POINT('Ctrl Pts',(-23.1789403142366,66.776336005612,12.));
#156578=CARTESIAN_POINT('Ctrl Pts',(-23.17807275663,66.7551422002204,0.));
#156579=CARTESIAN_POINT('Ctrl Pts',(-23.17807275663,66.7551422002204,12.));
#156580=CARTESIAN_POINT('Ctrl Pts',(-23.1771852569131,66.7339987580427,
0.));
#156581=CARTESIAN_POINT('Ctrl Pts',(-23.1771852569131,66.7339987580427,
12.));
#156582=CARTESIAN_POINT('Ctrl Pts',(-23.1762779004044,66.7129058377896,
0.));
#156583=CARTESIAN_POINT('Ctrl Pts',(-23.1762779004044,66.7129058377896,
12.));
#156584=CARTESIAN_POINT('Ctrl Pts',(-23.1753507727939,66.6918635985972,
0.));
#156585=CARTESIAN_POINT('Ctrl Pts',(-23.1753507727939,66.6918635985972,
12.));
#156586=CARTESIAN_POINT('Ctrl Pts',(-23.1744039601382,66.6708722000079,
0.));
#156587=CARTESIAN_POINT('Ctrl Pts',(-23.1744039601382,66.6708722000079,
12.));
#156588=CARTESIAN_POINT('Ctrl Pts',(-23.1734375490431,66.6499318023473,
0.));
#156589=CARTESIAN_POINT('Ctrl Pts',(-23.1734375490431,66.6499318023473,
12.));
#156590=CARTESIAN_POINT('Ctrl Pts',(-23.1724516268302,66.6290425670548,
0.));
#156591=CARTESIAN_POINT('Ctrl Pts',(-23.1724516268302,66.6290425670548,
12.));
#156592=CARTESIAN_POINT('Ctrl Pts',(-23.1714462816789,66.6082046569644,
0.));
#156593=CARTESIAN_POINT('Ctrl Pts',(-23.1714462816789,66.6082046569644,
12.));
#156594=CARTESIAN_POINT('Ctrl Pts',(-23.1704216028614,66.5874182367563,
0.));
#156595=CARTESIAN_POINT('Ctrl Pts',(-23.1704216028614,66.5874182367563,
12.));
#156596=CARTESIAN_POINT('Ctrl Pts',(-23.1693776805866,66.5666834726454,
0.));
#156597=CARTESIAN_POINT('Ctrl Pts',(-23.1693776805866,66.5666834726454,
12.));
#156598=CARTESIAN_POINT('Ctrl Pts',(-23.1683146055726,66.5460005315376,
0.));
#156599=CARTESIAN_POINT('Ctrl Pts',(-23.1683146055726,66.5460005315376,
12.));
#156600=CARTESIAN_POINT('Ctrl Pts',(-23.1672324686926,66.5253695803205,
0.));
#156601=CARTESIAN_POINT('Ctrl Pts',(-23.1672324686926,66.5253695803205,
12.));
#156602=CARTESIAN_POINT('Ctrl Pts',(-23.1661313606132,66.5047907851348,
0.));
#156603=CARTESIAN_POINT('Ctrl Pts',(-23.1661313606132,66.5047907851348,
12.));
#156604=CARTESIAN_POINT('Ctrl Pts',(-23.1650113713808,66.4842643105311,
0.));
#156605=CARTESIAN_POINT('Ctrl Pts',(-23.1650113713808,66.4842643105311,
12.));
#156606=CARTESIAN_POINT('Ctrl Pts',(-23.1638725912195,66.4637903210727,
0.));
#156607=CARTESIAN_POINT('Ctrl Pts',(-23.1638725912195,66.4637903210727,
12.));
#156608=CARTESIAN_POINT('Ctrl Pts',(-23.1627151114883,66.4433689832478,
0.));
#156609=CARTESIAN_POINT('Ctrl Pts',(-23.1627151114883,66.4433689832478,
12.));
#156610=CARTESIAN_POINT('Ctrl Pts',(-23.1615390254632,66.4230004670278,
0.));
#156611=CARTESIAN_POINT('Ctrl Pts',(-23.1615390254632,66.4230004670278,
12.));
#156612=CARTESIAN_POINT('Ctrl Pts',(-23.160344429474,66.4026849481232,0.));
#156613=CARTESIAN_POINT('Ctrl Pts',(-23.160344429474,66.4026849481232,12.));
#156614=CARTESIAN_POINT('Ctrl Pts',(-23.1591314230083,66.3824226081802,
0.));
#156615=CARTESIAN_POINT('Ctrl Pts',(-23.1591314230083,66.3824226081802,
12.));
#156616=CARTESIAN_POINT('Ctrl Pts',(-23.1579001063424,66.3622136300654,
0.));
#156617=CARTESIAN_POINT('Ctrl Pts',(-23.1579001063424,66.3622136300654,
12.));
#156618=CARTESIAN_POINT('Ctrl Pts',(-23.1566505784621,66.3420581937147,
0.));
#156619=CARTESIAN_POINT('Ctrl Pts',(-23.1566505784621,66.3420581937147,
12.));
#156620=CARTESIAN_POINT('Ctrl Pts',(-23.1553829352539,66.3219564725184,
0.));
#156621=CARTESIAN_POINT('Ctrl Pts',(-23.1553829352539,66.3219564725184,
12.));
#156622=CARTESIAN_POINT('Ctrl Pts',(-23.1540972666191,66.3019086275444,
0.));
#156623=CARTESIAN_POINT('Ctrl Pts',(-23.1540972666191,66.3019086275444,
12.));
#156624=CARTESIAN_POINT('Ctrl Pts',(-23.1527936592651,66.281914813114,0.));
#156625=CARTESIAN_POINT('Ctrl Pts',(-23.1527936592651,66.281914813114,12.));
#156626=CARTESIAN_POINT('Ctrl Pts',(-23.1514722022503,66.2619751878793,
0.));
#156627=CARTESIAN_POINT('Ctrl Pts',(-23.1514722022503,66.2619751878793,
12.));
#156628=CARTESIAN_POINT('Ctrl Pts',(-23.1501329914487,66.2420899237318,
0.));
#156629=CARTESIAN_POINT('Ctrl Pts',(-23.1501329914487,66.2420899237318,
12.));
#156630=CARTESIAN_POINT('Ctrl Pts',(-23.1487761349298,66.2222592165398,
0.));
#156631=CARTESIAN_POINT('Ctrl Pts',(-23.1487761349298,66.2222592165398,
12.));
#156632=CARTESIAN_POINT('Ctrl Pts',(-23.147401756643,66.2024832934733,0.));
#156633=CARTESIAN_POINT('Ctrl Pts',(-23.147401756643,66.2024832934733,12.));
#156634=CARTESIAN_POINT('Ctrl Pts',(-23.1460099850704,66.1827623902755,
0.));
#156635=CARTESIAN_POINT('Ctrl Pts',(-23.1460099850704,66.1827623902755,
12.));
#156636=CARTESIAN_POINT('Ctrl Pts',(-23.1446009424871,66.163096729667,0.));
#156637=CARTESIAN_POINT('Ctrl Pts',(-23.1446009424871,66.163096729667,12.));
#156638=CARTESIAN_POINT('Ctrl Pts',(-23.1431747350127,66.14348650151,0.));
#156639=CARTESIAN_POINT('Ctrl Pts',(-23.1431747350127,66.14348650151,12.));
#156640=CARTESIAN_POINT('Ctrl Pts',(-23.1417314398501,66.1239318368803,
0.));
#156641=CARTESIAN_POINT('Ctrl Pts',(-23.1417314398501,66.1239318368803,
12.));
#156642=CARTESIAN_POINT('Ctrl Pts',(-23.140271103958,66.1044328067739,0.));
#156643=CARTESIAN_POINT('Ctrl Pts',(-23.140271103958,66.1044328067739,12.));
#156644=CARTESIAN_POINT('Ctrl Pts',(-23.1390892229923,66.0888781152779,
0.));
#156645=CARTESIAN_POINT('Ctrl Pts',(-23.1390892229923,66.0888781152779,
12.));
#156646=CARTESIAN_POINT('Ctrl Pts',(-23.1381951597491,66.0772371487475,
0.));
#156647=CARTESIAN_POINT('Ctrl Pts',(-23.1381951597491,66.0772371487475,
12.));
#156648=CARTESIAN_POINT('Ctrl Pts',(-23.1375957166138,66.0694876382212,
0.));
#156649=CARTESIAN_POINT('Ctrl Pts',(-23.1375957166138,66.0694876382212,
12.));
#156650=CARTESIAN_POINT('Ctrl Pts',(-23.1372951448024,66.0656156664138,
0.));
#156651=CARTESIAN_POINT('Ctrl Pts',(-23.1372951448024,66.0656156664138,
12.));
#156652=CARTESIAN_POINT('',(-23.1372951448024,66.0656156664138,12.));
#156653=CARTESIAN_POINT('Ctrl Pts',(-23.1372951448024,66.0656156664138,
12.));
#156654=CARTESIAN_POINT('Ctrl Pts',(-23.1375957166138,66.0694876382212,
12.));
#156655=CARTESIAN_POINT('Ctrl Pts',(-23.1381951597491,66.0772371487475,
12.));
#156656=CARTESIAN_POINT('Ctrl Pts',(-23.1390892229923,66.0888781152779,
12.));
#156657=CARTESIAN_POINT('Ctrl Pts',(-23.140271103958,66.1044328067739,12.));
#156658=CARTESIAN_POINT('Ctrl Pts',(-23.1417314398501,66.1239318368803,
12.));
#156659=CARTESIAN_POINT('Ctrl Pts',(-23.1431747350127,66.14348650151,12.));
#156660=CARTESIAN_POINT('Ctrl Pts',(-23.1446009424871,66.163096729667,12.));
#156661=CARTESIAN_POINT('Ctrl Pts',(-23.1460099850704,66.1827623902755,
12.));
#156662=CARTESIAN_POINT('Ctrl Pts',(-23.147401756643,66.2024832934733,12.));
#156663=CARTESIAN_POINT('Ctrl Pts',(-23.1487761349298,66.2222592165398,
12.));
#156664=CARTESIAN_POINT('Ctrl Pts',(-23.1501329914487,66.2420899237318,
12.));
#156665=CARTESIAN_POINT('Ctrl Pts',(-23.1514722022503,66.2619751878793,
12.));
#156666=CARTESIAN_POINT('Ctrl Pts',(-23.1527936592651,66.281914813114,12.));
#156667=CARTESIAN_POINT('Ctrl Pts',(-23.1540972666191,66.3019086275444,
12.));
#156668=CARTESIAN_POINT('Ctrl Pts',(-23.1553829352539,66.3219564725184,
12.));
#156669=CARTESIAN_POINT('Ctrl Pts',(-23.1566505784621,66.3420581937147,
12.));
#156670=CARTESIAN_POINT('Ctrl Pts',(-23.1579001063424,66.3622136300654,
12.));
#156671=CARTESIAN_POINT('Ctrl Pts',(-23.1591314230083,66.3824226081802,
12.));
#156672=CARTESIAN_POINT('Ctrl Pts',(-23.160344429474,66.4026849481232,12.));
#156673=CARTESIAN_POINT('Ctrl Pts',(-23.1615390254632,66.4230004670278,
12.));
#156674=CARTESIAN_POINT('Ctrl Pts',(-23.1627151114883,66.4433689832478,
12.));
#156675=CARTESIAN_POINT('Ctrl Pts',(-23.1638725912195,66.4637903210727,
12.));
#156676=CARTESIAN_POINT('Ctrl Pts',(-23.1650113713808,66.4842643105311,
12.));
#156677=CARTESIAN_POINT('Ctrl Pts',(-23.1661313606132,66.5047907851348,
12.));
#156678=CARTESIAN_POINT('Ctrl Pts',(-23.1672324686926,66.5253695803205,
12.));
#156679=CARTESIAN_POINT('Ctrl Pts',(-23.1683146055726,66.5460005315376,
12.));
#156680=CARTESIAN_POINT('Ctrl Pts',(-23.1693776805866,66.5666834726454,
12.));
#156681=CARTESIAN_POINT('Ctrl Pts',(-23.1704216028614,66.5874182367563,
12.));
#156682=CARTESIAN_POINT('Ctrl Pts',(-23.1714462816789,66.6082046569644,
12.));
#156683=CARTESIAN_POINT('Ctrl Pts',(-23.1724516268302,66.6290425670548,
12.));
#156684=CARTESIAN_POINT('Ctrl Pts',(-23.1734375490431,66.6499318023473,
12.));
#156685=CARTESIAN_POINT('Ctrl Pts',(-23.1744039601382,66.6708722000079,
12.));
#156686=CARTESIAN_POINT('Ctrl Pts',(-23.1753507727939,66.6918635985972,
12.));
#156687=CARTESIAN_POINT('Ctrl Pts',(-23.1762779004044,66.7129058377896,
12.));
#156688=CARTESIAN_POINT('Ctrl Pts',(-23.1771852569131,66.7339987580427,
12.));
#156689=CARTESIAN_POINT('Ctrl Pts',(-23.17807275663,66.7551422002204,12.));
#156690=CARTESIAN_POINT('Ctrl Pts',(-23.1789403142366,66.776336005612,12.));
#156691=CARTESIAN_POINT('Ctrl Pts',(-23.1797878448639,66.7975800161,12.));
#156692=CARTESIAN_POINT('Ctrl Pts',(-23.1806152641475,66.8188740742727,
12.));
#156693=CARTESIAN_POINT('Ctrl Pts',(-23.1814224882953,66.8402180235566,
12.));
#156694=CARTESIAN_POINT('Ctrl Pts',(-23.1822094341517,66.8616117083331,
12.));
#156695=CARTESIAN_POINT('Ctrl Pts',(-23.1829760191591,66.8830549738795,
12.));
#156696=CARTESIAN_POINT('Ctrl Pts',(-23.1837221613235,66.9045476663063,
12.));
#156697=CARTESIAN_POINT('Ctrl Pts',(-23.1844477791814,66.9260896324949,
12.));
#156698=CARTESIAN_POINT('Ctrl Pts',(-23.1851527917657,66.9476807200203,
12.));
#156699=CARTESIAN_POINT('Ctrl Pts',(-23.1858371185842,66.9693207771031,
12.));
#156700=CARTESIAN_POINT('Ctrl Pts',(-23.1865006796283,66.9910096526462,
12.));
#156701=CARTESIAN_POINT('Ctrl Pts',(-23.1871433953793,67.0127471962501,
12.));
#156702=CARTESIAN_POINT('Ctrl Pts',(-23.1877651868158,67.0345332582306,
12.));
#156703=CARTESIAN_POINT('Ctrl Pts',(-23.1883659754271,67.0563676896325,
12.));
#156704=CARTESIAN_POINT('Ctrl Pts',(-23.1889456832119,67.0782503422305,
12.));
#156705=CARTESIAN_POINT('Ctrl Pts',(-23.1895042326626,67.1001810685143,
12.));
#156706=CARTESIAN_POINT('Ctrl Pts',(-23.1900415467574,67.1221597216741,
12.));
#156707=CARTESIAN_POINT('Ctrl Pts',(-23.1905575489504,67.1441861555817,
12.));
#156708=CARTESIAN_POINT('Ctrl Pts',(-23.1910521631657,67.1662602247639,
12.));
#156709=CARTESIAN_POINT('Ctrl Pts',(-23.1915253137924,67.1883817844038,
12.));
#156710=CARTESIAN_POINT('Ctrl Pts',(-23.1919769256803,67.2105506903447,
12.));
#156711=CARTESIAN_POINT('Ctrl Pts',(-23.1924069241385,67.232766799088,12.));
#156712=CARTESIAN_POINT('Ctrl Pts',(-23.1928152349343,67.2550299677888,
12.));
#156713=CARTESIAN_POINT('Ctrl Pts',(-23.1932017842953,67.2773400542477,
12.));
#156714=CARTESIAN_POINT('Ctrl Pts',(-23.1935664989018,67.2996969169098,
12.));
#156715=CARTESIAN_POINT('Ctrl Pts',(-23.1939093058801,67.3221004148603,
12.));
#156716=CARTESIAN_POINT('Ctrl Pts',(-23.1942301327978,67.3445504078176,
12.));
#156717=CARTESIAN_POINT('Ctrl Pts',(-23.194528907661,67.3670467561212,12.));
#156718=CARTESIAN_POINT('Ctrl Pts',(-23.1948055589129,67.3895893207182,
12.));
#156719=CARTESIAN_POINT('Ctrl Pts',(-23.1950600154265,67.412177963168,12.));
#156720=CARTESIAN_POINT('Ctrl Pts',(-23.1952922065012,67.4348125456398,
12.));
#156721=CARTESIAN_POINT('Ctrl Pts',(-23.195502061859,67.4574929309076,12.));
#156722=CARTESIAN_POINT('Ctrl Pts',(-23.195689511644,67.4802189823408,12.));
#156723=CARTESIAN_POINT('Ctrl Pts',(-23.1958544864215,67.5029905638949,
12.));
#156724=CARTESIAN_POINT('Ctrl Pts',(-23.1959969171701,67.5258075401146,
12.));
#156725=CARTESIAN_POINT('Ctrl Pts',(-23.1961167352772,67.5486697761288,
12.));
#156726=CARTESIAN_POINT('Ctrl Pts',(-23.196213872536,67.5715771376461,12.));
#156727=CARTESIAN_POINT('Ctrl Pts',(-23.1962882611453,67.5945294909426,
12.));
#156728=CARTESIAN_POINT('Ctrl Pts',(-23.1963398337068,67.6175267028555,
12.));
#156729=CARTESIAN_POINT('Ctrl Pts',(-23.1963685232187,67.6405686407863,
12.));
#156730=CARTESIAN_POINT('Ctrl Pts',(-23.1963742630714,67.6636551726964,
12.));
#156731=CARTESIAN_POINT('Ctrl Pts',(-23.1963569870451,67.6867861671031,
12.));
#156732=CARTESIAN_POINT('Ctrl Pts',(-23.1963166293102,67.7099614930671,
12.));
#156733=CARTESIAN_POINT('Ctrl Pts',(-23.1962531244245,67.7331810201883,
12.));
#156734=CARTESIAN_POINT('Ctrl Pts',(-23.1961664073262,67.7564446186079,
12.));
#156735=CARTESIAN_POINT('Ctrl Pts',(-23.1960564133304,67.7797521590045,
12.));
#156736=CARTESIAN_POINT('Ctrl Pts',(-23.1959230781269,67.8031035125887,
12.));
#156737=CARTESIAN_POINT('Ctrl Pts',(-23.1957663377806,67.8264985510917,
12.));
#156738=CARTESIAN_POINT('Ctrl Pts',(-23.1955861287286,67.8499371467616,
12.));
#156739=CARTESIAN_POINT('Ctrl Pts',(-23.1953823877734,67.8734191723667,
12.));
#156740=CARTESIAN_POINT('Ctrl Pts',(-23.1951550520802,67.8969445011916,
12.));
#156741=CARTESIAN_POINT('Ctrl Pts',(-23.1949040591744,67.9205130070324,
12.));
#156742=CARTESIAN_POINT('Ctrl Pts',(-23.1946293469427,67.9441245641842,
12.));
#156743=CARTESIAN_POINT('Ctrl Pts',(-23.1943308536297,67.9677790474385,
12.));
#156744=CARTESIAN_POINT('Ctrl Pts',(-23.1940085178313,67.991476332086,12.));
#156745=CARTESIAN_POINT('Ctrl Pts',(-23.1936622784919,68.0152162939121,
12.));
#156746=CARTESIAN_POINT('Ctrl Pts',(-23.1932920749023,68.0389988091933,
12.));
#156747=CARTESIAN_POINT('Ctrl Pts',(-23.1928978467021,68.0628237546863,
12.));
#156748=CARTESIAN_POINT('Ctrl Pts',(-23.1924795338749,68.0866910076251,
12.));
#156749=CARTESIAN_POINT('Ctrl Pts',(-23.1920370767425,68.110600445723,12.));
#156750=CARTESIAN_POINT('Ctrl Pts',(-23.1915704159623,68.1345519471695,
12.));
#156751=CARTESIAN_POINT('Ctrl Pts',(-23.1910794925251,68.1585453906257,
12.));
#156752=CARTESIAN_POINT('Ctrl Pts',(-23.1905642477571,68.1825806552129,
12.));
#156753=CARTESIAN_POINT('Ctrl Pts',(-23.1900246233165,68.2066576205116,
12.));
#156754=CARTESIAN_POINT('Ctrl Pts',(-23.1894605611871,68.2307761665633,
12.));
#156755=CARTESIAN_POINT('Ctrl Pts',(-23.1888720036757,68.2549361738681,
12.));
#156756=CARTESIAN_POINT('Ctrl Pts',(-23.1882588934107,68.2791375233795,
12.));
#156757=CARTESIAN_POINT('Ctrl Pts',(-23.1876211733436,68.3033800964939,
12.));
#156758=CARTESIAN_POINT('Ctrl Pts',(-23.1869587867459,68.3276637750485,
12.));
#156759=CARTESIAN_POINT('Ctrl Pts',(-23.186271677203,68.3519884413246,12.));
#156760=CARTESIAN_POINT('Ctrl Pts',(-23.1855597886116,68.376353978044,12.));
#156761=CARTESIAN_POINT('Ctrl Pts',(-23.1848230651776,68.4007602683652,
12.));
#156762=CARTESIAN_POINT('Ctrl Pts',(-23.1840614514192,68.4252071958729,
12.));
#156763=CARTESIAN_POINT('Ctrl Pts',(-23.183274892163,68.4496946445758,12.));
#156764=CARTESIAN_POINT('Ctrl Pts',(-23.1824633325385,68.4742224989099,
12.));
#156765=CARTESIAN_POINT('Ctrl Pts',(-23.1816267179751,68.4987906437356,
12.));
#156766=CARTESIAN_POINT('Ctrl Pts',(-23.180764994201,68.5233989643345,12.));
#156767=CARTESIAN_POINT('Ctrl Pts',(-23.179878107245,68.5480473463985,12.));
#156768=CARTESIAN_POINT('Ctrl Pts',(-23.1789660034342,68.5727356760278,
12.));
#156769=CARTESIAN_POINT('Ctrl Pts',(-23.1780286293875,68.597463839733,12.));
#156770=CARTESIAN_POINT('Ctrl Pts',(-23.1770659320138,68.6222317244341,
12.));
#156771=CARTESIAN_POINT('Ctrl Pts',(-23.1760778585092,68.6470392174564,
12.));
#156772=CARTESIAN_POINT('Ctrl Pts',(-23.1750643563601,68.6718862065216,
12.));
#156773=CARTESIAN_POINT('Ctrl Pts',(-23.1740253733417,68.696772579744,12.));
#156774=CARTESIAN_POINT('Ctrl Pts',(-23.172960857511,68.7216982256341,12.));
#156775=CARTESIAN_POINT('Ctrl Pts',(-23.1718707572043,68.746663033096,12.));
#156776=CARTESIAN_POINT('Ctrl Pts',(-23.170755021036,68.771666891425,12.));
#156777=CARTESIAN_POINT('Ctrl Pts',(-23.1696135978997,68.7967096902996,
12.));
#156778=CARTESIAN_POINT('Ctrl Pts',(-23.1684464369686,68.8217913197752,
12.));
#156779=CARTESIAN_POINT('Ctrl Pts',(-23.1672534876889,68.8469116702898,
12.));
#156780=CARTESIAN_POINT('Ctrl Pts',(-23.1660346997764,68.8720706326609,
12.));
#156781=CARTESIAN_POINT('Ctrl Pts',(-23.164790023215,68.8972680980842,12.));
#156782=CARTESIAN_POINT('Ctrl Pts',(-23.1635194082581,68.9225039581248,
12.));
#156783=CARTESIAN_POINT('Ctrl Pts',(-23.1622228054291,68.9477781047106,
12.));
#156784=CARTESIAN_POINT('Ctrl Pts',(-23.1609001655156,68.9730904301369,
12.));
#156785=CARTESIAN_POINT('Ctrl Pts',(-23.1595514395656,68.9984408270659,
12.));
#156786=CARTESIAN_POINT('Ctrl Pts',(-23.1581765788869,69.0238291885245,
12.));
#156787=CARTESIAN_POINT('Ctrl Pts',(-23.1567755350469,69.0492554078992,
12.));
#156788=CARTESIAN_POINT('Ctrl Pts',(-23.1553482598762,69.074719378928,12.));
#156789=CARTESIAN_POINT('Ctrl Pts',(-23.1538947054614,69.1002209957025,
12.));
#156790=CARTESIAN_POINT('Ctrl Pts',(-23.152414824141,69.1257601526687,12.));
#156791=CARTESIAN_POINT('Ctrl Pts',(-23.1509085685032,69.1513367446231,
12.));
#156792=CARTESIAN_POINT('Ctrl Pts',(-23.1493758913858,69.1769506667084,
12.));
#156793=CARTESIAN_POINT('Ctrl Pts',(-23.147816745879,69.2026018144028,12.));
#156794=CARTESIAN_POINT('Ctrl Pts',(-23.1462310853206,69.2282900835236,
12.));
#156795=CARTESIAN_POINT('Ctrl Pts',(-23.1446188632931,69.254015370231,12.));
#156796=CARTESIAN_POINT('Ctrl Pts',(-23.142980033622,69.2797775710273,12.));
#156797=CARTESIAN_POINT('Ctrl Pts',(-23.1413145503762,69.3055765827546,
12.));
#156798=CARTESIAN_POINT('Ctrl Pts',(-23.1396223678725,69.3314123025869,
12.));
#156799=CARTESIAN_POINT('Ctrl Pts',(-23.1379034406718,69.3572846280297,
12.));
#156800=CARTESIAN_POINT('Ctrl Pts',(-23.1361577235709,69.3831934569183,
12.));
#156801=CARTESIAN_POINT('Ctrl Pts',(-23.1343851715989,69.4091386874132,
12.));
#156802=CARTESIAN_POINT('Ctrl Pts',(-23.1325857400144,69.4351202179946,
12.));
#156803=CARTESIAN_POINT('Ctrl Pts',(-23.1307593843061,69.4611379474484,
12.));
#156804=CARTESIAN_POINT('Ctrl Pts',(-23.1289060601924,69.4871917748654,
12.));
#156805=CARTESIAN_POINT('Ctrl Pts',(-23.1270257236204,69.5132815996537,
12.));
#156806=CARTESIAN_POINT('Ctrl Pts',(-23.1251183307676,69.539407321546,12.));
#156807=CARTESIAN_POINT('Ctrl Pts',(-23.1231838380452,69.5655688406052,
12.));
#156808=CARTESIAN_POINT('Ctrl Pts',(-23.1212222021051,69.5917660572265,
12.));
#156809=CARTESIAN_POINT('Ctrl Pts',(-23.1192333798441,69.6179988721365,
12.));
#156810=CARTESIAN_POINT('Ctrl Pts',(-23.1172173283859,69.6442671863765,
12.));
#156811=CARTESIAN_POINT('Ctrl Pts',(-23.1151740050681,69.6705709012852,
12.));
#156812=CARTESIAN_POINT('Ctrl Pts',(-23.1131033674301,69.6969099184767,
12.));
#156813=CARTESIAN_POINT('Ctrl Pts',(-23.1110053732046,69.7232841398197,
12.));
#156814=CARTESIAN_POINT('Ctrl Pts',(-23.1088799803089,69.7496934674069,
12.));
#156815=CARTESIAN_POINT('Ctrl Pts',(-23.106727146861,69.7761378035964,12.));
#156816=CARTESIAN_POINT('Ctrl Pts',(-23.1045468311991,69.8026170510572,
12.));
#156817=CARTESIAN_POINT('Ctrl Pts',(-23.1023389919051,69.8291311128118,
12.));
#156818=CARTESIAN_POINT('Ctrl Pts',(-23.1001035878241,69.8556798922693,
12.));
#156819=CARTESIAN_POINT('Ctrl Pts',(-23.0978405781021,69.8822632932768,
12.));
#156820=CARTESIAN_POINT('Ctrl Pts',(-23.0955499221558,69.9088812200713,
12.));
#156821=CARTESIAN_POINT('Ctrl Pts',(-23.0932315796067,69.9355335771729,
12.));
#156822=CARTESIAN_POINT('Ctrl Pts',(-23.0908855102251,69.9622202692873,
12.));
#156823=CARTESIAN_POINT('Ctrl Pts',(-23.0885116738798,69.9889412012143,
12.));
#156824=CARTESIAN_POINT('Ctrl Pts',(-23.0861100304729,70.0156962777169,
12.));
#156825=CARTESIAN_POINT('Ctrl Pts',(-23.0836805399374,70.0424854035115,
12.));
#156826=CARTESIAN_POINT('Ctrl Pts',(-23.0812231623765,70.0693084835373,
12.));
#156827=CARTESIAN_POINT('Ctrl Pts',(-23.0787378581774,70.0961654231639,
12.));
#156828=CARTESIAN_POINT('Ctrl Pts',(-23.0762245881389,70.123056128422,12.));
#156829=CARTESIAN_POINT('Ctrl Pts',(-23.0736833135938,70.1499805062172,
12.));
#156830=CARTESIAN_POINT('Ctrl Pts',(-23.0711139965439,70.1769384645586,
12.));
#156831=CARTESIAN_POINT('Ctrl Pts',(-23.0685165993691,70.2039299120488,
12.));
#156832=CARTESIAN_POINT('Ctrl Pts',(-23.0658910845433,70.2309547573815,
12.));
#156833=CARTESIAN_POINT('Ctrl Pts',(-23.0632374143279,70.2580129087888,
12.));
#156834=CARTESIAN_POINT('Ctrl Pts',(-23.0605555505321,70.2851042736066,
12.));
#156835=CARTESIAN_POINT('Ctrl Pts',(-23.0578454541104,70.3122287575335,
12.));
#156836=CARTESIAN_POINT('Ctrl Pts',(-23.0551070854926,70.3393862652297,
12.));
#156837=CARTESIAN_POINT('Ctrl Pts',(-23.0523404053172,70.3665767016542,
12.));
#156838=CARTESIAN_POINT('Ctrl Pts',(-23.0495453750763,70.3937999732267,
12.));
#156839=CARTESIAN_POINT('Ctrl Pts',(-23.0467219577291,70.4210559889348,
12.));
#156840=CARTESIAN_POINT('Ctrl Pts',(-23.0438701185013,70.4483446617614,
12.));
#156841=CARTESIAN_POINT('Ctrl Pts',(-23.0409898250756,70.4756659090209,
12.));
#156842=CARTESIAN_POINT('Ctrl Pts',(-23.0384964376036,70.4991133648946,
12.));
#156843=CARTESIAN_POINT('Ctrl Pts',(-23.0365694096173,70.5171075702746,
12.));
#156844=CARTESIAN_POINT('Ctrl Pts',(-23.0352213647765,70.5296341535555,
12.));
#156845=CARTESIAN_POINT('Ctrl Pts',(-23.0344606623299,70.536683638166,12.));
#156846=CARTESIAN_POINT('Ctrl Pts',(-23.0342913834073,70.5382514078919,
12.));
#156847=CARTESIAN_POINT('',(-23.1372951448024,66.0656156664138,0.));
#156848=CARTESIAN_POINT('',(-23.1372951448024,66.0656156664138,0.));
#156849=CARTESIAN_POINT('Ctrl Pts',(-23.0342913834073,70.5382514078919,
0.));
#156850=CARTESIAN_POINT('Ctrl Pts',(-23.0344606623299,70.536683638166,0.));
#156851=CARTESIAN_POINT('Ctrl Pts',(-23.0352213647765,70.5296341535555,
0.));
#156852=CARTESIAN_POINT('Ctrl Pts',(-23.0365694096173,70.5171075702746,
0.));
#156853=CARTESIAN_POINT('Ctrl Pts',(-23.0384964376036,70.4991133648946,
0.));
#156854=CARTESIAN_POINT('Ctrl Pts',(-23.0409898250756,70.4756659090209,
0.));
#156855=CARTESIAN_POINT('Ctrl Pts',(-23.0438701185013,70.4483446617614,
0.));
#156856=CARTESIAN_POINT('Ctrl Pts',(-23.0467219577291,70.4210559889348,
0.));
#156857=CARTESIAN_POINT('Ctrl Pts',(-23.0495453750763,70.3937999732267,
0.));
#156858=CARTESIAN_POINT('Ctrl Pts',(-23.0523404053172,70.3665767016542,
0.));
#156859=CARTESIAN_POINT('Ctrl Pts',(-23.0551070854926,70.3393862652297,
0.));
#156860=CARTESIAN_POINT('Ctrl Pts',(-23.0578454541104,70.3122287575335,
0.));
#156861=CARTESIAN_POINT('Ctrl Pts',(-23.0605555505321,70.2851042736066,
0.));
#156862=CARTESIAN_POINT('Ctrl Pts',(-23.0632374143279,70.2580129087888,
0.));
#156863=CARTESIAN_POINT('Ctrl Pts',(-23.0658910845433,70.2309547573815,
0.));
#156864=CARTESIAN_POINT('Ctrl Pts',(-23.0685165993691,70.2039299120488,
0.));
#156865=CARTESIAN_POINT('Ctrl Pts',(-23.0711139965439,70.1769384645586,
0.));
#156866=CARTESIAN_POINT('Ctrl Pts',(-23.0736833135938,70.1499805062172,
0.));
#156867=CARTESIAN_POINT('Ctrl Pts',(-23.0762245881389,70.123056128422,0.));
#156868=CARTESIAN_POINT('Ctrl Pts',(-23.0787378581774,70.0961654231639,
0.));
#156869=CARTESIAN_POINT('Ctrl Pts',(-23.0812231623765,70.0693084835373,
0.));
#156870=CARTESIAN_POINT('Ctrl Pts',(-23.0836805399374,70.0424854035115,
0.));
#156871=CARTESIAN_POINT('Ctrl Pts',(-23.0861100304729,70.0156962777169,
0.));
#156872=CARTESIAN_POINT('Ctrl Pts',(-23.0885116738798,69.9889412012143,
0.));
#156873=CARTESIAN_POINT('Ctrl Pts',(-23.0908855102251,69.9622202692873,
0.));
#156874=CARTESIAN_POINT('Ctrl Pts',(-23.0932315796067,69.9355335771729,
0.));
#156875=CARTESIAN_POINT('Ctrl Pts',(-23.0955499221558,69.9088812200713,
0.));
#156876=CARTESIAN_POINT('Ctrl Pts',(-23.0978405781021,69.8822632932768,
0.));
#156877=CARTESIAN_POINT('Ctrl Pts',(-23.1001035878241,69.8556798922693,
0.));
#156878=CARTESIAN_POINT('Ctrl Pts',(-23.1023389919051,69.8291311128118,
0.));
#156879=CARTESIAN_POINT('Ctrl Pts',(-23.1045468311991,69.8026170510572,
0.));
#156880=CARTESIAN_POINT('Ctrl Pts',(-23.106727146861,69.7761378035964,0.));
#156881=CARTESIAN_POINT('Ctrl Pts',(-23.1088799803089,69.7496934674069,
0.));
#156882=CARTESIAN_POINT('Ctrl Pts',(-23.1110053732046,69.7232841398197,
0.));
#156883=CARTESIAN_POINT('Ctrl Pts',(-23.1131033674301,69.6969099184767,
0.));
#156884=CARTESIAN_POINT('Ctrl Pts',(-23.1151740050681,69.6705709012852,
0.));
#156885=CARTESIAN_POINT('Ctrl Pts',(-23.1172173283859,69.6442671863765,
0.));
#156886=CARTESIAN_POINT('Ctrl Pts',(-23.1192333798441,69.6179988721365,
0.));
#156887=CARTESIAN_POINT('Ctrl Pts',(-23.1212222021051,69.5917660572265,
0.));
#156888=CARTESIAN_POINT('Ctrl Pts',(-23.1231838380452,69.5655688406052,
0.));
#156889=CARTESIAN_POINT('Ctrl Pts',(-23.1251183307676,69.539407321546,0.));
#156890=CARTESIAN_POINT('Ctrl Pts',(-23.1270257236204,69.5132815996537,
0.));
#156891=CARTESIAN_POINT('Ctrl Pts',(-23.1289060601924,69.4871917748654,
0.));
#156892=CARTESIAN_POINT('Ctrl Pts',(-23.1307593843061,69.4611379474484,
0.));
#156893=CARTESIAN_POINT('Ctrl Pts',(-23.1325857400144,69.4351202179946,
0.));
#156894=CARTESIAN_POINT('Ctrl Pts',(-23.1343851715989,69.4091386874132,
0.));
#156895=CARTESIAN_POINT('Ctrl Pts',(-23.1361577235709,69.3831934569183,
0.));
#156896=CARTESIAN_POINT('Ctrl Pts',(-23.1379034406718,69.3572846280297,
0.));
#156897=CARTESIAN_POINT('Ctrl Pts',(-23.1396223678725,69.3314123025869,
0.));
#156898=CARTESIAN_POINT('Ctrl Pts',(-23.1413145503762,69.3055765827546,
0.));
#156899=CARTESIAN_POINT('Ctrl Pts',(-23.142980033622,69.2797775710273,0.));
#156900=CARTESIAN_POINT('Ctrl Pts',(-23.1446188632931,69.254015370231,0.));
#156901=CARTESIAN_POINT('Ctrl Pts',(-23.1462310853206,69.2282900835236,
0.));
#156902=CARTESIAN_POINT('Ctrl Pts',(-23.147816745879,69.2026018144028,0.));
#156903=CARTESIAN_POINT('Ctrl Pts',(-23.1493758913858,69.1769506667084,
0.));
#156904=CARTESIAN_POINT('Ctrl Pts',(-23.1509085685032,69.1513367446231,
0.));
#156905=CARTESIAN_POINT('Ctrl Pts',(-23.152414824141,69.1257601526687,0.));
#156906=CARTESIAN_POINT('Ctrl Pts',(-23.1538947054614,69.1002209957025,
0.));
#156907=CARTESIAN_POINT('Ctrl Pts',(-23.1553482598762,69.074719378928,0.));
#156908=CARTESIAN_POINT('Ctrl Pts',(-23.1567755350469,69.0492554078992,
0.));
#156909=CARTESIAN_POINT('Ctrl Pts',(-23.1581765788869,69.0238291885245,
0.));
#156910=CARTESIAN_POINT('Ctrl Pts',(-23.1595514395656,68.9984408270659,
0.));
#156911=CARTESIAN_POINT('Ctrl Pts',(-23.1609001655156,68.9730904301369,
0.));
#156912=CARTESIAN_POINT('Ctrl Pts',(-23.1622228054291,68.9477781047106,
0.));
#156913=CARTESIAN_POINT('Ctrl Pts',(-23.1635194082581,68.9225039581248,
0.));
#156914=CARTESIAN_POINT('Ctrl Pts',(-23.164790023215,68.8972680980842,0.));
#156915=CARTESIAN_POINT('Ctrl Pts',(-23.1660346997764,68.8720706326609,
0.));
#156916=CARTESIAN_POINT('Ctrl Pts',(-23.1672534876889,68.8469116702898,
0.));
#156917=CARTESIAN_POINT('Ctrl Pts',(-23.1684464369686,68.8217913197752,
0.));
#156918=CARTESIAN_POINT('Ctrl Pts',(-23.1696135978997,68.7967096902996,
0.));
#156919=CARTESIAN_POINT('Ctrl Pts',(-23.170755021036,68.771666891425,0.));
#156920=CARTESIAN_POINT('Ctrl Pts',(-23.1718707572043,68.746663033096,0.));
#156921=CARTESIAN_POINT('Ctrl Pts',(-23.172960857511,68.7216982256341,0.));
#156922=CARTESIAN_POINT('Ctrl Pts',(-23.1740253733417,68.696772579744,0.));
#156923=CARTESIAN_POINT('Ctrl Pts',(-23.1750643563601,68.6718862065216,
0.));
#156924=CARTESIAN_POINT('Ctrl Pts',(-23.1760778585092,68.6470392174564,
0.));
#156925=CARTESIAN_POINT('Ctrl Pts',(-23.1770659320138,68.6222317244341,
0.));
#156926=CARTESIAN_POINT('Ctrl Pts',(-23.1780286293875,68.597463839733,0.));
#156927=CARTESIAN_POINT('Ctrl Pts',(-23.1789660034342,68.5727356760278,
0.));
#156928=CARTESIAN_POINT('Ctrl Pts',(-23.179878107245,68.5480473463985,0.));
#156929=CARTESIAN_POINT('Ctrl Pts',(-23.180764994201,68.5233989643345,0.));
#156930=CARTESIAN_POINT('Ctrl Pts',(-23.1816267179751,68.4987906437356,
0.));
#156931=CARTESIAN_POINT('Ctrl Pts',(-23.1824633325385,68.4742224989099,
0.));
#156932=CARTESIAN_POINT('Ctrl Pts',(-23.183274892163,68.4496946445758,0.));
#156933=CARTESIAN_POINT('Ctrl Pts',(-23.1840614514192,68.4252071958729,
0.));
#156934=CARTESIAN_POINT('Ctrl Pts',(-23.1848230651776,68.4007602683652,
0.));
#156935=CARTESIAN_POINT('Ctrl Pts',(-23.1855597886116,68.376353978044,0.));
#156936=CARTESIAN_POINT('Ctrl Pts',(-23.186271677203,68.3519884413246,0.));
#156937=CARTESIAN_POINT('Ctrl Pts',(-23.1869587867459,68.3276637750485,
0.));
#156938=CARTESIAN_POINT('Ctrl Pts',(-23.1876211733436,68.3033800964939,
0.));
#156939=CARTESIAN_POINT('Ctrl Pts',(-23.1882588934107,68.2791375233795,
0.));
#156940=CARTESIAN_POINT('Ctrl Pts',(-23.1888720036757,68.2549361738681,
0.));
#156941=CARTESIAN_POINT('Ctrl Pts',(-23.1894605611871,68.2307761665633,
0.));
#156942=CARTESIAN_POINT('Ctrl Pts',(-23.1900246233165,68.2066576205116,
0.));
#156943=CARTESIAN_POINT('Ctrl Pts',(-23.1905642477571,68.1825806552129,
0.));
#156944=CARTESIAN_POINT('Ctrl Pts',(-23.1910794925251,68.1585453906257,
0.));
#156945=CARTESIAN_POINT('Ctrl Pts',(-23.1915704159623,68.1345519471695,
0.));
#156946=CARTESIAN_POINT('Ctrl Pts',(-23.1920370767425,68.110600445723,0.));
#156947=CARTESIAN_POINT('Ctrl Pts',(-23.1924795338749,68.0866910076251,
0.));
#156948=CARTESIAN_POINT('Ctrl Pts',(-23.1928978467021,68.0628237546863,
0.));
#156949=CARTESIAN_POINT('Ctrl Pts',(-23.1932920749023,68.0389988091933,
0.));
#156950=CARTESIAN_POINT('Ctrl Pts',(-23.1936622784919,68.0152162939121,
0.));
#156951=CARTESIAN_POINT('Ctrl Pts',(-23.1940085178313,67.991476332086,0.));
#156952=CARTESIAN_POINT('Ctrl Pts',(-23.1943308536297,67.9677790474385,
0.));
#156953=CARTESIAN_POINT('Ctrl Pts',(-23.1946293469427,67.9441245641842,
0.));
#156954=CARTESIAN_POINT('Ctrl Pts',(-23.1949040591744,67.9205130070324,
0.));
#156955=CARTESIAN_POINT('Ctrl Pts',(-23.1951550520802,67.8969445011916,
0.));
#156956=CARTESIAN_POINT('Ctrl Pts',(-23.1953823877734,67.8734191723667,
0.));
#156957=CARTESIAN_POINT('Ctrl Pts',(-23.1955861287286,67.8499371467616,
0.));
#156958=CARTESIAN_POINT('Ctrl Pts',(-23.1957663377806,67.8264985510917,
0.));
#156959=CARTESIAN_POINT('Ctrl Pts',(-23.1959230781269,67.8031035125887,
0.));
#156960=CARTESIAN_POINT('Ctrl Pts',(-23.1960564133304,67.7797521590045,
0.));
#156961=CARTESIAN_POINT('Ctrl Pts',(-23.1961664073262,67.7564446186079,
0.));
#156962=CARTESIAN_POINT('Ctrl Pts',(-23.1962531244245,67.7331810201883,
0.));
#156963=CARTESIAN_POINT('Ctrl Pts',(-23.1963166293102,67.7099614930671,
0.));
#156964=CARTESIAN_POINT('Ctrl Pts',(-23.1963569870451,67.6867861671031,
0.));
#156965=CARTESIAN_POINT('Ctrl Pts',(-23.1963742630714,67.6636551726964,
0.));
#156966=CARTESIAN_POINT('Ctrl Pts',(-23.1963685232187,67.6405686407863,
0.));
#156967=CARTESIAN_POINT('Ctrl Pts',(-23.1963398337068,67.6175267028555,
0.));
#156968=CARTESIAN_POINT('Ctrl Pts',(-23.1962882611453,67.5945294909426,
0.));
#156969=CARTESIAN_POINT('Ctrl Pts',(-23.196213872536,67.5715771376461,0.));
#156970=CARTESIAN_POINT('Ctrl Pts',(-23.1961167352772,67.5486697761288,
0.));
#156971=CARTESIAN_POINT('Ctrl Pts',(-23.1959969171701,67.5258075401146,
0.));
#156972=CARTESIAN_POINT('Ctrl Pts',(-23.1958544864215,67.5029905638949,
0.));
#156973=CARTESIAN_POINT('Ctrl Pts',(-23.195689511644,67.4802189823408,0.));
#156974=CARTESIAN_POINT('Ctrl Pts',(-23.195502061859,67.4574929309076,0.));
#156975=CARTESIAN_POINT('Ctrl Pts',(-23.1952922065012,67.4348125456398,
0.));
#156976=CARTESIAN_POINT('Ctrl Pts',(-23.1950600154265,67.412177963168,0.));
#156977=CARTESIAN_POINT('Ctrl Pts',(-23.1948055589129,67.3895893207182,
0.));
#156978=CARTESIAN_POINT('Ctrl Pts',(-23.194528907661,67.3670467561212,0.));
#156979=CARTESIAN_POINT('Ctrl Pts',(-23.1942301327978,67.3445504078176,
0.));
#156980=CARTESIAN_POINT('Ctrl Pts',(-23.1939093058801,67.3221004148603,
0.));
#156981=CARTESIAN_POINT('Ctrl Pts',(-23.1935664989018,67.2996969169098,
0.));
#156982=CARTESIAN_POINT('Ctrl Pts',(-23.1932017842953,67.2773400542477,
0.));
#156983=CARTESIAN_POINT('Ctrl Pts',(-23.1928152349343,67.2550299677888,
0.));
#156984=CARTESIAN_POINT('Ctrl Pts',(-23.1924069241385,67.232766799088,0.));
#156985=CARTESIAN_POINT('Ctrl Pts',(-23.1919769256803,67.2105506903447,
0.));
#156986=CARTESIAN_POINT('Ctrl Pts',(-23.1915253137924,67.1883817844038,
0.));
#156987=CARTESIAN_POINT('Ctrl Pts',(-23.1910521631657,67.1662602247639,
0.));
#156988=CARTESIAN_POINT('Ctrl Pts',(-23.1905575489504,67.1441861555817,
0.));
#156989=CARTESIAN_POINT('Ctrl Pts',(-23.1900415467574,67.1221597216741,
0.));
#156990=CARTESIAN_POINT('Ctrl Pts',(-23.1895042326626,67.1001810685143,
0.));
#156991=CARTESIAN_POINT('Ctrl Pts',(-23.1889456832119,67.0782503422305,
0.));
#156992=CARTESIAN_POINT('Ctrl Pts',(-23.1883659754271,67.0563676896325,
0.));
#156993=CARTESIAN_POINT('Ctrl Pts',(-23.1877651868158,67.0345332582306,
0.));
#156994=CARTESIAN_POINT('Ctrl Pts',(-23.1871433953793,67.0127471962501,
0.));
#156995=CARTESIAN_POINT('Ctrl Pts',(-23.1865006796283,66.9910096526462,
0.));
#156996=CARTESIAN_POINT('Ctrl Pts',(-23.1858371185842,66.9693207771031,
0.));
#156997=CARTESIAN_POINT('Ctrl Pts',(-23.1851527917657,66.9476807200203,
0.));
#156998=CARTESIAN_POINT('Ctrl Pts',(-23.1844477791814,66.9260896324949,
0.));
#156999=CARTESIAN_POINT('Ctrl Pts',(-23.1837221613235,66.9045476663063,
0.));
#157000=CARTESIAN_POINT('Ctrl Pts',(-23.1829760191591,66.8830549738795,
0.));
#157001=CARTESIAN_POINT('Ctrl Pts',(-23.1822094341517,66.8616117083331,
0.));
#157002=CARTESIAN_POINT('Ctrl Pts',(-23.1814224882953,66.8402180235566,
0.));
#157003=CARTESIAN_POINT('Ctrl Pts',(-23.1806152641475,66.8188740742727,
0.));
#157004=CARTESIAN_POINT('Ctrl Pts',(-23.1797878448639,66.7975800161,0.));
#157005=CARTESIAN_POINT('Ctrl Pts',(-23.1789403142366,66.776336005612,0.));
#157006=CARTESIAN_POINT('Ctrl Pts',(-23.17807275663,66.7551422002204,0.));
#157007=CARTESIAN_POINT('Ctrl Pts',(-23.1771852569131,66.7339987580427,
0.));
#157008=CARTESIAN_POINT('Ctrl Pts',(-23.1762779004044,66.7129058377896,
0.));
#157009=CARTESIAN_POINT('Ctrl Pts',(-23.1753507727939,66.6918635985972,
0.));
#157010=CARTESIAN_POINT('Ctrl Pts',(-23.1744039601382,66.6708722000079,
0.));
#157011=CARTESIAN_POINT('Ctrl Pts',(-23.1734375490431,66.6499318023473,
0.));
#157012=CARTESIAN_POINT('Ctrl Pts',(-23.1724516268302,66.6290425670548,
0.));
#157013=CARTESIAN_POINT('Ctrl Pts',(-23.1714462816789,66.6082046569644,
0.));
#157014=CARTESIAN_POINT('Ctrl Pts',(-23.1704216028614,66.5874182367563,
0.));
#157015=CARTESIAN_POINT('Ctrl Pts',(-23.1693776805866,66.5666834726454,
0.));
#157016=CARTESIAN_POINT('Ctrl Pts',(-23.1683146055726,66.5460005315376,
0.));
#157017=CARTESIAN_POINT('Ctrl Pts',(-23.1672324686926,66.5253695803205,
0.));
#157018=CARTESIAN_POINT('Ctrl Pts',(-23.1661313606132,66.5047907851348,
0.));
#157019=CARTESIAN_POINT('Ctrl Pts',(-23.1650113713808,66.4842643105311,
0.));
#157020=CARTESIAN_POINT('Ctrl Pts',(-23.1638725912195,66.4637903210727,
0.));
#157021=CARTESIAN_POINT('Ctrl Pts',(-23.1627151114883,66.4433689832478,
0.));
#157022=CARTESIAN_POINT('Ctrl Pts',(-23.1615390254632,66.4230004670278,
0.));
#157023=CARTESIAN_POINT('Ctrl Pts',(-23.160344429474,66.4026849481232,0.));
#157024=CARTESIAN_POINT('Ctrl Pts',(-23.1591314230083,66.3824226081802,
0.));
#157025=CARTESIAN_POINT('Ctrl Pts',(-23.1579001063424,66.3622136300654,
0.));
#157026=CARTESIAN_POINT('Ctrl Pts',(-23.1566505784621,66.3420581937147,
0.));
#157027=CARTESIAN_POINT('Ctrl Pts',(-23.1553829352539,66.3219564725184,
0.));
#157028=CARTESIAN_POINT('Ctrl Pts',(-23.1540972666191,66.3019086275444,
0.));
#157029=CARTESIAN_POINT('Ctrl Pts',(-23.1527936592651,66.281914813114,0.));
#157030=CARTESIAN_POINT('Ctrl Pts',(-23.1514722022503,66.2619751878793,
0.));
#157031=CARTESIAN_POINT('Ctrl Pts',(-23.1501329914487,66.2420899237318,
0.));
#157032=CARTESIAN_POINT('Ctrl Pts',(-23.1487761349298,66.2222592165398,
0.));
#157033=CARTESIAN_POINT('Ctrl Pts',(-23.147401756643,66.2024832934733,0.));
#157034=CARTESIAN_POINT('Ctrl Pts',(-23.1460099850704,66.1827623902755,
0.));
#157035=CARTESIAN_POINT('Ctrl Pts',(-23.1446009424871,66.163096729667,0.));
#157036=CARTESIAN_POINT('Ctrl Pts',(-23.1431747350127,66.14348650151,0.));
#157037=CARTESIAN_POINT('Ctrl Pts',(-23.1417314398501,66.1239318368803,
0.));
#157038=CARTESIAN_POINT('Ctrl Pts',(-23.140271103958,66.1044328067739,0.));
#157039=CARTESIAN_POINT('Ctrl Pts',(-23.1390892229923,66.0888781152779,
0.));
#157040=CARTESIAN_POINT('Ctrl Pts',(-23.1381951597491,66.0772371487475,
0.));
#157041=CARTESIAN_POINT('Ctrl Pts',(-23.1375957166138,66.0694876382212,
0.));
#157042=CARTESIAN_POINT('Ctrl Pts',(-23.1372951448024,66.0656156664138,
0.));
#157043=CARTESIAN_POINT('Ctrl Pts',(-16.7341474417544,72.5962692526112,
0.));
#157044=CARTESIAN_POINT('Ctrl Pts',(-16.7341474417544,72.5962692526112,
12.));
#157045=CARTESIAN_POINT('Ctrl Pts',(-16.7352885767485,72.5907910746008,
0.));
#157046=CARTESIAN_POINT('Ctrl Pts',(-16.7352885767485,72.5907910746008,
12.));
#157047=CARTESIAN_POINT('Ctrl Pts',(-16.7375676985344,72.5798376087774,
0.));
#157048=CARTESIAN_POINT('Ctrl Pts',(-16.7375676985344,72.5798376087774,
12.));
#157049=CARTESIAN_POINT('Ctrl Pts',(-16.7409769366072,72.5634160806351,
0.));
#157050=CARTESIAN_POINT('Ctrl Pts',(-16.7409769366072,72.5634160806351,
12.));
#157051=CARTESIAN_POINT('Ctrl Pts',(-16.7455036973866,72.5415380516637,
0.));
#157052=CARTESIAN_POINT('Ctrl Pts',(-16.7455036973866,72.5415380516637,
12.));
#157053=CARTESIAN_POINT('Ctrl Pts',(-16.7511306618915,72.514219427383,0.));
#157054=CARTESIAN_POINT('Ctrl Pts',(-16.7511306618915,72.514219427383,12.));
#157055=CARTESIAN_POINT('Ctrl Pts',(-16.7567261380687,72.4869297342427,
0.));
#157056=CARTESIAN_POINT('Ctrl Pts',(-16.7567261380687,72.4869297342427,
12.));
#157057=CARTESIAN_POINT('Ctrl Pts',(-16.7622901280758,72.4596690055437,
0.));
#157058=CARTESIAN_POINT('Ctrl Pts',(-16.7622901280758,72.4596690055437,
12.));
#157059=CARTESIAN_POINT('Ctrl Pts',(-16.7678226404162,72.4324372916746,
0.));
#157060=CARTESIAN_POINT('Ctrl Pts',(-16.7678226404162,72.4324372916746,
12.));
#157061=CARTESIAN_POINT('Ctrl Pts',(-16.7733236932135,72.4052346647799,
0.));
#157062=CARTESIAN_POINT('Ctrl Pts',(-16.7733236932135,72.4052346647799,
12.));
#157063=CARTESIAN_POINT('Ctrl Pts',(-16.7787933137498,72.3780612167786,
0.));
#157064=CARTESIAN_POINT('Ctrl Pts',(-16.7787933137498,72.3780612167786,
12.));
#157065=CARTESIAN_POINT('Ctrl Pts',(-16.7842315351363,72.3509170522838,
0.));
#157066=CARTESIAN_POINT('Ctrl Pts',(-16.7842315351363,72.3509170522838,
12.));
#157067=CARTESIAN_POINT('Ctrl Pts',(-16.7896383937822,72.3238022829223,
0.));
#157068=CARTESIAN_POINT('Ctrl Pts',(-16.7896383937822,72.3238022829223,
12.));
#157069=CARTESIAN_POINT('Ctrl Pts',(-16.7950139266122,72.2967170212353,
0.));
#157070=CARTESIAN_POINT('Ctrl Pts',(-16.7950139266122,72.2967170212353,
12.));
#157071=CARTESIAN_POINT('Ctrl Pts',(-16.8003581682248,72.2696613743782,
0.));
#157072=CARTESIAN_POINT('Ctrl Pts',(-16.8003581682248,72.2696613743782,
12.));
#157073=CARTESIAN_POINT('Ctrl Pts',(-16.8056711485821,72.2426354390213,
0.));
#157074=CARTESIAN_POINT('Ctrl Pts',(-16.8056711485821,72.2426354390213,
12.));
#157075=CARTESIAN_POINT('Ctrl Pts',(-16.8109528945896,72.2156393048975,
0.));
#157076=CARTESIAN_POINT('Ctrl Pts',(-16.8109528945896,72.2156393048975,
12.));
#157077=CARTESIAN_POINT('Ctrl Pts',(-16.8162034312269,72.1886730573452,
0.));
#157078=CARTESIAN_POINT('Ctrl Pts',(-16.8162034312269,72.1886730573452,
12.));
#157079=CARTESIAN_POINT('Ctrl Pts',(-16.8214227828943,72.1617367803235,
0.));
#157080=CARTESIAN_POINT('Ctrl Pts',(-16.8214227828943,72.1617367803235,
12.));
#157081=CARTESIAN_POINT('Ctrl Pts',(-16.8266109745795,72.13483055902,0.));
#157082=CARTESIAN_POINT('Ctrl Pts',(-16.8266109745795,72.13483055902,12.));
#157083=CARTESIAN_POINT('Ctrl Pts',(-16.8317680333404,72.1079544831513,
0.));
#157084=CARTESIAN_POINT('Ctrl Pts',(-16.8317680333404,72.1079544831513,
12.));
#157085=CARTESIAN_POINT('Ctrl Pts',(-16.8368939881446,72.0811086466121,
0.));
#157086=CARTESIAN_POINT('Ctrl Pts',(-16.8368939881446,72.0811086466121,
12.));
#157087=CARTESIAN_POINT('Ctrl Pts',(-16.8419888691976,72.0542931459825,
0.));
#157088=CARTESIAN_POINT('Ctrl Pts',(-16.8419888691976,72.0542931459825,
12.));
#157089=CARTESIAN_POINT('Ctrl Pts',(-16.8470527074275,72.0275080793727,
0.));
#157090=CARTESIAN_POINT('Ctrl Pts',(-16.8470527074275,72.0275080793727,
12.));
#157091=CARTESIAN_POINT('Ctrl Pts',(-16.8520855339446,72.0007535452081,
0.));
#157092=CARTESIAN_POINT('Ctrl Pts',(-16.8520855339446,72.0007535452081,
12.));
#157093=CARTESIAN_POINT('Ctrl Pts',(-16.8570873794269,71.9740296408347,
0.));
#157094=CARTESIAN_POINT('Ctrl Pts',(-16.8570873794269,71.9740296408347,
12.));
#157095=CARTESIAN_POINT('Ctrl Pts',(-16.8620582738437,71.9473364618922,
0.));
#157096=CARTESIAN_POINT('Ctrl Pts',(-16.8620582738437,71.9473364618922,
12.));
#157097=CARTESIAN_POINT('Ctrl Pts',(-16.866998246792,71.9206741030887,0.));
#157098=CARTESIAN_POINT('Ctrl Pts',(-16.866998246792,71.9206741030887,12.));
#157099=CARTESIAN_POINT('Ctrl Pts',(-16.871907327697,71.8940426586534,0.));
#157100=CARTESIAN_POINT('Ctrl Pts',(-16.871907327697,71.8940426586534,12.));
#157101=CARTESIAN_POINT('Ctrl Pts',(-16.87678554607,71.867442222915,0.));
#157102=CARTESIAN_POINT('Ctrl Pts',(-16.87678554607,71.867442222915,12.));
#157103=CARTESIAN_POINT('Ctrl Pts',(-16.881632931747,71.8408728908258,0.));
#157104=CARTESIAN_POINT('Ctrl Pts',(-16.881632931747,71.8408728908258,12.));
#157105=CARTESIAN_POINT('Ctrl Pts',(-16.8864495151344,71.8143347584962,
0.));
#157106=CARTESIAN_POINT('Ctrl Pts',(-16.8864495151344,71.8143347584962,
12.));
#157107=CARTESIAN_POINT('Ctrl Pts',(-16.8912353270942,71.7878279229546,
0.));
#157108=CARTESIAN_POINT('Ctrl Pts',(-16.8912353270942,71.7878279229546,
12.));
#157109=CARTESIAN_POINT('Ctrl Pts',(-16.895990398841,71.7613524819235,0.));
#157110=CARTESIAN_POINT('Ctrl Pts',(-16.895990398841,71.7613524819235,12.));
#157111=CARTESIAN_POINT('Ctrl Pts',(-16.9007147618344,71.7349085335796,
0.));
#157112=CARTESIAN_POINT('Ctrl Pts',(-16.9007147618344,71.7349085335796,
12.));
#157113=CARTESIAN_POINT('Ctrl Pts',(-16.9054084476847,71.7084961763357,
0.));
#157114=CARTESIAN_POINT('Ctrl Pts',(-16.9054084476847,71.7084961763357,
12.));
#157115=CARTESIAN_POINT('Ctrl Pts',(-16.9100714880368,71.6821155085612,
0.));
#157116=CARTESIAN_POINT('Ctrl Pts',(-16.9100714880368,71.6821155085612,
12.));
#157117=CARTESIAN_POINT('Ctrl Pts',(-16.9147039145717,71.6557666285917,
0.));
#157118=CARTESIAN_POINT('Ctrl Pts',(-16.9147039145717,71.6557666285917,
12.));
#157119=CARTESIAN_POINT('Ctrl Pts',(-16.9193057590607,71.6294496348653,
0.));
#157120=CARTESIAN_POINT('Ctrl Pts',(-16.9193057590607,71.6294496348653,
12.));
#157121=CARTESIAN_POINT('Ctrl Pts',(-16.9238770534071,71.6031646260174,
0.));
#157122=CARTESIAN_POINT('Ctrl Pts',(-16.9238770534071,71.6031646260174,
12.));
#157123=CARTESIAN_POINT('Ctrl Pts',(-16.9284178296933,71.5769117009842,
0.));
#157124=CARTESIAN_POINT('Ctrl Pts',(-16.9284178296933,71.5769117009842,
12.));
#157125=CARTESIAN_POINT('Ctrl Pts',(-16.9329281202377,71.5506909591129,
0.));
#157126=CARTESIAN_POINT('Ctrl Pts',(-16.9329281202377,71.5506909591129,
12.));
#157127=CARTESIAN_POINT('Ctrl Pts',(-16.9374079576201,71.5245025002139,
0.));
#157128=CARTESIAN_POINT('Ctrl Pts',(-16.9374079576201,71.5245025002139,
12.));
#157129=CARTESIAN_POINT('Ctrl Pts',(-16.9418573746489,71.4983464245055,
0.));
#157130=CARTESIAN_POINT('Ctrl Pts',(-16.9418573746489,71.4983464245055,
12.));
#157131=CARTESIAN_POINT('Ctrl Pts',(-16.9462764043443,71.4722228325794,
0.));
#157132=CARTESIAN_POINT('Ctrl Pts',(-16.9462764043443,71.4722228325794,
12.));
#157133=CARTESIAN_POINT('Ctrl Pts',(-16.9506650799189,71.4461318253563,
0.));
#157134=CARTESIAN_POINT('Ctrl Pts',(-16.9506650799189,71.4461318253563,
12.));
#157135=CARTESIAN_POINT('Ctrl Pts',(-16.9550234347621,71.4200735040384,
0.));
#157136=CARTESIAN_POINT('Ctrl Pts',(-16.9550234347621,71.4200735040384,
12.));
#157137=CARTESIAN_POINT('Ctrl Pts',(-16.9593515024276,71.3940479700677,
0.));
#157138=CARTESIAN_POINT('Ctrl Pts',(-16.9593515024276,71.3940479700677,
12.));
#157139=CARTESIAN_POINT('Ctrl Pts',(-16.9636493166397,71.3680553251562,
0.));
#157140=CARTESIAN_POINT('Ctrl Pts',(-16.9636493166397,71.3680553251562,
12.));
#157141=CARTESIAN_POINT('Ctrl Pts',(-16.9679169112994,71.3420956713082,
0.));
#157142=CARTESIAN_POINT('Ctrl Pts',(-16.9679169112994,71.3420956713082,
12.));
#157143=CARTESIAN_POINT('Ctrl Pts',(-16.9721543204951,71.3161691108427,
0.));
#157144=CARTESIAN_POINT('Ctrl Pts',(-16.9721543204951,71.3161691108427,
12.));
#157145=CARTESIAN_POINT('Ctrl Pts',(-16.9763615785137,71.290275746412,0.));
#157146=CARTESIAN_POINT('Ctrl Pts',(-16.9763615785137,71.290275746412,12.));
#157147=CARTESIAN_POINT('Ctrl Pts',(-16.9805387198571,71.2644156810198,
0.));
#157148=CARTESIAN_POINT('Ctrl Pts',(-16.9805387198571,71.2644156810198,
12.));
#157149=CARTESIAN_POINT('Ctrl Pts',(-16.9846857792384,71.2385890180221,
0.));
#157150=CARTESIAN_POINT('Ctrl Pts',(-16.9846857792384,71.2385890180221,
12.));
#157151=CARTESIAN_POINT('Ctrl Pts',(-16.9888027915742,71.212795861124,0.));
#157152=CARTESIAN_POINT('Ctrl Pts',(-16.9888027915742,71.212795861124,12.));
#157153=CARTESIAN_POINT('Ctrl Pts',(-16.9928897919828,71.187036314374,0.));
#157154=CARTESIAN_POINT('Ctrl Pts',(-16.9928897919828,71.187036314374,12.));
#157155=CARTESIAN_POINT('Ctrl Pts',(-16.9969468157824,71.1613104821568,
0.));
#157156=CARTESIAN_POINT('Ctrl Pts',(-16.9969468157824,71.1613104821568,
12.));
#157157=CARTESIAN_POINT('Ctrl Pts',(-17.0009738984936,71.1356184691806,
0.));
#157158=CARTESIAN_POINT('Ctrl Pts',(-17.0009738984936,71.1356184691806,
12.));
#157159=CARTESIAN_POINT('Ctrl Pts',(-17.0049710758394,71.1099603804786,
0.));
#157160=CARTESIAN_POINT('Ctrl Pts',(-17.0049710758394,71.1099603804786,
12.));
#157161=CARTESIAN_POINT('Ctrl Pts',(-17.0089383837437,71.0843363214221,
0.));
#157162=CARTESIAN_POINT('Ctrl Pts',(-17.0089383837437,71.0843363214221,
12.));
#157163=CARTESIAN_POINT('Ctrl Pts',(-17.0128758583335,71.0587463977268,
0.));
#157164=CARTESIAN_POINT('Ctrl Pts',(-17.0128758583335,71.0587463977268,
12.));
#157165=CARTESIAN_POINT('Ctrl Pts',(-17.0167835359419,71.0331907154574,
0.));
#157166=CARTESIAN_POINT('Ctrl Pts',(-17.0167835359419,71.0331907154574,
12.));
#157167=CARTESIAN_POINT('Ctrl Pts',(-17.0206614531166,71.0076693810301,
0.));
#157168=CARTESIAN_POINT('Ctrl Pts',(-17.0206614531166,71.0076693810301,
12.));
#157169=CARTESIAN_POINT('Ctrl Pts',(-17.0245096466229,70.9821825012136,
0.));
#157170=CARTESIAN_POINT('Ctrl Pts',(-17.0245096466229,70.9821825012136,
12.));
#157171=CARTESIAN_POINT('Ctrl Pts',(-17.0283281534392,70.956730183136,0.));
#157172=CARTESIAN_POINT('Ctrl Pts',(-17.0283281534392,70.956730183136,12.));
#157173=CARTESIAN_POINT('Ctrl Pts',(-17.0321170107564,70.9313125342876,
0.));
#157174=CARTESIAN_POINT('Ctrl Pts',(-17.0321170107564,70.9313125342876,
12.));
#157175=CARTESIAN_POINT('Ctrl Pts',(-17.0358762559786,70.9059296625214,
0.));
#157176=CARTESIAN_POINT('Ctrl Pts',(-17.0358762559786,70.9059296625214,
12.));
#157177=CARTESIAN_POINT('Ctrl Pts',(-17.0396059267277,70.8805816760501,
0.));
#157178=CARTESIAN_POINT('Ctrl Pts',(-17.0396059267277,70.8805816760501,
12.));
#157179=CARTESIAN_POINT('Ctrl Pts',(-17.0433060608475,70.8552686834423,
0.));
#157180=CARTESIAN_POINT('Ctrl Pts',(-17.0433060608475,70.8552686834423,
12.));
#157181=CARTESIAN_POINT('Ctrl Pts',(-17.0469766964001,70.8299907936334,
0.));
#157182=CARTESIAN_POINT('Ctrl Pts',(-17.0469766964001,70.8299907936334,
12.));
#157183=CARTESIAN_POINT('Ctrl Pts',(-17.0506178716662,70.8047481159298,
0.));
#157184=CARTESIAN_POINT('Ctrl Pts',(-17.0506178716662,70.8047481159298,
12.));
#157185=CARTESIAN_POINT('Ctrl Pts',(-17.0542296251462,70.7795407600127,
0.));
#157186=CARTESIAN_POINT('Ctrl Pts',(-17.0542296251462,70.7795407600127,
12.));
#157187=CARTESIAN_POINT('Ctrl Pts',(-17.0578119955651,70.754368835938,0.));
#157188=CARTESIAN_POINT('Ctrl Pts',(-17.0578119955651,70.754368835938,12.));
#157189=CARTESIAN_POINT('Ctrl Pts',(-17.0613650218789,70.7292324541348,
0.));
#157190=CARTESIAN_POINT('Ctrl Pts',(-17.0613650218789,70.7292324541348,
12.));
#157191=CARTESIAN_POINT('Ctrl Pts',(-17.0648887432714,70.7041317254128,
0.));
#157192=CARTESIAN_POINT('Ctrl Pts',(-17.0648887432714,70.7041317254128,
12.));
#157193=CARTESIAN_POINT('Ctrl Pts',(-17.0683831991532,70.6790667609678,
0.));
#157194=CARTESIAN_POINT('Ctrl Pts',(-17.0683831991532,70.6790667609678,
12.));
#157195=CARTESIAN_POINT('Ctrl Pts',(-17.0718484291623,70.6540376723839,
0.));
#157196=CARTESIAN_POINT('Ctrl Pts',(-17.0718484291623,70.6540376723839,
12.));
#157197=CARTESIAN_POINT('Ctrl Pts',(-17.0752844731679,70.6290445716341,
0.));
#157198=CARTESIAN_POINT('Ctrl Pts',(-17.0752844731679,70.6290445716341,
12.));
#157199=CARTESIAN_POINT('Ctrl Pts',(-17.0786913712767,70.6040875710762,
0.));
#157200=CARTESIAN_POINT('Ctrl Pts',(-17.0786913712767,70.6040875710762,
12.));
#157201=CARTESIAN_POINT('Ctrl Pts',(-17.0820691638314,70.5791667834599,
0.));
#157202=CARTESIAN_POINT('Ctrl Pts',(-17.0820691638314,70.5791667834599,
12.));
#157203=CARTESIAN_POINT('Ctrl Pts',(-17.085417891409,70.5542823219346,0.));
#157204=CARTESIAN_POINT('Ctrl Pts',(-17.085417891409,70.5542823219346,12.));
#157205=CARTESIAN_POINT('Ctrl Pts',(-17.0887375948221,70.5294343000516,
0.));
#157206=CARTESIAN_POINT('Ctrl Pts',(-17.0887375948221,70.5294343000516,
12.));
#157207=CARTESIAN_POINT('Ctrl Pts',(-17.0920283151217,70.5046228317669,
0.));
#157208=CARTESIAN_POINT('Ctrl Pts',(-17.0920283151217,70.5046228317669,
12.));
#157209=CARTESIAN_POINT('Ctrl Pts',(-17.0952900936044,70.4798480314364,
0.));
#157210=CARTESIAN_POINT('Ctrl Pts',(-17.0952900936044,70.4798480314364,
12.));
#157211=CARTESIAN_POINT('Ctrl Pts',(-17.098522971812,70.4551100138221,0.));
#157212=CARTESIAN_POINT('Ctrl Pts',(-17.098522971812,70.4551100138221,12.));
#157213=CARTESIAN_POINT('Ctrl Pts',(-17.1017269915289,70.4304088940998,
0.));
#157214=CARTESIAN_POINT('Ctrl Pts',(-17.1017269915289,70.4304088940998,
12.));
#157215=CARTESIAN_POINT('Ctrl Pts',(-17.1049021947833,70.4057447878621,
0.));
#157216=CARTESIAN_POINT('Ctrl Pts',(-17.1049021947833,70.4057447878621,
12.));
#157217=CARTESIAN_POINT('Ctrl Pts',(-17.10804862385,70.3811178111206,0.));
#157218=CARTESIAN_POINT('Ctrl Pts',(-17.10804862385,70.3811178111206,12.));
#157219=CARTESIAN_POINT('Ctrl Pts',(-17.111166321257,70.356528080303,0.));
#157220=CARTESIAN_POINT('Ctrl Pts',(-17.111166321257,70.356528080303,12.));
#157221=CARTESIAN_POINT('Ctrl Pts',(-17.1142553297869,70.3319757122577,
0.));
#157222=CARTESIAN_POINT('Ctrl Pts',(-17.1142553297869,70.3319757122577,
12.));
#157223=CARTESIAN_POINT('Ctrl Pts',(-17.1173156924734,70.3074608242613,
0.));
#157224=CARTESIAN_POINT('Ctrl Pts',(-17.1173156924734,70.3074608242613,
12.));
#157225=CARTESIAN_POINT('Ctrl Pts',(-17.1203474526031,70.2829835340239,
0.));
#157226=CARTESIAN_POINT('Ctrl Pts',(-17.1203474526031,70.2829835340239,
12.));
#157227=CARTESIAN_POINT('Ctrl Pts',(-17.1233506537176,70.2585439596899,
0.));
#157228=CARTESIAN_POINT('Ctrl Pts',(-17.1233506537176,70.2585439596899,
12.));
#157229=CARTESIAN_POINT('Ctrl Pts',(-17.1263253396202,70.2341422198363,
0.));
#157230=CARTESIAN_POINT('Ctrl Pts',(-17.1263253396202,70.2341422198363,
12.));
#157231=CARTESIAN_POINT('Ctrl Pts',(-17.1292715543779,70.2097784334749,
0.));
#157232=CARTESIAN_POINT('Ctrl Pts',(-17.1292715543779,70.2097784334749,
12.));
#157233=CARTESIAN_POINT('Ctrl Pts',(-17.1321893423183,70.1854527200636,
0.));
#157234=CARTESIAN_POINT('Ctrl Pts',(-17.1321893423183,70.1854527200636,
12.));
#157235=CARTESIAN_POINT('Ctrl Pts',(-17.1350787480313,70.1611651995085,
0.));
#157236=CARTESIAN_POINT('Ctrl Pts',(-17.1350787480313,70.1611651995085,
12.));
#157237=CARTESIAN_POINT('Ctrl Pts',(-17.1379398163708,70.1369159921686,
0.));
#157238=CARTESIAN_POINT('Ctrl Pts',(-17.1379398163708,70.1369159921686,
12.));
#157239=CARTESIAN_POINT('Ctrl Pts',(-17.1407725924615,70.1127052188515,
0.));
#157240=CARTESIAN_POINT('Ctrl Pts',(-17.1407725924615,70.1127052188515,
12.));
#157241=CARTESIAN_POINT('Ctrl Pts',(-17.1435771217015,70.0885330008169,
0.));
#157242=CARTESIAN_POINT('Ctrl Pts',(-17.1435771217015,70.0885330008169,
12.));
#157243=CARTESIAN_POINT('Ctrl Pts',(-17.1463534497592,70.0643994597865,
0.));
#157244=CARTESIAN_POINT('Ctrl Pts',(-17.1463534497592,70.0643994597865,
12.));
#157245=CARTESIAN_POINT('Ctrl Pts',(-17.1491016225748,70.0403047179481,
0.));
#157246=CARTESIAN_POINT('Ctrl Pts',(-17.1491016225748,70.0403047179481,
12.));
#157247=CARTESIAN_POINT('Ctrl Pts',(-17.1518216863624,70.0162488979587,
0.));
#157248=CARTESIAN_POINT('Ctrl Pts',(-17.1518216863624,70.0162488979587,
12.));
#157249=CARTESIAN_POINT('Ctrl Pts',(-17.1545136876162,69.9922321229428,
0.));
#157250=CARTESIAN_POINT('Ctrl Pts',(-17.1545136876162,69.9922321229428,
12.));
#157251=CARTESIAN_POINT('Ctrl Pts',(-17.157177673114,69.9682545164942,0.));
#157252=CARTESIAN_POINT('Ctrl Pts',(-17.157177673114,69.9682545164942,12.));
#157253=CARTESIAN_POINT('Ctrl Pts',(-17.1598136899144,69.9443162026865,
0.));
#157254=CARTESIAN_POINT('Ctrl Pts',(-17.1598136899144,69.9443162026865,
12.));
#157255=CARTESIAN_POINT('Ctrl Pts',(-17.1624217853577,69.9204173060779,
0.));
#157256=CARTESIAN_POINT('Ctrl Pts',(-17.1624217853577,69.9204173060779,
12.));
#157257=CARTESIAN_POINT('Ctrl Pts',(-17.1650020070686,69.8965579517147,
0.));
#157258=CARTESIAN_POINT('Ctrl Pts',(-17.1650020070686,69.8965579517147,
12.));
#157259=CARTESIAN_POINT('Ctrl Pts',(-17.1675544029622,69.8727382651292,
0.));
#157260=CARTESIAN_POINT('Ctrl Pts',(-17.1675544029622,69.8727382651292,
12.));
#157261=CARTESIAN_POINT('Ctrl Pts',(-17.1700790212476,69.8489583723417,
0.));
#157262=CARTESIAN_POINT('Ctrl Pts',(-17.1700790212476,69.8489583723417,
12.));
#157263=CARTESIAN_POINT('Ctrl Pts',(-17.1725759104254,69.8252183998713,
0.));
#157264=CARTESIAN_POINT('Ctrl Pts',(-17.1725759104254,69.8252183998713,
12.));
#157265=CARTESIAN_POINT('Ctrl Pts',(-17.1750451192887,69.8015184747404,
0.));
#157266=CARTESIAN_POINT('Ctrl Pts',(-17.1750451192887,69.8015184747404,
12.));
#157267=CARTESIAN_POINT('Ctrl Pts',(-17.1774866969256,69.7778587244788,
0.));
#157268=CARTESIAN_POINT('Ctrl Pts',(-17.1774866969256,69.7778587244788,
12.));
#157269=CARTESIAN_POINT('Ctrl Pts',(-17.1799006927256,69.7542392771216,
0.));
#157270=CARTESIAN_POINT('Ctrl Pts',(-17.1799006927256,69.7542392771216,
12.));
#157271=CARTESIAN_POINT('Ctrl Pts',(-17.1822871563835,69.7306602612125,
0.));
#157272=CARTESIAN_POINT('Ctrl Pts',(-17.1822871563835,69.7306602612125,
12.));
#157273=CARTESIAN_POINT('Ctrl Pts',(-17.1846461378966,69.7071218058149,
0.));
#157274=CARTESIAN_POINT('Ctrl Pts',(-17.1846461378966,69.7071218058149,
12.));
#157275=CARTESIAN_POINT('Ctrl Pts',(-17.1869776875663,69.6836240405152,
0.));
#157276=CARTESIAN_POINT('Ctrl Pts',(-17.1869776875663,69.6836240405152,
12.));
#157277=CARTESIAN_POINT('Ctrl Pts',(-17.1892818560004,69.6601670954277,
0.));
#157278=CARTESIAN_POINT('Ctrl Pts',(-17.1892818560004,69.6601670954277,
12.));
#157279=CARTESIAN_POINT('Ctrl Pts',(-17.1915586941198,69.6367511011927,
0.));
#157280=CARTESIAN_POINT('Ctrl Pts',(-17.1915586941198,69.6367511011927,
12.));
#157281=CARTESIAN_POINT('Ctrl Pts',(-17.193808253162,69.6133761889787,0.));
#157282=CARTESIAN_POINT('Ctrl Pts',(-17.193808253162,69.6133761889787,12.));
#157283=CARTESIAN_POINT('Ctrl Pts',(-17.1960305846787,69.5900424904954,
0.));
#157284=CARTESIAN_POINT('Ctrl Pts',(-17.1960305846787,69.5900424904954,
12.));
#157285=CARTESIAN_POINT('Ctrl Pts',(-17.198225740538,69.5667501379984,0.));
#157286=CARTESIAN_POINT('Ctrl Pts',(-17.198225740538,69.5667501379984,12.));
#157287=CARTESIAN_POINT('Ctrl Pts',(-17.2003937729266,69.5434992642932,
0.));
#157288=CARTESIAN_POINT('Ctrl Pts',(-17.2003937729266,69.5434992642932,
12.));
#157289=CARTESIAN_POINT('Ctrl Pts',(-17.2025347343568,69.5202900027329,
0.));
#157290=CARTESIAN_POINT('Ctrl Pts',(-17.2025347343568,69.5202900027329,
12.));
#157291=CARTESIAN_POINT('Ctrl Pts',(-17.2046486776697,69.497122487222,0.));
#157292=CARTESIAN_POINT('Ctrl Pts',(-17.2046486776697,69.497122487222,12.));
#157293=CARTESIAN_POINT('Ctrl Pts',(-17.2067356560326,69.4739968522271,
0.));
#157294=CARTESIAN_POINT('Ctrl Pts',(-17.2067356560326,69.4739968522271,
12.));
#157295=CARTESIAN_POINT('Ctrl Pts',(-17.208795722942,69.4509132327836,0.));
#157296=CARTESIAN_POINT('Ctrl Pts',(-17.208795722942,69.4509132327836,12.));
#157297=CARTESIAN_POINT('Ctrl Pts',(-17.2108289322258,69.4278717644989,
0.));
#157298=CARTESIAN_POINT('Ctrl Pts',(-17.2108289322258,69.4278717644989,
12.));
#157299=CARTESIAN_POINT('Ctrl Pts',(-17.2128353380511,69.4048725835516,
0.));
#157300=CARTESIAN_POINT('Ctrl Pts',(-17.2128353380511,69.4048725835516,
12.));
#157301=CARTESIAN_POINT('Ctrl Pts',(-17.2148149949261,69.3819158266955,
0.));
#157302=CARTESIAN_POINT('Ctrl Pts',(-17.2148149949261,69.3819158266955,
12.));
#157303=CARTESIAN_POINT('Ctrl Pts',(-17.2167679576991,69.359001631272,0.));
#157304=CARTESIAN_POINT('Ctrl Pts',(-17.2167679576991,69.359001631272,12.));
#157305=CARTESIAN_POINT('Ctrl Pts',(-17.2186942815604,69.3361301352149,
0.));
#157306=CARTESIAN_POINT('Ctrl Pts',(-17.2186942815604,69.3361301352149,
12.));
#157307=CARTESIAN_POINT('Ctrl Pts',(-17.2205940220455,69.3133014770541,
0.));
#157308=CARTESIAN_POINT('Ctrl Pts',(-17.2205940220455,69.3133014770541,
12.));
#157309=CARTESIAN_POINT('Ctrl Pts',(-17.2224672350432,69.2905157959142,
0.));
#157310=CARTESIAN_POINT('Ctrl Pts',(-17.2224672350432,69.2905157959142,
12.));
#157311=CARTESIAN_POINT('Ctrl Pts',(-17.2243139767963,69.26777323152,0.));
#157312=CARTESIAN_POINT('Ctrl Pts',(-17.2243139767963,69.26777323152,12.));
#157313=CARTESIAN_POINT('Ctrl Pts',(-17.2261343039015,69.2450739242092,
0.));
#157314=CARTESIAN_POINT('Ctrl Pts',(-17.2261343039015,69.2450739242092,
12.));
#157315=CARTESIAN_POINT('Ctrl Pts',(-17.2279282733119,69.2224180149377,
0.));
#157316=CARTESIAN_POINT('Ctrl Pts',(-17.2279282733119,69.2224180149377,
12.));
#157317=CARTESIAN_POINT('Ctrl Pts',(-17.229695942341,69.1998056452837,0.));
#157318=CARTESIAN_POINT('Ctrl Pts',(-17.229695942341,69.1998056452837,12.));
#157319=CARTESIAN_POINT('Ctrl Pts',(-17.2314373686705,69.1772369574462,
0.));
#157320=CARTESIAN_POINT('Ctrl Pts',(-17.2314373686705,69.1772369574462,
12.));
#157321=CARTESIAN_POINT('Ctrl Pts',(-17.2331526103511,69.1547120942542,
0.));
#157322=CARTESIAN_POINT('Ctrl Pts',(-17.2331526103511,69.1547120942542,
12.));
#157323=CARTESIAN_POINT('Ctrl Pts',(-17.2348417258017,69.1322311991759,
0.));
#157324=CARTESIAN_POINT('Ctrl Pts',(-17.2348417258017,69.1322311991759,
12.));
#157325=CARTESIAN_POINT('Ctrl Pts',(-17.2365047738125,69.1097944163243,
0.));
#157326=CARTESIAN_POINT('Ctrl Pts',(-17.2365047738125,69.1097944163243,
12.));
#157327=CARTESIAN_POINT('Ctrl Pts',(-17.238141813549,69.0874018904598,0.));
#157328=CARTESIAN_POINT('Ctrl Pts',(-17.238141813549,69.0874018904598,12.));
#157329=CARTESIAN_POINT('Ctrl Pts',(-17.2397529045587,69.0650537669859,
0.));
#157330=CARTESIAN_POINT('Ctrl Pts',(-17.2397529045587,69.0650537669859,
12.));
#157331=CARTESIAN_POINT('Ctrl Pts',(-17.2413381067722,69.0427501919636,
0.));
#157332=CARTESIAN_POINT('Ctrl Pts',(-17.2413381067722,69.0427501919636,
12.));
#157333=CARTESIAN_POINT('Ctrl Pts',(-17.2428974805043,69.0204913121226,
0.));
#157334=CARTESIAN_POINT('Ctrl Pts',(-17.2428974805043,69.0204913121226,
12.));
#157335=CARTESIAN_POINT('Ctrl Pts',(-17.2444310864585,68.9982772748694,
0.));
#157336=CARTESIAN_POINT('Ctrl Pts',(-17.2444310864585,68.9982772748694,
12.));
#157337=CARTESIAN_POINT('Ctrl Pts',(-17.2459389857327,68.9761082282922,
0.));
#157338=CARTESIAN_POINT('Ctrl Pts',(-17.2459389857327,68.9761082282922,
12.));
#157339=CARTESIAN_POINT('Ctrl Pts',(-17.2474212398275,68.9539843211618,
0.));
#157340=CARTESIAN_POINT('Ctrl Pts',(-17.2474212398275,68.9539843211618,
12.));
#157341=CARTESIAN_POINT('Ctrl Pts',(-17.248877910643,68.9319057029407,0.));
#157342=CARTESIAN_POINT('Ctrl Pts',(-17.248877910643,68.9319057029407,12.));
#157343=CARTESIAN_POINT('Ctrl Pts',(-17.2503090604792,68.9098725237868,
0.));
#157344=CARTESIAN_POINT('Ctrl Pts',(-17.2503090604792,68.9098725237868,
12.));
#157345=CARTESIAN_POINT('Ctrl Pts',(-17.2517147520376,68.8878849345557,
0.));
#157346=CARTESIAN_POINT('Ctrl Pts',(-17.2517147520376,68.8878849345557,
12.));
#157347=CARTESIAN_POINT('Ctrl Pts',(-17.2530950484259,68.8659430867977,
0.));
#157348=CARTESIAN_POINT('Ctrl Pts',(-17.2530950484259,68.8659430867977,
12.));
#157349=CARTESIAN_POINT('Ctrl Pts',(-17.2544500131627,68.8440471327563,
0.));
#157350=CARTESIAN_POINT('Ctrl Pts',(-17.2544500131627,68.8440471327563,
12.));
#157351=CARTESIAN_POINT('Ctrl Pts',(-17.2557797101816,68.8221972253954,
0.));
#157352=CARTESIAN_POINT('Ctrl Pts',(-17.2557797101816,68.8221972253954,
12.));
#157353=CARTESIAN_POINT('Ctrl Pts',(-17.2570842038385,68.8003935184193,
0.));
#157354=CARTESIAN_POINT('Ctrl Pts',(-17.2570842038385,68.8003935184193,
12.));
#157355=CARTESIAN_POINT('Ctrl Pts',(-17.2583635589197,68.7786361662876,
0.));
#157356=CARTESIAN_POINT('Ctrl Pts',(-17.2583635589197,68.7786361662876,
12.));
#157357=CARTESIAN_POINT('Ctrl Pts',(-17.2596178406545,68.7569253242312,
0.));
#157358=CARTESIAN_POINT('Ctrl Pts',(-17.2596178406545,68.7569253242312,
12.));
#157359=CARTESIAN_POINT('Ctrl Pts',(-17.2608471147178,68.7352611482519,
0.));
#157360=CARTESIAN_POINT('Ctrl Pts',(-17.2608471147178,68.7352611482519,
12.));
#157361=CARTESIAN_POINT('Ctrl Pts',(-17.2620514472176,68.7136437951075,
0.));
#157362=CARTESIAN_POINT('Ctrl Pts',(-17.2620514472176,68.7136437951075,
12.));
#157363=CARTESIAN_POINT('Ctrl Pts',(-17.263230904689,68.6920734222932,0.));
#157364=CARTESIAN_POINT('Ctrl Pts',(-17.263230904689,68.6920734222932,12.));
#157365=CARTESIAN_POINT('Ctrl Pts',(-17.2643855540896,68.6705501880263,
0.));
#157366=CARTESIAN_POINT('Ctrl Pts',(-17.2643855540896,68.6705501880263,
12.));
#157367=CARTESIAN_POINT('Ctrl Pts',(-17.2655154627935,68.6490742512085,
0.));
#157368=CARTESIAN_POINT('Ctrl Pts',(-17.2655154627935,68.6490742512085,
12.));
#157369=CARTESIAN_POINT('Ctrl Pts',(-17.2666206986091,68.6276457714757,
0.));
#157370=CARTESIAN_POINT('Ctrl Pts',(-17.2666206986091,68.6276457714757,
12.));
#157371=CARTESIAN_POINT('Ctrl Pts',(-17.2677013298061,68.6062649092781,
0.));
#157372=CARTESIAN_POINT('Ctrl Pts',(-17.2677013298061,68.6062649092781,
12.));
#157373=CARTESIAN_POINT('Ctrl Pts',(-17.2687574251429,68.5849318259449,
0.));
#157374=CARTESIAN_POINT('Ctrl Pts',(-17.2687574251429,68.5849318259449,
12.));
#157375=CARTESIAN_POINT('Ctrl Pts',(-17.2697890538956,68.5636466837502,
0.));
#157376=CARTESIAN_POINT('Ctrl Pts',(-17.2697890538956,68.5636466837502,
12.));
#157377=CARTESIAN_POINT('Ctrl Pts',(-17.2707962858912,68.5424096459746,
0.));
#157378=CARTESIAN_POINT('Ctrl Pts',(-17.2707962858912,68.5424096459746,
12.));
#157379=CARTESIAN_POINT('Ctrl Pts',(-17.2717791914538,68.5212208767835,
0.));
#157380=CARTESIAN_POINT('Ctrl Pts',(-17.2717791914538,68.5212208767835,
12.));
#157381=CARTESIAN_POINT('Ctrl Pts',(-17.2727378413485,68.5000805410897,
0.));
#157382=CARTESIAN_POINT('Ctrl Pts',(-17.2727378413485,68.5000805410897,
12.));
#157383=CARTESIAN_POINT('Ctrl Pts',(-17.2736723067367,68.4789888044357,
0.));
#157384=CARTESIAN_POINT('Ctrl Pts',(-17.2736723067367,68.4789888044357,
12.));
#157385=CARTESIAN_POINT('Ctrl Pts',(-17.2745826591125,68.4579458328208,
0.));
#157386=CARTESIAN_POINT('Ctrl Pts',(-17.2745826591125,68.4579458328208,
12.));
#157387=CARTESIAN_POINT('Ctrl Pts',(-17.2754689703001,68.4369517926803,
0.));
#157388=CARTESIAN_POINT('Ctrl Pts',(-17.2754689703001,68.4369517926803,
12.));
#157389=CARTESIAN_POINT('Ctrl Pts',(-17.2763313126026,68.4160068512781,
0.));
#157390=CARTESIAN_POINT('Ctrl Pts',(-17.2763313126026,68.4160068512781,
12.));
#157391=CARTESIAN_POINT('Ctrl Pts',(-17.2771697589387,68.3951111770498,
0.));
#157392=CARTESIAN_POINT('Ctrl Pts',(-17.2771697589387,68.3951111770498,
12.));
#157393=CARTESIAN_POINT('Ctrl Pts',(-17.2779843829605,68.374264939895,0.));
#157394=CARTESIAN_POINT('Ctrl Pts',(-17.2779843829605,68.374264939895,12.));
#157395=CARTESIAN_POINT('Ctrl Pts',(-17.2787752592475,68.353468311648,0.));
#157396=CARTESIAN_POINT('Ctrl Pts',(-17.2787752592475,68.353468311648,12.));
#157397=CARTESIAN_POINT('Ctrl Pts',(-17.2795424631789,68.3327214657533,
0.));
#157398=CARTESIAN_POINT('Ctrl Pts',(-17.2795424631789,68.3327214657533,
12.));
#157399=CARTESIAN_POINT('Ctrl Pts',(-17.2802860705807,68.3120245763884,
0.));
#157400=CARTESIAN_POINT('Ctrl Pts',(-17.2802860705807,68.3120245763884,
12.));
#157401=CARTESIAN_POINT('Ctrl Pts',(-17.2810061574352,68.2913778177258,
0.));
#157402=CARTESIAN_POINT('Ctrl Pts',(-17.2810061574352,68.2913778177258,
12.));
#157403=CARTESIAN_POINT('Ctrl Pts',(-17.2817027995838,68.2707813631761,
0.));
#157404=CARTESIAN_POINT('Ctrl Pts',(-17.2817027995838,68.2707813631761,
12.));
#157405=CARTESIAN_POINT('Ctrl Pts',(-17.2823760723886,68.250235384512,0.));
#157406=CARTESIAN_POINT('Ctrl Pts',(-17.2823760723886,68.250235384512,12.));
#157407=CARTESIAN_POINT('Ctrl Pts',(-17.2830260513879,68.2297400535339,
0.));
#157408=CARTESIAN_POINT('Ctrl Pts',(-17.2830260513879,68.2297400535339,
12.));
#157409=CARTESIAN_POINT('Ctrl Pts',(-17.2836528130825,68.2092955440591,
0.));
#157410=CARTESIAN_POINT('Ctrl Pts',(-17.2836528130825,68.2092955440591,
12.));
#157411=CARTESIAN_POINT('Ctrl Pts',(-17.2842564355796,68.1889020335418,
0.));
#157412=CARTESIAN_POINT('Ctrl Pts',(-17.2842564355796,68.1889020335418,
12.));
#157413=CARTESIAN_POINT('Ctrl Pts',(-17.2848369995283,68.1685597054193,
0.));
#157414=CARTESIAN_POINT('Ctrl Pts',(-17.2848369995283,68.1685597054193,
12.));
#157415=CARTESIAN_POINT('Ctrl Pts',(-17.2853945882059,68.1482687493176,
0.));
#157416=CARTESIAN_POINT('Ctrl Pts',(-17.2853945882059,68.1482687493176,
12.));
#157417=CARTESIAN_POINT('Ctrl Pts',(-17.2859292855694,68.1280293561473,
0.));
#157418=CARTESIAN_POINT('Ctrl Pts',(-17.2859292855694,68.1280293561473,
12.));
#157419=CARTESIAN_POINT('Ctrl Pts',(-17.2864411745455,68.1078417137865,
0.));
#157420=CARTESIAN_POINT('Ctrl Pts',(-17.2864411745455,68.1078417137865,
12.));
#157421=CARTESIAN_POINT('Ctrl Pts',(-17.2869303355438,68.0877060033229,
0.));
#157422=CARTESIAN_POINT('Ctrl Pts',(-17.2869303355438,68.0877060033229,
12.));
#157423=CARTESIAN_POINT('Ctrl Pts',(-17.2873968440855,68.0676223930469,
0.));
#157424=CARTESIAN_POINT('Ctrl Pts',(-17.2873968440855,68.0676223930469,
12.));
#157425=CARTESIAN_POINT('Ctrl Pts',(-17.2878407730981,68.0475910442494,
0.));
#157426=CARTESIAN_POINT('Ctrl Pts',(-17.2878407730981,68.0475910442494,
12.));
#157427=CARTESIAN_POINT('Ctrl Pts',(-17.2882621974737,68.027612122741,0.));
#157428=CARTESIAN_POINT('Ctrl Pts',(-17.2882621974737,68.027612122741,12.));
#157429=CARTESIAN_POINT('Ctrl Pts',(-17.28866119774,68.007685808115,0.));
#157430=CARTESIAN_POINT('Ctrl Pts',(-17.28866119774,68.007685808115,12.));
#157431=CARTESIAN_POINT('Ctrl Pts',(-17.2890378644843,67.9878123049133,
0.));
#157432=CARTESIAN_POINT('Ctrl Pts',(-17.2890378644843,67.9878123049133,
12.));
#157433=CARTESIAN_POINT('Ctrl Pts',(-17.2893923013852,67.9679918502441,
0.));
#157434=CARTESIAN_POINT('Ctrl Pts',(-17.2893923013852,67.9679918502441,
12.));
#157435=CARTESIAN_POINT('Ctrl Pts',(-17.2897246158895,67.9482246901517,
0.));
#157436=CARTESIAN_POINT('Ctrl Pts',(-17.2897246158895,67.9482246901517,
12.));
#157437=CARTESIAN_POINT('Ctrl Pts',(-17.2900349103956,67.9285110571662,
0.));
#157438=CARTESIAN_POINT('Ctrl Pts',(-17.2900349103956,67.9285110571662,
12.));
#157439=CARTESIAN_POINT('Ctrl Pts',(-17.2903232740717,67.908851149676,0.));
#157440=CARTESIAN_POINT('Ctrl Pts',(-17.2903232740717,67.908851149676,12.));
#157441=CARTESIAN_POINT('Ctrl Pts',(-17.2905897724029,67.8892451049871,
0.));
#157442=CARTESIAN_POINT('Ctrl Pts',(-17.2905897724029,67.8892451049871,
12.));
#157443=CARTESIAN_POINT('Ctrl Pts',(-17.2908344459816,67.8696929979178,
0.));
#157444=CARTESIAN_POINT('Ctrl Pts',(-17.2908344459816,67.8696929979178,
12.));
#157445=CARTESIAN_POINT('Ctrl Pts',(-17.2910127431203,67.8540944890057,
0.));
#157446=CARTESIAN_POINT('Ctrl Pts',(-17.2910127431203,67.8540944890057,
12.));
#157447=CARTESIAN_POINT('Ctrl Pts',(-17.2911366591419,67.8424198971214,
0.));
#157448=CARTESIAN_POINT('Ctrl Pts',(-17.2911366591419,67.8424198971214,
12.));
#157449=CARTESIAN_POINT('Ctrl Pts',(-17.2912149114145,67.8346476309106,
0.));
#157450=CARTESIAN_POINT('Ctrl Pts',(-17.2912149114145,67.8346476309106,
12.));
#157451=CARTESIAN_POINT('Ctrl Pts',(-17.2912529479484,67.8307641965655,
0.));
#157452=CARTESIAN_POINT('Ctrl Pts',(-17.2912529479484,67.8307641965655,
12.));
#157453=CARTESIAN_POINT('',(-17.2912529479484,67.8307641965655,12.));
#157454=CARTESIAN_POINT('Ctrl Pts',(-17.2912529479484,67.8307641965655,
12.));
#157455=CARTESIAN_POINT('Ctrl Pts',(-17.2912149114145,67.8346476309106,
12.));
#157456=CARTESIAN_POINT('Ctrl Pts',(-17.2911366591419,67.8424198971214,
12.));
#157457=CARTESIAN_POINT('Ctrl Pts',(-17.2910127431203,67.8540944890057,
12.));
#157458=CARTESIAN_POINT('Ctrl Pts',(-17.2908344459816,67.8696929979178,
12.));
#157459=CARTESIAN_POINT('Ctrl Pts',(-17.2905897724029,67.8892451049871,
12.));
#157460=CARTESIAN_POINT('Ctrl Pts',(-17.2903232740717,67.908851149676,12.));
#157461=CARTESIAN_POINT('Ctrl Pts',(-17.2900349103956,67.9285110571662,
12.));
#157462=CARTESIAN_POINT('Ctrl Pts',(-17.2897246158895,67.9482246901517,
12.));
#157463=CARTESIAN_POINT('Ctrl Pts',(-17.2893923013852,67.9679918502441,
12.));
#157464=CARTESIAN_POINT('Ctrl Pts',(-17.2890378644843,67.9878123049133,
12.));
#157465=CARTESIAN_POINT('Ctrl Pts',(-17.28866119774,68.007685808115,12.));
#157466=CARTESIAN_POINT('Ctrl Pts',(-17.2882621974737,68.027612122741,12.));
#157467=CARTESIAN_POINT('Ctrl Pts',(-17.2878407730981,68.0475910442494,
12.));
#157468=CARTESIAN_POINT('Ctrl Pts',(-17.2873968440855,68.0676223930469,
12.));
#157469=CARTESIAN_POINT('Ctrl Pts',(-17.2869303355438,68.0877060033229,
12.));
#157470=CARTESIAN_POINT('Ctrl Pts',(-17.2864411745455,68.1078417137865,
12.));
#157471=CARTESIAN_POINT('Ctrl Pts',(-17.2859292855694,68.1280293561473,
12.));
#157472=CARTESIAN_POINT('Ctrl Pts',(-17.2853945882059,68.1482687493176,
12.));
#157473=CARTESIAN_POINT('Ctrl Pts',(-17.2848369995283,68.1685597054193,
12.));
#157474=CARTESIAN_POINT('Ctrl Pts',(-17.2842564355796,68.1889020335418,
12.));
#157475=CARTESIAN_POINT('Ctrl Pts',(-17.2836528130825,68.2092955440591,
12.));
#157476=CARTESIAN_POINT('Ctrl Pts',(-17.2830260513879,68.2297400535339,
12.));
#157477=CARTESIAN_POINT('Ctrl Pts',(-17.2823760723886,68.250235384512,12.));
#157478=CARTESIAN_POINT('Ctrl Pts',(-17.2817027995838,68.2707813631761,
12.));
#157479=CARTESIAN_POINT('Ctrl Pts',(-17.2810061574352,68.2913778177258,
12.));
#157480=CARTESIAN_POINT('Ctrl Pts',(-17.2802860705807,68.3120245763884,
12.));
#157481=CARTESIAN_POINT('Ctrl Pts',(-17.2795424631789,68.3327214657533,
12.));
#157482=CARTESIAN_POINT('Ctrl Pts',(-17.2787752592475,68.353468311648,12.));
#157483=CARTESIAN_POINT('Ctrl Pts',(-17.2779843829605,68.374264939895,12.));
#157484=CARTESIAN_POINT('Ctrl Pts',(-17.2771697589387,68.3951111770498,
12.));
#157485=CARTESIAN_POINT('Ctrl Pts',(-17.2763313126026,68.4160068512781,
12.));
#157486=CARTESIAN_POINT('Ctrl Pts',(-17.2754689703001,68.4369517926803,
12.));
#157487=CARTESIAN_POINT('Ctrl Pts',(-17.2745826591125,68.4579458328208,
12.));
#157488=CARTESIAN_POINT('Ctrl Pts',(-17.2736723067367,68.4789888044357,
12.));
#157489=CARTESIAN_POINT('Ctrl Pts',(-17.2727378413485,68.5000805410897,
12.));
#157490=CARTESIAN_POINT('Ctrl Pts',(-17.2717791914538,68.5212208767835,
12.));
#157491=CARTESIAN_POINT('Ctrl Pts',(-17.2707962858912,68.5424096459746,
12.));
#157492=CARTESIAN_POINT('Ctrl Pts',(-17.2697890538956,68.5636466837502,
12.));
#157493=CARTESIAN_POINT('Ctrl Pts',(-17.2687574251429,68.5849318259449,
12.));
#157494=CARTESIAN_POINT('Ctrl Pts',(-17.2677013298061,68.6062649092781,
12.));
#157495=CARTESIAN_POINT('Ctrl Pts',(-17.2666206986091,68.6276457714757,
12.));
#157496=CARTESIAN_POINT('Ctrl Pts',(-17.2655154627935,68.6490742512085,
12.));
#157497=CARTESIAN_POINT('Ctrl Pts',(-17.2643855540896,68.6705501880263,
12.));
#157498=CARTESIAN_POINT('Ctrl Pts',(-17.263230904689,68.6920734222932,12.));
#157499=CARTESIAN_POINT('Ctrl Pts',(-17.2620514472176,68.7136437951075,
12.));
#157500=CARTESIAN_POINT('Ctrl Pts',(-17.2608471147178,68.7352611482519,
12.));
#157501=CARTESIAN_POINT('Ctrl Pts',(-17.2596178406545,68.7569253242312,
12.));
#157502=CARTESIAN_POINT('Ctrl Pts',(-17.2583635589197,68.7786361662876,
12.));
#157503=CARTESIAN_POINT('Ctrl Pts',(-17.2570842038385,68.8003935184193,
12.));
#157504=CARTESIAN_POINT('Ctrl Pts',(-17.2557797101816,68.8221972253954,
12.));
#157505=CARTESIAN_POINT('Ctrl Pts',(-17.2544500131627,68.8440471327563,
12.));
#157506=CARTESIAN_POINT('Ctrl Pts',(-17.2530950484259,68.8659430867977,
12.));
#157507=CARTESIAN_POINT('Ctrl Pts',(-17.2517147520376,68.8878849345557,
12.));
#157508=CARTESIAN_POINT('Ctrl Pts',(-17.2503090604792,68.9098725237868,
12.));
#157509=CARTESIAN_POINT('Ctrl Pts',(-17.248877910643,68.9319057029407,12.));
#157510=CARTESIAN_POINT('Ctrl Pts',(-17.2474212398275,68.9539843211618,
12.));
#157511=CARTESIAN_POINT('Ctrl Pts',(-17.2459389857327,68.9761082282922,
12.));
#157512=CARTESIAN_POINT('Ctrl Pts',(-17.2444310864585,68.9982772748694,
12.));
#157513=CARTESIAN_POINT('Ctrl Pts',(-17.2428974805043,69.0204913121226,
12.));
#157514=CARTESIAN_POINT('Ctrl Pts',(-17.2413381067722,69.0427501919636,
12.));
#157515=CARTESIAN_POINT('Ctrl Pts',(-17.2397529045587,69.0650537669859,
12.));
#157516=CARTESIAN_POINT('Ctrl Pts',(-17.238141813549,69.0874018904598,12.));
#157517=CARTESIAN_POINT('Ctrl Pts',(-17.2365047738125,69.1097944163243,
12.));
#157518=CARTESIAN_POINT('Ctrl Pts',(-17.2348417258017,69.1322311991759,
12.));
#157519=CARTESIAN_POINT('Ctrl Pts',(-17.2331526103511,69.1547120942542,
12.));
#157520=CARTESIAN_POINT('Ctrl Pts',(-17.2314373686705,69.1772369574462,
12.));
#157521=CARTESIAN_POINT('Ctrl Pts',(-17.229695942341,69.1998056452837,12.));
#157522=CARTESIAN_POINT('Ctrl Pts',(-17.2279282733119,69.2224180149377,
12.));
#157523=CARTESIAN_POINT('Ctrl Pts',(-17.2261343039015,69.2450739242092,
12.));
#157524=CARTESIAN_POINT('Ctrl Pts',(-17.2243139767963,69.26777323152,12.));
#157525=CARTESIAN_POINT('Ctrl Pts',(-17.2224672350432,69.2905157959142,
12.));
#157526=CARTESIAN_POINT('Ctrl Pts',(-17.2205940220455,69.3133014770541,
12.));
#157527=CARTESIAN_POINT('Ctrl Pts',(-17.2186942815604,69.3361301352149,
12.));
#157528=CARTESIAN_POINT('Ctrl Pts',(-17.2167679576991,69.359001631272,12.));
#157529=CARTESIAN_POINT('Ctrl Pts',(-17.2148149949261,69.3819158266955,
12.));
#157530=CARTESIAN_POINT('Ctrl Pts',(-17.2128353380511,69.4048725835516,
12.));
#157531=CARTESIAN_POINT('Ctrl Pts',(-17.2108289322258,69.4278717644989,
12.));
#157532=CARTESIAN_POINT('Ctrl Pts',(-17.208795722942,69.4509132327836,12.));
#157533=CARTESIAN_POINT('Ctrl Pts',(-17.2067356560326,69.4739968522271,
12.));
#157534=CARTESIAN_POINT('Ctrl Pts',(-17.2046486776697,69.497122487222,12.));
#157535=CARTESIAN_POINT('Ctrl Pts',(-17.2025347343568,69.5202900027329,
12.));
#157536=CARTESIAN_POINT('Ctrl Pts',(-17.2003937729266,69.5434992642932,
12.));
#157537=CARTESIAN_POINT('Ctrl Pts',(-17.198225740538,69.5667501379984,12.));
#157538=CARTESIAN_POINT('Ctrl Pts',(-17.1960305846787,69.5900424904954,
12.));
#157539=CARTESIAN_POINT('Ctrl Pts',(-17.193808253162,69.6133761889787,12.));
#157540=CARTESIAN_POINT('Ctrl Pts',(-17.1915586941198,69.6367511011927,
12.));
#157541=CARTESIAN_POINT('Ctrl Pts',(-17.1892818560004,69.6601670954277,
12.));
#157542=CARTESIAN_POINT('Ctrl Pts',(-17.1869776875663,69.6836240405152,
12.));
#157543=CARTESIAN_POINT('Ctrl Pts',(-17.1846461378966,69.7071218058149,
12.));
#157544=CARTESIAN_POINT('Ctrl Pts',(-17.1822871563835,69.7306602612125,
12.));
#157545=CARTESIAN_POINT('Ctrl Pts',(-17.1799006927256,69.7542392771216,
12.));
#157546=CARTESIAN_POINT('Ctrl Pts',(-17.1774866969256,69.7778587244788,
12.));
#157547=CARTESIAN_POINT('Ctrl Pts',(-17.1750451192887,69.8015184747404,
12.));
#157548=CARTESIAN_POINT('Ctrl Pts',(-17.1725759104254,69.8252183998713,
12.));
#157549=CARTESIAN_POINT('Ctrl Pts',(-17.1700790212476,69.8489583723417,
12.));
#157550=CARTESIAN_POINT('Ctrl Pts',(-17.1675544029622,69.8727382651292,
12.));
#157551=CARTESIAN_POINT('Ctrl Pts',(-17.1650020070686,69.8965579517147,
12.));
#157552=CARTESIAN_POINT('Ctrl Pts',(-17.1624217853577,69.9204173060779,
12.));
#157553=CARTESIAN_POINT('Ctrl Pts',(-17.1598136899144,69.9443162026865,
12.));
#157554=CARTESIAN_POINT('Ctrl Pts',(-17.157177673114,69.9682545164942,12.));
#157555=CARTESIAN_POINT('Ctrl Pts',(-17.1545136876162,69.9922321229428,
12.));
#157556=CARTESIAN_POINT('Ctrl Pts',(-17.1518216863624,70.0162488979587,
12.));
#157557=CARTESIAN_POINT('Ctrl Pts',(-17.1491016225748,70.0403047179481,
12.));
#157558=CARTESIAN_POINT('Ctrl Pts',(-17.1463534497592,70.0643994597865,
12.));
#157559=CARTESIAN_POINT('Ctrl Pts',(-17.1435771217015,70.0885330008169,
12.));
#157560=CARTESIAN_POINT('Ctrl Pts',(-17.1407725924615,70.1127052188515,
12.));
#157561=CARTESIAN_POINT('Ctrl Pts',(-17.1379398163708,70.1369159921686,
12.));
#157562=CARTESIAN_POINT('Ctrl Pts',(-17.1350787480313,70.1611651995085,
12.));
#157563=CARTESIAN_POINT('Ctrl Pts',(-17.1321893423183,70.1854527200636,
12.));
#157564=CARTESIAN_POINT('Ctrl Pts',(-17.1292715543779,70.2097784334749,
12.));
#157565=CARTESIAN_POINT('Ctrl Pts',(-17.1263253396202,70.2341422198363,
12.));
#157566=CARTESIAN_POINT('Ctrl Pts',(-17.1233506537176,70.2585439596899,
12.));
#157567=CARTESIAN_POINT('Ctrl Pts',(-17.1203474526031,70.2829835340239,
12.));
#157568=CARTESIAN_POINT('Ctrl Pts',(-17.1173156924734,70.3074608242613,
12.));
#157569=CARTESIAN_POINT('Ctrl Pts',(-17.1142553297869,70.3319757122577,
12.));
#157570=CARTESIAN_POINT('Ctrl Pts',(-17.111166321257,70.356528080303,12.));
#157571=CARTESIAN_POINT('Ctrl Pts',(-17.10804862385,70.3811178111206,12.));
#157572=CARTESIAN_POINT('Ctrl Pts',(-17.1049021947833,70.4057447878621,
12.));
#157573=CARTESIAN_POINT('Ctrl Pts',(-17.1017269915289,70.4304088940998,
12.));
#157574=CARTESIAN_POINT('Ctrl Pts',(-17.098522971812,70.4551100138221,12.));
#157575=CARTESIAN_POINT('Ctrl Pts',(-17.0952900936044,70.4798480314364,
12.));
#157576=CARTESIAN_POINT('Ctrl Pts',(-17.0920283151217,70.5046228317669,
12.));
#157577=CARTESIAN_POINT('Ctrl Pts',(-17.0887375948221,70.5294343000516,
12.));
#157578=CARTESIAN_POINT('Ctrl Pts',(-17.085417891409,70.5542823219346,12.));
#157579=CARTESIAN_POINT('Ctrl Pts',(-17.0820691638314,70.5791667834599,
12.));
#157580=CARTESIAN_POINT('Ctrl Pts',(-17.0786913712767,70.6040875710762,
12.));
#157581=CARTESIAN_POINT('Ctrl Pts',(-17.0752844731679,70.6290445716341,
12.));
#157582=CARTESIAN_POINT('Ctrl Pts',(-17.0718484291623,70.6540376723839,
12.));
#157583=CARTESIAN_POINT('Ctrl Pts',(-17.0683831991532,70.6790667609678,
12.));
#157584=CARTESIAN_POINT('Ctrl Pts',(-17.0648887432714,70.7041317254128,
12.));
#157585=CARTESIAN_POINT('Ctrl Pts',(-17.0613650218789,70.7292324541348,
12.));
#157586=CARTESIAN_POINT('Ctrl Pts',(-17.0578119955651,70.754368835938,12.));
#157587=CARTESIAN_POINT('Ctrl Pts',(-17.0542296251462,70.7795407600127,
12.));
#157588=CARTESIAN_POINT('Ctrl Pts',(-17.0506178716662,70.8047481159298,
12.));
#157589=CARTESIAN_POINT('Ctrl Pts',(-17.0469766964001,70.8299907936334,
12.));
#157590=CARTESIAN_POINT('Ctrl Pts',(-17.0433060608475,70.8552686834423,
12.));
#157591=CARTESIAN_POINT('Ctrl Pts',(-17.0396059267277,70.8805816760501,
12.));
#157592=CARTESIAN_POINT('Ctrl Pts',(-17.0358762559786,70.9059296625214,
12.));
#157593=CARTESIAN_POINT('Ctrl Pts',(-17.0321170107564,70.9313125342876,
12.));
#157594=CARTESIAN_POINT('Ctrl Pts',(-17.0283281534392,70.956730183136,12.));
#157595=CARTESIAN_POINT('Ctrl Pts',(-17.0245096466229,70.9821825012136,
12.));
#157596=CARTESIAN_POINT('Ctrl Pts',(-17.0206614531166,71.0076693810301,
12.));
#157597=CARTESIAN_POINT('Ctrl Pts',(-17.0167835359419,71.0331907154574,
12.));
#157598=CARTESIAN_POINT('Ctrl Pts',(-17.0128758583335,71.0587463977268,
12.));
#157599=CARTESIAN_POINT('Ctrl Pts',(-17.0089383837437,71.0843363214221,
12.));
#157600=CARTESIAN_POINT('Ctrl Pts',(-17.0049710758394,71.1099603804786,
12.));
#157601=CARTESIAN_POINT('Ctrl Pts',(-17.0009738984936,71.1356184691806,
12.));
#157602=CARTESIAN_POINT('Ctrl Pts',(-16.9969468157824,71.1613104821568,
12.));
#157603=CARTESIAN_POINT('Ctrl Pts',(-16.9928897919828,71.187036314374,12.));
#157604=CARTESIAN_POINT('Ctrl Pts',(-16.9888027915742,71.212795861124,12.));
#157605=CARTESIAN_POINT('Ctrl Pts',(-16.9846857792384,71.2385890180221,
12.));
#157606=CARTESIAN_POINT('Ctrl Pts',(-16.9805387198571,71.2644156810198,
12.));
#157607=CARTESIAN_POINT('Ctrl Pts',(-16.9763615785137,71.290275746412,12.));
#157608=CARTESIAN_POINT('Ctrl Pts',(-16.9721543204951,71.3161691108427,
12.));
#157609=CARTESIAN_POINT('Ctrl Pts',(-16.9679169112994,71.3420956713082,
12.));
#157610=CARTESIAN_POINT('Ctrl Pts',(-16.9636493166397,71.3680553251562,
12.));
#157611=CARTESIAN_POINT('Ctrl Pts',(-16.9593515024276,71.3940479700677,
12.));
#157612=CARTESIAN_POINT('Ctrl Pts',(-16.9550234347621,71.4200735040384,
12.));
#157613=CARTESIAN_POINT('Ctrl Pts',(-16.9506650799189,71.4461318253563,
12.));
#157614=CARTESIAN_POINT('Ctrl Pts',(-16.9462764043443,71.4722228325794,
12.));
#157615=CARTESIAN_POINT('Ctrl Pts',(-16.9418573746489,71.4983464245055,
12.));
#157616=CARTESIAN_POINT('Ctrl Pts',(-16.9374079576201,71.5245025002139,
12.));
#157617=CARTESIAN_POINT('Ctrl Pts',(-16.9329281202377,71.5506909591129,
12.));
#157618=CARTESIAN_POINT('Ctrl Pts',(-16.9284178296933,71.5769117009842,
12.));
#157619=CARTESIAN_POINT('Ctrl Pts',(-16.9238770534071,71.6031646260174,
12.));
#157620=CARTESIAN_POINT('Ctrl Pts',(-16.9193057590607,71.6294496348653,
12.));
#157621=CARTESIAN_POINT('Ctrl Pts',(-16.9147039145717,71.6557666285917,
12.));
#157622=CARTESIAN_POINT('Ctrl Pts',(-16.9100714880368,71.6821155085612,
12.));
#157623=CARTESIAN_POINT('Ctrl Pts',(-16.9054084476847,71.7084961763357,
12.));
#157624=CARTESIAN_POINT('Ctrl Pts',(-16.9007147618344,71.7349085335796,
12.));
#157625=CARTESIAN_POINT('Ctrl Pts',(-16.895990398841,71.7613524819235,12.));
#157626=CARTESIAN_POINT('Ctrl Pts',(-16.8912353270942,71.7878279229546,
12.));
#157627=CARTESIAN_POINT('Ctrl Pts',(-16.8864495151344,71.8143347584962,
12.));
#157628=CARTESIAN_POINT('Ctrl Pts',(-16.881632931747,71.8408728908258,12.));
#157629=CARTESIAN_POINT('Ctrl Pts',(-16.87678554607,71.867442222915,12.));
#157630=CARTESIAN_POINT('Ctrl Pts',(-16.871907327697,71.8940426586534,12.));
#157631=CARTESIAN_POINT('Ctrl Pts',(-16.866998246792,71.9206741030887,12.));
#157632=CARTESIAN_POINT('Ctrl Pts',(-16.8620582738437,71.9473364618922,
12.));
#157633=CARTESIAN_POINT('Ctrl Pts',(-16.8570873794269,71.9740296408347,
12.));
#157634=CARTESIAN_POINT('Ctrl Pts',(-16.8520855339446,72.0007535452081,
12.));
#157635=CARTESIAN_POINT('Ctrl Pts',(-16.8470527074275,72.0275080793727,
12.));
#157636=CARTESIAN_POINT('Ctrl Pts',(-16.8419888691976,72.0542931459825,
12.));
#157637=CARTESIAN_POINT('Ctrl Pts',(-16.8368939881446,72.0811086466121,
12.));
#157638=CARTESIAN_POINT('Ctrl Pts',(-16.8317680333404,72.1079544831513,
12.));
#157639=CARTESIAN_POINT('Ctrl Pts',(-16.8266109745795,72.13483055902,12.));
#157640=CARTESIAN_POINT('Ctrl Pts',(-16.8214227828943,72.1617367803235,
12.));
#157641=CARTESIAN_POINT('Ctrl Pts',(-16.8162034312269,72.1886730573452,
12.));
#157642=CARTESIAN_POINT('Ctrl Pts',(-16.8109528945896,72.2156393048975,
12.));
#157643=CARTESIAN_POINT('Ctrl Pts',(-16.8064254147776,72.2387802230856,
12.));
#157644=CARTESIAN_POINT('Ctrl Pts',(-16.8029374213794,72.256538003526,12.));
#157645=CARTESIAN_POINT('Ctrl Pts',(-16.8005027425863,72.2688994295264,
12.));
#157646=CARTESIAN_POINT('Ctrl Pts',(-16.7991305317749,72.2758557891329,
12.));
#157647=CARTESIAN_POINT('Ctrl Pts',(-16.7988252568748,72.2774028393914,
12.));
#157648=CARTESIAN_POINT('',(-17.2912529479484,67.8307641965655,0.));
#157649=CARTESIAN_POINT('',(-17.2912529479484,67.8307641965655,0.));
#157650=CARTESIAN_POINT('Ctrl Pts',(-16.7988252568748,72.2774028393914,
0.));
#157651=CARTESIAN_POINT('Ctrl Pts',(-16.7991305317749,72.2758557891329,
0.));
#157652=CARTESIAN_POINT('Ctrl Pts',(-16.8005027425863,72.2688994295264,
0.));
#157653=CARTESIAN_POINT('Ctrl Pts',(-16.8029374213794,72.256538003526,0.));
#157654=CARTESIAN_POINT('Ctrl Pts',(-16.8064254147776,72.2387802230856,
0.));
#157655=CARTESIAN_POINT('Ctrl Pts',(-16.8109528945896,72.2156393048975,
0.));
#157656=CARTESIAN_POINT('Ctrl Pts',(-16.8162034312269,72.1886730573452,
0.));
#157657=CARTESIAN_POINT('Ctrl Pts',(-16.8214227828943,72.1617367803235,
0.));
#157658=CARTESIAN_POINT('Ctrl Pts',(-16.8266109745795,72.13483055902,0.));
#157659=CARTESIAN_POINT('Ctrl Pts',(-16.8317680333404,72.1079544831513,
0.));
#157660=CARTESIAN_POINT('Ctrl Pts',(-16.8368939881446,72.0811086466121,
0.));
#157661=CARTESIAN_POINT('Ctrl Pts',(-16.8419888691976,72.0542931459825,
0.));
#157662=CARTESIAN_POINT('Ctrl Pts',(-16.8470527074275,72.0275080793727,
0.));
#157663=CARTESIAN_POINT('Ctrl Pts',(-16.8520855339446,72.0007535452081,
0.));
#157664=CARTESIAN_POINT('Ctrl Pts',(-16.8570873794269,71.9740296408347,
0.));
#157665=CARTESIAN_POINT('Ctrl Pts',(-16.8620582738437,71.9473364618922,
0.));
#157666=CARTESIAN_POINT('Ctrl Pts',(-16.866998246792,71.9206741030887,0.));
#157667=CARTESIAN_POINT('Ctrl Pts',(-16.871907327697,71.8940426586534,0.));
#157668=CARTESIAN_POINT('Ctrl Pts',(-16.87678554607,71.867442222915,0.));
#157669=CARTESIAN_POINT('Ctrl Pts',(-16.881632931747,71.8408728908258,0.));
#157670=CARTESIAN_POINT('Ctrl Pts',(-16.8864495151344,71.8143347584962,
0.));
#157671=CARTESIAN_POINT('Ctrl Pts',(-16.8912353270942,71.7878279229546,
0.));
#157672=CARTESIAN_POINT('Ctrl Pts',(-16.895990398841,71.7613524819235,0.));
#157673=CARTESIAN_POINT('Ctrl Pts',(-16.9007147618344,71.7349085335796,
0.));
#157674=CARTESIAN_POINT('Ctrl Pts',(-16.9054084476847,71.7084961763357,
0.));
#157675=CARTESIAN_POINT('Ctrl Pts',(-16.9100714880368,71.6821155085612,
0.));
#157676=CARTESIAN_POINT('Ctrl Pts',(-16.9147039145717,71.6557666285917,
0.));
#157677=CARTESIAN_POINT('Ctrl Pts',(-16.9193057590607,71.6294496348653,
0.));
#157678=CARTESIAN_POINT('Ctrl Pts',(-16.9238770534071,71.6031646260174,
0.));
#157679=CARTESIAN_POINT('Ctrl Pts',(-16.9284178296933,71.5769117009842,
0.));
#157680=CARTESIAN_POINT('Ctrl Pts',(-16.9329281202377,71.5506909591129,
0.));
#157681=CARTESIAN_POINT('Ctrl Pts',(-16.9374079576201,71.5245025002139,
0.));
#157682=CARTESIAN_POINT('Ctrl Pts',(-16.9418573746489,71.4983464245055,
0.));
#157683=CARTESIAN_POINT('Ctrl Pts',(-16.9462764043443,71.4722228325794,
0.));
#157684=CARTESIAN_POINT('Ctrl Pts',(-16.9506650799189,71.4461318253563,
0.));
#157685=CARTESIAN_POINT('Ctrl Pts',(-16.9550234347621,71.4200735040384,
0.));
#157686=CARTESIAN_POINT('Ctrl Pts',(-16.9593515024276,71.3940479700677,
0.));
#157687=CARTESIAN_POINT('Ctrl Pts',(-16.9636493166397,71.3680553251562,
0.));
#157688=CARTESIAN_POINT('Ctrl Pts',(-16.9679169112994,71.3420956713082,
0.));
#157689=CARTESIAN_POINT('Ctrl Pts',(-16.9721543204951,71.3161691108427,
0.));
#157690=CARTESIAN_POINT('Ctrl Pts',(-16.9763615785137,71.290275746412,0.));
#157691=CARTESIAN_POINT('Ctrl Pts',(-16.9805387198571,71.2644156810198,
0.));
#157692=CARTESIAN_POINT('Ctrl Pts',(-16.9846857792384,71.2385890180221,
0.));
#157693=CARTESIAN_POINT('Ctrl Pts',(-16.9888027915742,71.212795861124,0.));
#157694=CARTESIAN_POINT('Ctrl Pts',(-16.9928897919828,71.187036314374,0.));
#157695=CARTESIAN_POINT('Ctrl Pts',(-16.9969468157824,71.1613104821568,
0.));
#157696=CARTESIAN_POINT('Ctrl Pts',(-17.0009738984936,71.1356184691806,
0.));
#157697=CARTESIAN_POINT('Ctrl Pts',(-17.0049710758394,71.1099603804786,
0.));
#157698=CARTESIAN_POINT('Ctrl Pts',(-17.0089383837437,71.0843363214221,
0.));
#157699=CARTESIAN_POINT('Ctrl Pts',(-17.0128758583335,71.0587463977268,
0.));
#157700=CARTESIAN_POINT('Ctrl Pts',(-17.0167835359419,71.0331907154574,
0.));
#157701=CARTESIAN_POINT('Ctrl Pts',(-17.0206614531166,71.0076693810301,
0.));
#157702=CARTESIAN_POINT('Ctrl Pts',(-17.0245096466229,70.9821825012136,
0.));
#157703=CARTESIAN_POINT('Ctrl Pts',(-17.0283281534392,70.956730183136,0.));
#157704=CARTESIAN_POINT('Ctrl Pts',(-17.0321170107564,70.9313125342876,
0.));
#157705=CARTESIAN_POINT('Ctrl Pts',(-17.0358762559786,70.9059296625214,
0.));
#157706=CARTESIAN_POINT('Ctrl Pts',(-17.0396059267277,70.8805816760501,
0.));
#157707=CARTESIAN_POINT('Ctrl Pts',(-17.0433060608475,70.8552686834423,
0.));
#157708=CARTESIAN_POINT('Ctrl Pts',(-17.0469766964001,70.8299907936334,
0.));
#157709=CARTESIAN_POINT('Ctrl Pts',(-17.0506178716662,70.8047481159298,
0.));
#157710=CARTESIAN_POINT('Ctrl Pts',(-17.0542296251462,70.7795407600127,
0.));
#157711=CARTESIAN_POINT('Ctrl Pts',(-17.0578119955651,70.754368835938,0.));
#157712=CARTESIAN_POINT('Ctrl Pts',(-17.0613650218789,70.7292324541348,
0.));
#157713=CARTESIAN_POINT('Ctrl Pts',(-17.0648887432714,70.7041317254128,
0.));
#157714=CARTESIAN_POINT('Ctrl Pts',(-17.0683831991532,70.6790667609678,
0.));
#157715=CARTESIAN_POINT('Ctrl Pts',(-17.0718484291623,70.6540376723839,
0.));
#157716=CARTESIAN_POINT('Ctrl Pts',(-17.0752844731679,70.6290445716341,
0.));
#157717=CARTESIAN_POINT('Ctrl Pts',(-17.0786913712767,70.6040875710762,
0.));
#157718=CARTESIAN_POINT('Ctrl Pts',(-17.0820691638314,70.5791667834599,
0.));
#157719=CARTESIAN_POINT('Ctrl Pts',(-17.085417891409,70.5542823219346,0.));
#157720=CARTESIAN_POINT('Ctrl Pts',(-17.0887375948221,70.5294343000516,
0.));
#157721=CARTESIAN_POINT('Ctrl Pts',(-17.0920283151217,70.5046228317669,
0.));
#157722=CARTESIAN_POINT('Ctrl Pts',(-17.0952900936044,70.4798480314364,
0.));
#157723=CARTESIAN_POINT('Ctrl Pts',(-17.098522971812,70.4551100138221,0.));
#157724=CARTESIAN_POINT('Ctrl Pts',(-17.1017269915289,70.4304088940998,
0.));
#157725=CARTESIAN_POINT('Ctrl Pts',(-17.1049021947833,70.4057447878621,
0.));
#157726=CARTESIAN_POINT('Ctrl Pts',(-17.10804862385,70.3811178111206,0.));
#157727=CARTESIAN_POINT('Ctrl Pts',(-17.111166321257,70.356528080303,0.));
#157728=CARTESIAN_POINT('Ctrl Pts',(-17.1142553297869,70.3319757122577,
0.));
#157729=CARTESIAN_POINT('Ctrl Pts',(-17.1173156924734,70.3074608242613,
0.));
#157730=CARTESIAN_POINT('Ctrl Pts',(-17.1203474526031,70.2829835340239,
0.));
#157731=CARTESIAN_POINT('Ctrl Pts',(-17.1233506537176,70.2585439596899,
0.));
#157732=CARTESIAN_POINT('Ctrl Pts',(-17.1263253396202,70.2341422198363,
0.));
#157733=CARTESIAN_POINT('Ctrl Pts',(-17.1292715543779,70.2097784334749,
0.));
#157734=CARTESIAN_POINT('Ctrl Pts',(-17.1321893423183,70.1854527200636,
0.));
#157735=CARTESIAN_POINT('Ctrl Pts',(-17.1350787480313,70.1611651995085,
0.));
#157736=CARTESIAN_POINT('Ctrl Pts',(-17.1379398163708,70.1369159921686,
0.));
#157737=CARTESIAN_POINT('Ctrl Pts',(-17.1407725924615,70.1127052188515,
0.));
#157738=CARTESIAN_POINT('Ctrl Pts',(-17.1435771217015,70.0885330008169,
0.));
#157739=CARTESIAN_POINT('Ctrl Pts',(-17.1463534497592,70.0643994597865,
0.));
#157740=CARTESIAN_POINT('Ctrl Pts',(-17.1491016225748,70.0403047179481,
0.));
#157741=CARTESIAN_POINT('Ctrl Pts',(-17.1518216863624,70.0162488979587,
0.));
#157742=CARTESIAN_POINT('Ctrl Pts',(-17.1545136876162,69.9922321229428,
0.));
#157743=CARTESIAN_POINT('Ctrl Pts',(-17.157177673114,69.9682545164942,0.));
#157744=CARTESIAN_POINT('Ctrl Pts',(-17.1598136899144,69.9443162026865,
0.));
#157745=CARTESIAN_POINT('Ctrl Pts',(-17.1624217853577,69.9204173060779,
0.));
#157746=CARTESIAN_POINT('Ctrl Pts',(-17.1650020070686,69.8965579517147,
0.));
#157747=CARTESIAN_POINT('Ctrl Pts',(-17.1675544029622,69.8727382651292,
0.));
#157748=CARTESIAN_POINT('Ctrl Pts',(-17.1700790212476,69.8489583723417,
0.));
#157749=CARTESIAN_POINT('Ctrl Pts',(-17.1725759104254,69.8252183998713,
0.));
#157750=CARTESIAN_POINT('Ctrl Pts',(-17.1750451192887,69.8015184747404,
0.));
#157751=CARTESIAN_POINT('Ctrl Pts',(-17.1774866969256,69.7778587244788,
0.));
#157752=CARTESIAN_POINT('Ctrl Pts',(-17.1799006927256,69.7542392771216,
0.));
#157753=CARTESIAN_POINT('Ctrl Pts',(-17.1822871563835,69.7306602612125,
0.));
#157754=CARTESIAN_POINT('Ctrl Pts',(-17.1846461378966,69.7071218058149,
0.));
#157755=CARTESIAN_POINT('Ctrl Pts',(-17.1869776875663,69.6836240405152,
0.));
#157756=CARTESIAN_POINT('Ctrl Pts',(-17.1892818560004,69.6601670954277,
0.));
#157757=CARTESIAN_POINT('Ctrl Pts',(-17.1915586941198,69.6367511011927,
0.));
#157758=CARTESIAN_POINT('Ctrl Pts',(-17.193808253162,69.6133761889787,0.));
#157759=CARTESIAN_POINT('Ctrl Pts',(-17.1960305846787,69.5900424904954,
0.));
#157760=CARTESIAN_POINT('Ctrl Pts',(-17.198225740538,69.5667501379984,0.));
#157761=CARTESIAN_POINT('Ctrl Pts',(-17.2003937729266,69.5434992642932,
0.));
#157762=CARTESIAN_POINT('Ctrl Pts',(-17.2025347343568,69.5202900027329,
0.));
#157763=CARTESIAN_POINT('Ctrl Pts',(-17.2046486776697,69.497122487222,0.));
#157764=CARTESIAN_POINT('Ctrl Pts',(-17.2067356560326,69.4739968522271,
0.));
#157765=CARTESIAN_POINT('Ctrl Pts',(-17.208795722942,69.4509132327836,0.));
#157766=CARTESIAN_POINT('Ctrl Pts',(-17.2108289322258,69.4278717644989,
0.));
#157767=CARTESIAN_POINT('Ctrl Pts',(-17.2128353380511,69.4048725835516,
0.));
#157768=CARTESIAN_POINT('Ctrl Pts',(-17.2148149949261,69.3819158266955,
0.));
#157769=CARTESIAN_POINT('Ctrl Pts',(-17.2167679576991,69.359001631272,0.));
#157770=CARTESIAN_POINT('Ctrl Pts',(-17.2186942815604,69.3361301352149,
0.));
#157771=CARTESIAN_POINT('Ctrl Pts',(-17.2205940220455,69.3133014770541,
0.));
#157772=CARTESIAN_POINT('Ctrl Pts',(-17.2224672350432,69.2905157959142,
0.));
#157773=CARTESIAN_POINT('Ctrl Pts',(-17.2243139767963,69.26777323152,0.));
#157774=CARTESIAN_POINT('Ctrl Pts',(-17.2261343039015,69.2450739242092,
0.));
#157775=CARTESIAN_POINT('Ctrl Pts',(-17.2279282733119,69.2224180149377,
0.));
#157776=CARTESIAN_POINT('Ctrl Pts',(-17.229695942341,69.1998056452837,0.));
#157777=CARTESIAN_POINT('Ctrl Pts',(-17.2314373686705,69.1772369574462,
0.));
#157778=CARTESIAN_POINT('Ctrl Pts',(-17.2331526103511,69.1547120942542,
0.));
#157779=CARTESIAN_POINT('Ctrl Pts',(-17.2348417258017,69.1322311991759,
0.));
#157780=CARTESIAN_POINT('Ctrl Pts',(-17.2365047738125,69.1097944163243,
0.));
#157781=CARTESIAN_POINT('Ctrl Pts',(-17.238141813549,69.0874018904598,0.));
#157782=CARTESIAN_POINT('Ctrl Pts',(-17.2397529045587,69.0650537669859,
0.));
#157783=CARTESIAN_POINT('Ctrl Pts',(-17.2413381067722,69.0427501919636,
0.));
#157784=CARTESIAN_POINT('Ctrl Pts',(-17.2428974805043,69.0204913121226,
0.));
#157785=CARTESIAN_POINT('Ctrl Pts',(-17.2444310864585,68.9982772748694,
0.));
#157786=CARTESIAN_POINT('Ctrl Pts',(-17.2459389857327,68.9761082282922,
0.));
#157787=CARTESIAN_POINT('Ctrl Pts',(-17.2474212398275,68.9539843211618,
0.));
#157788=CARTESIAN_POINT('Ctrl Pts',(-17.248877910643,68.9319057029407,0.));
#157789=CARTESIAN_POINT('Ctrl Pts',(-17.2503090604792,68.9098725237868,
0.));
#157790=CARTESIAN_POINT('Ctrl Pts',(-17.2517147520376,68.8878849345557,
0.));
#157791=CARTESIAN_POINT('Ctrl Pts',(-17.2530950484259,68.8659430867977,
0.));
#157792=CARTESIAN_POINT('Ctrl Pts',(-17.2544500131627,68.8440471327563,
0.));
#157793=CARTESIAN_POINT('Ctrl Pts',(-17.2557797101816,68.8221972253954,
0.));
#157794=CARTESIAN_POINT('Ctrl Pts',(-17.2570842038385,68.8003935184193,
0.));
#157795=CARTESIAN_POINT('Ctrl Pts',(-17.2583635589197,68.7786361662876,
0.));
#157796=CARTESIAN_POINT('Ctrl Pts',(-17.2596178406545,68.7569253242312,
0.));
#157797=CARTESIAN_POINT('Ctrl Pts',(-17.2608471147178,68.7352611482519,
0.));
#157798=CARTESIAN_POINT('Ctrl Pts',(-17.2620514472176,68.7136437951075,
0.));
#157799=CARTESIAN_POINT('Ctrl Pts',(-17.263230904689,68.6920734222932,0.));
#157800=CARTESIAN_POINT('Ctrl Pts',(-17.2643855540896,68.6705501880263,
0.));
#157801=CARTESIAN_POINT('Ctrl Pts',(-17.2655154627935,68.6490742512085,
0.));
#157802=CARTESIAN_POINT('Ctrl Pts',(-17.2666206986091,68.6276457714757,
0.));
#157803=CARTESIAN_POINT('Ctrl Pts',(-17.2677013298061,68.6062649092781,
0.));
#157804=CARTESIAN_POINT('Ctrl Pts',(-17.2687574251429,68.5849318259449,
0.));
#157805=CARTESIAN_POINT('Ctrl Pts',(-17.2697890538956,68.5636466837502,
0.));
#157806=CARTESIAN_POINT('Ctrl Pts',(-17.2707962858912,68.5424096459746,
0.));
#157807=CARTESIAN_POINT('Ctrl Pts',(-17.2717791914538,68.5212208767835,
0.));
#157808=CARTESIAN_POINT('Ctrl Pts',(-17.2727378413485,68.5000805410897,
0.));
#157809=CARTESIAN_POINT('Ctrl Pts',(-17.2736723067367,68.4789888044357,
0.));
#157810=CARTESIAN_POINT('Ctrl Pts',(-17.2745826591125,68.4579458328208,
0.));
#157811=CARTESIAN_POINT('Ctrl Pts',(-17.2754689703001,68.4369517926803,
0.));
#157812=CARTESIAN_POINT('Ctrl Pts',(-17.2763313126026,68.4160068512781,
0.));
#157813=CARTESIAN_POINT('Ctrl Pts',(-17.2771697589387,68.3951111770498,
0.));
#157814=CARTESIAN_POINT('Ctrl Pts',(-17.2779843829605,68.374264939895,0.));
#157815=CARTESIAN_POINT('Ctrl Pts',(-17.2787752592475,68.353468311648,0.));
#157816=CARTESIAN_POINT('Ctrl Pts',(-17.2795424631789,68.3327214657533,
0.));
#157817=CARTESIAN_POINT('Ctrl Pts',(-17.2802860705807,68.3120245763884,
0.));
#157818=CARTESIAN_POINT('Ctrl Pts',(-17.2810061574352,68.2913778177258,
0.));
#157819=CARTESIAN_POINT('Ctrl Pts',(-17.2817027995838,68.2707813631761,
0.));
#157820=CARTESIAN_POINT('Ctrl Pts',(-17.2823760723886,68.250235384512,0.));
#157821=CARTESIAN_POINT('Ctrl Pts',(-17.2830260513879,68.2297400535339,
0.));
#157822=CARTESIAN_POINT('Ctrl Pts',(-17.2836528130825,68.2092955440591,
0.));
#157823=CARTESIAN_POINT('Ctrl Pts',(-17.2842564355796,68.1889020335418,
0.));
#157824=CARTESIAN_POINT('Ctrl Pts',(-17.2848369995283,68.1685597054193,
0.));
#157825=CARTESIAN_POINT('Ctrl Pts',(-17.2853945882059,68.1482687493176,
0.));
#157826=CARTESIAN_POINT('Ctrl Pts',(-17.2859292855694,68.1280293561473,
0.));
#157827=CARTESIAN_POINT('Ctrl Pts',(-17.2864411745455,68.1078417137865,
0.));
#157828=CARTESIAN_POINT('Ctrl Pts',(-17.2869303355438,68.0877060033229,
0.));
#157829=CARTESIAN_POINT('Ctrl Pts',(-17.2873968440855,68.0676223930469,
0.));
#157830=CARTESIAN_POINT('Ctrl Pts',(-17.2878407730981,68.0475910442494,
0.));
#157831=CARTESIAN_POINT('Ctrl Pts',(-17.2882621974737,68.027612122741,0.));
#157832=CARTESIAN_POINT('Ctrl Pts',(-17.28866119774,68.007685808115,0.));
#157833=CARTESIAN_POINT('Ctrl Pts',(-17.2890378644843,67.9878123049133,
0.));
#157834=CARTESIAN_POINT('Ctrl Pts',(-17.2893923013852,67.9679918502441,
0.));
#157835=CARTESIAN_POINT('Ctrl Pts',(-17.2897246158895,67.9482246901517,
0.));
#157836=CARTESIAN_POINT('Ctrl Pts',(-17.2900349103956,67.9285110571662,
0.));
#157837=CARTESIAN_POINT('Ctrl Pts',(-17.2903232740717,67.908851149676,0.));
#157838=CARTESIAN_POINT('Ctrl Pts',(-17.2905897724029,67.8892451049871,
0.));
#157839=CARTESIAN_POINT('Ctrl Pts',(-17.2908344459816,67.8696929979178,
0.));
#157840=CARTESIAN_POINT('Ctrl Pts',(-17.2910127431203,67.8540944890057,
0.));
#157841=CARTESIAN_POINT('Ctrl Pts',(-17.2911366591419,67.8424198971214,
0.));
#157842=CARTESIAN_POINT('Ctrl Pts',(-17.2912149114145,67.8346476309106,
0.));
#157843=CARTESIAN_POINT('Ctrl Pts',(-17.2912529479484,67.8307641965655,
0.));
#157844=CARTESIAN_POINT('Ctrl Pts',(-10.343287191141,73.778495580227,0.));
#157845=CARTESIAN_POINT('Ctrl Pts',(-10.343287191141,73.778495580227,12.));
#157846=CARTESIAN_POINT('Ctrl Pts',(-10.3449014384453,73.7731377048058,
0.));
#157847=CARTESIAN_POINT('Ctrl Pts',(-10.3449014384453,73.7731377048058,
12.));
#157848=CARTESIAN_POINT('Ctrl Pts',(-10.3481265449342,73.7624245587789,
0.));
#157849=CARTESIAN_POINT('Ctrl Pts',(-10.3481265449342,73.7624245587789,
12.));
#157850=CARTESIAN_POINT('Ctrl Pts',(-10.3529540403092,73.7463626541854,
0.));
#157851=CARTESIAN_POINT('Ctrl Pts',(-10.3529540403092,73.7463626541854,
12.));
#157852=CARTESIAN_POINT('Ctrl Pts',(-10.359370371262,73.7249624109173,0.));
#157853=CARTESIAN_POINT('Ctrl Pts',(-10.359370371262,73.7249624109173,12.));
#157854=CARTESIAN_POINT('Ctrl Pts',(-10.3673568984582,73.6982381645206,
0.));
#157855=CARTESIAN_POINT('Ctrl Pts',(-10.3673568984582,73.6982381645206,
12.));
#157856=CARTESIAN_POINT('Ctrl Pts',(-10.3753095356342,73.6715399947839,
0.));
#157857=CARTESIAN_POINT('Ctrl Pts',(-10.3753095356342,73.6715399947839,
12.));
#157858=CARTESIAN_POINT('Ctrl Pts',(-10.3832282820371,73.6448679350696,
0.));
#157859=CARTESIAN_POINT('Ctrl Pts',(-10.3832282820371,73.6448679350696,
12.));
#157860=CARTESIAN_POINT('Ctrl Pts',(-10.3911131417463,73.6182220363156,
0.));
#157861=CARTESIAN_POINT('Ctrl Pts',(-10.3911131417463,73.6182220363156,
12.));
#157862=CARTESIAN_POINT('Ctrl Pts',(-10.3989641265285,73.5916023719713,
0.));
#157863=CARTESIAN_POINT('Ctrl Pts',(-10.3989641265285,73.5916023719713,
12.));
#157864=CARTESIAN_POINT('Ctrl Pts',(-10.406781255551,73.5650090359839,0.));
#157865=CARTESIAN_POINT('Ctrl Pts',(-10.406781255551,73.5650090359839,12.));
#157866=CARTESIAN_POINT('Ctrl Pts',(-10.414564552681,73.5384421354543,0.));
#157867=CARTESIAN_POINT('Ctrl Pts',(-10.414564552681,73.5384421354543,12.));
#157868=CARTESIAN_POINT('Ctrl Pts',(-10.4223140444605,73.5119017847575,
0.));
#157869=CARTESIAN_POINT('Ctrl Pts',(-10.4223140444605,73.5119017847575,
12.));
#157870=CARTESIAN_POINT('Ctrl Pts',(-10.430029757865,73.485388099225,0.));
#157871=CARTESIAN_POINT('Ctrl Pts',(-10.430029757865,73.485388099225,12.));
#157872=CARTESIAN_POINT('Ctrl Pts',(-10.4377117180222,73.4589011886197,
0.));
#157873=CARTESIAN_POINT('Ctrl Pts',(-10.4377117180222,73.4589011886197,
12.));
#157874=CARTESIAN_POINT('Ctrl Pts',(-10.4453599463547,73.4324411518554,
0.));
#157875=CARTESIAN_POINT('Ctrl Pts',(-10.4453599463547,73.4324411518554,
12.));
#157876=CARTESIAN_POINT('Ctrl Pts',(-10.452974461845,73.4060080806686,0.));
#157877=CARTESIAN_POINT('Ctrl Pts',(-10.452974461845,73.4060080806686,12.));
#157878=CARTESIAN_POINT('Ctrl Pts',(-10.4605552819397,73.37960206225,0.));
#157879=CARTESIAN_POINT('Ctrl Pts',(-10.4605552819397,73.37960206225,12.));
#157880=CARTESIAN_POINT('Ctrl Pts',(-10.4681024236289,73.3532231823659,
0.));
#157881=CARTESIAN_POINT('Ctrl Pts',(-10.4681024236289,73.3532231823659,
12.));
#157882=CARTESIAN_POINT('Ctrl Pts',(-10.4756159043806,73.3268715280575,
0.));
#157883=CARTESIAN_POINT('Ctrl Pts',(-10.4756159043806,73.3268715280575,
12.));
#157884=CARTESIAN_POINT('Ctrl Pts',(-10.4830957433305,73.3005471910583,
0.));
#157885=CARTESIAN_POINT('Ctrl Pts',(-10.4830957433305,73.3005471910583,
12.));
#157886=CARTESIAN_POINT('Ctrl Pts',(-10.4905419611523,73.2742502674304,
0.));
#157887=CARTESIAN_POINT('Ctrl Pts',(-10.4905419611523,73.2742502674304,
12.));
#157888=CARTESIAN_POINT('Ctrl Pts',(-10.4979545795192,73.2479808560189,
0.));
#157889=CARTESIAN_POINT('Ctrl Pts',(-10.4979545795192,73.2479808560189,
12.));
#157890=CARTESIAN_POINT('Ctrl Pts',(-10.5053336206908,73.2217390572562,
0.));
#157891=CARTESIAN_POINT('Ctrl Pts',(-10.5053336206908,73.2217390572562,
12.));
#157892=CARTESIAN_POINT('Ctrl Pts',(-10.5126791070805,73.1955249719048,
0.));
#157893=CARTESIAN_POINT('Ctrl Pts',(-10.5126791070805,73.1955249719048,
12.));
#157894=CARTESIAN_POINT('Ctrl Pts',(-10.5199910607654,73.1693386996138,
0.));
#157895=CARTESIAN_POINT('Ctrl Pts',(-10.5199910607654,73.1693386996138,
12.));
#157896=CARTESIAN_POINT('Ctrl Pts',(-10.5272695032653,73.1431803382711,
0.));
#157897=CARTESIAN_POINT('Ctrl Pts',(-10.5272695032653,73.1431803382711,
12.));
#157898=CARTESIAN_POINT('Ctrl Pts',(-10.53451445581,73.1170499848039,0.));
#157899=CARTESIAN_POINT('Ctrl Pts',(-10.53451445581,73.1170499848039,12.));
#157900=CARTESIAN_POINT('Ctrl Pts',(-10.5417259395003,73.0909477356474,
0.));
#157901=CARTESIAN_POINT('Ctrl Pts',(-10.5417259395003,73.0909477356474,
12.));
#157902=CARTESIAN_POINT('Ctrl Pts',(-10.5489039755138,73.0648736873434,
0.));
#157903=CARTESIAN_POINT('Ctrl Pts',(-10.5489039755138,73.0648736873434,
12.));
#157904=CARTESIAN_POINT('Ctrl Pts',(-10.5560485852974,73.0388279370834,
0.));
#157905=CARTESIAN_POINT('Ctrl Pts',(-10.5560485852974,73.0388279370834,
12.));
#157906=CARTESIAN_POINT('Ctrl Pts',(-10.5631597907651,73.0128105832621,
0.));
#157907=CARTESIAN_POINT('Ctrl Pts',(-10.5631597907651,73.0128105832621,
12.));
#157908=CARTESIAN_POINT('Ctrl Pts',(-10.570237614205,72.9868217252283,0.));
#157909=CARTESIAN_POINT('Ctrl Pts',(-10.570237614205,72.9868217252283,12.));
#157910=CARTESIAN_POINT('Ctrl Pts',(-10.5772820781958,72.9608614630534,
0.));
#157911=CARTESIAN_POINT('Ctrl Pts',(-10.5772820781958,72.9608614630534,
12.));
#157912=CARTESIAN_POINT('Ctrl Pts',(-10.5842932055209,72.9349298972822,
0.));
#157913=CARTESIAN_POINT('Ctrl Pts',(-10.5842932055209,72.9349298972822,
12.));
#157914=CARTESIAN_POINT('Ctrl Pts',(-10.5912710190928,72.9090271287083,
0.));
#157915=CARTESIAN_POINT('Ctrl Pts',(-10.5912710190928,72.9090271287083,
12.));
#157916=CARTESIAN_POINT('Ctrl Pts',(-10.5982155418626,72.8831532580845,
0.));
#157917=CARTESIAN_POINT('Ctrl Pts',(-10.5982155418626,72.8831532580845,
12.));
#157918=CARTESIAN_POINT('Ctrl Pts',(-10.6051267968203,72.8573083861337,
0.));
#157919=CARTESIAN_POINT('Ctrl Pts',(-10.6051267968203,72.8573083861337,
12.));
#157920=CARTESIAN_POINT('Ctrl Pts',(-10.6120048070367,72.8314926136881,
0.));
#157921=CARTESIAN_POINT('Ctrl Pts',(-10.6120048070367,72.8314926136881,
12.));
#157922=CARTESIAN_POINT('Ctrl Pts',(-10.6188495956973,72.8057060417887,
0.));
#157923=CARTESIAN_POINT('Ctrl Pts',(-10.6188495956973,72.8057060417887,
12.));
#157924=CARTESIAN_POINT('Ctrl Pts',(-10.6256611861394,72.7799487717911,
0.));
#157925=CARTESIAN_POINT('Ctrl Pts',(-10.6256611861394,72.7799487717911,
12.));
#157926=CARTESIAN_POINT('Ctrl Pts',(-10.6324396018998,72.7542209054812,
0.));
#157927=CARTESIAN_POINT('Ctrl Pts',(-10.6324396018998,72.7542209054812,
12.));
#157928=CARTESIAN_POINT('Ctrl Pts',(-10.6391848667352,72.7285225451293,
0.));
#157929=CARTESIAN_POINT('Ctrl Pts',(-10.6391848667352,72.7285225451293,
12.));
#157930=CARTESIAN_POINT('Ctrl Pts',(-10.6458970045946,72.7028537934317,
0.));
#157931=CARTESIAN_POINT('Ctrl Pts',(-10.6458970045946,72.7028537934317,
12.));
#157932=CARTESIAN_POINT('Ctrl Pts',(-10.6525760396054,72.6772147534752,
0.));
#157933=CARTESIAN_POINT('Ctrl Pts',(-10.6525760396054,72.6772147534752,
12.));
#157934=CARTESIAN_POINT('Ctrl Pts',(-10.659221996058,72.651605528691,0.));
#157935=CARTESIAN_POINT('Ctrl Pts',(-10.659221996058,72.651605528691,12.));
#157936=CARTESIAN_POINT('Ctrl Pts',(-10.6658348983944,72.6260262228065,
0.));
#157937=CARTESIAN_POINT('Ctrl Pts',(-10.6658348983944,72.6260262228065,
12.));
#157938=CARTESIAN_POINT('Ctrl Pts',(-10.6724147711995,72.6004769398019,
0.));
#157939=CARTESIAN_POINT('Ctrl Pts',(-10.6724147711995,72.6004769398019,
12.));
#157940=CARTESIAN_POINT('Ctrl Pts',(-10.6789616392042,72.5749577839415,
0.));
#157941=CARTESIAN_POINT('Ctrl Pts',(-10.6789616392042,72.5749577839415,
12.));
#157942=CARTESIAN_POINT('Ctrl Pts',(-10.6854755272904,72.5494688597961,
0.));
#157943=CARTESIAN_POINT('Ctrl Pts',(-10.6854755272904,72.5494688597961,
12.));
#157944=CARTESIAN_POINT('Ctrl Pts',(-10.691956460499,72.5240102722664,0.));
#157945=CARTESIAN_POINT('Ctrl Pts',(-10.691956460499,72.5240102722664,12.));
#157946=CARTESIAN_POINT('Ctrl Pts',(-10.6984044640398,72.4985821266023,
0.));
#157947=CARTESIAN_POINT('Ctrl Pts',(-10.6984044640398,72.4985821266023,
12.));
#157948=CARTESIAN_POINT('Ctrl Pts',(-10.7048195633061,72.4731845284227,
0.));
#157949=CARTESIAN_POINT('Ctrl Pts',(-10.7048195633061,72.4731845284227,
12.));
#157950=CARTESIAN_POINT('Ctrl Pts',(-10.7112017838706,72.4478175837156,
0.));
#157951=CARTESIAN_POINT('Ctrl Pts',(-10.7112017838706,72.4478175837156,
12.));
#157952=CARTESIAN_POINT('Ctrl Pts',(-10.7175511514788,72.4224813988347,
0.));
#157953=CARTESIAN_POINT('Ctrl Pts',(-10.7175511514788,72.4224813988347,
12.));
#157954=CARTESIAN_POINT('Ctrl Pts',(-10.7238676920469,72.3971760804933,
0.));
#157955=CARTESIAN_POINT('Ctrl Pts',(-10.7238676920469,72.3971760804933,
12.));
#157956=CARTESIAN_POINT('Ctrl Pts',(-10.7301514316607,72.3719017357571,
0.));
#157957=CARTESIAN_POINT('Ctrl Pts',(-10.7301514316607,72.3719017357571,
12.));
#157958=CARTESIAN_POINT('Ctrl Pts',(-10.73640239658,72.3466584720318,0.));
#157959=CARTESIAN_POINT('Ctrl Pts',(-10.73640239658,72.3466584720318,12.));
#157960=CARTESIAN_POINT('Ctrl Pts',(-10.7426206132375,72.3214463970641,
0.));
#157961=CARTESIAN_POINT('Ctrl Pts',(-10.7426206132375,72.3214463970641,
12.));
#157962=CARTESIAN_POINT('Ctrl Pts',(-10.7488061082368,72.2962656189556,
0.));
#157963=CARTESIAN_POINT('Ctrl Pts',(-10.7488061082368,72.2962656189556,
12.));
#157964=CARTESIAN_POINT('Ctrl Pts',(-10.7549589083535,72.2711162461681,
0.));
#157965=CARTESIAN_POINT('Ctrl Pts',(-10.7549589083535,72.2711162461681,
12.));
#157966=CARTESIAN_POINT('Ctrl Pts',(-10.7610790405385,72.2459983875296,
0.));
#157967=CARTESIAN_POINT('Ctrl Pts',(-10.7610790405385,72.2459983875296,
12.));
#157968=CARTESIAN_POINT('Ctrl Pts',(-10.7671665319255,72.2209121522366,
0.));
#157969=CARTESIAN_POINT('Ctrl Pts',(-10.7671665319255,72.2209121522366,
12.));
#157970=CARTESIAN_POINT('Ctrl Pts',(-10.7732214098344,72.1958576498558,
0.));
#157971=CARTESIAN_POINT('Ctrl Pts',(-10.7732214098344,72.1958576498558,
12.));
#157972=CARTESIAN_POINT('Ctrl Pts',(-10.7792437017662,72.1708349903305,
0.));
#157973=CARTESIAN_POINT('Ctrl Pts',(-10.7792437017662,72.1708349903305,
12.));
#157974=CARTESIAN_POINT('Ctrl Pts',(-10.7852334354016,72.1458442839834,
0.));
#157975=CARTESIAN_POINT('Ctrl Pts',(-10.7852334354016,72.1458442839834,
12.));
#157976=CARTESIAN_POINT('Ctrl Pts',(-10.7911906386027,72.1208856415171,
0.));
#157977=CARTESIAN_POINT('Ctrl Pts',(-10.7911906386027,72.1208856415171,
12.));
#157978=CARTESIAN_POINT('Ctrl Pts',(-10.7971153394166,72.0959591740114,
0.));
#157979=CARTESIAN_POINT('Ctrl Pts',(-10.7971153394166,72.0959591740114,
12.));
#157980=CARTESIAN_POINT('Ctrl Pts',(-10.8030075660808,72.0710649929202,
0.));
#157981=CARTESIAN_POINT('Ctrl Pts',(-10.8030075660808,72.0710649929202,
12.));
#157982=CARTESIAN_POINT('Ctrl Pts',(-10.8088673470184,72.0462032100815,
0.));
#157983=CARTESIAN_POINT('Ctrl Pts',(-10.8088673470184,72.0462032100815,
12.));
#157984=CARTESIAN_POINT('Ctrl Pts',(-10.8146947108375,72.0213739377223,
0.));
#157985=CARTESIAN_POINT('Ctrl Pts',(-10.8146947108375,72.0213739377223,
12.));
#157986=CARTESIAN_POINT('Ctrl Pts',(-10.8204896863328,71.9965772884619,
0.));
#157987=CARTESIAN_POINT('Ctrl Pts',(-10.8204896863328,71.9965772884619,
12.));
#157988=CARTESIAN_POINT('Ctrl Pts',(-10.8262523024898,71.9718133753127,
0.));
#157989=CARTESIAN_POINT('Ctrl Pts',(-10.8262523024898,71.9718133753127,
12.));
#157990=CARTESIAN_POINT('Ctrl Pts',(-10.8319825884918,71.9470823116785,
0.));
#157991=CARTESIAN_POINT('Ctrl Pts',(-10.8319825884918,71.9470823116785,
12.));
#157992=CARTESIAN_POINT('Ctrl Pts',(-10.8376805737159,71.9223842113625,
0.));
#157993=CARTESIAN_POINT('Ctrl Pts',(-10.8376805737159,71.9223842113625,
12.));
#157994=CARTESIAN_POINT('Ctrl Pts',(-10.8433462877311,71.8977191885725,
0.));
#157995=CARTESIAN_POINT('Ctrl Pts',(-10.8433462877311,71.8977191885725,
12.));
#157996=CARTESIAN_POINT('Ctrl Pts',(-10.8489797602997,71.8730873579224,
0.));
#157997=CARTESIAN_POINT('Ctrl Pts',(-10.8489797602997,71.8730873579224,
12.));
#157998=CARTESIAN_POINT('Ctrl Pts',(-10.8545810213799,71.8484888344339,
0.));
#157999=CARTESIAN_POINT('Ctrl Pts',(-10.8545810213799,71.8484888344339,
12.));
#158000=CARTESIAN_POINT('Ctrl Pts',(-10.8601501011332,71.8239237335331,
0.));
#158001=CARTESIAN_POINT('Ctrl Pts',(-10.8601501011332,71.8239237335331,
12.));
#158002=CARTESIAN_POINT('Ctrl Pts',(-10.865687029922,71.7993921710564,0.));
#158003=CARTESIAN_POINT('Ctrl Pts',(-10.865687029922,71.7993921710564,12.));
#158004=CARTESIAN_POINT('Ctrl Pts',(-10.8711918383073,71.7748942632593,
0.));
#158005=CARTESIAN_POINT('Ctrl Pts',(-10.8711918383073,71.7748942632593,
12.));
#158006=CARTESIAN_POINT('Ctrl Pts',(-10.8766645570497,71.7504301268181,
0.));
#158007=CARTESIAN_POINT('Ctrl Pts',(-10.8766645570497,71.7504301268181,
12.));
#158008=CARTESIAN_POINT('Ctrl Pts',(-10.8821052171121,71.7259998788328,
0.));
#158009=CARTESIAN_POINT('Ctrl Pts',(-10.8821052171121,71.7259998788328,
12.));
#158010=CARTESIAN_POINT('Ctrl Pts',(-10.8875138496671,71.7016036368236,
0.));
#158011=CARTESIAN_POINT('Ctrl Pts',(-10.8875138496671,71.7016036368236,
12.));
#158012=CARTESIAN_POINT('Ctrl Pts',(-10.8928904860964,71.6772415187364,
0.));
#158013=CARTESIAN_POINT('Ctrl Pts',(-10.8928904860964,71.6772415187364,
12.));
#158014=CARTESIAN_POINT('Ctrl Pts',(-10.8982351579871,71.6529136429504,
0.));
#158015=CARTESIAN_POINT('Ctrl Pts',(-10.8982351579871,71.6529136429504,
12.));
#158016=CARTESIAN_POINT('Ctrl Pts',(-10.9035478971328,71.6286201282812,
0.));
#158017=CARTESIAN_POINT('Ctrl Pts',(-10.9035478971328,71.6286201282812,
12.));
#158018=CARTESIAN_POINT('Ctrl Pts',(-10.9088287355365,71.6043610939835,
0.));
#158019=CARTESIAN_POINT('Ctrl Pts',(-10.9088287355365,71.6043610939835,
12.));
#158020=CARTESIAN_POINT('Ctrl Pts',(-10.914077705417,71.5801366597488,0.));
#158021=CARTESIAN_POINT('Ctrl Pts',(-10.914077705417,71.5801366597488,12.));
#158022=CARTESIAN_POINT('Ctrl Pts',(-10.91929483921,71.5559469457091,0.));
#158023=CARTESIAN_POINT('Ctrl Pts',(-10.91929483921,71.5559469457091,12.));
#158024=CARTESIAN_POINT('Ctrl Pts',(-10.9244801695642,71.5317920724459,
0.));
#158025=CARTESIAN_POINT('Ctrl Pts',(-10.9244801695642,71.5317920724459,
12.));
#158026=CARTESIAN_POINT('Ctrl Pts',(-10.9296337293424,71.5076721609937,
0.));
#158027=CARTESIAN_POINT('Ctrl Pts',(-10.9296337293424,71.5076721609937,
12.));
#158028=CARTESIAN_POINT('Ctrl Pts',(-10.9347555516235,71.4835873328423,
0.));
#158029=CARTESIAN_POINT('Ctrl Pts',(-10.9347555516235,71.4835873328423,
12.));
#158030=CARTESIAN_POINT('Ctrl Pts',(-10.9398456697095,71.4595377099351,
0.));
#158031=CARTESIAN_POINT('Ctrl Pts',(-10.9398456697095,71.4595377099351,
12.));
#158032=CARTESIAN_POINT('Ctrl Pts',(-10.944904117127,71.435523414672,0.));
#158033=CARTESIAN_POINT('Ctrl Pts',(-10.944904117127,71.435523414672,12.));
#158034=CARTESIAN_POINT('Ctrl Pts',(-10.9499309276236,71.4115445699194,
0.));
#158035=CARTESIAN_POINT('Ctrl Pts',(-10.9499309276236,71.4115445699194,
12.));
#158036=CARTESIAN_POINT('Ctrl Pts',(-10.954926135169,71.3876012990138,0.));
#158037=CARTESIAN_POINT('Ctrl Pts',(-10.954926135169,71.3876012990138,12.));
#158038=CARTESIAN_POINT('Ctrl Pts',(-10.9598897739564,71.3636937257649,
0.));
#158039=CARTESIAN_POINT('Ctrl Pts',(-10.9598897739564,71.3636937257649,
12.));
#158040=CARTESIAN_POINT('Ctrl Pts',(-10.9648218784098,71.339821974454,0.));
#158041=CARTESIAN_POINT('Ctrl Pts',(-10.9648218784098,71.339821974454,12.));
#158042=CARTESIAN_POINT('Ctrl Pts',(-10.969722483186,71.3159861698358,0.));
#158043=CARTESIAN_POINT('Ctrl Pts',(-10.969722483186,71.3159861698358,12.));
#158044=CARTESIAN_POINT('Ctrl Pts',(-10.9745916231709,71.2921864371491,
0.));
#158045=CARTESIAN_POINT('Ctrl Pts',(-10.9745916231709,71.2921864371491,
12.));
#158046=CARTESIAN_POINT('Ctrl Pts',(-10.9794293334805,71.2684229021207,
0.));
#158047=CARTESIAN_POINT('Ctrl Pts',(-10.9794293334805,71.2684229021207,
12.));
#158048=CARTESIAN_POINT('Ctrl Pts',(-10.9842356494627,71.2446956909687,
0.));
#158049=CARTESIAN_POINT('Ctrl Pts',(-10.9842356494627,71.2446956909687,
12.));
#158050=CARTESIAN_POINT('Ctrl Pts',(-10.9890106067039,71.2210049304014,
0.));
#158051=CARTESIAN_POINT('Ctrl Pts',(-10.9890106067039,71.2210049304014,
12.));
#158052=CARTESIAN_POINT('Ctrl Pts',(-10.993754241032,71.1973507476191,0.));
#158053=CARTESIAN_POINT('Ctrl Pts',(-10.993754241032,71.1973507476191,12.));
#158054=CARTESIAN_POINT('Ctrl Pts',(-10.9984665885127,71.1737332703248,
0.));
#158055=CARTESIAN_POINT('Ctrl Pts',(-10.9984665885127,71.1737332703248,
12.));
#158056=CARTESIAN_POINT('Ctrl Pts',(-11.0031476854502,71.1501526267286,
0.));
#158057=CARTESIAN_POINT('Ctrl Pts',(-11.0031476854502,71.1501526267286,
12.));
#158058=CARTESIAN_POINT('Ctrl Pts',(-11.0077975683895,71.1266089455517,
0.));
#158059=CARTESIAN_POINT('Ctrl Pts',(-11.0077975683895,71.1266089455517,
12.));
#158060=CARTESIAN_POINT('Ctrl Pts',(-11.0124162741224,71.1031023560249,
0.));
#158061=CARTESIAN_POINT('Ctrl Pts',(-11.0124162741224,71.1031023560249,
12.));
#158062=CARTESIAN_POINT('Ctrl Pts',(-11.0170038396915,71.0796329878907,
0.));
#158063=CARTESIAN_POINT('Ctrl Pts',(-11.0170038396915,71.0796329878907,
12.));
#158064=CARTESIAN_POINT('Ctrl Pts',(-11.0215603023856,71.0562009714136,
0.));
#158065=CARTESIAN_POINT('Ctrl Pts',(-11.0215603023856,71.0562009714136,
12.));
#158066=CARTESIAN_POINT('Ctrl Pts',(-11.0260856997415,71.0328064373856,
0.));
#158067=CARTESIAN_POINT('Ctrl Pts',(-11.0260856997415,71.0328064373856,
12.));
#158068=CARTESIAN_POINT('Ctrl Pts',(-11.0305800695456,71.0094495171292,
0.));
#158069=CARTESIAN_POINT('Ctrl Pts',(-11.0305800695456,71.0094495171292,
12.));
#158070=CARTESIAN_POINT('Ctrl Pts',(-11.0350434498405,70.986130342497,0.));
#158071=CARTESIAN_POINT('Ctrl Pts',(-11.0350434498405,70.986130342497,12.));
#158072=CARTESIAN_POINT('Ctrl Pts',(-11.0394758789285,70.9628490458748,
0.));
#158073=CARTESIAN_POINT('Ctrl Pts',(-11.0394758789285,70.9628490458748,
12.));
#158074=CARTESIAN_POINT('Ctrl Pts',(-11.0438773953681,70.9396057601924,
0.));
#158075=CARTESIAN_POINT('Ctrl Pts',(-11.0438773953681,70.9396057601924,
12.));
#158076=CARTESIAN_POINT('Ctrl Pts',(-11.048248037975,70.916400618927,0.));
#158077=CARTESIAN_POINT('Ctrl Pts',(-11.048248037975,70.916400618927,12.));
#158078=CARTESIAN_POINT('Ctrl Pts',(-11.0525878458243,70.8932337561087,
0.));
#158079=CARTESIAN_POINT('Ctrl Pts',(-11.0525878458243,70.8932337561087,
12.));
#158080=CARTESIAN_POINT('Ctrl Pts',(-11.0568968582569,70.8701053063186,
0.));
#158081=CARTESIAN_POINT('Ctrl Pts',(-11.0568968582569,70.8701053063186,
12.));
#158082=CARTESIAN_POINT('Ctrl Pts',(-11.0611751148835,70.8470154046919,
0.));
#158083=CARTESIAN_POINT('Ctrl Pts',(-11.0611751148835,70.8470154046919,
12.));
#158084=CARTESIAN_POINT('Ctrl Pts',(-11.0654226555802,70.8239641869299,
0.));
#158085=CARTESIAN_POINT('Ctrl Pts',(-11.0654226555802,70.8239641869299,
12.));
#158086=CARTESIAN_POINT('Ctrl Pts',(-11.0696395204909,70.8009517893057,
0.));
#158087=CARTESIAN_POINT('Ctrl Pts',(-11.0696395204909,70.8009517893057,
12.));
#158088=CARTESIAN_POINT('Ctrl Pts',(-11.073825750029,70.7779783486677,0.));
#158089=CARTESIAN_POINT('Ctrl Pts',(-11.073825750029,70.7779783486677,12.));
#158090=CARTESIAN_POINT('Ctrl Pts',(-11.0779813848846,70.7550440024384,
0.));
#158091=CARTESIAN_POINT('Ctrl Pts',(-11.0779813848846,70.7550440024384,
12.));
#158092=CARTESIAN_POINT('Ctrl Pts',(-11.0821064660269,70.732148888618,0.));
#158093=CARTESIAN_POINT('Ctrl Pts',(-11.0821064660269,70.732148888618,12.));
#158094=CARTESIAN_POINT('Ctrl Pts',(-11.0862010347016,70.7092931457954,
0.));
#158095=CARTESIAN_POINT('Ctrl Pts',(-11.0862010347016,70.7092931457954,
12.));
#158096=CARTESIAN_POINT('Ctrl Pts',(-11.0902651324323,70.6864769131546,
0.));
#158097=CARTESIAN_POINT('Ctrl Pts',(-11.0902651324323,70.6864769131546,
12.));
#158098=CARTESIAN_POINT('Ctrl Pts',(-11.0942988010233,70.6637003304785,
0.));
#158099=CARTESIAN_POINT('Ctrl Pts',(-11.0942988010233,70.6637003304785,
12.));
#158100=CARTESIAN_POINT('Ctrl Pts',(-11.0983020825667,70.6409635381482,
0.));
#158101=CARTESIAN_POINT('Ctrl Pts',(-11.0983020825667,70.6409635381482,
12.));
#158102=CARTESIAN_POINT('Ctrl Pts',(-11.1022750194446,70.6182666771481,
0.));
#158103=CARTESIAN_POINT('Ctrl Pts',(-11.1022750194446,70.6182666771481,
12.));
#158104=CARTESIAN_POINT('Ctrl Pts',(-11.1062176543262,70.5956098890773,
0.));
#158105=CARTESIAN_POINT('Ctrl Pts',(-11.1062176543262,70.5956098890773,
12.));
#158106=CARTESIAN_POINT('Ctrl Pts',(-11.1101300301701,70.5729933161546,
0.));
#158107=CARTESIAN_POINT('Ctrl Pts',(-11.1101300301701,70.5729933161546,
12.));
#158108=CARTESIAN_POINT('Ctrl Pts',(-11.1140121902271,70.5504171012233,
0.));
#158109=CARTESIAN_POINT('Ctrl Pts',(-11.1140121902271,70.5504171012233,
12.));
#158110=CARTESIAN_POINT('Ctrl Pts',(-11.1178641780476,70.5278813877494,
0.));
#158111=CARTESIAN_POINT('Ctrl Pts',(-11.1178641780476,70.5278813877494,
12.));
#158112=CARTESIAN_POINT('Ctrl Pts',(-11.1216860374826,70.505386319828,0.));
#158113=CARTESIAN_POINT('Ctrl Pts',(-11.1216860374826,70.505386319828,12.));
#158114=CARTESIAN_POINT('Ctrl Pts',(-11.1254778126821,70.4829320421957,
0.));
#158115=CARTESIAN_POINT('Ctrl Pts',(-11.1254778126821,70.4829320421957,
12.));
#158116=CARTESIAN_POINT('Ctrl Pts',(-11.1292395480974,70.4605187002354,
0.));
#158117=CARTESIAN_POINT('Ctrl Pts',(-11.1292395480974,70.4605187002354,
12.));
#158118=CARTESIAN_POINT('Ctrl Pts',(-11.1329712884846,70.4381464399819,
0.));
#158119=CARTESIAN_POINT('Ctrl Pts',(-11.1329712884846,70.4381464399819,
12.));
#158120=CARTESIAN_POINT('Ctrl Pts',(-11.1366730789126,70.4158154081205,
0.));
#158121=CARTESIAN_POINT('Ctrl Pts',(-11.1366730789126,70.4158154081205,
12.));
#158122=CARTESIAN_POINT('Ctrl Pts',(-11.1403449647625,70.393525751996,0.));
#158123=CARTESIAN_POINT('Ctrl Pts',(-11.1403449647625,70.393525751996,12.));
#158124=CARTESIAN_POINT('Ctrl Pts',(-11.143986991727,70.3712776196223,0.));
#158125=CARTESIAN_POINT('Ctrl Pts',(-11.143986991727,70.3712776196223,12.));
#158126=CARTESIAN_POINT('Ctrl Pts',(-11.1475992058124,70.349071159688,0.));
#158127=CARTESIAN_POINT('Ctrl Pts',(-11.1475992058124,70.349071159688,12.));
#158128=CARTESIAN_POINT('Ctrl Pts',(-11.1511816533421,70.326906521559,0.));
#158129=CARTESIAN_POINT('Ctrl Pts',(-11.1511816533421,70.326906521559,12.));
#158130=CARTESIAN_POINT('Ctrl Pts',(-11.1547343809646,70.3047838552756,
0.));
#158131=CARTESIAN_POINT('Ctrl Pts',(-11.1547343809646,70.3047838552756,
12.));
#158132=CARTESIAN_POINT('Ctrl Pts',(-11.1582574356521,70.2827033115662,
0.));
#158133=CARTESIAN_POINT('Ctrl Pts',(-11.1582574356521,70.2827033115662,
12.));
#158134=CARTESIAN_POINT('Ctrl Pts',(-11.1617508647016,70.2606650418589,
0.));
#158135=CARTESIAN_POINT('Ctrl Pts',(-11.1617508647016,70.2606650418589,
12.));
#158136=CARTESIAN_POINT('Ctrl Pts',(-11.1652147157383,70.2386691982902,
0.));
#158137=CARTESIAN_POINT('Ctrl Pts',(-11.1652147157383,70.2386691982902,
12.));
#158138=CARTESIAN_POINT('Ctrl Pts',(-11.168649036721,70.2167159337094,0.));
#158139=CARTESIAN_POINT('Ctrl Pts',(-11.168649036721,70.2167159337094,12.));
#158140=CARTESIAN_POINT('Ctrl Pts',(-11.1720538759499,70.1948054016816,
0.));
#158141=CARTESIAN_POINT('Ctrl Pts',(-11.1720538759499,70.1948054016816,
12.));
#158142=CARTESIAN_POINT('Ctrl Pts',(-11.1754292820631,70.1729377564954,
0.));
#158143=CARTESIAN_POINT('Ctrl Pts',(-11.1754292820631,70.1729377564954,
12.));
#158144=CARTESIAN_POINT('Ctrl Pts',(-11.1787753040363,70.1511131531672,
0.));
#158145=CARTESIAN_POINT('Ctrl Pts',(-11.1787753040363,70.1511131531672,
12.));
#158146=CARTESIAN_POINT('Ctrl Pts',(-11.1820919911846,70.1293317474432,
0.));
#158147=CARTESIAN_POINT('Ctrl Pts',(-11.1820919911846,70.1293317474432,
12.));
#158148=CARTESIAN_POINT('Ctrl Pts',(-11.185379393167,70.1075936957973,0.));
#158149=CARTESIAN_POINT('Ctrl Pts',(-11.185379393167,70.1075936957973,12.));
#158150=CARTESIAN_POINT('Ctrl Pts',(-11.1886375599916,70.0858991554295,
0.));
#158151=CARTESIAN_POINT('Ctrl Pts',(-11.1886375599916,70.0858991554295,
12.));
#158152=CARTESIAN_POINT('Ctrl Pts',(-11.1918665420168,70.0642482842942,
0.));
#158153=CARTESIAN_POINT('Ctrl Pts',(-11.1918665420168,70.0642482842942,
12.));
#158154=CARTESIAN_POINT('Ctrl Pts',(-11.1950663899578,70.0426412411194,
0.));
#158155=CARTESIAN_POINT('Ctrl Pts',(-11.1950663899578,70.0426412411194,
12.));
#158156=CARTESIAN_POINT('Ctrl Pts',(-11.1982371548918,70.0210781854236,
0.));
#158157=CARTESIAN_POINT('Ctrl Pts',(-11.1982371548918,70.0210781854236,
12.));
#158158=CARTESIAN_POINT('Ctrl Pts',(-11.2013788882711,69.9995592775322,
0.));
#158159=CARTESIAN_POINT('Ctrl Pts',(-11.2013788882711,69.9995592775322,
12.));
#158160=CARTESIAN_POINT('Ctrl Pts',(-11.2044916419239,69.9780846785771,
0.));
#158161=CARTESIAN_POINT('Ctrl Pts',(-11.2044916419239,69.9780846785771,
12.));
#158162=CARTESIAN_POINT('Ctrl Pts',(-11.2075754680445,69.9566545504813,
0.));
#158163=CARTESIAN_POINT('Ctrl Pts',(-11.2075754680445,69.9566545504813,
12.));
#158164=CARTESIAN_POINT('Ctrl Pts',(-11.2106304191881,69.9352690559399,
0.));
#158165=CARTESIAN_POINT('Ctrl Pts',(-11.2106304191881,69.9352690559399,
12.));
#158166=CARTESIAN_POINT('Ctrl Pts',(-11.2136565482679,69.9139283584036,
0.));
#158167=CARTESIAN_POINT('Ctrl Pts',(-11.2136565482679,69.9139283584036,
12.));
#158168=CARTESIAN_POINT('Ctrl Pts',(-11.2166539085527,69.8926326220414,
0.));
#158169=CARTESIAN_POINT('Ctrl Pts',(-11.2166539085527,69.8926326220414,
12.));
#158170=CARTESIAN_POINT('Ctrl Pts',(-11.2196225536794,69.8713820117918,
0.));
#158171=CARTESIAN_POINT('Ctrl Pts',(-11.2196225536794,69.8713820117918,
12.));
#158172=CARTESIAN_POINT('Ctrl Pts',(-11.2225625376739,69.8501766934445,
0.));
#158173=CARTESIAN_POINT('Ctrl Pts',(-11.2225625376739,69.8501766934445,
12.));
#158174=CARTESIAN_POINT('Ctrl Pts',(-11.225473914972,69.8290168337076,0.));
#158175=CARTESIAN_POINT('Ctrl Pts',(-11.225473914972,69.8290168337076,12.));
#158176=CARTESIAN_POINT('Ctrl Pts',(-11.2283567404434,69.8079026002753,
0.));
#158177=CARTESIAN_POINT('Ctrl Pts',(-11.2283567404434,69.8079026002753,
12.));
#158178=CARTESIAN_POINT('Ctrl Pts',(-11.2312110694183,69.7868341618927,
0.));
#158179=CARTESIAN_POINT('Ctrl Pts',(-11.2312110694183,69.7868341618927,
12.));
#158180=CARTESIAN_POINT('Ctrl Pts',(-11.2340369576452,69.7658116882298,
0.));
#158181=CARTESIAN_POINT('Ctrl Pts',(-11.2340369576452,69.7658116882298,
12.));
#158182=CARTESIAN_POINT('Ctrl Pts',(-11.236834461247,69.7448353497394,0.));
#158183=CARTESIAN_POINT('Ctrl Pts',(-11.236834461247,69.7448353497394,12.));
#158184=CARTESIAN_POINT('Ctrl Pts',(-11.2396036366861,69.7239053175362,
0.));
#158185=CARTESIAN_POINT('Ctrl Pts',(-11.2396036366861,69.7239053175362,
12.));
#158186=CARTESIAN_POINT('Ctrl Pts',(-11.242344540717,69.7030217632187,0.));
#158187=CARTESIAN_POINT('Ctrl Pts',(-11.242344540717,69.7030217632187,12.));
#158188=CARTESIAN_POINT('Ctrl Pts',(-11.2450572303847,69.6821848588492,
0.));
#158189=CARTESIAN_POINT('Ctrl Pts',(-11.2450572303847,69.6821848588492,
12.));
#158190=CARTESIAN_POINT('Ctrl Pts',(-11.2477417631391,69.6613947773563,
0.));
#158191=CARTESIAN_POINT('Ctrl Pts',(-11.2477417631391,69.6613947773563,
12.));
#158192=CARTESIAN_POINT('Ctrl Pts',(-11.2503981969413,69.6406516928902,
0.));
#158193=CARTESIAN_POINT('Ctrl Pts',(-11.2503981969413,69.6406516928902,
12.));
#158194=CARTESIAN_POINT('Ctrl Pts',(-11.2530265903555,69.6199557811231,
0.));
#158195=CARTESIAN_POINT('Ctrl Pts',(-11.2530265903555,69.6199557811231,
12.));
#158196=CARTESIAN_POINT('Ctrl Pts',(-11.255627002701,69.5993072197355,0.));
#158197=CARTESIAN_POINT('Ctrl Pts',(-11.255627002701,69.5993072197355,12.));
#158198=CARTESIAN_POINT('Ctrl Pts',(-11.2581994939534,69.5787061880815,
0.));
#158199=CARTESIAN_POINT('Ctrl Pts',(-11.2581994939534,69.5787061880815,
12.));
#158200=CARTESIAN_POINT('Ctrl Pts',(-11.2607441244698,69.5581528662846,
0.));
#158201=CARTESIAN_POINT('Ctrl Pts',(-11.2607441244698,69.5581528662846,
12.));
#158202=CARTESIAN_POINT('Ctrl Pts',(-11.2632609547629,69.5376474344768,
0.));
#158203=CARTESIAN_POINT('Ctrl Pts',(-11.2632609547629,69.5376474344768,
12.));
#158204=CARTESIAN_POINT('Ctrl Pts',(-11.2657500452721,69.5171900720188,
0.));
#158205=CARTESIAN_POINT('Ctrl Pts',(-11.2657500452721,69.5171900720188,
12.));
#158206=CARTESIAN_POINT('Ctrl Pts',(-11.2682114561015,69.4967809565978,
0.));
#158207=CARTESIAN_POINT('Ctrl Pts',(-11.2682114561015,69.4967809565978,
12.));
#158208=CARTESIAN_POINT('Ctrl Pts',(-11.2706452475287,69.4764202659443,
0.));
#158209=CARTESIAN_POINT('Ctrl Pts',(-11.2706452475287,69.4764202659443,
12.));
#158210=CARTESIAN_POINT('Ctrl Pts',(-11.2730514806143,69.4561081798815,
0.));
#158211=CARTESIAN_POINT('Ctrl Pts',(-11.2730514806143,69.4561081798815,
12.));
#158212=CARTESIAN_POINT('Ctrl Pts',(-11.2754302177019,69.4358448819957,
0.));
#158213=CARTESIAN_POINT('Ctrl Pts',(-11.2754302177019,69.4358448819957,
12.));
#158214=CARTESIAN_POINT('Ctrl Pts',(-11.2777815231462,69.4156305620554,
0.));
#158215=CARTESIAN_POINT('Ctrl Pts',(-11.2777815231462,69.4156305620554,
12.));
#158216=CARTESIAN_POINT('Ctrl Pts',(-11.2801054633807,69.395465416223,0.));
#158217=CARTESIAN_POINT('Ctrl Pts',(-11.2801054633807,69.395465416223,12.));
#158218=CARTESIAN_POINT('Ctrl Pts',(-11.2824021054038,69.375349642,0.));
#158219=CARTESIAN_POINT('Ctrl Pts',(-11.2824021054038,69.375349642,12.));
#158220=CARTESIAN_POINT('Ctrl Pts',(-11.2846715154521,69.3552834337771,
0.));
#158221=CARTESIAN_POINT('Ctrl Pts',(-11.2846715154521,69.3552834337771,
12.));
#158222=CARTESIAN_POINT('Ctrl Pts',(-11.2869137578463,69.3352669789611,
0.));
#158223=CARTESIAN_POINT('Ctrl Pts',(-11.2869137578463,69.3352669789611,
12.));
#158224=CARTESIAN_POINT('Ctrl Pts',(-11.2891288931528,69.315300451784,0.));
#158225=CARTESIAN_POINT('Ctrl Pts',(-11.2891288931528,69.315300451784,12.));
#158226=CARTESIAN_POINT('Ctrl Pts',(-11.2913169799642,69.2953840192792,
0.));
#158227=CARTESIAN_POINT('Ctrl Pts',(-11.2913169799642,69.2953840192792,
12.));
#158228=CARTESIAN_POINT('Ctrl Pts',(-11.2934780784361,69.2755178531534,
0.));
#158229=CARTESIAN_POINT('Ctrl Pts',(-11.2934780784361,69.2755178531534,
12.));
#158230=CARTESIAN_POINT('Ctrl Pts',(-11.2956122531375,69.255702139335,0.));
#158231=CARTESIAN_POINT('Ctrl Pts',(-11.2956122531375,69.255702139335,12.));
#158232=CARTESIAN_POINT('Ctrl Pts',(-11.2977195764836,69.2359370894828,
0.));
#158233=CARTESIAN_POINT('Ctrl Pts',(-11.2977195764836,69.2359370894828,
12.));
#158234=CARTESIAN_POINT('Ctrl Pts',(-11.2998001310934,69.216222948839,0.));
#158235=CARTESIAN_POINT('Ctrl Pts',(-11.2998001310934,69.216222948839,12.));
#158236=CARTESIAN_POINT('Ctrl Pts',(-11.3018540025605,69.1965599718761,
0.));
#158237=CARTESIAN_POINT('Ctrl Pts',(-11.3018540025605,69.1965599718761,
12.));
#158238=CARTESIAN_POINT('Ctrl Pts',(-11.3038812726275,69.1769483991639,
0.));
#158239=CARTESIAN_POINT('Ctrl Pts',(-11.3038812726275,69.1769483991639,
12.));
#158240=CARTESIAN_POINT('Ctrl Pts',(-11.3058820128323,69.1573884361076,
0.));
#158241=CARTESIAN_POINT('Ctrl Pts',(-11.3058820128323,69.1573884361076,
12.));
#158242=CARTESIAN_POINT('Ctrl Pts',(-11.3078562764442,69.137880225198,0.));
#158243=CARTESIAN_POINT('Ctrl Pts',(-11.3078562764442,69.137880225198,12.));
#158244=CARTESIAN_POINT('Ctrl Pts',(-11.3098040973799,69.1184238445065,
0.));
#158245=CARTESIAN_POINT('Ctrl Pts',(-11.3098040973799,69.1184238445065,
12.));
#158246=CARTESIAN_POINT('Ctrl Pts',(-11.3113412156742,69.1029002322497,
0.));
#158247=CARTESIAN_POINT('Ctrl Pts',(-11.3113412156742,69.1029002322497,
12.));
#158248=CARTESIAN_POINT('Ctrl Pts',(-11.3124821678849,69.0912808657051,
0.));
#158249=CARTESIAN_POINT('Ctrl Pts',(-11.3124821678849,69.0912808657051,
12.));
#158250=CARTESIAN_POINT('Ctrl Pts',(-11.3132375200184,69.0835449954486,
0.));
#158251=CARTESIAN_POINT('Ctrl Pts',(-11.3132375200184,69.0835449954486,
12.));
#158252=CARTESIAN_POINT('Ctrl Pts',(-11.3136138754165,69.079679653846,0.));
#158253=CARTESIAN_POINT('Ctrl Pts',(-11.3136138754165,69.079679653846,12.));
#158254=CARTESIAN_POINT('',(-11.3136138754165,69.079679653846,12.));
#158255=CARTESIAN_POINT('Ctrl Pts',(-11.3136138754165,69.079679653846,12.));
#158256=CARTESIAN_POINT('Ctrl Pts',(-11.3132375200184,69.0835449954486,
12.));
#158257=CARTESIAN_POINT('Ctrl Pts',(-11.3124821678849,69.0912808657051,
12.));
#158258=CARTESIAN_POINT('Ctrl Pts',(-11.3113412156742,69.1029002322497,
12.));
#158259=CARTESIAN_POINT('Ctrl Pts',(-11.3098040973799,69.1184238445065,
12.));
#158260=CARTESIAN_POINT('Ctrl Pts',(-11.3078562764442,69.137880225198,12.));
#158261=CARTESIAN_POINT('Ctrl Pts',(-11.3058820128323,69.1573884361076,
12.));
#158262=CARTESIAN_POINT('Ctrl Pts',(-11.3038812726275,69.1769483991639,
12.));
#158263=CARTESIAN_POINT('Ctrl Pts',(-11.3018540025605,69.1965599718761,
12.));
#158264=CARTESIAN_POINT('Ctrl Pts',(-11.2998001310934,69.216222948839,12.));
#158265=CARTESIAN_POINT('Ctrl Pts',(-11.2977195764836,69.2359370894828,
12.));
#158266=CARTESIAN_POINT('Ctrl Pts',(-11.2956122531375,69.255702139335,12.));
#158267=CARTESIAN_POINT('Ctrl Pts',(-11.2934780784361,69.2755178531534,
12.));
#158268=CARTESIAN_POINT('Ctrl Pts',(-11.2913169799642,69.2953840192792,
12.));
#158269=CARTESIAN_POINT('Ctrl Pts',(-11.2891288931528,69.315300451784,12.));
#158270=CARTESIAN_POINT('Ctrl Pts',(-11.2869137578463,69.3352669789611,
12.));
#158271=CARTESIAN_POINT('Ctrl Pts',(-11.2846715154521,69.3552834337771,
12.));
#158272=CARTESIAN_POINT('Ctrl Pts',(-11.2824021054038,69.375349642,12.));
#158273=CARTESIAN_POINT('Ctrl Pts',(-11.2801054633807,69.395465416223,12.));
#158274=CARTESIAN_POINT('Ctrl Pts',(-11.2777815231462,69.4156305620554,
12.));
#158275=CARTESIAN_POINT('Ctrl Pts',(-11.2754302177019,69.4358448819957,
12.));
#158276=CARTESIAN_POINT('Ctrl Pts',(-11.2730514806143,69.4561081798815,
12.));
#158277=CARTESIAN_POINT('Ctrl Pts',(-11.2706452475287,69.4764202659443,
12.));
#158278=CARTESIAN_POINT('Ctrl Pts',(-11.2682114561015,69.4967809565978,
12.));
#158279=CARTESIAN_POINT('Ctrl Pts',(-11.2657500452721,69.5171900720188,
12.));
#158280=CARTESIAN_POINT('Ctrl Pts',(-11.2632609547629,69.5376474344768,
12.));
#158281=CARTESIAN_POINT('Ctrl Pts',(-11.2607441244698,69.5581528662846,
12.));
#158282=CARTESIAN_POINT('Ctrl Pts',(-11.2581994939534,69.5787061880815,
12.));
#158283=CARTESIAN_POINT('Ctrl Pts',(-11.255627002701,69.5993072197355,12.));
#158284=CARTESIAN_POINT('Ctrl Pts',(-11.2530265903555,69.6199557811231,
12.));
#158285=CARTESIAN_POINT('Ctrl Pts',(-11.2503981969413,69.6406516928902,
12.));
#158286=CARTESIAN_POINT('Ctrl Pts',(-11.2477417631391,69.6613947773563,
12.));
#158287=CARTESIAN_POINT('Ctrl Pts',(-11.2450572303847,69.6821848588492,
12.));
#158288=CARTESIAN_POINT('Ctrl Pts',(-11.242344540717,69.7030217632187,12.));
#158289=CARTESIAN_POINT('Ctrl Pts',(-11.2396036366861,69.7239053175362,
12.));
#158290=CARTESIAN_POINT('Ctrl Pts',(-11.236834461247,69.7448353497394,12.));
#158291=CARTESIAN_POINT('Ctrl Pts',(-11.2340369576452,69.7658116882298,
12.));
#158292=CARTESIAN_POINT('Ctrl Pts',(-11.2312110694183,69.7868341618927,
12.));
#158293=CARTESIAN_POINT('Ctrl Pts',(-11.2283567404434,69.8079026002753,
12.));
#158294=CARTESIAN_POINT('Ctrl Pts',(-11.225473914972,69.8290168337076,12.));
#158295=CARTESIAN_POINT('Ctrl Pts',(-11.2225625376739,69.8501766934445,
12.));
#158296=CARTESIAN_POINT('Ctrl Pts',(-11.2196225536794,69.8713820117918,
12.));
#158297=CARTESIAN_POINT('Ctrl Pts',(-11.2166539085527,69.8926326220414,
12.));
#158298=CARTESIAN_POINT('Ctrl Pts',(-11.2136565482679,69.9139283584036,
12.));
#158299=CARTESIAN_POINT('Ctrl Pts',(-11.2106304191881,69.9352690559399,
12.));
#158300=CARTESIAN_POINT('Ctrl Pts',(-11.2075754680445,69.9566545504813,
12.));
#158301=CARTESIAN_POINT('Ctrl Pts',(-11.2044916419239,69.9780846785771,
12.));
#158302=CARTESIAN_POINT('Ctrl Pts',(-11.2013788882711,69.9995592775322,
12.));
#158303=CARTESIAN_POINT('Ctrl Pts',(-11.1982371548918,70.0210781854236,
12.));
#158304=CARTESIAN_POINT('Ctrl Pts',(-11.1950663899578,70.0426412411194,
12.));
#158305=CARTESIAN_POINT('Ctrl Pts',(-11.1918665420168,70.0642482842942,
12.));
#158306=CARTESIAN_POINT('Ctrl Pts',(-11.1886375599916,70.0858991554295,
12.));
#158307=CARTESIAN_POINT('Ctrl Pts',(-11.185379393167,70.1075936957973,12.));
#158308=CARTESIAN_POINT('Ctrl Pts',(-11.1820919911846,70.1293317474432,
12.));
#158309=CARTESIAN_POINT('Ctrl Pts',(-11.1787753040363,70.1511131531672,
12.));
#158310=CARTESIAN_POINT('Ctrl Pts',(-11.1754292820631,70.1729377564954,
12.));
#158311=CARTESIAN_POINT('Ctrl Pts',(-11.1720538759499,70.1948054016816,
12.));
#158312=CARTESIAN_POINT('Ctrl Pts',(-11.168649036721,70.2167159337094,12.));
#158313=CARTESIAN_POINT('Ctrl Pts',(-11.1652147157383,70.2386691982902,
12.));
#158314=CARTESIAN_POINT('Ctrl Pts',(-11.1617508647016,70.2606650418589,
12.));
#158315=CARTESIAN_POINT('Ctrl Pts',(-11.1582574356521,70.2827033115662,
12.));
#158316=CARTESIAN_POINT('Ctrl Pts',(-11.1547343809646,70.3047838552756,
12.));
#158317=CARTESIAN_POINT('Ctrl Pts',(-11.1511816533421,70.326906521559,12.));
#158318=CARTESIAN_POINT('Ctrl Pts',(-11.1475992058124,70.349071159688,12.));
#158319=CARTESIAN_POINT('Ctrl Pts',(-11.143986991727,70.3712776196223,12.));
#158320=CARTESIAN_POINT('Ctrl Pts',(-11.1403449647625,70.393525751996,12.));
#158321=CARTESIAN_POINT('Ctrl Pts',(-11.1366730789126,70.4158154081205,
12.));
#158322=CARTESIAN_POINT('Ctrl Pts',(-11.1329712884846,70.4381464399819,
12.));
#158323=CARTESIAN_POINT('Ctrl Pts',(-11.1292395480974,70.4605187002354,
12.));
#158324=CARTESIAN_POINT('Ctrl Pts',(-11.1254778126821,70.4829320421957,
12.));
#158325=CARTESIAN_POINT('Ctrl Pts',(-11.1216860374826,70.505386319828,12.));
#158326=CARTESIAN_POINT('Ctrl Pts',(-11.1178641780476,70.5278813877494,
12.));
#158327=CARTESIAN_POINT('Ctrl Pts',(-11.1140121902271,70.5504171012233,
12.));
#158328=CARTESIAN_POINT('Ctrl Pts',(-11.1101300301701,70.5729933161546,
12.));
#158329=CARTESIAN_POINT('Ctrl Pts',(-11.1062176543262,70.5956098890773,
12.));
#158330=CARTESIAN_POINT('Ctrl Pts',(-11.1022750194446,70.6182666771481,
12.));
#158331=CARTESIAN_POINT('Ctrl Pts',(-11.0983020825667,70.6409635381482,
12.));
#158332=CARTESIAN_POINT('Ctrl Pts',(-11.0942988010233,70.6637003304785,
12.));
#158333=CARTESIAN_POINT('Ctrl Pts',(-11.0902651324323,70.6864769131546,
12.));
#158334=CARTESIAN_POINT('Ctrl Pts',(-11.0862010347016,70.7092931457954,
12.));
#158335=CARTESIAN_POINT('Ctrl Pts',(-11.0821064660269,70.732148888618,12.));
#158336=CARTESIAN_POINT('Ctrl Pts',(-11.0779813848846,70.7550440024384,
12.));
#158337=CARTESIAN_POINT('Ctrl Pts',(-11.073825750029,70.7779783486677,12.));
#158338=CARTESIAN_POINT('Ctrl Pts',(-11.0696395204909,70.8009517893057,
12.));
#158339=CARTESIAN_POINT('Ctrl Pts',(-11.0654226555802,70.8239641869299,
12.));
#158340=CARTESIAN_POINT('Ctrl Pts',(-11.0611751148835,70.8470154046919,
12.));
#158341=CARTESIAN_POINT('Ctrl Pts',(-11.0568968582569,70.8701053063186,
12.));
#158342=CARTESIAN_POINT('Ctrl Pts',(-11.0525878458243,70.8932337561087,
12.));
#158343=CARTESIAN_POINT('Ctrl Pts',(-11.048248037975,70.916400618927,12.));
#158344=CARTESIAN_POINT('Ctrl Pts',(-11.0438773953681,70.9396057601924,
12.));
#158345=CARTESIAN_POINT('Ctrl Pts',(-11.0394758789285,70.9628490458748,
12.));
#158346=CARTESIAN_POINT('Ctrl Pts',(-11.0350434498405,70.986130342497,12.));
#158347=CARTESIAN_POINT('Ctrl Pts',(-11.0305800695456,71.0094495171292,
12.));
#158348=CARTESIAN_POINT('Ctrl Pts',(-11.0260856997415,71.0328064373856,
12.));
#158349=CARTESIAN_POINT('Ctrl Pts',(-11.0215603023856,71.0562009714136,
12.));
#158350=CARTESIAN_POINT('Ctrl Pts',(-11.0170038396915,71.0796329878907,
12.));
#158351=CARTESIAN_POINT('Ctrl Pts',(-11.0124162741224,71.1031023560249,
12.));
#158352=CARTESIAN_POINT('Ctrl Pts',(-11.0077975683895,71.1266089455517,
12.));
#158353=CARTESIAN_POINT('Ctrl Pts',(-11.0031476854502,71.1501526267286,
12.));
#158354=CARTESIAN_POINT('Ctrl Pts',(-10.9984665885127,71.1737332703248,
12.));
#158355=CARTESIAN_POINT('Ctrl Pts',(-10.993754241032,71.1973507476191,12.));
#158356=CARTESIAN_POINT('Ctrl Pts',(-10.9890106067039,71.2210049304014,
12.));
#158357=CARTESIAN_POINT('Ctrl Pts',(-10.9842356494627,71.2446956909687,
12.));
#158358=CARTESIAN_POINT('Ctrl Pts',(-10.9794293334805,71.2684229021207,
12.));
#158359=CARTESIAN_POINT('Ctrl Pts',(-10.9745916231709,71.2921864371491,
12.));
#158360=CARTESIAN_POINT('Ctrl Pts',(-10.969722483186,71.3159861698358,12.));
#158361=CARTESIAN_POINT('Ctrl Pts',(-10.9648218784098,71.339821974454,12.));
#158362=CARTESIAN_POINT('Ctrl Pts',(-10.9598897739564,71.3636937257649,
12.));
#158363=CARTESIAN_POINT('Ctrl Pts',(-10.954926135169,71.3876012990138,12.));
#158364=CARTESIAN_POINT('Ctrl Pts',(-10.9499309276236,71.4115445699194,
12.));
#158365=CARTESIAN_POINT('Ctrl Pts',(-10.944904117127,71.435523414672,12.));
#158366=CARTESIAN_POINT('Ctrl Pts',(-10.9398456697095,71.4595377099351,
12.));
#158367=CARTESIAN_POINT('Ctrl Pts',(-10.9347555516235,71.4835873328423,
12.));
#158368=CARTESIAN_POINT('Ctrl Pts',(-10.9296337293424,71.5076721609937,
12.));
#158369=CARTESIAN_POINT('Ctrl Pts',(-10.9244801695642,71.5317920724459,
12.));
#158370=CARTESIAN_POINT('Ctrl Pts',(-10.91929483921,71.5559469457091,12.));
#158371=CARTESIAN_POINT('Ctrl Pts',(-10.914077705417,71.5801366597488,12.));
#158372=CARTESIAN_POINT('Ctrl Pts',(-10.9088287355365,71.6043610939835,
12.));
#158373=CARTESIAN_POINT('Ctrl Pts',(-10.9035478971328,71.6286201282812,
12.));
#158374=CARTESIAN_POINT('Ctrl Pts',(-10.8982351579871,71.6529136429504,
12.));
#158375=CARTESIAN_POINT('Ctrl Pts',(-10.8928904860964,71.6772415187364,
12.));
#158376=CARTESIAN_POINT('Ctrl Pts',(-10.8875138496671,71.7016036368236,
12.));
#158377=CARTESIAN_POINT('Ctrl Pts',(-10.8821052171121,71.7259998788328,
12.));
#158378=CARTESIAN_POINT('Ctrl Pts',(-10.8766645570497,71.7504301268181,
12.));
#158379=CARTESIAN_POINT('Ctrl Pts',(-10.8711918383073,71.7748942632593,
12.));
#158380=CARTESIAN_POINT('Ctrl Pts',(-10.865687029922,71.7993921710564,12.));
#158381=CARTESIAN_POINT('Ctrl Pts',(-10.8601501011332,71.8239237335331,
12.));
#158382=CARTESIAN_POINT('Ctrl Pts',(-10.8545810213799,71.8484888344339,
12.));
#158383=CARTESIAN_POINT('Ctrl Pts',(-10.8489797602997,71.8730873579224,
12.));
#158384=CARTESIAN_POINT('Ctrl Pts',(-10.8433462877311,71.8977191885725,
12.));
#158385=CARTESIAN_POINT('Ctrl Pts',(-10.8376805737159,71.9223842113625,
12.));
#158386=CARTESIAN_POINT('Ctrl Pts',(-10.8319825884918,71.9470823116785,
12.));
#158387=CARTESIAN_POINT('Ctrl Pts',(-10.8262523024898,71.9718133753127,
12.));
#158388=CARTESIAN_POINT('Ctrl Pts',(-10.8204896863328,71.9965772884619,
12.));
#158389=CARTESIAN_POINT('Ctrl Pts',(-10.8146947108375,72.0213739377223,
12.));
#158390=CARTESIAN_POINT('Ctrl Pts',(-10.8088673470184,72.0462032100815,
12.));
#158391=CARTESIAN_POINT('Ctrl Pts',(-10.8030075660808,72.0710649929202,
12.));
#158392=CARTESIAN_POINT('Ctrl Pts',(-10.7971153394166,72.0959591740114,
12.));
#158393=CARTESIAN_POINT('Ctrl Pts',(-10.7911906386027,72.1208856415171,
12.));
#158394=CARTESIAN_POINT('Ctrl Pts',(-10.7852334354016,72.1458442839834,
12.));
#158395=CARTESIAN_POINT('Ctrl Pts',(-10.7792437017662,72.1708349903305,
12.));
#158396=CARTESIAN_POINT('Ctrl Pts',(-10.7732214098344,72.1958576498558,
12.));
#158397=CARTESIAN_POINT('Ctrl Pts',(-10.7671665319255,72.2209121522366,
12.));
#158398=CARTESIAN_POINT('Ctrl Pts',(-10.7610790405385,72.2459983875296,
12.));
#158399=CARTESIAN_POINT('Ctrl Pts',(-10.7549589083535,72.2711162461681,
12.));
#158400=CARTESIAN_POINT('Ctrl Pts',(-10.7488061082368,72.2962656189556,
12.));
#158401=CARTESIAN_POINT('Ctrl Pts',(-10.7426206132375,72.3214463970641,
12.));
#158402=CARTESIAN_POINT('Ctrl Pts',(-10.73640239658,72.3466584720318,12.));
#158403=CARTESIAN_POINT('Ctrl Pts',(-10.7301514316607,72.3719017357571,
12.));
#158404=CARTESIAN_POINT('Ctrl Pts',(-10.7238676920469,72.3971760804933,
12.));
#158405=CARTESIAN_POINT('Ctrl Pts',(-10.7175511514788,72.4224813988347,
12.));
#158406=CARTESIAN_POINT('Ctrl Pts',(-10.7112017838706,72.4478175837156,
12.));
#158407=CARTESIAN_POINT('Ctrl Pts',(-10.7048195633061,72.4731845284227,
12.));
#158408=CARTESIAN_POINT('Ctrl Pts',(-10.6984044640398,72.4985821266023,
12.));
#158409=CARTESIAN_POINT('Ctrl Pts',(-10.691956460499,72.5240102722664,12.));
#158410=CARTESIAN_POINT('Ctrl Pts',(-10.6854755272904,72.5494688597961,
12.));
#158411=CARTESIAN_POINT('Ctrl Pts',(-10.6789616392042,72.5749577839415,
12.));
#158412=CARTESIAN_POINT('Ctrl Pts',(-10.6724147711995,72.6004769398019,
12.));
#158413=CARTESIAN_POINT('Ctrl Pts',(-10.6658348983944,72.6260262228065,
12.));
#158414=CARTESIAN_POINT('Ctrl Pts',(-10.659221996058,72.651605528691,12.));
#158415=CARTESIAN_POINT('Ctrl Pts',(-10.6525760396054,72.6772147534752,
12.));
#158416=CARTESIAN_POINT('Ctrl Pts',(-10.6458970045946,72.7028537934317,
12.));
#158417=CARTESIAN_POINT('Ctrl Pts',(-10.6391848667352,72.7285225451293,
12.));
#158418=CARTESIAN_POINT('Ctrl Pts',(-10.6324396018998,72.7542209054812,
12.));
#158419=CARTESIAN_POINT('Ctrl Pts',(-10.6256611861394,72.7799487717911,
12.));
#158420=CARTESIAN_POINT('Ctrl Pts',(-10.6188495956973,72.8057060417887,
12.));
#158421=CARTESIAN_POINT('Ctrl Pts',(-10.6120048070367,72.8314926136881,
12.));
#158422=CARTESIAN_POINT('Ctrl Pts',(-10.6051267968203,72.8573083861337,
12.));
#158423=CARTESIAN_POINT('Ctrl Pts',(-10.5982155418626,72.8831532580845,
12.));
#158424=CARTESIAN_POINT('Ctrl Pts',(-10.5912710190928,72.9090271287083,
12.));
#158425=CARTESIAN_POINT('Ctrl Pts',(-10.5842932055209,72.9349298972822,
12.));
#158426=CARTESIAN_POINT('Ctrl Pts',(-10.5772820781958,72.9608614630534,
12.));
#158427=CARTESIAN_POINT('Ctrl Pts',(-10.570237614205,72.9868217252283,12.));
#158428=CARTESIAN_POINT('Ctrl Pts',(-10.5631597907651,73.0128105832621,
12.));
#158429=CARTESIAN_POINT('Ctrl Pts',(-10.5560485852974,73.0388279370834,
12.));
#158430=CARTESIAN_POINT('Ctrl Pts',(-10.5489039755138,73.0648736873434,
12.));
#158431=CARTESIAN_POINT('Ctrl Pts',(-10.5417259395003,73.0909477356474,
12.));
#158432=CARTESIAN_POINT('Ctrl Pts',(-10.53451445581,73.1170499848039,12.));
#158433=CARTESIAN_POINT('Ctrl Pts',(-10.5272695032653,73.1431803382711,
12.));
#158434=CARTESIAN_POINT('Ctrl Pts',(-10.5199910607654,73.1693386996138,
12.));
#158435=CARTESIAN_POINT('Ctrl Pts',(-10.5126791070805,73.1955249719048,
12.));
#158436=CARTESIAN_POINT('Ctrl Pts',(-10.5053336206908,73.2217390572562,
12.));
#158437=CARTESIAN_POINT('Ctrl Pts',(-10.4979545795192,73.2479808560189,
12.));
#158438=CARTESIAN_POINT('Ctrl Pts',(-10.4905419611523,73.2742502674304,
12.));
#158439=CARTESIAN_POINT('Ctrl Pts',(-10.4830957433305,73.3005471910583,
12.));
#158440=CARTESIAN_POINT('Ctrl Pts',(-10.4756159043806,73.3268715280575,
12.));
#158441=CARTESIAN_POINT('Ctrl Pts',(-10.4681024236289,73.3532231823659,
12.));
#158442=CARTESIAN_POINT('Ctrl Pts',(-10.4605552819397,73.37960206225,12.));
#158443=CARTESIAN_POINT('Ctrl Pts',(-10.452974461845,73.4060080806686,12.));
#158444=CARTESIAN_POINT('Ctrl Pts',(-10.4464473465479,73.4286663448107,
12.));
#158445=CARTESIAN_POINT('Ctrl Pts',(-10.4414249334739,73.44605255288,12.));
#158446=CARTESIAN_POINT('Ctrl Pts',(-10.4379221501041,73.4581547436838,
12.));
#158447=CARTESIAN_POINT('Ctrl Pts',(-10.4359488742809,73.4649650361894,
12.));
#158448=CARTESIAN_POINT('Ctrl Pts',(-10.4355099267296,73.4664795929939,
12.));
#158449=CARTESIAN_POINT('',(-11.3136138754165,69.079679653846,0.));
#158450=CARTESIAN_POINT('',(-11.3136138754165,69.079679653846,0.));
#158451=CARTESIAN_POINT('Ctrl Pts',(-10.4355099267296,73.4664795929939,
0.));
#158452=CARTESIAN_POINT('Ctrl Pts',(-10.4359488742809,73.4649650361894,
0.));
#158453=CARTESIAN_POINT('Ctrl Pts',(-10.4379221501041,73.4581547436838,
0.));
#158454=CARTESIAN_POINT('Ctrl Pts',(-10.4414249334739,73.44605255288,0.));
#158455=CARTESIAN_POINT('Ctrl Pts',(-10.4464473465479,73.4286663448107,
0.));
#158456=CARTESIAN_POINT('Ctrl Pts',(-10.452974461845,73.4060080806686,0.));
#158457=CARTESIAN_POINT('Ctrl Pts',(-10.4605552819397,73.37960206225,0.));
#158458=CARTESIAN_POINT('Ctrl Pts',(-10.4681024236289,73.3532231823659,
0.));
#158459=CARTESIAN_POINT('Ctrl Pts',(-10.4756159043806,73.3268715280575,
0.));
#158460=CARTESIAN_POINT('Ctrl Pts',(-10.4830957433305,73.3005471910583,
0.));
#158461=CARTESIAN_POINT('Ctrl Pts',(-10.4905419611523,73.2742502674304,
0.));
#158462=CARTESIAN_POINT('Ctrl Pts',(-10.4979545795192,73.2479808560189,
0.));
#158463=CARTESIAN_POINT('Ctrl Pts',(-10.5053336206908,73.2217390572562,
0.));
#158464=CARTESIAN_POINT('Ctrl Pts',(-10.5126791070805,73.1955249719048,
0.));
#158465=CARTESIAN_POINT('Ctrl Pts',(-10.5199910607654,73.1693386996138,
0.));
#158466=CARTESIAN_POINT('Ctrl Pts',(-10.5272695032653,73.1431803382711,
0.));
#158467=CARTESIAN_POINT('Ctrl Pts',(-10.53451445581,73.1170499848039,0.));
#158468=CARTESIAN_POINT('Ctrl Pts',(-10.5417259395003,73.0909477356474,
0.));
#158469=CARTESIAN_POINT('Ctrl Pts',(-10.5489039755138,73.0648736873434,
0.));
#158470=CARTESIAN_POINT('Ctrl Pts',(-10.5560485852974,73.0388279370834,
0.));
#158471=CARTESIAN_POINT('Ctrl Pts',(-10.5631597907651,73.0128105832621,
0.));
#158472=CARTESIAN_POINT('Ctrl Pts',(-10.570237614205,72.9868217252283,0.));
#158473=CARTESIAN_POINT('Ctrl Pts',(-10.5772820781958,72.9608614630534,
0.));
#158474=CARTESIAN_POINT('Ctrl Pts',(-10.5842932055209,72.9349298972822,
0.));
#158475=CARTESIAN_POINT('Ctrl Pts',(-10.5912710190928,72.9090271287083,
0.));
#158476=CARTESIAN_POINT('Ctrl Pts',(-10.5982155418626,72.8831532580845,
0.));
#158477=CARTESIAN_POINT('Ctrl Pts',(-10.6051267968203,72.8573083861337,
0.));
#158478=CARTESIAN_POINT('Ctrl Pts',(-10.6120048070367,72.8314926136881,
0.));
#158479=CARTESIAN_POINT('Ctrl Pts',(-10.6188495956973,72.8057060417887,
0.));
#158480=CARTESIAN_POINT('Ctrl Pts',(-10.6256611861394,72.7799487717911,
0.));
#158481=CARTESIAN_POINT('Ctrl Pts',(-10.6324396018998,72.7542209054812,
0.));
#158482=CARTESIAN_POINT('Ctrl Pts',(-10.6391848667352,72.7285225451293,
0.));
#158483=CARTESIAN_POINT('Ctrl Pts',(-10.6458970045946,72.7028537934317,
0.));
#158484=CARTESIAN_POINT('Ctrl Pts',(-10.6525760396054,72.6772147534752,
0.));
#158485=CARTESIAN_POINT('Ctrl Pts',(-10.659221996058,72.651605528691,0.));
#158486=CARTESIAN_POINT('Ctrl Pts',(-10.6658348983944,72.6260262228065,
0.));
#158487=CARTESIAN_POINT('Ctrl Pts',(-10.6724147711995,72.6004769398019,
0.));
#158488=CARTESIAN_POINT('Ctrl Pts',(-10.6789616392042,72.5749577839415,
0.));
#158489=CARTESIAN_POINT('Ctrl Pts',(-10.6854755272904,72.5494688597961,
0.));
#158490=CARTESIAN_POINT('Ctrl Pts',(-10.691956460499,72.5240102722664,0.));
#158491=CARTESIAN_POINT('Ctrl Pts',(-10.6984044640398,72.4985821266023,
0.));
#158492=CARTESIAN_POINT('Ctrl Pts',(-10.7048195633061,72.4731845284227,
0.));
#158493=CARTESIAN_POINT('Ctrl Pts',(-10.7112017838706,72.4478175837156,
0.));
#158494=CARTESIAN_POINT('Ctrl Pts',(-10.7175511514788,72.4224813988347,
0.));
#158495=CARTESIAN_POINT('Ctrl Pts',(-10.7238676920469,72.3971760804933,
0.));
#158496=CARTESIAN_POINT('Ctrl Pts',(-10.7301514316607,72.3719017357571,
0.));
#158497=CARTESIAN_POINT('Ctrl Pts',(-10.73640239658,72.3466584720318,0.));
#158498=CARTESIAN_POINT('Ctrl Pts',(-10.7426206132375,72.3214463970641,
0.));
#158499=CARTESIAN_POINT('Ctrl Pts',(-10.7488061082368,72.2962656189556,
0.));
#158500=CARTESIAN_POINT('Ctrl Pts',(-10.7549589083535,72.2711162461681,
0.));
#158501=CARTESIAN_POINT('Ctrl Pts',(-10.7610790405385,72.2459983875296,
0.));
#158502=CARTESIAN_POINT('Ctrl Pts',(-10.7671665319255,72.2209121522366,
0.));
#158503=CARTESIAN_POINT('Ctrl Pts',(-10.7732214098344,72.1958576498558,
0.));
#158504=CARTESIAN_POINT('Ctrl Pts',(-10.7792437017662,72.1708349903305,
0.));
#158505=CARTESIAN_POINT('Ctrl Pts',(-10.7852334354016,72.1458442839834,
0.));
#158506=CARTESIAN_POINT('Ctrl Pts',(-10.7911906386027,72.1208856415171,
0.));
#158507=CARTESIAN_POINT('Ctrl Pts',(-10.7971153394166,72.0959591740114,
0.));
#158508=CARTESIAN_POINT('Ctrl Pts',(-10.8030075660808,72.0710649929202,
0.));
#158509=CARTESIAN_POINT('Ctrl Pts',(-10.8088673470184,72.0462032100815,
0.));
#158510=CARTESIAN_POINT('Ctrl Pts',(-10.8146947108375,72.0213739377223,
0.));
#158511=CARTESIAN_POINT('Ctrl Pts',(-10.8204896863328,71.9965772884619,
0.));
#158512=CARTESIAN_POINT('Ctrl Pts',(-10.8262523024898,71.9718133753127,
0.));
#158513=CARTESIAN_POINT('Ctrl Pts',(-10.8319825884918,71.9470823116785,
0.));
#158514=CARTESIAN_POINT('Ctrl Pts',(-10.8376805737159,71.9223842113625,
0.));
#158515=CARTESIAN_POINT('Ctrl Pts',(-10.8433462877311,71.8977191885725,
0.));
#158516=CARTESIAN_POINT('Ctrl Pts',(-10.8489797602997,71.8730873579224,
0.));
#158517=CARTESIAN_POINT('Ctrl Pts',(-10.8545810213799,71.8484888344339,
0.));
#158518=CARTESIAN_POINT('Ctrl Pts',(-10.8601501011332,71.8239237335331,
0.));
#158519=CARTESIAN_POINT('Ctrl Pts',(-10.865687029922,71.7993921710564,0.));
#158520=CARTESIAN_POINT('Ctrl Pts',(-10.8711918383073,71.7748942632593,
0.));
#158521=CARTESIAN_POINT('Ctrl Pts',(-10.8766645570497,71.7504301268181,
0.));
#158522=CARTESIAN_POINT('Ctrl Pts',(-10.8821052171121,71.7259998788328,
0.));
#158523=CARTESIAN_POINT('Ctrl Pts',(-10.8875138496671,71.7016036368236,
0.));
#158524=CARTESIAN_POINT('Ctrl Pts',(-10.8928904860964,71.6772415187364,
0.));
#158525=CARTESIAN_POINT('Ctrl Pts',(-10.8982351579871,71.6529136429504,
0.));
#158526=CARTESIAN_POINT('Ctrl Pts',(-10.9035478971328,71.6286201282812,
0.));
#158527=CARTESIAN_POINT('Ctrl Pts',(-10.9088287355365,71.6043610939835,
0.));
#158528=CARTESIAN_POINT('Ctrl Pts',(-10.914077705417,71.5801366597488,0.));
#158529=CARTESIAN_POINT('Ctrl Pts',(-10.91929483921,71.5559469457091,0.));
#158530=CARTESIAN_POINT('Ctrl Pts',(-10.9244801695642,71.5317920724459,
0.));
#158531=CARTESIAN_POINT('Ctrl Pts',(-10.9296337293424,71.5076721609937,
0.));
#158532=CARTESIAN_POINT('Ctrl Pts',(-10.9347555516235,71.4835873328423,
0.));
#158533=CARTESIAN_POINT('Ctrl Pts',(-10.9398456697095,71.4595377099351,
0.));
#158534=CARTESIAN_POINT('Ctrl Pts',(-10.944904117127,71.435523414672,0.));
#158535=CARTESIAN_POINT('Ctrl Pts',(-10.9499309276236,71.4115445699194,
0.));
#158536=CARTESIAN_POINT('Ctrl Pts',(-10.954926135169,71.3876012990138,0.));
#158537=CARTESIAN_POINT('Ctrl Pts',(-10.9598897739564,71.3636937257649,
0.));
#158538=CARTESIAN_POINT('Ctrl Pts',(-10.9648218784098,71.339821974454,0.));
#158539=CARTESIAN_POINT('Ctrl Pts',(-10.969722483186,71.3159861698358,0.));
#158540=CARTESIAN_POINT('Ctrl Pts',(-10.9745916231709,71.2921864371491,
0.));
#158541=CARTESIAN_POINT('Ctrl Pts',(-10.9794293334805,71.2684229021207,
0.));
#158542=CARTESIAN_POINT('Ctrl Pts',(-10.9842356494627,71.2446956909687,
0.));
#158543=CARTESIAN_POINT('Ctrl Pts',(-10.9890106067039,71.2210049304014,
0.));
#158544=CARTESIAN_POINT('Ctrl Pts',(-10.993754241032,71.1973507476191,0.));
#158545=CARTESIAN_POINT('Ctrl Pts',(-10.9984665885127,71.1737332703248,
0.));
#158546=CARTESIAN_POINT('Ctrl Pts',(-11.0031476854502,71.1501526267286,
0.));
#158547=CARTESIAN_POINT('Ctrl Pts',(-11.0077975683895,71.1266089455517,
0.));
#158548=CARTESIAN_POINT('Ctrl Pts',(-11.0124162741224,71.1031023560249,
0.));
#158549=CARTESIAN_POINT('Ctrl Pts',(-11.0170038396915,71.0796329878907,
0.));
#158550=CARTESIAN_POINT('Ctrl Pts',(-11.0215603023856,71.0562009714136,
0.));
#158551=CARTESIAN_POINT('Ctrl Pts',(-11.0260856997415,71.0328064373856,
0.));
#158552=CARTESIAN_POINT('Ctrl Pts',(-11.0305800695456,71.0094495171292,
0.));
#158553=CARTESIAN_POINT('Ctrl Pts',(-11.0350434498405,70.986130342497,0.));
#158554=CARTESIAN_POINT('Ctrl Pts',(-11.0394758789285,70.9628490458748,
0.));
#158555=CARTESIAN_POINT('Ctrl Pts',(-11.0438773953681,70.9396057601924,
0.));
#158556=CARTESIAN_POINT('Ctrl Pts',(-11.048248037975,70.916400618927,0.));
#158557=CARTESIAN_POINT('Ctrl Pts',(-11.0525878458243,70.8932337561087,
0.));
#158558=CARTESIAN_POINT('Ctrl Pts',(-11.0568968582569,70.8701053063186,
0.));
#158559=CARTESIAN_POINT('Ctrl Pts',(-11.0611751148835,70.8470154046919,
0.));
#158560=CARTESIAN_POINT('Ctrl Pts',(-11.0654226555802,70.8239641869299,
0.));
#158561=CARTESIAN_POINT('Ctrl Pts',(-11.0696395204909,70.8009517893057,
0.));
#158562=CARTESIAN_POINT('Ctrl Pts',(-11.073825750029,70.7779783486677,0.));
#158563=CARTESIAN_POINT('Ctrl Pts',(-11.0779813848846,70.7550440024384,
0.));
#158564=CARTESIAN_POINT('Ctrl Pts',(-11.0821064660269,70.732148888618,0.));
#158565=CARTESIAN_POINT('Ctrl Pts',(-11.0862010347016,70.7092931457954,
0.));
#158566=CARTESIAN_POINT('Ctrl Pts',(-11.0902651324323,70.6864769131546,
0.));
#158567=CARTESIAN_POINT('Ctrl Pts',(-11.0942988010233,70.6637003304785,
0.));
#158568=CARTESIAN_POINT('Ctrl Pts',(-11.0983020825667,70.6409635381482,
0.));
#158569=CARTESIAN_POINT('Ctrl Pts',(-11.1022750194446,70.6182666771481,
0.));
#158570=CARTESIAN_POINT('Ctrl Pts',(-11.1062176543262,70.5956098890773,
0.));
#158571=CARTESIAN_POINT('Ctrl Pts',(-11.1101300301701,70.5729933161546,
0.));
#158572=CARTESIAN_POINT('Ctrl Pts',(-11.1140121902271,70.5504171012233,
0.));
#158573=CARTESIAN_POINT('Ctrl Pts',(-11.1178641780476,70.5278813877494,
0.));
#158574=CARTESIAN_POINT('Ctrl Pts',(-11.1216860374826,70.505386319828,0.));
#158575=CARTESIAN_POINT('Ctrl Pts',(-11.1254778126821,70.4829320421957,
0.));
#158576=CARTESIAN_POINT('Ctrl Pts',(-11.1292395480974,70.4605187002354,
0.));
#158577=CARTESIAN_POINT('Ctrl Pts',(-11.1329712884846,70.4381464399819,
0.));
#158578=CARTESIAN_POINT('Ctrl Pts',(-11.1366730789126,70.4158154081205,
0.));
#158579=CARTESIAN_POINT('Ctrl Pts',(-11.1403449647625,70.393525751996,0.));
#158580=CARTESIAN_POINT('Ctrl Pts',(-11.143986991727,70.3712776196223,0.));
#158581=CARTESIAN_POINT('Ctrl Pts',(-11.1475992058124,70.349071159688,0.));
#158582=CARTESIAN_POINT('Ctrl Pts',(-11.1511816533421,70.326906521559,0.));
#158583=CARTESIAN_POINT('Ctrl Pts',(-11.1547343809646,70.3047838552756,
0.));
#158584=CARTESIAN_POINT('Ctrl Pts',(-11.1582574356521,70.2827033115662,
0.));
#158585=CARTESIAN_POINT('Ctrl Pts',(-11.1617508647016,70.2606650418589,
0.));
#158586=CARTESIAN_POINT('Ctrl Pts',(-11.1652147157383,70.2386691982902,
0.));
#158587=CARTESIAN_POINT('Ctrl Pts',(-11.168649036721,70.2167159337094,0.));
#158588=CARTESIAN_POINT('Ctrl Pts',(-11.1720538759499,70.1948054016816,
0.));
#158589=CARTESIAN_POINT('Ctrl Pts',(-11.1754292820631,70.1729377564954,
0.));
#158590=CARTESIAN_POINT('Ctrl Pts',(-11.1787753040363,70.1511131531672,
0.));
#158591=CARTESIAN_POINT('Ctrl Pts',(-11.1820919911846,70.1293317474432,
0.));
#158592=CARTESIAN_POINT('Ctrl Pts',(-11.185379393167,70.1075936957973,0.));
#158593=CARTESIAN_POINT('Ctrl Pts',(-11.1886375599916,70.0858991554295,
0.));
#158594=CARTESIAN_POINT('Ctrl Pts',(-11.1918665420168,70.0642482842942,
0.));
#158595=CARTESIAN_POINT('Ctrl Pts',(-11.1950663899578,70.0426412411194,
0.));
#158596=CARTESIAN_POINT('Ctrl Pts',(-11.1982371548918,70.0210781854236,
0.));
#158597=CARTESIAN_POINT('Ctrl Pts',(-11.2013788882711,69.9995592775322,
0.));
#158598=CARTESIAN_POINT('Ctrl Pts',(-11.2044916419239,69.9780846785771,
0.));
#158599=CARTESIAN_POINT('Ctrl Pts',(-11.2075754680445,69.9566545504813,
0.));
#158600=CARTESIAN_POINT('Ctrl Pts',(-11.2106304191881,69.9352690559399,
0.));
#158601=CARTESIAN_POINT('Ctrl Pts',(-11.2136565482679,69.9139283584036,
0.));
#158602=CARTESIAN_POINT('Ctrl Pts',(-11.2166539085527,69.8926326220414,
0.));
#158603=CARTESIAN_POINT('Ctrl Pts',(-11.2196225536794,69.8713820117918,
0.));
#158604=CARTESIAN_POINT('Ctrl Pts',(-11.2225625376739,69.8501766934445,
0.));
#158605=CARTESIAN_POINT('Ctrl Pts',(-11.225473914972,69.8290168337076,0.));
#158606=CARTESIAN_POINT('Ctrl Pts',(-11.2283567404434,69.8079026002753,
0.));
#158607=CARTESIAN_POINT('Ctrl Pts',(-11.2312110694183,69.7868341618927,
0.));
#158608=CARTESIAN_POINT('Ctrl Pts',(-11.2340369576452,69.7658116882298,
0.));
#158609=CARTESIAN_POINT('Ctrl Pts',(-11.236834461247,69.7448353497394,0.));
#158610=CARTESIAN_POINT('Ctrl Pts',(-11.2396036366861,69.7239053175362,
0.));
#158611=CARTESIAN_POINT('Ctrl Pts',(-11.242344540717,69.7030217632187,0.));
#158612=CARTESIAN_POINT('Ctrl Pts',(-11.2450572303847,69.6821848588492,
0.));
#158613=CARTESIAN_POINT('Ctrl Pts',(-11.2477417631391,69.6613947773563,
0.));
#158614=CARTESIAN_POINT('Ctrl Pts',(-11.2503981969413,69.6406516928902,
0.));
#158615=CARTESIAN_POINT('Ctrl Pts',(-11.2530265903555,69.6199557811231,
0.));
#158616=CARTESIAN_POINT('Ctrl Pts',(-11.255627002701,69.5993072197355,0.));
#158617=CARTESIAN_POINT('Ctrl Pts',(-11.2581994939534,69.5787061880815,
0.));
#158618=CARTESIAN_POINT('Ctrl Pts',(-11.2607441244698,69.5581528662846,
0.));
#158619=CARTESIAN_POINT('Ctrl Pts',(-11.2632609547629,69.5376474344768,
0.));
#158620=CARTESIAN_POINT('Ctrl Pts',(-11.2657500452721,69.5171900720188,
0.));
#158621=CARTESIAN_POINT('Ctrl Pts',(-11.2682114561015,69.4967809565978,
0.));
#158622=CARTESIAN_POINT('Ctrl Pts',(-11.2706452475287,69.4764202659443,
0.));
#158623=CARTESIAN_POINT('Ctrl Pts',(-11.2730514806143,69.4561081798815,
0.));
#158624=CARTESIAN_POINT('Ctrl Pts',(-11.2754302177019,69.4358448819957,
0.));
#158625=CARTESIAN_POINT('Ctrl Pts',(-11.2777815231462,69.4156305620554,
0.));
#158626=CARTESIAN_POINT('Ctrl Pts',(-11.2801054633807,69.395465416223,0.));
#158627=CARTESIAN_POINT('Ctrl Pts',(-11.2824021054038,69.375349642,0.));
#158628=CARTESIAN_POINT('Ctrl Pts',(-11.2846715154521,69.3552834337771,
0.));
#158629=CARTESIAN_POINT('Ctrl Pts',(-11.2869137578463,69.3352669789611,
0.));
#158630=CARTESIAN_POINT('Ctrl Pts',(-11.2891288931528,69.315300451784,0.));
#158631=CARTESIAN_POINT('Ctrl Pts',(-11.2913169799642,69.2953840192792,
0.));
#158632=CARTESIAN_POINT('Ctrl Pts',(-11.2934780784361,69.2755178531534,
0.));
#158633=CARTESIAN_POINT('Ctrl Pts',(-11.2956122531375,69.255702139335,0.));
#158634=CARTESIAN_POINT('Ctrl Pts',(-11.2977195764836,69.2359370894828,
0.));
#158635=CARTESIAN_POINT('Ctrl Pts',(-11.2998001310934,69.216222948839,0.));
#158636=CARTESIAN_POINT('Ctrl Pts',(-11.3018540025605,69.1965599718761,
0.));
#158637=CARTESIAN_POINT('Ctrl Pts',(-11.3038812726275,69.1769483991639,
0.));
#158638=CARTESIAN_POINT('Ctrl Pts',(-11.3058820128323,69.1573884361076,
0.));
#158639=CARTESIAN_POINT('Ctrl Pts',(-11.3078562764442,69.137880225198,0.));
#158640=CARTESIAN_POINT('Ctrl Pts',(-11.3098040973799,69.1184238445065,
0.));
#158641=CARTESIAN_POINT('Ctrl Pts',(-11.3113412156742,69.1029002322497,
0.));
#158642=CARTESIAN_POINT('Ctrl Pts',(-11.3124821678849,69.0912808657051,
0.));
#158643=CARTESIAN_POINT('Ctrl Pts',(-11.3132375200184,69.0835449954486,
0.));
#158644=CARTESIAN_POINT('Ctrl Pts',(-11.3136138754165,69.079679653846,0.));
#158645=CARTESIAN_POINT('Ctrl Pts',(-3.87370827955544,74.3992230078037,
0.));
#158646=CARTESIAN_POINT('Ctrl Pts',(-3.87370827955544,74.3992230078037,
12.));
#158647=CARTESIAN_POINT('Ctrl Pts',(-3.87578335377325,74.3940262116388,
0.));
#158648=CARTESIAN_POINT('Ctrl Pts',(-3.87578335377325,74.3940262116388,
12.));
#158649=CARTESIAN_POINT('Ctrl Pts',(-3.87992989995747,74.3836349189184,
0.));
#158650=CARTESIAN_POINT('Ctrl Pts',(-3.87992989995747,74.3836349189184,
12.));
#158651=CARTESIAN_POINT('Ctrl Pts',(-3.88613891247984,74.3680548786661,
0.));
#158652=CARTESIAN_POINT('Ctrl Pts',(-3.88613891247984,74.3680548786661,
12.));
#158653=CARTESIAN_POINT('Ctrl Pts',(-3.89439598145329,74.3472952898745,
0.));
#158654=CARTESIAN_POINT('Ctrl Pts',(-3.89439598145329,74.3472952898745,
12.));
#158655=CARTESIAN_POINT('Ctrl Pts',(-3.90468128904634,74.3213688090134,
0.));
#158656=CARTESIAN_POINT('Ctrl Pts',(-3.90468128904634,74.3213688090134,
12.));
#158657=CARTESIAN_POINT('Ctrl Pts',(-3.9149305628503,74.2954653518728,0.));
#158658=CARTESIAN_POINT('Ctrl Pts',(-3.9149305628503,74.2954653518728,12.));
#158659=CARTESIAN_POINT('Ctrl Pts',(-3.92514379920743,74.2695849516226,
0.));
#158660=CARTESIAN_POINT('Ctrl Pts',(-3.92514379920743,74.2695849516226,
12.));
#158661=CARTESIAN_POINT('Ctrl Pts',(-3.93532099774204,74.2437276593623,
0.));
#158662=CARTESIAN_POINT('Ctrl Pts',(-3.93532099774204,74.2437276593623,
12.));
#158663=CARTESIAN_POINT('Ctrl Pts',(-3.94546216377451,74.2178935492876,
0.));
#158664=CARTESIAN_POINT('Ctrl Pts',(-3.94546216377451,74.2178935492876,
12.));
#158665=CARTESIAN_POINT('Ctrl Pts',(-3.95556730821111,74.1920827166585,
0.));
#158666=CARTESIAN_POINT('Ctrl Pts',(-3.95556730821111,74.1920827166585,
12.));
#158667=CARTESIAN_POINT('Ctrl Pts',(-3.96563644549385,74.1662952702485,
0.));
#158668=CARTESIAN_POINT('Ctrl Pts',(-3.96563644549385,74.1662952702485,
12.));
#158669=CARTESIAN_POINT('Ctrl Pts',(-3.97566959209529,74.1405313263109,
0.));
#158670=CARTESIAN_POINT('Ctrl Pts',(-3.97566959209529,74.1405313263109,
12.));
#158671=CARTESIAN_POINT('Ctrl Pts',(-3.98566676483642,74.1147910020891,
0.));
#158672=CARTESIAN_POINT('Ctrl Pts',(-3.98566676483642,74.1147910020891,
12.));
#158673=CARTESIAN_POINT('Ctrl Pts',(-3.99562797918287,74.0890744091186,
0.));
#158674=CARTESIAN_POINT('Ctrl Pts',(-3.99562797918287,74.0890744091186,
12.));
#158675=CARTESIAN_POINT('Ctrl Pts',(-4.0055532478548,74.0633816478037,0.));
#158676=CARTESIAN_POINT('Ctrl Pts',(-4.0055532478548,74.0633816478037,12.));
#158677=CARTESIAN_POINT('Ctrl Pts',(-4.01544258176711,74.0377128111863,
0.));
#158678=CARTESIAN_POINT('Ctrl Pts',(-4.01544258176711,74.0377128111863,
12.));
#158679=CARTESIAN_POINT('Ctrl Pts',(-4.02529599070095,74.012067987646,0.));
#158680=CARTESIAN_POINT('Ctrl Pts',(-4.02529599070095,74.012067987646,12.));
#158681=CARTESIAN_POINT('Ctrl Pts',(-4.0351134841066,73.9864472641033,0.));
#158682=CARTESIAN_POINT('Ctrl Pts',(-4.0351134841066,73.9864472641033,12.));
#158683=CARTESIAN_POINT('Ctrl Pts',(-4.04489507179957,73.9608507287909,
0.));
#158684=CARTESIAN_POINT('Ctrl Pts',(-4.04489507179957,73.9608507287909,
12.));
#158685=CARTESIAN_POINT('Ctrl Pts',(-4.05464076484752,73.9352784747608,
0.));
#158686=CARTESIAN_POINT('Ctrl Pts',(-4.05464076484752,73.9352784747608,
12.));
#158687=CARTESIAN_POINT('Ctrl Pts',(-4.06435057547325,73.9097305995115,
0.));
#158688=CARTESIAN_POINT('Ctrl Pts',(-4.06435057547325,73.9097305995115,
12.));
#158689=CARTESIAN_POINT('Ctrl Pts',(-4.07402451665245,73.8842072034008,
0.));
#158690=CARTESIAN_POINT('Ctrl Pts',(-4.07402451665245,73.8842072034008,
12.));
#158691=CARTESIAN_POINT('Ctrl Pts',(-4.08366260180674,73.8587083884191,
0.));
#158692=CARTESIAN_POINT('Ctrl Pts',(-4.08366260180674,73.8587083884191,
12.));
#158693=CARTESIAN_POINT('Ctrl Pts',(-4.09326484448233,73.8332342568989,
0.));
#158694=CARTESIAN_POINT('Ctrl Pts',(-4.09326484448233,73.8332342568989,
12.));
#158695=CARTESIAN_POINT('Ctrl Pts',(-4.10283125798729,73.8077849100342,
0.));
#158696=CARTESIAN_POINT('Ctrl Pts',(-4.10283125798729,73.8077849100342,
12.));
#158697=CARTESIAN_POINT('Ctrl Pts',(-4.11236185522787,73.7823604472159,
0.));
#158698=CARTESIAN_POINT('Ctrl Pts',(-4.11236185522787,73.7823604472159,
12.));
#158699=CARTESIAN_POINT('Ctrl Pts',(-4.12185664890557,73.7569609668528,
0.));
#158700=CARTESIAN_POINT('Ctrl Pts',(-4.12185664890557,73.7569609668528,
12.));
#158701=CARTESIAN_POINT('Ctrl Pts',(-4.13131565163578,73.7315865668522,
0.));
#158702=CARTESIAN_POINT('Ctrl Pts',(-4.13131565163578,73.7315865668522,
12.));
#158703=CARTESIAN_POINT('Ctrl Pts',(-4.14073887610153,73.7062373452342,
0.));
#158704=CARTESIAN_POINT('Ctrl Pts',(-4.14073887610153,73.7062373452342,
12.));
#158705=CARTESIAN_POINT('Ctrl Pts',(-4.15012633519723,73.6809134006897,
0.));
#158706=CARTESIAN_POINT('Ctrl Pts',(-4.15012633519723,73.6809134006897,
12.));
#158707=CARTESIAN_POINT('Ctrl Pts',(-4.15947804217784,73.6556148331489,
0.));
#158708=CARTESIAN_POINT('Ctrl Pts',(-4.15947804217784,73.6556148331489,
12.));
#158709=CARTESIAN_POINT('Ctrl Pts',(-4.1687940105878,73.6303417435251,0.));
#158710=CARTESIAN_POINT('Ctrl Pts',(-4.1687940105878,73.6303417435251,12.));
#158711=CARTESIAN_POINT('Ctrl Pts',(-4.17807425419813,73.6050942334768,
0.));
#158712=CARTESIAN_POINT('Ctrl Pts',(-4.17807425419813,73.6050942334768,
12.));
#158713=CARTESIAN_POINT('Ctrl Pts',(-4.18731878694236,73.5798724051519,
0.));
#158714=CARTESIAN_POINT('Ctrl Pts',(-4.18731878694236,73.5798724051519,
12.));
#158715=CARTESIAN_POINT('Ctrl Pts',(-4.19652762286127,73.5546763609572,
0.));
#158716=CARTESIAN_POINT('Ctrl Pts',(-4.19652762286127,73.5546763609572,
12.));
#158717=CARTESIAN_POINT('Ctrl Pts',(-4.2057007760373,73.5295062032628,0.));
#158718=CARTESIAN_POINT('Ctrl Pts',(-4.2057007760373,73.5295062032628,12.));
#158719=CARTESIAN_POINT('Ctrl Pts',(-4.21483826059441,73.5043620344116,
0.));
#158720=CARTESIAN_POINT('Ctrl Pts',(-4.21483826059441,73.5043620344116,
12.));
#158721=CARTESIAN_POINT('Ctrl Pts',(-4.22394009072756,73.4792439568633,
0.));
#158722=CARTESIAN_POINT('Ctrl Pts',(-4.22394009072756,73.4792439568633,
12.));
#158723=CARTESIAN_POINT('Ctrl Pts',(-4.23300628072758,73.4541520732948,
0.));
#158724=CARTESIAN_POINT('Ctrl Pts',(-4.23300628072758,73.4541520732948,
12.));
#158725=CARTESIAN_POINT('Ctrl Pts',(-4.24203684500939,73.4290864867101,
0.));
#158726=CARTESIAN_POINT('Ctrl Pts',(-4.24203684500939,73.4290864867101,
12.));
#158727=CARTESIAN_POINT('Ctrl Pts',(-4.25103179814887,73.4040473005592,
0.));
#158728=CARTESIAN_POINT('Ctrl Pts',(-4.25103179814887,73.4040473005592,
12.));
#158729=CARTESIAN_POINT('Ctrl Pts',(-4.25999115489899,73.3790346187938,
0.));
#158730=CARTESIAN_POINT('Ctrl Pts',(-4.25999115489899,73.3790346187938,
12.));
#158731=CARTESIAN_POINT('Ctrl Pts',(-4.268914930167,73.3540485458065,0.));
#158732=CARTESIAN_POINT('Ctrl Pts',(-4.268914930167,73.3540485458065,12.));
#158733=CARTESIAN_POINT('Ctrl Pts',(-4.2778031390039,73.3290891863949,0.));
#158734=CARTESIAN_POINT('Ctrl Pts',(-4.2778031390039,73.3290891863949,12.));
#158735=CARTESIAN_POINT('Ctrl Pts',(-4.28665579659301,73.3041566457135,
0.));
#158736=CARTESIAN_POINT('Ctrl Pts',(-4.28665579659301,73.3041566457135,
12.));
#158737=CARTESIAN_POINT('Ctrl Pts',(-4.29547291824287,73.2792510292254,
0.));
#158738=CARTESIAN_POINT('Ctrl Pts',(-4.29547291824287,73.2792510292254,
12.));
#158739=CARTESIAN_POINT('Ctrl Pts',(-4.3042545193823,73.2543724426577,0.));
#158740=CARTESIAN_POINT('Ctrl Pts',(-4.3042545193823,73.2543724426577,12.));
#158741=CARTESIAN_POINT('Ctrl Pts',(-4.31300061556098,73.2295209920334,
0.));
#158742=CARTESIAN_POINT('Ctrl Pts',(-4.31300061556098,73.2295209920334,
12.));
#158743=CARTESIAN_POINT('Ctrl Pts',(-4.32171122245214,73.204696783694,0.));
#158744=CARTESIAN_POINT('Ctrl Pts',(-4.32171122245214,73.204696783694,12.));
#158745=CARTESIAN_POINT('Ctrl Pts',(-4.33038635585877,73.1798999243235,
0.));
#158746=CARTESIAN_POINT('Ctrl Pts',(-4.33038635585877,73.1798999243235,
12.));
#158747=CARTESIAN_POINT('Ctrl Pts',(-4.33902603172141,73.1551305209685,
0.));
#158748=CARTESIAN_POINT('Ctrl Pts',(-4.33902603172141,73.1551305209685,
12.));
#158749=CARTESIAN_POINT('Ctrl Pts',(-4.34763026613158,73.130388681059,0.));
#158750=CARTESIAN_POINT('Ctrl Pts',(-4.34763026613158,73.130388681059,12.));
#158751=CARTESIAN_POINT('Ctrl Pts',(-4.3561990753272,73.1056745124087,0.));
#158752=CARTESIAN_POINT('Ctrl Pts',(-4.3561990753272,73.1056745124087,12.));
#158753=CARTESIAN_POINT('Ctrl Pts',(-4.36473247568641,73.0809881232103,
0.));
#158754=CARTESIAN_POINT('Ctrl Pts',(-4.36473247568641,73.0809881232103,
12.));
#158755=CARTESIAN_POINT('Ctrl Pts',(-4.37323048372607,73.0563296220299,
0.));
#158756=CARTESIAN_POINT('Ctrl Pts',(-4.37323048372607,73.0563296220299,
12.));
#158757=CARTESIAN_POINT('Ctrl Pts',(-4.38169311610151,73.0316991177993,
0.));
#158758=CARTESIAN_POINT('Ctrl Pts',(-4.38169311610151,73.0316991177993,
12.));
#158759=CARTESIAN_POINT('Ctrl Pts',(-4.39012038961139,73.007096719804,0.));
#158760=CARTESIAN_POINT('Ctrl Pts',(-4.39012038961139,73.007096719804,12.));
#158761=CARTESIAN_POINT('Ctrl Pts',(-4.39851232119722,72.9825225376846,
0.));
#158762=CARTESIAN_POINT('Ctrl Pts',(-4.39851232119722,72.9825225376846,
12.));
#158763=CARTESIAN_POINT('Ctrl Pts',(-4.40686892793957,72.95797668145,0.));
#158764=CARTESIAN_POINT('Ctrl Pts',(-4.40686892793957,72.95797668145,12.));
#158765=CARTESIAN_POINT('Ctrl Pts',(-4.41519022705921,72.9334592614829,
0.));
#158766=CARTESIAN_POINT('Ctrl Pts',(-4.41519022705921,72.9334592614829,
12.));
#158767=CARTESIAN_POINT('Ctrl Pts',(-4.42347623591942,72.9089703885462,
0.));
#158768=CARTESIAN_POINT('Ctrl Pts',(-4.42347623591942,72.9089703885462,
12.));
#158769=CARTESIAN_POINT('Ctrl Pts',(-4.43172697203349,72.8845101737855,
0.));
#158770=CARTESIAN_POINT('Ctrl Pts',(-4.43172697203349,72.8845101737855,
12.));
#158771=CARTESIAN_POINT('Ctrl Pts',(-4.43994245306818,72.8600787287318,
0.));
#158772=CARTESIAN_POINT('Ctrl Pts',(-4.43994245306818,72.8600787287318,
12.));
#158773=CARTESIAN_POINT('Ctrl Pts',(-4.44812269683738,72.8356761653069,
0.));
#158774=CARTESIAN_POINT('Ctrl Pts',(-4.44812269683738,72.8356761653069,
12.));
#158775=CARTESIAN_POINT('Ctrl Pts',(-4.45626772130146,72.8113025958262,
0.));
#158776=CARTESIAN_POINT('Ctrl Pts',(-4.45626772130146,72.8113025958262,
12.));
#158777=CARTESIAN_POINT('Ctrl Pts',(-4.46437754456793,72.7869581329994,
0.));
#158778=CARTESIAN_POINT('Ctrl Pts',(-4.46437754456793,72.7869581329994,
12.));
#158779=CARTESIAN_POINT('Ctrl Pts',(-4.4724521848961,72.7626428899281,0.));
#158780=CARTESIAN_POINT('Ctrl Pts',(-4.4724521848961,72.7626428899281,12.));
#158781=CARTESIAN_POINT('Ctrl Pts',(-4.48049166070205,72.738356980103,0.));
#158782=CARTESIAN_POINT('Ctrl Pts',(-4.48049166070205,72.738356980103,12.));
#158783=CARTESIAN_POINT('Ctrl Pts',(-4.48849599055337,72.714100517414,0.));
#158784=CARTESIAN_POINT('Ctrl Pts',(-4.48849599055337,72.714100517414,12.));
#158785=CARTESIAN_POINT('Ctrl Pts',(-4.49646519316813,72.6898736161542,
0.));
#158786=CARTESIAN_POINT('Ctrl Pts',(-4.49646519316813,72.6898736161542,
12.));
#158787=CARTESIAN_POINT('Ctrl Pts',(-4.50439928741604,72.6656763910241,
0.));
#158788=CARTESIAN_POINT('Ctrl Pts',(-4.50439928741604,72.6656763910241,
12.));
#158789=CARTESIAN_POINT('Ctrl Pts',(-4.51229829232264,72.6415089571321,
0.));
#158790=CARTESIAN_POINT('Ctrl Pts',(-4.51229829232264,72.6415089571321,
12.));
#158791=CARTESIAN_POINT('Ctrl Pts',(-4.52016222707638,72.6173714299942,
0.));
#158792=CARTESIAN_POINT('Ctrl Pts',(-4.52016222707638,72.6173714299942,
12.));
#158793=CARTESIAN_POINT('Ctrl Pts',(-4.52799111102392,72.5932639255409,
0.));
#158794=CARTESIAN_POINT('Ctrl Pts',(-4.52799111102392,72.5932639255409,
12.));
#158795=CARTESIAN_POINT('Ctrl Pts',(-4.535784963668,72.5691865601223,0.));
#158796=CARTESIAN_POINT('Ctrl Pts',(-4.535784963668,72.5691865601223,12.));
#158797=CARTESIAN_POINT('Ctrl Pts',(-4.54354380466822,72.5451394505104,
0.));
#158798=CARTESIAN_POINT('Ctrl Pts',(-4.54354380466822,72.5451394505104,
12.));
#158799=CARTESIAN_POINT('Ctrl Pts',(-4.55126765384404,72.5211227139001,
0.));
#158800=CARTESIAN_POINT('Ctrl Pts',(-4.55126765384404,72.5211227139001,
12.));
#158801=CARTESIAN_POINT('Ctrl Pts',(-4.55895653118221,72.4971364679068,
0.));
#158802=CARTESIAN_POINT('Ctrl Pts',(-4.55895653118221,72.4971364679068,
12.));
#158803=CARTESIAN_POINT('Ctrl Pts',(-4.56661045683376,72.4731808305728,
0.));
#158804=CARTESIAN_POINT('Ctrl Pts',(-4.56661045683376,72.4731808305728,
12.));
#158805=CARTESIAN_POINT('Ctrl Pts',(-4.57422945111102,72.4492559203745,
0.));
#158806=CARTESIAN_POINT('Ctrl Pts',(-4.57422945111102,72.4492559203745,
12.));
#158807=CARTESIAN_POINT('Ctrl Pts',(-4.58181353448852,72.4253618562252,
0.));
#158808=CARTESIAN_POINT('Ctrl Pts',(-4.58181353448852,72.4253618562252,
12.));
#158809=CARTESIAN_POINT('Ctrl Pts',(-4.58936272760544,72.401498757478,0.));
#158810=CARTESIAN_POINT('Ctrl Pts',(-4.58936272760544,72.401498757478,12.));
#158811=CARTESIAN_POINT('Ctrl Pts',(-4.5968770512733,72.3776667439227,0.));
#158812=CARTESIAN_POINT('Ctrl Pts',(-4.5968770512733,72.3776667439227,12.));
#158813=CARTESIAN_POINT('Ctrl Pts',(-4.60435652647453,72.3538659357913,
0.));
#158814=CARTESIAN_POINT('Ctrl Pts',(-4.60435652647453,72.3538659357913,
12.));
#158815=CARTESIAN_POINT('Ctrl Pts',(-4.61180117435862,72.3300964537658,
0.));
#158816=CARTESIAN_POINT('Ctrl Pts',(-4.61180117435862,72.3300964537658,
12.));
#158817=CARTESIAN_POINT('Ctrl Pts',(-4.61921101624292,72.3063584189807,
0.));
#158818=CARTESIAN_POINT('Ctrl Pts',(-4.61921101624292,72.3063584189807,
12.));
#158819=CARTESIAN_POINT('Ctrl Pts',(-4.62658607361466,72.2826519530259,
0.));
#158820=CARTESIAN_POINT('Ctrl Pts',(-4.62658607361466,72.2826519530259,
12.));
#158821=CARTESIAN_POINT('Ctrl Pts',(-4.63392636813844,72.2589771779456,
0.));
#158822=CARTESIAN_POINT('Ctrl Pts',(-4.63392636813844,72.2589771779456,
12.));
#158823=CARTESIAN_POINT('Ctrl Pts',(-4.64123192165628,72.2353342162417,
0.));
#158824=CARTESIAN_POINT('Ctrl Pts',(-4.64123192165628,72.2353342162417,
12.));
#158825=CARTESIAN_POINT('Ctrl Pts',(-4.64850275618323,72.2117231908822,
0.));
#158826=CARTESIAN_POINT('Ctrl Pts',(-4.64850275618323,72.2117231908822,
12.));
#158827=CARTESIAN_POINT('Ctrl Pts',(-4.65573889390822,72.1881442253053,
0.));
#158828=CARTESIAN_POINT('Ctrl Pts',(-4.65573889390822,72.1881442253053,
12.));
#158829=CARTESIAN_POINT('Ctrl Pts',(-4.6629403571957,72.1645974434216,0.));
#158830=CARTESIAN_POINT('Ctrl Pts',(-4.6629403571957,72.1645974434216,12.));
#158831=CARTESIAN_POINT('Ctrl Pts',(-4.67010716859285,72.1410829696128,
0.));
#158832=CARTESIAN_POINT('Ctrl Pts',(-4.67010716859285,72.1410829696128,
12.));
#158833=CARTESIAN_POINT('Ctrl Pts',(-4.67723935083095,72.1176009287351,
0.));
#158834=CARTESIAN_POINT('Ctrl Pts',(-4.67723935083095,72.1176009287351,
12.));
#158835=CARTESIAN_POINT('Ctrl Pts',(-4.68433692682069,72.0941514461287,
0.));
#158836=CARTESIAN_POINT('Ctrl Pts',(-4.68433692682069,72.0941514461287,
12.));
#158837=CARTESIAN_POINT('Ctrl Pts',(-4.69139991965284,72.0707346476213,
0.));
#158838=CARTESIAN_POINT('Ctrl Pts',(-4.69139991965284,72.0707346476213,
12.));
#158839=CARTESIAN_POINT('Ctrl Pts',(-4.69842835259992,72.0473506595318,
0.));
#158840=CARTESIAN_POINT('Ctrl Pts',(-4.69842835259992,72.0473506595318,
12.));
#158841=CARTESIAN_POINT('Ctrl Pts',(-4.70542224912301,72.0239996086686,
0.));
#158842=CARTESIAN_POINT('Ctrl Pts',(-4.70542224912301,72.0239996086686,
12.));
#158843=CARTESIAN_POINT('Ctrl Pts',(-4.71238163287397,72.0006816223325,
0.));
#158844=CARTESIAN_POINT('Ctrl Pts',(-4.71238163287397,72.0006816223325,
12.));
#158845=CARTESIAN_POINT('Ctrl Pts',(-4.7193065276907,71.9773968283259,0.));
#158846=CARTESIAN_POINT('Ctrl Pts',(-4.7193065276907,71.9773968283259,12.));
#158847=CARTESIAN_POINT('Ctrl Pts',(-4.72619695759774,71.9541453549579,
0.));
#158848=CARTESIAN_POINT('Ctrl Pts',(-4.72619695759774,71.9541453549579,
12.));
#158849=CARTESIAN_POINT('Ctrl Pts',(-4.73305294680785,71.9309273310471,
0.));
#158850=CARTESIAN_POINT('Ctrl Pts',(-4.73305294680785,71.9309273310471,
12.));
#158851=CARTESIAN_POINT('Ctrl Pts',(-4.73987451972864,71.9077428859212,
0.));
#158852=CARTESIAN_POINT('Ctrl Pts',(-4.73987451972864,71.9077428859212,
12.));
#158853=CARTESIAN_POINT('Ctrl Pts',(-4.74666170096547,71.8845921494189,
0.));
#158854=CARTESIAN_POINT('Ctrl Pts',(-4.74666170096547,71.8845921494189,
12.));
#158855=CARTESIAN_POINT('Ctrl Pts',(-4.7534145153167,71.8614752519008,0.));
#158856=CARTESIAN_POINT('Ctrl Pts',(-4.7534145153167,71.8614752519008,12.));
#158857=CARTESIAN_POINT('Ctrl Pts',(-4.7601329877742,71.8383923242531,0.));
#158858=CARTESIAN_POINT('Ctrl Pts',(-4.7601329877742,71.8383923242531,12.));
#158859=CARTESIAN_POINT('Ctrl Pts',(-4.76681714352502,71.8153434978923,
0.));
#158860=CARTESIAN_POINT('Ctrl Pts',(-4.76681714352502,71.8153434978923,
12.));
#158861=CARTESIAN_POINT('Ctrl Pts',(-4.77346700795792,71.7923289047643,
0.));
#158862=CARTESIAN_POINT('Ctrl Pts',(-4.77346700795792,71.7923289047643,
12.));
#158863=CARTESIAN_POINT('Ctrl Pts',(-4.7800826066665,71.769348677346,0.));
#158864=CARTESIAN_POINT('Ctrl Pts',(-4.7800826066665,71.769348677346,12.));
#158865=CARTESIAN_POINT('Ctrl Pts',(-4.78666396544458,71.7464029486563,
0.));
#158866=CARTESIAN_POINT('Ctrl Pts',(-4.78666396544458,71.7464029486563,
12.));
#158867=CARTESIAN_POINT('Ctrl Pts',(-4.79321111028676,71.723491852261,0.));
#158868=CARTESIAN_POINT('Ctrl Pts',(-4.79321111028676,71.723491852261,12.));
#158869=CARTESIAN_POINT('Ctrl Pts',(-4.79972406739011,71.7006155222764,
0.));
#158870=CARTESIAN_POINT('Ctrl Pts',(-4.79972406739011,71.7006155222764,
12.));
#158871=CARTESIAN_POINT('Ctrl Pts',(-4.80620286316075,71.6777740933687,
0.));
#158872=CARTESIAN_POINT('Ctrl Pts',(-4.80620286316075,71.6777740933687,
12.));
#158873=CARTESIAN_POINT('Ctrl Pts',(-4.81264752421713,71.6549677007582,
0.));
#158874=CARTESIAN_POINT('Ctrl Pts',(-4.81264752421713,71.6549677007582,
12.));
#158875=CARTESIAN_POINT('Ctrl Pts',(-4.81905807738542,71.6321964802297,
0.));
#158876=CARTESIAN_POINT('Ctrl Pts',(-4.81905807738542,71.6321964802297,
12.));
#158877=CARTESIAN_POINT('Ctrl Pts',(-4.82543454970021,71.6094605681353,
0.));
#158878=CARTESIAN_POINT('Ctrl Pts',(-4.82543454970021,71.6094605681353,
12.));
#158879=CARTESIAN_POINT('Ctrl Pts',(-4.8317769684064,71.5867601014008,0.));
#158880=CARTESIAN_POINT('Ctrl Pts',(-4.8317769684064,71.5867601014008,12.));
#158881=CARTESIAN_POINT('Ctrl Pts',(-4.83808536096589,71.5640952175239,
0.));
#158882=CARTESIAN_POINT('Ctrl Pts',(-4.83808536096589,71.5640952175239,
12.));
#158883=CARTESIAN_POINT('Ctrl Pts',(-4.84435975506056,71.5414660545778,
0.));
#158884=CARTESIAN_POINT('Ctrl Pts',(-4.84435975506056,71.5414660545778,
12.));
#158885=CARTESIAN_POINT('Ctrl Pts',(-4.85060017858786,71.5188727512231,
0.));
#158886=CARTESIAN_POINT('Ctrl Pts',(-4.85060017858786,71.5188727512231,
12.));
#158887=CARTESIAN_POINT('Ctrl Pts',(-4.85680665966184,71.4963154467128,
0.));
#158888=CARTESIAN_POINT('Ctrl Pts',(-4.85680665966184,71.4963154467128,
12.));
#158889=CARTESIAN_POINT('Ctrl Pts',(-4.86297922661499,71.4737942808971,
0.));
#158890=CARTESIAN_POINT('Ctrl Pts',(-4.86297922661499,71.4737942808971,
12.));
#158891=CARTESIAN_POINT('Ctrl Pts',(-4.86911790800533,71.4513093942216,
0.));
#158892=CARTESIAN_POINT('Ctrl Pts',(-4.86911790800533,71.4513093942216,
12.));
#158893=CARTESIAN_POINT('Ctrl Pts',(-4.87522273261881,71.4288609277324,
0.));
#158894=CARTESIAN_POINT('Ctrl Pts',(-4.87522273261881,71.4288609277324,
12.));
#158895=CARTESIAN_POINT('Ctrl Pts',(-4.88129372946524,71.4064490230857,
0.));
#158896=CARTESIAN_POINT('Ctrl Pts',(-4.88129372946524,71.4064490230857,
12.));
#158897=CARTESIAN_POINT('Ctrl Pts',(-4.88733092777964,71.3840738225547,
0.));
#158898=CARTESIAN_POINT('Ctrl Pts',(-4.88733092777964,71.3840738225547,
12.));
#158899=CARTESIAN_POINT('Ctrl Pts',(-4.89333435702424,71.3617354690342,
0.));
#158900=CARTESIAN_POINT('Ctrl Pts',(-4.89333435702424,71.3617354690342,
12.));
#158901=CARTESIAN_POINT('Ctrl Pts',(-4.89930404689599,71.3394341060396,
0.));
#158902=CARTESIAN_POINT('Ctrl Pts',(-4.89930404689599,71.3394341060396,
12.));
#158903=CARTESIAN_POINT('Ctrl Pts',(-4.90524002732806,71.3171698777124,
0.));
#158904=CARTESIAN_POINT('Ctrl Pts',(-4.90524002732806,71.3171698777124,
12.));
#158905=CARTESIAN_POINT('Ctrl Pts',(-4.91114232848623,71.2949429288319,
0.));
#158906=CARTESIAN_POINT('Ctrl Pts',(-4.91114232848623,71.2949429288319,
12.));
#158907=CARTESIAN_POINT('Ctrl Pts',(-4.91701098077041,71.27275340482,0.));
#158908=CARTESIAN_POINT('Ctrl Pts',(-4.91701098077041,71.27275340482,12.));
#158909=CARTESIAN_POINT('Ctrl Pts',(-4.9228460148171,71.2506014517457,0.));
#158910=CARTESIAN_POINT('Ctrl Pts',(-4.9228460148171,71.2506014517457,12.));
#158911=CARTESIAN_POINT('Ctrl Pts',(-4.92864746150711,71.2284872163248,
0.));
#158912=CARTESIAN_POINT('Ctrl Pts',(-4.92864746150711,71.2284872163248,
12.));
#158913=CARTESIAN_POINT('Ctrl Pts',(-4.93441535196594,71.206410845926,0.));
#158914=CARTESIAN_POINT('Ctrl Pts',(-4.93441535196594,71.206410845926,12.));
#158915=CARTESIAN_POINT('Ctrl Pts',(-4.94014971756097,71.184372488583,0.));
#158916=CARTESIAN_POINT('Ctrl Pts',(-4.94014971756097,71.184372488583,12.));
#158917=CARTESIAN_POINT('Ctrl Pts',(-4.94585058990337,71.1623722929998,
0.));
#158918=CARTESIAN_POINT('Ctrl Pts',(-4.94585058990337,71.1623722929998,
12.));
#158919=CARTESIAN_POINT('Ctrl Pts',(-4.95151800085111,71.1404104085561,
0.));
#158920=CARTESIAN_POINT('Ctrl Pts',(-4.95151800085111,71.1404104085561,
12.));
#158921=CARTESIAN_POINT('Ctrl Pts',(-4.95715198251704,71.1184869853071,
0.));
#158922=CARTESIAN_POINT('Ctrl Pts',(-4.95715198251704,71.1184869853071,
12.));
#158923=CARTESIAN_POINT('Ctrl Pts',(-4.96275256726787,71.0966021739922,
0.));
#158924=CARTESIAN_POINT('Ctrl Pts',(-4.96275256726787,71.0966021739922,
12.));
#158925=CARTESIAN_POINT('Ctrl Pts',(-4.96831978772201,71.0747561260443,
0.));
#158926=CARTESIAN_POINT('Ctrl Pts',(-4.96831978772201,71.0747561260443,
12.));
#158927=CARTESIAN_POINT('Ctrl Pts',(-4.97385367675157,71.0529489935959,
0.));
#158928=CARTESIAN_POINT('Ctrl Pts',(-4.97385367675157,71.0529489935959,
12.));
#158929=CARTESIAN_POINT('Ctrl Pts',(-4.97935426748577,71.031180929482,0.));
#158930=CARTESIAN_POINT('Ctrl Pts',(-4.97935426748577,71.031180929482,12.));
#158931=CARTESIAN_POINT('Ctrl Pts',(-4.98482159331851,71.0094520872375,
0.));
#158932=CARTESIAN_POINT('Ctrl Pts',(-4.98482159331851,71.0094520872375,
12.));
#158933=CARTESIAN_POINT('Ctrl Pts',(-4.99025568790653,70.9877626211112,
0.));
#158934=CARTESIAN_POINT('Ctrl Pts',(-4.99025568790653,70.9877626211112,
12.));
#158935=CARTESIAN_POINT('Ctrl Pts',(-4.99565658516906,70.9661126860773,
0.));
#158936=CARTESIAN_POINT('Ctrl Pts',(-4.99565658516906,70.9661126860773,
12.));
#158937=CARTESIAN_POINT('Ctrl Pts',(-5.00102431929039,70.9445024378439,
0.));
#158938=CARTESIAN_POINT('Ctrl Pts',(-5.00102431929039,70.9445024378439,
12.));
#158939=CARTESIAN_POINT('Ctrl Pts',(-5.00635892472518,70.9229320328588,
0.));
#158940=CARTESIAN_POINT('Ctrl Pts',(-5.00635892472518,70.9229320328588,
12.));
#158941=CARTESIAN_POINT('Ctrl Pts',(-5.01166043620573,70.9014016283123,
0.));
#158942=CARTESIAN_POINT('Ctrl Pts',(-5.01166043620573,70.9014016283123,
12.));
#158943=CARTESIAN_POINT('Ctrl Pts',(-5.01692888873793,70.8799113821449,
0.));
#158944=CARTESIAN_POINT('Ctrl Pts',(-5.01692888873793,70.8799113821449,
12.));
#158945=CARTESIAN_POINT('Ctrl Pts',(-5.0221643176006,70.8584614530517,0.));
#158946=CARTESIAN_POINT('Ctrl Pts',(-5.0221643176006,70.8584614530517,12.));
#158947=CARTESIAN_POINT('Ctrl Pts',(-5.02736675834691,70.8370520004844,
0.));
#158948=CARTESIAN_POINT('Ctrl Pts',(-5.02736675834691,70.8370520004844,
12.));
#158949=CARTESIAN_POINT('Ctrl Pts',(-5.03253624680941,70.8156831846494,
0.));
#158950=CARTESIAN_POINT('Ctrl Pts',(-5.03253624680941,70.8156831846494,
12.));
#158951=CARTESIAN_POINT('Ctrl Pts',(-5.03767281910483,70.7943551665071,
0.));
#158952=CARTESIAN_POINT('Ctrl Pts',(-5.03767281910483,70.7943551665071,
12.));
#158953=CARTESIAN_POINT('Ctrl Pts',(-5.04277651163356,70.7730681077997,
0.));
#158954=CARTESIAN_POINT('Ctrl Pts',(-5.04277651163356,70.7730681077997,
12.));
#158955=CARTESIAN_POINT('Ctrl Pts',(-5.04784736108351,70.7518221710715,
0.));
#158956=CARTESIAN_POINT('Ctrl Pts',(-5.04784736108351,70.7518221710715,
12.));
#158957=CARTESIAN_POINT('Ctrl Pts',(-5.05288540443478,70.7306175196856,
0.));
#158958=CARTESIAN_POINT('Ctrl Pts',(-5.05288540443478,70.7306175196856,
12.));
#158959=CARTESIAN_POINT('Ctrl Pts',(-5.05789067897041,70.7094543178416,
0.));
#158960=CARTESIAN_POINT('Ctrl Pts',(-5.05789067897041,70.7094543178416,
12.));
#158961=CARTESIAN_POINT('Ctrl Pts',(-5.06286322227797,70.6883327305755,
0.));
#158962=CARTESIAN_POINT('Ctrl Pts',(-5.06286322227797,70.6883327305755,
12.));
#158963=CARTESIAN_POINT('Ctrl Pts',(-5.06780307224053,70.6672529237431,
0.));
#158964=CARTESIAN_POINT('Ctrl Pts',(-5.06780307224053,70.6672529237431,
12.));
#158965=CARTESIAN_POINT('Ctrl Pts',(-5.0727102670335,70.6462150640009,0.));
#158966=CARTESIAN_POINT('Ctrl Pts',(-5.0727102670335,70.6462150640009,12.));
#158967=CARTESIAN_POINT('Ctrl Pts',(-5.0775848451231,70.6252193187892,0.));
#158968=CARTESIAN_POINT('Ctrl Pts',(-5.0775848451231,70.6252193187892,12.));
#158969=CARTESIAN_POINT('Ctrl Pts',(-5.08242684526704,70.6042658562951,
0.));
#158970=CARTESIAN_POINT('Ctrl Pts',(-5.08242684526704,70.6042658562951,
12.));
#158971=CARTESIAN_POINT('Ctrl Pts',(-5.08723630652291,70.5833548455043,
0.));
#158972=CARTESIAN_POINT('Ctrl Pts',(-5.08723630652291,70.5833548455043,
12.));
#158973=CARTESIAN_POINT('Ctrl Pts',(-5.09201326826146,70.5624864562841,
0.));
#158974=CARTESIAN_POINT('Ctrl Pts',(-5.09201326826146,70.5624864562841,
12.));
#158975=CARTESIAN_POINT('Ctrl Pts',(-5.09675777018182,70.5416608594526,
0.));
#158976=CARTESIAN_POINT('Ctrl Pts',(-5.09675777018182,70.5416608594526,
12.));
#158977=CARTESIAN_POINT('Ctrl Pts',(-5.10146985232928,70.5208782268482,
0.));
#158978=CARTESIAN_POINT('Ctrl Pts',(-5.10146985232928,70.5208782268482,
12.));
#158979=CARTESIAN_POINT('Ctrl Pts',(-5.10614955511643,70.5001387313963,
0.));
#158980=CARTESIAN_POINT('Ctrl Pts',(-5.10614955511643,70.5001387313963,
12.));
#158981=CARTESIAN_POINT('Ctrl Pts',(-5.11079691929193,70.4794425469799,
0.));
#158982=CARTESIAN_POINT('Ctrl Pts',(-5.11079691929193,70.4794425469799,
12.));
#158983=CARTESIAN_POINT('Ctrl Pts',(-5.1154119859092,70.4587898482946,0.));
#158984=CARTESIAN_POINT('Ctrl Pts',(-5.1154119859092,70.4587898482946,12.));
#158985=CARTESIAN_POINT('Ctrl Pts',(-5.11999479630215,70.438180810725,0.));
#158986=CARTESIAN_POINT('Ctrl Pts',(-5.11999479630215,70.438180810725,12.));
#158987=CARTESIAN_POINT('Ctrl Pts',(-5.12454539205347,70.4176156101633,
0.));
#158988=CARTESIAN_POINT('Ctrl Pts',(-5.12454539205347,70.4176156101633,
12.));
#158989=CARTESIAN_POINT('Ctrl Pts',(-5.12906381499486,70.3970944229885,
0.));
#158990=CARTESIAN_POINT('Ctrl Pts',(-5.12906381499486,70.3970944229885,
12.));
#158991=CARTESIAN_POINT('Ctrl Pts',(-5.13355010728591,70.3766174264786,
0.));
#158992=CARTESIAN_POINT('Ctrl Pts',(-5.13355010728591,70.3766174264786,
12.));
#158993=CARTESIAN_POINT('Ctrl Pts',(-5.13800431148911,70.3561847991725,
0.));
#158994=CARTESIAN_POINT('Ctrl Pts',(-5.13800431148911,70.3561847991725,
12.));
#158995=CARTESIAN_POINT('Ctrl Pts',(-5.14242647063467,70.3357967211782,
0.));
#158996=CARTESIAN_POINT('Ctrl Pts',(-5.14242647063467,70.3357967211782,
12.));
#158997=CARTESIAN_POINT('Ctrl Pts',(-5.14681662833054,70.31545337467,0.));
#158998=CARTESIAN_POINT('Ctrl Pts',(-5.14681662833054,70.31545337467,12.));
#158999=CARTESIAN_POINT('Ctrl Pts',(-5.15117482869224,70.2951549435469,
0.));
#159000=CARTESIAN_POINT('Ctrl Pts',(-5.15117482869224,70.2951549435469,
12.));
#159001=CARTESIAN_POINT('Ctrl Pts',(-5.15550111614838,70.2749016125073,
0.));
#159002=CARTESIAN_POINT('Ctrl Pts',(-5.15550111614838,70.2749016125073,
12.));
#159003=CARTESIAN_POINT('Ctrl Pts',(-5.159795535282,70.2546935662719,0.));
#159004=CARTESIAN_POINT('Ctrl Pts',(-5.159795535282,70.2546935662719,12.));
#159005=CARTESIAN_POINT('Ctrl Pts',(-5.16405813066994,70.2345309887864,
0.));
#159006=CARTESIAN_POINT('Ctrl Pts',(-5.16405813066994,70.2345309887864,
12.));
#159007=CARTESIAN_POINT('Ctrl Pts',(-5.1682889467014,70.2144140623004,0.));
#159008=CARTESIAN_POINT('Ctrl Pts',(-5.1682889467014,70.2144140623004,12.));
#159009=CARTESIAN_POINT('Ctrl Pts',(-5.1724880279342,70.1943429691214,0.));
#159010=CARTESIAN_POINT('Ctrl Pts',(-5.1724880279342,70.1943429691214,12.));
#159011=CARTESIAN_POINT('Ctrl Pts',(-5.176655419524,70.1743178937102,0.));
#159012=CARTESIAN_POINT('Ctrl Pts',(-5.176655419524,70.1743178937102,12.));
#159013=CARTESIAN_POINT('Ctrl Pts',(-5.18079116757659,70.1543390243882,
0.));
#159014=CARTESIAN_POINT('Ctrl Pts',(-5.18079116757659,70.1543390243882,
12.));
#159015=CARTESIAN_POINT('Ctrl Pts',(-5.18489531966234,70.1344065558106,
0.));
#159016=CARTESIAN_POINT('Ctrl Pts',(-5.18489531966234,70.1344065558106,
12.));
#159017=CARTESIAN_POINT('Ctrl Pts',(-5.18896792486523,70.1145206891833,
0.));
#159018=CARTESIAN_POINT('Ctrl Pts',(-5.18896792486523,70.1145206891833,
12.));
#159019=CARTESIAN_POINT('Ctrl Pts',(-5.19300903271544,70.0946816270957,
0.));
#159020=CARTESIAN_POINT('Ctrl Pts',(-5.19300903271544,70.0946816270957,
12.));
#159021=CARTESIAN_POINT('Ctrl Pts',(-5.19701869225514,70.0748895689716,
0.));
#159022=CARTESIAN_POINT('Ctrl Pts',(-5.19701869225514,70.0748895689716,
12.));
#159023=CARTESIAN_POINT('Ctrl Pts',(-5.20099695122677,70.0551447071106,
0.));
#159024=CARTESIAN_POINT('Ctrl Pts',(-5.20099695122677,70.0551447071106,
12.));
#159025=CARTESIAN_POINT('Ctrl Pts',(-5.20494385478083,70.0354472203604,
0.));
#159026=CARTESIAN_POINT('Ctrl Pts',(-5.20494385478083,70.0354472203604,
12.));
#159027=CARTESIAN_POINT('Ctrl Pts',(-5.20885944672914,70.0157972802255,
0.));
#159028=CARTESIAN_POINT('Ctrl Pts',(-5.20885944672914,70.0157972802255,
12.));
#159029=CARTESIAN_POINT('Ctrl Pts',(-5.21274377203321,69.996195063002,0.));
#159030=CARTESIAN_POINT('Ctrl Pts',(-5.21274377203321,69.996195063002,12.));
#159031=CARTESIAN_POINT('Ctrl Pts',(-5.21659687881139,69.9766407595385,
0.));
#159032=CARTESIAN_POINT('Ctrl Pts',(-5.21659687881139,69.9766407595385,
12.));
#159033=CARTESIAN_POINT('Ctrl Pts',(-5.22041882075627,69.9571345869996,
0.));
#159034=CARTESIAN_POINT('Ctrl Pts',(-5.22041882075627,69.9571345869996,
12.));
#159035=CARTESIAN_POINT('Ctrl Pts',(-5.22420965879808,69.9376767968951,
0.));
#159036=CARTESIAN_POINT('Ctrl Pts',(-5.22420965879808,69.9376767968951,
12.));
#159037=CARTESIAN_POINT('Ctrl Pts',(-5.22796945602603,69.9182676501892,
0.));
#159038=CARTESIAN_POINT('Ctrl Pts',(-5.22796945602603,69.9182676501892,
12.));
#159039=CARTESIAN_POINT('Ctrl Pts',(-5.23169827290452,69.8989073936606,
0.));
#159040=CARTESIAN_POINT('Ctrl Pts',(-5.23169827290452,69.8989073936606,
12.));
#159041=CARTESIAN_POINT('Ctrl Pts',(-5.23539616279715,69.8795962381676,
0.));
#159042=CARTESIAN_POINT('Ctrl Pts',(-5.23539616279715,69.8795962381676,
12.));
#159043=CARTESIAN_POINT('Ctrl Pts',(-5.23906316635141,69.8603343303016,
0.));
#159044=CARTESIAN_POINT('Ctrl Pts',(-5.23906316635141,69.8603343303016,
12.));
#159045=CARTESIAN_POINT('Ctrl Pts',(-5.24269931055075,69.8411217507931,
0.));
#159046=CARTESIAN_POINT('Ctrl Pts',(-5.24269931055075,69.8411217507931,
12.));
#159047=CARTESIAN_POINT('Ctrl Pts',(-5.2455835516022,69.8257911792542,0.));
#159048=CARTESIAN_POINT('Ctrl Pts',(-5.2455835516022,69.8257911792542,12.));
#159049=CARTESIAN_POINT('Ctrl Pts',(-5.24773285666673,69.8143154684447,
0.));
#159050=CARTESIAN_POINT('Ctrl Pts',(-5.24773285666673,69.8143154684447,
12.));
#159051=CARTESIAN_POINT('Ctrl Pts',(-5.24915955997537,69.8066748687863,
0.));
#159052=CARTESIAN_POINT('Ctrl Pts',(-5.24915955997537,69.8066748687863,
12.));
#159053=CARTESIAN_POINT('Ctrl Pts',(-5.24987136994591,69.8028570375098,
0.));
#159054=CARTESIAN_POINT('Ctrl Pts',(-5.24987136994591,69.8028570375098,
12.));
#159055=CARTESIAN_POINT('',(-5.24987136994591,69.8028570375098,12.));
#159056=CARTESIAN_POINT('Ctrl Pts',(-5.24987136994591,69.8028570375098,
12.));
#159057=CARTESIAN_POINT('Ctrl Pts',(-5.24915955997537,69.8066748687863,
12.));
#159058=CARTESIAN_POINT('Ctrl Pts',(-5.24773285666673,69.8143154684447,
12.));
#159059=CARTESIAN_POINT('Ctrl Pts',(-5.2455835516022,69.8257911792542,12.));
#159060=CARTESIAN_POINT('Ctrl Pts',(-5.24269931055075,69.8411217507931,
12.));
#159061=CARTESIAN_POINT('Ctrl Pts',(-5.23906316635141,69.8603343303016,
12.));
#159062=CARTESIAN_POINT('Ctrl Pts',(-5.23539616279715,69.8795962381676,
12.));
#159063=CARTESIAN_POINT('Ctrl Pts',(-5.23169827290452,69.8989073936606,
12.));
#159064=CARTESIAN_POINT('Ctrl Pts',(-5.22796945602603,69.9182676501892,
12.));
#159065=CARTESIAN_POINT('Ctrl Pts',(-5.22420965879808,69.9376767968951,
12.));
#159066=CARTESIAN_POINT('Ctrl Pts',(-5.22041882075627,69.9571345869996,
12.));
#159067=CARTESIAN_POINT('Ctrl Pts',(-5.21659687881139,69.9766407595385,
12.));
#159068=CARTESIAN_POINT('Ctrl Pts',(-5.21274377203321,69.996195063002,12.));
#159069=CARTESIAN_POINT('Ctrl Pts',(-5.20885944672914,70.0157972802255,
12.));
#159070=CARTESIAN_POINT('Ctrl Pts',(-5.20494385478083,70.0354472203604,
12.));
#159071=CARTESIAN_POINT('Ctrl Pts',(-5.20099695122677,70.0551447071106,
12.));
#159072=CARTESIAN_POINT('Ctrl Pts',(-5.19701869225514,70.0748895689716,
12.));
#159073=CARTESIAN_POINT('Ctrl Pts',(-5.19300903271544,70.0946816270957,
12.));
#159074=CARTESIAN_POINT('Ctrl Pts',(-5.18896792486523,70.1145206891833,
12.));
#159075=CARTESIAN_POINT('Ctrl Pts',(-5.18489531966234,70.1344065558106,
12.));
#159076=CARTESIAN_POINT('Ctrl Pts',(-5.18079116757659,70.1543390243882,
12.));
#159077=CARTESIAN_POINT('Ctrl Pts',(-5.176655419524,70.1743178937102,12.));
#159078=CARTESIAN_POINT('Ctrl Pts',(-5.1724880279342,70.1943429691214,12.));
#159079=CARTESIAN_POINT('Ctrl Pts',(-5.1682889467014,70.2144140623004,12.));
#159080=CARTESIAN_POINT('Ctrl Pts',(-5.16405813066994,70.2345309887864,
12.));
#159081=CARTESIAN_POINT('Ctrl Pts',(-5.159795535282,70.2546935662719,12.));
#159082=CARTESIAN_POINT('Ctrl Pts',(-5.15550111614838,70.2749016125073,
12.));
#159083=CARTESIAN_POINT('Ctrl Pts',(-5.15117482869224,70.2951549435469,
12.));
#159084=CARTESIAN_POINT('Ctrl Pts',(-5.14681662833054,70.31545337467,12.));
#159085=CARTESIAN_POINT('Ctrl Pts',(-5.14242647063467,70.3357967211782,
12.));
#159086=CARTESIAN_POINT('Ctrl Pts',(-5.13800431148911,70.3561847991725,
12.));
#159087=CARTESIAN_POINT('Ctrl Pts',(-5.13355010728591,70.3766174264786,
12.));
#159088=CARTESIAN_POINT('Ctrl Pts',(-5.12906381499486,70.3970944229885,
12.));
#159089=CARTESIAN_POINT('Ctrl Pts',(-5.12454539205347,70.4176156101633,
12.));
#159090=CARTESIAN_POINT('Ctrl Pts',(-5.11999479630215,70.438180810725,12.));
#159091=CARTESIAN_POINT('Ctrl Pts',(-5.1154119859092,70.4587898482946,12.));
#159092=CARTESIAN_POINT('Ctrl Pts',(-5.11079691929193,70.4794425469799,
12.));
#159093=CARTESIAN_POINT('Ctrl Pts',(-5.10614955511643,70.5001387313963,
12.));
#159094=CARTESIAN_POINT('Ctrl Pts',(-5.10146985232928,70.5208782268482,
12.));
#159095=CARTESIAN_POINT('Ctrl Pts',(-5.09675777018182,70.5416608594526,
12.));
#159096=CARTESIAN_POINT('Ctrl Pts',(-5.09201326826146,70.5624864562841,
12.));
#159097=CARTESIAN_POINT('Ctrl Pts',(-5.08723630652291,70.5833548455043,
12.));
#159098=CARTESIAN_POINT('Ctrl Pts',(-5.08242684526704,70.6042658562951,
12.));
#159099=CARTESIAN_POINT('Ctrl Pts',(-5.0775848451231,70.6252193187892,12.));
#159100=CARTESIAN_POINT('Ctrl Pts',(-5.0727102670335,70.6462150640009,12.));
#159101=CARTESIAN_POINT('Ctrl Pts',(-5.06780307224053,70.6672529237431,
12.));
#159102=CARTESIAN_POINT('Ctrl Pts',(-5.06286322227797,70.6883327305755,
12.));
#159103=CARTESIAN_POINT('Ctrl Pts',(-5.05789067897041,70.7094543178416,
12.));
#159104=CARTESIAN_POINT('Ctrl Pts',(-5.05288540443478,70.7306175196856,
12.));
#159105=CARTESIAN_POINT('Ctrl Pts',(-5.04784736108351,70.7518221710715,
12.));
#159106=CARTESIAN_POINT('Ctrl Pts',(-5.04277651163356,70.7730681077997,
12.));
#159107=CARTESIAN_POINT('Ctrl Pts',(-5.03767281910483,70.7943551665071,
12.));
#159108=CARTESIAN_POINT('Ctrl Pts',(-5.03253624680941,70.8156831846494,
12.));
#159109=CARTESIAN_POINT('Ctrl Pts',(-5.02736675834691,70.8370520004844,
12.));
#159110=CARTESIAN_POINT('Ctrl Pts',(-5.0221643176006,70.8584614530517,12.));
#159111=CARTESIAN_POINT('Ctrl Pts',(-5.01692888873793,70.8799113821449,
12.));
#159112=CARTESIAN_POINT('Ctrl Pts',(-5.01166043620573,70.9014016283123,
12.));
#159113=CARTESIAN_POINT('Ctrl Pts',(-5.00635892472518,70.9229320328588,
12.));
#159114=CARTESIAN_POINT('Ctrl Pts',(-5.00102431929039,70.9445024378439,
12.));
#159115=CARTESIAN_POINT('Ctrl Pts',(-4.99565658516906,70.9661126860773,
12.));
#159116=CARTESIAN_POINT('Ctrl Pts',(-4.99025568790653,70.9877626211112,
12.));
#159117=CARTESIAN_POINT('Ctrl Pts',(-4.98482159331851,71.0094520872375,
12.));
#159118=CARTESIAN_POINT('Ctrl Pts',(-4.97935426748577,71.031180929482,12.));
#159119=CARTESIAN_POINT('Ctrl Pts',(-4.97385367675157,71.0529489935959,
12.));
#159120=CARTESIAN_POINT('Ctrl Pts',(-4.96831978772201,71.0747561260443,
12.));
#159121=CARTESIAN_POINT('Ctrl Pts',(-4.96275256726787,71.0966021739922,
12.));
#159122=CARTESIAN_POINT('Ctrl Pts',(-4.95715198251704,71.1184869853071,
12.));
#159123=CARTESIAN_POINT('Ctrl Pts',(-4.95151800085111,71.1404104085561,
12.));
#159124=CARTESIAN_POINT('Ctrl Pts',(-4.94585058990337,71.1623722929998,
12.));
#159125=CARTESIAN_POINT('Ctrl Pts',(-4.94014971756097,71.184372488583,12.));
#159126=CARTESIAN_POINT('Ctrl Pts',(-4.93441535196594,71.206410845926,12.));
#159127=CARTESIAN_POINT('Ctrl Pts',(-4.92864746150711,71.2284872163248,
12.));
#159128=CARTESIAN_POINT('Ctrl Pts',(-4.9228460148171,71.2506014517457,12.));
#159129=CARTESIAN_POINT('Ctrl Pts',(-4.91701098077041,71.27275340482,12.));
#159130=CARTESIAN_POINT('Ctrl Pts',(-4.91114232848623,71.2949429288319,
12.));
#159131=CARTESIAN_POINT('Ctrl Pts',(-4.90524002732806,71.3171698777124,
12.));
#159132=CARTESIAN_POINT('Ctrl Pts',(-4.89930404689599,71.3394341060396,
12.));
#159133=CARTESIAN_POINT('Ctrl Pts',(-4.89333435702424,71.3617354690342,
12.));
#159134=CARTESIAN_POINT('Ctrl Pts',(-4.88733092777964,71.3840738225547,
12.));
#159135=CARTESIAN_POINT('Ctrl Pts',(-4.88129372946524,71.4064490230857,
12.));
#159136=CARTESIAN_POINT('Ctrl Pts',(-4.87522273261881,71.4288609277324,
12.));
#159137=CARTESIAN_POINT('Ctrl Pts',(-4.86911790800533,71.4513093942216,
12.));
#159138=CARTESIAN_POINT('Ctrl Pts',(-4.86297922661499,71.4737942808971,
12.));
#159139=CARTESIAN_POINT('Ctrl Pts',(-4.85680665966184,71.4963154467128,
12.));
#159140=CARTESIAN_POINT('Ctrl Pts',(-4.85060017858786,71.5188727512231,
12.));
#159141=CARTESIAN_POINT('Ctrl Pts',(-4.84435975506056,71.5414660545778,
12.));
#159142=CARTESIAN_POINT('Ctrl Pts',(-4.83808536096589,71.5640952175239,
12.));
#159143=CARTESIAN_POINT('Ctrl Pts',(-4.8317769684064,71.5867601014008,12.));
#159144=CARTESIAN_POINT('Ctrl Pts',(-4.82543454970021,71.6094605681353,
12.));
#159145=CARTESIAN_POINT('Ctrl Pts',(-4.81905807738542,71.6321964802297,
12.));
#159146=CARTESIAN_POINT('Ctrl Pts',(-4.81264752421713,71.6549677007582,
12.));
#159147=CARTESIAN_POINT('Ctrl Pts',(-4.80620286316075,71.6777740933687,
12.));
#159148=CARTESIAN_POINT('Ctrl Pts',(-4.79972406739011,71.7006155222764,
12.));
#159149=CARTESIAN_POINT('Ctrl Pts',(-4.79321111028676,71.723491852261,12.));
#159150=CARTESIAN_POINT('Ctrl Pts',(-4.78666396544458,71.7464029486563,
12.));
#159151=CARTESIAN_POINT('Ctrl Pts',(-4.7800826066665,71.769348677346,12.));
#159152=CARTESIAN_POINT('Ctrl Pts',(-4.77346700795792,71.7923289047643,
12.));
#159153=CARTESIAN_POINT('Ctrl Pts',(-4.76681714352502,71.8153434978923,
12.));
#159154=CARTESIAN_POINT('Ctrl Pts',(-4.7601329877742,71.8383923242531,12.));
#159155=CARTESIAN_POINT('Ctrl Pts',(-4.7534145153167,71.8614752519008,12.));
#159156=CARTESIAN_POINT('Ctrl Pts',(-4.74666170096547,71.8845921494189,
12.));
#159157=CARTESIAN_POINT('Ctrl Pts',(-4.73987451972864,71.9077428859212,
12.));
#159158=CARTESIAN_POINT('Ctrl Pts',(-4.73305294680785,71.9309273310471,
12.));
#159159=CARTESIAN_POINT('Ctrl Pts',(-4.72619695759774,71.9541453549579,
12.));
#159160=CARTESIAN_POINT('Ctrl Pts',(-4.7193065276907,71.9773968283259,12.));
#159161=CARTESIAN_POINT('Ctrl Pts',(-4.71238163287397,72.0006816223325,
12.));
#159162=CARTESIAN_POINT('Ctrl Pts',(-4.70542224912301,72.0239996086686,
12.));
#159163=CARTESIAN_POINT('Ctrl Pts',(-4.69842835259992,72.0473506595318,
12.));
#159164=CARTESIAN_POINT('Ctrl Pts',(-4.69139991965284,72.0707346476213,
12.));
#159165=CARTESIAN_POINT('Ctrl Pts',(-4.68433692682069,72.0941514461287,
12.));
#159166=CARTESIAN_POINT('Ctrl Pts',(-4.67723935083095,72.1176009287351,
12.));
#159167=CARTESIAN_POINT('Ctrl Pts',(-4.67010716859285,72.1410829696128,
12.));
#159168=CARTESIAN_POINT('Ctrl Pts',(-4.6629403571957,72.1645974434216,12.));
#159169=CARTESIAN_POINT('Ctrl Pts',(-4.65573889390822,72.1881442253053,
12.));
#159170=CARTESIAN_POINT('Ctrl Pts',(-4.64850275618323,72.2117231908822,
12.));
#159171=CARTESIAN_POINT('Ctrl Pts',(-4.64123192165628,72.2353342162417,
12.));
#159172=CARTESIAN_POINT('Ctrl Pts',(-4.63392636813844,72.2589771779456,
12.));
#159173=CARTESIAN_POINT('Ctrl Pts',(-4.62658607361466,72.2826519530259,
12.));
#159174=CARTESIAN_POINT('Ctrl Pts',(-4.61921101624292,72.3063584189807,
12.));
#159175=CARTESIAN_POINT('Ctrl Pts',(-4.61180117435862,72.3300964537658,
12.));
#159176=CARTESIAN_POINT('Ctrl Pts',(-4.60435652647453,72.3538659357913,
12.));
#159177=CARTESIAN_POINT('Ctrl Pts',(-4.5968770512733,72.3776667439227,12.));
#159178=CARTESIAN_POINT('Ctrl Pts',(-4.58936272760544,72.401498757478,12.));
#159179=CARTESIAN_POINT('Ctrl Pts',(-4.58181353448852,72.4253618562252,
12.));
#159180=CARTESIAN_POINT('Ctrl Pts',(-4.57422945111102,72.4492559203745,
12.));
#159181=CARTESIAN_POINT('Ctrl Pts',(-4.56661045683376,72.4731808305728,
12.));
#159182=CARTESIAN_POINT('Ctrl Pts',(-4.55895653118221,72.4971364679068,
12.));
#159183=CARTESIAN_POINT('Ctrl Pts',(-4.55126765384404,72.5211227139001,
12.));
#159184=CARTESIAN_POINT('Ctrl Pts',(-4.54354380466822,72.5451394505104,
12.));
#159185=CARTESIAN_POINT('Ctrl Pts',(-4.535784963668,72.5691865601223,12.));
#159186=CARTESIAN_POINT('Ctrl Pts',(-4.52799111102392,72.5932639255409,
12.));
#159187=CARTESIAN_POINT('Ctrl Pts',(-4.52016222707638,72.6173714299942,
12.));
#159188=CARTESIAN_POINT('Ctrl Pts',(-4.51229829232264,72.6415089571321,
12.));
#159189=CARTESIAN_POINT('Ctrl Pts',(-4.50439928741604,72.6656763910241,
12.));
#159190=CARTESIAN_POINT('Ctrl Pts',(-4.49646519316813,72.6898736161542,
12.));
#159191=CARTESIAN_POINT('Ctrl Pts',(-4.48849599055337,72.714100517414,12.));
#159192=CARTESIAN_POINT('Ctrl Pts',(-4.48049166070205,72.738356980103,12.));
#159193=CARTESIAN_POINT('Ctrl Pts',(-4.4724521848961,72.7626428899281,12.));
#159194=CARTESIAN_POINT('Ctrl Pts',(-4.46437754456793,72.7869581329994,
12.));
#159195=CARTESIAN_POINT('Ctrl Pts',(-4.45626772130146,72.8113025958262,
12.));
#159196=CARTESIAN_POINT('Ctrl Pts',(-4.44812269683738,72.8356761653069,
12.));
#159197=CARTESIAN_POINT('Ctrl Pts',(-4.43994245306818,72.8600787287318,
12.));
#159198=CARTESIAN_POINT('Ctrl Pts',(-4.43172697203349,72.8845101737855,
12.));
#159199=CARTESIAN_POINT('Ctrl Pts',(-4.42347623591942,72.9089703885462,
12.));
#159200=CARTESIAN_POINT('Ctrl Pts',(-4.41519022705921,72.9334592614829,
12.));
#159201=CARTESIAN_POINT('Ctrl Pts',(-4.40686892793957,72.95797668145,12.));
#159202=CARTESIAN_POINT('Ctrl Pts',(-4.39851232119722,72.9825225376846,
12.));
#159203=CARTESIAN_POINT('Ctrl Pts',(-4.39012038961139,73.007096719804,12.));
#159204=CARTESIAN_POINT('Ctrl Pts',(-4.38169311610151,73.0316991177993,
12.));
#159205=CARTESIAN_POINT('Ctrl Pts',(-4.37323048372607,73.0563296220299,
12.));
#159206=CARTESIAN_POINT('Ctrl Pts',(-4.36473247568641,73.0809881232103,
12.));
#159207=CARTESIAN_POINT('Ctrl Pts',(-4.3561990753272,73.1056745124087,12.));
#159208=CARTESIAN_POINT('Ctrl Pts',(-4.34763026613158,73.130388681059,12.));
#159209=CARTESIAN_POINT('Ctrl Pts',(-4.33902603172141,73.1551305209685,
12.));
#159210=CARTESIAN_POINT('Ctrl Pts',(-4.33038635585877,73.1798999243235,
12.));
#159211=CARTESIAN_POINT('Ctrl Pts',(-4.32171122245214,73.204696783694,12.));
#159212=CARTESIAN_POINT('Ctrl Pts',(-4.31300061556098,73.2295209920334,
12.));
#159213=CARTESIAN_POINT('Ctrl Pts',(-4.3042545193823,73.2543724426577,12.));
#159214=CARTESIAN_POINT('Ctrl Pts',(-4.29547291824287,73.2792510292254,
12.));
#159215=CARTESIAN_POINT('Ctrl Pts',(-4.28665579659301,73.3041566457135,
12.));
#159216=CARTESIAN_POINT('Ctrl Pts',(-4.2778031390039,73.3290891863949,12.));
#159217=CARTESIAN_POINT('Ctrl Pts',(-4.268914930167,73.3540485458065,12.));
#159218=CARTESIAN_POINT('Ctrl Pts',(-4.25999115489899,73.3790346187938,
12.));
#159219=CARTESIAN_POINT('Ctrl Pts',(-4.25103179814887,73.4040473005592,
12.));
#159220=CARTESIAN_POINT('Ctrl Pts',(-4.24203684500939,73.4290864867101,
12.));
#159221=CARTESIAN_POINT('Ctrl Pts',(-4.23300628072758,73.4541520732948,
12.));
#159222=CARTESIAN_POINT('Ctrl Pts',(-4.22394009072756,73.4792439568633,
12.));
#159223=CARTESIAN_POINT('Ctrl Pts',(-4.21483826059441,73.5043620344116,
12.));
#159224=CARTESIAN_POINT('Ctrl Pts',(-4.2057007760373,73.5295062032628,12.));
#159225=CARTESIAN_POINT('Ctrl Pts',(-4.19652762286127,73.5546763609572,
12.));
#159226=CARTESIAN_POINT('Ctrl Pts',(-4.18731878694236,73.5798724051519,
12.));
#159227=CARTESIAN_POINT('Ctrl Pts',(-4.17807425419813,73.6050942334768,
12.));
#159228=CARTESIAN_POINT('Ctrl Pts',(-4.1687940105878,73.6303417435251,12.));
#159229=CARTESIAN_POINT('Ctrl Pts',(-4.15947804217784,73.6556148331489,
12.));
#159230=CARTESIAN_POINT('Ctrl Pts',(-4.15012633519723,73.6809134006897,
12.));
#159231=CARTESIAN_POINT('Ctrl Pts',(-4.14073887610153,73.7062373452342,
12.));
#159232=CARTESIAN_POINT('Ctrl Pts',(-4.13131565163578,73.7315865668522,
12.));
#159233=CARTESIAN_POINT('Ctrl Pts',(-4.12185664890557,73.7569609668528,
12.));
#159234=CARTESIAN_POINT('Ctrl Pts',(-4.11236185522787,73.7823604472159,
12.));
#159235=CARTESIAN_POINT('Ctrl Pts',(-4.10283125798729,73.8077849100342,
12.));
#159236=CARTESIAN_POINT('Ctrl Pts',(-4.09326484448233,73.8332342568989,
12.));
#159237=CARTESIAN_POINT('Ctrl Pts',(-4.08366260180674,73.8587083884191,
12.));
#159238=CARTESIAN_POINT('Ctrl Pts',(-4.07402451665245,73.8842072034008,
12.));
#159239=CARTESIAN_POINT('Ctrl Pts',(-4.06435057547325,73.9097305995115,
12.));
#159240=CARTESIAN_POINT('Ctrl Pts',(-4.05464076484752,73.9352784747608,
12.));
#159241=CARTESIAN_POINT('Ctrl Pts',(-4.04489507179957,73.9608507287909,
12.));
#159242=CARTESIAN_POINT('Ctrl Pts',(-4.0351134841066,73.9864472641033,12.));
#159243=CARTESIAN_POINT('Ctrl Pts',(-4.02529599070095,74.012067987646,12.));
#159244=CARTESIAN_POINT('Ctrl Pts',(-4.01544258176711,74.0377128111863,
12.));
#159245=CARTESIAN_POINT('Ctrl Pts',(-4.00696550627365,74.0597159782109,
12.));
#159246=CARTESIAN_POINT('Ctrl Pts',(-4.00044689711984,74.0765982943677,
12.));
#159247=CARTESIAN_POINT('Ctrl Pts',(-3.99590266746992,74.0883491449954,
12.));
#159248=CARTESIAN_POINT('Ctrl Pts',(-3.99334334445529,74.0949615399619,
12.));
#159249=CARTESIAN_POINT('Ctrl Pts',(-3.99277406490873,74.0964320766207,
12.));
#159250=CARTESIAN_POINT('',(-5.24987136994591,69.8028570375098,0.));
#159251=CARTESIAN_POINT('',(-5.24987136994591,69.8028570375097,0.));
#159252=CARTESIAN_POINT('Ctrl Pts',(-3.99277406490868,74.0964320766208,
0.));
#159253=CARTESIAN_POINT('Ctrl Pts',(-3.99334334445525,74.094961539962,0.));
#159254=CARTESIAN_POINT('Ctrl Pts',(-3.99590266746989,74.0883491449955,
0.));
#159255=CARTESIAN_POINT('Ctrl Pts',(-4.00044689711982,74.0765982943677,
0.));
#159256=CARTESIAN_POINT('Ctrl Pts',(-4.00696550627364,74.059715978211,0.));
#159257=CARTESIAN_POINT('Ctrl Pts',(-4.01544258176711,74.0377128111863,
0.));
#159258=CARTESIAN_POINT('Ctrl Pts',(-4.02529599070095,74.012067987646,0.));
#159259=CARTESIAN_POINT('Ctrl Pts',(-4.0351134841066,73.9864472641033,0.));
#159260=CARTESIAN_POINT('Ctrl Pts',(-4.04489507179957,73.9608507287909,
0.));
#159261=CARTESIAN_POINT('Ctrl Pts',(-4.05464076484752,73.9352784747608,
0.));
#159262=CARTESIAN_POINT('Ctrl Pts',(-4.06435057547325,73.9097305995115,
0.));
#159263=CARTESIAN_POINT('Ctrl Pts',(-4.07402451665245,73.8842072034008,
0.));
#159264=CARTESIAN_POINT('Ctrl Pts',(-4.08366260180674,73.8587083884191,
0.));
#159265=CARTESIAN_POINT('Ctrl Pts',(-4.09326484448233,73.8332342568989,
0.));
#159266=CARTESIAN_POINT('Ctrl Pts',(-4.10283125798729,73.8077849100342,
0.));
#159267=CARTESIAN_POINT('Ctrl Pts',(-4.11236185522787,73.7823604472159,
0.));
#159268=CARTESIAN_POINT('Ctrl Pts',(-4.12185664890557,73.7569609668528,
0.));
#159269=CARTESIAN_POINT('Ctrl Pts',(-4.13131565163578,73.7315865668522,
0.));
#159270=CARTESIAN_POINT('Ctrl Pts',(-4.14073887610153,73.7062373452342,
0.));
#159271=CARTESIAN_POINT('Ctrl Pts',(-4.15012633519723,73.6809134006897,
0.));
#159272=CARTESIAN_POINT('Ctrl Pts',(-4.15947804217784,73.6556148331489,
0.));
#159273=CARTESIAN_POINT('Ctrl Pts',(-4.1687940105878,73.6303417435251,0.));
#159274=CARTESIAN_POINT('Ctrl Pts',(-4.17807425419813,73.6050942334768,
0.));
#159275=CARTESIAN_POINT('Ctrl Pts',(-4.18731878694236,73.5798724051519,
0.));
#159276=CARTESIAN_POINT('Ctrl Pts',(-4.19652762286127,73.5546763609572,
0.));
#159277=CARTESIAN_POINT('Ctrl Pts',(-4.2057007760373,73.5295062032628,0.));
#159278=CARTESIAN_POINT('Ctrl Pts',(-4.21483826059441,73.5043620344116,
0.));
#159279=CARTESIAN_POINT('Ctrl Pts',(-4.22394009072756,73.4792439568633,
0.));
#159280=CARTESIAN_POINT('Ctrl Pts',(-4.23300628072758,73.4541520732948,
0.));
#159281=CARTESIAN_POINT('Ctrl Pts',(-4.24203684500939,73.4290864867101,
0.));
#159282=CARTESIAN_POINT('Ctrl Pts',(-4.25103179814887,73.4040473005592,
0.));
#159283=CARTESIAN_POINT('Ctrl Pts',(-4.25999115489899,73.3790346187938,
0.));
#159284=CARTESIAN_POINT('Ctrl Pts',(-4.268914930167,73.3540485458065,0.));
#159285=CARTESIAN_POINT('Ctrl Pts',(-4.2778031390039,73.3290891863949,0.));
#159286=CARTESIAN_POINT('Ctrl Pts',(-4.28665579659301,73.3041566457135,
0.));
#159287=CARTESIAN_POINT('Ctrl Pts',(-4.29547291824287,73.2792510292254,
0.));
#159288=CARTESIAN_POINT('Ctrl Pts',(-4.3042545193823,73.2543724426577,0.));
#159289=CARTESIAN_POINT('Ctrl Pts',(-4.31300061556098,73.2295209920334,
0.));
#159290=CARTESIAN_POINT('Ctrl Pts',(-4.32171122245214,73.204696783694,0.));
#159291=CARTESIAN_POINT('Ctrl Pts',(-4.33038635585877,73.1798999243235,
0.));
#159292=CARTESIAN_POINT('Ctrl Pts',(-4.33902603172141,73.1551305209685,
0.));
#159293=CARTESIAN_POINT('Ctrl Pts',(-4.34763026613158,73.130388681059,0.));
#159294=CARTESIAN_POINT('Ctrl Pts',(-4.3561990753272,73.1056745124087,0.));
#159295=CARTESIAN_POINT('Ctrl Pts',(-4.36473247568641,73.0809881232103,
0.));
#159296=CARTESIAN_POINT('Ctrl Pts',(-4.37323048372607,73.0563296220299,
0.));
#159297=CARTESIAN_POINT('Ctrl Pts',(-4.38169311610151,73.0316991177993,
0.));
#159298=CARTESIAN_POINT('Ctrl Pts',(-4.39012038961139,73.007096719804,0.));
#159299=CARTESIAN_POINT('Ctrl Pts',(-4.39851232119722,72.9825225376846,
0.));
#159300=CARTESIAN_POINT('Ctrl Pts',(-4.40686892793957,72.95797668145,0.));
#159301=CARTESIAN_POINT('Ctrl Pts',(-4.41519022705921,72.9334592614829,
0.));
#159302=CARTESIAN_POINT('Ctrl Pts',(-4.42347623591942,72.9089703885462,
0.));
#159303=CARTESIAN_POINT('Ctrl Pts',(-4.43172697203349,72.8845101737855,
0.));
#159304=CARTESIAN_POINT('Ctrl Pts',(-4.43994245306818,72.8600787287318,
0.));
#159305=CARTESIAN_POINT('Ctrl Pts',(-4.44812269683738,72.8356761653069,
0.));
#159306=CARTESIAN_POINT('Ctrl Pts',(-4.45626772130146,72.8113025958262,
0.));
#159307=CARTESIAN_POINT('Ctrl Pts',(-4.46437754456793,72.7869581329994,
0.));
#159308=CARTESIAN_POINT('Ctrl Pts',(-4.4724521848961,72.7626428899281,0.));
#159309=CARTESIAN_POINT('Ctrl Pts',(-4.48049166070205,72.738356980103,0.));
#159310=CARTESIAN_POINT('Ctrl Pts',(-4.48849599055337,72.714100517414,0.));
#159311=CARTESIAN_POINT('Ctrl Pts',(-4.49646519316813,72.6898736161542,
0.));
#159312=CARTESIAN_POINT('Ctrl Pts',(-4.50439928741604,72.6656763910241,
0.));
#159313=CARTESIAN_POINT('Ctrl Pts',(-4.51229829232264,72.6415089571321,
0.));
#159314=CARTESIAN_POINT('Ctrl Pts',(-4.52016222707638,72.6173714299942,
0.));
#159315=CARTESIAN_POINT('Ctrl Pts',(-4.52799111102392,72.5932639255409,
0.));
#159316=CARTESIAN_POINT('Ctrl Pts',(-4.535784963668,72.5691865601223,0.));
#159317=CARTESIAN_POINT('Ctrl Pts',(-4.54354380466822,72.5451394505104,
0.));
#159318=CARTESIAN_POINT('Ctrl Pts',(-4.55126765384404,72.5211227139001,
0.));
#159319=CARTESIAN_POINT('Ctrl Pts',(-4.55895653118221,72.4971364679068,
0.));
#159320=CARTESIAN_POINT('Ctrl Pts',(-4.56661045683376,72.4731808305728,
0.));
#159321=CARTESIAN_POINT('Ctrl Pts',(-4.57422945111102,72.4492559203745,
0.));
#159322=CARTESIAN_POINT('Ctrl Pts',(-4.58181353448852,72.4253618562252,
0.));
#159323=CARTESIAN_POINT('Ctrl Pts',(-4.58936272760544,72.401498757478,0.));
#159324=CARTESIAN_POINT('Ctrl Pts',(-4.5968770512733,72.3776667439227,0.));
#159325=CARTESIAN_POINT('Ctrl Pts',(-4.60435652647453,72.3538659357913,
0.));
#159326=CARTESIAN_POINT('Ctrl Pts',(-4.61180117435862,72.3300964537658,
0.));
#159327=CARTESIAN_POINT('Ctrl Pts',(-4.61921101624292,72.3063584189807,
0.));
#159328=CARTESIAN_POINT('Ctrl Pts',(-4.62658607361466,72.2826519530259,
0.));
#159329=CARTESIAN_POINT('Ctrl Pts',(-4.63392636813844,72.2589771779456,
0.));
#159330=CARTESIAN_POINT('Ctrl Pts',(-4.64123192165628,72.2353342162417,
0.));
#159331=CARTESIAN_POINT('Ctrl Pts',(-4.64850275618323,72.2117231908822,
0.));
#159332=CARTESIAN_POINT('Ctrl Pts',(-4.65573889390822,72.1881442253053,
0.));
#159333=CARTESIAN_POINT('Ctrl Pts',(-4.6629403571957,72.1645974434216,0.));
#159334=CARTESIAN_POINT('Ctrl Pts',(-4.67010716859285,72.1410829696128,
0.));
#159335=CARTESIAN_POINT('Ctrl Pts',(-4.67723935083095,72.1176009287351,
0.));
#159336=CARTESIAN_POINT('Ctrl Pts',(-4.68433692682069,72.0941514461287,
0.));
#159337=CARTESIAN_POINT('Ctrl Pts',(-4.69139991965284,72.0707346476213,
0.));
#159338=CARTESIAN_POINT('Ctrl Pts',(-4.69842835259992,72.0473506595318,
0.));
#159339=CARTESIAN_POINT('Ctrl Pts',(-4.70542224912301,72.0239996086686,
0.));
#159340=CARTESIAN_POINT('Ctrl Pts',(-4.71238163287397,72.0006816223325,
0.));
#159341=CARTESIAN_POINT('Ctrl Pts',(-4.7193065276907,71.9773968283259,0.));
#159342=CARTESIAN_POINT('Ctrl Pts',(-4.72619695759774,71.9541453549579,
0.));
#159343=CARTESIAN_POINT('Ctrl Pts',(-4.73305294680785,71.9309273310471,
0.));
#159344=CARTESIAN_POINT('Ctrl Pts',(-4.73987451972864,71.9077428859212,
0.));
#159345=CARTESIAN_POINT('Ctrl Pts',(-4.74666170096547,71.8845921494189,
0.));
#159346=CARTESIAN_POINT('Ctrl Pts',(-4.7534145153167,71.8614752519008,0.));
#159347=CARTESIAN_POINT('Ctrl Pts',(-4.7601329877742,71.8383923242531,0.));
#159348=CARTESIAN_POINT('Ctrl Pts',(-4.76681714352502,71.8153434978923,
0.));
#159349=CARTESIAN_POINT('Ctrl Pts',(-4.77346700795792,71.7923289047643,
0.));
#159350=CARTESIAN_POINT('Ctrl Pts',(-4.7800826066665,71.769348677346,0.));
#159351=CARTESIAN_POINT('Ctrl Pts',(-4.78666396544458,71.7464029486563,
0.));
#159352=CARTESIAN_POINT('Ctrl Pts',(-4.79321111028676,71.723491852261,0.));
#159353=CARTESIAN_POINT('Ctrl Pts',(-4.79972406739011,71.7006155222764,
0.));
#159354=CARTESIAN_POINT('Ctrl Pts',(-4.80620286316075,71.6777740933687,
0.));
#159355=CARTESIAN_POINT('Ctrl Pts',(-4.81264752421713,71.6549677007582,
0.));
#159356=CARTESIAN_POINT('Ctrl Pts',(-4.81905807738542,71.6321964802297,
0.));
#159357=CARTESIAN_POINT('Ctrl Pts',(-4.82543454970021,71.6094605681353,
0.));
#159358=CARTESIAN_POINT('Ctrl Pts',(-4.8317769684064,71.5867601014008,0.));
#159359=CARTESIAN_POINT('Ctrl Pts',(-4.83808536096589,71.5640952175239,
0.));
#159360=CARTESIAN_POINT('Ctrl Pts',(-4.84435975506056,71.5414660545778,
0.));
#159361=CARTESIAN_POINT('Ctrl Pts',(-4.85060017858786,71.5188727512231,
0.));
#159362=CARTESIAN_POINT('Ctrl Pts',(-4.85680665966184,71.4963154467128,
0.));
#159363=CARTESIAN_POINT('Ctrl Pts',(-4.86297922661499,71.4737942808971,
0.));
#159364=CARTESIAN_POINT('Ctrl Pts',(-4.86911790800533,71.4513093942216,
0.));
#159365=CARTESIAN_POINT('Ctrl Pts',(-4.87522273261881,71.4288609277324,
0.));
#159366=CARTESIAN_POINT('Ctrl Pts',(-4.88129372946524,71.4064490230857,
0.));
#159367=CARTESIAN_POINT('Ctrl Pts',(-4.88733092777964,71.3840738225547,
0.));
#159368=CARTESIAN_POINT('Ctrl Pts',(-4.89333435702424,71.3617354690342,
0.));
#159369=CARTESIAN_POINT('Ctrl Pts',(-4.89930404689599,71.3394341060396,
0.));
#159370=CARTESIAN_POINT('Ctrl Pts',(-4.90524002732806,71.3171698777124,
0.));
#159371=CARTESIAN_POINT('Ctrl Pts',(-4.91114232848623,71.2949429288319,
0.));
#159372=CARTESIAN_POINT('Ctrl Pts',(-4.91701098077041,71.27275340482,0.));
#159373=CARTESIAN_POINT('Ctrl Pts',(-4.9228460148171,71.2506014517457,0.));
#159374=CARTESIAN_POINT('Ctrl Pts',(-4.92864746150711,71.2284872163248,
0.));
#159375=CARTESIAN_POINT('Ctrl Pts',(-4.93441535196594,71.206410845926,0.));
#159376=CARTESIAN_POINT('Ctrl Pts',(-4.94014971756097,71.184372488583,0.));
#159377=CARTESIAN_POINT('Ctrl Pts',(-4.94585058990337,71.1623722929998,
0.));
#159378=CARTESIAN_POINT('Ctrl Pts',(-4.95151800085111,71.1404104085561,
0.));
#159379=CARTESIAN_POINT('Ctrl Pts',(-4.95715198251704,71.1184869853071,
0.));
#159380=CARTESIAN_POINT('Ctrl Pts',(-4.96275256726787,71.0966021739922,
0.));
#159381=CARTESIAN_POINT('Ctrl Pts',(-4.96831978772201,71.0747561260443,
0.));
#159382=CARTESIAN_POINT('Ctrl Pts',(-4.97385367675157,71.0529489935959,
0.));
#159383=CARTESIAN_POINT('Ctrl Pts',(-4.97935426748577,71.031180929482,0.));
#159384=CARTESIAN_POINT('Ctrl Pts',(-4.98482159331851,71.0094520872375,
0.));
#159385=CARTESIAN_POINT('Ctrl Pts',(-4.99025568790653,70.9877626211112,
0.));
#159386=CARTESIAN_POINT('Ctrl Pts',(-4.99565658516906,70.9661126860773,
0.));
#159387=CARTESIAN_POINT('Ctrl Pts',(-5.00102431929039,70.9445024378439,
0.));
#159388=CARTESIAN_POINT('Ctrl Pts',(-5.00635892472518,70.9229320328588,
0.));
#159389=CARTESIAN_POINT('Ctrl Pts',(-5.01166043620573,70.9014016283123,
0.));
#159390=CARTESIAN_POINT('Ctrl Pts',(-5.01692888873793,70.8799113821449,
0.));
#159391=CARTESIAN_POINT('Ctrl Pts',(-5.0221643176006,70.8584614530517,0.));
#159392=CARTESIAN_POINT('Ctrl Pts',(-5.02736675834691,70.8370520004844,
0.));
#159393=CARTESIAN_POINT('Ctrl Pts',(-5.03253624680941,70.8156831846494,
0.));
#159394=CARTESIAN_POINT('Ctrl Pts',(-5.03767281910483,70.7943551665071,
0.));
#159395=CARTESIAN_POINT('Ctrl Pts',(-5.04277651163356,70.7730681077997,
0.));
#159396=CARTESIAN_POINT('Ctrl Pts',(-5.04784736108351,70.7518221710715,
0.));
#159397=CARTESIAN_POINT('Ctrl Pts',(-5.05288540443478,70.7306175196856,
0.));
#159398=CARTESIAN_POINT('Ctrl Pts',(-5.05789067897041,70.7094543178416,
0.));
#159399=CARTESIAN_POINT('Ctrl Pts',(-5.06286322227797,70.6883327305755,
0.));
#159400=CARTESIAN_POINT('Ctrl Pts',(-5.06780307224053,70.6672529237431,
0.));
#159401=CARTESIAN_POINT('Ctrl Pts',(-5.0727102670335,70.6462150640009,0.));
#159402=CARTESIAN_POINT('Ctrl Pts',(-5.0775848451231,70.6252193187892,0.));
#159403=CARTESIAN_POINT('Ctrl Pts',(-5.08242684526704,70.6042658562951,
0.));
#159404=CARTESIAN_POINT('Ctrl Pts',(-5.08723630652291,70.5833548455043,
0.));
#159405=CARTESIAN_POINT('Ctrl Pts',(-5.09201326826146,70.5624864562841,
0.));
#159406=CARTESIAN_POINT('Ctrl Pts',(-5.09675777018182,70.5416608594526,
0.));
#159407=CARTESIAN_POINT('Ctrl Pts',(-5.10146985232928,70.5208782268482,
0.));
#159408=CARTESIAN_POINT('Ctrl Pts',(-5.10614955511643,70.5001387313963,
0.));
#159409=CARTESIAN_POINT('Ctrl Pts',(-5.11079691929193,70.4794425469799,
0.));
#159410=CARTESIAN_POINT('Ctrl Pts',(-5.1154119859092,70.4587898482946,0.));
#159411=CARTESIAN_POINT('Ctrl Pts',(-5.11999479630215,70.438180810725,0.));
#159412=CARTESIAN_POINT('Ctrl Pts',(-5.12454539205347,70.4176156101633,
0.));
#159413=CARTESIAN_POINT('Ctrl Pts',(-5.12906381499486,70.3970944229885,
0.));
#159414=CARTESIAN_POINT('Ctrl Pts',(-5.13355010728591,70.3766174264786,
0.));
#159415=CARTESIAN_POINT('Ctrl Pts',(-5.13800431148911,70.3561847991725,
0.));
#159416=CARTESIAN_POINT('Ctrl Pts',(-5.14242647063467,70.3357967211782,
0.));
#159417=CARTESIAN_POINT('Ctrl Pts',(-5.14681662833054,70.31545337467,0.));
#159418=CARTESIAN_POINT('Ctrl Pts',(-5.15117482869224,70.2951549435469,
0.));
#159419=CARTESIAN_POINT('Ctrl Pts',(-5.15550111614838,70.2749016125073,
0.));
#159420=CARTESIAN_POINT('Ctrl Pts',(-5.159795535282,70.2546935662719,0.));
#159421=CARTESIAN_POINT('Ctrl Pts',(-5.16405813066994,70.2345309887864,
0.));
#159422=CARTESIAN_POINT('Ctrl Pts',(-5.1682889467014,70.2144140623004,0.));
#159423=CARTESIAN_POINT('Ctrl Pts',(-5.1724880279342,70.1943429691214,0.));
#159424=CARTESIAN_POINT('Ctrl Pts',(-5.176655419524,70.1743178937102,0.));
#159425=CARTESIAN_POINT('Ctrl Pts',(-5.18079116757659,70.1543390243882,
0.));
#159426=CARTESIAN_POINT('Ctrl Pts',(-5.18489531966234,70.1344065558106,
0.));
#159427=CARTESIAN_POINT('Ctrl Pts',(-5.18896792486523,70.1145206891833,
0.));
#159428=CARTESIAN_POINT('Ctrl Pts',(-5.19300903271544,70.0946816270957,
0.));
#159429=CARTESIAN_POINT('Ctrl Pts',(-5.19701869225514,70.0748895689716,
0.));
#159430=CARTESIAN_POINT('Ctrl Pts',(-5.20099695122677,70.0551447071106,
0.));
#159431=CARTESIAN_POINT('Ctrl Pts',(-5.20494385478083,70.0354472203604,
0.));
#159432=CARTESIAN_POINT('Ctrl Pts',(-5.20885944672914,70.0157972802255,
0.));
#159433=CARTESIAN_POINT('Ctrl Pts',(-5.21274377203321,69.996195063002,0.));
#159434=CARTESIAN_POINT('Ctrl Pts',(-5.21659687881139,69.9766407595385,
0.));
#159435=CARTESIAN_POINT('Ctrl Pts',(-5.22041882075627,69.9571345869996,
0.));
#159436=CARTESIAN_POINT('Ctrl Pts',(-5.22420965879808,69.9376767968951,
0.));
#159437=CARTESIAN_POINT('Ctrl Pts',(-5.22796945602603,69.9182676501892,
0.));
#159438=CARTESIAN_POINT('Ctrl Pts',(-5.23169827290452,69.8989073936606,
0.));
#159439=CARTESIAN_POINT('Ctrl Pts',(-5.23539616279715,69.8795962381676,
0.));
#159440=CARTESIAN_POINT('Ctrl Pts',(-5.23906316635141,69.8603343303016,
0.));
#159441=CARTESIAN_POINT('Ctrl Pts',(-5.24269931055075,69.8411217507931,
0.));
#159442=CARTESIAN_POINT('Ctrl Pts',(-5.2455835516022,69.8257911792542,0.));
#159443=CARTESIAN_POINT('Ctrl Pts',(-5.24773285666673,69.8143154684447,
0.));
#159444=CARTESIAN_POINT('Ctrl Pts',(-5.24915955997537,69.8066748687863,
0.));
#159445=CARTESIAN_POINT('Ctrl Pts',(-5.24987136994591,69.8028570375098,
0.));
#159446=CARTESIAN_POINT('Ctrl Pts',(2.62535189104657,74.4537274248118,0.));
#159447=CARTESIAN_POINT('Ctrl Pts',(2.62535189104657,74.4537274248118,12.));
#159448=CARTESIAN_POINT('Ctrl Pts',(2.62283178248298,74.4487312586601,0.));
#159449=CARTESIAN_POINT('Ctrl Pts',(2.62283178248298,74.4487312586601,12.));
#159450=CARTESIAN_POINT('Ctrl Pts',(2.61779535432371,74.4387409032582,0.));
#159451=CARTESIAN_POINT('Ctrl Pts',(2.61779535432371,74.4387409032582,12.));
#159452=CARTESIAN_POINT('Ctrl Pts',(2.61025207898832,74.4237613008609,0.));
#159453=CARTESIAN_POINT('Ctrl Pts',(2.61025207898832,74.4237613008609,12.));
#159454=CARTESIAN_POINT('Ctrl Pts',(2.60021711327492,74.4038003595514,0.));
#159455=CARTESIAN_POINT('Ctrl Pts',(2.60021711327492,74.4038003595514,12.));
#159456=CARTESIAN_POINT('Ctrl Pts',(2.5877113026862,74.3788689604,0.));
#159457=CARTESIAN_POINT('Ctrl Pts',(2.5877113026862,74.3788689604,12.));
#159458=CARTESIAN_POINT('Ctrl Pts',(2.57524339541658,74.3539573568054,0.));
#159459=CARTESIAN_POINT('Ctrl Pts',(2.57524339541658,74.3539573568054,12.));
#159460=CARTESIAN_POINT('Ctrl Pts',(2.56281339800083,74.3290655814922,0.));
#159461=CARTESIAN_POINT('Ctrl Pts',(2.56281339800083,74.3290655814922,12.));
#159462=CARTESIAN_POINT('Ctrl Pts',(2.55042131526685,74.3041936853329,0.));
#159463=CARTESIAN_POINT('Ctrl Pts',(2.55042131526685,74.3041936853329,12.));
#159464=CARTESIAN_POINT('Ctrl Pts',(2.53806714838104,74.2793417427044,0.));
#159465=CARTESIAN_POINT('Ctrl Pts',(2.53806714838104,74.2793417427044,12.));
#159466=CARTESIAN_POINT('Ctrl Pts',(2.52575089478113,74.2545098494549,0.));
#159467=CARTESIAN_POINT('Ctrl Pts',(2.52575089478113,74.2545098494549,12.));
#159468=CARTESIAN_POINT('Ctrl Pts',(2.51347254956027,74.2296981152027,0.));
#159469=CARTESIAN_POINT('Ctrl Pts',(2.51347254956027,74.2296981152027,12.));
#159470=CARTESIAN_POINT('Ctrl Pts',(2.50123210644075,74.2049066571942,0.));
#159471=CARTESIAN_POINT('Ctrl Pts',(2.50123210644075,74.2049066571942,12.));
#159472=CARTESIAN_POINT('Ctrl Pts',(2.48902955888402,74.180135593693,0.));
#159473=CARTESIAN_POINT('Ctrl Pts',(2.48902955888402,74.180135593693,12.));
#159474=CARTESIAN_POINT('Ctrl Pts',(2.47686490120424,74.1553850371577,0.));
#159475=CARTESIAN_POINT('Ctrl Pts',(2.47686490120424,74.1553850371577,12.));
#159476=CARTESIAN_POINT('Ctrl Pts',(2.46473812948049,74.1306550887196,0.));
#159477=CARTESIAN_POINT('Ctrl Pts',(2.46473812948049,74.1306550887196,12.));
#159478=CARTESIAN_POINT('Ctrl Pts',(2.45264924094853,74.1059458420175,0.));
#159479=CARTESIAN_POINT('Ctrl Pts',(2.45264924094853,74.1059458420175,12.));
#159480=CARTESIAN_POINT('Ctrl Pts',(2.44059823356722,74.0812573859474,0.));
#159481=CARTESIAN_POINT('Ctrl Pts',(2.44059823356722,74.0812573859474,12.));
#159482=CARTESIAN_POINT('Ctrl Pts',(2.42858510549787,74.0565898079227,0.));
#159483=CARTESIAN_POINT('Ctrl Pts',(2.42858510549787,74.0565898079227,12.));
#159484=CARTESIAN_POINT('Ctrl Pts',(2.41660985465229,74.0319431966956,0.));
#159485=CARTESIAN_POINT('Ctrl Pts',(2.41660985465229,74.0319431966956,12.));
#159486=CARTESIAN_POINT('Ctrl Pts',(2.40467247811497,74.0073176459287,0.));
#159487=CARTESIAN_POINT('Ctrl Pts',(2.40467247811497,74.0073176459287,12.));
#159488=CARTESIAN_POINT('Ctrl Pts',(2.39277297220717,73.9827132538149,0.));
#159489=CARTESIAN_POINT('Ctrl Pts',(2.39277297220717,73.9827132538149,12.));
#159490=CARTESIAN_POINT('Ctrl Pts',(2.38091133274933,73.9581301214609,0.));
#159491=CARTESIAN_POINT('Ctrl Pts',(2.38091133274933,73.9581301214609,12.));
#159492=CARTESIAN_POINT('Ctrl Pts',(2.36908755525995,73.9335683516388,0.));
#159493=CARTESIAN_POINT('Ctrl Pts',(2.36908755525995,73.9335683516388,12.));
#159494=CARTESIAN_POINT('Ctrl Pts',(2.35730163516325,73.9090280474723,0.));
#159495=CARTESIAN_POINT('Ctrl Pts',(2.35730163516325,73.9090280474723,12.));
#159496=CARTESIAN_POINT('Ctrl Pts',(2.34555356802141,73.8845093109302,0.));
#159497=CARTESIAN_POINT('Ctrl Pts',(2.34555356802141,73.8845093109302,12.));
#159498=CARTESIAN_POINT('Ctrl Pts',(2.33384334963981,73.8600122421502,0.));
#159499=CARTESIAN_POINT('Ctrl Pts',(2.33384334963981,73.8600122421502,12.));
#159500=CARTESIAN_POINT('Ctrl Pts',(2.32217097594216,73.8355369402733,0.));
#159501=CARTESIAN_POINT('Ctrl Pts',(2.32217097594216,73.8355369402733,12.));
#159502=CARTESIAN_POINT('Ctrl Pts',(2.31053644289426,73.8110835039341,0.));
#159503=CARTESIAN_POINT('Ctrl Pts',(2.31053644289426,73.8110835039341,12.));
#159504=CARTESIAN_POINT('Ctrl Pts',(2.29893974640436,73.7866520318849,0.));
#159505=CARTESIAN_POINT('Ctrl Pts',(2.29893974640436,73.7866520318849,12.));
#159506=CARTESIAN_POINT('Ctrl Pts',(2.28738088222859,73.7622426235648,0.));
#159507=CARTESIAN_POINT('Ctrl Pts',(2.28738088222859,73.7622426235648,12.));
#159508=CARTESIAN_POINT('Ctrl Pts',(2.27585984587193,73.7378553796792,0.));
#159509=CARTESIAN_POINT('Ctrl Pts',(2.27585984587193,73.7378553796792,12.));
#159510=CARTESIAN_POINT('Ctrl Pts',(2.26437663263664,73.7134904019378,0.));
#159511=CARTESIAN_POINT('Ctrl Pts',(2.26437663263664,73.7134904019378,12.));
#159512=CARTESIAN_POINT('Ctrl Pts',(2.25293123766425,73.6891477928124,0.));
#159513=CARTESIAN_POINT('Ctrl Pts',(2.25293123766425,73.6891477928124,12.));
#159514=CARTESIAN_POINT('Ctrl Pts',(2.241523655977,73.6648276552766,0.));
#159515=CARTESIAN_POINT('Ctrl Pts',(2.241523655977,73.6648276552766,12.));
#159516=CARTESIAN_POINT('Ctrl Pts',(2.2301538825129,73.6405300925714,0.));
#159517=CARTESIAN_POINT('Ctrl Pts',(2.2301538825129,73.6405300925714,12.));
#159518=CARTESIAN_POINT('Ctrl Pts',(2.21882191216522,73.6162552079044,0.));
#159519=CARTESIAN_POINT('Ctrl Pts',(2.21882191216522,73.6162552079044,12.));
#159520=CARTESIAN_POINT('Ctrl Pts',(2.20752773978354,73.5920031044604,0.));
#159521=CARTESIAN_POINT('Ctrl Pts',(2.20752773978354,73.5920031044604,12.));
#159522=CARTESIAN_POINT('Ctrl Pts',(2.19627136015683,73.5677738855461,0.));
#159523=CARTESIAN_POINT('Ctrl Pts',(2.19627136015683,73.5677738855461,12.));
#159524=CARTESIAN_POINT('Ctrl Pts',(2.18505276799757,73.5435676546934,0.));
#159525=CARTESIAN_POINT('Ctrl Pts',(2.18505276799757,73.5435676546934,12.));
#159526=CARTESIAN_POINT('Ctrl Pts',(2.17387195792306,73.5193845157705,0.));
#159527=CARTESIAN_POINT('Ctrl Pts',(2.17387195792306,73.5193845157705,12.));
#159528=CARTESIAN_POINT('Ctrl Pts',(2.16272892442916,73.4952245731044,0.));
#159529=CARTESIAN_POINT('Ctrl Pts',(2.16272892442916,73.4952245731044,12.));
#159530=CARTESIAN_POINT('Ctrl Pts',(2.151623661879,73.4710879315367,0.));
#159531=CARTESIAN_POINT('Ctrl Pts',(2.151623661879,73.4710879315367,12.));
#159532=CARTESIAN_POINT('Ctrl Pts',(2.14055616452049,73.4469746963622,0.));
#159533=CARTESIAN_POINT('Ctrl Pts',(2.14055616452049,73.4469746963622,12.));
#159534=CARTESIAN_POINT('Ctrl Pts',(2.12952642649361,73.4228849732915,0.));
#159535=CARTESIAN_POINT('Ctrl Pts',(2.12952642649361,73.4228849732915,12.));
#159536=CARTESIAN_POINT('Ctrl Pts',(2.11853444183764,73.3988188684022,0.));
#159537=CARTESIAN_POINT('Ctrl Pts',(2.11853444183764,73.3988188684022,12.));
#159538=CARTESIAN_POINT('Ctrl Pts',(2.10758020449401,73.3747764880903,0.));
#159539=CARTESIAN_POINT('Ctrl Pts',(2.10758020449401,73.3747764880903,12.));
#159540=CARTESIAN_POINT('Ctrl Pts',(2.09666370830734,73.3507579390254,0.));
#159541=CARTESIAN_POINT('Ctrl Pts',(2.09666370830734,73.3507579390254,12.));
#159542=CARTESIAN_POINT('Ctrl Pts',(2.08578494702762,73.3267633281822,0.));
#159543=CARTESIAN_POINT('Ctrl Pts',(2.08578494702762,73.3267633281822,12.));
#159544=CARTESIAN_POINT('Ctrl Pts',(2.07494391430955,73.3027927628636,0.));
#159545=CARTESIAN_POINT('Ctrl Pts',(2.07494391430955,73.3027927628636,12.));
#159546=CARTESIAN_POINT('Ctrl Pts',(2.06414060370838,73.2788463507248,0.));
#159547=CARTESIAN_POINT('Ctrl Pts',(2.06414060370838,73.2788463507248,12.));
#159548=CARTESIAN_POINT('Ctrl Pts',(2.05337500867396,73.2549241997946,0.));
#159549=CARTESIAN_POINT('Ctrl Pts',(2.05337500867396,73.2549241997946,12.));
#159550=CARTESIAN_POINT('Ctrl Pts',(2.04264712253916,73.2310264184965,0.));
#159551=CARTESIAN_POINT('Ctrl Pts',(2.04264712253916,73.2310264184965,12.));
#159552=CARTESIAN_POINT('Ctrl Pts',(2.03195693852441,73.2071531156492,0.));
#159553=CARTESIAN_POINT('Ctrl Pts',(2.03195693852441,73.2071531156492,12.));
#159554=CARTESIAN_POINT('Ctrl Pts',(2.02130444974352,73.1833044004612,0.));
#159555=CARTESIAN_POINT('Ctrl Pts',(2.02130444974352,73.1833044004612,12.));
#159556=CARTESIAN_POINT('Ctrl Pts',(2.01068964920465,73.159480382525,0.));
#159557=CARTESIAN_POINT('Ctrl Pts',(2.01068964920465,73.159480382525,12.));
#159558=CARTESIAN_POINT('Ctrl Pts',(2.00011252980988,73.1356811718094,0.));
#159559=CARTESIAN_POINT('Ctrl Pts',(2.00011252980988,73.1356811718094,12.));
#159560=CARTESIAN_POINT('Ctrl Pts',(1.98957308434931,73.1119068786482,0.));
#159561=CARTESIAN_POINT('Ctrl Pts',(1.98957308434931,73.1119068786482,12.));
#159562=CARTESIAN_POINT('Ctrl Pts',(1.97907130550173,73.0881576137415,0.));
#159563=CARTESIAN_POINT('Ctrl Pts',(1.97907130550173,73.0881576137415,12.));
#159564=CARTESIAN_POINT('Ctrl Pts',(1.96860718583945,73.0644334881679,0.));
#159565=CARTESIAN_POINT('Ctrl Pts',(1.96860718583945,73.0644334881679,12.));
#159566=CARTESIAN_POINT('Ctrl Pts',(1.95818071782774,73.0407346133912,0.));
#159567=CARTESIAN_POINT('Ctrl Pts',(1.95818071782774,73.0407346133912,12.));
#159568=CARTESIAN_POINT('Ctrl Pts',(1.94779189382301,73.0170611012659,0.));
#159569=CARTESIAN_POINT('Ctrl Pts',(1.94779189382301,73.0170611012659,12.));
#159570=CARTESIAN_POINT('Ctrl Pts',(1.93744070606558,72.9934130640414,0.));
#159571=CARTESIAN_POINT('Ctrl Pts',(1.93744070606558,72.9934130640414,12.));
#159572=CARTESIAN_POINT('Ctrl Pts',(1.92712714667649,72.9697906143638,0.));
#159573=CARTESIAN_POINT('Ctrl Pts',(1.92712714667649,72.9697906143638,12.));
#159574=CARTESIAN_POINT('Ctrl Pts',(1.91685120766428,72.9461938652816,0.));
#159575=CARTESIAN_POINT('Ctrl Pts',(1.91685120766428,72.9461938652816,12.));
#159576=CARTESIAN_POINT('Ctrl Pts',(1.90661288092583,72.9226229302483,0.));
#159577=CARTESIAN_POINT('Ctrl Pts',(1.90661288092583,72.9226229302483,12.));
#159578=CARTESIAN_POINT('Ctrl Pts',(1.89641215824585,72.8990779231226,0.));
#159579=CARTESIAN_POINT('Ctrl Pts',(1.89641215824585,72.8990779231226,12.));
#159580=CARTESIAN_POINT('Ctrl Pts',(1.88624903129196,72.8755589581674,0.));
#159581=CARTESIAN_POINT('Ctrl Pts',(1.88624903129196,72.8755589581674,12.));
#159582=CARTESIAN_POINT('Ctrl Pts',(1.87612349160953,72.8520661500465,0.));
#159583=CARTESIAN_POINT('Ctrl Pts',(1.87612349160953,72.8520661500465,12.));
#159584=CARTESIAN_POINT('Ctrl Pts',(1.86603553062777,72.8285996138346,0.));
#159585=CARTESIAN_POINT('Ctrl Pts',(1.86603553062777,72.8285996138346,12.));
#159586=CARTESIAN_POINT('Ctrl Pts',(1.85598513966116,72.8051594650214,0.));
#159587=CARTESIAN_POINT('Ctrl Pts',(1.85598513966116,72.8051594650214,12.));
#159588=CARTESIAN_POINT('Ctrl Pts',(1.84597230990859,72.7817458195155,0.));
#159589=CARTESIAN_POINT('Ctrl Pts',(1.84597230990859,72.7817458195155,12.));
#159590=CARTESIAN_POINT('Ctrl Pts',(1.83599703244927,72.7583587936454,0.));
#159591=CARTESIAN_POINT('Ctrl Pts',(1.83599703244927,72.7583587936454,12.));
#159592=CARTESIAN_POINT('Ctrl Pts',(1.82605929823566,72.73499850416,0.));
#159593=CARTESIAN_POINT('Ctrl Pts',(1.82605929823566,72.73499850416,12.));
#159594=CARTESIAN_POINT('Ctrl Pts',(1.81615909809873,72.7116650682347,0.));
#159595=CARTESIAN_POINT('Ctrl Pts',(1.81615909809873,72.7116650682347,12.));
#159596=CARTESIAN_POINT('Ctrl Pts',(1.80629642275052,72.6883586034768,0.));
#159597=CARTESIAN_POINT('Ctrl Pts',(1.80629642275052,72.6883586034768,12.));
#159598=CARTESIAN_POINT('Ctrl Pts',(1.7964712627836,72.6650792279271,0.));
#159599=CARTESIAN_POINT('Ctrl Pts',(1.7964712627836,72.6650792279271,12.));
#159600=CARTESIAN_POINT('Ctrl Pts',(1.78668360866814,72.6418270600623,0.));
#159601=CARTESIAN_POINT('Ctrl Pts',(1.78668360866814,72.6418270600623,12.));
#159602=CARTESIAN_POINT('Ctrl Pts',(1.77693345074431,72.618602218792,0.));
#159603=CARTESIAN_POINT('Ctrl Pts',(1.77693345074431,72.618602218792,12.));
#159604=CARTESIAN_POINT('Ctrl Pts',(1.76722077922581,72.5954048234655,0.));
#159605=CARTESIAN_POINT('Ctrl Pts',(1.76722077922581,72.5954048234655,12.));
#159606=CARTESIAN_POINT('Ctrl Pts',(1.75754558420351,72.5722349938789,0.));
#159607=CARTESIAN_POINT('Ctrl Pts',(1.75754558420351,72.5722349938789,12.));
#159608=CARTESIAN_POINT('Ctrl Pts',(1.74790785564477,72.5490928502773,0.));
#159609=CARTESIAN_POINT('Ctrl Pts',(1.74790785564477,72.5490928502773,12.));
#159610=CARTESIAN_POINT('Ctrl Pts',(1.73830758339124,72.5259785133586,0.));
#159611=CARTESIAN_POINT('Ctrl Pts',(1.73830758339124,72.5259785133586,12.));
#159612=CARTESIAN_POINT('Ctrl Pts',(1.72874475715099,72.5028921042704,0.));
#159613=CARTESIAN_POINT('Ctrl Pts',(1.72874475715099,72.5028921042704,12.));
#159614=CARTESIAN_POINT('Ctrl Pts',(1.71921936650033,72.4798337446162,0.));
#159615=CARTESIAN_POINT('Ctrl Pts',(1.71921936650033,72.4798337446162,12.));
#159616=CARTESIAN_POINT('Ctrl Pts',(1.70973140088838,72.4568035564618,0.));
#159617=CARTESIAN_POINT('Ctrl Pts',(1.70973140088838,72.4568035564618,12.));
#159618=CARTESIAN_POINT('Ctrl Pts',(1.70028084963648,72.4338016623388,0.));
#159619=CARTESIAN_POINT('Ctrl Pts',(1.70028084963648,72.4338016623388,12.));
#159620=CARTESIAN_POINT('Ctrl Pts',(1.69086770193642,72.4108281852473,0.));
#159621=CARTESIAN_POINT('Ctrl Pts',(1.69086770193642,72.4108281852473,12.));
#159622=CARTESIAN_POINT('Ctrl Pts',(1.68149194684289,72.3878832486549,0.));
#159623=CARTESIAN_POINT('Ctrl Pts',(1.68149194684289,72.3878832486549,12.));
#159624=CARTESIAN_POINT('Ctrl Pts',(1.67215357327373,72.3649669765013,0.));
#159625=CARTESIAN_POINT('Ctrl Pts',(1.67215357327373,72.3649669765013,12.));
#159626=CARTESIAN_POINT('Ctrl Pts',(1.66285257001503,72.3420794932052,0.));
#159627=CARTESIAN_POINT('Ctrl Pts',(1.66285257001503,72.3420794932052,12.));
#159628=CARTESIAN_POINT('Ctrl Pts',(1.65358892572066,72.3192209236691,0.));
#159629=CARTESIAN_POINT('Ctrl Pts',(1.65358892572066,72.3192209236691,12.));
#159630=CARTESIAN_POINT('Ctrl Pts',(1.64436262891079,72.2963913932811,0.));
#159631=CARTESIAN_POINT('Ctrl Pts',(1.64436262891079,72.2963913932811,12.));
#159632=CARTESIAN_POINT('Ctrl Pts',(1.63517366796459,72.2735910279149,0.));
#159633=CARTESIAN_POINT('Ctrl Pts',(1.63517366796459,72.2735910279149,12.));
#159634=CARTESIAN_POINT('Ctrl Pts',(1.62602203111925,72.2508199539325,0.));
#159635=CARTESIAN_POINT('Ctrl Pts',(1.62602203111925,72.2508199539325,12.));
#159636=CARTESIAN_POINT('Ctrl Pts',(1.61690770647536,72.2280782981941,0.));
#159637=CARTESIAN_POINT('Ctrl Pts',(1.61690770647536,72.2280782981941,12.));
#159638=CARTESIAN_POINT('Ctrl Pts',(1.60783068199663,72.2053661880611,0.));
#159639=CARTESIAN_POINT('Ctrl Pts',(1.60783068199663,72.2053661880611,12.));
#159640=CARTESIAN_POINT('Ctrl Pts',(1.59879094550851,72.1826837514,0.));
#159641=CARTESIAN_POINT('Ctrl Pts',(1.59879094550851,72.1826837514,12.));
#159642=CARTESIAN_POINT('Ctrl Pts',(1.58978848469129,72.1600311165813,0.));
#159643=CARTESIAN_POINT('Ctrl Pts',(1.58978848469129,72.1600311165813,12.));
#159644=CARTESIAN_POINT('Ctrl Pts',(1.58082328707809,72.1374084124829,0.));
#159645=CARTESIAN_POINT('Ctrl Pts',(1.58082328707809,72.1374084124829,12.));
#159646=CARTESIAN_POINT('Ctrl Pts',(1.57189534006044,72.1148157684987,0.));
#159647=CARTESIAN_POINT('Ctrl Pts',(1.57189534006044,72.1148157684987,12.));
#159648=CARTESIAN_POINT('Ctrl Pts',(1.56300463088812,72.092253314543,0.));
#159649=CARTESIAN_POINT('Ctrl Pts',(1.56300463088812,72.092253314543,12.));
#159650=CARTESIAN_POINT('Ctrl Pts',(1.55415114666775,72.0697211810548,0.));
#159651=CARTESIAN_POINT('Ctrl Pts',(1.55415114666775,72.0697211810548,12.));
#159652=CARTESIAN_POINT('Ctrl Pts',(1.54533487435627,72.0472194989968,0.));
#159653=CARTESIAN_POINT('Ctrl Pts',(1.54533487435627,72.0472194989968,12.));
#159654=CARTESIAN_POINT('Ctrl Pts',(1.53655580075814,72.0247483998582,0.));
#159655=CARTESIAN_POINT('Ctrl Pts',(1.53655580075814,72.0247483998582,12.));
#159656=CARTESIAN_POINT('Ctrl Pts',(1.52781391253104,72.0023080156647,0.));
#159657=CARTESIAN_POINT('Ctrl Pts',(1.52781391253104,72.0023080156647,12.));
#159658=CARTESIAN_POINT('Ctrl Pts',(1.51910919618568,71.9798984789828,0.));
#159659=CARTESIAN_POINT('Ctrl Pts',(1.51910919618568,71.9798984789828,12.));
#159660=CARTESIAN_POINT('Ctrl Pts',(1.51044163808456,71.9575199229241,0.));
#159661=CARTESIAN_POINT('Ctrl Pts',(1.51044163808456,71.9575199229241,12.));
#159662=CARTESIAN_POINT('Ctrl Pts',(1.50181122443536,71.935172481145,0.));
#159663=CARTESIAN_POINT('Ctrl Pts',(1.50181122443536,71.935172481145,12.));
#159664=CARTESIAN_POINT('Ctrl Pts',(1.49321794128801,71.9128562878491,0.));
#159665=CARTESIAN_POINT('Ctrl Pts',(1.49321794128801,71.9128562878491,12.));
#159666=CARTESIAN_POINT('Ctrl Pts',(1.48466177454022,71.8905714777972,0.));
#159667=CARTESIAN_POINT('Ctrl Pts',(1.48466177454022,71.8905714777972,12.));
#159668=CARTESIAN_POINT('Ctrl Pts',(1.47614270993731,71.8683181863123,0.));
#159669=CARTESIAN_POINT('Ctrl Pts',(1.47614270993731,71.8683181863123,12.));
#159670=CARTESIAN_POINT('Ctrl Pts',(1.4676607330709,71.8460965492836,0.));
#159671=CARTESIAN_POINT('Ctrl Pts',(1.4676607330709,71.8460965492836,12.));
#159672=CARTESIAN_POINT('Ctrl Pts',(1.4592158293723,71.8239067031664,0.));
#159673=CARTESIAN_POINT('Ctrl Pts',(1.4592158293723,71.8239067031664,12.));
#159674=CARTESIAN_POINT('Ctrl Pts',(1.45080798410958,71.8017487849865,0.));
#159675=CARTESIAN_POINT('Ctrl Pts',(1.45080798410958,71.8017487849865,12.));
#159676=CARTESIAN_POINT('Ctrl Pts',(1.44243718239306,71.7796229323496,0.));
#159677=CARTESIAN_POINT('Ctrl Pts',(1.44243718239306,71.7796229323496,12.));
#159678=CARTESIAN_POINT('Ctrl Pts',(1.4341034091749,71.7575292834456,0.));
#159679=CARTESIAN_POINT('Ctrl Pts',(1.4341034091749,71.7575292834456,12.));
#159680=CARTESIAN_POINT('Ctrl Pts',(1.42580664924775,71.7354679770537,0.));
#159681=CARTESIAN_POINT('Ctrl Pts',(1.42580664924775,71.7354679770537,12.));
#159682=CARTESIAN_POINT('Ctrl Pts',(1.41754688723792,71.7134391525417,0.));
#159683=CARTESIAN_POINT('Ctrl Pts',(1.41754688723792,71.7134391525417,12.));
#159684=CARTESIAN_POINT('Ctrl Pts',(1.40932410760276,71.6914429498702,0.));
#159685=CARTESIAN_POINT('Ctrl Pts',(1.40932410760276,71.6914429498702,12.));
#159686=CARTESIAN_POINT('Ctrl Pts',(1.401138294636,71.6694795096034,0.));
#159687=CARTESIAN_POINT('Ctrl Pts',(1.401138294636,71.6694795096034,12.));
#159688=CARTESIAN_POINT('Ctrl Pts',(1.39298943246732,71.6475489729149,0.));
#159689=CARTESIAN_POINT('Ctrl Pts',(1.39298943246732,71.6475489729149,12.));
#159690=CARTESIAN_POINT('Ctrl Pts',(1.38487750506077,71.6256514815918,0.));
#159691=CARTESIAN_POINT('Ctrl Pts',(1.38487750506077,71.6256514815918,12.));
#159692=CARTESIAN_POINT('Ctrl Pts',(1.37680249620764,71.6037871780347,0.));
#159693=CARTESIAN_POINT('Ctrl Pts',(1.37680249620764,71.6037871780347,12.));
#159694=CARTESIAN_POINT('Ctrl Pts',(1.3687643895245,71.5819562052613,0.));
#159695=CARTESIAN_POINT('Ctrl Pts',(1.3687643895245,71.5819562052613,12.));
#159696=CARTESIAN_POINT('Ctrl Pts',(1.36076316845807,71.5601587069175,0.));
#159697=CARTESIAN_POINT('Ctrl Pts',(1.36076316845807,71.5601587069175,12.));
#159698=CARTESIAN_POINT('Ctrl Pts',(1.35279881628454,71.538394827283,0.));
#159699=CARTESIAN_POINT('Ctrl Pts',(1.35279881628454,71.538394827283,12.));
#159700=CARTESIAN_POINT('Ctrl Pts',(1.34487131610786,71.5166647112766,0.));
#159701=CARTESIAN_POINT('Ctrl Pts',(1.34487131610786,71.5166647112766,12.));
#159702=CARTESIAN_POINT('Ctrl Pts',(1.33698065085229,71.4949685044559,0.));
#159703=CARTESIAN_POINT('Ctrl Pts',(1.33698065085229,71.4949685044559,12.));
#159704=CARTESIAN_POINT('Ctrl Pts',(1.32912680326132,71.4733063530227,0.));
#159705=CARTESIAN_POINT('Ctrl Pts',(1.32912680326132,71.4733063530227,12.));
#159706=CARTESIAN_POINT('Ctrl Pts',(1.32130975590232,71.4516784038346,0.));
#159707=CARTESIAN_POINT('Ctrl Pts',(1.32130975590232,71.4516784038346,12.));
#159708=CARTESIAN_POINT('Ctrl Pts',(1.31352949116539,71.4300848044095,0.));
#159709=CARTESIAN_POINT('Ctrl Pts',(1.31352949116539,71.4300848044095,12.));
#159710=CARTESIAN_POINT('Ctrl Pts',(1.3057859912614,71.4085257029308,0.));
#159711=CARTESIAN_POINT('Ctrl Pts',(1.3057859912614,71.4085257029308,12.));
#159712=CARTESIAN_POINT('Ctrl Pts',(1.29807923821415,71.3870012482474,0.));
#159713=CARTESIAN_POINT('Ctrl Pts',(1.29807923821415,71.3870012482474,12.));
#159714=CARTESIAN_POINT('Ctrl Pts',(1.29040921386062,71.3655115898801,0.));
#159715=CARTESIAN_POINT('Ctrl Pts',(1.29040921386062,71.3655115898801,12.));
#159716=CARTESIAN_POINT('Ctrl Pts',(1.28277589985475,71.344056878033,0.));
#159717=CARTESIAN_POINT('Ctrl Pts',(1.28277589985475,71.344056878033,12.));
#159718=CARTESIAN_POINT('Ctrl Pts',(1.27517927766612,71.3226372635993,0.));
#159719=CARTESIAN_POINT('Ctrl Pts',(1.27517927766612,71.3226372635993,12.));
#159720=CARTESIAN_POINT('Ctrl Pts',(1.26761932857724,71.301252898167,0.));
#159721=CARTESIAN_POINT('Ctrl Pts',(1.26761932857724,71.301252898167,12.));
#159722=CARTESIAN_POINT('Ctrl Pts',(1.26009603367565,71.2799039340191,0.));
#159723=CARTESIAN_POINT('Ctrl Pts',(1.26009603367565,71.2799039340191,12.));
#159724=CARTESIAN_POINT('Ctrl Pts',(1.25260937385562,71.2585905241422,0.));
#159725=CARTESIAN_POINT('Ctrl Pts',(1.25260937385562,71.2585905241422,12.));
#159726=CARTESIAN_POINT('Ctrl Pts',(1.24515932982109,71.2373128222359,0.));
#159727=CARTESIAN_POINT('Ctrl Pts',(1.24515932982109,71.2373128222359,12.));
#159728=CARTESIAN_POINT('Ctrl Pts',(1.23774588208428,71.2160709827189,0.));
#159729=CARTESIAN_POINT('Ctrl Pts',(1.23774588208428,71.2160709827189,12.));
#159730=CARTESIAN_POINT('Ctrl Pts',(1.23036901096247,71.1948651607319,0.));
#159731=CARTESIAN_POINT('Ctrl Pts',(1.23036901096247,71.1948651607319,12.));
#159732=CARTESIAN_POINT('Ctrl Pts',(1.22302869657029,71.1736955121361,0.));
#159733=CARTESIAN_POINT('Ctrl Pts',(1.22302869657029,71.1736955121361,12.));
#159734=CARTESIAN_POINT('Ctrl Pts',(1.21572491882274,71.1525621935266,0.));
#159735=CARTESIAN_POINT('Ctrl Pts',(1.21572491882274,71.1525621935266,12.));
#159736=CARTESIAN_POINT('Ctrl Pts',(1.20845765743655,71.1314653622442,0.));
#159737=CARTESIAN_POINT('Ctrl Pts',(1.20845765743655,71.1314653622442,12.));
#159738=CARTESIAN_POINT('Ctrl Pts',(1.20122689192837,71.1104051763839,0.));
#159739=CARTESIAN_POINT('Ctrl Pts',(1.20122689192837,71.1104051763839,12.));
#159740=CARTESIAN_POINT('Ctrl Pts',(1.19403260160998,71.089381794801,0.));
#159741=CARTESIAN_POINT('Ctrl Pts',(1.19403260160998,71.089381794801,12.));
#159742=CARTESIAN_POINT('Ctrl Pts',(1.18687476558127,71.0683953771147,0.));
#159743=CARTESIAN_POINT('Ctrl Pts',(1.18687476558127,71.0683953771147,12.));
#159744=CARTESIAN_POINT('Ctrl Pts',(1.179753362735,71.0474460837157,0.));
#159745=CARTESIAN_POINT('Ctrl Pts',(1.179753362735,71.0474460837157,12.));
#159746=CARTESIAN_POINT('Ctrl Pts',(1.17266837175777,71.0265340757697,0.));
#159747=CARTESIAN_POINT('Ctrl Pts',(1.17266837175777,71.0265340757697,12.));
#159748=CARTESIAN_POINT('Ctrl Pts',(1.16561977112883,71.0056595152204,0.));
#159749=CARTESIAN_POINT('Ctrl Pts',(1.16561977112883,71.0056595152204,12.));
#159750=CARTESIAN_POINT('Ctrl Pts',(1.15860753911491,70.9848225647876,0.));
#159751=CARTESIAN_POINT('Ctrl Pts',(1.15860753911491,70.9848225647876,12.));
#159752=CARTESIAN_POINT('Ctrl Pts',(1.15163165376531,70.9640233879671,0.));
#159753=CARTESIAN_POINT('Ctrl Pts',(1.15163165376531,70.9640233879671,12.));
#159754=CARTESIAN_POINT('Ctrl Pts',(1.14469209291495,70.943262149058,0.));
#159755=CARTESIAN_POINT('Ctrl Pts',(1.14469209291495,70.943262149058,12.));
#159756=CARTESIAN_POINT('Ctrl Pts',(1.13778883418217,70.9225390131835,0.));
#159757=CARTESIAN_POINT('Ctrl Pts',(1.13778883418217,70.9225390131835,12.));
#159758=CARTESIAN_POINT('Ctrl Pts',(1.13092185496564,70.9018541463083,0.));
#159759=CARTESIAN_POINT('Ctrl Pts',(1.13092185496564,70.9018541463083,12.));
#159760=CARTESIAN_POINT('Ctrl Pts',(1.12409113243512,70.8812077152564,0.));
#159761=CARTESIAN_POINT('Ctrl Pts',(1.12409113243512,70.8812077152564,12.));
#159762=CARTESIAN_POINT('Ctrl Pts',(1.11729664352991,70.860599887712,0.));
#159763=CARTESIAN_POINT('Ctrl Pts',(1.11729664352991,70.860599887712,12.));
#159764=CARTESIAN_POINT('Ctrl Pts',(1.11053836496639,70.8400308322013,0.));
#159765=CARTESIAN_POINT('Ctrl Pts',(1.11053836496639,70.8400308322013,12.));
#159766=CARTESIAN_POINT('Ctrl Pts',(1.10381627323946,70.8195007180739,0.));
#159767=CARTESIAN_POINT('Ctrl Pts',(1.10381627323946,70.8195007180739,12.));
#159768=CARTESIAN_POINT('Ctrl Pts',(1.09713034462271,70.7990097154855,0.));
#159769=CARTESIAN_POINT('Ctrl Pts',(1.09713034462271,70.7990097154855,12.));
#159770=CARTESIAN_POINT('Ctrl Pts',(1.09048055516435,70.7785579953611,0.));
#159771=CARTESIAN_POINT('Ctrl Pts',(1.09048055516435,70.7785579953611,12.));
#159772=CARTESIAN_POINT('Ctrl Pts',(1.08386688068349,70.7581457294475,0.));
#159773=CARTESIAN_POINT('Ctrl Pts',(1.08386688068349,70.7581457294475,12.));
#159774=CARTESIAN_POINT('Ctrl Pts',(1.07728929676413,70.7377730903971,0.));
#159775=CARTESIAN_POINT('Ctrl Pts',(1.07728929676413,70.7377730903971,12.));
#159776=CARTESIAN_POINT('Ctrl Pts',(1.07074777874597,70.7174402518378,0.));
#159777=CARTESIAN_POINT('Ctrl Pts',(1.07074777874597,70.7174402518378,12.));
#159778=CARTESIAN_POINT('Ctrl Pts',(1.06424230171281,70.6971473884443,0.));
#159779=CARTESIAN_POINT('Ctrl Pts',(1.06424230171281,70.6971473884443,12.));
#159780=CARTESIAN_POINT('Ctrl Pts',(1.05777284047728,70.6768946760063,0.));
#159781=CARTESIAN_POINT('Ctrl Pts',(1.05777284047728,70.6768946760063,12.));
#159782=CARTESIAN_POINT('Ctrl Pts',(1.0513393696007,70.6566822912965,0.));
#159783=CARTESIAN_POINT('Ctrl Pts',(1.0513393696007,70.6566822912965,12.));
#159784=CARTESIAN_POINT('Ctrl Pts',(1.04494186341157,70.6365104119238,0.));
#159785=CARTESIAN_POINT('Ctrl Pts',(1.04494186341157,70.6365104119238,12.));
#159786=CARTESIAN_POINT('Ctrl Pts',(1.03858029601906,70.6163792162079,0.));
#159787=CARTESIAN_POINT('Ctrl Pts',(1.03858029601906,70.6163792162079,12.));
#159788=CARTESIAN_POINT('Ctrl Pts',(1.03225464132873,70.5962888829958,0.));
#159789=CARTESIAN_POINT('Ctrl Pts',(1.03225464132873,70.5962888829958,12.));
#159790=CARTESIAN_POINT('Ctrl Pts',(1.0259648730405,70.5762395916412,0.));
#159791=CARTESIAN_POINT('Ctrl Pts',(1.0259648730405,70.5762395916412,12.));
#159792=CARTESIAN_POINT('Ctrl Pts',(1.019710964606,70.5562315224219,0.));
#159793=CARTESIAN_POINT('Ctrl Pts',(1.019710964606,70.5562315224219,12.));
#159794=CARTESIAN_POINT('Ctrl Pts',(1.01349288918541,70.5362648569072,0.));
#159795=CARTESIAN_POINT('Ctrl Pts',(1.01349288918541,70.5362648569072,12.));
#159796=CARTESIAN_POINT('Ctrl Pts',(1.00731061960968,70.5163397782699,0.));
#159797=CARTESIAN_POINT('Ctrl Pts',(1.00731061960968,70.5163397782699,12.));
#159798=CARTESIAN_POINT('Ctrl Pts',(1.00116412831439,70.4964564717917,0.));
#159799=CARTESIAN_POINT('Ctrl Pts',(1.00116412831439,70.4964564717917,12.));
#159800=CARTESIAN_POINT('Ctrl Pts',(0.995053387379687,70.476615124517,0.));
#159801=CARTESIAN_POINT('Ctrl Pts',(0.995053387379687,70.476615124517,12.));
#159802=CARTESIAN_POINT('Ctrl Pts',(0.988978368643597,70.4568159243131,
0.));
#159803=CARTESIAN_POINT('Ctrl Pts',(0.988978368643597,70.4568159243131,
12.));
#159804=CARTESIAN_POINT('Ctrl Pts',(0.982939043792167,70.4370590590839,
0.));
#159805=CARTESIAN_POINT('Ctrl Pts',(0.982939043792167,70.4370590590839,
12.));
#159806=CARTESIAN_POINT('Ctrl Pts',(0.976935384450135,70.41734471596,0.));
#159807=CARTESIAN_POINT('Ctrl Pts',(0.976935384450135,70.41734471596,12.));
#159808=CARTESIAN_POINT('Ctrl Pts',(0.97096736228131,70.3976730803664,0.));
#159809=CARTESIAN_POINT('Ctrl Pts',(0.97096736228131,70.3976730803664,12.));
#159810=CARTESIAN_POINT('Ctrl Pts',(0.965034948786566,70.3780443378003,
0.));
#159811=CARTESIAN_POINT('Ctrl Pts',(0.965034948786566,70.3780443378003,
12.));
#159812=CARTESIAN_POINT('Ctrl Pts',(0.959138115058893,70.3584586759561,
0.));
#159813=CARTESIAN_POINT('Ctrl Pts',(0.959138115058893,70.3584586759561,
12.));
#159814=CARTESIAN_POINT('Ctrl Pts',(0.953276831581241,70.338916286457,0.));
#159815=CARTESIAN_POINT('Ctrl Pts',(0.953276831581241,70.338916286457,12.));
#159816=CARTESIAN_POINT('Ctrl Pts',(0.94745106792957,70.3194173673635,0.));
#159817=CARTESIAN_POINT('Ctrl Pts',(0.94745106792957,70.3194173673635,12.));
#159818=CARTESIAN_POINT('Ctrl Pts',(0.941660792742961,70.2999621233938,
0.));
#159819=CARTESIAN_POINT('Ctrl Pts',(0.941660792742961,70.2999621233938,
12.));
#159820=CARTESIAN_POINT('Ctrl Pts',(0.935905974336497,70.2805507606832,
0.));
#159821=CARTESIAN_POINT('Ctrl Pts',(0.935905974336497,70.2805507606832,
12.));
#159822=CARTESIAN_POINT('Ctrl Pts',(0.930186581235583,70.2611834821711,
0.));
#159823=CARTESIAN_POINT('Ctrl Pts',(0.930186581235583,70.2611834821711,
12.));
#159824=CARTESIAN_POINT('Ctrl Pts',(0.924502582639459,70.241860483586,0.));
#159825=CARTESIAN_POINT('Ctrl Pts',(0.924502582639459,70.241860483586,12.));
#159826=CARTESIAN_POINT('Ctrl Pts',(0.918853949157051,70.2225819470306,
0.));
#159827=CARTESIAN_POINT('Ctrl Pts',(0.918853949157051,70.2225819470306,
12.));
#159828=CARTESIAN_POINT('Ctrl Pts',(0.913240652090848,70.2033480471749,
0.));
#159829=CARTESIAN_POINT('Ctrl Pts',(0.913240652090848,70.2033480471749,
12.));
#159830=CARTESIAN_POINT('Ctrl Pts',(0.907662662015657,70.184158963563,0.));
#159831=CARTESIAN_POINT('Ctrl Pts',(0.907662662015657,70.184158963563,12.));
#159832=CARTESIAN_POINT('Ctrl Pts',(0.902119947629781,70.1650148905109,
0.));
#159833=CARTESIAN_POINT('Ctrl Pts',(0.902119947629781,70.1650148905109,
12.));
#159834=CARTESIAN_POINT('Ctrl Pts',(0.896612474372092,70.1459160490366,
0.));
#159835=CARTESIAN_POINT('Ctrl Pts',(0.896612474372092,70.1459160490366,
12.));
#159836=CARTESIAN_POINT('Ctrl Pts',(0.891140203464733,70.1268626950031,
0.));
#159837=CARTESIAN_POINT('Ctrl Pts',(0.891140203464733,70.1268626950031,
12.));
#159838=CARTESIAN_POINT('Ctrl Pts',(0.885703094803093,70.1078550938801,
0.));
#159839=CARTESIAN_POINT('Ctrl Pts',(0.885703094803093,70.1078550938801,
12.));
#159840=CARTESIAN_POINT('Ctrl Pts',(0.880301109661046,70.0888934967772,
0.));
#159841=CARTESIAN_POINT('Ctrl Pts',(0.880301109661046,70.0888934967772,
12.));
#159842=CARTESIAN_POINT('Ctrl Pts',(0.874934213255579,70.0699781184013,
0.));
#159843=CARTESIAN_POINT('Ctrl Pts',(0.874934213255579,70.0699781184013,
12.));
#159844=CARTESIAN_POINT('Ctrl Pts',(0.869602377870148,70.0511091083285,
0.));
#159845=CARTESIAN_POINT('Ctrl Pts',(0.869602377870148,70.0511091083285,
12.));
#159846=CARTESIAN_POINT('Ctrl Pts',(0.864305583660099,70.0322865493339,
0.));
#159847=CARTESIAN_POINT('Ctrl Pts',(0.864305583660099,70.0322865493339,
12.));
#159848=CARTESIAN_POINT('Ctrl Pts',(0.860096170667407,70.0172656934192,
0.));
#159849=CARTESIAN_POINT('Ctrl Pts',(0.860096170667407,70.0172656934192,
12.));
#159850=CARTESIAN_POINT('Ctrl Pts',(0.85695487025838,70.0060209754332,0.));
#159851=CARTESIAN_POINT('Ctrl Pts',(0.85695487025838,70.0060209754332,12.));
#159852=CARTESIAN_POINT('Ctrl Pts',(0.8548676738483,69.9985337959499,0.));
#159853=CARTESIAN_POINT('Ctrl Pts',(0.8548676738483,69.9985337959499,12.));
#159854=CARTESIAN_POINT('Ctrl Pts',(0.853825826608999,69.9947925310006,
0.));
#159855=CARTESIAN_POINT('Ctrl Pts',(0.853825826608999,69.9947925310006,
12.));
#159856=CARTESIAN_POINT('',(0.853825826608999,69.9947925310006,12.));
#159857=CARTESIAN_POINT('Ctrl Pts',(0.853825826608999,69.9947925310006,
12.));
#159858=CARTESIAN_POINT('Ctrl Pts',(0.8548676738483,69.9985337959499,12.));
#159859=CARTESIAN_POINT('Ctrl Pts',(0.85695487025838,70.0060209754332,12.));
#159860=CARTESIAN_POINT('Ctrl Pts',(0.860096170667407,70.0172656934192,
12.));
#159861=CARTESIAN_POINT('Ctrl Pts',(0.864305583660099,70.0322865493339,
12.));
#159862=CARTESIAN_POINT('Ctrl Pts',(0.869602377870148,70.0511091083285,
12.));
#159863=CARTESIAN_POINT('Ctrl Pts',(0.874934213255579,70.0699781184013,
12.));
#159864=CARTESIAN_POINT('Ctrl Pts',(0.880301109661046,70.0888934967772,
12.));
#159865=CARTESIAN_POINT('Ctrl Pts',(0.885703094803093,70.1078550938801,
12.));
#159866=CARTESIAN_POINT('Ctrl Pts',(0.891140203464733,70.1268626950031,
12.));
#159867=CARTESIAN_POINT('Ctrl Pts',(0.896612474372092,70.1459160490366,
12.));
#159868=CARTESIAN_POINT('Ctrl Pts',(0.902119947629781,70.1650148905109,
12.));
#159869=CARTESIAN_POINT('Ctrl Pts',(0.907662662015657,70.184158963563,12.));
#159870=CARTESIAN_POINT('Ctrl Pts',(0.913240652090848,70.2033480471749,
12.));
#159871=CARTESIAN_POINT('Ctrl Pts',(0.918853949157051,70.2225819470306,
12.));
#159872=CARTESIAN_POINT('Ctrl Pts',(0.924502582639459,70.241860483586,12.));
#159873=CARTESIAN_POINT('Ctrl Pts',(0.930186581235583,70.2611834821711,
12.));
#159874=CARTESIAN_POINT('Ctrl Pts',(0.935905974336497,70.2805507606832,
12.));
#159875=CARTESIAN_POINT('Ctrl Pts',(0.941660792742961,70.2999621233938,
12.));
#159876=CARTESIAN_POINT('Ctrl Pts',(0.94745106792957,70.3194173673635,12.));
#159877=CARTESIAN_POINT('Ctrl Pts',(0.953276831581241,70.338916286457,12.));
#159878=CARTESIAN_POINT('Ctrl Pts',(0.959138115058893,70.3584586759561,
12.));
#159879=CARTESIAN_POINT('Ctrl Pts',(0.965034948786566,70.3780443378003,
12.));
#159880=CARTESIAN_POINT('Ctrl Pts',(0.97096736228131,70.3976730803664,12.));
#159881=CARTESIAN_POINT('Ctrl Pts',(0.976935384450135,70.41734471596,12.));
#159882=CARTESIAN_POINT('Ctrl Pts',(0.982939043792167,70.4370590590839,
12.));
#159883=CARTESIAN_POINT('Ctrl Pts',(0.988978368643597,70.4568159243131,
12.));
#159884=CARTESIAN_POINT('Ctrl Pts',(0.995053387379687,70.476615124517,12.));
#159885=CARTESIAN_POINT('Ctrl Pts',(1.00116412831439,70.4964564717917,12.));
#159886=CARTESIAN_POINT('Ctrl Pts',(1.00731061960968,70.5163397782699,12.));
#159887=CARTESIAN_POINT('Ctrl Pts',(1.01349288918541,70.5362648569072,12.));
#159888=CARTESIAN_POINT('Ctrl Pts',(1.019710964606,70.5562315224219,12.));
#159889=CARTESIAN_POINT('Ctrl Pts',(1.0259648730405,70.5762395916412,12.));
#159890=CARTESIAN_POINT('Ctrl Pts',(1.03225464132873,70.5962888829958,12.));
#159891=CARTESIAN_POINT('Ctrl Pts',(1.03858029601906,70.6163792162079,12.));
#159892=CARTESIAN_POINT('Ctrl Pts',(1.04494186341157,70.6365104119238,12.));
#159893=CARTESIAN_POINT('Ctrl Pts',(1.0513393696007,70.6566822912965,12.));
#159894=CARTESIAN_POINT('Ctrl Pts',(1.05777284047728,70.6768946760063,12.));
#159895=CARTESIAN_POINT('Ctrl Pts',(1.06424230171281,70.6971473884443,12.));
#159896=CARTESIAN_POINT('Ctrl Pts',(1.07074777874597,70.7174402518378,12.));
#159897=CARTESIAN_POINT('Ctrl Pts',(1.07728929676413,70.7377730903971,12.));
#159898=CARTESIAN_POINT('Ctrl Pts',(1.08386688068349,70.7581457294475,12.));
#159899=CARTESIAN_POINT('Ctrl Pts',(1.09048055516435,70.7785579953611,12.));
#159900=CARTESIAN_POINT('Ctrl Pts',(1.09713034462271,70.7990097154855,12.));
#159901=CARTESIAN_POINT('Ctrl Pts',(1.10381627323946,70.8195007180739,12.));
#159902=CARTESIAN_POINT('Ctrl Pts',(1.11053836496639,70.8400308322013,12.));
#159903=CARTESIAN_POINT('Ctrl Pts',(1.11729664352991,70.860599887712,12.));
#159904=CARTESIAN_POINT('Ctrl Pts',(1.12409113243512,70.8812077152564,12.));
#159905=CARTESIAN_POINT('Ctrl Pts',(1.13092185496564,70.9018541463083,12.));
#159906=CARTESIAN_POINT('Ctrl Pts',(1.13778883418217,70.9225390131835,12.));
#159907=CARTESIAN_POINT('Ctrl Pts',(1.14469209291495,70.943262149058,12.));
#159908=CARTESIAN_POINT('Ctrl Pts',(1.15163165376531,70.9640233879671,12.));
#159909=CARTESIAN_POINT('Ctrl Pts',(1.15860753911491,70.9848225647876,12.));
#159910=CARTESIAN_POINT('Ctrl Pts',(1.16561977112883,71.0056595152204,12.));
#159911=CARTESIAN_POINT('Ctrl Pts',(1.17266837175777,71.0265340757697,12.));
#159912=CARTESIAN_POINT('Ctrl Pts',(1.179753362735,71.0474460837157,12.));
#159913=CARTESIAN_POINT('Ctrl Pts',(1.18687476558127,71.0683953771147,12.));
#159914=CARTESIAN_POINT('Ctrl Pts',(1.19403260160998,71.089381794801,12.));
#159915=CARTESIAN_POINT('Ctrl Pts',(1.20122689192837,71.1104051763839,12.));
#159916=CARTESIAN_POINT('Ctrl Pts',(1.20845765743655,71.1314653622442,12.));
#159917=CARTESIAN_POINT('Ctrl Pts',(1.21572491882274,71.1525621935266,12.));
#159918=CARTESIAN_POINT('Ctrl Pts',(1.22302869657029,71.1736955121361,12.));
#159919=CARTESIAN_POINT('Ctrl Pts',(1.23036901096247,71.1948651607319,12.));
#159920=CARTESIAN_POINT('Ctrl Pts',(1.23774588208428,71.2160709827189,12.));
#159921=CARTESIAN_POINT('Ctrl Pts',(1.24515932982109,71.2373128222359,12.));
#159922=CARTESIAN_POINT('Ctrl Pts',(1.25260937385562,71.2585905241422,12.));
#159923=CARTESIAN_POINT('Ctrl Pts',(1.26009603367565,71.2799039340191,12.));
#159924=CARTESIAN_POINT('Ctrl Pts',(1.26761932857724,71.301252898167,12.));
#159925=CARTESIAN_POINT('Ctrl Pts',(1.27517927766612,71.3226372635993,12.));
#159926=CARTESIAN_POINT('Ctrl Pts',(1.28277589985475,71.344056878033,12.));
#159927=CARTESIAN_POINT('Ctrl Pts',(1.29040921386062,71.3655115898801,12.));
#159928=CARTESIAN_POINT('Ctrl Pts',(1.29807923821415,71.3870012482474,12.));
#159929=CARTESIAN_POINT('Ctrl Pts',(1.3057859912614,71.4085257029308,12.));
#159930=CARTESIAN_POINT('Ctrl Pts',(1.31352949116539,71.4300848044095,12.));
#159931=CARTESIAN_POINT('Ctrl Pts',(1.32130975590232,71.4516784038346,12.));
#159932=CARTESIAN_POINT('Ctrl Pts',(1.32912680326132,71.4733063530227,12.));
#159933=CARTESIAN_POINT('Ctrl Pts',(1.33698065085229,71.4949685044559,12.));
#159934=CARTESIAN_POINT('Ctrl Pts',(1.34487131610786,71.5166647112766,12.));
#159935=CARTESIAN_POINT('Ctrl Pts',(1.35279881628454,71.538394827283,12.));
#159936=CARTESIAN_POINT('Ctrl Pts',(1.36076316845807,71.5601587069175,12.));
#159937=CARTESIAN_POINT('Ctrl Pts',(1.3687643895245,71.5819562052613,12.));
#159938=CARTESIAN_POINT('Ctrl Pts',(1.37680249620764,71.6037871780347,12.));
#159939=CARTESIAN_POINT('Ctrl Pts',(1.38487750506077,71.6256514815918,12.));
#159940=CARTESIAN_POINT('Ctrl Pts',(1.39298943246732,71.6475489729149,12.));
#159941=CARTESIAN_POINT('Ctrl Pts',(1.401138294636,71.6694795096034,12.));
#159942=CARTESIAN_POINT('Ctrl Pts',(1.40932410760276,71.6914429498702,12.));
#159943=CARTESIAN_POINT('Ctrl Pts',(1.41754688723792,71.7134391525417,12.));
#159944=CARTESIAN_POINT('Ctrl Pts',(1.42580664924775,71.7354679770537,12.));
#159945=CARTESIAN_POINT('Ctrl Pts',(1.4341034091749,71.7575292834456,12.));
#159946=CARTESIAN_POINT('Ctrl Pts',(1.44243718239306,71.7796229323496,12.));
#159947=CARTESIAN_POINT('Ctrl Pts',(1.45080798410958,71.8017487849865,12.));
#159948=CARTESIAN_POINT('Ctrl Pts',(1.4592158293723,71.8239067031664,12.));
#159949=CARTESIAN_POINT('Ctrl Pts',(1.4676607330709,71.8460965492836,12.));
#159950=CARTESIAN_POINT('Ctrl Pts',(1.47614270993731,71.8683181863123,12.));
#159951=CARTESIAN_POINT('Ctrl Pts',(1.48466177454022,71.8905714777972,12.));
#159952=CARTESIAN_POINT('Ctrl Pts',(1.49321794128801,71.9128562878491,12.));
#159953=CARTESIAN_POINT('Ctrl Pts',(1.50181122443536,71.935172481145,12.));
#159954=CARTESIAN_POINT('Ctrl Pts',(1.51044163808456,71.9575199229241,12.));
#159955=CARTESIAN_POINT('Ctrl Pts',(1.51910919618568,71.9798984789828,12.));
#159956=CARTESIAN_POINT('Ctrl Pts',(1.52781391253104,72.0023080156647,12.));
#159957=CARTESIAN_POINT('Ctrl Pts',(1.53655580075814,72.0247483998582,12.));
#159958=CARTESIAN_POINT('Ctrl Pts',(1.54533487435627,72.0472194989968,12.));
#159959=CARTESIAN_POINT('Ctrl Pts',(1.55415114666775,72.0697211810548,12.));
#159960=CARTESIAN_POINT('Ctrl Pts',(1.56300463088812,72.092253314543,12.));
#159961=CARTESIAN_POINT('Ctrl Pts',(1.57189534006044,72.1148157684987,12.));
#159962=CARTESIAN_POINT('Ctrl Pts',(1.58082328707809,72.1374084124829,12.));
#159963=CARTESIAN_POINT('Ctrl Pts',(1.58978848469129,72.1600311165813,12.));
#159964=CARTESIAN_POINT('Ctrl Pts',(1.59879094550851,72.1826837514,12.));
#159965=CARTESIAN_POINT('Ctrl Pts',(1.60783068199663,72.2053661880611,12.));
#159966=CARTESIAN_POINT('Ctrl Pts',(1.61690770647536,72.2280782981941,12.));
#159967=CARTESIAN_POINT('Ctrl Pts',(1.62602203111925,72.2508199539325,12.));
#159968=CARTESIAN_POINT('Ctrl Pts',(1.63517366796459,72.2735910279149,12.));
#159969=CARTESIAN_POINT('Ctrl Pts',(1.64436262891079,72.2963913932811,12.));
#159970=CARTESIAN_POINT('Ctrl Pts',(1.65358892572066,72.3192209236691,12.));
#159971=CARTESIAN_POINT('Ctrl Pts',(1.66285257001503,72.3420794932052,12.));
#159972=CARTESIAN_POINT('Ctrl Pts',(1.67215357327373,72.3649669765013,12.));
#159973=CARTESIAN_POINT('Ctrl Pts',(1.68149194684289,72.3878832486549,12.));
#159974=CARTESIAN_POINT('Ctrl Pts',(1.69086770193642,72.4108281852473,12.));
#159975=CARTESIAN_POINT('Ctrl Pts',(1.70028084963648,72.4338016623388,12.));
#159976=CARTESIAN_POINT('Ctrl Pts',(1.70973140088838,72.4568035564618,12.));
#159977=CARTESIAN_POINT('Ctrl Pts',(1.71921936650033,72.4798337446162,12.));
#159978=CARTESIAN_POINT('Ctrl Pts',(1.72874475715099,72.5028921042704,12.));
#159979=CARTESIAN_POINT('Ctrl Pts',(1.73830758339124,72.5259785133586,12.));
#159980=CARTESIAN_POINT('Ctrl Pts',(1.74790785564477,72.5490928502773,12.));
#159981=CARTESIAN_POINT('Ctrl Pts',(1.75754558420351,72.5722349938789,12.));
#159982=CARTESIAN_POINT('Ctrl Pts',(1.76722077922581,72.5954048234655,12.));
#159983=CARTESIAN_POINT('Ctrl Pts',(1.77693345074431,72.618602218792,12.));
#159984=CARTESIAN_POINT('Ctrl Pts',(1.78668360866814,72.6418270600623,12.));
#159985=CARTESIAN_POINT('Ctrl Pts',(1.7964712627836,72.6650792279271,12.));
#159986=CARTESIAN_POINT('Ctrl Pts',(1.80629642275052,72.6883586034768,12.));
#159987=CARTESIAN_POINT('Ctrl Pts',(1.81615909809873,72.7116650682347,12.));
#159988=CARTESIAN_POINT('Ctrl Pts',(1.82605929823566,72.73499850416,12.));
#159989=CARTESIAN_POINT('Ctrl Pts',(1.83599703244927,72.7583587936454,12.));
#159990=CARTESIAN_POINT('Ctrl Pts',(1.84597230990859,72.7817458195155,12.));
#159991=CARTESIAN_POINT('Ctrl Pts',(1.85598513966116,72.8051594650214,12.));
#159992=CARTESIAN_POINT('Ctrl Pts',(1.86603553062777,72.8285996138346,12.));
#159993=CARTESIAN_POINT('Ctrl Pts',(1.87612349160953,72.8520661500465,12.));
#159994=CARTESIAN_POINT('Ctrl Pts',(1.88624903129196,72.8755589581674,12.));
#159995=CARTESIAN_POINT('Ctrl Pts',(1.89641215824585,72.8990779231226,12.));
#159996=CARTESIAN_POINT('Ctrl Pts',(1.90661288092583,72.9226229302483,12.));
#159997=CARTESIAN_POINT('Ctrl Pts',(1.91685120766428,72.9461938652816,12.));
#159998=CARTESIAN_POINT('Ctrl Pts',(1.92712714667649,72.9697906143638,12.));
#159999=CARTESIAN_POINT('Ctrl Pts',(1.93744070606558,72.9934130640414,12.));
#160000=CARTESIAN_POINT('Ctrl Pts',(1.94779189382301,73.0170611012659,12.));
#160001=CARTESIAN_POINT('Ctrl Pts',(1.95818071782774,73.0407346133912,12.));
#160002=CARTESIAN_POINT('Ctrl Pts',(1.96860718583945,73.0644334881679,12.));
#160003=CARTESIAN_POINT('Ctrl Pts',(1.97907130550173,73.0881576137415,12.));
#160004=CARTESIAN_POINT('Ctrl Pts',(1.98957308434931,73.1119068786482,12.));
#160005=CARTESIAN_POINT('Ctrl Pts',(2.00011252980988,73.1356811718094,12.));
#160006=CARTESIAN_POINT('Ctrl Pts',(2.01068964920465,73.159480382525,12.));
#160007=CARTESIAN_POINT('Ctrl Pts',(2.02130444974352,73.1833044004612,12.));
#160008=CARTESIAN_POINT('Ctrl Pts',(2.03195693852441,73.2071531156492,12.));
#160009=CARTESIAN_POINT('Ctrl Pts',(2.04264712253916,73.2310264184965,12.));
#160010=CARTESIAN_POINT('Ctrl Pts',(2.05337500867396,73.2549241997946,12.));
#160011=CARTESIAN_POINT('Ctrl Pts',(2.06414060370838,73.2788463507248,12.));
#160012=CARTESIAN_POINT('Ctrl Pts',(2.07494391430955,73.3027927628636,12.));
#160013=CARTESIAN_POINT('Ctrl Pts',(2.08578494702762,73.3267633281822,12.));
#160014=CARTESIAN_POINT('Ctrl Pts',(2.09666370830734,73.3507579390254,12.));
#160015=CARTESIAN_POINT('Ctrl Pts',(2.10758020449401,73.3747764880903,12.));
#160016=CARTESIAN_POINT('Ctrl Pts',(2.11853444183764,73.3988188684022,12.));
#160017=CARTESIAN_POINT('Ctrl Pts',(2.12952642649361,73.4228849732915,12.));
#160018=CARTESIAN_POINT('Ctrl Pts',(2.14055616452049,73.4469746963622,12.));
#160019=CARTESIAN_POINT('Ctrl Pts',(2.151623661879,73.4710879315367,12.));
#160020=CARTESIAN_POINT('Ctrl Pts',(2.16272892442916,73.4952245731044,12.));
#160021=CARTESIAN_POINT('Ctrl Pts',(2.17387195792306,73.5193845157705,12.));
#160022=CARTESIAN_POINT('Ctrl Pts',(2.18505276799757,73.5435676546934,12.));
#160023=CARTESIAN_POINT('Ctrl Pts',(2.19627136015683,73.5677738855461,12.));
#160024=CARTESIAN_POINT('Ctrl Pts',(2.20752773978354,73.5920031044604,12.));
#160025=CARTESIAN_POINT('Ctrl Pts',(2.21882191216522,73.6162552079044,12.));
#160026=CARTESIAN_POINT('Ctrl Pts',(2.2301538825129,73.6405300925714,12.));
#160027=CARTESIAN_POINT('Ctrl Pts',(2.241523655977,73.6648276552766,12.));
#160028=CARTESIAN_POINT('Ctrl Pts',(2.25293123766425,73.6891477928124,12.));
#160029=CARTESIAN_POINT('Ctrl Pts',(2.26437663263664,73.7134904019378,12.));
#160030=CARTESIAN_POINT('Ctrl Pts',(2.27585984587193,73.7378553796792,12.));
#160031=CARTESIAN_POINT('Ctrl Pts',(2.28738088222859,73.7622426235648,12.));
#160032=CARTESIAN_POINT('Ctrl Pts',(2.29893974640436,73.7866520318849,12.));
#160033=CARTESIAN_POINT('Ctrl Pts',(2.31053644289426,73.8110835039341,12.));
#160034=CARTESIAN_POINT('Ctrl Pts',(2.32217097594216,73.8355369402733,12.));
#160035=CARTESIAN_POINT('Ctrl Pts',(2.33384334963981,73.8600122421502,12.));
#160036=CARTESIAN_POINT('Ctrl Pts',(2.34555356802141,73.8845093109302,12.));
#160037=CARTESIAN_POINT('Ctrl Pts',(2.35730163516325,73.9090280474723,12.));
#160038=CARTESIAN_POINT('Ctrl Pts',(2.36908755525995,73.9335683516388,12.));
#160039=CARTESIAN_POINT('Ctrl Pts',(2.38091133274933,73.9581301214609,12.));
#160040=CARTESIAN_POINT('Ctrl Pts',(2.39277297220717,73.9827132538149,12.));
#160041=CARTESIAN_POINT('Ctrl Pts',(2.40467247811497,74.0073176459287,12.));
#160042=CARTESIAN_POINT('Ctrl Pts',(2.41660985465229,74.0319431966956,12.));
#160043=CARTESIAN_POINT('Ctrl Pts',(2.42858510549787,74.0565898079227,12.));
#160044=CARTESIAN_POINT('Ctrl Pts',(2.44059823356722,74.0812573859474,12.));
#160045=CARTESIAN_POINT('Ctrl Pts',(2.45264924094853,74.1059458420175,12.));
#160046=CARTESIAN_POINT('Ctrl Pts',(2.46301176097527,74.1271264545378,12.));
#160047=CARTESIAN_POINT('Ctrl Pts',(2.47097695565715,74.1433763941621,12.));
#160048=CARTESIAN_POINT('Ctrl Pts',(2.47652804725569,74.1546864735452,12.));
#160049=CARTESIAN_POINT('Ctrl Pts',(2.4796539394682,74.1610506466542,12.));
#160050=CARTESIAN_POINT('Ctrl Pts',(2.48034921844894,74.1624659714953,12.));
#160051=CARTESIAN_POINT('',(0.853825826608999,69.9947925310006,0.));
#160052=CARTESIAN_POINT('',(0.853825826608999,69.9947925310006,0.));
#160053=CARTESIAN_POINT('Ctrl Pts',(2.48034921844894,74.1624659714953,0.));
#160054=CARTESIAN_POINT('Ctrl Pts',(2.47965393946819,74.1610506466542,0.));
#160055=CARTESIAN_POINT('Ctrl Pts',(2.47652804725569,74.1546864735452,0.));
#160056=CARTESIAN_POINT('Ctrl Pts',(2.47097695565715,74.1433763941621,0.));
#160057=CARTESIAN_POINT('Ctrl Pts',(2.46301176097527,74.1271264545378,0.));
#160058=CARTESIAN_POINT('Ctrl Pts',(2.45264924094853,74.1059458420175,0.));
#160059=CARTESIAN_POINT('Ctrl Pts',(2.44059823356722,74.0812573859474,0.));
#160060=CARTESIAN_POINT('Ctrl Pts',(2.42858510549787,74.0565898079227,0.));
#160061=CARTESIAN_POINT('Ctrl Pts',(2.41660985465229,74.0319431966956,0.));
#160062=CARTESIAN_POINT('Ctrl Pts',(2.40467247811497,74.0073176459287,0.));
#160063=CARTESIAN_POINT('Ctrl Pts',(2.39277297220717,73.9827132538149,0.));
#160064=CARTESIAN_POINT('Ctrl Pts',(2.38091133274933,73.9581301214609,0.));
#160065=CARTESIAN_POINT('Ctrl Pts',(2.36908755525995,73.9335683516388,0.));
#160066=CARTESIAN_POINT('Ctrl Pts',(2.35730163516325,73.9090280474723,0.));
#160067=CARTESIAN_POINT('Ctrl Pts',(2.34555356802141,73.8845093109302,0.));
#160068=CARTESIAN_POINT('Ctrl Pts',(2.33384334963981,73.8600122421502,0.));
#160069=CARTESIAN_POINT('Ctrl Pts',(2.32217097594216,73.8355369402733,0.));
#160070=CARTESIAN_POINT('Ctrl Pts',(2.31053644289426,73.8110835039341,0.));
#160071=CARTESIAN_POINT('Ctrl Pts',(2.29893974640436,73.7866520318849,0.));
#160072=CARTESIAN_POINT('Ctrl Pts',(2.28738088222859,73.7622426235648,0.));
#160073=CARTESIAN_POINT('Ctrl Pts',(2.27585984587193,73.7378553796792,0.));
#160074=CARTESIAN_POINT('Ctrl Pts',(2.26437663263664,73.7134904019378,0.));
#160075=CARTESIAN_POINT('Ctrl Pts',(2.25293123766425,73.6891477928124,0.));
#160076=CARTESIAN_POINT('Ctrl Pts',(2.241523655977,73.6648276552766,0.));
#160077=CARTESIAN_POINT('Ctrl Pts',(2.2301538825129,73.6405300925714,0.));
#160078=CARTESIAN_POINT('Ctrl Pts',(2.21882191216522,73.6162552079044,0.));
#160079=CARTESIAN_POINT('Ctrl Pts',(2.20752773978354,73.5920031044604,0.));
#160080=CARTESIAN_POINT('Ctrl Pts',(2.19627136015683,73.5677738855461,0.));
#160081=CARTESIAN_POINT('Ctrl Pts',(2.18505276799757,73.5435676546934,0.));
#160082=CARTESIAN_POINT('Ctrl Pts',(2.17387195792306,73.5193845157705,0.));
#160083=CARTESIAN_POINT('Ctrl Pts',(2.16272892442916,73.4952245731044,0.));
#160084=CARTESIAN_POINT('Ctrl Pts',(2.151623661879,73.4710879315367,0.));
#160085=CARTESIAN_POINT('Ctrl Pts',(2.14055616452049,73.4469746963622,0.));
#160086=CARTESIAN_POINT('Ctrl Pts',(2.12952642649361,73.4228849732915,0.));
#160087=CARTESIAN_POINT('Ctrl Pts',(2.11853444183764,73.3988188684022,0.));
#160088=CARTESIAN_POINT('Ctrl Pts',(2.10758020449401,73.3747764880903,0.));
#160089=CARTESIAN_POINT('Ctrl Pts',(2.09666370830734,73.3507579390254,0.));
#160090=CARTESIAN_POINT('Ctrl Pts',(2.08578494702762,73.3267633281822,0.));
#160091=CARTESIAN_POINT('Ctrl Pts',(2.07494391430955,73.3027927628636,0.));
#160092=CARTESIAN_POINT('Ctrl Pts',(2.06414060370838,73.2788463507248,0.));
#160093=CARTESIAN_POINT('Ctrl Pts',(2.05337500867396,73.2549241997946,0.));
#160094=CARTESIAN_POINT('Ctrl Pts',(2.04264712253916,73.2310264184965,0.));
#160095=CARTESIAN_POINT('Ctrl Pts',(2.03195693852441,73.2071531156492,0.));
#160096=CARTESIAN_POINT('Ctrl Pts',(2.02130444974352,73.1833044004612,0.));
#160097=CARTESIAN_POINT('Ctrl Pts',(2.01068964920465,73.159480382525,0.));
#160098=CARTESIAN_POINT('Ctrl Pts',(2.00011252980988,73.1356811718094,0.));
#160099=CARTESIAN_POINT('Ctrl Pts',(1.98957308434931,73.1119068786482,0.));
#160100=CARTESIAN_POINT('Ctrl Pts',(1.97907130550173,73.0881576137415,0.));
#160101=CARTESIAN_POINT('Ctrl Pts',(1.96860718583945,73.0644334881679,0.));
#160102=CARTESIAN_POINT('Ctrl Pts',(1.95818071782774,73.0407346133912,0.));
#160103=CARTESIAN_POINT('Ctrl Pts',(1.94779189382301,73.0170611012659,0.));
#160104=CARTESIAN_POINT('Ctrl Pts',(1.93744070606558,72.9934130640414,0.));
#160105=CARTESIAN_POINT('Ctrl Pts',(1.92712714667649,72.9697906143638,0.));
#160106=CARTESIAN_POINT('Ctrl Pts',(1.91685120766428,72.9461938652816,0.));
#160107=CARTESIAN_POINT('Ctrl Pts',(1.90661288092583,72.9226229302483,0.));
#160108=CARTESIAN_POINT('Ctrl Pts',(1.89641215824585,72.8990779231226,0.));
#160109=CARTESIAN_POINT('Ctrl Pts',(1.88624903129196,72.8755589581674,0.));
#160110=CARTESIAN_POINT('Ctrl Pts',(1.87612349160953,72.8520661500465,0.));
#160111=CARTESIAN_POINT('Ctrl Pts',(1.86603553062777,72.8285996138346,0.));
#160112=CARTESIAN_POINT('Ctrl Pts',(1.85598513966116,72.8051594650214,0.));
#160113=CARTESIAN_POINT('Ctrl Pts',(1.84597230990859,72.7817458195155,0.));
#160114=CARTESIAN_POINT('Ctrl Pts',(1.83599703244927,72.7583587936454,0.));
#160115=CARTESIAN_POINT('Ctrl Pts',(1.82605929823566,72.73499850416,0.));
#160116=CARTESIAN_POINT('Ctrl Pts',(1.81615909809873,72.7116650682347,0.));
#160117=CARTESIAN_POINT('Ctrl Pts',(1.80629642275052,72.6883586034768,0.));
#160118=CARTESIAN_POINT('Ctrl Pts',(1.7964712627836,72.6650792279271,0.));
#160119=CARTESIAN_POINT('Ctrl Pts',(1.78668360866814,72.6418270600623,0.));
#160120=CARTESIAN_POINT('Ctrl Pts',(1.77693345074431,72.618602218792,0.));
#160121=CARTESIAN_POINT('Ctrl Pts',(1.76722077922581,72.5954048234655,0.));
#160122=CARTESIAN_POINT('Ctrl Pts',(1.75754558420351,72.5722349938789,0.));
#160123=CARTESIAN_POINT('Ctrl Pts',(1.74790785564477,72.5490928502773,0.));
#160124=CARTESIAN_POINT('Ctrl Pts',(1.73830758339124,72.5259785133586,0.));
#160125=CARTESIAN_POINT('Ctrl Pts',(1.72874475715099,72.5028921042704,0.));
#160126=CARTESIAN_POINT('Ctrl Pts',(1.71921936650033,72.4798337446162,0.));
#160127=CARTESIAN_POINT('Ctrl Pts',(1.70973140088838,72.4568035564618,0.));
#160128=CARTESIAN_POINT('Ctrl Pts',(1.70028084963648,72.4338016623388,0.));
#160129=CARTESIAN_POINT('Ctrl Pts',(1.69086770193642,72.4108281852473,0.));
#160130=CARTESIAN_POINT('Ctrl Pts',(1.68149194684289,72.3878832486549,0.));
#160131=CARTESIAN_POINT('Ctrl Pts',(1.67215357327373,72.3649669765013,0.));
#160132=CARTESIAN_POINT('Ctrl Pts',(1.66285257001503,72.3420794932052,0.));
#160133=CARTESIAN_POINT('Ctrl Pts',(1.65358892572066,72.3192209236691,0.));
#160134=CARTESIAN_POINT('Ctrl Pts',(1.64436262891079,72.2963913932811,0.));
#160135=CARTESIAN_POINT('Ctrl Pts',(1.63517366796459,72.2735910279149,0.));
#160136=CARTESIAN_POINT('Ctrl Pts',(1.62602203111925,72.2508199539325,0.));
#160137=CARTESIAN_POINT('Ctrl Pts',(1.61690770647536,72.2280782981941,0.));
#160138=CARTESIAN_POINT('Ctrl Pts',(1.60783068199663,72.2053661880611,0.));
#160139=CARTESIAN_POINT('Ctrl Pts',(1.59879094550851,72.1826837514,0.));
#160140=CARTESIAN_POINT('Ctrl Pts',(1.58978848469129,72.1600311165813,0.));
#160141=CARTESIAN_POINT('Ctrl Pts',(1.58082328707809,72.1374084124829,0.));
#160142=CARTESIAN_POINT('Ctrl Pts',(1.57189534006044,72.1148157684987,0.));
#160143=CARTESIAN_POINT('Ctrl Pts',(1.56300463088812,72.092253314543,0.));
#160144=CARTESIAN_POINT('Ctrl Pts',(1.55415114666775,72.0697211810548,0.));
#160145=CARTESIAN_POINT('Ctrl Pts',(1.54533487435627,72.0472194989968,0.));
#160146=CARTESIAN_POINT('Ctrl Pts',(1.53655580075814,72.0247483998582,0.));
#160147=CARTESIAN_POINT('Ctrl Pts',(1.52781391253104,72.0023080156647,0.));
#160148=CARTESIAN_POINT('Ctrl Pts',(1.51910919618568,71.9798984789828,0.));
#160149=CARTESIAN_POINT('Ctrl Pts',(1.51044163808456,71.9575199229241,0.));
#160150=CARTESIAN_POINT('Ctrl Pts',(1.50181122443536,71.935172481145,0.));
#160151=CARTESIAN_POINT('Ctrl Pts',(1.49321794128801,71.9128562878491,0.));
#160152=CARTESIAN_POINT('Ctrl Pts',(1.48466177454022,71.8905714777972,0.));
#160153=CARTESIAN_POINT('Ctrl Pts',(1.47614270993731,71.8683181863123,0.));
#160154=CARTESIAN_POINT('Ctrl Pts',(1.4676607330709,71.8460965492836,0.));
#160155=CARTESIAN_POINT('Ctrl Pts',(1.4592158293723,71.8239067031664,0.));
#160156=CARTESIAN_POINT('Ctrl Pts',(1.45080798410958,71.8017487849865,0.));
#160157=CARTESIAN_POINT('Ctrl Pts',(1.44243718239306,71.7796229323496,0.));
#160158=CARTESIAN_POINT('Ctrl Pts',(1.4341034091749,71.7575292834456,0.));
#160159=CARTESIAN_POINT('Ctrl Pts',(1.42580664924775,71.7354679770537,0.));
#160160=CARTESIAN_POINT('Ctrl Pts',(1.41754688723792,71.7134391525417,0.));
#160161=CARTESIAN_POINT('Ctrl Pts',(1.40932410760276,71.6914429498702,0.));
#160162=CARTESIAN_POINT('Ctrl Pts',(1.401138294636,71.6694795096034,0.));
#160163=CARTESIAN_POINT('Ctrl Pts',(1.39298943246732,71.6475489729149,0.));
#160164=CARTESIAN_POINT('Ctrl Pts',(1.38487750506077,71.6256514815918,0.));
#160165=CARTESIAN_POINT('Ctrl Pts',(1.37680249620764,71.6037871780347,0.));
#160166=CARTESIAN_POINT('Ctrl Pts',(1.3687643895245,71.5819562052613,0.));
#160167=CARTESIAN_POINT('Ctrl Pts',(1.36076316845807,71.5601587069175,0.));
#160168=CARTESIAN_POINT('Ctrl Pts',(1.35279881628454,71.538394827283,0.));
#160169=CARTESIAN_POINT('Ctrl Pts',(1.34487131610786,71.5166647112766,0.));
#160170=CARTESIAN_POINT('Ctrl Pts',(1.33698065085229,71.4949685044559,0.));
#160171=CARTESIAN_POINT('Ctrl Pts',(1.32912680326132,71.4733063530227,0.));
#160172=CARTESIAN_POINT('Ctrl Pts',(1.32130975590232,71.4516784038346,0.));
#160173=CARTESIAN_POINT('Ctrl Pts',(1.31352949116539,71.4300848044095,0.));
#160174=CARTESIAN_POINT('Ctrl Pts',(1.3057859912614,71.4085257029308,0.));
#160175=CARTESIAN_POINT('Ctrl Pts',(1.29807923821415,71.3870012482474,0.));
#160176=CARTESIAN_POINT('Ctrl Pts',(1.29040921386062,71.3655115898801,0.));
#160177=CARTESIAN_POINT('Ctrl Pts',(1.28277589985475,71.344056878033,0.));
#160178=CARTESIAN_POINT('Ctrl Pts',(1.27517927766612,71.3226372635993,0.));
#160179=CARTESIAN_POINT('Ctrl Pts',(1.26761932857724,71.301252898167,0.));
#160180=CARTESIAN_POINT('Ctrl Pts',(1.26009603367565,71.2799039340191,0.));
#160181=CARTESIAN_POINT('Ctrl Pts',(1.25260937385562,71.2585905241422,0.));
#160182=CARTESIAN_POINT('Ctrl Pts',(1.24515932982109,71.2373128222359,0.));
#160183=CARTESIAN_POINT('Ctrl Pts',(1.23774588208428,71.2160709827189,0.));
#160184=CARTESIAN_POINT('Ctrl Pts',(1.23036901096247,71.1948651607319,0.));
#160185=CARTESIAN_POINT('Ctrl Pts',(1.22302869657029,71.1736955121361,0.));
#160186=CARTESIAN_POINT('Ctrl Pts',(1.21572491882274,71.1525621935266,0.));
#160187=CARTESIAN_POINT('Ctrl Pts',(1.20845765743655,71.1314653622442,0.));
#160188=CARTESIAN_POINT('Ctrl Pts',(1.20122689192837,71.1104051763839,0.));
#160189=CARTESIAN_POINT('Ctrl Pts',(1.19403260160998,71.089381794801,0.));
#160190=CARTESIAN_POINT('Ctrl Pts',(1.18687476558127,71.0683953771147,0.));
#160191=CARTESIAN_POINT('Ctrl Pts',(1.179753362735,71.0474460837157,0.));
#160192=CARTESIAN_POINT('Ctrl Pts',(1.17266837175777,71.0265340757697,0.));
#160193=CARTESIAN_POINT('Ctrl Pts',(1.16561977112883,71.0056595152204,0.));
#160194=CARTESIAN_POINT('Ctrl Pts',(1.15860753911491,70.9848225647876,0.));
#160195=CARTESIAN_POINT('Ctrl Pts',(1.15163165376531,70.9640233879671,0.));
#160196=CARTESIAN_POINT('Ctrl Pts',(1.14469209291495,70.943262149058,0.));
#160197=CARTESIAN_POINT('Ctrl Pts',(1.13778883418217,70.9225390131835,0.));
#160198=CARTESIAN_POINT('Ctrl Pts',(1.13092185496564,70.9018541463083,0.));
#160199=CARTESIAN_POINT('Ctrl Pts',(1.12409113243512,70.8812077152564,0.));
#160200=CARTESIAN_POINT('Ctrl Pts',(1.11729664352991,70.860599887712,0.));
#160201=CARTESIAN_POINT('Ctrl Pts',(1.11053836496639,70.8400308322013,0.));
#160202=CARTESIAN_POINT('Ctrl Pts',(1.10381627323946,70.8195007180739,0.));
#160203=CARTESIAN_POINT('Ctrl Pts',(1.09713034462271,70.7990097154855,0.));
#160204=CARTESIAN_POINT('Ctrl Pts',(1.09048055516435,70.7785579953611,0.));
#160205=CARTESIAN_POINT('Ctrl Pts',(1.08386688068349,70.7581457294475,0.));
#160206=CARTESIAN_POINT('Ctrl Pts',(1.07728929676413,70.7377730903971,0.));
#160207=CARTESIAN_POINT('Ctrl Pts',(1.07074777874597,70.7174402518378,0.));
#160208=CARTESIAN_POINT('Ctrl Pts',(1.06424230171281,70.6971473884443,0.));
#160209=CARTESIAN_POINT('Ctrl Pts',(1.05777284047728,70.6768946760063,0.));
#160210=CARTESIAN_POINT('Ctrl Pts',(1.0513393696007,70.6566822912965,0.));
#160211=CARTESIAN_POINT('Ctrl Pts',(1.04494186341157,70.6365104119238,0.));
#160212=CARTESIAN_POINT('Ctrl Pts',(1.03858029601906,70.6163792162079,0.));
#160213=CARTESIAN_POINT('Ctrl Pts',(1.03225464132873,70.5962888829958,0.));
#160214=CARTESIAN_POINT('Ctrl Pts',(1.0259648730405,70.5762395916412,0.));
#160215=CARTESIAN_POINT('Ctrl Pts',(1.019710964606,70.5562315224219,0.));
#160216=CARTESIAN_POINT('Ctrl Pts',(1.01349288918541,70.5362648569072,0.));
#160217=CARTESIAN_POINT('Ctrl Pts',(1.00731061960968,70.5163397782699,0.));
#160218=CARTESIAN_POINT('Ctrl Pts',(1.00116412831439,70.4964564717917,0.));
#160219=CARTESIAN_POINT('Ctrl Pts',(0.995053387379687,70.476615124517,0.));
#160220=CARTESIAN_POINT('Ctrl Pts',(0.988978368643597,70.4568159243131,
0.));
#160221=CARTESIAN_POINT('Ctrl Pts',(0.982939043792167,70.4370590590839,
0.));
#160222=CARTESIAN_POINT('Ctrl Pts',(0.976935384450135,70.41734471596,0.));
#160223=CARTESIAN_POINT('Ctrl Pts',(0.97096736228131,70.3976730803664,0.));
#160224=CARTESIAN_POINT('Ctrl Pts',(0.965034948786566,70.3780443378003,
0.));
#160225=CARTESIAN_POINT('Ctrl Pts',(0.959138115058893,70.3584586759561,
0.));
#160226=CARTESIAN_POINT('Ctrl Pts',(0.953276831581241,70.338916286457,0.));
#160227=CARTESIAN_POINT('Ctrl Pts',(0.94745106792957,70.3194173673635,0.));
#160228=CARTESIAN_POINT('Ctrl Pts',(0.941660792742961,70.2999621233938,
0.));
#160229=CARTESIAN_POINT('Ctrl Pts',(0.935905974336497,70.2805507606832,
0.));
#160230=CARTESIAN_POINT('Ctrl Pts',(0.930186581235583,70.2611834821711,
0.));
#160231=CARTESIAN_POINT('Ctrl Pts',(0.924502582639459,70.241860483586,0.));
#160232=CARTESIAN_POINT('Ctrl Pts',(0.918853949157051,70.2225819470306,
0.));
#160233=CARTESIAN_POINT('Ctrl Pts',(0.913240652090848,70.2033480471749,
0.));
#160234=CARTESIAN_POINT('Ctrl Pts',(0.907662662015657,70.184158963563,0.));
#160235=CARTESIAN_POINT('Ctrl Pts',(0.902119947629781,70.1650148905109,
0.));
#160236=CARTESIAN_POINT('Ctrl Pts',(0.896612474372092,70.1459160490366,
0.));
#160237=CARTESIAN_POINT('Ctrl Pts',(0.891140203464733,70.1268626950031,
0.));
#160238=CARTESIAN_POINT('Ctrl Pts',(0.885703094803093,70.1078550938801,
0.));
#160239=CARTESIAN_POINT('Ctrl Pts',(0.880301109661046,70.0888934967772,
0.));
#160240=CARTESIAN_POINT('Ctrl Pts',(0.874934213255579,70.0699781184013,
0.));
#160241=CARTESIAN_POINT('Ctrl Pts',(0.869602377870148,70.0511091083285,
0.));
#160242=CARTESIAN_POINT('Ctrl Pts',(0.864305583660099,70.0322865493339,
0.));
#160243=CARTESIAN_POINT('Ctrl Pts',(0.860096170667407,70.0172656934192,
0.));
#160244=CARTESIAN_POINT('Ctrl Pts',(0.85695487025838,70.0060209754332,0.));
#160245=CARTESIAN_POINT('Ctrl Pts',(0.8548676738483,69.9985337959499,0.));
#160246=CARTESIAN_POINT('Ctrl Pts',(0.853825826608999,69.9947925310006,
0.));
#160247=CARTESIAN_POINT('Ctrl Pts',(9.10443154852689,73.9415940197274,0.));
#160248=CARTESIAN_POINT('Ctrl Pts',(9.10443154852689,73.9415940197274,12.));
#160249=CARTESIAN_POINT('Ctrl Pts',(9.10148558516538,73.9368365074299,0.));
#160250=CARTESIAN_POINT('Ctrl Pts',(9.10148558516538,73.9368365074299,12.));
#160251=CARTESIAN_POINT('Ctrl Pts',(9.09559760529043,73.9273231219835,0.));
#160252=CARTESIAN_POINT('Ctrl Pts',(9.09559760529043,73.9273231219835,12.));
#160253=CARTESIAN_POINT('Ctrl Pts',(9.08677747602206,73.9130579612604,0.));
#160254=CARTESIAN_POINT('Ctrl Pts',(9.08677747602206,73.9130579612604,12.));
#160255=CARTESIAN_POINT('Ctrl Pts',(9.07504098571708,73.8940475822492,0.));
#160256=CARTESIAN_POINT('Ctrl Pts',(9.07504098571708,73.8940475822492,12.));
#160257=CARTESIAN_POINT('Ctrl Pts',(9.06040984890247,73.8703010078091,0.));
#160258=CARTESIAN_POINT('Ctrl Pts',(9.06040984890247,73.8703010078091,12.));
#160259=CARTESIAN_POINT('Ctrl Pts',(9.04581819646985,73.8465708501057,0.));
#160260=CARTESIAN_POINT('Ctrl Pts',(9.04581819646985,73.8465708501057,12.));
#160261=CARTESIAN_POINT('Ctrl Pts',(9.03126603778126,73.8228571411697,0.));
#160262=CARTESIAN_POINT('Ctrl Pts',(9.03126603778126,73.8228571411697,12.));
#160263=CARTESIAN_POINT('Ctrl Pts',(9.01675338208005,73.7991599312592,0.));
#160264=CARTESIAN_POINT('Ctrl Pts',(9.01675338208005,73.7991599312592,12.));
#160265=CARTESIAN_POINT('Ctrl Pts',(9.00228023701056,73.7754792943665,0.));
#160266=CARTESIAN_POINT('Ctrl Pts',(9.00228023701056,73.7754792943665,12.));
#160267=CARTESIAN_POINT('Ctrl Pts',(8.98784660837398,73.7518153261981,0.));
#160268=CARTESIAN_POINT('Ctrl Pts',(8.98784660837398,73.7518153261981,12.));
#160269=CARTESIAN_POINT('Ctrl Pts',(8.97345250083601,73.728168136383,0.));
#160270=CARTESIAN_POINT('Ctrl Pts',(8.97345250083601,73.728168136383,12.));
#160271=CARTESIAN_POINT('Ctrl Pts',(8.95909791836153,73.7045378422686,0.));
#160272=CARTESIAN_POINT('Ctrl Pts',(8.95909791836153,73.7045378422686,12.));
#160273=CARTESIAN_POINT('Ctrl Pts',(8.9447828647442,73.6809245622383,0.));
#160274=CARTESIAN_POINT('Ctrl Pts',(8.9447828647442,73.6809245622383,12.));
#160275=CARTESIAN_POINT('Ctrl Pts',(8.93050734412125,73.6573284088184,0.));
#160276=CARTESIAN_POINT('Ctrl Pts',(8.93050734412125,73.6573284088184,12.));
#160277=CARTESIAN_POINT('Ctrl Pts',(8.91627136140085,73.633749483097,0.));
#160278=CARTESIAN_POINT('Ctrl Pts',(8.91627136140085,73.633749483097,12.));
#160279=CARTESIAN_POINT('Ctrl Pts',(8.90207492199043,73.6101878785976,0.));
#160280=CARTESIAN_POINT('Ctrl Pts',(8.90207492199043,73.6101878785976,12.));
#160281=CARTESIAN_POINT('Ctrl Pts',(8.88791803160443,73.5866436840556,0.));
#160282=CARTESIAN_POINT('Ctrl Pts',(8.88791803160443,73.5866436840556,12.));
#160283=CARTESIAN_POINT('Ctrl Pts',(8.87380069602971,73.5631169867122,0.));
#160284=CARTESIAN_POINT('Ctrl Pts',(8.87380069602971,73.5631169867122,12.));
#160285=CARTESIAN_POINT('Ctrl Pts',(8.85972292092131,73.5396078751639,0.));
#160286=CARTESIAN_POINT('Ctrl Pts',(8.85972292092131,73.5396078751639,12.));
#160287=CARTESIAN_POINT('Ctrl Pts',(8.84568471153806,73.5161164429709,0.));
#160288=CARTESIAN_POINT('Ctrl Pts',(8.84568471153806,73.5161164429709,12.));
#160289=CARTESIAN_POINT('Ctrl Pts',(8.83168607277326,73.492642788273,0.));
#160290=CARTESIAN_POINT('Ctrl Pts',(8.83168607277326,73.492642788273,12.));
#160291=CARTESIAN_POINT('Ctrl Pts',(8.81772700927531,73.4691870121567,0.));
#160292=CARTESIAN_POINT('Ctrl Pts',(8.81772700927531,73.4691870121567,12.));
#160293=CARTESIAN_POINT('Ctrl Pts',(8.80380752553692,73.4457492173933,0.));
#160294=CARTESIAN_POINT('Ctrl Pts',(8.80380752553692,73.4457492173933,12.));
#160295=CARTESIAN_POINT('Ctrl Pts',(8.78992762598757,73.422329507113,0.));
#160296=CARTESIAN_POINT('Ctrl Pts',(8.78992762598757,73.422329507113,12.));
#160297=CARTESIAN_POINT('Ctrl Pts',(8.77608731509348,73.3989279832835,0.));
#160298=CARTESIAN_POINT('Ctrl Pts',(8.77608731509348,73.3989279832835,12.));
#160299=CARTESIAN_POINT('Ctrl Pts',(8.76228659740358,73.3755447460269,0.));
#160300=CARTESIAN_POINT('Ctrl Pts',(8.76228659740358,73.3755447460269,12.));
#160301=CARTESIAN_POINT('Ctrl Pts',(8.74852547749778,73.3521798944622,0.));
#160302=CARTESIAN_POINT('Ctrl Pts',(8.74852547749778,73.3521798944622,12.));
#160303=CARTESIAN_POINT('Ctrl Pts',(8.7348039599538,73.3288335272002,0.));
#160304=CARTESIAN_POINT('Ctrl Pts',(8.7348039599538,73.3288335272002,12.));
#160305=CARTESIAN_POINT('Ctrl Pts',(8.72112204930232,73.3055057429742,0.));
#160306=CARTESIAN_POINT('Ctrl Pts',(8.72112204930232,73.3055057429742,12.));
#160307=CARTESIAN_POINT('Ctrl Pts',(8.7074797499823,73.2821966412148,0.));
#160308=CARTESIAN_POINT('Ctrl Pts',(8.7074797499823,73.2821966412148,12.));
#160309=CARTESIAN_POINT('Ctrl Pts',(8.69387706629286,73.2589063226358,0.));
#160310=CARTESIAN_POINT('Ctrl Pts',(8.69387706629286,73.2589063226358,12.));
#160311=CARTESIAN_POINT('Ctrl Pts',(8.68031400241872,73.2356348889693,0.));
#160312=CARTESIAN_POINT('Ctrl Pts',(8.68031400241872,73.2356348889693,12.));
#160313=CARTESIAN_POINT('Ctrl Pts',(8.66679056245092,73.2123824427208,0.));
#160314=CARTESIAN_POINT('Ctrl Pts',(8.66679056245092,73.2123824427208,12.));
#160315=CARTESIAN_POINT('Ctrl Pts',(8.65330675040537,73.1891490869056,0.));
#160316=CARTESIAN_POINT('Ctrl Pts',(8.65330675040537,73.1891490869056,12.));
#160317=CARTESIAN_POINT('Ctrl Pts',(8.63986257023739,73.1659349248133,0.));
#160318=CARTESIAN_POINT('Ctrl Pts',(8.63986257023739,73.1659349248133,12.));
#160319=CARTESIAN_POINT('Ctrl Pts',(8.62645802585484,73.1427400597037,0.));
#160320=CARTESIAN_POINT('Ctrl Pts',(8.62645802585484,73.1427400597037,12.));
#160321=CARTESIAN_POINT('Ctrl Pts',(8.61309312112002,73.1195645948178,0.));
#160322=CARTESIAN_POINT('Ctrl Pts',(8.61309312112002,73.1195645948178,12.));
#160323=CARTESIAN_POINT('Ctrl Pts',(8.59976785984552,73.0964086335235,0.));
#160324=CARTESIAN_POINT('Ctrl Pts',(8.59976785984552,73.0964086335235,12.));
#160325=CARTESIAN_POINT('Ctrl Pts',(8.58648224578732,73.0732722794195,0.));
#160326=CARTESIAN_POINT('Ctrl Pts',(8.58648224578732,73.0732722794195,12.));
#160327=CARTESIAN_POINT('Ctrl Pts',(8.57323628263593,73.0501556364479,0.));
#160328=CARTESIAN_POINT('Ctrl Pts',(8.57323628263593,73.0501556364479,12.));
#160329=CARTESIAN_POINT('Ctrl Pts',(8.56002997400084,73.0270588090183,0.));
#160330=CARTESIAN_POINT('Ctrl Pts',(8.56002997400084,73.0270588090183,12.));
#160331=CARTESIAN_POINT('Ctrl Pts',(8.54686332340418,73.0039819020648,0.));
#160332=CARTESIAN_POINT('Ctrl Pts',(8.54686332340418,73.0039819020648,12.));
#160333=CARTESIAN_POINT('Ctrl Pts',(8.53373633429281,72.9809250209828,0.));
#160334=CARTESIAN_POINT('Ctrl Pts',(8.53373633429281,72.9809250209828,12.));
#160335=CARTESIAN_POINT('Ctrl Pts',(8.52064901004228,72.9578882715912,0.));
#160336=CARTESIAN_POINT('Ctrl Pts',(8.52064901004228,72.9578882715912,12.));
#160337=CARTESIAN_POINT('Ctrl Pts',(8.50760135395984,72.9348717600838,0.));
#160338=CARTESIAN_POINT('Ctrl Pts',(8.50760135395984,72.9348717600838,12.));
#160339=CARTESIAN_POINT('Ctrl Pts',(8.49459336928296,72.9118755929795,0.));
#160340=CARTESIAN_POINT('Ctrl Pts',(8.49459336928296,72.9118755929795,12.));
#160341=CARTESIAN_POINT('Ctrl Pts',(8.48162505917658,72.8888998770785,0.));
#160342=CARTESIAN_POINT('Ctrl Pts',(8.48162505917658,72.8888998770785,12.));
#160343=CARTESIAN_POINT('Ctrl Pts',(8.46869642673795,72.8659447194933,0.));
#160344=CARTESIAN_POINT('Ctrl Pts',(8.46869642673795,72.8659447194933,12.));
#160345=CARTESIAN_POINT('Ctrl Pts',(8.45580747499793,72.8430102276713,0.));
#160346=CARTESIAN_POINT('Ctrl Pts',(8.45580747499793,72.8430102276713,12.));
#160347=CARTESIAN_POINT('Ctrl Pts',(8.44295820691912,72.8200965094199,0.));
#160348=CARTESIAN_POINT('Ctrl Pts',(8.44295820691912,72.8200965094199,12.));
#160349=CARTESIAN_POINT('Ctrl Pts',(8.43014862539158,72.7972036729276,0.));
#160350=CARTESIAN_POINT('Ctrl Pts',(8.43014862539158,72.7972036729276,12.));
#160351=CARTESIAN_POINT('Ctrl Pts',(8.4173787332233,72.7743318267865,0.));
#160352=CARTESIAN_POINT('Ctrl Pts',(8.4173787332233,72.7743318267865,12.));
#160353=CARTESIAN_POINT('Ctrl Pts',(8.40464853314469,72.751481079992,0.));
#160354=CARTESIAN_POINT('Ctrl Pts',(8.40464853314469,72.751481079992,12.));
#160355=CARTESIAN_POINT('Ctrl Pts',(8.39195802781391,72.7286515419373,0.));
#160356=CARTESIAN_POINT('Ctrl Pts',(8.39195802781391,72.7286515419373,12.));
#160357=CARTESIAN_POINT('Ctrl Pts',(8.37930721981731,72.705843322407,0.));
#160358=CARTESIAN_POINT('Ctrl Pts',(8.37930721981731,72.705843322407,12.));
#160359=CARTESIAN_POINT('Ctrl Pts',(8.36669611166843,72.6830565315703,0.));
#160360=CARTESIAN_POINT('Ctrl Pts',(8.36669611166843,72.6830565315703,12.));
#160361=CARTESIAN_POINT('Ctrl Pts',(8.35412470580102,72.6602912799696,0.));
#160362=CARTESIAN_POINT('Ctrl Pts',(8.35412470580102,72.6602912799696,12.));
#160363=CARTESIAN_POINT('Ctrl Pts',(8.34159300456987,72.6375476785215,0.));
#160364=CARTESIAN_POINT('Ctrl Pts',(8.34159300456987,72.6375476785215,12.));
#160365=CARTESIAN_POINT('Ctrl Pts',(8.32910101025671,72.6148258385296,0.));
#160366=CARTESIAN_POINT('Ctrl Pts',(8.32910101025671,72.6148258385296,12.));
#160367=CARTESIAN_POINT('Ctrl Pts',(8.31664872507017,72.5921258716901,0.));
#160368=CARTESIAN_POINT('Ctrl Pts',(8.31664872507017,72.5921258716901,12.));
#160369=CARTESIAN_POINT('Ctrl Pts',(8.30423615114453,72.5694478900982,0.));
#160370=CARTESIAN_POINT('Ctrl Pts',(8.30423615114453,72.5694478900982,12.));
#160371=CARTESIAN_POINT('Ctrl Pts',(8.29186329053279,72.5467920062521,0.));
#160372=CARTESIAN_POINT('Ctrl Pts',(8.29186329053279,72.5467920062521,12.));
#160373=CARTESIAN_POINT('Ctrl Pts',(8.27953014520376,72.5241583330562,0.));
#160374=CARTESIAN_POINT('Ctrl Pts',(8.27953014520376,72.5241583330562,12.));
#160375=CARTESIAN_POINT('Ctrl Pts',(8.2672367170492,72.5015469838254,0.));
#160376=CARTESIAN_POINT('Ctrl Pts',(8.2672367170492,72.5015469838254,12.));
#160377=CARTESIAN_POINT('Ctrl Pts',(8.25498300788494,72.4789580722875,0.));
#160378=CARTESIAN_POINT('Ctrl Pts',(8.25498300788494,72.4789580722875,12.));
#160379=CARTESIAN_POINT('Ctrl Pts',(8.2427690194504,72.4563917125842,0.));
#160380=CARTESIAN_POINT('Ctrl Pts',(8.2427690194504,72.4563917125842,12.));
#160381=CARTESIAN_POINT('Ctrl Pts',(8.23059475340357,72.4338480192695,0.));
#160382=CARTESIAN_POINT('Ctrl Pts',(8.23059475340357,72.4338480192695,12.));
#160383=CARTESIAN_POINT('Ctrl Pts',(8.21846021131561,72.4113271073079,0.));
#160384=CARTESIAN_POINT('Ctrl Pts',(8.21846021131561,72.4113271073079,12.));
#160385=CARTESIAN_POINT('Ctrl Pts',(8.20636539467776,72.3888290920832,0.));
#160386=CARTESIAN_POINT('Ctrl Pts',(8.20636539467776,72.3888290920832,12.));
#160387=CARTESIAN_POINT('Ctrl Pts',(8.19431030490315,72.3663540894026,0.));
#160388=CARTESIAN_POINT('Ctrl Pts',(8.19431030490315,72.3663540894026,12.));
#160389=CARTESIAN_POINT('Ctrl Pts',(8.18229494332624,72.3439022155007,0.));
#160390=CARTESIAN_POINT('Ctrl Pts',(8.18229494332624,72.3439022155007,12.));
#160391=CARTESIAN_POINT('Ctrl Pts',(8.17031931119891,72.3214735870409,0.));
#160392=CARTESIAN_POINT('Ctrl Pts',(8.17031931119891,72.3214735870409,12.));
#160393=CARTESIAN_POINT('Ctrl Pts',(8.15838340968336,72.2990683211162,0.));
#160394=CARTESIAN_POINT('Ctrl Pts',(8.15838340968336,72.2990683211162,12.));
#160395=CARTESIAN_POINT('Ctrl Pts',(8.14648723985798,72.2766865352555,0.));
#160396=CARTESIAN_POINT('Ctrl Pts',(8.14648723985798,72.2766865352555,12.));
#160397=CARTESIAN_POINT('Ctrl Pts',(8.13463080272029,72.2543283474278,0.));
#160398=CARTESIAN_POINT('Ctrl Pts',(8.13463080272029,72.2543283474278,12.));
#160399=CARTESIAN_POINT('Ctrl Pts',(8.12281409918661,72.2319938760449,0.));
#160400=CARTESIAN_POINT('Ctrl Pts',(8.12281409918661,72.2319938760449,12.));
#160401=CARTESIAN_POINT('Ctrl Pts',(8.11103713008928,72.209683239963,0.));
#160402=CARTESIAN_POINT('Ctrl Pts',(8.11103713008928,72.209683239963,12.));
#160403=CARTESIAN_POINT('Ctrl Pts',(8.0992998961689,72.1873965584813,0.));
#160404=CARTESIAN_POINT('Ctrl Pts',(8.0992998961689,72.1873965584813,12.));
#160405=CARTESIAN_POINT('Ctrl Pts',(8.08760239807837,72.1651339513477,0.));
#160406=CARTESIAN_POINT('Ctrl Pts',(8.08760239807837,72.1651339513477,12.));
#160407=CARTESIAN_POINT('Ctrl Pts',(8.07594463638719,72.1428955387663,0.));
#160408=CARTESIAN_POINT('Ctrl Pts',(8.07594463638719,72.1428955387663,12.));
#160409=CARTESIAN_POINT('Ctrl Pts',(8.06432661158096,72.1206814413988,0.));
#160410=CARTESIAN_POINT('Ctrl Pts',(8.06432661158096,72.1206814413988,12.));
#160411=CARTESIAN_POINT('Ctrl Pts',(8.05274832405949,72.0984917803693,0.));
#160412=CARTESIAN_POINT('Ctrl Pts',(8.05274832405949,72.0984917803693,12.));
#160413=CARTESIAN_POINT('Ctrl Pts',(8.04120977412872,72.0763266772615,0.));
#160414=CARTESIAN_POINT('Ctrl Pts',(8.04120977412872,72.0763266772615,12.));
#160415=CARTESIAN_POINT('Ctrl Pts',(8.02971096200308,72.0541862541243,0.));
#160416=CARTESIAN_POINT('Ctrl Pts',(8.02971096200308,72.0541862541243,12.));
#160417=CARTESIAN_POINT('Ctrl Pts',(8.01825188781057,72.032070633479,0.));
#160418=CARTESIAN_POINT('Ctrl Pts',(8.01825188781057,72.032070633479,12.));
#160419=CARTESIAN_POINT('Ctrl Pts',(8.00683255159248,72.0099799383213,0.));
#160420=CARTESIAN_POINT('Ctrl Pts',(8.00683255159248,72.0099799383213,12.));
#160421=CARTESIAN_POINT('Ctrl Pts',(7.99545295330191,71.9879142921254,0.));
#160422=CARTESIAN_POINT('Ctrl Pts',(7.99545295330191,71.9879142921254,12.));
#160423=CARTESIAN_POINT('Ctrl Pts',(7.98411309279613,71.965873818843,0.));
#160424=CARTESIAN_POINT('Ctrl Pts',(7.98411309279613,71.965873818843,12.));
#160425=CARTESIAN_POINT('Ctrl Pts',(7.97281296983718,71.9438586429081,0.));
#160426=CARTESIAN_POINT('Ctrl Pts',(7.97281296983718,71.9438586429081,12.));
#160427=CARTESIAN_POINT('Ctrl Pts',(7.96155258409764,71.9218688892431,0.));
#160428=CARTESIAN_POINT('Ctrl Pts',(7.96155258409764,71.9218688892431,12.));
#160429=CARTESIAN_POINT('Ctrl Pts',(7.95033193516051,71.8999046832643,0.));
#160430=CARTESIAN_POINT('Ctrl Pts',(7.95033193516051,71.8999046832643,12.));
#160431=CARTESIAN_POINT('Ctrl Pts',(7.93915102251795,71.8779661508832,0.));
#160432=CARTESIAN_POINT('Ctrl Pts',(7.93915102251795,71.8779661508832,12.));
#160433=CARTESIAN_POINT('Ctrl Pts',(7.92800984556396,71.8560534185071,0.));
#160434=CARTESIAN_POINT('Ctrl Pts',(7.92800984556396,71.8560534185071,12.));
#160435=CARTESIAN_POINT('Ctrl Pts',(7.91690840359367,71.8341666130426,0.));
#160436=CARTESIAN_POINT('Ctrl Pts',(7.91690840359367,71.8341666130426,12.));
#160437=CARTESIAN_POINT('Ctrl Pts',(7.90584669580956,71.8123058619042,0.));
#160438=CARTESIAN_POINT('Ctrl Pts',(7.90584669580956,71.8123058619042,12.));
#160439=CARTESIAN_POINT('Ctrl Pts',(7.89482472132137,71.7904712930175,0.));
#160440=CARTESIAN_POINT('Ctrl Pts',(7.89482472132137,71.7904712930175,12.));
#160441=CARTESIAN_POINT('Ctrl Pts',(7.88384247914524,71.7686630348238,0.));
#160442=CARTESIAN_POINT('Ctrl Pts',(7.88384247914524,71.7686630348238,12.));
#160443=CARTESIAN_POINT('Ctrl Pts',(7.87289996819654,71.7468812162788,0.));
#160444=CARTESIAN_POINT('Ctrl Pts',(7.87289996819654,71.7468812162788,12.));
#160445=CARTESIAN_POINT('Ctrl Pts',(7.86199718728826,71.7251259668563,0.));
#160446=CARTESIAN_POINT('Ctrl Pts',(7.86199718728826,71.7251259668563,12.));
#160447=CARTESIAN_POINT('Ctrl Pts',(7.85113413513736,71.7033974165568,0.));
#160448=CARTESIAN_POINT('Ctrl Pts',(7.85113413513736,71.7033974165568,12.));
#160449=CARTESIAN_POINT('Ctrl Pts',(7.8403108103649,71.6816956959117,0.));
#160450=CARTESIAN_POINT('Ctrl Pts',(7.8403108103649,71.6816956959117,12.));
#160451=CARTESIAN_POINT('Ctrl Pts',(7.82952721149508,71.6600209359872,0.));
#160452=CARTESIAN_POINT('Ctrl Pts',(7.82952721149508,71.6600209359872,12.));
#160453=CARTESIAN_POINT('Ctrl Pts',(7.81878333694861,71.6383732683844,0.));
#160454=CARTESIAN_POINT('Ctrl Pts',(7.81878333694861,71.6383732683844,12.));
#160455=CARTESIAN_POINT('Ctrl Pts',(7.80807918504022,71.6167528252423,0.));
#160456=CARTESIAN_POINT('Ctrl Pts',(7.80807918504022,71.6167528252423,12.));
#160457=CARTESIAN_POINT('Ctrl Pts',(7.79741475398514,71.5951597392471,0.));
#160458=CARTESIAN_POINT('Ctrl Pts',(7.79741475398514,71.5951597392471,12.));
#160459=CARTESIAN_POINT('Ctrl Pts',(7.78679004189935,71.5735941436364,0.));
#160460=CARTESIAN_POINT('Ctrl Pts',(7.78679004189935,71.5735941436364,12.));
#160461=CARTESIAN_POINT('Ctrl Pts',(7.7762050467987,71.5520561722039,0.));
#160462=CARTESIAN_POINT('Ctrl Pts',(7.7762050467987,71.5520561722039,12.));
#160463=CARTESIAN_POINT('Ctrl Pts',(7.76565976659226,71.5305459592994,0.));
#160464=CARTESIAN_POINT('Ctrl Pts',(7.76565976659226,71.5305459592994,12.));
#160465=CARTESIAN_POINT('Ctrl Pts',(7.75515419907967,71.5090636398318,0.));
#160466=CARTESIAN_POINT('Ctrl Pts',(7.75515419907967,71.5090636398318,12.));
#160467=CARTESIAN_POINT('Ctrl Pts',(7.74468834195746,71.4876093492781,0.));
#160468=CARTESIAN_POINT('Ctrl Pts',(7.74468834195746,71.4876093492781,12.));
#160469=CARTESIAN_POINT('Ctrl Pts',(7.7342621928194,71.4661832236888,0.));
#160470=CARTESIAN_POINT('Ctrl Pts',(7.7342621928194,71.4661832236888,12.));
#160471=CARTESIAN_POINT('Ctrl Pts',(7.72387574915544,71.4447853996916,0.));
#160472=CARTESIAN_POINT('Ctrl Pts',(7.72387574915544,71.4447853996916,12.));
#160473=CARTESIAN_POINT('Ctrl Pts',(7.7135290083452,71.4234160144925,0.));
#160474=CARTESIAN_POINT('Ctrl Pts',(7.7135290083452,71.4234160144925,12.));
#160475=CARTESIAN_POINT('Ctrl Pts',(7.70322196765539,71.4020752058796,0.));
#160476=CARTESIAN_POINT('Ctrl Pts',(7.70322196765539,71.4020752058796,12.));
#160477=CARTESIAN_POINT('Ctrl Pts',(7.69295462424612,71.3807631122331,0.));
#160478=CARTESIAN_POINT('Ctrl Pts',(7.69295462424612,71.3807631122331,12.));
#160479=CARTESIAN_POINT('Ctrl Pts',(7.68272697517086,71.3594798725281,0.));
#160480=CARTESIAN_POINT('Ctrl Pts',(7.68272697517086,71.3594798725281,12.));
#160481=CARTESIAN_POINT('Ctrl Pts',(7.67253901737553,71.3382256263414,0.));
#160482=CARTESIAN_POINT('Ctrl Pts',(7.67253901737553,71.3382256263414,12.));
#160483=CARTESIAN_POINT('Ctrl Pts',(7.66239074769163,71.3170005138502,0.));
#160484=CARTESIAN_POINT('Ctrl Pts',(7.66239074769163,71.3170005138502,12.));
#160485=CARTESIAN_POINT('Ctrl Pts',(7.65228216283404,71.2958046758372,0.));
#160486=CARTESIAN_POINT('Ctrl Pts',(7.65228216283404,71.2958046758372,12.));
#160487=CARTESIAN_POINT('Ctrl Pts',(7.64221325940725,71.2746382537007,0.));
#160488=CARTESIAN_POINT('Ctrl Pts',(7.64221325940725,71.2746382537007,12.));
#160489=CARTESIAN_POINT('Ctrl Pts',(7.63218403390538,71.2535013894602,0.));
#160490=CARTESIAN_POINT('Ctrl Pts',(7.63218403390538,71.2535013894602,12.));
#160491=CARTESIAN_POINT('Ctrl Pts',(7.62219448271109,71.2323942257609,0.));
#160492=CARTESIAN_POINT('Ctrl Pts',(7.62219448271109,71.2323942257609,12.));
#160493=CARTESIAN_POINT('Ctrl Pts',(7.61224460208838,71.211316905874,0.));
#160494=CARTESIAN_POINT('Ctrl Pts',(7.61224460208838,71.211316905874,12.));
#160495=CARTESIAN_POINT('Ctrl Pts',(7.60233438818097,71.1902695737013,0.));
#160496=CARTESIAN_POINT('Ctrl Pts',(7.60233438818097,71.1902695737013,12.));
#160497=CARTESIAN_POINT('Ctrl Pts',(7.59246383701814,71.1692523737844,0.));
#160498=CARTESIAN_POINT('Ctrl Pts',(7.59246383701814,71.1692523737844,12.));
#160499=CARTESIAN_POINT('Ctrl Pts',(7.58263294451452,71.1482654513119,0.));
#160500=CARTESIAN_POINT('Ctrl Pts',(7.58263294451452,71.1482654513119,12.));
#160501=CARTESIAN_POINT('Ctrl Pts',(7.57284170646886,71.1273089521234,0.));
#160502=CARTESIAN_POINT('Ctrl Pts',(7.57284170646886,71.1273089521234,12.));
#160503=CARTESIAN_POINT('Ctrl Pts',(7.56309011855657,71.106383022711,0.));
#160504=CARTESIAN_POINT('Ctrl Pts',(7.56309011855657,71.106383022711,12.));
#160505=CARTESIAN_POINT('Ctrl Pts',(7.55337817632917,71.0854878102243,0.));
#160506=CARTESIAN_POINT('Ctrl Pts',(7.55337817632917,71.0854878102243,12.));
#160507=CARTESIAN_POINT('Ctrl Pts',(7.5437058752198,71.0646234624811,0.));
#160508=CARTESIAN_POINT('Ctrl Pts',(7.5437058752198,71.0646234624811,12.));
#160509=CARTESIAN_POINT('Ctrl Pts',(7.53407321054263,71.043790127973,0.));
#160510=CARTESIAN_POINT('Ctrl Pts',(7.53407321054263,71.043790127973,12.));
#160511=CARTESIAN_POINT('Ctrl Pts',(7.52448017749125,71.0229879558699,0.));
#160512=CARTESIAN_POINT('Ctrl Pts',(7.52448017749125,71.0229879558699,12.));
#160513=CARTESIAN_POINT('Ctrl Pts',(7.51492677113091,71.002217096021,0.));
#160514=CARTESIAN_POINT('Ctrl Pts',(7.51492677113091,71.002217096021,12.));
#160515=CARTESIAN_POINT('Ctrl Pts',(7.50541298639928,70.9814776989612,0.));
#160516=CARTESIAN_POINT('Ctrl Pts',(7.50541298639928,70.9814776989612,12.));
#160517=CARTESIAN_POINT('Ctrl Pts',(7.4959388181113,70.9607699159218,0.));
#160518=CARTESIAN_POINT('Ctrl Pts',(7.4959388181113,70.9607699159218,12.));
#160519=CARTESIAN_POINT('Ctrl Pts',(7.48650426095824,70.940093898837,0.));
#160520=CARTESIAN_POINT('Ctrl Pts',(7.48650426095824,70.940093898837,12.));
#160521=CARTESIAN_POINT('Ctrl Pts',(7.47710930950563,70.9194498003493,0.));
#160522=CARTESIAN_POINT('Ctrl Pts',(7.47710930950563,70.9194498003493,12.));
#160523=CARTESIAN_POINT('Ctrl Pts',(7.46775395818527,70.8988377738104,0.));
#160524=CARTESIAN_POINT('Ctrl Pts',(7.46775395818527,70.8988377738104,12.));
#160525=CARTESIAN_POINT('Ctrl Pts',(7.45843820129782,70.87825797329,0.));
#160526=CARTESIAN_POINT('Ctrl Pts',(7.45843820129782,70.87825797329,12.));
#160527=CARTESIAN_POINT('Ctrl Pts',(7.44916203301648,70.8577105535848,0.));
#160528=CARTESIAN_POINT('Ctrl Pts',(7.44916203301648,70.8577105535848,12.));
#160529=CARTESIAN_POINT('Ctrl Pts',(7.43992544738606,70.8371956702241,0.));
#160530=CARTESIAN_POINT('Ctrl Pts',(7.43992544738606,70.8371956702241,12.));
#160531=CARTESIAN_POINT('Ctrl Pts',(7.43072843832015,70.8167134794737,0.));
#160532=CARTESIAN_POINT('Ctrl Pts',(7.43072843832015,70.8167134794737,12.));
#160533=CARTESIAN_POINT('Ctrl Pts',(7.42157099959326,70.796264138335,0.));
#160534=CARTESIAN_POINT('Ctrl Pts',(7.42157099959326,70.796264138335,12.));
#160535=CARTESIAN_POINT('Ctrl Pts',(7.41245312484498,70.7758478045576,0.));
#160536=CARTESIAN_POINT('Ctrl Pts',(7.41245312484498,70.7758478045576,12.));
#160537=CARTESIAN_POINT('Ctrl Pts',(7.40337480758237,70.7554646366514,0.));
#160538=CARTESIAN_POINT('Ctrl Pts',(7.40337480758237,70.7554646366514,12.));
#160539=CARTESIAN_POINT('Ctrl Pts',(7.39433604117891,70.735114793895,0.));
#160540=CARTESIAN_POINT('Ctrl Pts',(7.39433604117891,70.735114793895,12.));
#160541=CARTESIAN_POINT('Ctrl Pts',(7.38533681887028,70.7147984363423,0.));
#160542=CARTESIAN_POINT('Ctrl Pts',(7.38533681887028,70.7147984363423,12.));
#160543=CARTESIAN_POINT('Ctrl Pts',(7.37637713374761,70.6945157248269,0.));
#160544=CARTESIAN_POINT('Ctrl Pts',(7.37637713374761,70.6945157248269,12.));
#160545=CARTESIAN_POINT('Ctrl Pts',(7.36745697876295,70.6742668209685,0.));
#160546=CARTESIAN_POINT('Ctrl Pts',(7.36745697876295,70.6742668209685,12.));
#160547=CARTESIAN_POINT('Ctrl Pts',(7.35857634673052,70.6540518871772,0.));
#160548=CARTESIAN_POINT('Ctrl Pts',(7.35857634673052,70.6540518871772,12.));
#160549=CARTESIAN_POINT('Ctrl Pts',(7.34973523032581,70.6338710866562,0.));
#160550=CARTESIAN_POINT('Ctrl Pts',(7.34973523032581,70.6338710866562,12.));
#160551=CARTESIAN_POINT('Ctrl Pts',(7.34093362208018,70.6137245834002,0.));
#160552=CARTESIAN_POINT('Ctrl Pts',(7.34093362208018,70.6137245834002,12.));
#160553=CARTESIAN_POINT('Ctrl Pts',(7.33217151437608,70.5936125421958,0.));
#160554=CARTESIAN_POINT('Ctrl Pts',(7.33217151437608,70.5936125421958,12.));
#160555=CARTESIAN_POINT('Ctrl Pts',(7.32344889945237,70.573535128649,0.));
#160556=CARTESIAN_POINT('Ctrl Pts',(7.32344889945237,70.573535128649,12.));
#160557=CARTESIAN_POINT('Ctrl Pts',(7.31476576940404,70.5534925092053,0.));
#160558=CARTESIAN_POINT('Ctrl Pts',(7.31476576940404,70.5534925092053,12.));
#160559=CARTESIAN_POINT('Ctrl Pts',(7.30612211618047,70.5334848511675,0.));
#160560=CARTESIAN_POINT('Ctrl Pts',(7.30612211618047,70.5334848511675,12.));
#160561=CARTESIAN_POINT('Ctrl Pts',(7.29751793157801,70.5135123227147,0.));
#160562=CARTESIAN_POINT('Ctrl Pts',(7.29751793157801,70.5135123227147,12.));
#160563=CARTESIAN_POINT('Ctrl Pts',(7.28895320723836,70.4935750929029,0.));
#160564=CARTESIAN_POINT('Ctrl Pts',(7.28895320723836,70.4935750929029,12.));
#160565=CARTESIAN_POINT('Ctrl Pts',(7.2804279346545,70.4736733316463,0.));
#160566=CARTESIAN_POINT('Ctrl Pts',(7.2804279346545,70.4736733316463,12.));
#160567=CARTESIAN_POINT('Ctrl Pts',(7.27194210517058,70.4538072096986,0.));
#160568=CARTESIAN_POINT('Ctrl Pts',(7.27194210517058,70.4538072096986,12.));
#160569=CARTESIAN_POINT('Ctrl Pts',(7.26349570998051,70.433976898636,0.));
#160570=CARTESIAN_POINT('Ctrl Pts',(7.26349570998051,70.433976898636,12.));
#160571=CARTESIAN_POINT('Ctrl Pts',(7.25508874012076,70.4141825708207,0.));
#160572=CARTESIAN_POINT('Ctrl Pts',(7.25508874012076,70.4141825708207,12.));
#160573=CARTESIAN_POINT('Ctrl Pts',(7.24672118647116,70.3944243994532,0.));
#160574=CARTESIAN_POINT('Ctrl Pts',(7.24672118647116,70.3944243994532,12.));
#160575=CARTESIAN_POINT('Ctrl Pts',(7.23839303975626,70.3747025586569,0.));
#160576=CARTESIAN_POINT('Ctrl Pts',(7.23839303975626,70.3747025586569,12.));
#160577=CARTESIAN_POINT('Ctrl Pts',(7.23010429054231,70.3550172235486,0.));
#160578=CARTESIAN_POINT('Ctrl Pts',(7.23010429054231,70.3550172235486,12.));
#160579=CARTESIAN_POINT('Ctrl Pts',(7.22185492923178,70.3353685703097,0.));
#160580=CARTESIAN_POINT('Ctrl Pts',(7.22185492923178,70.3353685703097,12.));
#160581=CARTESIAN_POINT('Ctrl Pts',(7.21364494605425,70.3157567762561,0.));
#160582=CARTESIAN_POINT('Ctrl Pts',(7.21364494605425,70.3157567762561,12.));
#160583=CARTESIAN_POINT('Ctrl Pts',(7.20547433107458,70.2961820197051,0.));
#160584=CARTESIAN_POINT('Ctrl Pts',(7.20547433107458,70.2961820197051,12.));
#160585=CARTESIAN_POINT('Ctrl Pts',(7.19734307419861,70.276644479827,0.));
#160586=CARTESIAN_POINT('Ctrl Pts',(7.19734307419861,70.276644479827,12.));
#160587=CARTESIAN_POINT('Ctrl Pts',(7.18925116517563,70.2571443365198,0.));
#160588=CARTESIAN_POINT('Ctrl Pts',(7.18925116517563,70.2571443365198,12.));
#160589=CARTESIAN_POINT('Ctrl Pts',(7.18119859359801,70.2376817702239,0.));
#160590=CARTESIAN_POINT('Ctrl Pts',(7.18119859359801,70.2376817702239,12.));
#160591=CARTESIAN_POINT('Ctrl Pts',(7.17318534889747,70.2182569619028,0.));
#160592=CARTESIAN_POINT('Ctrl Pts',(7.17318534889747,70.2182569619028,12.));
#160593=CARTESIAN_POINT('Ctrl Pts',(7.16521142033893,70.1988700934622,0.));
#160594=CARTESIAN_POINT('Ctrl Pts',(7.16521142033893,70.1988700934622,12.));
#160595=CARTESIAN_POINT('Ctrl Pts',(7.15727679700946,70.1795213481196,0.));
#160596=CARTESIAN_POINT('Ctrl Pts',(7.15727679700946,70.1795213481196,12.));
#160597=CARTESIAN_POINT('Ctrl Pts',(7.14938146780801,70.1602109107188,0.));
#160598=CARTESIAN_POINT('Ctrl Pts',(7.14938146780801,70.1602109107188,12.));
#160599=CARTESIAN_POINT('Ctrl Pts',(7.14152542142339,70.1409389682389,0.));
#160600=CARTESIAN_POINT('Ctrl Pts',(7.14152542142339,70.1409389682389,12.));
#160601=CARTESIAN_POINT('Ctrl Pts',(7.13370864634399,70.1217057094456,0.));
#160602=CARTESIAN_POINT('Ctrl Pts',(7.13370864634399,70.1217057094456,12.));
#160603=CARTESIAN_POINT('Ctrl Pts',(7.12593113088871,70.1025113239463,0.));
#160604=CARTESIAN_POINT('Ctrl Pts',(7.12593113088871,70.1025113239463,12.));
#160605=CARTESIAN_POINT('Ctrl Pts',(7.11819286322824,70.0833560013971,0.));
#160606=CARTESIAN_POINT('Ctrl Pts',(7.11819286322824,70.0833560013971,12.));
#160607=CARTESIAN_POINT('Ctrl Pts',(7.11049383140482,70.06423993069,0.));
#160608=CARTESIAN_POINT('Ctrl Pts',(7.11049383140482,70.06423993069,12.));
#160609=CARTESIAN_POINT('Ctrl Pts',(7.10283402335091,70.0451632990137,0.));
#160610=CARTESIAN_POINT('Ctrl Pts',(7.10283402335091,70.0451632990137,12.));
#160611=CARTESIAN_POINT('Ctrl Pts',(7.09521342684301,70.0261262936435,0.));
#160612=CARTESIAN_POINT('Ctrl Pts',(7.09521342684301,70.0261262936435,12.));
#160613=CARTESIAN_POINT('Ctrl Pts',(7.08763202944274,70.0071291040791,0.));
#160614=CARTESIAN_POINT('Ctrl Pts',(7.08763202944274,70.0071291040791,12.));
#160615=CARTESIAN_POINT('Ctrl Pts',(7.08008981844643,69.988171923787,0.));
#160616=CARTESIAN_POINT('Ctrl Pts',(7.08008981844643,69.988171923787,12.));
#160617=CARTESIAN_POINT('Ctrl Pts',(7.07258678080793,69.9692549527256,0.));
#160618=CARTESIAN_POINT('Ctrl Pts',(7.07258678080793,69.9692549527256,12.));
#160619=CARTESIAN_POINT('Ctrl Pts',(7.06512290312803,69.9503783975676,0.));
#160620=CARTESIAN_POINT('Ctrl Pts',(7.06512290312803,69.9503783975676,12.));
#160621=CARTESIAN_POINT('Ctrl Pts',(7.05769817180825,69.9315424664252,0.));
#160622=CARTESIAN_POINT('Ctrl Pts',(7.05769817180825,69.9315424664252,12.));
#160623=CARTESIAN_POINT('Ctrl Pts',(7.05031257318108,69.9127473642087,0.));
#160624=CARTESIAN_POINT('Ctrl Pts',(7.05031257318108,69.9127473642087,12.));
#160625=CARTESIAN_POINT('Ctrl Pts',(7.04296609362187,69.8939932885864,0.));
#160626=CARTESIAN_POINT('Ctrl Pts',(7.04296609362187,69.8939932885864,12.));
#160627=CARTESIAN_POINT('Ctrl Pts',(7.03565871972266,69.8752804235296,0.));
#160628=CARTESIAN_POINT('Ctrl Pts',(7.03565871972266,69.8752804235296,12.));
#160629=CARTESIAN_POINT('Ctrl Pts',(7.02839043811863,69.8566089455448,0.));
#160630=CARTESIAN_POINT('Ctrl Pts',(7.02839043811863,69.8566089455448,12.));
#160631=CARTESIAN_POINT('Ctrl Pts',(7.02116123514488,69.8379790360574,0.));
#160632=CARTESIAN_POINT('Ctrl Pts',(7.02116123514488,69.8379790360574,12.));
#160633=CARTESIAN_POINT('Ctrl Pts',(7.01397109655456,69.8193908913722,0.));
#160634=CARTESIAN_POINT('Ctrl Pts',(7.01397109655456,69.8193908913722,12.));
#160635=CARTESIAN_POINT('Ctrl Pts',(7.00682000718105,69.8008447346782,0.));
#160636=CARTESIAN_POINT('Ctrl Pts',(7.00682000718105,69.8008447346782,12.));
#160637=CARTESIAN_POINT('Ctrl Pts',(6.99970795069399,69.7823408242446,0.));
#160638=CARTESIAN_POINT('Ctrl Pts',(6.99970795069399,69.7823408242446,12.));
#160639=CARTESIAN_POINT('Ctrl Pts',(6.9926349102786,69.7638794280263,0.));
#160640=CARTESIAN_POINT('Ctrl Pts',(6.9926349102786,69.7638794280263,12.));
#160641=CARTESIAN_POINT('Ctrl Pts',(6.98560086924173,69.7454607995524,0.));
#160642=CARTESIAN_POINT('Ctrl Pts',(6.98560086924173,69.7454607995524,12.));
#160643=CARTESIAN_POINT('Ctrl Pts',(6.97860581164569,69.7270851557443,0.));
#160644=CARTESIAN_POINT('Ctrl Pts',(6.97860581164569,69.7270851557443,12.));
#160645=CARTESIAN_POINT('Ctrl Pts',(6.97164972291582,69.7087526480249,0.));
#160646=CARTESIAN_POINT('Ctrl Pts',(6.97164972291582,69.7087526480249,12.));
#160647=CARTESIAN_POINT('Ctrl Pts',(6.9647325904973,69.6904633605834,0.));
#160648=CARTESIAN_POINT('Ctrl Pts',(6.9647325904973,69.6904633605834,12.));
#160649=CARTESIAN_POINT('Ctrl Pts',(6.95923004173796,69.6758665380764,0.));
#160650=CARTESIAN_POINT('Ctrl Pts',(6.95923004173796,69.6758665380764,12.));
#160651=CARTESIAN_POINT('Ctrl Pts',(6.95512065317731,69.6649383920075,0.));
#160652=CARTESIAN_POINT('Ctrl Pts',(6.95512065317731,69.6649383920075,12.));
#160653=CARTESIAN_POINT('Ctrl Pts',(6.95238884849076,69.6576616146559,0.));
#160654=CARTESIAN_POINT('Ctrl Pts',(6.95238884849076,69.6576616146559,12.));
#160655=CARTESIAN_POINT('Ctrl Pts',(6.95102489306928,69.6540253893193,0.));
#160656=CARTESIAN_POINT('Ctrl Pts',(6.95102489306928,69.6540253893193,12.));
#160657=CARTESIAN_POINT('',(6.95102489306928,69.6540253893193,12.));
#160658=CARTESIAN_POINT('Ctrl Pts',(6.95102489306928,69.6540253893193,12.));
#160659=CARTESIAN_POINT('Ctrl Pts',(6.95238884849076,69.6576616146559,12.));
#160660=CARTESIAN_POINT('Ctrl Pts',(6.95512065317731,69.6649383920075,12.));
#160661=CARTESIAN_POINT('Ctrl Pts',(6.95923004173796,69.6758665380764,12.));
#160662=CARTESIAN_POINT('Ctrl Pts',(6.9647325904973,69.6904633605834,12.));
#160663=CARTESIAN_POINT('Ctrl Pts',(6.97164972291582,69.7087526480249,12.));
#160664=CARTESIAN_POINT('Ctrl Pts',(6.97860581164569,69.7270851557443,12.));
#160665=CARTESIAN_POINT('Ctrl Pts',(6.98560086924173,69.7454607995524,12.));
#160666=CARTESIAN_POINT('Ctrl Pts',(6.9926349102786,69.7638794280263,12.));
#160667=CARTESIAN_POINT('Ctrl Pts',(6.99970795069399,69.7823408242446,12.));
#160668=CARTESIAN_POINT('Ctrl Pts',(7.00682000718105,69.8008447346782,12.));
#160669=CARTESIAN_POINT('Ctrl Pts',(7.01397109655456,69.8193908913722,12.));
#160670=CARTESIAN_POINT('Ctrl Pts',(7.02116123514488,69.8379790360574,12.));
#160671=CARTESIAN_POINT('Ctrl Pts',(7.02839043811863,69.8566089455448,12.));
#160672=CARTESIAN_POINT('Ctrl Pts',(7.03565871972266,69.8752804235296,12.));
#160673=CARTESIAN_POINT('Ctrl Pts',(7.04296609362187,69.8939932885864,12.));
#160674=CARTESIAN_POINT('Ctrl Pts',(7.05031257318108,69.9127473642087,12.));
#160675=CARTESIAN_POINT('Ctrl Pts',(7.05769817180825,69.9315424664252,12.));
#160676=CARTESIAN_POINT('Ctrl Pts',(7.06512290312803,69.9503783975676,12.));
#160677=CARTESIAN_POINT('Ctrl Pts',(7.07258678080793,69.9692549527256,12.));
#160678=CARTESIAN_POINT('Ctrl Pts',(7.08008981844643,69.988171923787,12.));
#160679=CARTESIAN_POINT('Ctrl Pts',(7.08763202944274,70.0071291040791,12.));
#160680=CARTESIAN_POINT('Ctrl Pts',(7.09521342684301,70.0261262936435,12.));
#160681=CARTESIAN_POINT('Ctrl Pts',(7.10283402335091,70.0451632990137,12.));
#160682=CARTESIAN_POINT('Ctrl Pts',(7.11049383140482,70.06423993069,12.));
#160683=CARTESIAN_POINT('Ctrl Pts',(7.11819286322824,70.0833560013971,12.));
#160684=CARTESIAN_POINT('Ctrl Pts',(7.12593113088871,70.1025113239463,12.));
#160685=CARTESIAN_POINT('Ctrl Pts',(7.13370864634399,70.1217057094456,12.));
#160686=CARTESIAN_POINT('Ctrl Pts',(7.14152542142339,70.1409389682389,12.));
#160687=CARTESIAN_POINT('Ctrl Pts',(7.14938146780801,70.1602109107188,12.));
#160688=CARTESIAN_POINT('Ctrl Pts',(7.15727679700946,70.1795213481196,12.));
#160689=CARTESIAN_POINT('Ctrl Pts',(7.16521142033893,70.1988700934622,12.));
#160690=CARTESIAN_POINT('Ctrl Pts',(7.17318534889747,70.2182569619028,12.));
#160691=CARTESIAN_POINT('Ctrl Pts',(7.18119859359801,70.2376817702239,12.));
#160692=CARTESIAN_POINT('Ctrl Pts',(7.18925116517563,70.2571443365198,12.));
#160693=CARTESIAN_POINT('Ctrl Pts',(7.19734307419861,70.276644479827,12.));
#160694=CARTESIAN_POINT('Ctrl Pts',(7.20547433107458,70.2961820197051,12.));
#160695=CARTESIAN_POINT('Ctrl Pts',(7.21364494605425,70.3157567762561,12.));
#160696=CARTESIAN_POINT('Ctrl Pts',(7.22185492923178,70.3353685703097,12.));
#160697=CARTESIAN_POINT('Ctrl Pts',(7.23010429054231,70.3550172235486,12.));
#160698=CARTESIAN_POINT('Ctrl Pts',(7.23839303975626,70.3747025586569,12.));
#160699=CARTESIAN_POINT('Ctrl Pts',(7.24672118647116,70.3944243994532,12.));
#160700=CARTESIAN_POINT('Ctrl Pts',(7.25508874012076,70.4141825708207,12.));
#160701=CARTESIAN_POINT('Ctrl Pts',(7.26349570998051,70.433976898636,12.));
#160702=CARTESIAN_POINT('Ctrl Pts',(7.27194210517058,70.4538072096986,12.));
#160703=CARTESIAN_POINT('Ctrl Pts',(7.2804279346545,70.4736733316463,12.));
#160704=CARTESIAN_POINT('Ctrl Pts',(7.28895320723836,70.4935750929029,12.));
#160705=CARTESIAN_POINT('Ctrl Pts',(7.29751793157801,70.5135123227147,12.));
#160706=CARTESIAN_POINT('Ctrl Pts',(7.30612211618047,70.5334848511675,12.));
#160707=CARTESIAN_POINT('Ctrl Pts',(7.31476576940404,70.5534925092053,12.));
#160708=CARTESIAN_POINT('Ctrl Pts',(7.32344889945237,70.573535128649,12.));
#160709=CARTESIAN_POINT('Ctrl Pts',(7.33217151437608,70.5936125421958,12.));
#160710=CARTESIAN_POINT('Ctrl Pts',(7.34093362208018,70.6137245834002,12.));
#160711=CARTESIAN_POINT('Ctrl Pts',(7.34973523032581,70.6338710866562,12.));
#160712=CARTESIAN_POINT('Ctrl Pts',(7.35857634673052,70.6540518871772,12.));
#160713=CARTESIAN_POINT('Ctrl Pts',(7.36745697876295,70.6742668209685,12.));
#160714=CARTESIAN_POINT('Ctrl Pts',(7.37637713374761,70.6945157248269,12.));
#160715=CARTESIAN_POINT('Ctrl Pts',(7.38533681887028,70.7147984363423,12.));
#160716=CARTESIAN_POINT('Ctrl Pts',(7.39433604117891,70.735114793895,12.));
#160717=CARTESIAN_POINT('Ctrl Pts',(7.40337480758237,70.7554646366514,12.));
#160718=CARTESIAN_POINT('Ctrl Pts',(7.41245312484498,70.7758478045576,12.));
#160719=CARTESIAN_POINT('Ctrl Pts',(7.42157099959326,70.796264138335,12.));
#160720=CARTESIAN_POINT('Ctrl Pts',(7.43072843832015,70.8167134794737,12.));
#160721=CARTESIAN_POINT('Ctrl Pts',(7.43992544738606,70.8371956702241,12.));
#160722=CARTESIAN_POINT('Ctrl Pts',(7.44916203301648,70.8577105535848,12.));
#160723=CARTESIAN_POINT('Ctrl Pts',(7.45843820129782,70.87825797329,12.));
#160724=CARTESIAN_POINT('Ctrl Pts',(7.46775395818527,70.8988377738104,12.));
#160725=CARTESIAN_POINT('Ctrl Pts',(7.47710930950563,70.9194498003493,12.));
#160726=CARTESIAN_POINT('Ctrl Pts',(7.48650426095824,70.940093898837,12.));
#160727=CARTESIAN_POINT('Ctrl Pts',(7.4959388181113,70.9607699159218,12.));
#160728=CARTESIAN_POINT('Ctrl Pts',(7.50541298639928,70.9814776989612,12.));
#160729=CARTESIAN_POINT('Ctrl Pts',(7.51492677113091,71.002217096021,12.));
#160730=CARTESIAN_POINT('Ctrl Pts',(7.52448017749125,71.0229879558699,12.));
#160731=CARTESIAN_POINT('Ctrl Pts',(7.53407321054263,71.043790127973,12.));
#160732=CARTESIAN_POINT('Ctrl Pts',(7.5437058752198,71.0646234624811,12.));
#160733=CARTESIAN_POINT('Ctrl Pts',(7.55337817632917,71.0854878102243,12.));
#160734=CARTESIAN_POINT('Ctrl Pts',(7.56309011855657,71.106383022711,12.));
#160735=CARTESIAN_POINT('Ctrl Pts',(7.57284170646886,71.1273089521234,12.));
#160736=CARTESIAN_POINT('Ctrl Pts',(7.58263294451452,71.1482654513119,12.));
#160737=CARTESIAN_POINT('Ctrl Pts',(7.59246383701814,71.1692523737844,12.));
#160738=CARTESIAN_POINT('Ctrl Pts',(7.60233438818097,71.1902695737013,12.));
#160739=CARTESIAN_POINT('Ctrl Pts',(7.61224460208838,71.211316905874,12.));
#160740=CARTESIAN_POINT('Ctrl Pts',(7.62219448271109,71.2323942257609,12.));
#160741=CARTESIAN_POINT('Ctrl Pts',(7.63218403390538,71.2535013894602,12.));
#160742=CARTESIAN_POINT('Ctrl Pts',(7.64221325940725,71.2746382537007,12.));
#160743=CARTESIAN_POINT('Ctrl Pts',(7.65228216283404,71.2958046758372,12.));
#160744=CARTESIAN_POINT('Ctrl Pts',(7.66239074769163,71.3170005138502,12.));
#160745=CARTESIAN_POINT('Ctrl Pts',(7.67253901737553,71.3382256263414,12.));
#160746=CARTESIAN_POINT('Ctrl Pts',(7.68272697517086,71.3594798725281,12.));
#160747=CARTESIAN_POINT('Ctrl Pts',(7.69295462424612,71.3807631122331,12.));
#160748=CARTESIAN_POINT('Ctrl Pts',(7.70322196765539,71.4020752058796,12.));
#160749=CARTESIAN_POINT('Ctrl Pts',(7.7135290083452,71.4234160144925,12.));
#160750=CARTESIAN_POINT('Ctrl Pts',(7.72387574915544,71.4447853996916,12.));
#160751=CARTESIAN_POINT('Ctrl Pts',(7.7342621928194,71.4661832236888,12.));
#160752=CARTESIAN_POINT('Ctrl Pts',(7.74468834195746,71.4876093492781,12.));
#160753=CARTESIAN_POINT('Ctrl Pts',(7.75515419907967,71.5090636398318,12.));
#160754=CARTESIAN_POINT('Ctrl Pts',(7.76565976659226,71.5305459592994,12.));
#160755=CARTESIAN_POINT('Ctrl Pts',(7.7762050467987,71.5520561722039,12.));
#160756=CARTESIAN_POINT('Ctrl Pts',(7.78679004189935,71.5735941436364,12.));
#160757=CARTESIAN_POINT('Ctrl Pts',(7.79741475398514,71.5951597392471,12.));
#160758=CARTESIAN_POINT('Ctrl Pts',(7.80807918504022,71.6167528252423,12.));
#160759=CARTESIAN_POINT('Ctrl Pts',(7.81878333694861,71.6383732683844,12.));
#160760=CARTESIAN_POINT('Ctrl Pts',(7.82952721149508,71.6600209359872,12.));
#160761=CARTESIAN_POINT('Ctrl Pts',(7.8403108103649,71.6816956959117,12.));
#160762=CARTESIAN_POINT('Ctrl Pts',(7.85113413513736,71.7033974165568,12.));
#160763=CARTESIAN_POINT('Ctrl Pts',(7.86199718728826,71.7251259668563,12.));
#160764=CARTESIAN_POINT('Ctrl Pts',(7.87289996819654,71.7468812162788,12.));
#160765=CARTESIAN_POINT('Ctrl Pts',(7.88384247914524,71.7686630348238,12.));
#160766=CARTESIAN_POINT('Ctrl Pts',(7.89482472132137,71.7904712930175,12.));
#160767=CARTESIAN_POINT('Ctrl Pts',(7.90584669580956,71.8123058619042,12.));
#160768=CARTESIAN_POINT('Ctrl Pts',(7.91690840359367,71.8341666130426,12.));
#160769=CARTESIAN_POINT('Ctrl Pts',(7.92800984556396,71.8560534185071,12.));
#160770=CARTESIAN_POINT('Ctrl Pts',(7.93915102251795,71.8779661508832,12.));
#160771=CARTESIAN_POINT('Ctrl Pts',(7.95033193516051,71.8999046832643,12.));
#160772=CARTESIAN_POINT('Ctrl Pts',(7.96155258409764,71.9218688892431,12.));
#160773=CARTESIAN_POINT('Ctrl Pts',(7.97281296983718,71.9438586429081,12.));
#160774=CARTESIAN_POINT('Ctrl Pts',(7.98411309279613,71.965873818843,12.));
#160775=CARTESIAN_POINT('Ctrl Pts',(7.99545295330191,71.9879142921254,12.));
#160776=CARTESIAN_POINT('Ctrl Pts',(8.00683255159248,72.0099799383213,12.));
#160777=CARTESIAN_POINT('Ctrl Pts',(8.01825188781057,72.032070633479,12.));
#160778=CARTESIAN_POINT('Ctrl Pts',(8.02971096200308,72.0541862541243,12.));
#160779=CARTESIAN_POINT('Ctrl Pts',(8.04120977412872,72.0763266772615,12.));
#160780=CARTESIAN_POINT('Ctrl Pts',(8.05274832405949,72.0984917803693,12.));
#160781=CARTESIAN_POINT('Ctrl Pts',(8.06432661158096,72.1206814413988,12.));
#160782=CARTESIAN_POINT('Ctrl Pts',(8.07594463638719,72.1428955387663,12.));
#160783=CARTESIAN_POINT('Ctrl Pts',(8.08760239807837,72.1651339513477,12.));
#160784=CARTESIAN_POINT('Ctrl Pts',(8.0992998961689,72.1873965584813,12.));
#160785=CARTESIAN_POINT('Ctrl Pts',(8.11103713008928,72.209683239963,12.));
#160786=CARTESIAN_POINT('Ctrl Pts',(8.12281409918661,72.2319938760449,12.));
#160787=CARTESIAN_POINT('Ctrl Pts',(8.13463080272029,72.2543283474278,12.));
#160788=CARTESIAN_POINT('Ctrl Pts',(8.14648723985798,72.2766865352555,12.));
#160789=CARTESIAN_POINT('Ctrl Pts',(8.15838340968336,72.2990683211162,12.));
#160790=CARTESIAN_POINT('Ctrl Pts',(8.17031931119891,72.3214735870409,12.));
#160791=CARTESIAN_POINT('Ctrl Pts',(8.18229494332624,72.3439022155007,12.));
#160792=CARTESIAN_POINT('Ctrl Pts',(8.19431030490315,72.3663540894026,12.));
#160793=CARTESIAN_POINT('Ctrl Pts',(8.20636539467776,72.3888290920832,12.));
#160794=CARTESIAN_POINT('Ctrl Pts',(8.21846021131561,72.4113271073079,12.));
#160795=CARTESIAN_POINT('Ctrl Pts',(8.23059475340357,72.4338480192695,12.));
#160796=CARTESIAN_POINT('Ctrl Pts',(8.2427690194504,72.4563917125842,12.));
#160797=CARTESIAN_POINT('Ctrl Pts',(8.25498300788494,72.4789580722875,12.));
#160798=CARTESIAN_POINT('Ctrl Pts',(8.2672367170492,72.5015469838254,12.));
#160799=CARTESIAN_POINT('Ctrl Pts',(8.27953014520376,72.5241583330562,12.));
#160800=CARTESIAN_POINT('Ctrl Pts',(8.29186329053279,72.5467920062521,12.));
#160801=CARTESIAN_POINT('Ctrl Pts',(8.30423615114453,72.5694478900982,12.));
#160802=CARTESIAN_POINT('Ctrl Pts',(8.31664872507017,72.5921258716901,12.));
#160803=CARTESIAN_POINT('Ctrl Pts',(8.32910101025671,72.6148258385296,12.));
#160804=CARTESIAN_POINT('Ctrl Pts',(8.34159300456987,72.6375476785215,12.));
#160805=CARTESIAN_POINT('Ctrl Pts',(8.35412470580102,72.6602912799696,12.));
#160806=CARTESIAN_POINT('Ctrl Pts',(8.36669611166843,72.6830565315703,12.));
#160807=CARTESIAN_POINT('Ctrl Pts',(8.37930721981731,72.705843322407,12.));
#160808=CARTESIAN_POINT('Ctrl Pts',(8.39195802781391,72.7286515419373,12.));
#160809=CARTESIAN_POINT('Ctrl Pts',(8.40464853314469,72.751481079992,12.));
#160810=CARTESIAN_POINT('Ctrl Pts',(8.4173787332233,72.7743318267865,12.));
#160811=CARTESIAN_POINT('Ctrl Pts',(8.43014862539158,72.7972036729276,12.));
#160812=CARTESIAN_POINT('Ctrl Pts',(8.44295820691912,72.8200965094199,12.));
#160813=CARTESIAN_POINT('Ctrl Pts',(8.45580747499793,72.8430102276713,12.));
#160814=CARTESIAN_POINT('Ctrl Pts',(8.46869642673795,72.8659447194933,12.));
#160815=CARTESIAN_POINT('Ctrl Pts',(8.48162505917658,72.8888998770785,12.));
#160816=CARTESIAN_POINT('Ctrl Pts',(8.49459336928296,72.9118755929795,12.));
#160817=CARTESIAN_POINT('Ctrl Pts',(8.50760135395984,72.9348717600838,12.));
#160818=CARTESIAN_POINT('Ctrl Pts',(8.52064901004228,72.9578882715912,12.));
#160819=CARTESIAN_POINT('Ctrl Pts',(8.53373633429281,72.9809250209828,12.));
#160820=CARTESIAN_POINT('Ctrl Pts',(8.54686332340418,73.0039819020648,12.));
#160821=CARTESIAN_POINT('Ctrl Pts',(8.56002997400084,73.0270588090183,12.));
#160822=CARTESIAN_POINT('Ctrl Pts',(8.57323628263593,73.0501556364479,12.));
#160823=CARTESIAN_POINT('Ctrl Pts',(8.58648224578732,73.0732722794195,12.));
#160824=CARTESIAN_POINT('Ctrl Pts',(8.59976785984552,73.0964086335235,12.));
#160825=CARTESIAN_POINT('Ctrl Pts',(8.61309312112002,73.1195645948178,12.));
#160826=CARTESIAN_POINT('Ctrl Pts',(8.62645802585484,73.1427400597037,12.));
#160827=CARTESIAN_POINT('Ctrl Pts',(8.63986257023739,73.1659349248133,12.));
#160828=CARTESIAN_POINT('Ctrl Pts',(8.65330675040537,73.1891490869056,12.));
#160829=CARTESIAN_POINT('Ctrl Pts',(8.66679056245092,73.2123824427208,12.));
#160830=CARTESIAN_POINT('Ctrl Pts',(8.68031400241872,73.2356348889693,12.));
#160831=CARTESIAN_POINT('Ctrl Pts',(8.69387706629286,73.2589063226358,12.));
#160832=CARTESIAN_POINT('Ctrl Pts',(8.7074797499823,73.2821966412148,12.));
#160833=CARTESIAN_POINT('Ctrl Pts',(8.72112204930232,73.3055057429742,12.));
#160834=CARTESIAN_POINT('Ctrl Pts',(8.7348039599538,73.3288335272002,12.));
#160835=CARTESIAN_POINT('Ctrl Pts',(8.74852547749778,73.3521798944622,12.));
#160836=CARTESIAN_POINT('Ctrl Pts',(8.76228659740358,73.3755447460269,12.));
#160837=CARTESIAN_POINT('Ctrl Pts',(8.77608731509348,73.3989279832835,12.));
#160838=CARTESIAN_POINT('Ctrl Pts',(8.78992762598757,73.422329507113,12.));
#160839=CARTESIAN_POINT('Ctrl Pts',(8.80380752553692,73.4457492173933,12.));
#160840=CARTESIAN_POINT('Ctrl Pts',(8.81772700927531,73.4691870121567,12.));
#160841=CARTESIAN_POINT('Ctrl Pts',(8.83168607277326,73.492642788273,12.));
#160842=CARTESIAN_POINT('Ctrl Pts',(8.84568471153806,73.5161164429709,12.));
#160843=CARTESIAN_POINT('Ctrl Pts',(8.85972292092131,73.5396078751639,12.));
#160844=CARTESIAN_POINT('Ctrl Pts',(8.87380069602971,73.5631169867122,12.));
#160845=CARTESIAN_POINT('Ctrl Pts',(8.88791803160443,73.5866436840556,12.));
#160846=CARTESIAN_POINT('Ctrl Pts',(8.90207492199043,73.6101878785976,12.));
#160847=CARTESIAN_POINT('Ctrl Pts',(8.91424402151598,73.6303847393629,12.));
#160848=CARTESIAN_POINT('Ctrl Pts',(8.9235951817849,73.6458786306023,12.));
#160849=CARTESIAN_POINT('Ctrl Pts',(8.93011088817314,73.6566618622074,12.));
#160850=CARTESIAN_POINT('Ctrl Pts',(8.93377955965632,73.6627293782587,12.));
#160851=CARTESIAN_POINT('Ctrl Pts',(8.93459554657838,73.6640787198055,12.));
#160852=CARTESIAN_POINT('',(6.95102489306928,69.6540253893193,0.));
#160853=CARTESIAN_POINT('',(6.95102489306928,69.6540253893193,0.));
#160854=CARTESIAN_POINT('Ctrl Pts',(8.93459554657838,73.6640787198055,0.));
#160855=CARTESIAN_POINT('Ctrl Pts',(8.93377955965632,73.6627293782587,0.));
#160856=CARTESIAN_POINT('Ctrl Pts',(8.93011088817314,73.6566618622074,0.));
#160857=CARTESIAN_POINT('Ctrl Pts',(8.9235951817849,73.6458786306023,0.));
#160858=CARTESIAN_POINT('Ctrl Pts',(8.91424402151598,73.6303847393629,0.));
#160859=CARTESIAN_POINT('Ctrl Pts',(8.90207492199043,73.6101878785976,0.));
#160860=CARTESIAN_POINT('Ctrl Pts',(8.88791803160443,73.5866436840556,0.));
#160861=CARTESIAN_POINT('Ctrl Pts',(8.87380069602971,73.5631169867122,0.));
#160862=CARTESIAN_POINT('Ctrl Pts',(8.85972292092131,73.5396078751639,0.));
#160863=CARTESIAN_POINT('Ctrl Pts',(8.84568471153806,73.5161164429709,0.));
#160864=CARTESIAN_POINT('Ctrl Pts',(8.83168607277326,73.492642788273,0.));
#160865=CARTESIAN_POINT('Ctrl Pts',(8.81772700927531,73.4691870121567,0.));
#160866=CARTESIAN_POINT('Ctrl Pts',(8.80380752553692,73.4457492173933,0.));
#160867=CARTESIAN_POINT('Ctrl Pts',(8.78992762598757,73.422329507113,0.));
#160868=CARTESIAN_POINT('Ctrl Pts',(8.77608731509348,73.3989279832835,0.));
#160869=CARTESIAN_POINT('Ctrl Pts',(8.76228659740358,73.3755447460269,0.));
#160870=CARTESIAN_POINT('Ctrl Pts',(8.74852547749778,73.3521798944622,0.));
#160871=CARTESIAN_POINT('Ctrl Pts',(8.7348039599538,73.3288335272002,0.));
#160872=CARTESIAN_POINT('Ctrl Pts',(8.72112204930232,73.3055057429742,0.));
#160873=CARTESIAN_POINT('Ctrl Pts',(8.7074797499823,73.2821966412148,0.));
#160874=CARTESIAN_POINT('Ctrl Pts',(8.69387706629286,73.2589063226358,0.));
#160875=CARTESIAN_POINT('Ctrl Pts',(8.68031400241872,73.2356348889693,0.));
#160876=CARTESIAN_POINT('Ctrl Pts',(8.66679056245092,73.2123824427208,0.));
#160877=CARTESIAN_POINT('Ctrl Pts',(8.65330675040537,73.1891490869056,0.));
#160878=CARTESIAN_POINT('Ctrl Pts',(8.63986257023739,73.1659349248133,0.));
#160879=CARTESIAN_POINT('Ctrl Pts',(8.62645802585484,73.1427400597037,0.));
#160880=CARTESIAN_POINT('Ctrl Pts',(8.61309312112002,73.1195645948178,0.));
#160881=CARTESIAN_POINT('Ctrl Pts',(8.59976785984552,73.0964086335235,0.));
#160882=CARTESIAN_POINT('Ctrl Pts',(8.58648224578732,73.0732722794195,0.));
#160883=CARTESIAN_POINT('Ctrl Pts',(8.57323628263593,73.0501556364479,0.));
#160884=CARTESIAN_POINT('Ctrl Pts',(8.56002997400084,73.0270588090183,0.));
#160885=CARTESIAN_POINT('Ctrl Pts',(8.54686332340418,73.0039819020648,0.));
#160886=CARTESIAN_POINT('Ctrl Pts',(8.53373633429281,72.9809250209828,0.));
#160887=CARTESIAN_POINT('Ctrl Pts',(8.52064901004228,72.9578882715912,0.));
#160888=CARTESIAN_POINT('Ctrl Pts',(8.50760135395984,72.9348717600838,0.));
#160889=CARTESIAN_POINT('Ctrl Pts',(8.49459336928296,72.9118755929795,0.));
#160890=CARTESIAN_POINT('Ctrl Pts',(8.48162505917658,72.8888998770785,0.));
#160891=CARTESIAN_POINT('Ctrl Pts',(8.46869642673795,72.8659447194933,0.));
#160892=CARTESIAN_POINT('Ctrl Pts',(8.45580747499793,72.8430102276713,0.));
#160893=CARTESIAN_POINT('Ctrl Pts',(8.44295820691912,72.8200965094199,0.));
#160894=CARTESIAN_POINT('Ctrl Pts',(8.43014862539158,72.7972036729276,0.));
#160895=CARTESIAN_POINT('Ctrl Pts',(8.4173787332233,72.7743318267865,0.));
#160896=CARTESIAN_POINT('Ctrl Pts',(8.40464853314469,72.751481079992,0.));
#160897=CARTESIAN_POINT('Ctrl Pts',(8.39195802781391,72.7286515419373,0.));
#160898=CARTESIAN_POINT('Ctrl Pts',(8.37930721981731,72.705843322407,0.));
#160899=CARTESIAN_POINT('Ctrl Pts',(8.36669611166843,72.6830565315703,0.));
#160900=CARTESIAN_POINT('Ctrl Pts',(8.35412470580102,72.6602912799696,0.));
#160901=CARTESIAN_POINT('Ctrl Pts',(8.34159300456987,72.6375476785215,0.));
#160902=CARTESIAN_POINT('Ctrl Pts',(8.32910101025671,72.6148258385296,0.));
#160903=CARTESIAN_POINT('Ctrl Pts',(8.31664872507017,72.5921258716901,0.));
#160904=CARTESIAN_POINT('Ctrl Pts',(8.30423615114453,72.5694478900982,0.));
#160905=CARTESIAN_POINT('Ctrl Pts',(8.29186329053279,72.5467920062521,0.));
#160906=CARTESIAN_POINT('Ctrl Pts',(8.27953014520376,72.5241583330562,0.));
#160907=CARTESIAN_POINT('Ctrl Pts',(8.2672367170492,72.5015469838254,0.));
#160908=CARTESIAN_POINT('Ctrl Pts',(8.25498300788494,72.4789580722875,0.));
#160909=CARTESIAN_POINT('Ctrl Pts',(8.2427690194504,72.4563917125842,0.));
#160910=CARTESIAN_POINT('Ctrl Pts',(8.23059475340357,72.4338480192695,0.));
#160911=CARTESIAN_POINT('Ctrl Pts',(8.21846021131561,72.4113271073079,0.));
#160912=CARTESIAN_POINT('Ctrl Pts',(8.20636539467776,72.3888290920832,0.));
#160913=CARTESIAN_POINT('Ctrl Pts',(8.19431030490315,72.3663540894026,0.));
#160914=CARTESIAN_POINT('Ctrl Pts',(8.18229494332624,72.3439022155007,0.));
#160915=CARTESIAN_POINT('Ctrl Pts',(8.17031931119891,72.3214735870409,0.));
#160916=CARTESIAN_POINT('Ctrl Pts',(8.15838340968336,72.2990683211162,0.));
#160917=CARTESIAN_POINT('Ctrl Pts',(8.14648723985798,72.2766865352555,0.));
#160918=CARTESIAN_POINT('Ctrl Pts',(8.13463080272029,72.2543283474278,0.));
#160919=CARTESIAN_POINT('Ctrl Pts',(8.12281409918661,72.2319938760449,0.));
#160920=CARTESIAN_POINT('Ctrl Pts',(8.11103713008928,72.209683239963,0.));
#160921=CARTESIAN_POINT('Ctrl Pts',(8.0992998961689,72.1873965584813,0.));
#160922=CARTESIAN_POINT('Ctrl Pts',(8.08760239807837,72.1651339513477,0.));
#160923=CARTESIAN_POINT('Ctrl Pts',(8.07594463638719,72.1428955387663,0.));
#160924=CARTESIAN_POINT('Ctrl Pts',(8.06432661158096,72.1206814413988,0.));
#160925=CARTESIAN_POINT('Ctrl Pts',(8.05274832405949,72.0984917803693,0.));
#160926=CARTESIAN_POINT('Ctrl Pts',(8.04120977412872,72.0763266772615,0.));
#160927=CARTESIAN_POINT('Ctrl Pts',(8.02971096200308,72.0541862541243,0.));
#160928=CARTESIAN_POINT('Ctrl Pts',(8.01825188781057,72.032070633479,0.));
#160929=CARTESIAN_POINT('Ctrl Pts',(8.00683255159248,72.0099799383213,0.));
#160930=CARTESIAN_POINT('Ctrl Pts',(7.99545295330191,71.9879142921254,0.));
#160931=CARTESIAN_POINT('Ctrl Pts',(7.98411309279613,71.965873818843,0.));
#160932=CARTESIAN_POINT('Ctrl Pts',(7.97281296983718,71.9438586429081,0.));
#160933=CARTESIAN_POINT('Ctrl Pts',(7.96155258409764,71.9218688892431,0.));
#160934=CARTESIAN_POINT('Ctrl Pts',(7.95033193516051,71.8999046832643,0.));
#160935=CARTESIAN_POINT('Ctrl Pts',(7.93915102251795,71.8779661508832,0.));
#160936=CARTESIAN_POINT('Ctrl Pts',(7.92800984556396,71.8560534185071,0.));
#160937=CARTESIAN_POINT('Ctrl Pts',(7.91690840359367,71.8341666130426,0.));
#160938=CARTESIAN_POINT('Ctrl Pts',(7.90584669580956,71.8123058619042,0.));
#160939=CARTESIAN_POINT('Ctrl Pts',(7.89482472132137,71.7904712930175,0.));
#160940=CARTESIAN_POINT('Ctrl Pts',(7.88384247914524,71.7686630348238,0.));
#160941=CARTESIAN_POINT('Ctrl Pts',(7.87289996819654,71.7468812162788,0.));
#160942=CARTESIAN_POINT('Ctrl Pts',(7.86199718728826,71.7251259668563,0.));
#160943=CARTESIAN_POINT('Ctrl Pts',(7.85113413513736,71.7033974165568,0.));
#160944=CARTESIAN_POINT('Ctrl Pts',(7.8403108103649,71.6816956959117,0.));
#160945=CARTESIAN_POINT('Ctrl Pts',(7.82952721149508,71.6600209359872,0.));
#160946=CARTESIAN_POINT('Ctrl Pts',(7.81878333694861,71.6383732683844,0.));
#160947=CARTESIAN_POINT('Ctrl Pts',(7.80807918504022,71.6167528252423,0.));
#160948=CARTESIAN_POINT('Ctrl Pts',(7.79741475398514,71.5951597392471,0.));
#160949=CARTESIAN_POINT('Ctrl Pts',(7.78679004189935,71.5735941436364,0.));
#160950=CARTESIAN_POINT('Ctrl Pts',(7.7762050467987,71.5520561722039,0.));
#160951=CARTESIAN_POINT('Ctrl Pts',(7.76565976659226,71.5305459592994,0.));
#160952=CARTESIAN_POINT('Ctrl Pts',(7.75515419907967,71.5090636398318,0.));
#160953=CARTESIAN_POINT('Ctrl Pts',(7.74468834195746,71.4876093492781,0.));
#160954=CARTESIAN_POINT('Ctrl Pts',(7.7342621928194,71.4661832236888,0.));
#160955=CARTESIAN_POINT('Ctrl Pts',(7.72387574915544,71.4447853996916,0.));
#160956=CARTESIAN_POINT('Ctrl Pts',(7.7135290083452,71.4234160144925,0.));
#160957=CARTESIAN_POINT('Ctrl Pts',(7.70322196765539,71.4020752058796,0.));
#160958=CARTESIAN_POINT('Ctrl Pts',(7.69295462424612,71.3807631122331,0.));
#160959=CARTESIAN_POINT('Ctrl Pts',(7.68272697517086,71.3594798725281,0.));
#160960=CARTESIAN_POINT('Ctrl Pts',(7.67253901737553,71.3382256263414,0.));
#160961=CARTESIAN_POINT('Ctrl Pts',(7.66239074769163,71.3170005138502,0.));
#160962=CARTESIAN_POINT('Ctrl Pts',(7.65228216283404,71.2958046758372,0.));
#160963=CARTESIAN_POINT('Ctrl Pts',(7.64221325940725,71.2746382537007,0.));
#160964=CARTESIAN_POINT('Ctrl Pts',(7.63218403390538,71.2535013894602,0.));
#160965=CARTESIAN_POINT('Ctrl Pts',(7.62219448271109,71.2323942257609,0.));
#160966=CARTESIAN_POINT('Ctrl Pts',(7.61224460208838,71.211316905874,0.));
#160967=CARTESIAN_POINT('Ctrl Pts',(7.60233438818097,71.1902695737013,0.));
#160968=CARTESIAN_POINT('Ctrl Pts',(7.59246383701814,71.1692523737844,0.));
#160969=CARTESIAN_POINT('Ctrl Pts',(7.58263294451452,71.1482654513119,0.));
#160970=CARTESIAN_POINT('Ctrl Pts',(7.57284170646886,71.1273089521234,0.));
#160971=CARTESIAN_POINT('Ctrl Pts',(7.56309011855657,71.106383022711,0.));
#160972=CARTESIAN_POINT('Ctrl Pts',(7.55337817632917,71.0854878102243,0.));
#160973=CARTESIAN_POINT('Ctrl Pts',(7.5437058752198,71.0646234624811,0.));
#160974=CARTESIAN_POINT('Ctrl Pts',(7.53407321054263,71.043790127973,0.));
#160975=CARTESIAN_POINT('Ctrl Pts',(7.52448017749125,71.0229879558699,0.));
#160976=CARTESIAN_POINT('Ctrl Pts',(7.51492677113091,71.002217096021,0.));
#160977=CARTESIAN_POINT('Ctrl Pts',(7.50541298639928,70.9814776989612,0.));
#160978=CARTESIAN_POINT('Ctrl Pts',(7.4959388181113,70.9607699159218,0.));
#160979=CARTESIAN_POINT('Ctrl Pts',(7.48650426095824,70.940093898837,0.));
#160980=CARTESIAN_POINT('Ctrl Pts',(7.47710930950563,70.9194498003493,0.));
#160981=CARTESIAN_POINT('Ctrl Pts',(7.46775395818527,70.8988377738104,0.));
#160982=CARTESIAN_POINT('Ctrl Pts',(7.45843820129782,70.87825797329,0.));
#160983=CARTESIAN_POINT('Ctrl Pts',(7.44916203301648,70.8577105535848,0.));
#160984=CARTESIAN_POINT('Ctrl Pts',(7.43992544738606,70.8371956702241,0.));
#160985=CARTESIAN_POINT('Ctrl Pts',(7.43072843832015,70.8167134794737,0.));
#160986=CARTESIAN_POINT('Ctrl Pts',(7.42157099959326,70.796264138335,0.));
#160987=CARTESIAN_POINT('Ctrl Pts',(7.41245312484498,70.7758478045576,0.));
#160988=CARTESIAN_POINT('Ctrl Pts',(7.40337480758237,70.7554646366514,0.));
#160989=CARTESIAN_POINT('Ctrl Pts',(7.39433604117891,70.735114793895,0.));
#160990=CARTESIAN_POINT('Ctrl Pts',(7.38533681887028,70.7147984363423,0.));
#160991=CARTESIAN_POINT('Ctrl Pts',(7.37637713374761,70.6945157248269,0.));
#160992=CARTESIAN_POINT('Ctrl Pts',(7.36745697876295,70.6742668209685,0.));
#160993=CARTESIAN_POINT('Ctrl Pts',(7.35857634673052,70.6540518871772,0.));
#160994=CARTESIAN_POINT('Ctrl Pts',(7.34973523032581,70.6338710866562,0.));
#160995=CARTESIAN_POINT('Ctrl Pts',(7.34093362208018,70.6137245834002,0.));
#160996=CARTESIAN_POINT('Ctrl Pts',(7.33217151437608,70.5936125421958,0.));
#160997=CARTESIAN_POINT('Ctrl Pts',(7.32344889945237,70.573535128649,0.));
#160998=CARTESIAN_POINT('Ctrl Pts',(7.31476576940404,70.5534925092053,0.));
#160999=CARTESIAN_POINT('Ctrl Pts',(7.30612211618047,70.5334848511675,0.));
#161000=CARTESIAN_POINT('Ctrl Pts',(7.29751793157801,70.5135123227147,0.));
#161001=CARTESIAN_POINT('Ctrl Pts',(7.28895320723836,70.4935750929029,0.));
#161002=CARTESIAN_POINT('Ctrl Pts',(7.2804279346545,70.4736733316463,0.));
#161003=CARTESIAN_POINT('Ctrl Pts',(7.27194210517058,70.4538072096986,0.));
#161004=CARTESIAN_POINT('Ctrl Pts',(7.26349570998051,70.433976898636,0.));
#161005=CARTESIAN_POINT('Ctrl Pts',(7.25508874012076,70.4141825708207,0.));
#161006=CARTESIAN_POINT('Ctrl Pts',(7.24672118647116,70.3944243994532,0.));
#161007=CARTESIAN_POINT('Ctrl Pts',(7.23839303975626,70.3747025586569,0.));
#161008=CARTESIAN_POINT('Ctrl Pts',(7.23010429054231,70.3550172235486,0.));
#161009=CARTESIAN_POINT('Ctrl Pts',(7.22185492923178,70.3353685703097,0.));
#161010=CARTESIAN_POINT('Ctrl Pts',(7.21364494605425,70.3157567762561,0.));
#161011=CARTESIAN_POINT('Ctrl Pts',(7.20547433107458,70.2961820197051,0.));
#161012=CARTESIAN_POINT('Ctrl Pts',(7.19734307419861,70.276644479827,0.));
#161013=CARTESIAN_POINT('Ctrl Pts',(7.18925116517563,70.2571443365198,0.));
#161014=CARTESIAN_POINT('Ctrl Pts',(7.18119859359801,70.2376817702239,0.));
#161015=CARTESIAN_POINT('Ctrl Pts',(7.17318534889747,70.2182569619028,0.));
#161016=CARTESIAN_POINT('Ctrl Pts',(7.16521142033893,70.1988700934622,0.));
#161017=CARTESIAN_POINT('Ctrl Pts',(7.15727679700946,70.1795213481196,0.));
#161018=CARTESIAN_POINT('Ctrl Pts',(7.14938146780801,70.1602109107188,0.));
#161019=CARTESIAN_POINT('Ctrl Pts',(7.14152542142339,70.1409389682389,0.));
#161020=CARTESIAN_POINT('Ctrl Pts',(7.13370864634399,70.1217057094456,0.));
#161021=CARTESIAN_POINT('Ctrl Pts',(7.12593113088871,70.1025113239463,0.));
#161022=CARTESIAN_POINT('Ctrl Pts',(7.11819286322824,70.0833560013971,0.));
#161023=CARTESIAN_POINT('Ctrl Pts',(7.11049383140482,70.06423993069,0.));
#161024=CARTESIAN_POINT('Ctrl Pts',(7.10283402335091,70.0451632990137,0.));
#161025=CARTESIAN_POINT('Ctrl Pts',(7.09521342684301,70.0261262936435,0.));
#161026=CARTESIAN_POINT('Ctrl Pts',(7.08763202944274,70.0071291040791,0.));
#161027=CARTESIAN_POINT('Ctrl Pts',(7.08008981844643,69.988171923787,0.));
#161028=CARTESIAN_POINT('Ctrl Pts',(7.07258678080793,69.9692549527256,0.));
#161029=CARTESIAN_POINT('Ctrl Pts',(7.06512290312803,69.9503783975676,0.));
#161030=CARTESIAN_POINT('Ctrl Pts',(7.05769817180825,69.9315424664252,0.));
#161031=CARTESIAN_POINT('Ctrl Pts',(7.05031257318108,69.9127473642087,0.));
#161032=CARTESIAN_POINT('Ctrl Pts',(7.04296609362187,69.8939932885864,0.));
#161033=CARTESIAN_POINT('Ctrl Pts',(7.03565871972266,69.8752804235296,0.));
#161034=CARTESIAN_POINT('Ctrl Pts',(7.02839043811863,69.8566089455448,0.));
#161035=CARTESIAN_POINT('Ctrl Pts',(7.02116123514488,69.8379790360574,0.));
#161036=CARTESIAN_POINT('Ctrl Pts',(7.01397109655456,69.8193908913722,0.));
#161037=CARTESIAN_POINT('Ctrl Pts',(7.00682000718105,69.8008447346782,0.));
#161038=CARTESIAN_POINT('Ctrl Pts',(6.99970795069399,69.7823408242446,0.));
#161039=CARTESIAN_POINT('Ctrl Pts',(6.9926349102786,69.7638794280263,0.));
#161040=CARTESIAN_POINT('Ctrl Pts',(6.98560086924173,69.7454607995524,0.));
#161041=CARTESIAN_POINT('Ctrl Pts',(6.97860581164569,69.7270851557443,0.));
#161042=CARTESIAN_POINT('Ctrl Pts',(6.97164972291582,69.7087526480249,0.));
#161043=CARTESIAN_POINT('Ctrl Pts',(6.9647325904973,69.6904633605834,0.));
#161044=CARTESIAN_POINT('Ctrl Pts',(6.95923004173796,69.6758665380764,0.));
#161045=CARTESIAN_POINT('Ctrl Pts',(6.95512065317731,69.6649383920075,0.));
#161046=CARTESIAN_POINT('Ctrl Pts',(6.95238884849076,69.6576616146559,0.));
#161047=CARTESIAN_POINT('Ctrl Pts',(6.95102489306928,69.6540253893193,0.));
#161048=CARTESIAN_POINT('Ctrl Pts',(15.5142209845168,72.8667204369977,0.));
#161049=CARTESIAN_POINT('Ctrl Pts',(15.5142209845168,72.8667204369977,12.));
#161050=CARTESIAN_POINT('Ctrl Pts',(15.5108715869174,72.8622377860957,0.));
#161051=CARTESIAN_POINT('Ctrl Pts',(15.5108715869174,72.8622377860957,12.));
#161052=CARTESIAN_POINT('Ctrl Pts',(15.5041768664089,72.8532737732124,0.));
#161053=CARTESIAN_POINT('Ctrl Pts',(15.5041768664089,72.8532737732124,12.));
#161054=CARTESIAN_POINT('Ctrl Pts',(15.494147009717,72.8398316206501,0.));
#161055=CARTESIAN_POINT('Ctrl Pts',(15.494147009717,72.8398316206501,12.));
#161056=CARTESIAN_POINT('Ctrl Pts',(15.4807983165984,72.8219164844002,0.));
#161057=CARTESIAN_POINT('Ctrl Pts',(15.4807983165984,72.8219164844002,12.));
#161058=CARTESIAN_POINT('Ctrl Pts',(15.4641532053435,72.7995354604414,0.));
#161059=CARTESIAN_POINT('Ctrl Pts',(15.4641532053435,72.7995354604414,12.));
#161060=CARTESIAN_POINT('Ctrl Pts',(15.4475488590336,72.7771673494582,0.));
#161061=CARTESIAN_POINT('Ctrl Pts',(15.4475488590336,72.7771673494582,12.));
#161062=CARTESIAN_POINT('Ctrl Pts',(15.4309852897866,72.7548121825431,0.));
#161063=CARTESIAN_POINT('Ctrl Pts',(15.4309852897866,72.7548121825431,12.));
#161064=CARTESIAN_POINT('Ctrl Pts',(15.4144625111911,72.7324700089576,0.));
#161065=CARTESIAN_POINT('Ctrl Pts',(15.4144625111911,72.7324700089576,12.));
#161066=CARTESIAN_POINT('Ctrl Pts',(15.397980537311,72.710140901746,0.));
#161067=CARTESIAN_POINT('Ctrl Pts',(15.397980537311,72.710140901746,12.));
#161068=CARTESIAN_POINT('Ctrl Pts',(15.3815393822669,72.6878249557452,0.));
#161069=CARTESIAN_POINT('Ctrl Pts',(15.3815393822669,72.6878249557452,12.));
#161070=CARTESIAN_POINT('Ctrl Pts',(15.3651390602616,72.6655222797603,0.));
#161071=CARTESIAN_POINT('Ctrl Pts',(15.3651390602616,72.6655222797603,12.));
#161072=CARTESIAN_POINT('Ctrl Pts',(15.3487795854723,72.6432329903466,0.));
#161073=CARTESIAN_POINT('Ctrl Pts',(15.3487795854723,72.6432329903466,12.));
#161074=CARTESIAN_POINT('Ctrl Pts',(15.3324609719961,72.6209572051064,0.));
#161075=CARTESIAN_POINT('Ctrl Pts',(15.3324609719961,72.6209572051064,12.));
#161076=CARTESIAN_POINT('Ctrl Pts',(15.3161832337617,72.5986950357771,0.));
#161077=CARTESIAN_POINT('Ctrl Pts',(15.3161832337617,72.5986950357771,12.));
#161078=CARTESIAN_POINT('Ctrl Pts',(15.2999463844691,72.5764465826345,0.));
#161079=CARTESIAN_POINT('Ctrl Pts',(15.2999463844691,72.5764465826345,12.));
#161080=CARTESIAN_POINT('Ctrl Pts',(15.2837504376562,72.5542119383748,0.));
#161081=CARTESIAN_POINT('Ctrl Pts',(15.2837504376562,72.5542119383748,12.));
#161082=CARTESIAN_POINT('Ctrl Pts',(15.2675954067495,72.5319911908978,0.));
#161083=CARTESIAN_POINT('Ctrl Pts',(15.2675954067495,72.5319911908978,12.));
#161084=CARTESIAN_POINT('Ctrl Pts',(15.2514813051174,72.5097844266083,0.));
#161085=CARTESIAN_POINT('Ctrl Pts',(15.2514813051174,72.5097844266083,12.));
#161086=CARTESIAN_POINT('Ctrl Pts',(15.2354081461152,72.4875917332729,0.));
#161087=CARTESIAN_POINT('Ctrl Pts',(15.2354081461152,72.4875917332729,12.));
#161088=CARTESIAN_POINT('Ctrl Pts',(15.2193759431359,72.4654132036373,0.));
#161089=CARTESIAN_POINT('Ctrl Pts',(15.2193759431359,72.4654132036373,12.));
#161090=CARTESIAN_POINT('Ctrl Pts',(15.2033847096077,72.4432489350415,0.));
#161091=CARTESIAN_POINT('Ctrl Pts',(15.2033847096077,72.4432489350415,12.));
#161092=CARTESIAN_POINT('Ctrl Pts',(15.1874344589716,72.4210990277819,0.));
#161093=CARTESIAN_POINT('Ctrl Pts',(15.1874344589716,72.4210990277819,12.));
#161094=CARTESIAN_POINT('Ctrl Pts',(15.1715252046602,72.3989635838476,0.));
#161095=CARTESIAN_POINT('Ctrl Pts',(15.1715252046602,72.3989635838476,12.));
#161096=CARTESIAN_POINT('Ctrl Pts',(15.1556569600747,72.37684270559,0.));
#161097=CARTESIAN_POINT('Ctrl Pts',(15.1556569600747,72.37684270559,12.));
#161098=CARTESIAN_POINT('Ctrl Pts',(15.1398297385513,72.3547364941996,0.));
#161099=CARTESIAN_POINT('Ctrl Pts',(15.1398297385513,72.3547364941996,12.));
#161100=CARTESIAN_POINT('Ctrl Pts',(15.1240435533478,72.332645049021,0.));
#161101=CARTESIAN_POINT('Ctrl Pts',(15.1240435533478,72.332645049021,12.));
#161102=CARTESIAN_POINT('Ctrl Pts',(15.1082984176655,72.3105684683971,0.));
#161103=CARTESIAN_POINT('Ctrl Pts',(15.1082984176655,72.3105684683971,12.));
#161104=CARTESIAN_POINT('Ctrl Pts',(15.0925943446593,72.2885068501641,0.));
#161105=CARTESIAN_POINT('Ctrl Pts',(15.0925943446593,72.2885068501641,12.));
#161106=CARTESIAN_POINT('Ctrl Pts',(15.0769313474476,72.266460292285,0.));
#161107=CARTESIAN_POINT('Ctrl Pts',(15.0769313474476,72.266460292285,12.));
#161108=CARTESIAN_POINT('Ctrl Pts',(15.0613094391186,72.244428893425,0.));
#161109=CARTESIAN_POINT('Ctrl Pts',(15.0613094391186,72.244428893425,12.));
#161110=CARTESIAN_POINT('Ctrl Pts',(15.0457286327328,72.2224127535401,0.));
#161111=CARTESIAN_POINT('Ctrl Pts',(15.0457286327328,72.2224127535401,12.));
#161112=CARTESIAN_POINT('Ctrl Pts',(15.0301889413255,72.2004119736104,0.));
#161113=CARTESIAN_POINT('Ctrl Pts',(15.0301889413255,72.2004119736104,12.));
#161114=CARTESIAN_POINT('Ctrl Pts',(15.0146903779061,72.1784266553948,0.));
#161115=CARTESIAN_POINT('Ctrl Pts',(15.0146903779061,72.1784266553948,12.));
#161116=CARTESIAN_POINT('Ctrl Pts',(14.9992329554537,72.1564569011668,0.));
#161117=CARTESIAN_POINT('Ctrl Pts',(14.9992329554537,72.1564569011668,12.));
#161118=CARTESIAN_POINT('Ctrl Pts',(14.9838166869107,72.1345028134779,0.));
#161119=CARTESIAN_POINT('Ctrl Pts',(14.9838166869107,72.1345028134779,12.));
#161120=CARTESIAN_POINT('Ctrl Pts',(14.9684415851699,72.1125644948547,0.));
#161121=CARTESIAN_POINT('Ctrl Pts',(14.9684415851699,72.1125644948547,12.));
#161122=CARTESIAN_POINT('Ctrl Pts',(14.953107663077,72.0906420478085,0.));
#161123=CARTESIAN_POINT('Ctrl Pts',(14.953107663077,72.0906420478085,12.));
#161124=CARTESIAN_POINT('Ctrl Pts',(14.937814933439,72.0687355749815,0.));
#161125=CARTESIAN_POINT('Ctrl Pts',(14.937814933439,72.0687355749815,12.));
#161126=CARTESIAN_POINT('Ctrl Pts',(14.9225634090269,72.046845179251,0.));
#161127=CARTESIAN_POINT('Ctrl Pts',(14.9225634090269,72.046845179251,12.));
#161128=CARTESIAN_POINT('Ctrl Pts',(14.9073531025763,72.0249709638419,0.));
#161129=CARTESIAN_POINT('Ctrl Pts',(14.9073531025763,72.0249709638419,12.));
#161130=CARTESIAN_POINT('Ctrl Pts',(14.892184026783,72.0031130324519,0.));
#161131=CARTESIAN_POINT('Ctrl Pts',(14.892184026783,72.0031130324519,12.));
#161132=CARTESIAN_POINT('Ctrl Pts',(14.8770561943011,71.9812714893087,0.));
#161133=CARTESIAN_POINT('Ctrl Pts',(14.8770561943011,71.9812714893087,12.));
#161134=CARTESIAN_POINT('Ctrl Pts',(14.8619696177503,71.9594464391063,0.));
#161135=CARTESIAN_POINT('Ctrl Pts',(14.8619696177503,71.9594464391063,12.));
#161136=CARTESIAN_POINT('Ctrl Pts',(14.846924309716,71.9376379869668,0.));
#161137=CARTESIAN_POINT('Ctrl Pts',(14.846924309716,71.9376379869668,12.));
#161138=CARTESIAN_POINT('Ctrl Pts',(14.8319202827482,71.9158462383915,0.));
#161139=CARTESIAN_POINT('Ctrl Pts',(14.8319202827482,71.9158462383915,12.));
#161140=CARTESIAN_POINT('Ctrl Pts',(14.816957549356,71.8940712992119,0.));
#161141=CARTESIAN_POINT('Ctrl Pts',(14.816957549356,71.8940712992119,12.));
#161142=CARTESIAN_POINT('Ctrl Pts',(14.8020361220003,71.872313275546,0.));
#161143=CARTESIAN_POINT('Ctrl Pts',(14.8020361220003,71.872313275546,12.));
#161144=CARTESIAN_POINT('Ctrl Pts',(14.7871560131021,71.8505722738286,0.));
#161145=CARTESIAN_POINT('Ctrl Pts',(14.7871560131021,71.8505722738286,12.));
#161146=CARTESIAN_POINT('Ctrl Pts',(14.7723172350454,71.8288484008343,0.));
#161147=CARTESIAN_POINT('Ctrl Pts',(14.7723172350454,71.8288484008343,12.));
#161148=CARTESIAN_POINT('Ctrl Pts',(14.7575198001776,71.8071417637019,0.));
#161149=CARTESIAN_POINT('Ctrl Pts',(14.7575198001776,71.8071417637019,12.));
#161150=CARTESIAN_POINT('Ctrl Pts',(14.7427637208071,71.7854524699563,0.));
#161151=CARTESIAN_POINT('Ctrl Pts',(14.7427637208071,71.7854524699563,12.));
#161152=CARTESIAN_POINT('Ctrl Pts',(14.7280490091954,71.7637806275316,0.));
#161153=CARTESIAN_POINT('Ctrl Pts',(14.7280490091954,71.7637806275316,12.));
#161154=CARTESIAN_POINT('Ctrl Pts',(14.7133756775622,71.7421263447707,0.));
#161155=CARTESIAN_POINT('Ctrl Pts',(14.7133756775622,71.7421263447707,12.));
#161156=CARTESIAN_POINT('Ctrl Pts',(14.6987437380898,71.7204897304186,0.));
#161157=CARTESIAN_POINT('Ctrl Pts',(14.6987437380898,71.7204897304186,12.));
#161158=CARTESIAN_POINT('Ctrl Pts',(14.6841532029231,71.698870893617,0.));
#161159=CARTESIAN_POINT('Ctrl Pts',(14.6841532029231,71.698870893617,12.));
#161160=CARTESIAN_POINT('Ctrl Pts',(14.6696040841679,71.6772699438966,0.));
#161161=CARTESIAN_POINT('Ctrl Pts',(14.6696040841679,71.6772699438966,12.));
#161162=CARTESIAN_POINT('Ctrl Pts',(14.6550963938832,71.6556869911669,0.));
#161163=CARTESIAN_POINT('Ctrl Pts',(14.6550963938832,71.6556869911669,12.));
#161164=CARTESIAN_POINT('Ctrl Pts',(14.6406301440817,71.6341221457175,0.));
#161165=CARTESIAN_POINT('Ctrl Pts',(14.6406301440817,71.6341221457175,12.));
#161166=CARTESIAN_POINT('Ctrl Pts',(14.6262053467372,71.6125755182295,0.));
#161167=CARTESIAN_POINT('Ctrl Pts',(14.6262053467372,71.6125755182295,12.));
#161168=CARTESIAN_POINT('Ctrl Pts',(14.611822013785,71.5910472197815,0.));
#161169=CARTESIAN_POINT('Ctrl Pts',(14.611822013785,71.5910472197815,12.));
#161170=CARTESIAN_POINT('Ctrl Pts',(14.597480157121,71.569537361856,0.));
#161171=CARTESIAN_POINT('Ctrl Pts',(14.597480157121,71.569537361856,12.));
#161172=CARTESIAN_POINT('Ctrl Pts',(14.5831797885951,71.5480460563445,0.));
#161173=CARTESIAN_POINT('Ctrl Pts',(14.5831797885951,71.5480460563445,12.));
#161174=CARTESIAN_POINT('Ctrl Pts',(14.568920920009,71.5265734155501,0.));
#161175=CARTESIAN_POINT('Ctrl Pts',(14.568920920009,71.5265734155501,12.));
#161176=CARTESIAN_POINT('Ctrl Pts',(14.5547035631234,71.5051195521914,0.));
#161177=CARTESIAN_POINT('Ctrl Pts',(14.5547035631234,71.5051195521914,12.));
#161178=CARTESIAN_POINT('Ctrl Pts',(14.540527729659,71.4836845794052,0.));
#161179=CARTESIAN_POINT('Ctrl Pts',(14.540527729659,71.4836845794052,12.));
#161180=CARTESIAN_POINT('Ctrl Pts',(14.5263934312969,71.4622686107475,0.));
#161181=CARTESIAN_POINT('Ctrl Pts',(14.5263934312969,71.4622686107475,12.));
#161182=CARTESIAN_POINT('Ctrl Pts',(14.5123006796728,71.4408717601917,0.));
#161183=CARTESIAN_POINT('Ctrl Pts',(14.5123006796728,71.4408717601917,12.));
#161184=CARTESIAN_POINT('Ctrl Pts',(14.4982494863716,71.4194941421279,0.));
#161185=CARTESIAN_POINT('Ctrl Pts',(14.4982494863716,71.4194941421279,12.));
#161186=CARTESIAN_POINT('Ctrl Pts',(14.4842398629353,71.398135871371,0.));
#161187=CARTESIAN_POINT('Ctrl Pts',(14.4842398629353,71.398135871371,12.));
#161188=CARTESIAN_POINT('Ctrl Pts',(14.470271820865,71.3767970631642,0.));
#161189=CARTESIAN_POINT('Ctrl Pts',(14.470271820865,71.3767970631642,12.));
#161190=CARTESIAN_POINT('Ctrl Pts',(14.4563453716204,71.3554778331835,0.));
#161191=CARTESIAN_POINT('Ctrl Pts',(14.4563453716204,71.3554778331835,12.));
#161192=CARTESIAN_POINT('Ctrl Pts',(14.4424605266166,71.3341782975393,0.));
#161193=CARTESIAN_POINT('Ctrl Pts',(14.4424605266166,71.3341782975393,12.));
#161194=CARTESIAN_POINT('Ctrl Pts',(14.4286172972168,71.3128985727777,0.));
#161195=CARTESIAN_POINT('Ctrl Pts',(14.4286172972168,71.3128985727777,12.));
#161196=CARTESIAN_POINT('Ctrl Pts',(14.4148156947384,71.2916387758864,0.));
#161197=CARTESIAN_POINT('Ctrl Pts',(14.4148156947384,71.2916387758864,12.));
#161198=CARTESIAN_POINT('Ctrl Pts',(14.401055730457,71.2703990242986,0.));
#161199=CARTESIAN_POINT('Ctrl Pts',(14.401055730457,71.2703990242986,12.));
#161200=CARTESIAN_POINT('Ctrl Pts',(14.3873374156056,71.2491794358956,0.));
#161201=CARTESIAN_POINT('Ctrl Pts',(14.3873374156056,71.2491794358956,12.));
#161202=CARTESIAN_POINT('Ctrl Pts',(14.3736607613723,71.2279801290088,0.));
#161203=CARTESIAN_POINT('Ctrl Pts',(14.3736607613723,71.2279801290088,12.));
#161204=CARTESIAN_POINT('Ctrl Pts',(14.3600257788927,71.2068012224187,0.));
#161205=CARTESIAN_POINT('Ctrl Pts',(14.3600257788927,71.2068012224187,12.));
#161206=CARTESIAN_POINT('Ctrl Pts',(14.3464324792537,71.185642835361,0.));
#161207=CARTESIAN_POINT('Ctrl Pts',(14.3464324792537,71.185642835361,12.));
#161208=CARTESIAN_POINT('Ctrl Pts',(14.3328808734993,71.1645050875323,0.));
#161209=CARTESIAN_POINT('Ctrl Pts',(14.3328808734993,71.1645050875323,12.));
#161210=CARTESIAN_POINT('Ctrl Pts',(14.3193709726295,71.1433880990932,0.));
#161211=CARTESIAN_POINT('Ctrl Pts',(14.3193709726295,71.1433880990932,12.));
#161212=CARTESIAN_POINT('Ctrl Pts',(14.3059027875993,71.1222919906719,0.));
#161213=CARTESIAN_POINT('Ctrl Pts',(14.3059027875993,71.1222919906719,12.));
#161214=CARTESIAN_POINT('Ctrl Pts',(14.2924763293101,71.1012168833626,0.));
#161215=CARTESIAN_POINT('Ctrl Pts',(14.2924763293101,71.1012168833626,12.));
#161216=CARTESIAN_POINT('Ctrl Pts',(14.2790916086129,71.0801628987314,0.));
#161217=CARTESIAN_POINT('Ctrl Pts',(14.2790916086129,71.0801628987314,12.));
#161218=CARTESIAN_POINT('Ctrl Pts',(14.2657486363136,71.059130158822,0.));
#161219=CARTESIAN_POINT('Ctrl Pts',(14.2657486363136,71.059130158822,12.));
#161220=CARTESIAN_POINT('Ctrl Pts',(14.2524474231732,71.0381187861585,0.));
#161221=CARTESIAN_POINT('Ctrl Pts',(14.2524474231732,71.0381187861585,12.));
#161222=CARTESIAN_POINT('Ctrl Pts',(14.2391879799063,71.0171289037493,0.));
#161223=CARTESIAN_POINT('Ctrl Pts',(14.2391879799063,71.0171289037493,12.));
#161224=CARTESIAN_POINT('Ctrl Pts',(14.2259703171739,70.996160635087,0.));
#161225=CARTESIAN_POINT('Ctrl Pts',(14.2259703171739,70.996160635087,12.));
#161226=CARTESIAN_POINT('Ctrl Pts',(14.2127944455841,70.9752141041527,0.));
#161227=CARTESIAN_POINT('Ctrl Pts',(14.2127944455841,70.9752141041527,12.));
#161228=CARTESIAN_POINT('Ctrl Pts',(14.1996603756984,70.9542894354221,0.));
#161229=CARTESIAN_POINT('Ctrl Pts',(14.1996603756984,70.9542894354221,12.));
#161230=CARTESIAN_POINT('Ctrl Pts',(14.1865681180321,70.9333867538705,0.));
#161231=CARTESIAN_POINT('Ctrl Pts',(14.1865681180321,70.9333867538705,12.));
#161232=CARTESIAN_POINT('Ctrl Pts',(14.1735176830533,70.9125061849744,0.));
#161233=CARTESIAN_POINT('Ctrl Pts',(14.1735176830533,70.9125061849744,12.));
#161234=CARTESIAN_POINT('Ctrl Pts',(14.1605090811754,70.8916478547131,0.));
#161235=CARTESIAN_POINT('Ctrl Pts',(14.1605090811754,70.8916478547131,12.));
#161236=CARTESIAN_POINT('Ctrl Pts',(14.1475423227567,70.8708118895718,0.));
#161237=CARTESIAN_POINT('Ctrl Pts',(14.1475423227567,70.8708118895718,12.));
#161238=CARTESIAN_POINT('Ctrl Pts',(14.1346174181079,70.8499984165493,0.));
#161239=CARTESIAN_POINT('Ctrl Pts',(14.1346174181079,70.8499984165493,12.));
#161240=CARTESIAN_POINT('Ctrl Pts',(14.1217343774914,70.8292075631624,0.));
#161241=CARTESIAN_POINT('Ctrl Pts',(14.1217343774914,70.8292075631624,12.));
#161242=CARTESIAN_POINT('Ctrl Pts',(14.1088932111214,70.8084394574491,0.));
#161243=CARTESIAN_POINT('Ctrl Pts',(14.1088932111214,70.8084394574491,12.));
#161244=CARTESIAN_POINT('Ctrl Pts',(14.0960939291568,70.787694227969,0.));
#161245=CARTESIAN_POINT('Ctrl Pts',(14.0960939291568,70.787694227969,12.));
#161246=CARTESIAN_POINT('Ctrl Pts',(14.0833365416995,70.7669720038067,0.));
#161247=CARTESIAN_POINT('Ctrl Pts',(14.0833365416995,70.7669720038067,12.));
#161248=CARTESIAN_POINT('Ctrl Pts',(14.0706210588015,70.7462729145799,0.));
#161249=CARTESIAN_POINT('Ctrl Pts',(14.0706210588015,70.7462729145799,12.));
#161250=CARTESIAN_POINT('Ctrl Pts',(14.0579474904657,70.7255970904433,0.));
#161251=CARTESIAN_POINT('Ctrl Pts',(14.0579474904657,70.7255970904433,12.));
#161252=CARTESIAN_POINT('Ctrl Pts',(14.0453158466451,70.7049446620931,0.));
#161253=CARTESIAN_POINT('Ctrl Pts',(14.0453158466451,70.7049446620931,12.));
#161254=CARTESIAN_POINT('Ctrl Pts',(14.0327261372363,70.6843157607672,0.));
#161255=CARTESIAN_POINT('Ctrl Pts',(14.0327261372363,70.6843157607672,12.));
#161256=CARTESIAN_POINT('Ctrl Pts',(14.020178372077,70.6637105182487,0.));
#161257=CARTESIAN_POINT('Ctrl Pts',(14.020178372077,70.6637105182487,12.));
#161258=CARTESIAN_POINT('Ctrl Pts',(14.0076725609537,70.6431290668744,0.));
#161259=CARTESIAN_POINT('Ctrl Pts',(14.0076725609537,70.6431290668744,12.));
#161260=CARTESIAN_POINT('Ctrl Pts',(13.9952087136018,70.6225715395392,0.));
#161261=CARTESIAN_POINT('Ctrl Pts',(13.9952087136018,70.6225715395392,12.));
#161262=CARTESIAN_POINT('Ctrl Pts',(13.9827868397057,70.6020380697004,0.));
#161263=CARTESIAN_POINT('Ctrl Pts',(13.9827868397057,70.6020380697004,12.));
#161264=CARTESIAN_POINT('Ctrl Pts',(13.9704069488918,70.5815287913791,0.));
#161265=CARTESIAN_POINT('Ctrl Pts',(13.9704069488918,70.5815287913791,12.));
#161266=CARTESIAN_POINT('Ctrl Pts',(13.9580690507262,70.5610438391622,0.));
#161267=CARTESIAN_POINT('Ctrl Pts',(13.9580690507262,70.5610438391622,12.));
#161268=CARTESIAN_POINT('Ctrl Pts',(13.9457731547217,70.5405833482123,0.));
#161269=CARTESIAN_POINT('Ctrl Pts',(13.9457731547217,70.5405833482123,12.));
#161270=CARTESIAN_POINT('Ctrl Pts',(13.9335192703389,70.5201474542717,0.));
#161271=CARTESIAN_POINT('Ctrl Pts',(13.9335192703389,70.5201474542717,12.));
#161272=CARTESIAN_POINT('Ctrl Pts',(13.9213074069852,70.4997362936671,0.));
#161273=CARTESIAN_POINT('Ctrl Pts',(13.9213074069852,70.4997362936671,12.));
#161274=CARTESIAN_POINT('Ctrl Pts',(13.9091375740084,70.4793500033106,0.));
#161275=CARTESIAN_POINT('Ctrl Pts',(13.9091375740084,70.4793500033106,12.));
#161276=CARTESIAN_POINT('Ctrl Pts',(13.8970097806947,70.4589887207043,0.));
#161277=CARTESIAN_POINT('Ctrl Pts',(13.8970097806947,70.4589887207043,12.));
#161278=CARTESIAN_POINT('Ctrl Pts',(13.8849240362757,70.4386525839492,0.));
#161279=CARTESIAN_POINT('Ctrl Pts',(13.8849240362757,70.4386525839492,12.));
#161280=CARTESIAN_POINT('Ctrl Pts',(13.8728803499284,70.4183417317486,0.));
#161281=CARTESIAN_POINT('Ctrl Pts',(13.8728803499284,70.4183417317486,12.));
#161282=CARTESIAN_POINT('Ctrl Pts',(13.8608787307754,70.3980563034142,0.));
#161283=CARTESIAN_POINT('Ctrl Pts',(13.8608787307754,70.3980563034142,12.));
#161284=CARTESIAN_POINT('Ctrl Pts',(13.8489191878774,70.377796438866,0.));
#161285=CARTESIAN_POINT('Ctrl Pts',(13.8489191878774,70.377796438866,12.));
#161286=CARTESIAN_POINT('Ctrl Pts',(13.8370017302319,70.3575622786373,0.));
#161287=CARTESIAN_POINT('Ctrl Pts',(13.8370017302319,70.3575622786373,12.));
#161288=CARTESIAN_POINT('Ctrl Pts',(13.8251263667799,70.3373539638841,0.));
#161289=CARTESIAN_POINT('Ctrl Pts',(13.8251263667799,70.3373539638841,12.));
#161290=CARTESIAN_POINT('Ctrl Pts',(13.8132931064067,70.3171716363912,0.));
#161291=CARTESIAN_POINT('Ctrl Pts',(13.8132931064067,70.3171716363912,12.));
#161292=CARTESIAN_POINT('Ctrl Pts',(13.8015019579411,70.2970154385763,0.));
#161293=CARTESIAN_POINT('Ctrl Pts',(13.8015019579411,70.2970154385763,12.));
#161294=CARTESIAN_POINT('Ctrl Pts',(13.7897529301483,70.2768855134909,0.));
#161295=CARTESIAN_POINT('Ctrl Pts',(13.7897529301483,70.2768855134909,12.));
#161296=CARTESIAN_POINT('Ctrl Pts',(13.7780460317284,70.2567820048253,0.));
#161297=CARTESIAN_POINT('Ctrl Pts',(13.7780460317284,70.2567820048253,12.));
#161298=CARTESIAN_POINT('Ctrl Pts',(13.7663812713235,70.2367050569174,0.));
#161299=CARTESIAN_POINT('Ctrl Pts',(13.7663812713235,70.2367050569174,12.));
#161300=CARTESIAN_POINT('Ctrl Pts',(13.7547586575178,70.216654814759,0.));
#161301=CARTESIAN_POINT('Ctrl Pts',(13.7547586575178,70.216654814759,12.));
#161302=CARTESIAN_POINT('Ctrl Pts',(13.7431781988368,70.1966314240012,0.));
#161303=CARTESIAN_POINT('Ctrl Pts',(13.7431781988368,70.1966314240012,12.));
#161304=CARTESIAN_POINT('Ctrl Pts',(13.73163990374,70.1766350309554,0.));
#161305=CARTESIAN_POINT('Ctrl Pts',(13.73163990374,70.1766350309554,12.));
#161306=CARTESIAN_POINT('Ctrl Pts',(13.7201437806207,70.1566657825989,0.));
#161307=CARTESIAN_POINT('Ctrl Pts',(13.7201437806207,70.1566657825989,12.));
#161308=CARTESIAN_POINT('Ctrl Pts',(13.7086898378127,70.1367238265853,0.));
#161309=CARTESIAN_POINT('Ctrl Pts',(13.7086898378127,70.1367238265853,12.));
#161310=CARTESIAN_POINT('Ctrl Pts',(13.6972780835898,70.1168093112493,0.));
#161311=CARTESIAN_POINT('Ctrl Pts',(13.6972780835898,70.1168093112493,12.));
#161312=CARTESIAN_POINT('Ctrl Pts',(13.685908526165,70.0969223856123,0.));
#161313=CARTESIAN_POINT('Ctrl Pts',(13.685908526165,70.0969223856123,12.));
#161314=CARTESIAN_POINT('Ctrl Pts',(13.6745811736825,70.0770631993831,0.));
#161315=CARTESIAN_POINT('Ctrl Pts',(13.6745811736825,70.0770631993831,12.));
#161316=CARTESIAN_POINT('Ctrl Pts',(13.6632960342192,70.057231902965,0.));
#161317=CARTESIAN_POINT('Ctrl Pts',(13.6632960342192,70.057231902965,12.));
#161318=CARTESIAN_POINT('Ctrl Pts',(13.6520531157904,70.037428647466,0.));
#161319=CARTESIAN_POINT('Ctrl Pts',(13.6520531157904,70.037428647466,12.));
#161320=CARTESIAN_POINT('Ctrl Pts',(13.6408524263496,70.0176535847047,0.));
#161321=CARTESIAN_POINT('Ctrl Pts',(13.6408524263496,70.0176535847047,12.));
#161322=CARTESIAN_POINT('Ctrl Pts',(13.6296939737866,69.9979068672163,0.));
#161323=CARTESIAN_POINT('Ctrl Pts',(13.6296939737866,69.9979068672163,12.));
#161324=CARTESIAN_POINT('Ctrl Pts',(13.61857776592,69.9781886482543,0.));
#161325=CARTESIAN_POINT('Ctrl Pts',(13.61857776592,69.9781886482543,12.));
#161326=CARTESIAN_POINT('Ctrl Pts',(13.6075038105,69.9584990817989,0.));
#161327=CARTESIAN_POINT('Ctrl Pts',(13.6075038105,69.9584990817989,12.));
#161328=CARTESIAN_POINT('Ctrl Pts',(13.5964721152136,69.9388383225655,0.));
#161329=CARTESIAN_POINT('Ctrl Pts',(13.5964721152136,69.9388383225655,12.));
#161330=CARTESIAN_POINT('Ctrl Pts',(13.5854826876834,69.9192065260107,0.));
#161331=CARTESIAN_POINT('Ctrl Pts',(13.5854826876834,69.9192065260107,12.));
#161332=CARTESIAN_POINT('Ctrl Pts',(13.5745355354657,69.899603848336,0.));
#161333=CARTESIAN_POINT('Ctrl Pts',(13.5745355354657,69.899603848336,12.));
#161334=CARTESIAN_POINT('Ctrl Pts',(13.5636306660422,69.880030446488,0.));
#161335=CARTESIAN_POINT('Ctrl Pts',(13.5636306660422,69.880030446488,12.));
#161336=CARTESIAN_POINT('Ctrl Pts',(13.5527680868256,69.8604864781705,0.));
#161337=CARTESIAN_POINT('Ctrl Pts',(13.5527680868256,69.8604864781705,12.));
#161338=CARTESIAN_POINT('Ctrl Pts',(13.5419478051626,69.840972101856,0.));
#161339=CARTESIAN_POINT('Ctrl Pts',(13.5419478051626,69.840972101856,12.));
#161340=CARTESIAN_POINT('Ctrl Pts',(13.5311698283339,69.8214874767944,0.));
#161341=CARTESIAN_POINT('Ctrl Pts',(13.5311698283339,69.8214874767944,12.));
#161342=CARTESIAN_POINT('Ctrl Pts',(13.5204341635507,69.8020327630204,0.));
#161343=CARTESIAN_POINT('Ctrl Pts',(13.5204341635507,69.8020327630204,12.));
#161344=CARTESIAN_POINT('Ctrl Pts',(13.5097408179478,69.7826081213575,0.));
#161345=CARTESIAN_POINT('Ctrl Pts',(13.5097408179478,69.7826081213575,12.));
#161346=CARTESIAN_POINT('Ctrl Pts',(13.4990897985904,69.7632137134247,0.));
#161347=CARTESIAN_POINT('Ctrl Pts',(13.4990897985904,69.7632137134247,12.));
#161348=CARTESIAN_POINT('Ctrl Pts',(13.4884811124748,69.7438497016404,0.));
#161349=CARTESIAN_POINT('Ctrl Pts',(13.4884811124748,69.7438497016404,12.));
#161350=CARTESIAN_POINT('Ctrl Pts',(13.4779147665285,69.7245162492251,0.));
#161351=CARTESIAN_POINT('Ctrl Pts',(13.4779147665285,69.7245162492251,12.));
#161352=CARTESIAN_POINT('Ctrl Pts',(13.4673907676045,69.7052135202003,0.));
#161353=CARTESIAN_POINT('Ctrl Pts',(13.4673907676045,69.7052135202003,12.));
#161354=CARTESIAN_POINT('Ctrl Pts',(13.4569091224762,69.6859416793898,0.));
#161355=CARTESIAN_POINT('Ctrl Pts',(13.4569091224762,69.6859416793898,12.));
#161356=CARTESIAN_POINT('Ctrl Pts',(13.4464698378456,69.6667008924454,0.));
#161357=CARTESIAN_POINT('Ctrl Pts',(13.4464698378456,69.6667008924454,12.));
#161358=CARTESIAN_POINT('Ctrl Pts',(13.4360729203444,69.6474913258684,0.));
#161359=CARTESIAN_POINT('Ctrl Pts',(13.4360729203444,69.6474913258684,12.));
#161360=CARTESIAN_POINT('Ctrl Pts',(13.425718376534,69.6283131470267,0.));
#161361=CARTESIAN_POINT('Ctrl Pts',(13.425718376534,69.6283131470267,12.));
#161362=CARTESIAN_POINT('Ctrl Pts',(13.4154062128998,69.6091665241743,0.));
#161363=CARTESIAN_POINT('Ctrl Pts',(13.4154062128998,69.6091665241743,12.));
#161364=CARTESIAN_POINT('Ctrl Pts',(13.4051364358494,69.5900516264524,0.));
#161365=CARTESIAN_POINT('Ctrl Pts',(13.4051364358494,69.5900516264524,12.));
#161366=CARTESIAN_POINT('Ctrl Pts',(13.3949090517173,69.5709686238701,0.));
#161367=CARTESIAN_POINT('Ctrl Pts',(13.3949090517173,69.5709686238701,12.));
#161368=CARTESIAN_POINT('Ctrl Pts',(13.3847240667626,69.5519176872857,0.));
#161369=CARTESIAN_POINT('Ctrl Pts',(13.3847240667626,69.5519176872857,12.));
#161370=CARTESIAN_POINT('Ctrl Pts',(13.3745814871667,69.5328989883899,0.));
#161371=CARTESIAN_POINT('Ctrl Pts',(13.3745814871667,69.5328989883899,12.));
#161372=CARTESIAN_POINT('Ctrl Pts',(13.3644813190225,69.5139126996703,0.));
#161373=CARTESIAN_POINT('Ctrl Pts',(13.3644813190225,69.5139126996703,12.));
#161374=CARTESIAN_POINT('Ctrl Pts',(13.3544235683399,69.4949589944633,0.));
#161375=CARTESIAN_POINT('Ctrl Pts',(13.3544235683399,69.4949589944633,12.));
#161376=CARTESIAN_POINT('Ctrl Pts',(13.3444082410546,69.4760380470382,0.));
#161377=CARTESIAN_POINT('Ctrl Pts',(13.3444082410546,69.4760380470382,12.));
#161378=CARTESIAN_POINT('Ctrl Pts',(13.3344353430313,69.4571500326673,0.));
#161379=CARTESIAN_POINT('Ctrl Pts',(13.3344353430313,69.4571500326673,12.));
#161380=CARTESIAN_POINT('Ctrl Pts',(13.3245048800641,69.4382951276983,0.));
#161381=CARTESIAN_POINT('Ctrl Pts',(13.3245048800641,69.4382951276983,12.));
#161382=CARTESIAN_POINT('Ctrl Pts',(13.3146168578738,69.4194735096238,0.));
#161383=CARTESIAN_POINT('Ctrl Pts',(13.3146168578738,69.4194735096238,12.));
#161384=CARTESIAN_POINT('Ctrl Pts',(13.3047712821046,69.4006853569485,0.));
#161385=CARTESIAN_POINT('Ctrl Pts',(13.3047712821046,69.4006853569485,12.));
#161386=CARTESIAN_POINT('Ctrl Pts',(13.2949681583164,69.3819308490408,0.));
#161387=CARTESIAN_POINT('Ctrl Pts',(13.2949681583164,69.3819308490408,12.));
#161388=CARTESIAN_POINT('Ctrl Pts',(13.2852074919767,69.3632101660072,0.));
#161389=CARTESIAN_POINT('Ctrl Pts',(13.2852074919767,69.3632101660072,12.));
#161390=CARTESIAN_POINT('Ctrl Pts',(13.2754892884437,69.3445234885088,0.));
#161391=CARTESIAN_POINT('Ctrl Pts',(13.2754892884437,69.3445234885088,12.));
#161392=CARTESIAN_POINT('Ctrl Pts',(13.2658135529616,69.3258709977416,0.));
#161393=CARTESIAN_POINT('Ctrl Pts',(13.2658135529616,69.3258709977416,12.));
#161394=CARTESIAN_POINT('Ctrl Pts',(13.2561802906901,69.3072528758546,0.));
#161395=CARTESIAN_POINT('Ctrl Pts',(13.2561802906901,69.3072528758546,12.));
#161396=CARTESIAN_POINT('Ctrl Pts',(13.2465895067264,69.2886693063193,0.));
#161397=CARTESIAN_POINT('Ctrl Pts',(13.2465895067264,69.2886693063193,12.));
#161398=CARTESIAN_POINT('Ctrl Pts',(13.2370412061218,69.2701204742436,0.));
#161399=CARTESIAN_POINT('Ctrl Pts',(13.2370412061218,69.2701204742436,12.));
#161400=CARTESIAN_POINT('Ctrl Pts',(13.2275353939044,69.2516065668809,0.));
#161401=CARTESIAN_POINT('Ctrl Pts',(13.2275353939044,69.2516065668809,12.));
#161402=CARTESIAN_POINT('Ctrl Pts',(13.2180720750586,69.2331277732819,0.));
#161403=CARTESIAN_POINT('Ctrl Pts',(13.2180720750586,69.2331277732819,12.));
#161404=CARTESIAN_POINT('Ctrl Pts',(13.2086512544729,69.2146842833506,0.));
#161405=CARTESIAN_POINT('Ctrl Pts',(13.2086512544729,69.2146842833506,12.));
#161406=CARTESIAN_POINT('Ctrl Pts',(13.1992729368928,69.1962762870524,0.));
#161407=CARTESIAN_POINT('Ctrl Pts',(13.1992729368928,69.1962762870524,12.));
#161408=CARTESIAN_POINT('Ctrl Pts',(13.1899371268689,69.1779039736026,0.));
#161409=CARTESIAN_POINT('Ctrl Pts',(13.1899371268689,69.1779039736026,12.));
#161410=CARTESIAN_POINT('Ctrl Pts',(13.1806438286944,69.1595675305294,0.));
#161411=CARTESIAN_POINT('Ctrl Pts',(13.1806438286944,69.1595675305294,12.));
#161412=CARTESIAN_POINT('Ctrl Pts',(13.1713930465142,69.141267145461,0.));
#161413=CARTESIAN_POINT('Ctrl Pts',(13.1713930465142,69.141267145461,12.));
#161414=CARTESIAN_POINT('Ctrl Pts',(13.1621847844533,69.1230030082598,0.));
#161415=CARTESIAN_POINT('Ctrl Pts',(13.1621847844533,69.1230030082598,12.));
#161416=CARTESIAN_POINT('Ctrl Pts',(13.1530190467181,69.1047753127633,0.));
#161417=CARTESIAN_POINT('Ctrl Pts',(13.1530190467181,69.1047753127633,12.));
#161418=CARTESIAN_POINT('Ctrl Pts',(13.1438958377397,69.0865842593063,0.));
#161419=CARTESIAN_POINT('Ctrl Pts',(13.1438958377397,69.0865842593063,12.));
#161420=CARTESIAN_POINT('Ctrl Pts',(13.1348151621824,69.0684300549426,0.));
#161421=CARTESIAN_POINT('Ctrl Pts',(13.1348151621824,69.0684300549426,12.));
#161422=CARTESIAN_POINT('Ctrl Pts',(13.1257770246379,69.0503129081778,0.));
#161423=CARTESIAN_POINT('Ctrl Pts',(13.1257770246379,69.0503129081778,12.));
#161424=CARTESIAN_POINT('Ctrl Pts',(13.1167814293495,69.0322330243336,0.));
#161425=CARTESIAN_POINT('Ctrl Pts',(13.1167814293495,69.0322330243336,12.));
#161426=CARTESIAN_POINT('Ctrl Pts',(13.1078283799726,69.0141906015137,0.));
#161427=CARTESIAN_POINT('Ctrl Pts',(13.1078283799726,69.0141906015137,12.));
#161428=CARTESIAN_POINT('Ctrl Pts',(13.0989178791843,68.9961858241577,0.));
#161429=CARTESIAN_POINT('Ctrl Pts',(13.0989178791843,68.9961858241577,12.));
#161430=CARTESIAN_POINT('Ctrl Pts',(13.0900499290542,68.9782188692654,0.));
#161431=CARTESIAN_POINT('Ctrl Pts',(13.0900499290542,68.9782188692654,12.));
#161432=CARTESIAN_POINT('Ctrl Pts',(13.0812245317816,68.9602899187628,0.));
#161433=CARTESIAN_POINT('Ctrl Pts',(13.0812245317816,68.9602899187628,12.));
#161434=CARTESIAN_POINT('Ctrl Pts',(13.072441690283,68.9423991694493,0.));
#161435=CARTESIAN_POINT('Ctrl Pts',(13.072441690283,68.9423991694493,12.));
#161436=CARTESIAN_POINT('Ctrl Pts',(13.0637014089018,68.9245468449865,0.));
#161437=CARTESIAN_POINT('Ctrl Pts',(13.0637014089018,68.9245468449865,12.));
#161438=CARTESIAN_POINT('Ctrl Pts',(13.0550036938793,68.9067332040842,0.));
#161439=CARTESIAN_POINT('Ctrl Pts',(13.0550036938793,68.9067332040842,12.));
#161440=CARTESIAN_POINT('Ctrl Pts',(13.0463485518185,68.8889585151431,0.));
#161441=CARTESIAN_POINT('Ctrl Pts',(13.0463485518185,68.8889585151431,12.));
#161442=CARTESIAN_POINT('Ctrl Pts',(13.0377359881864,68.8712230321823,0.));
#161443=CARTESIAN_POINT('Ctrl Pts',(13.0377359881864,68.8712230321823,12.));
#161444=CARTESIAN_POINT('Ctrl Pts',(13.0291660060118,68.8535269726871,0.));
#161445=CARTESIAN_POINT('Ctrl Pts',(13.0291660060118,68.8535269726871,12.));
#161446=CARTESIAN_POINT('Ctrl Pts',(13.0206386039729,68.835870488774,0.));
#161447=CARTESIAN_POINT('Ctrl Pts',(13.0206386039729,68.835870488774,12.));
#161448=CARTESIAN_POINT('Ctrl Pts',(13.0121537769003,68.8182536654067,0.));
#161449=CARTESIAN_POINT('Ctrl Pts',(13.0121537769003,68.8182536654067,12.));
#161450=CARTESIAN_POINT('Ctrl Pts',(13.0053999700929,68.8041919669403,0.));
#161451=CARTESIAN_POINT('Ctrl Pts',(13.0053999700929,68.8041919669403,12.));
#161452=CARTESIAN_POINT('Ctrl Pts',(13.0003537683089,68.7936635625788,0.));
#161453=CARTESIAN_POINT('Ctrl Pts',(13.0003537683089,68.7936635625788,12.));
#161454=CARTESIAN_POINT('Ctrl Pts',(12.996998146029,68.7866525680284,0.));
#161455=CARTESIAN_POINT('Ctrl Pts',(12.996998146029,68.7866525680284,12.));
#161456=CARTESIAN_POINT('Ctrl Pts',(12.9953224629497,68.7831490561748,0.));
#161457=CARTESIAN_POINT('Ctrl Pts',(12.9953224629497,68.7831490561748,12.));
#161458=CARTESIAN_POINT('',(12.9953224629497,68.7831490561748,12.));
#161459=CARTESIAN_POINT('Ctrl Pts',(12.9953224629497,68.7831490561748,12.));
#161460=CARTESIAN_POINT('Ctrl Pts',(12.996998146029,68.7866525680284,12.));
#161461=CARTESIAN_POINT('Ctrl Pts',(13.0003537683089,68.7936635625788,12.));
#161462=CARTESIAN_POINT('Ctrl Pts',(13.0053999700929,68.8041919669403,12.));
#161463=CARTESIAN_POINT('Ctrl Pts',(13.0121537769003,68.8182536654067,12.));
#161464=CARTESIAN_POINT('Ctrl Pts',(13.0206386039729,68.835870488774,12.));
#161465=CARTESIAN_POINT('Ctrl Pts',(13.0291660060118,68.8535269726871,12.));
#161466=CARTESIAN_POINT('Ctrl Pts',(13.0377359881864,68.8712230321823,12.));
#161467=CARTESIAN_POINT('Ctrl Pts',(13.0463485518185,68.8889585151431,12.));
#161468=CARTESIAN_POINT('Ctrl Pts',(13.0550036938793,68.9067332040842,12.));
#161469=CARTESIAN_POINT('Ctrl Pts',(13.0637014089018,68.9245468449865,12.));
#161470=CARTESIAN_POINT('Ctrl Pts',(13.072441690283,68.9423991694493,12.));
#161471=CARTESIAN_POINT('Ctrl Pts',(13.0812245317816,68.9602899187628,12.));
#161472=CARTESIAN_POINT('Ctrl Pts',(13.0900499290542,68.9782188692654,12.));
#161473=CARTESIAN_POINT('Ctrl Pts',(13.0989178791843,68.9961858241577,12.));
#161474=CARTESIAN_POINT('Ctrl Pts',(13.1078283799726,69.0141906015137,12.));
#161475=CARTESIAN_POINT('Ctrl Pts',(13.1167814293495,69.0322330243336,12.));
#161476=CARTESIAN_POINT('Ctrl Pts',(13.1257770246379,69.0503129081778,12.));
#161477=CARTESIAN_POINT('Ctrl Pts',(13.1348151621824,69.0684300549426,12.));
#161478=CARTESIAN_POINT('Ctrl Pts',(13.1438958377397,69.0865842593063,12.));
#161479=CARTESIAN_POINT('Ctrl Pts',(13.1530190467181,69.1047753127633,12.));
#161480=CARTESIAN_POINT('Ctrl Pts',(13.1621847844533,69.1230030082598,12.));
#161481=CARTESIAN_POINT('Ctrl Pts',(13.1713930465142,69.141267145461,12.));
#161482=CARTESIAN_POINT('Ctrl Pts',(13.1806438286944,69.1595675305294,12.));
#161483=CARTESIAN_POINT('Ctrl Pts',(13.1899371268689,69.1779039736026,12.));
#161484=CARTESIAN_POINT('Ctrl Pts',(13.1992729368928,69.1962762870524,12.));
#161485=CARTESIAN_POINT('Ctrl Pts',(13.2086512544729,69.2146842833506,12.));
#161486=CARTESIAN_POINT('Ctrl Pts',(13.2180720750586,69.2331277732819,12.));
#161487=CARTESIAN_POINT('Ctrl Pts',(13.2275353939044,69.2516065668809,12.));
#161488=CARTESIAN_POINT('Ctrl Pts',(13.2370412061218,69.2701204742436,12.));
#161489=CARTESIAN_POINT('Ctrl Pts',(13.2465895067264,69.2886693063193,12.));
#161490=CARTESIAN_POINT('Ctrl Pts',(13.2561802906901,69.3072528758546,12.));
#161491=CARTESIAN_POINT('Ctrl Pts',(13.2658135529616,69.3258709977416,12.));
#161492=CARTESIAN_POINT('Ctrl Pts',(13.2754892884437,69.3445234885088,12.));
#161493=CARTESIAN_POINT('Ctrl Pts',(13.2852074919767,69.3632101660072,12.));
#161494=CARTESIAN_POINT('Ctrl Pts',(13.2949681583164,69.3819308490408,12.));
#161495=CARTESIAN_POINT('Ctrl Pts',(13.3047712821046,69.4006853569485,12.));
#161496=CARTESIAN_POINT('Ctrl Pts',(13.3146168578738,69.4194735096238,12.));
#161497=CARTESIAN_POINT('Ctrl Pts',(13.3245048800641,69.4382951276983,12.));
#161498=CARTESIAN_POINT('Ctrl Pts',(13.3344353430313,69.4571500326673,12.));
#161499=CARTESIAN_POINT('Ctrl Pts',(13.3444082410546,69.4760380470382,12.));
#161500=CARTESIAN_POINT('Ctrl Pts',(13.3544235683399,69.4949589944633,12.));
#161501=CARTESIAN_POINT('Ctrl Pts',(13.3644813190225,69.5139126996703,12.));
#161502=CARTESIAN_POINT('Ctrl Pts',(13.3745814871667,69.5328989883899,12.));
#161503=CARTESIAN_POINT('Ctrl Pts',(13.3847240667626,69.5519176872857,12.));
#161504=CARTESIAN_POINT('Ctrl Pts',(13.3949090517173,69.5709686238701,12.));
#161505=CARTESIAN_POINT('Ctrl Pts',(13.4051364358494,69.5900516264524,12.));
#161506=CARTESIAN_POINT('Ctrl Pts',(13.4154062128998,69.6091665241743,12.));
#161507=CARTESIAN_POINT('Ctrl Pts',(13.425718376534,69.6283131470267,12.));
#161508=CARTESIAN_POINT('Ctrl Pts',(13.4360729203444,69.6474913258684,12.));
#161509=CARTESIAN_POINT('Ctrl Pts',(13.4464698378456,69.6667008924454,12.));
#161510=CARTESIAN_POINT('Ctrl Pts',(13.4569091224762,69.6859416793898,12.));
#161511=CARTESIAN_POINT('Ctrl Pts',(13.4673907676045,69.7052135202003,12.));
#161512=CARTESIAN_POINT('Ctrl Pts',(13.4779147665285,69.7245162492251,12.));
#161513=CARTESIAN_POINT('Ctrl Pts',(13.4884811124748,69.7438497016404,12.));
#161514=CARTESIAN_POINT('Ctrl Pts',(13.4990897985904,69.7632137134247,12.));
#161515=CARTESIAN_POINT('Ctrl Pts',(13.5097408179478,69.7826081213575,12.));
#161516=CARTESIAN_POINT('Ctrl Pts',(13.5204341635507,69.8020327630204,12.));
#161517=CARTESIAN_POINT('Ctrl Pts',(13.5311698283339,69.8214874767944,12.));
#161518=CARTESIAN_POINT('Ctrl Pts',(13.5419478051626,69.840972101856,12.));
#161519=CARTESIAN_POINT('Ctrl Pts',(13.5527680868256,69.8604864781705,12.));
#161520=CARTESIAN_POINT('Ctrl Pts',(13.5636306660422,69.880030446488,12.));
#161521=CARTESIAN_POINT('Ctrl Pts',(13.5745355354657,69.899603848336,12.));
#161522=CARTESIAN_POINT('Ctrl Pts',(13.5854826876834,69.9192065260107,12.));
#161523=CARTESIAN_POINT('Ctrl Pts',(13.5964721152136,69.9388383225655,12.));
#161524=CARTESIAN_POINT('Ctrl Pts',(13.6075038105,69.9584990817989,12.));
#161525=CARTESIAN_POINT('Ctrl Pts',(13.61857776592,69.9781886482543,12.));
#161526=CARTESIAN_POINT('Ctrl Pts',(13.6296939737866,69.9979068672163,12.));
#161527=CARTESIAN_POINT('Ctrl Pts',(13.6408524263496,70.0176535847047,12.));
#161528=CARTESIAN_POINT('Ctrl Pts',(13.6520531157904,70.037428647466,12.));
#161529=CARTESIAN_POINT('Ctrl Pts',(13.6632960342192,70.057231902965,12.));
#161530=CARTESIAN_POINT('Ctrl Pts',(13.6745811736825,70.0770631993831,12.));
#161531=CARTESIAN_POINT('Ctrl Pts',(13.685908526165,70.0969223856123,12.));
#161532=CARTESIAN_POINT('Ctrl Pts',(13.6972780835898,70.1168093112493,12.));
#161533=CARTESIAN_POINT('Ctrl Pts',(13.7086898378127,70.1367238265853,12.));
#161534=CARTESIAN_POINT('Ctrl Pts',(13.7201437806207,70.1566657825989,12.));
#161535=CARTESIAN_POINT('Ctrl Pts',(13.73163990374,70.1766350309554,12.));
#161536=CARTESIAN_POINT('Ctrl Pts',(13.7431781988368,70.1966314240012,12.));
#161537=CARTESIAN_POINT('Ctrl Pts',(13.7547586575178,70.216654814759,12.));
#161538=CARTESIAN_POINT('Ctrl Pts',(13.7663812713235,70.2367050569174,12.));
#161539=CARTESIAN_POINT('Ctrl Pts',(13.7780460317284,70.2567820048253,12.));
#161540=CARTESIAN_POINT('Ctrl Pts',(13.7897529301483,70.2768855134909,12.));
#161541=CARTESIAN_POINT('Ctrl Pts',(13.8015019579411,70.2970154385763,12.));
#161542=CARTESIAN_POINT('Ctrl Pts',(13.8132931064067,70.3171716363912,12.));
#161543=CARTESIAN_POINT('Ctrl Pts',(13.8251263667799,70.3373539638841,12.));
#161544=CARTESIAN_POINT('Ctrl Pts',(13.8370017302319,70.3575622786373,12.));
#161545=CARTESIAN_POINT('Ctrl Pts',(13.8489191878774,70.377796438866,12.));
#161546=CARTESIAN_POINT('Ctrl Pts',(13.8608787307754,70.3980563034142,12.));
#161547=CARTESIAN_POINT('Ctrl Pts',(13.8728803499284,70.4183417317486,12.));
#161548=CARTESIAN_POINT('Ctrl Pts',(13.8849240362757,70.4386525839492,12.));
#161549=CARTESIAN_POINT('Ctrl Pts',(13.8970097806947,70.4589887207043,12.));
#161550=CARTESIAN_POINT('Ctrl Pts',(13.9091375740084,70.4793500033106,12.));
#161551=CARTESIAN_POINT('Ctrl Pts',(13.9213074069852,70.4997362936671,12.));
#161552=CARTESIAN_POINT('Ctrl Pts',(13.9335192703389,70.5201474542717,12.));
#161553=CARTESIAN_POINT('Ctrl Pts',(13.9457731547217,70.5405833482123,12.));
#161554=CARTESIAN_POINT('Ctrl Pts',(13.9580690507262,70.5610438391622,12.));
#161555=CARTESIAN_POINT('Ctrl Pts',(13.9704069488918,70.5815287913791,12.));
#161556=CARTESIAN_POINT('Ctrl Pts',(13.9827868397057,70.6020380697004,12.));
#161557=CARTESIAN_POINT('Ctrl Pts',(13.9952087136018,70.6225715395392,12.));
#161558=CARTESIAN_POINT('Ctrl Pts',(14.0076725609537,70.6431290668744,12.));
#161559=CARTESIAN_POINT('Ctrl Pts',(14.020178372077,70.6637105182487,12.));
#161560=CARTESIAN_POINT('Ctrl Pts',(14.0327261372363,70.6843157607672,12.));
#161561=CARTESIAN_POINT('Ctrl Pts',(14.0453158466451,70.7049446620931,12.));
#161562=CARTESIAN_POINT('Ctrl Pts',(14.0579474904657,70.7255970904433,12.));
#161563=CARTESIAN_POINT('Ctrl Pts',(14.0706210588015,70.7462729145799,12.));
#161564=CARTESIAN_POINT('Ctrl Pts',(14.0833365416995,70.7669720038067,12.));
#161565=CARTESIAN_POINT('Ctrl Pts',(14.0960939291568,70.787694227969,12.));
#161566=CARTESIAN_POINT('Ctrl Pts',(14.1088932111214,70.8084394574491,12.));
#161567=CARTESIAN_POINT('Ctrl Pts',(14.1217343774914,70.8292075631624,12.));
#161568=CARTESIAN_POINT('Ctrl Pts',(14.1346174181079,70.8499984165493,12.));
#161569=CARTESIAN_POINT('Ctrl Pts',(14.1475423227567,70.8708118895718,12.));
#161570=CARTESIAN_POINT('Ctrl Pts',(14.1605090811754,70.8916478547131,12.));
#161571=CARTESIAN_POINT('Ctrl Pts',(14.1735176830533,70.9125061849744,12.));
#161572=CARTESIAN_POINT('Ctrl Pts',(14.1865681180321,70.9333867538705,12.));
#161573=CARTESIAN_POINT('Ctrl Pts',(14.1996603756984,70.9542894354221,12.));
#161574=CARTESIAN_POINT('Ctrl Pts',(14.2127944455841,70.9752141041527,12.));
#161575=CARTESIAN_POINT('Ctrl Pts',(14.2259703171739,70.996160635087,12.));
#161576=CARTESIAN_POINT('Ctrl Pts',(14.2391879799063,71.0171289037493,12.));
#161577=CARTESIAN_POINT('Ctrl Pts',(14.2524474231732,71.0381187861585,12.));
#161578=CARTESIAN_POINT('Ctrl Pts',(14.2657486363136,71.059130158822,12.));
#161579=CARTESIAN_POINT('Ctrl Pts',(14.2790916086129,71.0801628987314,12.));
#161580=CARTESIAN_POINT('Ctrl Pts',(14.2924763293101,71.1012168833626,12.));
#161581=CARTESIAN_POINT('Ctrl Pts',(14.3059027875993,71.1222919906719,12.));
#161582=CARTESIAN_POINT('Ctrl Pts',(14.3193709726295,71.1433880990932,12.));
#161583=CARTESIAN_POINT('Ctrl Pts',(14.3328808734993,71.1645050875323,12.));
#161584=CARTESIAN_POINT('Ctrl Pts',(14.3464324792537,71.185642835361,12.));
#161585=CARTESIAN_POINT('Ctrl Pts',(14.3600257788927,71.2068012224187,12.));
#161586=CARTESIAN_POINT('Ctrl Pts',(14.3736607613723,71.2279801290088,12.));
#161587=CARTESIAN_POINT('Ctrl Pts',(14.3873374156056,71.2491794358956,12.));
#161588=CARTESIAN_POINT('Ctrl Pts',(14.401055730457,71.2703990242986,12.));
#161589=CARTESIAN_POINT('Ctrl Pts',(14.4148156947384,71.2916387758864,12.));
#161590=CARTESIAN_POINT('Ctrl Pts',(14.4286172972168,71.3128985727777,12.));
#161591=CARTESIAN_POINT('Ctrl Pts',(14.4424605266166,71.3341782975393,12.));
#161592=CARTESIAN_POINT('Ctrl Pts',(14.4563453716204,71.3554778331835,12.));
#161593=CARTESIAN_POINT('Ctrl Pts',(14.470271820865,71.3767970631642,12.));
#161594=CARTESIAN_POINT('Ctrl Pts',(14.4842398629353,71.398135871371,12.));
#161595=CARTESIAN_POINT('Ctrl Pts',(14.4982494863716,71.4194941421279,12.));
#161596=CARTESIAN_POINT('Ctrl Pts',(14.5123006796728,71.4408717601917,12.));
#161597=CARTESIAN_POINT('Ctrl Pts',(14.5263934312969,71.4622686107475,12.));
#161598=CARTESIAN_POINT('Ctrl Pts',(14.540527729659,71.4836845794052,12.));
#161599=CARTESIAN_POINT('Ctrl Pts',(14.5547035631234,71.5051195521914,12.));
#161600=CARTESIAN_POINT('Ctrl Pts',(14.568920920009,71.5265734155501,12.));
#161601=CARTESIAN_POINT('Ctrl Pts',(14.5831797885951,71.5480460563445,12.));
#161602=CARTESIAN_POINT('Ctrl Pts',(14.597480157121,71.569537361856,12.));
#161603=CARTESIAN_POINT('Ctrl Pts',(14.611822013785,71.5910472197815,12.));
#161604=CARTESIAN_POINT('Ctrl Pts',(14.6262053467372,71.6125755182295,12.));
#161605=CARTESIAN_POINT('Ctrl Pts',(14.6406301440817,71.6341221457175,12.));
#161606=CARTESIAN_POINT('Ctrl Pts',(14.6550963938832,71.6556869911669,12.));
#161607=CARTESIAN_POINT('Ctrl Pts',(14.6696040841679,71.6772699438966,12.));
#161608=CARTESIAN_POINT('Ctrl Pts',(14.6841532029231,71.698870893617,12.));
#161609=CARTESIAN_POINT('Ctrl Pts',(14.6987437380898,71.7204897304186,12.));
#161610=CARTESIAN_POINT('Ctrl Pts',(14.7133756775622,71.7421263447707,12.));
#161611=CARTESIAN_POINT('Ctrl Pts',(14.7280490091954,71.7637806275316,12.));
#161612=CARTESIAN_POINT('Ctrl Pts',(14.7427637208071,71.7854524699563,12.));
#161613=CARTESIAN_POINT('Ctrl Pts',(14.7575198001776,71.8071417637019,12.));
#161614=CARTESIAN_POINT('Ctrl Pts',(14.7723172350454,71.8288484008343,12.));
#161615=CARTESIAN_POINT('Ctrl Pts',(14.7871560131021,71.8505722738286,12.));
#161616=CARTESIAN_POINT('Ctrl Pts',(14.8020361220003,71.872313275546,12.));
#161617=CARTESIAN_POINT('Ctrl Pts',(14.816957549356,71.8940712992119,12.));
#161618=CARTESIAN_POINT('Ctrl Pts',(14.8319202827482,71.9158462383915,12.));
#161619=CARTESIAN_POINT('Ctrl Pts',(14.846924309716,71.9376379869668,12.));
#161620=CARTESIAN_POINT('Ctrl Pts',(14.8619696177503,71.9594464391063,12.));
#161621=CARTESIAN_POINT('Ctrl Pts',(14.8770561943011,71.9812714893087,12.));
#161622=CARTESIAN_POINT('Ctrl Pts',(14.892184026783,72.0031130324519,12.));
#161623=CARTESIAN_POINT('Ctrl Pts',(14.9073531025763,72.0249709638419,12.));
#161624=CARTESIAN_POINT('Ctrl Pts',(14.9225634090269,72.046845179251,12.));
#161625=CARTESIAN_POINT('Ctrl Pts',(14.937814933439,72.0687355749815,12.));
#161626=CARTESIAN_POINT('Ctrl Pts',(14.953107663077,72.0906420478085,12.));
#161627=CARTESIAN_POINT('Ctrl Pts',(14.9684415851699,72.1125644948547,12.));
#161628=CARTESIAN_POINT('Ctrl Pts',(14.9838166869107,72.1345028134779,12.));
#161629=CARTESIAN_POINT('Ctrl Pts',(14.9992329554537,72.1564569011668,12.));
#161630=CARTESIAN_POINT('Ctrl Pts',(15.0146903779061,72.1784266553948,12.));
#161631=CARTESIAN_POINT('Ctrl Pts',(15.0301889413255,72.2004119736104,12.));
#161632=CARTESIAN_POINT('Ctrl Pts',(15.0457286327328,72.2224127535401,12.));
#161633=CARTESIAN_POINT('Ctrl Pts',(15.0613094391186,72.244428893425,12.));
#161634=CARTESIAN_POINT('Ctrl Pts',(15.0769313474476,72.266460292285,12.));
#161635=CARTESIAN_POINT('Ctrl Pts',(15.0925943446593,72.2885068501641,12.));
#161636=CARTESIAN_POINT('Ctrl Pts',(15.1082984176655,72.3105684683971,12.));
#161637=CARTESIAN_POINT('Ctrl Pts',(15.1240435533478,72.332645049021,12.));
#161638=CARTESIAN_POINT('Ctrl Pts',(15.1398297385513,72.3547364941996,12.));
#161639=CARTESIAN_POINT('Ctrl Pts',(15.1556569600747,72.37684270559,12.));
#161640=CARTESIAN_POINT('Ctrl Pts',(15.1715252046602,72.3989635838476,12.));
#161641=CARTESIAN_POINT('Ctrl Pts',(15.1874344589716,72.4210990277819,12.));
#161642=CARTESIAN_POINT('Ctrl Pts',(15.2033847096077,72.4432489350415,12.));
#161643=CARTESIAN_POINT('Ctrl Pts',(15.2193759431359,72.4654132036373,12.));
#161644=CARTESIAN_POINT('Ctrl Pts',(15.2354081461152,72.4875917332729,12.));
#161645=CARTESIAN_POINT('Ctrl Pts',(15.2514813051174,72.5097844266083,12.));
#161646=CARTESIAN_POINT('Ctrl Pts',(15.2675954067495,72.5319911908978,12.));
#161647=CARTESIAN_POINT('Ctrl Pts',(15.2837504376562,72.5542119383748,12.));
#161648=CARTESIAN_POINT('Ctrl Pts',(15.2976335024853,72.5732713370797,12.));
#161649=CARTESIAN_POINT('Ctrl Pts',(15.3082994603653,72.5878912620665,12.));
#161650=CARTESIAN_POINT('Ctrl Pts',(15.3157301930835,72.5980655789901,12.));
#161651=CARTESIAN_POINT('Ctrl Pts',(15.3199137230322,72.6037902605231,12.));
#161652=CARTESIAN_POINT('Ctrl Pts',(15.3208442077425,72.6050633494718,12.));
#161653=CARTESIAN_POINT('',(12.9953224629497,68.7831490561748,0.));
#161654=CARTESIAN_POINT('',(12.9953224629497,68.7831490561748,0.));
#161655=CARTESIAN_POINT('Ctrl Pts',(15.3208442077425,72.6050633494718,0.));
#161656=CARTESIAN_POINT('Ctrl Pts',(15.3199137230322,72.6037902605231,0.));
#161657=CARTESIAN_POINT('Ctrl Pts',(15.3157301930835,72.5980655789901,0.));
#161658=CARTESIAN_POINT('Ctrl Pts',(15.3082994603653,72.5878912620665,0.));
#161659=CARTESIAN_POINT('Ctrl Pts',(15.2976335024853,72.5732713370797,0.));
#161660=CARTESIAN_POINT('Ctrl Pts',(15.2837504376562,72.5542119383748,0.));
#161661=CARTESIAN_POINT('Ctrl Pts',(15.2675954067495,72.5319911908978,0.));
#161662=CARTESIAN_POINT('Ctrl Pts',(15.2514813051174,72.5097844266083,0.));
#161663=CARTESIAN_POINT('Ctrl Pts',(15.2354081461152,72.4875917332729,0.));
#161664=CARTESIAN_POINT('Ctrl Pts',(15.2193759431359,72.4654132036373,0.));
#161665=CARTESIAN_POINT('Ctrl Pts',(15.2033847096077,72.4432489350415,0.));
#161666=CARTESIAN_POINT('Ctrl Pts',(15.1874344589716,72.4210990277819,0.));
#161667=CARTESIAN_POINT('Ctrl Pts',(15.1715252046602,72.3989635838476,0.));
#161668=CARTESIAN_POINT('Ctrl Pts',(15.1556569600747,72.37684270559,0.));
#161669=CARTESIAN_POINT('Ctrl Pts',(15.1398297385513,72.3547364941996,0.));
#161670=CARTESIAN_POINT('Ctrl Pts',(15.1240435533478,72.332645049021,0.));
#161671=CARTESIAN_POINT('Ctrl Pts',(15.1082984176655,72.3105684683971,0.));
#161672=CARTESIAN_POINT('Ctrl Pts',(15.0925943446593,72.2885068501641,0.));
#161673=CARTESIAN_POINT('Ctrl Pts',(15.0769313474476,72.266460292285,0.));
#161674=CARTESIAN_POINT('Ctrl Pts',(15.0613094391186,72.244428893425,0.));
#161675=CARTESIAN_POINT('Ctrl Pts',(15.0457286327328,72.2224127535401,0.));
#161676=CARTESIAN_POINT('Ctrl Pts',(15.0301889413255,72.2004119736104,0.));
#161677=CARTESIAN_POINT('Ctrl Pts',(15.0146903779061,72.1784266553948,0.));
#161678=CARTESIAN_POINT('Ctrl Pts',(14.9992329554537,72.1564569011668,0.));
#161679=CARTESIAN_POINT('Ctrl Pts',(14.9838166869107,72.1345028134779,0.));
#161680=CARTESIAN_POINT('Ctrl Pts',(14.9684415851699,72.1125644948547,0.));
#161681=CARTESIAN_POINT('Ctrl Pts',(14.953107663077,72.0906420478085,0.));
#161682=CARTESIAN_POINT('Ctrl Pts',(14.937814933439,72.0687355749815,0.));
#161683=CARTESIAN_POINT('Ctrl Pts',(14.9225634090269,72.046845179251,0.));
#161684=CARTESIAN_POINT('Ctrl Pts',(14.9073531025763,72.0249709638419,0.));
#161685=CARTESIAN_POINT('Ctrl Pts',(14.892184026783,72.0031130324519,0.));
#161686=CARTESIAN_POINT('Ctrl Pts',(14.8770561943011,71.9812714893087,0.));
#161687=CARTESIAN_POINT('Ctrl Pts',(14.8619696177503,71.9594464391063,0.));
#161688=CARTESIAN_POINT('Ctrl Pts',(14.846924309716,71.9376379869668,0.));
#161689=CARTESIAN_POINT('Ctrl Pts',(14.8319202827482,71.9158462383915,0.));
#161690=CARTESIAN_POINT('Ctrl Pts',(14.816957549356,71.8940712992119,0.));
#161691=CARTESIAN_POINT('Ctrl Pts',(14.8020361220003,71.872313275546,0.));
#161692=CARTESIAN_POINT('Ctrl Pts',(14.7871560131021,71.8505722738286,0.));
#161693=CARTESIAN_POINT('Ctrl Pts',(14.7723172350454,71.8288484008343,0.));
#161694=CARTESIAN_POINT('Ctrl Pts',(14.7575198001776,71.8071417637019,0.));
#161695=CARTESIAN_POINT('Ctrl Pts',(14.7427637208071,71.7854524699563,0.));
#161696=CARTESIAN_POINT('Ctrl Pts',(14.7280490091954,71.7637806275316,0.));
#161697=CARTESIAN_POINT('Ctrl Pts',(14.7133756775622,71.7421263447707,0.));
#161698=CARTESIAN_POINT('Ctrl Pts',(14.6987437380898,71.7204897304186,0.));
#161699=CARTESIAN_POINT('Ctrl Pts',(14.6841532029231,71.698870893617,0.));
#161700=CARTESIAN_POINT('Ctrl Pts',(14.6696040841679,71.6772699438966,0.));
#161701=CARTESIAN_POINT('Ctrl Pts',(14.6550963938832,71.6556869911669,0.));
#161702=CARTESIAN_POINT('Ctrl Pts',(14.6406301440817,71.6341221457175,0.));
#161703=CARTESIAN_POINT('Ctrl Pts',(14.6262053467372,71.6125755182295,0.));
#161704=CARTESIAN_POINT('Ctrl Pts',(14.611822013785,71.5910472197815,0.));
#161705=CARTESIAN_POINT('Ctrl Pts',(14.597480157121,71.569537361856,0.));
#161706=CARTESIAN_POINT('Ctrl Pts',(14.5831797885951,71.5480460563445,0.));
#161707=CARTESIAN_POINT('Ctrl Pts',(14.568920920009,71.5265734155501,0.));
#161708=CARTESIAN_POINT('Ctrl Pts',(14.5547035631234,71.5051195521914,0.));
#161709=CARTESIAN_POINT('Ctrl Pts',(14.540527729659,71.4836845794052,0.));
#161710=CARTESIAN_POINT('Ctrl Pts',(14.5263934312969,71.4622686107475,0.));
#161711=CARTESIAN_POINT('Ctrl Pts',(14.5123006796728,71.4408717601917,0.));
#161712=CARTESIAN_POINT('Ctrl Pts',(14.4982494863716,71.4194941421279,0.));
#161713=CARTESIAN_POINT('Ctrl Pts',(14.4842398629353,71.398135871371,0.));
#161714=CARTESIAN_POINT('Ctrl Pts',(14.470271820865,71.3767970631642,0.));
#161715=CARTESIAN_POINT('Ctrl Pts',(14.4563453716204,71.3554778331835,0.));
#161716=CARTESIAN_POINT('Ctrl Pts',(14.4424605266166,71.3341782975393,0.));
#161717=CARTESIAN_POINT('Ctrl Pts',(14.4286172972168,71.3128985727777,0.));
#161718=CARTESIAN_POINT('Ctrl Pts',(14.4148156947384,71.2916387758864,0.));
#161719=CARTESIAN_POINT('Ctrl Pts',(14.401055730457,71.2703990242986,0.));
#161720=CARTESIAN_POINT('Ctrl Pts',(14.3873374156056,71.2491794358956,0.));
#161721=CARTESIAN_POINT('Ctrl Pts',(14.3736607613723,71.2279801290088,0.));
#161722=CARTESIAN_POINT('Ctrl Pts',(14.3600257788927,71.2068012224187,0.));
#161723=CARTESIAN_POINT('Ctrl Pts',(14.3464324792537,71.185642835361,0.));
#161724=CARTESIAN_POINT('Ctrl Pts',(14.3328808734993,71.1645050875323,0.));
#161725=CARTESIAN_POINT('Ctrl Pts',(14.3193709726295,71.1433880990932,0.));
#161726=CARTESIAN_POINT('Ctrl Pts',(14.3059027875993,71.1222919906719,0.));
#161727=CARTESIAN_POINT('Ctrl Pts',(14.2924763293101,71.1012168833626,0.));
#161728=CARTESIAN_POINT('Ctrl Pts',(14.2790916086129,71.0801628987314,0.));
#161729=CARTESIAN_POINT('Ctrl Pts',(14.2657486363136,71.059130158822,0.));
#161730=CARTESIAN_POINT('Ctrl Pts',(14.2524474231732,71.0381187861585,0.));
#161731=CARTESIAN_POINT('Ctrl Pts',(14.2391879799063,71.0171289037493,0.));
#161732=CARTESIAN_POINT('Ctrl Pts',(14.2259703171739,70.996160635087,0.));
#161733=CARTESIAN_POINT('Ctrl Pts',(14.2127944455841,70.9752141041527,0.));
#161734=CARTESIAN_POINT('Ctrl Pts',(14.1996603756984,70.9542894354221,0.));
#161735=CARTESIAN_POINT('Ctrl Pts',(14.1865681180321,70.9333867538705,0.));
#161736=CARTESIAN_POINT('Ctrl Pts',(14.1735176830533,70.9125061849744,0.));
#161737=CARTESIAN_POINT('Ctrl Pts',(14.1605090811754,70.8916478547131,0.));
#161738=CARTESIAN_POINT('Ctrl Pts',(14.1475423227567,70.8708118895718,0.));
#161739=CARTESIAN_POINT('Ctrl Pts',(14.1346174181079,70.8499984165493,0.));
#161740=CARTESIAN_POINT('Ctrl Pts',(14.1217343774914,70.8292075631624,0.));
#161741=CARTESIAN_POINT('Ctrl Pts',(14.1088932111214,70.8084394574491,0.));
#161742=CARTESIAN_POINT('Ctrl Pts',(14.0960939291568,70.787694227969,0.));
#161743=CARTESIAN_POINT('Ctrl Pts',(14.0833365416995,70.7669720038067,0.));
#161744=CARTESIAN_POINT('Ctrl Pts',(14.0706210588015,70.7462729145799,0.));
#161745=CARTESIAN_POINT('Ctrl Pts',(14.0579474904657,70.7255970904433,0.));
#161746=CARTESIAN_POINT('Ctrl Pts',(14.0453158466451,70.7049446620931,0.));
#161747=CARTESIAN_POINT('Ctrl Pts',(14.0327261372363,70.6843157607672,0.));
#161748=CARTESIAN_POINT('Ctrl Pts',(14.020178372077,70.6637105182487,0.));
#161749=CARTESIAN_POINT('Ctrl Pts',(14.0076725609537,70.6431290668744,0.));
#161750=CARTESIAN_POINT('Ctrl Pts',(13.9952087136018,70.6225715395392,0.));
#161751=CARTESIAN_POINT('Ctrl Pts',(13.9827868397057,70.6020380697004,0.));
#161752=CARTESIAN_POINT('Ctrl Pts',(13.9704069488918,70.5815287913791,0.));
#161753=CARTESIAN_POINT('Ctrl Pts',(13.9580690507262,70.5610438391622,0.));
#161754=CARTESIAN_POINT('Ctrl Pts',(13.9457731547217,70.5405833482123,0.));
#161755=CARTESIAN_POINT('Ctrl Pts',(13.9335192703389,70.5201474542717,0.));
#161756=CARTESIAN_POINT('Ctrl Pts',(13.9213074069852,70.4997362936671,0.));
#161757=CARTESIAN_POINT('Ctrl Pts',(13.9091375740084,70.4793500033106,0.));
#161758=CARTESIAN_POINT('Ctrl Pts',(13.8970097806947,70.4589887207043,0.));
#161759=CARTESIAN_POINT('Ctrl Pts',(13.8849240362757,70.4386525839492,0.));
#161760=CARTESIAN_POINT('Ctrl Pts',(13.8728803499284,70.4183417317486,0.));
#161761=CARTESIAN_POINT('Ctrl Pts',(13.8608787307754,70.3980563034142,0.));
#161762=CARTESIAN_POINT('Ctrl Pts',(13.8489191878774,70.377796438866,0.));
#161763=CARTESIAN_POINT('Ctrl Pts',(13.8370017302319,70.3575622786373,0.));
#161764=CARTESIAN_POINT('Ctrl Pts',(13.8251263667799,70.3373539638841,0.));
#161765=CARTESIAN_POINT('Ctrl Pts',(13.8132931064067,70.3171716363912,0.));
#161766=CARTESIAN_POINT('Ctrl Pts',(13.8015019579411,70.2970154385763,0.));
#161767=CARTESIAN_POINT('Ctrl Pts',(13.7897529301483,70.2768855134909,0.));
#161768=CARTESIAN_POINT('Ctrl Pts',(13.7780460317284,70.2567820048253,0.));
#161769=CARTESIAN_POINT('Ctrl Pts',(13.7663812713235,70.2367050569174,0.));
#161770=CARTESIAN_POINT('Ctrl Pts',(13.7547586575178,70.216654814759,0.));
#161771=CARTESIAN_POINT('Ctrl Pts',(13.7431781988368,70.1966314240012,0.));
#161772=CARTESIAN_POINT('Ctrl Pts',(13.73163990374,70.1766350309554,0.));
#161773=CARTESIAN_POINT('Ctrl Pts',(13.7201437806207,70.1566657825989,0.));
#161774=CARTESIAN_POINT('Ctrl Pts',(13.7086898378127,70.1367238265853,0.));
#161775=CARTESIAN_POINT('Ctrl Pts',(13.6972780835898,70.1168093112493,0.));
#161776=CARTESIAN_POINT('Ctrl Pts',(13.685908526165,70.0969223856123,0.));
#161777=CARTESIAN_POINT('Ctrl Pts',(13.6745811736825,70.0770631993831,0.));
#161778=CARTESIAN_POINT('Ctrl Pts',(13.6632960342192,70.057231902965,0.));
#161779=CARTESIAN_POINT('Ctrl Pts',(13.6520531157904,70.037428647466,0.));
#161780=CARTESIAN_POINT('Ctrl Pts',(13.6408524263496,70.0176535847047,0.));
#161781=CARTESIAN_POINT('Ctrl Pts',(13.6296939737866,69.9979068672163,0.));
#161782=CARTESIAN_POINT('Ctrl Pts',(13.61857776592,69.9781886482543,0.));
#161783=CARTESIAN_POINT('Ctrl Pts',(13.6075038105,69.9584990817989,0.));
#161784=CARTESIAN_POINT('Ctrl Pts',(13.5964721152136,69.9388383225655,0.));
#161785=CARTESIAN_POINT('Ctrl Pts',(13.5854826876834,69.9192065260107,0.));
#161786=CARTESIAN_POINT('Ctrl Pts',(13.5745355354657,69.899603848336,0.));
#161787=CARTESIAN_POINT('Ctrl Pts',(13.5636306660422,69.880030446488,0.));
#161788=CARTESIAN_POINT('Ctrl Pts',(13.5527680868256,69.8604864781705,0.));
#161789=CARTESIAN_POINT('Ctrl Pts',(13.5419478051626,69.840972101856,0.));
#161790=CARTESIAN_POINT('Ctrl Pts',(13.5311698283339,69.8214874767944,0.));
#161791=CARTESIAN_POINT('Ctrl Pts',(13.5204341635507,69.8020327630204,0.));
#161792=CARTESIAN_POINT('Ctrl Pts',(13.5097408179478,69.7826081213575,0.));
#161793=CARTESIAN_POINT('Ctrl Pts',(13.4990897985904,69.7632137134247,0.));
#161794=CARTESIAN_POINT('Ctrl Pts',(13.4884811124748,69.7438497016404,0.));
#161795=CARTESIAN_POINT('Ctrl Pts',(13.4779147665285,69.7245162492251,0.));
#161796=CARTESIAN_POINT('Ctrl Pts',(13.4673907676045,69.7052135202003,0.));
#161797=CARTESIAN_POINT('Ctrl Pts',(13.4569091224762,69.6859416793898,0.));
#161798=CARTESIAN_POINT('Ctrl Pts',(13.4464698378456,69.6667008924454,0.));
#161799=CARTESIAN_POINT('Ctrl Pts',(13.4360729203444,69.6474913258684,0.));
#161800=CARTESIAN_POINT('Ctrl Pts',(13.425718376534,69.6283131470267,0.));
#161801=CARTESIAN_POINT('Ctrl Pts',(13.4154062128998,69.6091665241743,0.));
#161802=CARTESIAN_POINT('Ctrl Pts',(13.4051364358494,69.5900516264524,0.));
#161803=CARTESIAN_POINT('Ctrl Pts',(13.3949090517173,69.5709686238701,0.));
#161804=CARTESIAN_POINT('Ctrl Pts',(13.3847240667626,69.5519176872857,0.));
#161805=CARTESIAN_POINT('Ctrl Pts',(13.3745814871667,69.5328989883899,0.));
#161806=CARTESIAN_POINT('Ctrl Pts',(13.3644813190225,69.5139126996703,0.));
#161807=CARTESIAN_POINT('Ctrl Pts',(13.3544235683399,69.4949589944633,0.));
#161808=CARTESIAN_POINT('Ctrl Pts',(13.3444082410546,69.4760380470382,0.));
#161809=CARTESIAN_POINT('Ctrl Pts',(13.3344353430313,69.4571500326673,0.));
#161810=CARTESIAN_POINT('Ctrl Pts',(13.3245048800641,69.4382951276983,0.));
#161811=CARTESIAN_POINT('Ctrl Pts',(13.3146168578738,69.4194735096238,0.));
#161812=CARTESIAN_POINT('Ctrl Pts',(13.3047712821046,69.4006853569485,0.));
#161813=CARTESIAN_POINT('Ctrl Pts',(13.2949681583164,69.3819308490408,0.));
#161814=CARTESIAN_POINT('Ctrl Pts',(13.2852074919767,69.3632101660072,0.));
#161815=CARTESIAN_POINT('Ctrl Pts',(13.2754892884437,69.3445234885088,0.));
#161816=CARTESIAN_POINT('Ctrl Pts',(13.2658135529616,69.3258709977416,0.));
#161817=CARTESIAN_POINT('Ctrl Pts',(13.2561802906901,69.3072528758546,0.));
#161818=CARTESIAN_POINT('Ctrl Pts',(13.2465895067264,69.2886693063193,0.));
#161819=CARTESIAN_POINT('Ctrl Pts',(13.2370412061218,69.2701204742436,0.));
#161820=CARTESIAN_POINT('Ctrl Pts',(13.2275353939044,69.2516065668809,0.));
#161821=CARTESIAN_POINT('Ctrl Pts',(13.2180720750586,69.2331277732819,0.));
#161822=CARTESIAN_POINT('Ctrl Pts',(13.2086512544729,69.2146842833506,0.));
#161823=CARTESIAN_POINT('Ctrl Pts',(13.1992729368928,69.1962762870524,0.));
#161824=CARTESIAN_POINT('Ctrl Pts',(13.1899371268689,69.1779039736026,0.));
#161825=CARTESIAN_POINT('Ctrl Pts',(13.1806438286944,69.1595675305294,0.));
#161826=CARTESIAN_POINT('Ctrl Pts',(13.1713930465142,69.141267145461,0.));
#161827=CARTESIAN_POINT('Ctrl Pts',(13.1621847844533,69.1230030082598,0.));
#161828=CARTESIAN_POINT('Ctrl Pts',(13.1530190467181,69.1047753127633,0.));
#161829=CARTESIAN_POINT('Ctrl Pts',(13.1438958377397,69.0865842593063,0.));
#161830=CARTESIAN_POINT('Ctrl Pts',(13.1348151621824,69.0684300549426,0.));
#161831=CARTESIAN_POINT('Ctrl Pts',(13.1257770246379,69.0503129081778,0.));
#161832=CARTESIAN_POINT('Ctrl Pts',(13.1167814293495,69.0322330243336,0.));
#161833=CARTESIAN_POINT('Ctrl Pts',(13.1078283799726,69.0141906015137,0.));
#161834=CARTESIAN_POINT('Ctrl Pts',(13.0989178791843,68.9961858241577,0.));
#161835=CARTESIAN_POINT('Ctrl Pts',(13.0900499290542,68.9782188692654,0.));
#161836=CARTESIAN_POINT('Ctrl Pts',(13.0812245317816,68.9602899187628,0.));
#161837=CARTESIAN_POINT('Ctrl Pts',(13.072441690283,68.9423991694493,0.));
#161838=CARTESIAN_POINT('Ctrl Pts',(13.0637014089018,68.9245468449865,0.));
#161839=CARTESIAN_POINT('Ctrl Pts',(13.0550036938793,68.9067332040842,0.));
#161840=CARTESIAN_POINT('Ctrl Pts',(13.0463485518185,68.8889585151431,0.));
#161841=CARTESIAN_POINT('Ctrl Pts',(13.0377359881864,68.8712230321823,0.));
#161842=CARTESIAN_POINT('Ctrl Pts',(13.0291660060118,68.8535269726871,0.));
#161843=CARTESIAN_POINT('Ctrl Pts',(13.0206386039729,68.835870488774,0.));
#161844=CARTESIAN_POINT('Ctrl Pts',(13.0121537769003,68.8182536654067,0.));
#161845=CARTESIAN_POINT('Ctrl Pts',(13.0053999700929,68.8041919669403,0.));
#161846=CARTESIAN_POINT('Ctrl Pts',(13.0003537683089,68.7936635625788,0.));
#161847=CARTESIAN_POINT('Ctrl Pts',(12.996998146029,68.7866525680284,0.));
#161848=CARTESIAN_POINT('Ctrl Pts',(12.9953224629497,68.7831490561748,0.));
#161849=CARTESIAN_POINT('Ctrl Pts',(21.8059378310719,71.2372871136137,0.));
#161850=CARTESIAN_POINT('Ctrl Pts',(21.8059378310719,71.2372871136137,12.));
#161851=CARTESIAN_POINT('Ctrl Pts',(21.8022104901727,71.2331134397872,0.));
#161852=CARTESIAN_POINT('Ctrl Pts',(21.8022104901727,71.2331134397872,12.));
#161853=CARTESIAN_POINT('Ctrl Pts',(21.794759979896,71.2247670210176,0.));
#161854=CARTESIAN_POINT('Ctrl Pts',(21.794759979896,71.2247670210176,12.));
#161855=CARTESIAN_POINT('Ctrl Pts',(21.7835967290463,71.2122501795138,0.));
#161856=CARTESIAN_POINT('Ctrl Pts',(21.7835967290463,71.2122501795138,12.));
#161857=CARTESIAN_POINT('Ctrl Pts',(21.7687374247287,71.1955666310295,0.));
#161858=CARTESIAN_POINT('Ctrl Pts',(21.7687374247287,71.1955666310295,12.));
#161859=CARTESIAN_POINT('Ctrl Pts',(21.750205018381,71.1747214906585,0.));
#161860=CARTESIAN_POINT('Ctrl Pts',(21.750205018381,71.1747214906585,12.));
#161861=CARTESIAN_POINT('Ctrl Pts',(21.7317143472951,71.1538856612261,0.));
#161862=CARTESIAN_POINT('Ctrl Pts',(21.7317143472951,71.1538856612261,12.));
#161863=CARTESIAN_POINT('Ctrl Pts',(21.7132654262531,71.1330591726507,0.));
#161864=CARTESIAN_POINT('Ctrl Pts',(21.7132654262531,71.1330591726507,12.));
#161865=CARTESIAN_POINT('Ctrl Pts',(21.694858273085,71.1122420728217,0.));
#161866=CARTESIAN_POINT('Ctrl Pts',(21.694858273085,71.1122420728217,12.));
#161867=CARTESIAN_POINT('Ctrl Pts',(21.6764929081677,71.0914344332798,0.));
#161868=CARTESIAN_POINT('Ctrl Pts',(21.6764929081677,71.0914344332798,12.));
#161869=CARTESIAN_POINT('Ctrl Pts',(21.6581693538335,71.0706363472704,0.));
#161870=CARTESIAN_POINT('Ctrl Pts',(21.6581693538335,71.0706363472704,12.));
#161871=CARTESIAN_POINT('Ctrl Pts',(21.639887633714,71.0498479219467,0.));
#161872=CARTESIAN_POINT('Ctrl Pts',(21.639887633714,71.0498479219467,12.));
#161873=CARTESIAN_POINT('Ctrl Pts',(21.6216477720912,71.0290692721848,0.));
#161874=CARTESIAN_POINT('Ctrl Pts',(21.6216477720912,71.0290692721848,12.));
#161875=CARTESIAN_POINT('Ctrl Pts',(21.6034497932581,71.0083005139107,0.));
#161876=CARTESIAN_POINT('Ctrl Pts',(21.6034497932581,71.0083005139107,12.));
#161877=CARTESIAN_POINT('Ctrl Pts',(21.585293720829,70.987541757223,0.));
#161878=CARTESIAN_POINT('Ctrl Pts',(21.585293720829,70.987541757223,12.));
#161879=CARTESIAN_POINT('Ctrl Pts',(21.5671795771913,70.9667931008215,0.));
#161880=CARTESIAN_POINT('Ctrl Pts',(21.5671795771913,70.9667931008215,12.));
#161881=CARTESIAN_POINT('Ctrl Pts',(21.5491073839106,70.94605463587,0.));
#161882=CARTESIAN_POINT('Ctrl Pts',(21.5491073839106,70.94605463587,12.));
#161883=CARTESIAN_POINT('Ctrl Pts',(21.531077162023,70.9253264487637,0.));
#161884=CARTESIAN_POINT('Ctrl Pts',(21.531077162023,70.9253264487637,12.));
#161885=CARTESIAN_POINT('Ctrl Pts',(21.513088932377,70.9046086244131,0.));
#161886=CARTESIAN_POINT('Ctrl Pts',(21.513088932377,70.9046086244131,12.));
#161887=CARTESIAN_POINT('Ctrl Pts',(21.4951427159261,70.8839012490871,0.));
#161888=CARTESIAN_POINT('Ctrl Pts',(21.4951427159261,70.8839012490871,12.));
#161889=CARTESIAN_POINT('Ctrl Pts',(21.477238534096,70.8632044140112,0.));
#161890=CARTESIAN_POINT('Ctrl Pts',(21.477238534096,70.8632044140112,12.));
#161891=CARTESIAN_POINT('Ctrl Pts',(21.4593764087473,70.8425182149846,0.));
#161892=CARTESIAN_POINT('Ctrl Pts',(21.4593764087473,70.8425182149846,12.));
#161893=CARTESIAN_POINT('Ctrl Pts',(21.4415563620114,70.8218427507506,0.));
#161894=CARTESIAN_POINT('Ctrl Pts',(21.4415563620114,70.8218427507506,12.));
#161895=CARTESIAN_POINT('Ctrl Pts',(21.4237784161587,70.8011781217394,0.));
#161896=CARTESIAN_POINT('Ctrl Pts',(21.4237784161587,70.8011781217394,12.));
#161897=CARTESIAN_POINT('Ctrl Pts',(21.4060425934598,70.780524428745,0.));
#161898=CARTESIAN_POINT('Ctrl Pts',(21.4060425934598,70.780524428745,12.));
#161899=CARTESIAN_POINT('Ctrl Pts',(21.3883489160196,70.7598817714105,0.));
#161900=CARTESIAN_POINT('Ctrl Pts',(21.3883489160196,70.7598817714105,12.));
#161901=CARTESIAN_POINT('Ctrl Pts',(21.3706974057039,70.7392502475469,0.));
#161902=CARTESIAN_POINT('Ctrl Pts',(21.3706974057039,70.7392502475469,12.));
#161903=CARTESIAN_POINT('Ctrl Pts',(21.3530880842349,70.7186299539724,0.));
#161904=CARTESIAN_POINT('Ctrl Pts',(21.3530880842349,70.7186299539724,12.));
#161905=CARTESIAN_POINT('Ctrl Pts',(21.3355209732443,70.6980209870045,0.));
#161906=CARTESIAN_POINT('Ctrl Pts',(21.3355209732443,70.6980209870045,12.));
#161907=CARTESIAN_POINT('Ctrl Pts',(21.3179960943388,70.6774234430897,0.));
#161908=CARTESIAN_POINT('Ctrl Pts',(21.3179960943388,70.6774234430897,12.));
#161909=CARTESIAN_POINT('Ctrl Pts',(21.300513469156,70.6568374193774,0.));
#161910=CARTESIAN_POINT('Ctrl Pts',(21.300513469156,70.6568374193774,12.));
#161911=CARTESIAN_POINT('Ctrl Pts',(21.2830731194183,70.6362630143047,0.));
#161912=CARTESIAN_POINT('Ctrl Pts',(21.2830731194183,70.6362630143047,12.));
#161913=CARTESIAN_POINT('Ctrl Pts',(21.2656750669126,70.6157003273316,0.));
#161914=CARTESIAN_POINT('Ctrl Pts',(21.2656750669126,70.6157003273316,12.));
#161915=CARTESIAN_POINT('Ctrl Pts',(21.2483193334675,70.5951494586957,0.));
#161916=CARTESIAN_POINT('Ctrl Pts',(21.2483193334675,70.5951494586957,12.));
#161917=CARTESIAN_POINT('Ctrl Pts',(21.2310059409265,70.5746105091502,0.));
#161918=CARTESIAN_POINT('Ctrl Pts',(21.2310059409265,70.5746105091502,12.));
#161919=CARTESIAN_POINT('Ctrl Pts',(21.2137349111208,70.5540835797283,0.));
#161920=CARTESIAN_POINT('Ctrl Pts',(21.2137349111208,70.5540835797283,12.));
#161921=CARTESIAN_POINT('Ctrl Pts',(21.1965062658298,70.5335687714429,0.));
#161922=CARTESIAN_POINT('Ctrl Pts',(21.1965062658298,70.5335687714429,12.));
#161923=CARTESIAN_POINT('Ctrl Pts',(21.1793200267846,70.5130661852955,0.));
#161924=CARTESIAN_POINT('Ctrl Pts',(21.1793200267846,70.5130661852955,12.));
#161925=CARTESIAN_POINT('Ctrl Pts',(21.1621762156897,70.4925759224216,0.));
#161926=CARTESIAN_POINT('Ctrl Pts',(21.1621762156897,70.4925759224216,12.));
#161927=CARTESIAN_POINT('Ctrl Pts',(21.1450748542336,70.4720980841939,0.));
#161928=CARTESIAN_POINT('Ctrl Pts',(21.1450748542336,70.4720980841939,12.));
#161929=CARTESIAN_POINT('Ctrl Pts',(21.1280159641002,70.4516327723346,0.));
#161930=CARTESIAN_POINT('Ctrl Pts',(21.1280159641002,70.4516327723346,12.));
#161931=CARTESIAN_POINT('Ctrl Pts',(21.1109995669747,70.4311800890402,0.));
#161932=CARTESIAN_POINT('Ctrl Pts',(21.1109995669747,70.4311800890402,12.));
#161933=CARTESIAN_POINT('Ctrl Pts',(21.0940256845472,70.4107401370389,0.));
#161934=CARTESIAN_POINT('Ctrl Pts',(21.0940256845472,70.4107401370389,12.));
#161935=CARTESIAN_POINT('Ctrl Pts',(21.0770943385141,70.3903130195265,0.));
#161936=CARTESIAN_POINT('Ctrl Pts',(21.0770943385141,70.3903130195265,12.));
#161937=CARTESIAN_POINT('Ctrl Pts',(21.0602055505748,70.3698988401281,0.));
#161938=CARTESIAN_POINT('Ctrl Pts',(21.0602055505748,70.3698988401281,12.));
#161939=CARTESIAN_POINT('Ctrl Pts',(21.0433593424266,70.3494977028498,0.));
#161940=CARTESIAN_POINT('Ctrl Pts',(21.0433593424266,70.3494977028498,12.));
#161941=CARTESIAN_POINT('Ctrl Pts',(21.0265557357548,70.3291097120302,0.));
#161942=CARTESIAN_POINT('Ctrl Pts',(21.0265557357548,70.3291097120302,12.));
#161943=CARTESIAN_POINT('Ctrl Pts',(21.0097947522218,70.3087349722973,0.));
#161944=CARTESIAN_POINT('Ctrl Pts',(21.0097947522218,70.3087349722973,12.));
#161945=CARTESIAN_POINT('Ctrl Pts',(20.9930764134776,70.2883735885984,0.));
#161946=CARTESIAN_POINT('Ctrl Pts',(20.9930764134776,70.2883735885984,12.));
#161947=CARTESIAN_POINT('Ctrl Pts',(20.9764007411652,70.2680256662224,0.));
#161948=CARTESIAN_POINT('Ctrl Pts',(20.9764007411652,70.2680256662224,12.));
#161949=CARTESIAN_POINT('Ctrl Pts',(20.9597677569228,70.2476913108244,0.));
#161950=CARTESIAN_POINT('Ctrl Pts',(20.9597677569228,70.2476913108244,12.));
#161951=CARTESIAN_POINT('Ctrl Pts',(20.9431774823831,70.2273706284472,0.));
#161952=CARTESIAN_POINT('Ctrl Pts',(20.9431774823831,70.2273706284472,12.));
#161953=CARTESIAN_POINT('Ctrl Pts',(20.9266299391684,70.2070637255458,0.));
#161954=CARTESIAN_POINT('Ctrl Pts',(20.9266299391684,70.2070637255458,12.));
#161955=CARTESIAN_POINT('Ctrl Pts',(20.9101251488943,70.1867707089854,0.));
#161956=CARTESIAN_POINT('Ctrl Pts',(20.9101251488943,70.1867707089854,12.));
#161957=CARTESIAN_POINT('Ctrl Pts',(20.8936631331748,70.1664916860358,0.));
#161958=CARTESIAN_POINT('Ctrl Pts',(20.8936631331748,70.1664916860358,12.));
#161959=CARTESIAN_POINT('Ctrl Pts',(20.8772439136206,70.1462267643647,0.));
#161960=CARTESIAN_POINT('Ctrl Pts',(20.8772439136206,70.1462267643647,12.));
#161961=CARTESIAN_POINT('Ctrl Pts',(20.8608675118378,70.1259760520309,0.));
#161962=CARTESIAN_POINT('Ctrl Pts',(20.8608675118378,70.1259760520309,12.));
#161963=CARTESIAN_POINT('Ctrl Pts',(20.8445339494187,70.1057396574747,0.));
#161964=CARTESIAN_POINT('Ctrl Pts',(20.8445339494187,70.1057396574747,12.));
#161965=CARTESIAN_POINT('Ctrl Pts',(20.8282432479428,70.0855176895191,0.));
#161966=CARTESIAN_POINT('Ctrl Pts',(20.8282432479428,70.0855176895191,12.));
#161967=CARTESIAN_POINT('Ctrl Pts',(20.8119954289848,70.0653102573803,0.));
#161968=CARTESIAN_POINT('Ctrl Pts',(20.8119954289848,70.0653102573803,12.));
#161969=CARTESIAN_POINT('Ctrl Pts',(20.7957905141156,70.0451174706741,0.));
#161970=CARTESIAN_POINT('Ctrl Pts',(20.7957905141156,70.0451174706741,12.));
#161971=CARTESIAN_POINT('Ctrl Pts',(20.7796285249022,70.024939439422,0.));
#161972=CARTESIAN_POINT('Ctrl Pts',(20.7796285249022,70.024939439422,12.));
#161973=CARTESIAN_POINT('Ctrl Pts',(20.7635094829015,70.0047762740568,0.));
#161974=CARTESIAN_POINT('Ctrl Pts',(20.7635094829015,70.0047762740568,12.));
#161975=CARTESIAN_POINT('Ctrl Pts',(20.7474334096581,69.9846280854257,0.));
#161976=CARTESIAN_POINT('Ctrl Pts',(20.7474334096581,69.9846280854257,12.));
#161977=CARTESIAN_POINT('Ctrl Pts',(20.7314003267119,69.9644949847934,0.));
#161978=CARTESIAN_POINT('Ctrl Pts',(20.7314003267119,69.9644949847934,12.));
#161979=CARTESIAN_POINT('Ctrl Pts',(20.7154102555997,69.9443770838448,0.));
#161980=CARTESIAN_POINT('Ctrl Pts',(20.7154102555997,69.9443770838448,12.));
#161981=CARTESIAN_POINT('Ctrl Pts',(20.6994632178551,69.9242744946854,0.));
#161982=CARTESIAN_POINT('Ctrl Pts',(20.6994632178551,69.9242744946854,12.));
#161983=CARTESIAN_POINT('Ctrl Pts',(20.683559235003,69.904187329841,0.));
#161984=CARTESIAN_POINT('Ctrl Pts',(20.683559235003,69.904187329841,12.));
#161985=CARTESIAN_POINT('Ctrl Pts',(20.667698328554,69.8841157022568,0.));
#161986=CARTESIAN_POINT('Ctrl Pts',(20.667698328554,69.8841157022568,12.));
#161987=CARTESIAN_POINT('Ctrl Pts',(20.6518805200129,69.8640597253045,0.));
#161988=CARTESIAN_POINT('Ctrl Pts',(20.6518805200129,69.8640597253045,12.));
#161989=CARTESIAN_POINT('Ctrl Pts',(20.636105830881,69.8440195127866,0.));
#161990=CARTESIAN_POINT('Ctrl Pts',(20.636105830881,69.8440195127866,12.));
#161991=CARTESIAN_POINT('Ctrl Pts',(20.6203742826566,69.8239951789402,0.));
#161992=CARTESIAN_POINT('Ctrl Pts',(20.6203742826566,69.8239951789402,12.));
#161993=CARTESIAN_POINT('Ctrl Pts',(20.6046858968307,69.8039868384389,0.));
#161994=CARTESIAN_POINT('Ctrl Pts',(20.6046858968307,69.8039868384389,12.));
#161995=CARTESIAN_POINT('Ctrl Pts',(20.5890406948811,69.7839946063949,0.));
#161996=CARTESIAN_POINT('Ctrl Pts',(20.5890406948811,69.7839946063949,12.));
#161997=CARTESIAN_POINT('Ctrl Pts',(20.5734386982782,69.7640185983644,0.));
#161998=CARTESIAN_POINT('Ctrl Pts',(20.5734386982782,69.7640185983644,12.));
#161999=CARTESIAN_POINT('Ctrl Pts',(20.5578799284897,69.744058930351,0.));
#162000=CARTESIAN_POINT('Ctrl Pts',(20.5578799284897,69.744058930351,12.));
#162001=CARTESIAN_POINT('Ctrl Pts',(20.5423644069799,69.7241157188083,0.));
#162002=CARTESIAN_POINT('Ctrl Pts',(20.5423644069799,69.7241157188083,12.));
#162003=CARTESIAN_POINT('Ctrl Pts',(20.5268921552077,69.7041890806425,0.));
#162004=CARTESIAN_POINT('Ctrl Pts',(20.5268921552077,69.7041890806425,12.));
#162005=CARTESIAN_POINT('Ctrl Pts',(20.5114631946184,69.6842791332115,0.));
#162006=CARTESIAN_POINT('Ctrl Pts',(20.5114631946184,69.6842791332115,12.));
#162007=CARTESIAN_POINT('Ctrl Pts',(20.4960775466492,69.6643859943308,0.));
#162008=CARTESIAN_POINT('Ctrl Pts',(20.4960775466492,69.6643859943308,12.));
#162009=CARTESIAN_POINT('Ctrl Pts',(20.4807352327339,69.6445097822792,0.));
#162010=CARTESIAN_POINT('Ctrl Pts',(20.4807352327339,69.6445097822792,12.));
#162011=CARTESIAN_POINT('Ctrl Pts',(20.4654362743037,69.6246506158013,0.));
#162012=CARTESIAN_POINT('Ctrl Pts',(20.4654362743037,69.6246506158013,12.));
#162013=CARTESIAN_POINT('Ctrl Pts',(20.4501806927851,69.6048086141113,0.));
#162014=CARTESIAN_POINT('Ctrl Pts',(20.4501806927851,69.6048086141113,12.));
#162015=CARTESIAN_POINT('Ctrl Pts',(20.4349685095923,69.5849838968928,0.));
#162016=CARTESIAN_POINT('Ctrl Pts',(20.4349685095923,69.5849838968928,12.));
#162017=CARTESIAN_POINT('Ctrl Pts',(20.41979974613,69.5651765843033,0.));
#162018=CARTESIAN_POINT('Ctrl Pts',(20.41979974613,69.5651765843033,12.));
#162019=CARTESIAN_POINT('Ctrl Pts',(20.4046744237999,69.5453867969804,0.));
#162020=CARTESIAN_POINT('Ctrl Pts',(20.4046744237999,69.5453867969804,12.));
#162021=CARTESIAN_POINT('Ctrl Pts',(20.3895925640005,69.5256146560441,0.));
#162022=CARTESIAN_POINT('Ctrl Pts',(20.3895925640005,69.5256146560441,12.));
#162023=CARTESIAN_POINT('Ctrl Pts',(20.3745541881268,69.5058602831008,0.));
#162024=CARTESIAN_POINT('Ctrl Pts',(20.3745541881268,69.5058602831008,12.));
#162025=CARTESIAN_POINT('Ctrl Pts',(20.3595593175622,69.4861238002441,0.));
#162026=CARTESIAN_POINT('Ctrl Pts',(20.3595593175622,69.4861238002441,12.));
#162027=CARTESIAN_POINT('Ctrl Pts',(20.3446079736802,69.4664053300587,0.));
#162028=CARTESIAN_POINT('Ctrl Pts',(20.3446079736802,69.4664053300587,12.));
#162029=CARTESIAN_POINT('Ctrl Pts',(20.3297001778507,69.4467049956262,0.));
#162030=CARTESIAN_POINT('Ctrl Pts',(20.3297001778507,69.4467049956262,12.));
#162031=CARTESIAN_POINT('Ctrl Pts',(20.3148359514415,69.4270229205297,0.));
#162032=CARTESIAN_POINT('Ctrl Pts',(20.3148359514415,69.4270229205297,12.));
#162033=CARTESIAN_POINT('Ctrl Pts',(20.3000153158166,69.407359228856,0.));
#162034=CARTESIAN_POINT('Ctrl Pts',(20.3000153158166,69.407359228856,12.));
#162035=CARTESIAN_POINT('Ctrl Pts',(20.2852382923299,69.3877140451975,0.));
#162036=CARTESIAN_POINT('Ctrl Pts',(20.2852382923299,69.3877140451975,12.));
#162037=CARTESIAN_POINT('Ctrl Pts',(20.2705049023241,69.368087494655,0.));
#162038=CARTESIAN_POINT('Ctrl Pts',(20.2705049023241,69.368087494655,12.));
#162039=CARTESIAN_POINT('Ctrl Pts',(20.2558151671391,69.3484797028458,0.));
#162040=CARTESIAN_POINT('Ctrl Pts',(20.2558151671391,69.3484797028458,12.));
#162041=CARTESIAN_POINT('Ctrl Pts',(20.2411691081123,69.3288907959067,0.));
#162042=CARTESIAN_POINT('Ctrl Pts',(20.2411691081123,69.3288907959067,12.));
#162043=CARTESIAN_POINT('Ctrl Pts',(20.2265667465784,69.3093209004984,0.));
#162044=CARTESIAN_POINT('Ctrl Pts',(20.2265667465784,69.3093209004984,12.));
#162045=CARTESIAN_POINT('Ctrl Pts',(20.212008103862,69.2897701438059,0.));
#162046=CARTESIAN_POINT('Ctrl Pts',(20.212008103862,69.2897701438059,12.));
#162047=CARTESIAN_POINT('Ctrl Pts',(20.1974932012773,69.2702386535422,0.));
#162048=CARTESIAN_POINT('Ctrl Pts',(20.1974932012773,69.2702386535422,12.));
#162049=CARTESIAN_POINT('Ctrl Pts',(20.1830220601348,69.2507265579554,0.));
#162050=CARTESIAN_POINT('Ctrl Pts',(20.1830220601348,69.2507265579554,12.));
#162051=CARTESIAN_POINT('Ctrl Pts',(20.1685947017433,69.2312339858335,0.));
#162052=CARTESIAN_POINT('Ctrl Pts',(20.1685947017433,69.2312339858335,12.));
#162053=CARTESIAN_POINT('Ctrl Pts',(20.1542111474087,69.2117610665076,0.));
#162054=CARTESIAN_POINT('Ctrl Pts',(20.1542111474087,69.2117610665076,12.));
#162055=CARTESIAN_POINT('Ctrl Pts',(20.1398714184279,69.1923079298538,0.));
#162056=CARTESIAN_POINT('Ctrl Pts',(20.1398714184279,69.1923079298538,12.));
#162057=CARTESIAN_POINT('Ctrl Pts',(20.1255755360872,69.1728747062963,0.));
#162058=CARTESIAN_POINT('Ctrl Pts',(20.1255755360872,69.1728747062963,12.));
#162059=CARTESIAN_POINT('Ctrl Pts',(20.1113235216694,69.1534615268153,0.));
#162060=CARTESIAN_POINT('Ctrl Pts',(20.1113235216694,69.1534615268153,12.));
#162061=CARTESIAN_POINT('Ctrl Pts',(20.0971153964557,69.1340685229514,0.));
#162062=CARTESIAN_POINT('Ctrl Pts',(20.0971153964557,69.1340685229514,12.));
#162063=CARTESIAN_POINT('Ctrl Pts',(20.0829511817251,69.1146958268104,0.));
#162064=CARTESIAN_POINT('Ctrl Pts',(20.0829511817251,69.1146958268104,12.));
#162065=CARTESIAN_POINT('Ctrl Pts',(20.068830898748,69.095343571064,0.));
#162066=CARTESIAN_POINT('Ctrl Pts',(20.068830898748,69.095343571064,12.));
#162067=CARTESIAN_POINT('Ctrl Pts',(20.0547545687842,69.0760118889535,0.));
#162068=CARTESIAN_POINT('Ctrl Pts',(20.0547545687842,69.0760118889535,12.));
#162069=CARTESIAN_POINT('Ctrl Pts',(20.0407222130905,69.0567009142978,0.));
#162070=CARTESIAN_POINT('Ctrl Pts',(20.0407222130905,69.0567009142978,12.));
#162071=CARTESIAN_POINT('Ctrl Pts',(20.0267338529223,69.0374107814984,0.));
#162072=CARTESIAN_POINT('Ctrl Pts',(20.0267338529223,69.0374107814984,12.));
#162073=CARTESIAN_POINT('Ctrl Pts',(20.0127895095326,69.0181416255431,0.));
#162074=CARTESIAN_POINT('Ctrl Pts',(20.0127895095326,69.0181416255431,12.));
#162075=CARTESIAN_POINT('Ctrl Pts',(19.9988892041666,68.9988935820084,0.));
#162076=CARTESIAN_POINT('Ctrl Pts',(19.9988892041666,68.9988935820084,12.));
#162077=CARTESIAN_POINT('Ctrl Pts',(19.9850329580591,68.9796667870638,0.));
#162078=CARTESIAN_POINT('Ctrl Pts',(19.9850329580591,68.9796667870638,12.));
#162079=CARTESIAN_POINT('Ctrl Pts',(19.9712207924428,68.9604613774802,0.));
#162080=CARTESIAN_POINT('Ctrl Pts',(19.9712207924428,68.9604613774802,12.));
#162081=CARTESIAN_POINT('Ctrl Pts',(19.9574527285488,68.9412774906333,0.));
#162082=CARTESIAN_POINT('Ctrl Pts',(19.9574527285488,68.9412774906333,12.));
#162083=CARTESIAN_POINT('Ctrl Pts',(19.9437287876066,68.9221152645095,0.));
#162084=CARTESIAN_POINT('Ctrl Pts',(19.9437287876066,68.9221152645095,12.));
#162085=CARTESIAN_POINT('Ctrl Pts',(19.9300489908374,68.9029748377067,0.));
#162086=CARTESIAN_POINT('Ctrl Pts',(19.9300489908374,68.9029748377067,12.));
#162087=CARTESIAN_POINT('Ctrl Pts',(19.9164133594525,68.8838563494393,0.));
#162088=CARTESIAN_POINT('Ctrl Pts',(19.9164133594525,68.8838563494393,12.));
#162089=CARTESIAN_POINT('Ctrl Pts',(19.9028219146618,68.8647599395469,0.));
#162090=CARTESIAN_POINT('Ctrl Pts',(19.9028219146618,68.8647599395469,12.));
#162091=CARTESIAN_POINT('Ctrl Pts',(19.8892746776739,68.8456857485002,0.));
#162092=CARTESIAN_POINT('Ctrl Pts',(19.8892746776739,68.8456857485002,12.));
#162093=CARTESIAN_POINT('Ctrl Pts',(19.8757716696965,68.8266339174056,0.));
#162094=CARTESIAN_POINT('Ctrl Pts',(19.8757716696965,68.8266339174056,12.));
#162095=CARTESIAN_POINT('Ctrl Pts',(19.8623129119293,68.8076045880065,0.));
#162096=CARTESIAN_POINT('Ctrl Pts',(19.8623129119293,68.8076045880065,12.));
#162097=CARTESIAN_POINT('Ctrl Pts',(19.8488984255627,68.7885979026879,0.));
#162098=CARTESIAN_POINT('Ctrl Pts',(19.8488984255627,68.7885979026879,12.));
#162099=CARTESIAN_POINT('Ctrl Pts',(19.8355282317858,68.7696140044851,0.));
#162100=CARTESIAN_POINT('Ctrl Pts',(19.8355282317858,68.7696140044851,12.));
#162101=CARTESIAN_POINT('Ctrl Pts',(19.822202351787,68.7506530370904,0.));
#162102=CARTESIAN_POINT('Ctrl Pts',(19.822202351787,68.7506530370904,12.));
#162103=CARTESIAN_POINT('Ctrl Pts',(19.8089208067537,68.7317151448573,0.));
#162104=CARTESIAN_POINT('Ctrl Pts',(19.8089208067537,68.7317151448573,12.));
#162105=CARTESIAN_POINT('Ctrl Pts',(19.7956836178651,68.7128004728034,0.));
#162106=CARTESIAN_POINT('Ctrl Pts',(19.7956836178651,68.7128004728034,12.));
#162107=CARTESIAN_POINT('Ctrl Pts',(19.7824908062924,68.693909166615,0.));
#162108=CARTESIAN_POINT('Ctrl Pts',(19.7824908062924,68.693909166615,12.));
#162109=CARTESIAN_POINT('Ctrl Pts',(19.7693423932066,68.6750413726575,0.));
#162110=CARTESIAN_POINT('Ctrl Pts',(19.7693423932066,68.6750413726575,12.));
#162111=CARTESIAN_POINT('Ctrl Pts',(19.7562383997783,68.65619723798,0.));
#162112=CARTESIAN_POINT('Ctrl Pts',(19.7562383997783,68.65619723798,12.));
#162113=CARTESIAN_POINT('Ctrl Pts',(19.7431788471772,68.6373769103211,0.));
#162114=CARTESIAN_POINT('Ctrl Pts',(19.7431788471772,68.6373769103211,12.));
#162115=CARTESIAN_POINT('Ctrl Pts',(19.7301637565645,68.6185805381102,0.));
#162116=CARTESIAN_POINT('Ctrl Pts',(19.7301637565645,68.6185805381102,12.));
#162117=CARTESIAN_POINT('Ctrl Pts',(19.717193149095,68.5998082704741,0.));
#162118=CARTESIAN_POINT('Ctrl Pts',(19.717193149095,68.5998082704741,12.));
#162119=CARTESIAN_POINT('Ctrl Pts',(19.7042670459233,68.5810602572474,0.));
#162120=CARTESIAN_POINT('Ctrl Pts',(19.7042670459233,68.5810602572474,12.));
#162121=CARTESIAN_POINT('Ctrl Pts',(19.6913854682046,68.5623366489776,0.));
#162122=CARTESIAN_POINT('Ctrl Pts',(19.6913854682046,68.5623366489776,12.));
#162123=CARTESIAN_POINT('Ctrl Pts',(19.6785484370929,68.543637596932,0.));
#162124=CARTESIAN_POINT('Ctrl Pts',(19.6785484370929,68.543637596932,12.));
#162125=CARTESIAN_POINT('Ctrl Pts',(19.665755973734,68.5249632530994,0.));
#162126=CARTESIAN_POINT('Ctrl Pts',(19.665755973734,68.5249632530994,12.));
#162127=CARTESIAN_POINT('Ctrl Pts',(19.6530080992689,68.5063137701986,0.));
#162128=CARTESIAN_POINT('Ctrl Pts',(19.6530080992689,68.5063137701986,12.));
#162129=CARTESIAN_POINT('Ctrl Pts',(19.6403048348396,68.4876893016863,0.));
#162130=CARTESIAN_POINT('Ctrl Pts',(19.6403048348396,68.4876893016863,12.));
#162131=CARTESIAN_POINT('Ctrl Pts',(19.6276462015888,68.4690900017631,0.));
#162132=CARTESIAN_POINT('Ctrl Pts',(19.6276462015888,68.4690900017631,12.));
#162133=CARTESIAN_POINT('Ctrl Pts',(19.6150322206577,68.4505160253777,0.));
#162134=CARTESIAN_POINT('Ctrl Pts',(19.6150322206577,68.4505160253777,12.));
#162135=CARTESIAN_POINT('Ctrl Pts',(19.6024629131785,68.4319675282273,0.));
#162136=CARTESIAN_POINT('Ctrl Pts',(19.6024629131785,68.4319675282273,12.));
#162137=CARTESIAN_POINT('Ctrl Pts',(19.5899383002803,68.4134446667695,0.));
#162138=CARTESIAN_POINT('Ctrl Pts',(19.5899383002803,68.4134446667695,12.));
#162139=CARTESIAN_POINT('Ctrl Pts',(19.5774584030938,68.3949475982334,0.));
#162140=CARTESIAN_POINT('Ctrl Pts',(19.5774584030938,68.3949475982334,12.));
#162141=CARTESIAN_POINT('Ctrl Pts',(19.5650232427516,68.3764764806287,0.));
#162142=CARTESIAN_POINT('Ctrl Pts',(19.5650232427516,68.3764764806287,12.));
#162143=CARTESIAN_POINT('Ctrl Pts',(19.5526328403851,68.3580314727522,0.));
#162144=CARTESIAN_POINT('Ctrl Pts',(19.5526328403851,68.3580314727522,12.));
#162145=CARTESIAN_POINT('Ctrl Pts',(19.540287217119,68.3396127341937,0.));
#162146=CARTESIAN_POINT('Ctrl Pts',(19.540287217119,68.3396127341937,12.));
#162147=CARTESIAN_POINT('Ctrl Pts',(19.5279863940772,68.3212204253416,0.));
#162148=CARTESIAN_POINT('Ctrl Pts',(19.5279863940772,68.3212204253416,12.));
#162149=CARTESIAN_POINT('Ctrl Pts',(19.5157303923855,68.3028547073862,0.));
#162150=CARTESIAN_POINT('Ctrl Pts',(19.5157303923855,68.3028547073862,12.));
#162151=CARTESIAN_POINT('Ctrl Pts',(19.5035192331706,68.2845157423234,0.));
#162152=CARTESIAN_POINT('Ctrl Pts',(19.5035192331706,68.2845157423234,12.));
#162153=CARTESIAN_POINT('Ctrl Pts',(19.4913529375545,68.2662036929531,0.));
#162154=CARTESIAN_POINT('Ctrl Pts',(19.4913529375545,68.2662036929531,12.));
#162155=CARTESIAN_POINT('Ctrl Pts',(19.4792315266505,68.2479187228815,0.));
#162156=CARTESIAN_POINT('Ctrl Pts',(19.4792315266505,68.2479187228815,12.));
#162157=CARTESIAN_POINT('Ctrl Pts',(19.4671550215724,68.2296609965461,0.));
#162158=CARTESIAN_POINT('Ctrl Pts',(19.4671550215724,68.2296609965461,12.));
#162159=CARTESIAN_POINT('Ctrl Pts',(19.4551234434383,68.2114306792366,0.));
#162160=CARTESIAN_POINT('Ctrl Pts',(19.4551234434383,68.2114306792366,12.));
#162161=CARTESIAN_POINT('Ctrl Pts',(19.4431368133718,68.1932279371121,0.));
#162162=CARTESIAN_POINT('Ctrl Pts',(19.4431368133718,68.1932279371121,12.));
#162163=CARTESIAN_POINT('Ctrl Pts',(19.4311951524977,68.1750529372211,0.));
#162164=CARTESIAN_POINT('Ctrl Pts',(19.4311951524977,68.1750529372211,12.));
#162165=CARTESIAN_POINT('Ctrl Pts',(19.419298481941,68.1569058475026,0.));
#162166=CARTESIAN_POINT('Ctrl Pts',(19.419298481941,68.1569058475026,12.));
#162167=CARTESIAN_POINT('Ctrl Pts',(19.4074468228293,68.1387868367668,0.));
#162168=CARTESIAN_POINT('Ctrl Pts',(19.4074468228293,68.1387868367668,12.));
#162169=CARTESIAN_POINT('Ctrl Pts',(19.3956401962893,68.1206960746763,0.));
#162170=CARTESIAN_POINT('Ctrl Pts',(19.3956401962893,68.1206960746763,12.));
#162171=CARTESIAN_POINT('Ctrl Pts',(19.3838786234425,68.1026337317298,0.));
#162172=CARTESIAN_POINT('Ctrl Pts',(19.3838786234425,68.1026337317298,12.));
#162173=CARTESIAN_POINT('Ctrl Pts',(19.372162125392,68.0845999792274,0.));
#162174=CARTESIAN_POINT('Ctrl Pts',(19.372162125392,68.0845999792274,12.));
#162175=CARTESIAN_POINT('Ctrl Pts',(19.3604907232322,68.0665949893222,0.));
#162176=CARTESIAN_POINT('Ctrl Pts',(19.3604907232322,68.0665949893222,12.));
#162177=CARTESIAN_POINT('Ctrl Pts',(19.3488644380646,68.0486189351027,0.));
#162178=CARTESIAN_POINT('Ctrl Pts',(19.3488644380646,68.0486189351027,12.));
#162179=CARTESIAN_POINT('Ctrl Pts',(19.3372832910076,68.0306719906636,0.));
#162180=CARTESIAN_POINT('Ctrl Pts',(19.3372832910076,68.0306719906636,12.));
#162181=CARTESIAN_POINT('Ctrl Pts',(19.3257473032031,68.0127543311761,0.));
#162182=CARTESIAN_POINT('Ctrl Pts',(19.3257473032031,68.0127543311761,12.));
#162183=CARTESIAN_POINT('Ctrl Pts',(19.3142564958195,67.9948661329592,0.));
#162184=CARTESIAN_POINT('Ctrl Pts',(19.3142564958195,67.9948661329592,12.));
#162185=CARTESIAN_POINT('Ctrl Pts',(19.3028108900373,67.977007573346,0.));
#162186=CARTESIAN_POINT('Ctrl Pts',(19.3028108900373,67.977007573346,12.));
#162187=CARTESIAN_POINT('Ctrl Pts',(19.2914105070282,67.959178830538,0.));
#162188=CARTESIAN_POINT('Ctrl Pts',(19.2914105070282,67.959178830538,12.));
#162189=CARTESIAN_POINT('Ctrl Pts',(19.2800553679362,67.9413800834798,0.));
#162190=CARTESIAN_POINT('Ctrl Pts',(19.2800553679362,67.9413800834798,12.));
#162191=CARTESIAN_POINT('Ctrl Pts',(19.2687454938448,67.9236115116781,0.));
#162192=CARTESIAN_POINT('Ctrl Pts',(19.2687454938448,67.9236115116781,12.));
#162193=CARTESIAN_POINT('Ctrl Pts',(19.2574809057705,67.9058732951822,0.));
#162194=CARTESIAN_POINT('Ctrl Pts',(19.2574809057705,67.9058732951822,12.));
#162195=CARTESIAN_POINT('Ctrl Pts',(19.2462616247287,67.8881656149983,0.));
#162196=CARTESIAN_POINT('Ctrl Pts',(19.2462616247287,67.8881656149983,12.));
#162197=CARTESIAN_POINT('Ctrl Pts',(19.2350876717877,67.8704886534555,0.));
#162198=CARTESIAN_POINT('Ctrl Pts',(19.2350876717877,67.8704886534555,12.));
#162199=CARTESIAN_POINT('Ctrl Pts',(19.2239590681129,67.852842594517,0.));
#162200=CARTESIAN_POINT('Ctrl Pts',(19.2239590681129,67.852842594517,12.));
#162201=CARTESIAN_POINT('Ctrl Pts',(19.2128758350336,67.8352276242856,0.));
#162202=CARTESIAN_POINT('Ctrl Pts',(19.2128758350336,67.8352276242856,12.));
#162203=CARTESIAN_POINT('Ctrl Pts',(19.2018379939918,67.817643930658,0.));
#162204=CARTESIAN_POINT('Ctrl Pts',(19.2018379939918,67.817643930658,12.));
#162205=CARTESIAN_POINT('Ctrl Pts',(19.1908455664089,67.8000917023896,0.));
#162206=CARTESIAN_POINT('Ctrl Pts',(19.1908455664089,67.8000917023896,12.));
#162207=CARTESIAN_POINT('Ctrl Pts',(19.1798985735687,67.7825711283092,0.));
#162208=CARTESIAN_POINT('Ctrl Pts',(19.1798985735687,67.7825711283092,12.));
#162209=CARTESIAN_POINT('Ctrl Pts',(19.1689970364958,67.7650823965156,0.));
#162210=CARTESIAN_POINT('Ctrl Pts',(19.1689970364958,67.7650823965156,12.));
#162211=CARTESIAN_POINT('Ctrl Pts',(19.1581409758111,67.7476256934493,0.));
#162212=CARTESIAN_POINT('Ctrl Pts',(19.1581409758111,67.7476256934493,12.));
#162213=CARTESIAN_POINT('Ctrl Pts',(19.1473304119968,67.730201205663,0.));
#162214=CARTESIAN_POINT('Ctrl Pts',(19.1473304119968,67.730201205663,12.));
#162215=CARTESIAN_POINT('Ctrl Pts',(19.1365653657097,67.7128091219372,0.));
#162216=CARTESIAN_POINT('Ctrl Pts',(19.1365653657097,67.7128091219372,12.));
#162217=CARTESIAN_POINT('Ctrl Pts',(19.1258458580343,67.6954496350053,0.));
#162218=CARTESIAN_POINT('Ctrl Pts',(19.1258458580343,67.6954496350053,12.));
#162219=CARTESIAN_POINT('Ctrl Pts',(19.115171910845,67.6781229440535,0.));
#162220=CARTESIAN_POINT('Ctrl Pts',(19.115171910845,67.6781229440535,12.));
#162221=CARTESIAN_POINT('Ctrl Pts',(19.1045435468344,67.6608292549412,0.));
#162222=CARTESIAN_POINT('Ctrl Pts',(19.1045435468344,67.6608292549412,12.));
#162223=CARTESIAN_POINT('Ctrl Pts',(19.0939607887491,67.6435687749803,0.));
#162224=CARTESIAN_POINT('Ctrl Pts',(19.0939607887491,67.6435687749803,12.));
#162225=CARTESIAN_POINT('Ctrl Pts',(19.0834236587115,67.6263417083414,0.));
#162226=CARTESIAN_POINT('Ctrl Pts',(19.0834236587115,67.6263417083414,12.));
#162227=CARTESIAN_POINT('Ctrl Pts',(19.0729321776286,67.6091482520558,0.));
#162228=CARTESIAN_POINT('Ctrl Pts',(19.0729321776286,67.6091482520558,12.));
#162229=CARTESIAN_POINT('Ctrl Pts',(19.0624863642425,67.5919885896278,0.));
#162230=CARTESIAN_POINT('Ctrl Pts',(19.0624863642425,67.5919885896278,12.));
#162231=CARTESIAN_POINT('Ctrl Pts',(19.0520862360413,67.5748628972035,0.));
#162232=CARTESIAN_POINT('Ctrl Pts',(19.0520862360413,67.5748628972035,12.));
#162233=CARTESIAN_POINT('Ctrl Pts',(19.0417318110721,67.5577713558248,0.));
#162234=CARTESIAN_POINT('Ctrl Pts',(19.0417318110721,67.5577713558248,12.));
#162235=CARTESIAN_POINT('Ctrl Pts',(19.0314231093923,67.5407141612881,0.));
#162236=CARTESIAN_POINT('Ctrl Pts',(19.0314231093923,67.5407141612881,12.));
#162237=CARTESIAN_POINT('Ctrl Pts',(19.0211601548222,67.5236915360253,0.));
#162238=CARTESIAN_POINT('Ctrl Pts',(19.0211601548222,67.5236915360253,12.));
#162239=CARTESIAN_POINT('Ctrl Pts',(19.0109429761274,67.5067037372177,0.));
#162240=CARTESIAN_POINT('Ctrl Pts',(19.0109429761274,67.5067037372177,12.));
#162241=CARTESIAN_POINT('Ctrl Pts',(19.0007716032784,67.4897510316692,0.));
#162242=CARTESIAN_POINT('Ctrl Pts',(19.0007716032784,67.4897510316692,12.));
#162243=CARTESIAN_POINT('Ctrl Pts',(18.9906460638607,67.4728336719559,0.));
#162244=CARTESIAN_POINT('Ctrl Pts',(18.9906460638607,67.4728336719559,12.));
#162245=CARTESIAN_POINT('Ctrl Pts',(18.9805663798466,67.4559518744714,0.));
#162246=CARTESIAN_POINT('Ctrl Pts',(18.9805663798466,67.4559518744714,12.));
#162247=CARTESIAN_POINT('Ctrl Pts',(18.9705325631772,67.4391057908687,0.));
#162248=CARTESIAN_POINT('Ctrl Pts',(18.9705325631772,67.4391057908687,12.));
#162249=CARTESIAN_POINT('Ctrl Pts',(18.9605446161078,67.4222955062385,0.));
#162250=CARTESIAN_POINT('Ctrl Pts',(18.9605446161078,67.4222955062385,12.));
#162251=CARTESIAN_POINT('Ctrl Pts',(18.9525909518002,67.4088759498287,0.));
#162252=CARTESIAN_POINT('Ctrl Pts',(18.9525909518002,67.4088759498287,12.));
#162253=CARTESIAN_POINT('Ctrl Pts',(18.9466463414354,67.398827414689,0.));
#162254=CARTESIAN_POINT('Ctrl Pts',(18.9466463414354,67.398827414689,12.));
#162255=CARTESIAN_POINT('Ctrl Pts',(18.942692439874,67.3921355608417,0.));
#162256=CARTESIAN_POINT('Ctrl Pts',(18.942692439874,67.3921355608417,12.));
#162257=CARTESIAN_POINT('Ctrl Pts',(18.9407177820969,67.3887914263119,0.));
#162258=CARTESIAN_POINT('Ctrl Pts',(18.9407177820969,67.3887914263119,12.));
#162259=CARTESIAN_POINT('',(18.9407177820969,67.3887914263119,12.));
#162260=CARTESIAN_POINT('Ctrl Pts',(18.9407177820969,67.3887914263119,12.));
#162261=CARTESIAN_POINT('Ctrl Pts',(18.942692439874,67.3921355608417,12.));
#162262=CARTESIAN_POINT('Ctrl Pts',(18.9466463414354,67.398827414689,12.));
#162263=CARTESIAN_POINT('Ctrl Pts',(18.9525909518002,67.4088759498287,12.));
#162264=CARTESIAN_POINT('Ctrl Pts',(18.9605446161078,67.4222955062385,12.));
#162265=CARTESIAN_POINT('Ctrl Pts',(18.9705325631772,67.4391057908687,12.));
#162266=CARTESIAN_POINT('Ctrl Pts',(18.9805663798466,67.4559518744714,12.));
#162267=CARTESIAN_POINT('Ctrl Pts',(18.9906460638607,67.4728336719559,12.));
#162268=CARTESIAN_POINT('Ctrl Pts',(19.0007716032784,67.4897510316692,12.));
#162269=CARTESIAN_POINT('Ctrl Pts',(19.0109429761274,67.5067037372177,12.));
#162270=CARTESIAN_POINT('Ctrl Pts',(19.0211601548222,67.5236915360253,12.));
#162271=CARTESIAN_POINT('Ctrl Pts',(19.0314231093923,67.5407141612881,12.));
#162272=CARTESIAN_POINT('Ctrl Pts',(19.0417318110721,67.5577713558248,12.));
#162273=CARTESIAN_POINT('Ctrl Pts',(19.0520862360413,67.5748628972035,12.));
#162274=CARTESIAN_POINT('Ctrl Pts',(19.0624863642425,67.5919885896278,12.));
#162275=CARTESIAN_POINT('Ctrl Pts',(19.0729321776286,67.6091482520558,12.));
#162276=CARTESIAN_POINT('Ctrl Pts',(19.0834236587115,67.6263417083414,12.));
#162277=CARTESIAN_POINT('Ctrl Pts',(19.0939607887491,67.6435687749803,12.));
#162278=CARTESIAN_POINT('Ctrl Pts',(19.1045435468344,67.6608292549412,12.));
#162279=CARTESIAN_POINT('Ctrl Pts',(19.115171910845,67.6781229440535,12.));
#162280=CARTESIAN_POINT('Ctrl Pts',(19.1258458580343,67.6954496350053,12.));
#162281=CARTESIAN_POINT('Ctrl Pts',(19.1365653657097,67.7128091219372,12.));
#162282=CARTESIAN_POINT('Ctrl Pts',(19.1473304119968,67.730201205663,12.));
#162283=CARTESIAN_POINT('Ctrl Pts',(19.1581409758111,67.7476256934493,12.));
#162284=CARTESIAN_POINT('Ctrl Pts',(19.1689970364958,67.7650823965156,12.));
#162285=CARTESIAN_POINT('Ctrl Pts',(19.1798985735687,67.7825711283092,12.));
#162286=CARTESIAN_POINT('Ctrl Pts',(19.1908455664089,67.8000917023896,12.));
#162287=CARTESIAN_POINT('Ctrl Pts',(19.2018379939918,67.817643930658,12.));
#162288=CARTESIAN_POINT('Ctrl Pts',(19.2128758350336,67.8352276242856,12.));
#162289=CARTESIAN_POINT('Ctrl Pts',(19.2239590681129,67.852842594517,12.));
#162290=CARTESIAN_POINT('Ctrl Pts',(19.2350876717877,67.8704886534555,12.));
#162291=CARTESIAN_POINT('Ctrl Pts',(19.2462616247287,67.8881656149983,12.));
#162292=CARTESIAN_POINT('Ctrl Pts',(19.2574809057705,67.9058732951822,12.));
#162293=CARTESIAN_POINT('Ctrl Pts',(19.2687454938448,67.9236115116781,12.));
#162294=CARTESIAN_POINT('Ctrl Pts',(19.2800553679362,67.9413800834798,12.));
#162295=CARTESIAN_POINT('Ctrl Pts',(19.2914105070282,67.959178830538,12.));
#162296=CARTESIAN_POINT('Ctrl Pts',(19.3028108900373,67.977007573346,12.));
#162297=CARTESIAN_POINT('Ctrl Pts',(19.3142564958195,67.9948661329592,12.));
#162298=CARTESIAN_POINT('Ctrl Pts',(19.3257473032031,68.0127543311761,12.));
#162299=CARTESIAN_POINT('Ctrl Pts',(19.3372832910076,68.0306719906636,12.));
#162300=CARTESIAN_POINT('Ctrl Pts',(19.3488644380646,68.0486189351027,12.));
#162301=CARTESIAN_POINT('Ctrl Pts',(19.3604907232322,68.0665949893222,12.));
#162302=CARTESIAN_POINT('Ctrl Pts',(19.372162125392,68.0845999792274,12.));
#162303=CARTESIAN_POINT('Ctrl Pts',(19.3838786234425,68.1026337317298,12.));
#162304=CARTESIAN_POINT('Ctrl Pts',(19.3956401962893,68.1206960746763,12.));
#162305=CARTESIAN_POINT('Ctrl Pts',(19.4074468228293,68.1387868367668,12.));
#162306=CARTESIAN_POINT('Ctrl Pts',(19.419298481941,68.1569058475026,12.));
#162307=CARTESIAN_POINT('Ctrl Pts',(19.4311951524977,68.1750529372211,12.));
#162308=CARTESIAN_POINT('Ctrl Pts',(19.4431368133718,68.1932279371121,12.));
#162309=CARTESIAN_POINT('Ctrl Pts',(19.4551234434383,68.2114306792366,12.));
#162310=CARTESIAN_POINT('Ctrl Pts',(19.4671550215724,68.2296609965461,12.));
#162311=CARTESIAN_POINT('Ctrl Pts',(19.4792315266505,68.2479187228815,12.));
#162312=CARTESIAN_POINT('Ctrl Pts',(19.4913529375545,68.2662036929531,12.));
#162313=CARTESIAN_POINT('Ctrl Pts',(19.5035192331706,68.2845157423234,12.));
#162314=CARTESIAN_POINT('Ctrl Pts',(19.5157303923855,68.3028547073862,12.));
#162315=CARTESIAN_POINT('Ctrl Pts',(19.5279863940772,68.3212204253416,12.));
#162316=CARTESIAN_POINT('Ctrl Pts',(19.540287217119,68.3396127341937,12.));
#162317=CARTESIAN_POINT('Ctrl Pts',(19.5526328403851,68.3580314727522,12.));
#162318=CARTESIAN_POINT('Ctrl Pts',(19.5650232427516,68.3764764806287,12.));
#162319=CARTESIAN_POINT('Ctrl Pts',(19.5774584030938,68.3949475982334,12.));
#162320=CARTESIAN_POINT('Ctrl Pts',(19.5899383002803,68.4134446667695,12.));
#162321=CARTESIAN_POINT('Ctrl Pts',(19.6024629131785,68.4319675282273,12.));
#162322=CARTESIAN_POINT('Ctrl Pts',(19.6150322206577,68.4505160253777,12.));
#162323=CARTESIAN_POINT('Ctrl Pts',(19.6276462015888,68.4690900017631,12.));
#162324=CARTESIAN_POINT('Ctrl Pts',(19.6403048348396,68.4876893016863,12.));
#162325=CARTESIAN_POINT('Ctrl Pts',(19.6530080992689,68.5063137701986,12.));
#162326=CARTESIAN_POINT('Ctrl Pts',(19.665755973734,68.5249632530994,12.));
#162327=CARTESIAN_POINT('Ctrl Pts',(19.6785484370929,68.543637596932,12.));
#162328=CARTESIAN_POINT('Ctrl Pts',(19.6913854682046,68.5623366489776,12.));
#162329=CARTESIAN_POINT('Ctrl Pts',(19.7042670459233,68.5810602572474,12.));
#162330=CARTESIAN_POINT('Ctrl Pts',(19.717193149095,68.5998082704741,12.));
#162331=CARTESIAN_POINT('Ctrl Pts',(19.7301637565645,68.6185805381102,12.));
#162332=CARTESIAN_POINT('Ctrl Pts',(19.7431788471772,68.6373769103211,12.));
#162333=CARTESIAN_POINT('Ctrl Pts',(19.7562383997783,68.65619723798,12.));
#162334=CARTESIAN_POINT('Ctrl Pts',(19.7693423932066,68.6750413726575,12.));
#162335=CARTESIAN_POINT('Ctrl Pts',(19.7824908062924,68.693909166615,12.));
#162336=CARTESIAN_POINT('Ctrl Pts',(19.7956836178651,68.7128004728034,12.));
#162337=CARTESIAN_POINT('Ctrl Pts',(19.8089208067537,68.7317151448573,12.));
#162338=CARTESIAN_POINT('Ctrl Pts',(19.822202351787,68.7506530370904,12.));
#162339=CARTESIAN_POINT('Ctrl Pts',(19.8355282317858,68.7696140044851,12.));
#162340=CARTESIAN_POINT('Ctrl Pts',(19.8488984255627,68.7885979026879,12.));
#162341=CARTESIAN_POINT('Ctrl Pts',(19.8623129119293,68.8076045880065,12.));
#162342=CARTESIAN_POINT('Ctrl Pts',(19.8757716696965,68.8266339174056,12.));
#162343=CARTESIAN_POINT('Ctrl Pts',(19.8892746776739,68.8456857485002,12.));
#162344=CARTESIAN_POINT('Ctrl Pts',(19.9028219146618,68.8647599395469,12.));
#162345=CARTESIAN_POINT('Ctrl Pts',(19.9164133594525,68.8838563494393,12.));
#162346=CARTESIAN_POINT('Ctrl Pts',(19.9300489908374,68.9029748377067,12.));
#162347=CARTESIAN_POINT('Ctrl Pts',(19.9437287876066,68.9221152645095,12.));
#162348=CARTESIAN_POINT('Ctrl Pts',(19.9574527285488,68.9412774906333,12.));
#162349=CARTESIAN_POINT('Ctrl Pts',(19.9712207924428,68.9604613774802,12.));
#162350=CARTESIAN_POINT('Ctrl Pts',(19.9850329580591,68.9796667870638,12.));
#162351=CARTESIAN_POINT('Ctrl Pts',(19.9988892041666,68.9988935820084,12.));
#162352=CARTESIAN_POINT('Ctrl Pts',(20.0127895095326,69.0181416255431,12.));
#162353=CARTESIAN_POINT('Ctrl Pts',(20.0267338529223,69.0374107814984,12.));
#162354=CARTESIAN_POINT('Ctrl Pts',(20.0407222130905,69.0567009142978,12.));
#162355=CARTESIAN_POINT('Ctrl Pts',(20.0547545687842,69.0760118889535,12.));
#162356=CARTESIAN_POINT('Ctrl Pts',(20.068830898748,69.095343571064,12.));
#162357=CARTESIAN_POINT('Ctrl Pts',(20.0829511817251,69.1146958268104,12.));
#162358=CARTESIAN_POINT('Ctrl Pts',(20.0971153964557,69.1340685229514,12.));
#162359=CARTESIAN_POINT('Ctrl Pts',(20.1113235216694,69.1534615268153,12.));
#162360=CARTESIAN_POINT('Ctrl Pts',(20.1255755360872,69.1728747062963,12.));
#162361=CARTESIAN_POINT('Ctrl Pts',(20.1398714184279,69.1923079298538,12.));
#162362=CARTESIAN_POINT('Ctrl Pts',(20.1542111474087,69.2117610665076,12.));
#162363=CARTESIAN_POINT('Ctrl Pts',(20.1685947017433,69.2312339858335,12.));
#162364=CARTESIAN_POINT('Ctrl Pts',(20.1830220601348,69.2507265579554,12.));
#162365=CARTESIAN_POINT('Ctrl Pts',(20.1974932012773,69.2702386535422,12.));
#162366=CARTESIAN_POINT('Ctrl Pts',(20.212008103862,69.2897701438059,12.));
#162367=CARTESIAN_POINT('Ctrl Pts',(20.2265667465784,69.3093209004984,12.));
#162368=CARTESIAN_POINT('Ctrl Pts',(20.2411691081123,69.3288907959067,12.));
#162369=CARTESIAN_POINT('Ctrl Pts',(20.2558151671391,69.3484797028458,12.));
#162370=CARTESIAN_POINT('Ctrl Pts',(20.2705049023241,69.368087494655,12.));
#162371=CARTESIAN_POINT('Ctrl Pts',(20.2852382923299,69.3877140451975,12.));
#162372=CARTESIAN_POINT('Ctrl Pts',(20.3000153158166,69.407359228856,12.));
#162373=CARTESIAN_POINT('Ctrl Pts',(20.3148359514415,69.4270229205297,12.));
#162374=CARTESIAN_POINT('Ctrl Pts',(20.3297001778507,69.4467049956262,12.));
#162375=CARTESIAN_POINT('Ctrl Pts',(20.3446079736802,69.4664053300587,12.));
#162376=CARTESIAN_POINT('Ctrl Pts',(20.3595593175622,69.4861238002441,12.));
#162377=CARTESIAN_POINT('Ctrl Pts',(20.3745541881268,69.5058602831008,12.));
#162378=CARTESIAN_POINT('Ctrl Pts',(20.3895925640005,69.5256146560441,12.));
#162379=CARTESIAN_POINT('Ctrl Pts',(20.4046744237999,69.5453867969804,12.));
#162380=CARTESIAN_POINT('Ctrl Pts',(20.41979974613,69.5651765843033,12.));
#162381=CARTESIAN_POINT('Ctrl Pts',(20.4349685095923,69.5849838968928,12.));
#162382=CARTESIAN_POINT('Ctrl Pts',(20.4501806927851,69.6048086141113,12.));
#162383=CARTESIAN_POINT('Ctrl Pts',(20.4654362743037,69.6246506158013,12.));
#162384=CARTESIAN_POINT('Ctrl Pts',(20.4807352327339,69.6445097822792,12.));
#162385=CARTESIAN_POINT('Ctrl Pts',(20.4960775466492,69.6643859943308,12.));
#162386=CARTESIAN_POINT('Ctrl Pts',(20.5114631946184,69.6842791332115,12.));
#162387=CARTESIAN_POINT('Ctrl Pts',(20.5268921552077,69.7041890806425,12.));
#162388=CARTESIAN_POINT('Ctrl Pts',(20.5423644069799,69.7241157188083,12.));
#162389=CARTESIAN_POINT('Ctrl Pts',(20.5578799284897,69.744058930351,12.));
#162390=CARTESIAN_POINT('Ctrl Pts',(20.5734386982782,69.7640185983644,12.));
#162391=CARTESIAN_POINT('Ctrl Pts',(20.5890406948811,69.7839946063949,12.));
#162392=CARTESIAN_POINT('Ctrl Pts',(20.6046858968307,69.8039868384389,12.));
#162393=CARTESIAN_POINT('Ctrl Pts',(20.6203742826566,69.8239951789402,12.));
#162394=CARTESIAN_POINT('Ctrl Pts',(20.636105830881,69.8440195127866,12.));
#162395=CARTESIAN_POINT('Ctrl Pts',(20.6518805200129,69.8640597253045,12.));
#162396=CARTESIAN_POINT('Ctrl Pts',(20.667698328554,69.8841157022568,12.));
#162397=CARTESIAN_POINT('Ctrl Pts',(20.683559235003,69.904187329841,12.));
#162398=CARTESIAN_POINT('Ctrl Pts',(20.6994632178551,69.9242744946854,12.));
#162399=CARTESIAN_POINT('Ctrl Pts',(20.7154102555997,69.9443770838448,12.));
#162400=CARTESIAN_POINT('Ctrl Pts',(20.7314003267119,69.9644949847934,12.));
#162401=CARTESIAN_POINT('Ctrl Pts',(20.7474334096581,69.9846280854257,12.));
#162402=CARTESIAN_POINT('Ctrl Pts',(20.7635094829015,70.0047762740568,12.));
#162403=CARTESIAN_POINT('Ctrl Pts',(20.7796285249022,70.024939439422,12.));
#162404=CARTESIAN_POINT('Ctrl Pts',(20.7957905141156,70.0451174706741,12.));
#162405=CARTESIAN_POINT('Ctrl Pts',(20.8119954289848,70.0653102573803,12.));
#162406=CARTESIAN_POINT('Ctrl Pts',(20.8282432479428,70.0855176895191,12.));
#162407=CARTESIAN_POINT('Ctrl Pts',(20.8445339494187,70.1057396574747,12.));
#162408=CARTESIAN_POINT('Ctrl Pts',(20.8608675118378,70.1259760520309,12.));
#162409=CARTESIAN_POINT('Ctrl Pts',(20.8772439136206,70.1462267643647,12.));
#162410=CARTESIAN_POINT('Ctrl Pts',(20.8936631331748,70.1664916860358,12.));
#162411=CARTESIAN_POINT('Ctrl Pts',(20.9101251488943,70.1867707089854,12.));
#162412=CARTESIAN_POINT('Ctrl Pts',(20.9266299391684,70.2070637255458,12.));
#162413=CARTESIAN_POINT('Ctrl Pts',(20.9431774823831,70.2273706284472,12.));
#162414=CARTESIAN_POINT('Ctrl Pts',(20.9597677569228,70.2476913108244,12.));
#162415=CARTESIAN_POINT('Ctrl Pts',(20.9764007411652,70.2680256662224,12.));
#162416=CARTESIAN_POINT('Ctrl Pts',(20.9930764134776,70.2883735885984,12.));
#162417=CARTESIAN_POINT('Ctrl Pts',(21.0097947522218,70.3087349722973,12.));
#162418=CARTESIAN_POINT('Ctrl Pts',(21.0265557357548,70.3291097120302,12.));
#162419=CARTESIAN_POINT('Ctrl Pts',(21.0433593424266,70.3494977028498,12.));
#162420=CARTESIAN_POINT('Ctrl Pts',(21.0602055505748,70.3698988401281,12.));
#162421=CARTESIAN_POINT('Ctrl Pts',(21.0770943385141,70.3903130195265,12.));
#162422=CARTESIAN_POINT('Ctrl Pts',(21.0940256845472,70.4107401370389,12.));
#162423=CARTESIAN_POINT('Ctrl Pts',(21.1109995669747,70.4311800890402,12.));
#162424=CARTESIAN_POINT('Ctrl Pts',(21.1280159641002,70.4516327723346,12.));
#162425=CARTESIAN_POINT('Ctrl Pts',(21.1450748542336,70.4720980841939,12.));
#162426=CARTESIAN_POINT('Ctrl Pts',(21.1621762156897,70.4925759224216,12.));
#162427=CARTESIAN_POINT('Ctrl Pts',(21.1793200267846,70.5130661852955,12.));
#162428=CARTESIAN_POINT('Ctrl Pts',(21.1965062658298,70.5335687714429,12.));
#162429=CARTESIAN_POINT('Ctrl Pts',(21.2137349111208,70.5540835797283,12.));
#162430=CARTESIAN_POINT('Ctrl Pts',(21.2310059409265,70.5746105091502,12.));
#162431=CARTESIAN_POINT('Ctrl Pts',(21.2483193334675,70.5951494586957,12.));
#162432=CARTESIAN_POINT('Ctrl Pts',(21.2656750669126,70.6157003273316,12.));
#162433=CARTESIAN_POINT('Ctrl Pts',(21.2830731194183,70.6362630143047,12.));
#162434=CARTESIAN_POINT('Ctrl Pts',(21.300513469156,70.6568374193774,12.));
#162435=CARTESIAN_POINT('Ctrl Pts',(21.3179960943388,70.6774234430897,12.));
#162436=CARTESIAN_POINT('Ctrl Pts',(21.3355209732443,70.6980209870045,12.));
#162437=CARTESIAN_POINT('Ctrl Pts',(21.3530880842349,70.7186299539724,12.));
#162438=CARTESIAN_POINT('Ctrl Pts',(21.3706974057039,70.7392502475469,12.));
#162439=CARTESIAN_POINT('Ctrl Pts',(21.3883489160196,70.7598817714105,12.));
#162440=CARTESIAN_POINT('Ctrl Pts',(21.4060425934598,70.780524428745,12.));
#162441=CARTESIAN_POINT('Ctrl Pts',(21.4237784161587,70.8011781217394,12.));
#162442=CARTESIAN_POINT('Ctrl Pts',(21.4415563620114,70.8218427507506,12.));
#162443=CARTESIAN_POINT('Ctrl Pts',(21.4593764087473,70.8425182149846,12.));
#162444=CARTESIAN_POINT('Ctrl Pts',(21.477238534096,70.8632044140112,12.));
#162445=CARTESIAN_POINT('Ctrl Pts',(21.4951427159261,70.8839012490871,12.));
#162446=CARTESIAN_POINT('Ctrl Pts',(21.513088932377,70.9046086244131,12.));
#162447=CARTESIAN_POINT('Ctrl Pts',(21.531077162023,70.9253264487637,12.));
#162448=CARTESIAN_POINT('Ctrl Pts',(21.5491073839106,70.94605463587,12.));
#162449=CARTESIAN_POINT('Ctrl Pts',(21.564598755537,70.9638315189818,12.));
#162450=CARTESIAN_POINT('Ctrl Pts',(21.5764983366483,70.977466211259,12.));
#162451=CARTESIAN_POINT('Ctrl Pts',(21.5847875433334,70.9869541808057,12.));
#162452=CARTESIAN_POINT('Ctrl Pts',(21.5894540925586,70.9922924595372,12.));
#162453=CARTESIAN_POINT('Ctrl Pts',(21.5904919935065,70.993479606912,12.));
#162454=CARTESIAN_POINT('',(18.9407177820969,67.3887914263119,0.));
#162455=CARTESIAN_POINT('',(18.9407177820969,67.3887914263118,0.));
#162456=CARTESIAN_POINT('Ctrl Pts',(21.5904919935065,70.993479606912,0.));
#162457=CARTESIAN_POINT('Ctrl Pts',(21.5894540925586,70.9922924595372,0.));
#162458=CARTESIAN_POINT('Ctrl Pts',(21.5847875433334,70.9869541808057,0.));
#162459=CARTESIAN_POINT('Ctrl Pts',(21.5764983366483,70.977466211259,0.));
#162460=CARTESIAN_POINT('Ctrl Pts',(21.564598755537,70.9638315189818,0.));
#162461=CARTESIAN_POINT('Ctrl Pts',(21.5491073839106,70.94605463587,0.));
#162462=CARTESIAN_POINT('Ctrl Pts',(21.531077162023,70.9253264487637,0.));
#162463=CARTESIAN_POINT('Ctrl Pts',(21.513088932377,70.9046086244131,0.));
#162464=CARTESIAN_POINT('Ctrl Pts',(21.4951427159261,70.8839012490871,0.));
#162465=CARTESIAN_POINT('Ctrl Pts',(21.477238534096,70.8632044140112,0.));
#162466=CARTESIAN_POINT('Ctrl Pts',(21.4593764087473,70.8425182149846,0.));
#162467=CARTESIAN_POINT('Ctrl Pts',(21.4415563620114,70.8218427507506,0.));
#162468=CARTESIAN_POINT('Ctrl Pts',(21.4237784161587,70.8011781217394,0.));
#162469=CARTESIAN_POINT('Ctrl Pts',(21.4060425934598,70.780524428745,0.));
#162470=CARTESIAN_POINT('Ctrl Pts',(21.3883489160196,70.7598817714105,0.));
#162471=CARTESIAN_POINT('Ctrl Pts',(21.3706974057039,70.7392502475469,0.));
#162472=CARTESIAN_POINT('Ctrl Pts',(21.3530880842349,70.7186299539724,0.));
#162473=CARTESIAN_POINT('Ctrl Pts',(21.3355209732443,70.6980209870045,0.));
#162474=CARTESIAN_POINT('Ctrl Pts',(21.3179960943388,70.6774234430897,0.));
#162475=CARTESIAN_POINT('Ctrl Pts',(21.300513469156,70.6568374193774,0.));
#162476=CARTESIAN_POINT('Ctrl Pts',(21.2830731194183,70.6362630143047,0.));
#162477=CARTESIAN_POINT('Ctrl Pts',(21.2656750669126,70.6157003273316,0.));
#162478=CARTESIAN_POINT('Ctrl Pts',(21.2483193334675,70.5951494586957,0.));
#162479=CARTESIAN_POINT('Ctrl Pts',(21.2310059409265,70.5746105091502,0.));
#162480=CARTESIAN_POINT('Ctrl Pts',(21.2137349111208,70.5540835797283,0.));
#162481=CARTESIAN_POINT('Ctrl Pts',(21.1965062658298,70.5335687714429,0.));
#162482=CARTESIAN_POINT('Ctrl Pts',(21.1793200267846,70.5130661852955,0.));
#162483=CARTESIAN_POINT('Ctrl Pts',(21.1621762156897,70.4925759224216,0.));
#162484=CARTESIAN_POINT('Ctrl Pts',(21.1450748542336,70.4720980841939,0.));
#162485=CARTESIAN_POINT('Ctrl Pts',(21.1280159641002,70.4516327723346,0.));
#162486=CARTESIAN_POINT('Ctrl Pts',(21.1109995669747,70.4311800890402,0.));
#162487=CARTESIAN_POINT('Ctrl Pts',(21.0940256845472,70.4107401370389,0.));
#162488=CARTESIAN_POINT('Ctrl Pts',(21.0770943385141,70.3903130195265,0.));
#162489=CARTESIAN_POINT('Ctrl Pts',(21.0602055505748,70.3698988401281,0.));
#162490=CARTESIAN_POINT('Ctrl Pts',(21.0433593424266,70.3494977028498,0.));
#162491=CARTESIAN_POINT('Ctrl Pts',(21.0265557357548,70.3291097120302,0.));
#162492=CARTESIAN_POINT('Ctrl Pts',(21.0097947522218,70.3087349722973,0.));
#162493=CARTESIAN_POINT('Ctrl Pts',(20.9930764134776,70.2883735885984,0.));
#162494=CARTESIAN_POINT('Ctrl Pts',(20.9764007411652,70.2680256662224,0.));
#162495=CARTESIAN_POINT('Ctrl Pts',(20.9597677569228,70.2476913108244,0.));
#162496=CARTESIAN_POINT('Ctrl Pts',(20.9431774823831,70.2273706284472,0.));
#162497=CARTESIAN_POINT('Ctrl Pts',(20.9266299391684,70.2070637255458,0.));
#162498=CARTESIAN_POINT('Ctrl Pts',(20.9101251488943,70.1867707089854,0.));
#162499=CARTESIAN_POINT('Ctrl Pts',(20.8936631331748,70.1664916860358,0.));
#162500=CARTESIAN_POINT('Ctrl Pts',(20.8772439136206,70.1462267643647,0.));
#162501=CARTESIAN_POINT('Ctrl Pts',(20.8608675118378,70.1259760520309,0.));
#162502=CARTESIAN_POINT('Ctrl Pts',(20.8445339494187,70.1057396574747,0.));
#162503=CARTESIAN_POINT('Ctrl Pts',(20.8282432479428,70.0855176895191,0.));
#162504=CARTESIAN_POINT('Ctrl Pts',(20.8119954289848,70.0653102573803,0.));
#162505=CARTESIAN_POINT('Ctrl Pts',(20.7957905141156,70.0451174706741,0.));
#162506=CARTESIAN_POINT('Ctrl Pts',(20.7796285249022,70.024939439422,0.));
#162507=CARTESIAN_POINT('Ctrl Pts',(20.7635094829015,70.0047762740568,0.));
#162508=CARTESIAN_POINT('Ctrl Pts',(20.7474334096581,69.9846280854257,0.));
#162509=CARTESIAN_POINT('Ctrl Pts',(20.7314003267119,69.9644949847934,0.));
#162510=CARTESIAN_POINT('Ctrl Pts',(20.7154102555997,69.9443770838448,0.));
#162511=CARTESIAN_POINT('Ctrl Pts',(20.6994632178551,69.9242744946854,0.));
#162512=CARTESIAN_POINT('Ctrl Pts',(20.683559235003,69.904187329841,0.));
#162513=CARTESIAN_POINT('Ctrl Pts',(20.667698328554,69.8841157022568,0.));
#162514=CARTESIAN_POINT('Ctrl Pts',(20.6518805200129,69.8640597253045,0.));
#162515=CARTESIAN_POINT('Ctrl Pts',(20.636105830881,69.8440195127866,0.));
#162516=CARTESIAN_POINT('Ctrl Pts',(20.6203742826566,69.8239951789402,0.));
#162517=CARTESIAN_POINT('Ctrl Pts',(20.6046858968307,69.8039868384389,0.));
#162518=CARTESIAN_POINT('Ctrl Pts',(20.5890406948811,69.7839946063949,0.));
#162519=CARTESIAN_POINT('Ctrl Pts',(20.5734386982782,69.7640185983644,0.));
#162520=CARTESIAN_POINT('Ctrl Pts',(20.5578799284897,69.744058930351,0.));
#162521=CARTESIAN_POINT('Ctrl Pts',(20.5423644069799,69.7241157188083,0.));
#162522=CARTESIAN_POINT('Ctrl Pts',(20.5268921552077,69.7041890806425,0.));
#162523=CARTESIAN_POINT('Ctrl Pts',(20.5114631946184,69.6842791332115,0.));
#162524=CARTESIAN_POINT('Ctrl Pts',(20.4960775466492,69.6643859943308,0.));
#162525=CARTESIAN_POINT('Ctrl Pts',(20.4807352327339,69.6445097822792,0.));
#162526=CARTESIAN_POINT('Ctrl Pts',(20.4654362743037,69.6246506158013,0.));
#162527=CARTESIAN_POINT('Ctrl Pts',(20.4501806927851,69.6048086141113,0.));
#162528=CARTESIAN_POINT('Ctrl Pts',(20.4349685095923,69.5849838968928,0.));
#162529=CARTESIAN_POINT('Ctrl Pts',(20.41979974613,69.5651765843033,0.));
#162530=CARTESIAN_POINT('Ctrl Pts',(20.4046744237999,69.5453867969804,0.));
#162531=CARTESIAN_POINT('Ctrl Pts',(20.3895925640005,69.5256146560441,0.));
#162532=CARTESIAN_POINT('Ctrl Pts',(20.3745541881268,69.5058602831008,0.));
#162533=CARTESIAN_POINT('Ctrl Pts',(20.3595593175622,69.4861238002441,0.));
#162534=CARTESIAN_POINT('Ctrl Pts',(20.3446079736802,69.4664053300587,0.));
#162535=CARTESIAN_POINT('Ctrl Pts',(20.3297001778507,69.4467049956262,0.));
#162536=CARTESIAN_POINT('Ctrl Pts',(20.3148359514415,69.4270229205297,0.));
#162537=CARTESIAN_POINT('Ctrl Pts',(20.3000153158166,69.407359228856,0.));
#162538=CARTESIAN_POINT('Ctrl Pts',(20.2852382923299,69.3877140451975,0.));
#162539=CARTESIAN_POINT('Ctrl Pts',(20.2705049023241,69.368087494655,0.));
#162540=CARTESIAN_POINT('Ctrl Pts',(20.2558151671391,69.3484797028458,0.));
#162541=CARTESIAN_POINT('Ctrl Pts',(20.2411691081123,69.3288907959067,0.));
#162542=CARTESIAN_POINT('Ctrl Pts',(20.2265667465784,69.3093209004984,0.));
#162543=CARTESIAN_POINT('Ctrl Pts',(20.212008103862,69.2897701438059,0.));
#162544=CARTESIAN_POINT('Ctrl Pts',(20.1974932012773,69.2702386535422,0.));
#162545=CARTESIAN_POINT('Ctrl Pts',(20.1830220601348,69.2507265579554,0.));
#162546=CARTESIAN_POINT('Ctrl Pts',(20.1685947017433,69.2312339858335,0.));
#162547=CARTESIAN_POINT('Ctrl Pts',(20.1542111474087,69.2117610665076,0.));
#162548=CARTESIAN_POINT('Ctrl Pts',(20.1398714184279,69.1923079298538,0.));
#162549=CARTESIAN_POINT('Ctrl Pts',(20.1255755360872,69.1728747062963,0.));
#162550=CARTESIAN_POINT('Ctrl Pts',(20.1113235216694,69.1534615268153,0.));
#162551=CARTESIAN_POINT('Ctrl Pts',(20.0971153964557,69.1340685229514,0.));
#162552=CARTESIAN_POINT('Ctrl Pts',(20.0829511817251,69.1146958268104,0.));
#162553=CARTESIAN_POINT('Ctrl Pts',(20.068830898748,69.095343571064,0.));
#162554=CARTESIAN_POINT('Ctrl Pts',(20.0547545687842,69.0760118889535,0.));
#162555=CARTESIAN_POINT('Ctrl Pts',(20.0407222130905,69.0567009142978,0.));
#162556=CARTESIAN_POINT('Ctrl Pts',(20.0267338529223,69.0374107814984,0.));
#162557=CARTESIAN_POINT('Ctrl Pts',(20.0127895095326,69.0181416255431,0.));
#162558=CARTESIAN_POINT('Ctrl Pts',(19.9988892041666,68.9988935820084,0.));
#162559=CARTESIAN_POINT('Ctrl Pts',(19.9850329580591,68.9796667870638,0.));
#162560=CARTESIAN_POINT('Ctrl Pts',(19.9712207924428,68.9604613774802,0.));
#162561=CARTESIAN_POINT('Ctrl Pts',(19.9574527285488,68.9412774906333,0.));
#162562=CARTESIAN_POINT('Ctrl Pts',(19.9437287876066,68.9221152645095,0.));
#162563=CARTESIAN_POINT('Ctrl Pts',(19.9300489908374,68.9029748377067,0.));
#162564=CARTESIAN_POINT('Ctrl Pts',(19.9164133594525,68.8838563494393,0.));
#162565=CARTESIAN_POINT('Ctrl Pts',(19.9028219146618,68.8647599395469,0.));
#162566=CARTESIAN_POINT('Ctrl Pts',(19.8892746776739,68.8456857485002,0.));
#162567=CARTESIAN_POINT('Ctrl Pts',(19.8757716696965,68.8266339174056,0.));
#162568=CARTESIAN_POINT('Ctrl Pts',(19.8623129119293,68.8076045880065,0.));
#162569=CARTESIAN_POINT('Ctrl Pts',(19.8488984255627,68.7885979026879,0.));
#162570=CARTESIAN_POINT('Ctrl Pts',(19.8355282317858,68.7696140044851,0.));
#162571=CARTESIAN_POINT('Ctrl Pts',(19.822202351787,68.7506530370904,0.));
#162572=CARTESIAN_POINT('Ctrl Pts',(19.8089208067537,68.7317151448573,0.));
#162573=CARTESIAN_POINT('Ctrl Pts',(19.7956836178651,68.7128004728034,0.));
#162574=CARTESIAN_POINT('Ctrl Pts',(19.7824908062924,68.693909166615,0.));
#162575=CARTESIAN_POINT('Ctrl Pts',(19.7693423932066,68.6750413726575,0.));
#162576=CARTESIAN_POINT('Ctrl Pts',(19.7562383997783,68.65619723798,0.));
#162577=CARTESIAN_POINT('Ctrl Pts',(19.7431788471772,68.6373769103211,0.));
#162578=CARTESIAN_POINT('Ctrl Pts',(19.7301637565645,68.6185805381102,0.));
#162579=CARTESIAN_POINT('Ctrl Pts',(19.717193149095,68.5998082704741,0.));
#162580=CARTESIAN_POINT('Ctrl Pts',(19.7042670459233,68.5810602572474,0.));
#162581=CARTESIAN_POINT('Ctrl Pts',(19.6913854682046,68.5623366489776,0.));
#162582=CARTESIAN_POINT('Ctrl Pts',(19.6785484370929,68.543637596932,0.));
#162583=CARTESIAN_POINT('Ctrl Pts',(19.665755973734,68.5249632530994,0.));
#162584=CARTESIAN_POINT('Ctrl Pts',(19.6530080992689,68.5063137701986,0.));
#162585=CARTESIAN_POINT('Ctrl Pts',(19.6403048348396,68.4876893016863,0.));
#162586=CARTESIAN_POINT('Ctrl Pts',(19.6276462015888,68.4690900017631,0.));
#162587=CARTESIAN_POINT('Ctrl Pts',(19.6150322206577,68.4505160253777,0.));
#162588=CARTESIAN_POINT('Ctrl Pts',(19.6024629131785,68.4319675282273,0.));
#162589=CARTESIAN_POINT('Ctrl Pts',(19.5899383002803,68.4134446667695,0.));
#162590=CARTESIAN_POINT('Ctrl Pts',(19.5774584030938,68.3949475982334,0.));
#162591=CARTESIAN_POINT('Ctrl Pts',(19.5650232427516,68.3764764806287,0.));
#162592=CARTESIAN_POINT('Ctrl Pts',(19.5526328403851,68.3580314727522,0.));
#162593=CARTESIAN_POINT('Ctrl Pts',(19.540287217119,68.3396127341937,0.));
#162594=CARTESIAN_POINT('Ctrl Pts',(19.5279863940772,68.3212204253416,0.));
#162595=CARTESIAN_POINT('Ctrl Pts',(19.5157303923855,68.3028547073862,0.));
#162596=CARTESIAN_POINT('Ctrl Pts',(19.5035192331706,68.2845157423234,0.));
#162597=CARTESIAN_POINT('Ctrl Pts',(19.4913529375545,68.2662036929531,0.));
#162598=CARTESIAN_POINT('Ctrl Pts',(19.4792315266505,68.2479187228815,0.));
#162599=CARTESIAN_POINT('Ctrl Pts',(19.4671550215724,68.2296609965461,0.));
#162600=CARTESIAN_POINT('Ctrl Pts',(19.4551234434383,68.2114306792366,0.));
#162601=CARTESIAN_POINT('Ctrl Pts',(19.4431368133718,68.1932279371121,0.));
#162602=CARTESIAN_POINT('Ctrl Pts',(19.4311951524977,68.1750529372211,0.));
#162603=CARTESIAN_POINT('Ctrl Pts',(19.419298481941,68.1569058475026,0.));
#162604=CARTESIAN_POINT('Ctrl Pts',(19.4074468228293,68.1387868367668,0.));
#162605=CARTESIAN_POINT('Ctrl Pts',(19.3956401962893,68.1206960746763,0.));
#162606=CARTESIAN_POINT('Ctrl Pts',(19.3838786234425,68.1026337317298,0.));
#162607=CARTESIAN_POINT('Ctrl Pts',(19.372162125392,68.0845999792274,0.));
#162608=CARTESIAN_POINT('Ctrl Pts',(19.3604907232322,68.0665949893222,0.));
#162609=CARTESIAN_POINT('Ctrl Pts',(19.3488644380646,68.0486189351027,0.));
#162610=CARTESIAN_POINT('Ctrl Pts',(19.3372832910076,68.0306719906636,0.));
#162611=CARTESIAN_POINT('Ctrl Pts',(19.3257473032031,68.0127543311761,0.));
#162612=CARTESIAN_POINT('Ctrl Pts',(19.3142564958195,67.9948661329592,0.));
#162613=CARTESIAN_POINT('Ctrl Pts',(19.3028108900373,67.977007573346,0.));
#162614=CARTESIAN_POINT('Ctrl Pts',(19.2914105070282,67.959178830538,0.));
#162615=CARTESIAN_POINT('Ctrl Pts',(19.2800553679362,67.9413800834798,0.));
#162616=CARTESIAN_POINT('Ctrl Pts',(19.2687454938448,67.9236115116781,0.));
#162617=CARTESIAN_POINT('Ctrl Pts',(19.2574809057705,67.9058732951822,0.));
#162618=CARTESIAN_POINT('Ctrl Pts',(19.2462616247287,67.8881656149983,0.));
#162619=CARTESIAN_POINT('Ctrl Pts',(19.2350876717877,67.8704886534555,0.));
#162620=CARTESIAN_POINT('Ctrl Pts',(19.2239590681129,67.852842594517,0.));
#162621=CARTESIAN_POINT('Ctrl Pts',(19.2128758350336,67.8352276242856,0.));
#162622=CARTESIAN_POINT('Ctrl Pts',(19.2018379939918,67.817643930658,0.));
#162623=CARTESIAN_POINT('Ctrl Pts',(19.1908455664089,67.8000917023896,0.));
#162624=CARTESIAN_POINT('Ctrl Pts',(19.1798985735687,67.7825711283092,0.));
#162625=CARTESIAN_POINT('Ctrl Pts',(19.1689970364958,67.7650823965156,0.));
#162626=CARTESIAN_POINT('Ctrl Pts',(19.1581409758111,67.7476256934493,0.));
#162627=CARTESIAN_POINT('Ctrl Pts',(19.1473304119968,67.730201205663,0.));
#162628=CARTESIAN_POINT('Ctrl Pts',(19.1365653657097,67.7128091219372,0.));
#162629=CARTESIAN_POINT('Ctrl Pts',(19.1258458580343,67.6954496350053,0.));
#162630=CARTESIAN_POINT('Ctrl Pts',(19.115171910845,67.6781229440535,0.));
#162631=CARTESIAN_POINT('Ctrl Pts',(19.1045435468344,67.6608292549412,0.));
#162632=CARTESIAN_POINT('Ctrl Pts',(19.0939607887491,67.6435687749803,0.));
#162633=CARTESIAN_POINT('Ctrl Pts',(19.0834236587115,67.6263417083414,0.));
#162634=CARTESIAN_POINT('Ctrl Pts',(19.0729321776286,67.6091482520558,0.));
#162635=CARTESIAN_POINT('Ctrl Pts',(19.0624863642425,67.5919885896278,0.));
#162636=CARTESIAN_POINT('Ctrl Pts',(19.0520862360413,67.5748628972035,0.));
#162637=CARTESIAN_POINT('Ctrl Pts',(19.0417318110721,67.5577713558248,0.));
#162638=CARTESIAN_POINT('Ctrl Pts',(19.0314231093923,67.5407141612881,0.));
#162639=CARTESIAN_POINT('Ctrl Pts',(19.0211601548222,67.5236915360253,0.));
#162640=CARTESIAN_POINT('Ctrl Pts',(19.0109429761274,67.5067037372177,0.));
#162641=CARTESIAN_POINT('Ctrl Pts',(19.0007716032784,67.4897510316692,0.));
#162642=CARTESIAN_POINT('Ctrl Pts',(18.9906460638607,67.4728336719559,0.));
#162643=CARTESIAN_POINT('Ctrl Pts',(18.9805663798466,67.4559518744714,0.));
#162644=CARTESIAN_POINT('Ctrl Pts',(18.9705325631772,67.4391057908687,0.));
#162645=CARTESIAN_POINT('Ctrl Pts',(18.9605446161078,67.4222955062385,0.));
#162646=CARTESIAN_POINT('Ctrl Pts',(18.9525909518002,67.4088759498287,0.));
#162647=CARTESIAN_POINT('Ctrl Pts',(18.9466463414354,67.398827414689,0.));
#162648=CARTESIAN_POINT('Ctrl Pts',(18.942692439874,67.3921355608417,0.));
#162649=CARTESIAN_POINT('Ctrl Pts',(18.9407177820969,67.3887914263119,0.));
#162650=CARTESIAN_POINT('Ctrl Pts',(27.9316983239472,69.065695021045,0.));
#162651=CARTESIAN_POINT('Ctrl Pts',(27.9316983239472,69.065695021045,12.));
#162652=CARTESIAN_POINT('Ctrl Pts',(27.9276214070631,69.0618620884721,0.));
#162653=CARTESIAN_POINT('Ctrl Pts',(27.9276214070631,69.0618620884721,12.));
#162654=CARTESIAN_POINT('Ctrl Pts',(27.9194718099003,69.0541967851028,0.));
#162655=CARTESIAN_POINT('Ctrl Pts',(27.9194718099003,69.0541967851028,12.));
#162656=CARTESIAN_POINT('Ctrl Pts',(27.9072601239722,69.0427005153791,0.));
#162657=CARTESIAN_POINT('Ctrl Pts',(27.9072601239722,69.0427005153791,12.));
#162658=CARTESIAN_POINT('Ctrl Pts',(27.8910032967339,69.0273755265383,0.));
#162659=CARTESIAN_POINT('Ctrl Pts',(27.8910032967339,69.0273755265383,12.));
#162660=CARTESIAN_POINT('Ctrl Pts',(27.8707246380956,69.0082249138598,0.));
#162661=CARTESIAN_POINT('Ctrl Pts',(27.8707246380956,69.0082249138598,12.));
#162662=CARTESIAN_POINT('Ctrl Pts',(27.8504883674058,68.9890799392213,0.));
#162663=CARTESIAN_POINT('Ctrl Pts',(27.8504883674058,68.9890799392213,12.));
#162664=CARTESIAN_POINT('Ctrl Pts',(27.8302945019976,68.9699406311389,0.));
#162665=CARTESIAN_POINT('Ctrl Pts',(27.8302945019976,68.9699406311389,12.));
#162666=CARTESIAN_POINT('Ctrl Pts',(27.8101430638071,68.9508070357658,0.));
#162667=CARTESIAN_POINT('Ctrl Pts',(27.8101430638071,68.9508070357658,12.));
#162668=CARTESIAN_POINT('Ctrl Pts',(27.7900340793689,68.9316792225946,0.));
#162669=CARTESIAN_POINT('Ctrl Pts',(27.7900340793689,68.9316792225946,12.));
#162670=CARTESIAN_POINT('Ctrl Pts',(27.7699675790571,68.9125572825694,0.));
#162671=CARTESIAN_POINT('Ctrl Pts',(27.7699675790571,68.9125572825694,12.));
#162672=CARTESIAN_POINT('Ctrl Pts',(27.7499435957525,68.8934413203759,0.));
#162673=CARTESIAN_POINT('Ctrl Pts',(27.7499435957525,68.8934413203759,12.));
#162674=CARTESIAN_POINT('Ctrl Pts',(27.7299621636566,68.8743314483369,0.));
#162675=CARTESIAN_POINT('Ctrl Pts',(27.7299621636566,68.8743314483369,12.));
#162676=CARTESIAN_POINT('Ctrl Pts',(27.7100233170737,68.85522777982,0.));
#162677=CARTESIAN_POINT('Ctrl Pts',(27.7100233170737,68.85522777982,12.));
#162678=CARTESIAN_POINT('Ctrl Pts',(27.6901270891241,68.8361304224467,0.));
#162679=CARTESIAN_POINT('Ctrl Pts',(27.6901270891241,68.8361304224467,12.));
#162680=CARTESIAN_POINT('Ctrl Pts',(27.6702735107121,68.81703947259,0.));
#162681=CARTESIAN_POINT('Ctrl Pts',(27.6702735107121,68.81703947259,12.));
#162682=CARTESIAN_POINT('Ctrl Pts',(27.6504626112666,68.7979550191872,0.));
#162683=CARTESIAN_POINT('Ctrl Pts',(27.6504626112666,68.7979550191872,12.));
#162684=CARTESIAN_POINT('Ctrl Pts',(27.6306944192737,68.7788771464713,0.));
#162685=CARTESIAN_POINT('Ctrl Pts',(27.6306944192737,68.7788771464713,12.));
#162686=CARTESIAN_POINT('Ctrl Pts',(27.6109689629029,68.7598059372129,0.));
#162687=CARTESIAN_POINT('Ctrl Pts',(27.6109689629029,68.7598059372129,12.));
#162688=CARTESIAN_POINT('Ctrl Pts',(27.5912862705468,68.740741475526,0.));
#162689=CARTESIAN_POINT('Ctrl Pts',(27.5912862705468,68.740741475526,12.));
#162690=CARTESIAN_POINT('Ctrl Pts',(27.5716463715004,68.7216838504218,0.));
#162691=CARTESIAN_POINT('Ctrl Pts',(27.5716463715004,68.7216838504218,12.));
#162692=CARTESIAN_POINT('Ctrl Pts',(27.5520492958906,68.7026331554296,0.));
#162693=CARTESIAN_POINT('Ctrl Pts',(27.5520492958906,68.7026331554296,12.));
#162694=CARTESIAN_POINT('Ctrl Pts',(27.5324950743706,68.6835894869882,0.));
#162695=CARTESIAN_POINT('Ctrl Pts',(27.5324950743706,68.6835894869882,12.));
#162696=CARTESIAN_POINT('Ctrl Pts',(27.5129837378791,68.6645529432045,0.));
#162697=CARTESIAN_POINT('Ctrl Pts',(27.5129837378791,68.6645529432045,12.));
#162698=CARTESIAN_POINT('Ctrl Pts',(27.4935153173868,68.645523622548,0.));
#162699=CARTESIAN_POINT('Ctrl Pts',(27.4935153173868,68.645523622548,12.));
#162700=CARTESIAN_POINT('Ctrl Pts',(27.4740898435988,68.6265016223561,0.));
#162701=CARTESIAN_POINT('Ctrl Pts',(27.4740898435988,68.6265016223561,12.));
#162702=CARTESIAN_POINT('Ctrl Pts',(27.4547073468226,68.6074870381619,0.));
#162703=CARTESIAN_POINT('Ctrl Pts',(27.4547073468226,68.6074870381619,12.));
#162704=CARTESIAN_POINT('Ctrl Pts',(27.435367857136,68.5884799645218,0.));
#162705=CARTESIAN_POINT('Ctrl Pts',(27.435367857136,68.5884799645218,12.));
#162706=CARTESIAN_POINT('Ctrl Pts',(27.4160714044831,68.5694804955014,0.));
#162707=CARTESIAN_POINT('Ctrl Pts',(27.4160714044831,68.5694804955014,12.));
#162708=CARTESIAN_POINT('Ctrl Pts',(27.3968180187941,68.5504887252975,0.));
#162709=CARTESIAN_POINT('Ctrl Pts',(27.3968180187941,68.5504887252975,12.));
#162710=CARTESIAN_POINT('Ctrl Pts',(27.3776077300914,68.5315047488035,0.));
#162711=CARTESIAN_POINT('Ctrl Pts',(27.3776077300914,68.5315047488035,12.));
#162712=CARTESIAN_POINT('Ctrl Pts',(27.3584405685941,68.5125286621888,0.));
#162713=CARTESIAN_POINT('Ctrl Pts',(27.3584405685941,68.5125286621888,12.));
#162714=CARTESIAN_POINT('Ctrl Pts',(27.3393165646748,68.4935605626362,0.));
#162715=CARTESIAN_POINT('Ctrl Pts',(27.3393165646748,68.4935605626362,12.));
#162716=CARTESIAN_POINT('Ctrl Pts',(27.3202357488153,68.4746005480993,0.));
#162717=CARTESIAN_POINT('Ctrl Pts',(27.3202357488153,68.4746005480993,12.));
#162718=CARTESIAN_POINT('Ctrl Pts',(27.301198151557,68.455648717044,0.));
#162719=CARTESIAN_POINT('Ctrl Pts',(27.301198151557,68.455648717044,12.));
#162720=CARTESIAN_POINT('Ctrl Pts',(27.2822038034539,68.4367051682166,0.));
#162721=CARTESIAN_POINT('Ctrl Pts',(27.2822038034539,68.4367051682166,12.));
#162722=CARTESIAN_POINT('Ctrl Pts',(27.2632527350062,68.4177700003471,0.));
#162723=CARTESIAN_POINT('Ctrl Pts',(27.2632527350062,68.4177700003471,12.));
#162724=CARTESIAN_POINT('Ctrl Pts',(27.2443449766654,68.398843312159,0.));
#162725=CARTESIAN_POINT('Ctrl Pts',(27.2443449766654,68.398843312159,12.));
#162726=CARTESIAN_POINT('Ctrl Pts',(27.2254805588677,68.379925202511,0.));
#162727=CARTESIAN_POINT('Ctrl Pts',(27.2254805588677,68.379925202511,12.));
#162728=CARTESIAN_POINT('Ctrl Pts',(27.2066595120544,68.3610157704999,0.));
#162729=CARTESIAN_POINT('Ctrl Pts',(27.2066595120544,68.3610157704999,12.));
#162730=CARTESIAN_POINT('Ctrl Pts',(27.1878818666925,68.3421151155708,0.));
#162731=CARTESIAN_POINT('Ctrl Pts',(27.1878818666925,68.3421151155708,12.));
#162732=CARTESIAN_POINT('Ctrl Pts',(27.1691476532917,68.3232233376415,0.));
#162733=CARTESIAN_POINT('Ctrl Pts',(27.1691476532917,68.3232233376415,12.));
#162734=CARTESIAN_POINT('Ctrl Pts',(27.150456902413,68.3043405371589,0.));
#162735=CARTESIAN_POINT('Ctrl Pts',(27.150456902413,68.3043405371589,12.));
#162736=CARTESIAN_POINT('Ctrl Pts',(27.1318096446643,68.285466815035,0.));
#162737=CARTESIAN_POINT('Ctrl Pts',(27.1318096446643,68.285466815035,12.));
#162738=CARTESIAN_POINT('Ctrl Pts',(27.1132059106938,68.2666022726094,0.));
#162739=CARTESIAN_POINT('Ctrl Pts',(27.1132059106938,68.2666022726094,12.));
#162740=CARTESIAN_POINT('Ctrl Pts',(27.0946457311813,68.2477470116014,0.));
#162741=CARTESIAN_POINT('Ctrl Pts',(27.0946457311813,68.2477470116014,12.));
#162742=CARTESIAN_POINT('Ctrl Pts',(27.076129136823,68.2289011340624,0.));
#162743=CARTESIAN_POINT('Ctrl Pts',(27.076129136823,68.2289011340624,12.));
#162744=CARTESIAN_POINT('Ctrl Pts',(27.0576561583179,68.2100647423345,0.));
#162745=CARTESIAN_POINT('Ctrl Pts',(27.0576561583179,68.2100647423345,12.));
#162746=CARTESIAN_POINT('Ctrl Pts',(27.0392268263804,68.1912379390787,0.));
#162747=CARTESIAN_POINT('Ctrl Pts',(27.0392268263804,68.1912379390787,12.));
#162748=CARTESIAN_POINT('Ctrl Pts',(27.0208411717477,68.1724208272967,0.));
#162749=CARTESIAN_POINT('Ctrl Pts',(27.0208411717477,68.1724208272967,12.));
#162750=CARTESIAN_POINT('Ctrl Pts',(27.0024992251839,68.1536135103558,0.));
#162751=CARTESIAN_POINT('Ctrl Pts',(27.0024992251839,68.1536135103558,12.));
#162752=CARTESIAN_POINT('Ctrl Pts',(26.9842010174818,68.13481609201,0.));
#162753=CARTESIAN_POINT('Ctrl Pts',(26.9842010174818,68.13481609201,12.));
#162754=CARTESIAN_POINT('Ctrl Pts',(26.9659465794596,68.1160286764244,0.));
#162755=CARTESIAN_POINT('Ctrl Pts',(26.9659465794596,68.1160286764244,12.));
#162756=CARTESIAN_POINT('Ctrl Pts',(26.9477359419646,68.0972513681739,0.));
#162757=CARTESIAN_POINT('Ctrl Pts',(26.9477359419646,68.0972513681739,12.));
#162758=CARTESIAN_POINT('Ctrl Pts',(26.9295691358775,68.0784842722362,0.));
#162759=CARTESIAN_POINT('Ctrl Pts',(26.9295691358775,68.0784842722362,12.));
#162760=CARTESIAN_POINT('Ctrl Pts',(26.9114461921108,68.0597274939857,0.));
#162761=CARTESIAN_POINT('Ctrl Pts',(26.9114461921108,68.0597274939857,12.));
#162762=CARTESIAN_POINT('Ctrl Pts',(26.8933671416064,68.0409811391872,0.));
#162763=CARTESIAN_POINT('Ctrl Pts',(26.8933671416064,68.0409811391872,12.));
#162764=CARTESIAN_POINT('Ctrl Pts',(26.8753320153255,68.0222453139862,0.));
#162765=CARTESIAN_POINT('Ctrl Pts',(26.8753320153255,68.0222453139862,12.));
#162766=CARTESIAN_POINT('Ctrl Pts',(26.85734084425,68.0035201249108,0.));
#162767=CARTESIAN_POINT('Ctrl Pts',(26.85734084425,68.0035201249108,12.));
#162768=CARTESIAN_POINT('Ctrl Pts',(26.8393936593914,67.9848056788814,0.));
#162769=CARTESIAN_POINT('Ctrl Pts',(26.8393936593914,67.9848056788814,12.));
#162770=CARTESIAN_POINT('Ctrl Pts',(26.8214904917921,67.9661020832165,0.));
#162771=CARTESIAN_POINT('Ctrl Pts',(26.8214904917921,67.9661020832165,12.));
#162772=CARTESIAN_POINT('Ctrl Pts',(26.8036313725262,67.9474094456395,0.));
#162773=CARTESIAN_POINT('Ctrl Pts',(26.8036313725262,67.9474094456395,12.));
#162774=CARTESIAN_POINT('Ctrl Pts',(26.7858163326932,67.9287278742839,0.));
#162775=CARTESIAN_POINT('Ctrl Pts',(26.7858163326932,67.9287278742839,12.));
#162776=CARTESIAN_POINT('Ctrl Pts',(26.7680454034168,67.9100574776974,0.));
#162777=CARTESIAN_POINT('Ctrl Pts',(26.7680454034168,67.9100574776974,12.));
#162778=CARTESIAN_POINT('Ctrl Pts',(26.7503186158523,67.8913983648441,0.));
#162779=CARTESIAN_POINT('Ctrl Pts',(26.7503186158523,67.8913983648441,12.));
#162780=CARTESIAN_POINT('Ctrl Pts',(26.7326360011886,67.8727506451068,0.));
#162781=CARTESIAN_POINT('Ctrl Pts',(26.7326360011886,67.8727506451068,12.));
#162782=CARTESIAN_POINT('Ctrl Pts',(26.7149975906478,67.8541144282875,0.));
#162783=CARTESIAN_POINT('Ctrl Pts',(26.7149975906478,67.8541144282875,12.));
#162784=CARTESIAN_POINT('Ctrl Pts',(26.6974034154802,67.8354898246079,0.));
#162785=CARTESIAN_POINT('Ctrl Pts',(26.6974034154802,67.8354898246079,12.));
#162786=CARTESIAN_POINT('Ctrl Pts',(26.6798535069586,67.8168769447086,0.));
#162787=CARTESIAN_POINT('Ctrl Pts',(26.6798535069586,67.8168769447086,12.));
#162788=CARTESIAN_POINT('Ctrl Pts',(26.6623478963867,67.7982758996557,0.));
#162789=CARTESIAN_POINT('Ctrl Pts',(26.6623478963867,67.7982758996557,12.));
#162790=CARTESIAN_POINT('Ctrl Pts',(26.6448866151027,67.7796868009447,0.));
#162791=CARTESIAN_POINT('Ctrl Pts',(26.6448866151027,67.7796868009447,12.));
#162792=CARTESIAN_POINT('Ctrl Pts',(26.6274696944793,67.7611097605042,0.));
#162793=CARTESIAN_POINT('Ctrl Pts',(26.6274696944793,67.7611097605042,12.));
#162794=CARTESIAN_POINT('Ctrl Pts',(26.6100971659204,67.7425448906983,0.));
#162795=CARTESIAN_POINT('Ctrl Pts',(26.6100971659204,67.7425448906983,12.));
#162796=CARTESIAN_POINT('Ctrl Pts',(26.5927690608546,67.7239923043295,0.));
#162797=CARTESIAN_POINT('Ctrl Pts',(26.5927690608546,67.7239923043295,12.));
#162798=CARTESIAN_POINT('Ctrl Pts',(26.5754854107422,67.7054521146427,0.));
#162799=CARTESIAN_POINT('Ctrl Pts',(26.5754854107422,67.7054521146427,12.));
#162800=CARTESIAN_POINT('Ctrl Pts',(26.5582462470794,67.6869244353292,0.));
#162801=CARTESIAN_POINT('Ctrl Pts',(26.5582462470794,67.6869244353292,12.));
#162802=CARTESIAN_POINT('Ctrl Pts',(26.5410516013984,67.6684093805288,0.));
#162803=CARTESIAN_POINT('Ctrl Pts',(26.5410516013984,67.6684093805288,12.));
#162804=CARTESIAN_POINT('Ctrl Pts',(26.5239015052655,67.6499070648323,0.));
#162805=CARTESIAN_POINT('Ctrl Pts',(26.5239015052655,67.6499070648323,12.));
#162806=CARTESIAN_POINT('Ctrl Pts',(26.506795990273,67.6314176032823,0.));
#162807=CARTESIAN_POINT('Ctrl Pts',(26.506795990273,67.6314176032823,12.));
#162808=CARTESIAN_POINT('Ctrl Pts',(26.4897350880446,67.6129411113774,0.));
#162809=CARTESIAN_POINT('Ctrl Pts',(26.4897350880446,67.6129411113774,12.));
#162810=CARTESIAN_POINT('Ctrl Pts',(26.4727188302415,67.5944777050782,0.));
#162811=CARTESIAN_POINT('Ctrl Pts',(26.4727188302415,67.5944777050782,12.));
#162812=CARTESIAN_POINT('Ctrl Pts',(26.4557472485622,67.5760275008096,0.));
#162813=CARTESIAN_POINT('Ctrl Pts',(26.4557472485622,67.5760275008096,12.));
#162814=CARTESIAN_POINT('Ctrl Pts',(26.4388203747422,67.5575906154648,0.));
#162815=CARTESIAN_POINT('Ctrl Pts',(26.4388203747422,67.5575906154648,12.));
#162816=CARTESIAN_POINT('Ctrl Pts',(26.4219382405452,67.5391671664055,0.));
#162817=CARTESIAN_POINT('Ctrl Pts',(26.4219382405452,67.5391671664055,12.));
#162818=CARTESIAN_POINT('Ctrl Pts',(26.4051008777668,67.5207572714666,0.));
#162819=CARTESIAN_POINT('Ctrl Pts',(26.4051008777668,67.5207572714666,12.));
#162820=CARTESIAN_POINT('Ctrl Pts',(26.3883083182417,67.5023610489611,0.));
#162821=CARTESIAN_POINT('Ctrl Pts',(26.3883083182417,67.5023610489611,12.));
#162822=CARTESIAN_POINT('Ctrl Pts',(26.3715605938432,67.4839786176833,0.));
#162823=CARTESIAN_POINT('Ctrl Pts',(26.3715605938432,67.4839786176833,12.));
#162824=CARTESIAN_POINT('Ctrl Pts',(26.3548577364835,67.4656100969121,0.));
#162825=CARTESIAN_POINT('Ctrl Pts',(26.3548577364835,67.4656100969121,12.));
#162826=CARTESIAN_POINT('Ctrl Pts',(26.3381997781059,67.4472556064127,0.));
#162827=CARTESIAN_POINT('Ctrl Pts',(26.3381997781059,67.4472556064127,12.));
#162828=CARTESIAN_POINT('Ctrl Pts',(26.3215867506864,67.4289152664406,0.));
#162829=CARTESIAN_POINT('Ctrl Pts',(26.3215867506864,67.4289152664406,12.));
#162830=CARTESIAN_POINT('Ctrl Pts',(26.305018686241,67.4105891977465,0.));
#162831=CARTESIAN_POINT('Ctrl Pts',(26.305018686241,67.4105891977465,12.));
#162832=CARTESIAN_POINT('Ctrl Pts',(26.288495616827,67.392277521581,0.));
#162833=CARTESIAN_POINT('Ctrl Pts',(26.288495616827,67.392277521581,12.));
#162834=CARTESIAN_POINT('Ctrl Pts',(26.2720175745422,67.3739803596967,0.));
#162835=CARTESIAN_POINT('Ctrl Pts',(26.2720175745422,67.3739803596967,12.));
#162836=CARTESIAN_POINT('Ctrl Pts',(26.255584591518,67.3556978343506,0.));
#162837=CARTESIAN_POINT('Ctrl Pts',(26.255584591518,67.3556978343506,12.));
#162838=CARTESIAN_POINT('Ctrl Pts',(26.2391966999192,67.3374300683076,0.));
#162839=CARTESIAN_POINT('Ctrl Pts',(26.2391966999192,67.3374300683076,12.));
#162840=CARTESIAN_POINT('Ctrl Pts',(26.2228539319527,67.3191771848468,0.));
#162841=CARTESIAN_POINT('Ctrl Pts',(26.2228539319527,67.3191771848468,12.));
#162842=CARTESIAN_POINT('Ctrl Pts',(26.2065563198684,67.3009393077654,0.));
#162843=CARTESIAN_POINT('Ctrl Pts',(26.2065563198684,67.3009393077654,12.));
#162844=CARTESIAN_POINT('Ctrl Pts',(26.1903038959589,67.2827165613828,0.));
#162845=CARTESIAN_POINT('Ctrl Pts',(26.1903038959589,67.2827165613828,12.));
#162846=CARTESIAN_POINT('Ctrl Pts',(26.1740966925527,67.2645090705414,0.));
#162847=CARTESIAN_POINT('Ctrl Pts',(26.1740966925527,67.2645090705414,12.));
#162848=CARTESIAN_POINT('Ctrl Pts',(26.1579347420135,67.2463169606105,0.));
#162849=CARTESIAN_POINT('Ctrl Pts',(26.1579347420135,67.2463169606105,12.));
#162850=CARTESIAN_POINT('Ctrl Pts',(26.1418180767486,67.228140357493,0.));
#162851=CARTESIAN_POINT('Ctrl Pts',(26.1418180767486,67.228140357493,12.));
#162852=CARTESIAN_POINT('Ctrl Pts',(26.1257467292102,67.2099793876295,0.));
#162853=CARTESIAN_POINT('Ctrl Pts',(26.1257467292102,67.2099793876295,12.));
#162854=CARTESIAN_POINT('Ctrl Pts',(26.109720731895,67.191834178002,0.));
#162855=CARTESIAN_POINT('Ctrl Pts',(26.109720731895,67.191834178002,12.));
#162856=CARTESIAN_POINT('Ctrl Pts',(26.0937401173385,67.1737048561364,0.));
#162857=CARTESIAN_POINT('Ctrl Pts',(26.0937401173385,67.1737048561364,12.));
#162858=CARTESIAN_POINT('Ctrl Pts',(26.0778049181129,67.1555915501052,0.));
#162859=CARTESIAN_POINT('Ctrl Pts',(26.0778049181129,67.1555915501052,12.));
#162860=CARTESIAN_POINT('Ctrl Pts',(26.061915166836,67.1374943885353,0.));
#162861=CARTESIAN_POINT('Ctrl Pts',(26.061915166836,67.1374943885353,12.));
#162862=CARTESIAN_POINT('Ctrl Pts',(26.0460708961724,67.1194135006122,0.));
#162863=CARTESIAN_POINT('Ctrl Pts',(26.0460708961724,67.1194135006122,12.));
#162864=CARTESIAN_POINT('Ctrl Pts',(26.030272138834,67.101349016084,0.));
#162865=CARTESIAN_POINT('Ctrl Pts',(26.030272138834,67.101349016084,12.));
#162866=CARTESIAN_POINT('Ctrl Pts',(26.0145189275732,67.083301065264,0.));
#162867=CARTESIAN_POINT('Ctrl Pts',(26.0145189275732,67.083301065264,12.));
#162868=CARTESIAN_POINT('Ctrl Pts',(25.9988112951818,67.0652697790335,0.));
#162869=CARTESIAN_POINT('Ctrl Pts',(25.9988112951818,67.0652697790335,12.));
#162870=CARTESIAN_POINT('Ctrl Pts',(25.9831492744988,67.0472552888495,0.));
#162871=CARTESIAN_POINT('Ctrl Pts',(25.9831492744988,67.0472552888495,12.));
#162872=CARTESIAN_POINT('Ctrl Pts',(25.9675328984123,67.0292577267495,0.));
#162873=CARTESIAN_POINT('Ctrl Pts',(25.9675328984123,67.0292577267495,12.));
#162874=CARTESIAN_POINT('Ctrl Pts',(25.9519621998598,67.0112772253553,0.));
#162875=CARTESIAN_POINT('Ctrl Pts',(25.9519621998598,67.0112772253553,12.));
#162876=CARTESIAN_POINT('Ctrl Pts',(25.9364372118216,66.993313917876,0.));
#162877=CARTESIAN_POINT('Ctrl Pts',(25.9364372118216,66.993313917876,12.));
#162878=CARTESIAN_POINT('Ctrl Pts',(25.9209579673198,66.9753679381122,0.));
#162879=CARTESIAN_POINT('Ctrl Pts',(25.9209579673198,66.9753679381122,12.));
#162880=CARTESIAN_POINT('Ctrl Pts',(25.9055244994266,66.9574394204635,0.));
#162881=CARTESIAN_POINT('Ctrl Pts',(25.9055244994266,66.9574394204635,12.));
#162882=CARTESIAN_POINT('Ctrl Pts',(25.8901368412655,66.9395284999327,0.));
#162883=CARTESIAN_POINT('Ctrl Pts',(25.8901368412655,66.9395284999327,12.));
#162884=CARTESIAN_POINT('Ctrl Pts',(25.8747950260114,66.9216353121308,0.));
#162885=CARTESIAN_POINT('Ctrl Pts',(25.8747950260114,66.9216353121308,12.));
#162886=CARTESIAN_POINT('Ctrl Pts',(25.8594990868844,66.9037599932787,0.));
#162887=CARTESIAN_POINT('Ctrl Pts',(25.8594990868844,66.9037599932787,12.));
#162888=CARTESIAN_POINT('Ctrl Pts',(25.8442490571486,66.8859026802123,0.));
#162889=CARTESIAN_POINT('Ctrl Pts',(25.8442490571486,66.8859026802123,12.));
#162890=CARTESIAN_POINT('Ctrl Pts',(25.8290449701206,66.8680635103907,0.));
#162891=CARTESIAN_POINT('Ctrl Pts',(25.8290449701206,66.8680635103907,12.));
#162892=CARTESIAN_POINT('Ctrl Pts',(25.8138868591715,66.8502426219015,0.));
#162893=CARTESIAN_POINT('Ctrl Pts',(25.8138868591715,66.8502426219015,12.));
#162894=CARTESIAN_POINT('Ctrl Pts',(25.7987747577264,66.8324401534657,0.));
#162895=CARTESIAN_POINT('Ctrl Pts',(25.7987747577264,66.8324401534657,12.));
#162896=CARTESIAN_POINT('Ctrl Pts',(25.783708699258,66.8146562444397,0.));
#162897=CARTESIAN_POINT('Ctrl Pts',(25.783708699258,66.8146562444397,12.));
#162898=CARTESIAN_POINT('Ctrl Pts',(25.7686887172859,66.7968910348199,0.));
#162899=CARTESIAN_POINT('Ctrl Pts',(25.7686887172859,66.7968910348199,12.));
#162900=CARTESIAN_POINT('Ctrl Pts',(25.7537148453848,66.7791446652505,0.));
#162901=CARTESIAN_POINT('Ctrl Pts',(25.7537148453848,66.7791446652505,12.));
#162902=CARTESIAN_POINT('Ctrl Pts',(25.7387871171861,66.7614172770302,0.));
#162903=CARTESIAN_POINT('Ctrl Pts',(25.7387871171861,66.7614172770302,12.));
#162904=CARTESIAN_POINT('Ctrl Pts',(25.7239055663778,66.7437090121168,0.));
#162905=CARTESIAN_POINT('Ctrl Pts',(25.7239055663778,66.7437090121168,12.));
#162906=CARTESIAN_POINT('Ctrl Pts',(25.7090702266976,66.72602001313,0.));
#162907=CARTESIAN_POINT('Ctrl Pts',(25.7090702266976,66.72602001313,12.));
#162908=CARTESIAN_POINT('Ctrl Pts',(25.6942811319337,66.7083504233566,0.));
#162909=CARTESIAN_POINT('Ctrl Pts',(25.6942811319337,66.7083504233566,12.));
#162910=CARTESIAN_POINT('Ctrl Pts',(25.6795383159329,66.6907003867599,0.));
#162911=CARTESIAN_POINT('Ctrl Pts',(25.6795383159329,66.6907003867599,12.));
#162912=CARTESIAN_POINT('Ctrl Pts',(25.6648418126016,66.6730700479844,0.));
#162913=CARTESIAN_POINT('Ctrl Pts',(25.6648418126016,66.6730700479844,12.));
#162914=CARTESIAN_POINT('Ctrl Pts',(25.650191655905,66.6554595523611,0.));
#162915=CARTESIAN_POINT('Ctrl Pts',(25.650191655905,66.6554595523611,12.));
#162916=CARTESIAN_POINT('Ctrl Pts',(25.6355878798605,66.6378690459105,0.));
#162917=CARTESIAN_POINT('Ctrl Pts',(25.6355878798605,66.6378690459105,12.));
#162918=CARTESIAN_POINT('Ctrl Pts',(25.6210305185394,66.6202986753482,0.));
#162919=CARTESIAN_POINT('Ctrl Pts',(25.6210305185394,66.6202986753482,12.));
#162920=CARTESIAN_POINT('Ctrl Pts',(25.606519606075,66.6027485880947,0.));
#162921=CARTESIAN_POINT('Ctrl Pts',(25.606519606075,66.6027485880947,12.));
#162922=CARTESIAN_POINT('Ctrl Pts',(25.5920551766629,66.5852189322811,0.));
#162923=CARTESIAN_POINT('Ctrl Pts',(25.5920551766629,66.5852189322811,12.));
#162924=CARTESIAN_POINT('Ctrl Pts',(25.5776372645605,66.5677098567551,0.));
#162925=CARTESIAN_POINT('Ctrl Pts',(25.5776372645605,66.5677098567551,12.));
#162926=CARTESIAN_POINT('Ctrl Pts',(25.5632659040797,66.5502215110843,0.));
#162927=CARTESIAN_POINT('Ctrl Pts',(25.5632659040797,66.5502215110843,12.));
#162928=CARTESIAN_POINT('Ctrl Pts',(25.5489411295916,66.5327540455639,0.));
#162929=CARTESIAN_POINT('Ctrl Pts',(25.5489411295916,66.5327540455639,12.));
#162930=CARTESIAN_POINT('Ctrl Pts',(25.5346629755322,66.5153076112237,0.));
#162931=CARTESIAN_POINT('Ctrl Pts',(25.5346629755322,66.5153076112237,12.));
#162932=CARTESIAN_POINT('Ctrl Pts',(25.5204314764033,66.4978823598352,0.));
#162933=CARTESIAN_POINT('Ctrl Pts',(25.5204314764033,66.4978823598352,12.));
#162934=CARTESIAN_POINT('Ctrl Pts',(25.5062466667703,66.4804784439146,0.));
#162935=CARTESIAN_POINT('Ctrl Pts',(25.5062466667703,66.4804784439146,12.));
#162936=CARTESIAN_POINT('Ctrl Pts',(25.4921085812548,66.463096016725,0.));
#162937=CARTESIAN_POINT('Ctrl Pts',(25.4921085812548,66.463096016725,12.));
#162938=CARTESIAN_POINT('Ctrl Pts',(25.4780172545418,66.445735232287,0.));
#162939=CARTESIAN_POINT('Ctrl Pts',(25.4780172545418,66.445735232287,12.));
#162940=CARTESIAN_POINT('Ctrl Pts',(25.463972721385,66.4283962453899,0.));
#162941=CARTESIAN_POINT('Ctrl Pts',(25.463972721385,66.4283962453899,12.));
#162942=CARTESIAN_POINT('Ctrl Pts',(25.4499750166079,66.4110792116,0.));
#162943=CARTESIAN_POINT('Ctrl Pts',(25.4499750166079,66.4110792116,12.));
#162944=CARTESIAN_POINT('Ctrl Pts',(25.4360241751017,66.3937842872684,0.));
#162945=CARTESIAN_POINT('Ctrl Pts',(25.4360241751017,66.3937842872684,12.));
#162946=CARTESIAN_POINT('Ctrl Pts',(25.4221202318198,66.3765116295364,0.));
#162947=CARTESIAN_POINT('Ctrl Pts',(25.4221202318198,66.3765116295364,12.));
#162948=CARTESIAN_POINT('Ctrl Pts',(25.4082632217846,66.3592613963407,0.));
#162949=CARTESIAN_POINT('Ctrl Pts',(25.4082632217846,66.3592613963407,12.));
#162950=CARTESIAN_POINT('Ctrl Pts',(25.39445318009,66.3420337464176,0.));
#162951=CARTESIAN_POINT('Ctrl Pts',(25.39445318009,66.3420337464176,12.));
#162952=CARTESIAN_POINT('Ctrl Pts',(25.3806901419012,66.3248288393046,0.));
#162953=CARTESIAN_POINT('Ctrl Pts',(25.3806901419012,66.3248288393046,12.));
#162954=CARTESIAN_POINT('Ctrl Pts',(25.366974142449,66.3076468353417,0.));
#162955=CARTESIAN_POINT('Ctrl Pts',(25.366974142449,66.3076468353417,12.));
#162956=CARTESIAN_POINT('Ctrl Pts',(25.3533052170253,66.2904878956721,0.));
#162957=CARTESIAN_POINT('Ctrl Pts',(25.3533052170253,66.2904878956721,12.));
#162958=CARTESIAN_POINT('Ctrl Pts',(25.3396834009954,66.2733521822675,0.));
#162959=CARTESIAN_POINT('Ctrl Pts',(25.3396834009954,66.2733521822675,12.));
#162960=CARTESIAN_POINT('Ctrl Pts',(25.3261087298029,66.2562398579479,0.));
#162961=CARTESIAN_POINT('Ctrl Pts',(25.3261087298029,66.2562398579479,12.));
#162962=CARTESIAN_POINT('Ctrl Pts',(25.3125812389727,66.2391510863992,0.));
#162963=CARTESIAN_POINT('Ctrl Pts',(25.3125812389727,66.2391510863992,12.));
#162964=CARTESIAN_POINT('Ctrl Pts',(25.2991009641086,66.2220860321931,0.));
#162965=CARTESIAN_POINT('Ctrl Pts',(25.2991009641086,66.2220860321931,12.));
#162966=CARTESIAN_POINT('Ctrl Pts',(25.285667940892,66.2050448607883,0.));
#162967=CARTESIAN_POINT('Ctrl Pts',(25.285667940892,66.2050448607883,12.));
#162968=CARTESIAN_POINT('Ctrl Pts',(25.2722822050828,66.1880277385114,0.));
#162969=CARTESIAN_POINT('Ctrl Pts',(25.2722822050828,66.1880277385114,12.));
#162970=CARTESIAN_POINT('Ctrl Pts',(25.2589437925144,66.1710348325378,0.));
#162971=CARTESIAN_POINT('Ctrl Pts',(25.2589437925144,66.1710348325378,12.));
#162972=CARTESIAN_POINT('Ctrl Pts',(25.245652739088,66.1540663108767,0.));
#162973=CARTESIAN_POINT('Ctrl Pts',(25.245652739088,66.1540663108767,12.));
#162974=CARTESIAN_POINT('Ctrl Pts',(25.232409080756,66.1371223423372,0.));
#162975=CARTESIAN_POINT('Ctrl Pts',(25.232409080756,66.1371223423372,12.));
#162976=CARTESIAN_POINT('Ctrl Pts',(25.2192128535367,66.1202030965785,0.));
#162977=CARTESIAN_POINT('Ctrl Pts',(25.2192128535367,66.1202030965785,12.));
#162978=CARTESIAN_POINT('Ctrl Pts',(25.2060640935371,66.1033087441916,0.));
#162979=CARTESIAN_POINT('Ctrl Pts',(25.2060640935371,66.1033087441916,12.));
#162980=CARTESIAN_POINT('Ctrl Pts',(25.1929628369685,66.086439456768,0.));
#162981=CARTESIAN_POINT('Ctrl Pts',(25.1929628369685,66.086439456768,12.));
#162982=CARTESIAN_POINT('Ctrl Pts',(25.1799091201594,66.0695954069699,0.));
#162983=CARTESIAN_POINT('Ctrl Pts',(25.1799091201594,66.0695954069699,12.));
#162984=CARTESIAN_POINT('Ctrl Pts',(25.1669029795651,66.0527767686,0.));
#162985=CARTESIAN_POINT('Ctrl Pts',(25.1669029795651,66.0527767686,12.));
#162986=CARTESIAN_POINT('Ctrl Pts',(25.1539444517409,66.0359837164709,0.));
#162987=CARTESIAN_POINT('Ctrl Pts',(25.1539444517409,66.0359837164709,12.));
#162988=CARTESIAN_POINT('Ctrl Pts',(25.1410335733094,66.0192164262607,0.));
#162989=CARTESIAN_POINT('Ctrl Pts',(25.1410335733094,66.0192164262607,12.));
#162990=CARTESIAN_POINT('Ctrl Pts',(25.1281703809299,66.0024750743902,0.));
#162991=CARTESIAN_POINT('Ctrl Pts',(25.1281703809299,66.0024750743902,12.));
#162992=CARTESIAN_POINT('Ctrl Pts',(25.1153549112511,65.9857598378455,0.));
#162993=CARTESIAN_POINT('Ctrl Pts',(25.1153549112511,65.9857598378455,12.));
#162994=CARTESIAN_POINT('Ctrl Pts',(25.1025872009015,65.9690708941591,0.));
#162995=CARTESIAN_POINT('Ctrl Pts',(25.1025872009015,65.9690708941591,12.));
#162996=CARTESIAN_POINT('Ctrl Pts',(25.0898672865925,65.9524084218167,0.));
#162997=CARTESIAN_POINT('Ctrl Pts',(25.0898672865925,65.9524084218167,12.));
#162998=CARTESIAN_POINT('Ctrl Pts',(25.0771952052032,65.9357726006174,0.));
#162999=CARTESIAN_POINT('Ctrl Pts',(25.0771952052032,65.9357726006174,12.));
#163000=CARTESIAN_POINT('Ctrl Pts',(25.0645709938519,65.9191636119796,0.));
#163001=CARTESIAN_POINT('Ctrl Pts',(25.0645709938519,65.9191636119796,12.));
#163002=CARTESIAN_POINT('Ctrl Pts',(25.0519946900066,65.9025816394391,0.));
#163003=CARTESIAN_POINT('Ctrl Pts',(25.0519946900066,65.9025816394391,12.));
#163004=CARTESIAN_POINT('Ctrl Pts',(25.039466331404,65.8860268683088,0.));
#163005=CARTESIAN_POINT('Ctrl Pts',(25.039466331404,65.8860268683088,12.));
#163006=CARTESIAN_POINT('Ctrl Pts',(25.0269859558351,65.8694994847587,0.));
#163007=CARTESIAN_POINT('Ctrl Pts',(25.0269859558351,65.8694994847587,12.));
#163008=CARTESIAN_POINT('Ctrl Pts',(25.0145536009603,65.8529996750441,0.));
#163009=CARTESIAN_POINT('Ctrl Pts',(25.0145536009603,65.8529996750441,12.));
#163010=CARTESIAN_POINT('Ctrl Pts',(25.0021693041181,65.8365276247157,0.));
#163011=CARTESIAN_POINT('Ctrl Pts',(25.0021693041181,65.8365276247157,12.));
#163012=CARTESIAN_POINT('Ctrl Pts',(24.9898331021002,65.8200835177071,0.));
#163013=CARTESIAN_POINT('Ctrl Pts',(24.9898331021002,65.8200835177071,12.));
#163014=CARTESIAN_POINT('Ctrl Pts',(24.97754503157,65.8036675380761,0.));
#163015=CARTESIAN_POINT('Ctrl Pts',(24.97754503157,65.8036675380761,12.));
#163016=CARTESIAN_POINT('Ctrl Pts',(24.965305129559,65.7872798720847,0.));
#163017=CARTESIAN_POINT('Ctrl Pts',(24.965305129559,65.7872798720847,12.));
#163018=CARTESIAN_POINT('Ctrl Pts',(24.9531134338693,65.7709207098949,0.));
#163019=CARTESIAN_POINT('Ctrl Pts',(24.9531134338693,65.7709207098949,12.));
#163020=CARTESIAN_POINT('Ctrl Pts',(24.9409699836523,65.7545902480286,0.));
#163021=CARTESIAN_POINT('Ctrl Pts',(24.9409699836523,65.7545902480286,12.));
#163022=CARTESIAN_POINT('Ctrl Pts',(24.9288748194562,65.7382886895839,0.));
#163023=CARTESIAN_POINT('Ctrl Pts',(24.9288748194562,65.7382886895839,12.));
#163024=CARTESIAN_POINT('Ctrl Pts',(24.9168279820093,65.7220162391016,0.));
#163025=CARTESIAN_POINT('Ctrl Pts',(24.9168279820093,65.7220162391016,12.));
#163026=CARTESIAN_POINT('Ctrl Pts',(24.9048295111444,65.7057730980471,0.));
#163027=CARTESIAN_POINT('Ctrl Pts',(24.9048295111444,65.7057730980471,12.));
#163028=CARTESIAN_POINT('Ctrl Pts',(24.8928794448615,65.6895594608798,0.));
#163029=CARTESIAN_POINT('Ctrl Pts',(24.8928794448615,65.6895594608798,12.));
#163030=CARTESIAN_POINT('Ctrl Pts',(24.8809778178248,65.6733755087724,0.));
#163031=CARTESIAN_POINT('Ctrl Pts',(24.8809778178248,65.6733755087724,12.));
#163032=CARTESIAN_POINT('Ctrl Pts',(24.869124662808,65.6572214156761,0.));
#163033=CARTESIAN_POINT('Ctrl Pts',(24.869124662808,65.6572214156761,12.));
#163034=CARTESIAN_POINT('Ctrl Pts',(24.8573200135683,65.6410973603713,0.));
#163035=CARTESIAN_POINT('Ctrl Pts',(24.8573200135683,65.6410973603713,12.));
#163036=CARTESIAN_POINT('Ctrl Pts',(24.8455639071517,65.6250035361612,0.));
#163037=CARTESIAN_POINT('Ctrl Pts',(24.8455639071517,65.6250035361612,12.));
#163038=CARTESIAN_POINT('Ctrl Pts',(24.8338563866739,65.6089401625552,0.));
#163039=CARTESIAN_POINT('Ctrl Pts',(24.8338563866739,65.6089401625552,12.));
#163040=CARTESIAN_POINT('Ctrl Pts',(24.8221975032059,65.5929074932487,0.));
#163041=CARTESIAN_POINT('Ctrl Pts',(24.8221975032059,65.5929074932487,12.));
#163042=CARTESIAN_POINT('Ctrl Pts',(24.8105873098578,65.5769057914184,0.));
#163043=CARTESIAN_POINT('Ctrl Pts',(24.8105873098578,65.5769057914184,12.));
#163044=CARTESIAN_POINT('Ctrl Pts',(24.7990258561234,65.560935306275,0.));
#163045=CARTESIAN_POINT('Ctrl Pts',(24.7990258561234,65.560935306275,12.));
#163046=CARTESIAN_POINT('Ctrl Pts',(24.7875131827515,65.5449962514735,0.));
#163047=CARTESIAN_POINT('Ctrl Pts',(24.7875131827515,65.5449962514735,12.));
#163048=CARTESIAN_POINT('Ctrl Pts',(24.776049314855,65.5290887770494,0.));
#163049=CARTESIAN_POINT('Ctrl Pts',(24.776049314855,65.5290887770494,12.));
#163050=CARTESIAN_POINT('Ctrl Pts',(24.7646342620969,65.5132129675727,0.));
#163051=CARTESIAN_POINT('Ctrl Pts',(24.7646342620969,65.5132129675727,12.));
#163052=CARTESIAN_POINT('Ctrl Pts',(24.755541272477,65.5005376841469,0.));
#163053=CARTESIAN_POINT('Ctrl Pts',(24.755541272477,65.5005376841469,12.));
#163054=CARTESIAN_POINT('Ctrl Pts',(24.7487434956058,65.4910454936487,0.));
#163055=CARTESIAN_POINT('Ctrl Pts',(24.7487434956058,65.4910454936487,12.));
#163056=CARTESIAN_POINT('Ctrl Pts',(24.7442214063411,65.484723709553,0.));
#163057=CARTESIAN_POINT('Ctrl Pts',(24.7442214063411,65.484723709553,12.));
#163058=CARTESIAN_POINT('Ctrl Pts',(24.7419628022042,65.4815644032299,0.));
#163059=CARTESIAN_POINT('Ctrl Pts',(24.7419628022042,65.4815644032299,12.));
#163060=CARTESIAN_POINT('',(24.7419628022042,65.4815644032299,12.));
#163061=CARTESIAN_POINT('Ctrl Pts',(24.7419628022042,65.4815644032299,12.));
#163062=CARTESIAN_POINT('Ctrl Pts',(24.7442214063411,65.484723709553,12.));
#163063=CARTESIAN_POINT('Ctrl Pts',(24.7487434956058,65.4910454936487,12.));
#163064=CARTESIAN_POINT('Ctrl Pts',(24.755541272477,65.5005376841469,12.));
#163065=CARTESIAN_POINT('Ctrl Pts',(24.7646342620969,65.5132129675727,12.));
#163066=CARTESIAN_POINT('Ctrl Pts',(24.776049314855,65.5290887770494,12.));
#163067=CARTESIAN_POINT('Ctrl Pts',(24.7875131827515,65.5449962514735,12.));
#163068=CARTESIAN_POINT('Ctrl Pts',(24.7990258561234,65.560935306275,12.));
#163069=CARTESIAN_POINT('Ctrl Pts',(24.8105873098578,65.5769057914184,12.));
#163070=CARTESIAN_POINT('Ctrl Pts',(24.8221975032059,65.5929074932487,12.));
#163071=CARTESIAN_POINT('Ctrl Pts',(24.8338563866739,65.6089401625552,12.));
#163072=CARTESIAN_POINT('Ctrl Pts',(24.8455639071517,65.6250035361612,12.));
#163073=CARTESIAN_POINT('Ctrl Pts',(24.8573200135683,65.6410973603713,12.));
#163074=CARTESIAN_POINT('Ctrl Pts',(24.869124662808,65.6572214156761,12.));
#163075=CARTESIAN_POINT('Ctrl Pts',(24.8809778178248,65.6733755087724,12.));
#163076=CARTESIAN_POINT('Ctrl Pts',(24.8928794448615,65.6895594608798,12.));
#163077=CARTESIAN_POINT('Ctrl Pts',(24.9048295111444,65.7057730980471,12.));
#163078=CARTESIAN_POINT('Ctrl Pts',(24.9168279820093,65.7220162391016,12.));
#163079=CARTESIAN_POINT('Ctrl Pts',(24.9288748194562,65.7382886895839,12.));
#163080=CARTESIAN_POINT('Ctrl Pts',(24.9409699836523,65.7545902480286,12.));
#163081=CARTESIAN_POINT('Ctrl Pts',(24.9531134338693,65.7709207098949,12.));
#163082=CARTESIAN_POINT('Ctrl Pts',(24.965305129559,65.7872798720847,12.));
#163083=CARTESIAN_POINT('Ctrl Pts',(24.97754503157,65.8036675380761,12.));
#163084=CARTESIAN_POINT('Ctrl Pts',(24.9898331021002,65.8200835177071,12.));
#163085=CARTESIAN_POINT('Ctrl Pts',(25.0021693041181,65.8365276247157,12.));
#163086=CARTESIAN_POINT('Ctrl Pts',(25.0145536009603,65.8529996750441,12.));
#163087=CARTESIAN_POINT('Ctrl Pts',(25.0269859558351,65.8694994847587,12.));
#163088=CARTESIAN_POINT('Ctrl Pts',(25.039466331404,65.8860268683088,12.));
#163089=CARTESIAN_POINT('Ctrl Pts',(25.0519946900066,65.9025816394391,12.));
#163090=CARTESIAN_POINT('Ctrl Pts',(25.0645709938519,65.9191636119796,12.));
#163091=CARTESIAN_POINT('Ctrl Pts',(25.0771952052032,65.9357726006174,12.));
#163092=CARTESIAN_POINT('Ctrl Pts',(25.0898672865925,65.9524084218167,12.));
#163093=CARTESIAN_POINT('Ctrl Pts',(25.1025872009015,65.9690708941591,12.));
#163094=CARTESIAN_POINT('Ctrl Pts',(25.1153549112511,65.9857598378455,12.));
#163095=CARTESIAN_POINT('Ctrl Pts',(25.1281703809299,66.0024750743902,12.));
#163096=CARTESIAN_POINT('Ctrl Pts',(25.1410335733094,66.0192164262607,12.));
#163097=CARTESIAN_POINT('Ctrl Pts',(25.1539444517409,66.0359837164709,12.));
#163098=CARTESIAN_POINT('Ctrl Pts',(25.1669029795651,66.0527767686,12.));
#163099=CARTESIAN_POINT('Ctrl Pts',(25.1799091201594,66.0695954069699,12.));
#163100=CARTESIAN_POINT('Ctrl Pts',(25.1929628369685,66.086439456768,12.));
#163101=CARTESIAN_POINT('Ctrl Pts',(25.2060640935371,66.1033087441916,12.));
#163102=CARTESIAN_POINT('Ctrl Pts',(25.2192128535367,66.1202030965785,12.));
#163103=CARTESIAN_POINT('Ctrl Pts',(25.232409080756,66.1371223423372,12.));
#163104=CARTESIAN_POINT('Ctrl Pts',(25.245652739088,66.1540663108767,12.));
#163105=CARTESIAN_POINT('Ctrl Pts',(25.2589437925144,66.1710348325378,12.));
#163106=CARTESIAN_POINT('Ctrl Pts',(25.2722822050828,66.1880277385114,12.));
#163107=CARTESIAN_POINT('Ctrl Pts',(25.285667940892,66.2050448607883,12.));
#163108=CARTESIAN_POINT('Ctrl Pts',(25.2991009641086,66.2220860321931,12.));
#163109=CARTESIAN_POINT('Ctrl Pts',(25.3125812389727,66.2391510863992,12.));
#163110=CARTESIAN_POINT('Ctrl Pts',(25.3261087298029,66.2562398579479,12.));
#163111=CARTESIAN_POINT('Ctrl Pts',(25.3396834009954,66.2733521822675,12.));
#163112=CARTESIAN_POINT('Ctrl Pts',(25.3533052170253,66.2904878956721,12.));
#163113=CARTESIAN_POINT('Ctrl Pts',(25.366974142449,66.3076468353417,12.));
#163114=CARTESIAN_POINT('Ctrl Pts',(25.3806901419012,66.3248288393046,12.));
#163115=CARTESIAN_POINT('Ctrl Pts',(25.39445318009,66.3420337464176,12.));
#163116=CARTESIAN_POINT('Ctrl Pts',(25.4082632217846,66.3592613963407,12.));
#163117=CARTESIAN_POINT('Ctrl Pts',(25.4221202318198,66.3765116295364,12.));
#163118=CARTESIAN_POINT('Ctrl Pts',(25.4360241751017,66.3937842872684,12.));
#163119=CARTESIAN_POINT('Ctrl Pts',(25.4499750166079,66.4110792116,12.));
#163120=CARTESIAN_POINT('Ctrl Pts',(25.463972721385,66.4283962453899,12.));
#163121=CARTESIAN_POINT('Ctrl Pts',(25.4780172545418,66.445735232287,12.));
#163122=CARTESIAN_POINT('Ctrl Pts',(25.4921085812548,66.463096016725,12.));
#163123=CARTESIAN_POINT('Ctrl Pts',(25.5062466667703,66.4804784439146,12.));
#163124=CARTESIAN_POINT('Ctrl Pts',(25.5204314764033,66.4978823598352,12.));
#163125=CARTESIAN_POINT('Ctrl Pts',(25.5346629755322,66.5153076112237,12.));
#163126=CARTESIAN_POINT('Ctrl Pts',(25.5489411295916,66.5327540455639,12.));
#163127=CARTESIAN_POINT('Ctrl Pts',(25.5632659040797,66.5502215110843,12.));
#163128=CARTESIAN_POINT('Ctrl Pts',(25.5776372645605,66.5677098567551,12.));
#163129=CARTESIAN_POINT('Ctrl Pts',(25.5920551766629,66.5852189322811,12.));
#163130=CARTESIAN_POINT('Ctrl Pts',(25.606519606075,66.6027485880947,12.));
#163131=CARTESIAN_POINT('Ctrl Pts',(25.6210305185394,66.6202986753482,12.));
#163132=CARTESIAN_POINT('Ctrl Pts',(25.6355878798605,66.6378690459105,12.));
#163133=CARTESIAN_POINT('Ctrl Pts',(25.650191655905,66.6554595523611,12.));
#163134=CARTESIAN_POINT('Ctrl Pts',(25.6648418126016,66.6730700479844,12.));
#163135=CARTESIAN_POINT('Ctrl Pts',(25.6795383159329,66.6907003867599,12.));
#163136=CARTESIAN_POINT('Ctrl Pts',(25.6942811319337,66.7083504233566,12.));
#163137=CARTESIAN_POINT('Ctrl Pts',(25.7090702266976,66.72602001313,12.));
#163138=CARTESIAN_POINT('Ctrl Pts',(25.7239055663778,66.7437090121168,12.));
#163139=CARTESIAN_POINT('Ctrl Pts',(25.7387871171861,66.7614172770302,12.));
#163140=CARTESIAN_POINT('Ctrl Pts',(25.7537148453848,66.7791446652505,12.));
#163141=CARTESIAN_POINT('Ctrl Pts',(25.7686887172859,66.7968910348199,12.));
#163142=CARTESIAN_POINT('Ctrl Pts',(25.783708699258,66.8146562444397,12.));
#163143=CARTESIAN_POINT('Ctrl Pts',(25.7987747577264,66.8324401534657,12.));
#163144=CARTESIAN_POINT('Ctrl Pts',(25.8138868591715,66.8502426219015,12.));
#163145=CARTESIAN_POINT('Ctrl Pts',(25.8290449701206,66.8680635103907,12.));
#163146=CARTESIAN_POINT('Ctrl Pts',(25.8442490571486,66.8859026802123,12.));
#163147=CARTESIAN_POINT('Ctrl Pts',(25.8594990868844,66.9037599932787,12.));
#163148=CARTESIAN_POINT('Ctrl Pts',(25.8747950260114,66.9216353121308,12.));
#163149=CARTESIAN_POINT('Ctrl Pts',(25.8901368412655,66.9395284999327,12.));
#163150=CARTESIAN_POINT('Ctrl Pts',(25.9055244994266,66.9574394204635,12.));
#163151=CARTESIAN_POINT('Ctrl Pts',(25.9209579673198,66.9753679381122,12.));
#163152=CARTESIAN_POINT('Ctrl Pts',(25.9364372118216,66.993313917876,12.));
#163153=CARTESIAN_POINT('Ctrl Pts',(25.9519621998598,67.0112772253553,12.));
#163154=CARTESIAN_POINT('Ctrl Pts',(25.9675328984123,67.0292577267495,12.));
#163155=CARTESIAN_POINT('Ctrl Pts',(25.9831492744988,67.0472552888495,12.));
#163156=CARTESIAN_POINT('Ctrl Pts',(25.9988112951818,67.0652697790335,12.));
#163157=CARTESIAN_POINT('Ctrl Pts',(26.0145189275732,67.083301065264,12.));
#163158=CARTESIAN_POINT('Ctrl Pts',(26.030272138834,67.101349016084,12.));
#163159=CARTESIAN_POINT('Ctrl Pts',(26.0460708961724,67.1194135006122,12.));
#163160=CARTESIAN_POINT('Ctrl Pts',(26.061915166836,67.1374943885353,12.));
#163161=CARTESIAN_POINT('Ctrl Pts',(26.0778049181129,67.1555915501052,12.));
#163162=CARTESIAN_POINT('Ctrl Pts',(26.0937401173385,67.1737048561364,12.));
#163163=CARTESIAN_POINT('Ctrl Pts',(26.109720731895,67.191834178002,12.));
#163164=CARTESIAN_POINT('Ctrl Pts',(26.1257467292102,67.2099793876295,12.));
#163165=CARTESIAN_POINT('Ctrl Pts',(26.1418180767486,67.228140357493,12.));
#163166=CARTESIAN_POINT('Ctrl Pts',(26.1579347420135,67.2463169606105,12.));
#163167=CARTESIAN_POINT('Ctrl Pts',(26.1740966925527,67.2645090705414,12.));
#163168=CARTESIAN_POINT('Ctrl Pts',(26.1903038959589,67.2827165613828,12.));
#163169=CARTESIAN_POINT('Ctrl Pts',(26.2065563198684,67.3009393077654,12.));
#163170=CARTESIAN_POINT('Ctrl Pts',(26.2228539319527,67.3191771848468,12.));
#163171=CARTESIAN_POINT('Ctrl Pts',(26.2391966999192,67.3374300683076,12.));
#163172=CARTESIAN_POINT('Ctrl Pts',(26.255584591518,67.3556978343506,12.));
#163173=CARTESIAN_POINT('Ctrl Pts',(26.2720175745422,67.3739803596967,12.));
#163174=CARTESIAN_POINT('Ctrl Pts',(26.288495616827,67.392277521581,12.));
#163175=CARTESIAN_POINT('Ctrl Pts',(26.305018686241,67.4105891977465,12.));
#163176=CARTESIAN_POINT('Ctrl Pts',(26.3215867506864,67.4289152664406,12.));
#163177=CARTESIAN_POINT('Ctrl Pts',(26.3381997781059,67.4472556064127,12.));
#163178=CARTESIAN_POINT('Ctrl Pts',(26.3548577364835,67.4656100969121,12.));
#163179=CARTESIAN_POINT('Ctrl Pts',(26.3715605938432,67.4839786176833,12.));
#163180=CARTESIAN_POINT('Ctrl Pts',(26.3883083182417,67.5023610489611,12.));
#163181=CARTESIAN_POINT('Ctrl Pts',(26.4051008777668,67.5207572714666,12.));
#163182=CARTESIAN_POINT('Ctrl Pts',(26.4219382405452,67.5391671664055,12.));
#163183=CARTESIAN_POINT('Ctrl Pts',(26.4388203747422,67.5575906154648,12.));
#163184=CARTESIAN_POINT('Ctrl Pts',(26.4557472485622,67.5760275008096,12.));
#163185=CARTESIAN_POINT('Ctrl Pts',(26.4727188302415,67.5944777050782,12.));
#163186=CARTESIAN_POINT('Ctrl Pts',(26.4897350880446,67.6129411113774,12.));
#163187=CARTESIAN_POINT('Ctrl Pts',(26.506795990273,67.6314176032823,12.));
#163188=CARTESIAN_POINT('Ctrl Pts',(26.5239015052655,67.6499070648323,12.));
#163189=CARTESIAN_POINT('Ctrl Pts',(26.5410516013984,67.6684093805288,12.));
#163190=CARTESIAN_POINT('Ctrl Pts',(26.5582462470794,67.6869244353292,12.));
#163191=CARTESIAN_POINT('Ctrl Pts',(26.5754854107422,67.7054521146427,12.));
#163192=CARTESIAN_POINT('Ctrl Pts',(26.5927690608546,67.7239923043295,12.));
#163193=CARTESIAN_POINT('Ctrl Pts',(26.6100971659204,67.7425448906983,12.));
#163194=CARTESIAN_POINT('Ctrl Pts',(26.6274696944793,67.7611097605042,12.));
#163195=CARTESIAN_POINT('Ctrl Pts',(26.6448866151027,67.7796868009447,12.));
#163196=CARTESIAN_POINT('Ctrl Pts',(26.6623478963867,67.7982758996557,12.));
#163197=CARTESIAN_POINT('Ctrl Pts',(26.6798535069586,67.8168769447086,12.));
#163198=CARTESIAN_POINT('Ctrl Pts',(26.6974034154802,67.8354898246079,12.));
#163199=CARTESIAN_POINT('Ctrl Pts',(26.7149975906478,67.8541144282875,12.));
#163200=CARTESIAN_POINT('Ctrl Pts',(26.7326360011886,67.8727506451068,12.));
#163201=CARTESIAN_POINT('Ctrl Pts',(26.7503186158523,67.8913983648441,12.));
#163202=CARTESIAN_POINT('Ctrl Pts',(26.7680454034168,67.9100574776974,12.));
#163203=CARTESIAN_POINT('Ctrl Pts',(26.7858163326932,67.9287278742839,12.));
#163204=CARTESIAN_POINT('Ctrl Pts',(26.8036313725262,67.9474094456395,12.));
#163205=CARTESIAN_POINT('Ctrl Pts',(26.8214904917921,67.9661020832165,12.));
#163206=CARTESIAN_POINT('Ctrl Pts',(26.8393936593914,67.9848056788814,12.));
#163207=CARTESIAN_POINT('Ctrl Pts',(26.85734084425,68.0035201249108,12.));
#163208=CARTESIAN_POINT('Ctrl Pts',(26.8753320153255,68.0222453139862,12.));
#163209=CARTESIAN_POINT('Ctrl Pts',(26.8933671416064,68.0409811391872,12.));
#163210=CARTESIAN_POINT('Ctrl Pts',(26.9114461921108,68.0597274939857,12.));
#163211=CARTESIAN_POINT('Ctrl Pts',(26.9295691358775,68.0784842722362,12.));
#163212=CARTESIAN_POINT('Ctrl Pts',(26.9477359419646,68.0972513681739,12.));
#163213=CARTESIAN_POINT('Ctrl Pts',(26.9659465794596,68.1160286764244,12.));
#163214=CARTESIAN_POINT('Ctrl Pts',(26.9842010174818,68.13481609201,12.));
#163215=CARTESIAN_POINT('Ctrl Pts',(27.0024992251839,68.1536135103558,12.));
#163216=CARTESIAN_POINT('Ctrl Pts',(27.0208411717477,68.1724208272967,12.));
#163217=CARTESIAN_POINT('Ctrl Pts',(27.0392268263804,68.1912379390787,12.));
#163218=CARTESIAN_POINT('Ctrl Pts',(27.0576561583179,68.2100647423345,12.));
#163219=CARTESIAN_POINT('Ctrl Pts',(27.076129136823,68.2289011340624,12.));
#163220=CARTESIAN_POINT('Ctrl Pts',(27.0946457311813,68.2477470116014,12.));
#163221=CARTESIAN_POINT('Ctrl Pts',(27.1132059106938,68.2666022726094,12.));
#163222=CARTESIAN_POINT('Ctrl Pts',(27.1318096446643,68.285466815035,12.));
#163223=CARTESIAN_POINT('Ctrl Pts',(27.150456902413,68.3043405371589,12.));
#163224=CARTESIAN_POINT('Ctrl Pts',(27.1691476532917,68.3232233376415,12.));
#163225=CARTESIAN_POINT('Ctrl Pts',(27.1878818666925,68.3421151155708,12.));
#163226=CARTESIAN_POINT('Ctrl Pts',(27.2066595120544,68.3610157704999,12.));
#163227=CARTESIAN_POINT('Ctrl Pts',(27.2254805588677,68.379925202511,12.));
#163228=CARTESIAN_POINT('Ctrl Pts',(27.2443449766654,68.398843312159,12.));
#163229=CARTESIAN_POINT('Ctrl Pts',(27.2632527350062,68.4177700003471,12.));
#163230=CARTESIAN_POINT('Ctrl Pts',(27.2822038034539,68.4367051682166,12.));
#163231=CARTESIAN_POINT('Ctrl Pts',(27.301198151557,68.455648717044,12.));
#163232=CARTESIAN_POINT('Ctrl Pts',(27.3202357488153,68.4746005480993,12.));
#163233=CARTESIAN_POINT('Ctrl Pts',(27.3393165646748,68.4935605626362,12.));
#163234=CARTESIAN_POINT('Ctrl Pts',(27.3584405685941,68.5125286621888,12.));
#163235=CARTESIAN_POINT('Ctrl Pts',(27.3776077300914,68.5315047488035,12.));
#163236=CARTESIAN_POINT('Ctrl Pts',(27.3968180187941,68.5504887252975,12.));
#163237=CARTESIAN_POINT('Ctrl Pts',(27.4160714044831,68.5694804955014,12.));
#163238=CARTESIAN_POINT('Ctrl Pts',(27.435367857136,68.5884799645218,12.));
#163239=CARTESIAN_POINT('Ctrl Pts',(27.4547073468226,68.6074870381619,12.));
#163240=CARTESIAN_POINT('Ctrl Pts',(27.4740898435988,68.6265016223561,12.));
#163241=CARTESIAN_POINT('Ctrl Pts',(27.4935153173868,68.645523622548,12.));
#163242=CARTESIAN_POINT('Ctrl Pts',(27.5129837378791,68.6645529432045,12.));
#163243=CARTESIAN_POINT('Ctrl Pts',(27.5324950743706,68.6835894869882,12.));
#163244=CARTESIAN_POINT('Ctrl Pts',(27.5520492958906,68.7026331554296,12.));
#163245=CARTESIAN_POINT('Ctrl Pts',(27.5716463715004,68.7216838504218,12.));
#163246=CARTESIAN_POINT('Ctrl Pts',(27.5912862705468,68.740741475526,12.));
#163247=CARTESIAN_POINT('Ctrl Pts',(27.6109689629029,68.7598059372129,12.));
#163248=CARTESIAN_POINT('Ctrl Pts',(27.6306944192737,68.7788771464713,12.));
#163249=CARTESIAN_POINT('Ctrl Pts',(27.6504626112666,68.7979550191872,12.));
#163250=CARTESIAN_POINT('Ctrl Pts',(27.6674443909983,68.8143140938915,12.));
#163251=CARTESIAN_POINT('Ctrl Pts',(27.6804870323433,68.8268597852179,12.));
#163252=CARTESIAN_POINT('Ctrl Pts',(27.6895716271274,68.8355891982106,12.));
#163253=CARTESIAN_POINT('Ctrl Pts',(27.6946856803717,68.8405004466159,12.));
#163254=CARTESIAN_POINT('Ctrl Pts',(27.6958230985043,68.8415926175084,12.));
#163255=CARTESIAN_POINT('',(24.7419628022042,65.4815644032299,0.));
#163256=CARTESIAN_POINT('',(24.7419628022042,65.4815644032299,0.));
#163257=CARTESIAN_POINT('Ctrl Pts',(27.6958230985043,68.8415926175085,0.));
#163258=CARTESIAN_POINT('Ctrl Pts',(27.6946856803717,68.8405004466159,0.));
#163259=CARTESIAN_POINT('Ctrl Pts',(27.6895716271274,68.8355891982106,0.));
#163260=CARTESIAN_POINT('Ctrl Pts',(27.6804870323433,68.8268597852179,0.));
#163261=CARTESIAN_POINT('Ctrl Pts',(27.6674443909983,68.8143140938915,0.));
#163262=CARTESIAN_POINT('Ctrl Pts',(27.6504626112666,68.7979550191872,0.));
#163263=CARTESIAN_POINT('Ctrl Pts',(27.6306944192737,68.7788771464713,0.));
#163264=CARTESIAN_POINT('Ctrl Pts',(27.6109689629029,68.7598059372129,0.));
#163265=CARTESIAN_POINT('Ctrl Pts',(27.5912862705468,68.740741475526,0.));
#163266=CARTESIAN_POINT('Ctrl Pts',(27.5716463715004,68.7216838504218,0.));
#163267=CARTESIAN_POINT('Ctrl Pts',(27.5520492958906,68.7026331554296,0.));
#163268=CARTESIAN_POINT('Ctrl Pts',(27.5324950743706,68.6835894869882,0.));
#163269=CARTESIAN_POINT('Ctrl Pts',(27.5129837378791,68.6645529432045,0.));
#163270=CARTESIAN_POINT('Ctrl Pts',(27.4935153173868,68.645523622548,0.));
#163271=CARTESIAN_POINT('Ctrl Pts',(27.4740898435988,68.6265016223561,0.));
#163272=CARTESIAN_POINT('Ctrl Pts',(27.4547073468226,68.6074870381619,0.));
#163273=CARTESIAN_POINT('Ctrl Pts',(27.435367857136,68.5884799645218,0.));
#163274=CARTESIAN_POINT('Ctrl Pts',(27.4160714044831,68.5694804955014,0.));
#163275=CARTESIAN_POINT('Ctrl Pts',(27.3968180187941,68.5504887252975,0.));
#163276=CARTESIAN_POINT('Ctrl Pts',(27.3776077300914,68.5315047488035,0.));
#163277=CARTESIAN_POINT('Ctrl Pts',(27.3584405685941,68.5125286621888,0.));
#163278=CARTESIAN_POINT('Ctrl Pts',(27.3393165646748,68.4935605626362,0.));
#163279=CARTESIAN_POINT('Ctrl Pts',(27.3202357488153,68.4746005480993,0.));
#163280=CARTESIAN_POINT('Ctrl Pts',(27.301198151557,68.455648717044,0.));
#163281=CARTESIAN_POINT('Ctrl Pts',(27.2822038034539,68.4367051682166,0.));
#163282=CARTESIAN_POINT('Ctrl Pts',(27.2632527350062,68.4177700003471,0.));
#163283=CARTESIAN_POINT('Ctrl Pts',(27.2443449766654,68.398843312159,0.));
#163284=CARTESIAN_POINT('Ctrl Pts',(27.2254805588677,68.379925202511,0.));
#163285=CARTESIAN_POINT('Ctrl Pts',(27.2066595120544,68.3610157704999,0.));
#163286=CARTESIAN_POINT('Ctrl Pts',(27.1878818666925,68.3421151155708,0.));
#163287=CARTESIAN_POINT('Ctrl Pts',(27.1691476532917,68.3232233376415,0.));
#163288=CARTESIAN_POINT('Ctrl Pts',(27.150456902413,68.3043405371589,0.));
#163289=CARTESIAN_POINT('Ctrl Pts',(27.1318096446643,68.285466815035,0.));
#163290=CARTESIAN_POINT('Ctrl Pts',(27.1132059106938,68.2666022726094,0.));
#163291=CARTESIAN_POINT('Ctrl Pts',(27.0946457311813,68.2477470116014,0.));
#163292=CARTESIAN_POINT('Ctrl Pts',(27.076129136823,68.2289011340624,0.));
#163293=CARTESIAN_POINT('Ctrl Pts',(27.0576561583179,68.2100647423345,0.));
#163294=CARTESIAN_POINT('Ctrl Pts',(27.0392268263804,68.1912379390787,0.));
#163295=CARTESIAN_POINT('Ctrl Pts',(27.0208411717477,68.1724208272967,0.));
#163296=CARTESIAN_POINT('Ctrl Pts',(27.0024992251839,68.1536135103558,0.));
#163297=CARTESIAN_POINT('Ctrl Pts',(26.9842010174818,68.13481609201,0.));
#163298=CARTESIAN_POINT('Ctrl Pts',(26.9659465794596,68.1160286764244,0.));
#163299=CARTESIAN_POINT('Ctrl Pts',(26.9477359419646,68.0972513681739,0.));
#163300=CARTESIAN_POINT('Ctrl Pts',(26.9295691358775,68.0784842722362,0.));
#163301=CARTESIAN_POINT('Ctrl Pts',(26.9114461921108,68.0597274939857,0.));
#163302=CARTESIAN_POINT('Ctrl Pts',(26.8933671416064,68.0409811391872,0.));
#163303=CARTESIAN_POINT('Ctrl Pts',(26.8753320153255,68.0222453139862,0.));
#163304=CARTESIAN_POINT('Ctrl Pts',(26.85734084425,68.0035201249108,0.));
#163305=CARTESIAN_POINT('Ctrl Pts',(26.8393936593914,67.9848056788814,0.));
#163306=CARTESIAN_POINT('Ctrl Pts',(26.8214904917921,67.9661020832165,0.));
#163307=CARTESIAN_POINT('Ctrl Pts',(26.8036313725262,67.9474094456395,0.));
#163308=CARTESIAN_POINT('Ctrl Pts',(26.7858163326932,67.9287278742839,0.));
#163309=CARTESIAN_POINT('Ctrl Pts',(26.7680454034168,67.9100574776974,0.));
#163310=CARTESIAN_POINT('Ctrl Pts',(26.7503186158523,67.8913983648441,0.));
#163311=CARTESIAN_POINT('Ctrl Pts',(26.7326360011886,67.8727506451068,0.));
#163312=CARTESIAN_POINT('Ctrl Pts',(26.7149975906478,67.8541144282875,0.));
#163313=CARTESIAN_POINT('Ctrl Pts',(26.6974034154802,67.8354898246079,0.));
#163314=CARTESIAN_POINT('Ctrl Pts',(26.6798535069586,67.8168769447086,0.));
#163315=CARTESIAN_POINT('Ctrl Pts',(26.6623478963867,67.7982758996557,0.));
#163316=CARTESIAN_POINT('Ctrl Pts',(26.6448866151027,67.7796868009447,0.));
#163317=CARTESIAN_POINT('Ctrl Pts',(26.6274696944793,67.7611097605042,0.));
#163318=CARTESIAN_POINT('Ctrl Pts',(26.6100971659204,67.7425448906983,0.));
#163319=CARTESIAN_POINT('Ctrl Pts',(26.5927690608546,67.7239923043295,0.));
#163320=CARTESIAN_POINT('Ctrl Pts',(26.5754854107422,67.7054521146427,0.));
#163321=CARTESIAN_POINT('Ctrl Pts',(26.5582462470794,67.6869244353292,0.));
#163322=CARTESIAN_POINT('Ctrl Pts',(26.5410516013984,67.6684093805288,0.));
#163323=CARTESIAN_POINT('Ctrl Pts',(26.5239015052655,67.6499070648323,0.));
#163324=CARTESIAN_POINT('Ctrl Pts',(26.506795990273,67.6314176032823,0.));
#163325=CARTESIAN_POINT('Ctrl Pts',(26.4897350880446,67.6129411113774,0.));
#163326=CARTESIAN_POINT('Ctrl Pts',(26.4727188302415,67.5944777050782,0.));
#163327=CARTESIAN_POINT('Ctrl Pts',(26.4557472485622,67.5760275008096,0.));
#163328=CARTESIAN_POINT('Ctrl Pts',(26.4388203747422,67.5575906154648,0.));
#163329=CARTESIAN_POINT('Ctrl Pts',(26.4219382405452,67.5391671664055,0.));
#163330=CARTESIAN_POINT('Ctrl Pts',(26.4051008777668,67.5207572714666,0.));
#163331=CARTESIAN_POINT('Ctrl Pts',(26.3883083182417,67.5023610489611,0.));
#163332=CARTESIAN_POINT('Ctrl Pts',(26.3715605938432,67.4839786176833,0.));
#163333=CARTESIAN_POINT('Ctrl Pts',(26.3548577364835,67.4656100969121,0.));
#163334=CARTESIAN_POINT('Ctrl Pts',(26.3381997781059,67.4472556064127,0.));
#163335=CARTESIAN_POINT('Ctrl Pts',(26.3215867506864,67.4289152664406,0.));
#163336=CARTESIAN_POINT('Ctrl Pts',(26.305018686241,67.4105891977465,0.));
#163337=CARTESIAN_POINT('Ctrl Pts',(26.288495616827,67.392277521581,0.));
#163338=CARTESIAN_POINT('Ctrl Pts',(26.2720175745422,67.3739803596967,0.));
#163339=CARTESIAN_POINT('Ctrl Pts',(26.255584591518,67.3556978343506,0.));
#163340=CARTESIAN_POINT('Ctrl Pts',(26.2391966999192,67.3374300683076,0.));
#163341=CARTESIAN_POINT('Ctrl Pts',(26.2228539319527,67.3191771848468,0.));
#163342=CARTESIAN_POINT('Ctrl Pts',(26.2065563198684,67.3009393077654,0.));
#163343=CARTESIAN_POINT('Ctrl Pts',(26.1903038959589,67.2827165613828,0.));
#163344=CARTESIAN_POINT('Ctrl Pts',(26.1740966925527,67.2645090705414,0.));
#163345=CARTESIAN_POINT('Ctrl Pts',(26.1579347420135,67.2463169606105,0.));
#163346=CARTESIAN_POINT('Ctrl Pts',(26.1418180767486,67.228140357493,0.));
#163347=CARTESIAN_POINT('Ctrl Pts',(26.1257467292102,67.2099793876295,0.));
#163348=CARTESIAN_POINT('Ctrl Pts',(26.109720731895,67.191834178002,0.));
#163349=CARTESIAN_POINT('Ctrl Pts',(26.0937401173385,67.1737048561364,0.));
#163350=CARTESIAN_POINT('Ctrl Pts',(26.0778049181129,67.1555915501052,0.));
#163351=CARTESIAN_POINT('Ctrl Pts',(26.061915166836,67.1374943885353,0.));
#163352=CARTESIAN_POINT('Ctrl Pts',(26.0460708961724,67.1194135006122,0.));
#163353=CARTESIAN_POINT('Ctrl Pts',(26.030272138834,67.101349016084,0.));
#163354=CARTESIAN_POINT('Ctrl Pts',(26.0145189275732,67.083301065264,0.));
#163355=CARTESIAN_POINT('Ctrl Pts',(25.9988112951818,67.0652697790335,0.));
#163356=CARTESIAN_POINT('Ctrl Pts',(25.9831492744988,67.0472552888495,0.));
#163357=CARTESIAN_POINT('Ctrl Pts',(25.9675328984123,67.0292577267495,0.));
#163358=CARTESIAN_POINT('Ctrl Pts',(25.9519621998598,67.0112772253553,0.));
#163359=CARTESIAN_POINT('Ctrl Pts',(25.9364372118216,66.993313917876,0.));
#163360=CARTESIAN_POINT('Ctrl Pts',(25.9209579673198,66.9753679381122,0.));
#163361=CARTESIAN_POINT('Ctrl Pts',(25.9055244994266,66.9574394204635,0.));
#163362=CARTESIAN_POINT('Ctrl Pts',(25.8901368412655,66.9395284999327,0.));
#163363=CARTESIAN_POINT('Ctrl Pts',(25.8747950260114,66.9216353121308,0.));
#163364=CARTESIAN_POINT('Ctrl Pts',(25.8594990868844,66.9037599932787,0.));
#163365=CARTESIAN_POINT('Ctrl Pts',(25.8442490571486,66.8859026802123,0.));
#163366=CARTESIAN_POINT('Ctrl Pts',(25.8290449701206,66.8680635103907,0.));
#163367=CARTESIAN_POINT('Ctrl Pts',(25.8138868591715,66.8502426219015,0.));
#163368=CARTESIAN_POINT('Ctrl Pts',(25.7987747577264,66.8324401534657,0.));
#163369=CARTESIAN_POINT('Ctrl Pts',(25.783708699258,66.8146562444397,0.));
#163370=CARTESIAN_POINT('Ctrl Pts',(25.7686887172859,66.7968910348199,0.));
#163371=CARTESIAN_POINT('Ctrl Pts',(25.7537148453848,66.7791446652505,0.));
#163372=CARTESIAN_POINT('Ctrl Pts',(25.7387871171861,66.7614172770302,0.));
#163373=CARTESIAN_POINT('Ctrl Pts',(25.7239055663778,66.7437090121168,0.));
#163374=CARTESIAN_POINT('Ctrl Pts',(25.7090702266976,66.72602001313,0.));
#163375=CARTESIAN_POINT('Ctrl Pts',(25.6942811319337,66.7083504233566,0.));
#163376=CARTESIAN_POINT('Ctrl Pts',(25.6795383159329,66.6907003867599,0.));
#163377=CARTESIAN_POINT('Ctrl Pts',(25.6648418126016,66.6730700479844,0.));
#163378=CARTESIAN_POINT('Ctrl Pts',(25.650191655905,66.6554595523611,0.));
#163379=CARTESIAN_POINT('Ctrl Pts',(25.6355878798605,66.6378690459105,0.));
#163380=CARTESIAN_POINT('Ctrl Pts',(25.6210305185394,66.6202986753482,0.));
#163381=CARTESIAN_POINT('Ctrl Pts',(25.606519606075,66.6027485880947,0.));
#163382=CARTESIAN_POINT('Ctrl Pts',(25.5920551766629,66.5852189322811,0.));
#163383=CARTESIAN_POINT('Ctrl Pts',(25.5776372645605,66.5677098567551,0.));
#163384=CARTESIAN_POINT('Ctrl Pts',(25.5632659040797,66.5502215110843,0.));
#163385=CARTESIAN_POINT('Ctrl Pts',(25.5489411295916,66.5327540455639,0.));
#163386=CARTESIAN_POINT('Ctrl Pts',(25.5346629755322,66.5153076112237,0.));
#163387=CARTESIAN_POINT('Ctrl Pts',(25.5204314764033,66.4978823598352,0.));
#163388=CARTESIAN_POINT('Ctrl Pts',(25.5062466667703,66.4804784439146,0.));
#163389=CARTESIAN_POINT('Ctrl Pts',(25.4921085812548,66.463096016725,0.));
#163390=CARTESIAN_POINT('Ctrl Pts',(25.4780172545418,66.445735232287,0.));
#163391=CARTESIAN_POINT('Ctrl Pts',(25.463972721385,66.4283962453899,0.));
#163392=CARTESIAN_POINT('Ctrl Pts',(25.4499750166079,66.4110792116,0.));
#163393=CARTESIAN_POINT('Ctrl Pts',(25.4360241751017,66.3937842872684,0.));
#163394=CARTESIAN_POINT('Ctrl Pts',(25.4221202318198,66.3765116295364,0.));
#163395=CARTESIAN_POINT('Ctrl Pts',(25.4082632217846,66.3592613963407,0.));
#163396=CARTESIAN_POINT('Ctrl Pts',(25.39445318009,66.3420337464176,0.));
#163397=CARTESIAN_POINT('Ctrl Pts',(25.3806901419012,66.3248288393046,0.));
#163398=CARTESIAN_POINT('Ctrl Pts',(25.366974142449,66.3076468353417,0.));
#163399=CARTESIAN_POINT('Ctrl Pts',(25.3533052170253,66.2904878956721,0.));
#163400=CARTESIAN_POINT('Ctrl Pts',(25.3396834009954,66.2733521822675,0.));
#163401=CARTESIAN_POINT('Ctrl Pts',(25.3261087298029,66.2562398579479,0.));
#163402=CARTESIAN_POINT('Ctrl Pts',(25.3125812389727,66.2391510863992,0.));
#163403=CARTESIAN_POINT('Ctrl Pts',(25.2991009641086,66.2220860321931,0.));
#163404=CARTESIAN_POINT('Ctrl Pts',(25.285667940892,66.2050448607883,0.));
#163405=CARTESIAN_POINT('Ctrl Pts',(25.2722822050828,66.1880277385114,0.));
#163406=CARTESIAN_POINT('Ctrl Pts',(25.2589437925144,66.1710348325378,0.));
#163407=CARTESIAN_POINT('Ctrl Pts',(25.245652739088,66.1540663108767,0.));
#163408=CARTESIAN_POINT('Ctrl Pts',(25.232409080756,66.1371223423372,0.));
#163409=CARTESIAN_POINT('Ctrl Pts',(25.2192128535367,66.1202030965785,0.));
#163410=CARTESIAN_POINT('Ctrl Pts',(25.2060640935371,66.1033087441916,0.));
#163411=CARTESIAN_POINT('Ctrl Pts',(25.1929628369685,66.086439456768,0.));
#163412=CARTESIAN_POINT('Ctrl Pts',(25.1799091201594,66.0695954069699,0.));
#163413=CARTESIAN_POINT('Ctrl Pts',(25.1669029795651,66.0527767686,0.));
#163414=CARTESIAN_POINT('Ctrl Pts',(25.1539444517409,66.0359837164709,0.));
#163415=CARTESIAN_POINT('Ctrl Pts',(25.1410335733094,66.0192164262607,0.));
#163416=CARTESIAN_POINT('Ctrl Pts',(25.1281703809299,66.0024750743902,0.));
#163417=CARTESIAN_POINT('Ctrl Pts',(25.1153549112511,65.9857598378455,0.));
#163418=CARTESIAN_POINT('Ctrl Pts',(25.1025872009015,65.9690708941591,0.));
#163419=CARTESIAN_POINT('Ctrl Pts',(25.0898672865925,65.9524084218167,0.));
#163420=CARTESIAN_POINT('Ctrl Pts',(25.0771952052032,65.9357726006174,0.));
#163421=CARTESIAN_POINT('Ctrl Pts',(25.0645709938519,65.9191636119796,0.));
#163422=CARTESIAN_POINT('Ctrl Pts',(25.0519946900066,65.9025816394391,0.));
#163423=CARTESIAN_POINT('Ctrl Pts',(25.039466331404,65.8860268683088,0.));
#163424=CARTESIAN_POINT('Ctrl Pts',(25.0269859558351,65.8694994847587,0.));
#163425=CARTESIAN_POINT('Ctrl Pts',(25.0145536009603,65.8529996750441,0.));
#163426=CARTESIAN_POINT('Ctrl Pts',(25.0021693041181,65.8365276247157,0.));
#163427=CARTESIAN_POINT('Ctrl Pts',(24.9898331021002,65.8200835177071,0.));
#163428=CARTESIAN_POINT('Ctrl Pts',(24.97754503157,65.8036675380761,0.));
#163429=CARTESIAN_POINT('Ctrl Pts',(24.965305129559,65.7872798720847,0.));
#163430=CARTESIAN_POINT('Ctrl Pts',(24.9531134338693,65.7709207098949,0.));
#163431=CARTESIAN_POINT('Ctrl Pts',(24.9409699836523,65.7545902480286,0.));
#163432=CARTESIAN_POINT('Ctrl Pts',(24.9288748194562,65.7382886895839,0.));
#163433=CARTESIAN_POINT('Ctrl Pts',(24.9168279820093,65.7220162391016,0.));
#163434=CARTESIAN_POINT('Ctrl Pts',(24.9048295111444,65.7057730980471,0.));
#163435=CARTESIAN_POINT('Ctrl Pts',(24.8928794448615,65.6895594608798,0.));
#163436=CARTESIAN_POINT('Ctrl Pts',(24.8809778178248,65.6733755087724,0.));
#163437=CARTESIAN_POINT('Ctrl Pts',(24.869124662808,65.6572214156761,0.));
#163438=CARTESIAN_POINT('Ctrl Pts',(24.8573200135683,65.6410973603713,0.));
#163439=CARTESIAN_POINT('Ctrl Pts',(24.8455639071517,65.6250035361612,0.));
#163440=CARTESIAN_POINT('Ctrl Pts',(24.8338563866739,65.6089401625552,0.));
#163441=CARTESIAN_POINT('Ctrl Pts',(24.8221975032059,65.5929074932487,0.));
#163442=CARTESIAN_POINT('Ctrl Pts',(24.8105873098578,65.5769057914184,0.));
#163443=CARTESIAN_POINT('Ctrl Pts',(24.7990258561234,65.560935306275,0.));
#163444=CARTESIAN_POINT('Ctrl Pts',(24.7875131827515,65.5449962514735,0.));
#163445=CARTESIAN_POINT('Ctrl Pts',(24.776049314855,65.5290887770494,0.));
#163446=CARTESIAN_POINT('Ctrl Pts',(24.7646342620969,65.5132129675727,0.));
#163447=CARTESIAN_POINT('Ctrl Pts',(24.755541272477,65.5005376841469,0.));
#163448=CARTESIAN_POINT('Ctrl Pts',(24.7487434956058,65.4910454936487,0.));
#163449=CARTESIAN_POINT('Ctrl Pts',(24.7442214063411,65.484723709553,0.));
#163450=CARTESIAN_POINT('Ctrl Pts',(24.7419628022042,65.4815644032299,0.));
#163451=CARTESIAN_POINT('Ctrl Pts',(33.8448817269567,66.3684712863594,0.));
#163452=CARTESIAN_POINT('Ctrl Pts',(33.8448817269567,66.3684712863594,12.));
#163453=CARTESIAN_POINT('Ctrl Pts',(33.8404862618869,66.3650082659713,0.));
#163454=CARTESIAN_POINT('Ctrl Pts',(33.8404862618869,66.3650082659713,12.));
#163455=CARTESIAN_POINT('Ctrl Pts',(33.8316996011932,66.3580824155893,0.));
#163456=CARTESIAN_POINT('Ctrl Pts',(33.8316996011932,66.3580824155893,12.));
#163457=CARTESIAN_POINT('Ctrl Pts',(33.8185324184903,66.3476942112,0.));
#163458=CARTESIAN_POINT('Ctrl Pts',(33.8185324184903,66.3476942112,12.));
#163459=CARTESIAN_POINT('Ctrl Pts',(33.8010017926027,66.3338444144211,0.));
#163460=CARTESIAN_POINT('Ctrl Pts',(33.8010017926027,66.3338444144211,12.));
#163461=CARTESIAN_POINT('Ctrl Pts',(33.7791312145108,66.3165340771611,0.));
#163462=CARTESIAN_POINT('Ctrl Pts',(33.7791312145108,66.3165340771611,12.));
#163463=CARTESIAN_POINT('Ctrl Pts',(33.7573033544559,66.2992256621336,0.));
#163464=CARTESIAN_POINT('Ctrl Pts',(33.7573033544559,66.2992256621336,12.));
#163465=CARTESIAN_POINT('Ctrl Pts',(33.7355182321907,66.2819191962353,0.));
#163466=CARTESIAN_POINT('Ctrl Pts',(33.7355182321907,66.2819191962353,12.));
#163467=CARTESIAN_POINT('Ctrl Pts',(33.7137758735902,66.2646147235322,0.));
#163468=CARTESIAN_POINT('Ctrl Pts',(33.7137758735902,66.2646147235322,12.));
#163469=CARTESIAN_POINT('Ctrl Pts',(33.6920763111448,66.2473123109395,0.));
#163470=CARTESIAN_POINT('Ctrl Pts',(33.6920763111448,66.2473123109395,12.));
#163471=CARTESIAN_POINT('Ctrl Pts',(33.6704195830392,66.2300120464082,0.));
#163472=CARTESIAN_POINT('Ctrl Pts',(33.6704195830392,66.2300120464082,12.));
#163473=CARTESIAN_POINT('Ctrl Pts',(33.6488057311532,66.2127140313598,0.));
#163474=CARTESIAN_POINT('Ctrl Pts',(33.6488057311532,66.2127140313598,12.));
#163475=CARTESIAN_POINT('Ctrl Pts',(33.6272347993476,66.1954183747089,0.));
#163476=CARTESIAN_POINT('Ctrl Pts',(33.6272347993476,66.1954183747089,12.));
#163477=CARTESIAN_POINT('Ctrl Pts',(33.6057068316769,66.1781251864017,0.));
#163478=CARTESIAN_POINT('Ctrl Pts',(33.6057068316769,66.1781251864017,12.));
#163479=CARTESIAN_POINT('Ctrl Pts',(33.584221870515,66.1608345707637,0.));
#163480=CARTESIAN_POINT('Ctrl Pts',(33.584221870515,66.1608345707637,12.));
#163481=CARTESIAN_POINT('Ctrl Pts',(33.5627799550483,66.1435466211076,0.));
#163482=CARTESIAN_POINT('Ctrl Pts',(33.5627799550483,66.1435466211076,12.));
#163483=CARTESIAN_POINT('Ctrl Pts',(33.541381122345,66.1262614234674,0.));
#163484=CARTESIAN_POINT('Ctrl Pts',(33.541381122345,66.1262614234674,12.));
#163485=CARTESIAN_POINT('Ctrl Pts',(33.5200254081243,66.1089790592729,0.));
#163486=CARTESIAN_POINT('Ctrl Pts',(33.5200254081243,66.1089790592729,12.));
#163487=CARTESIAN_POINT('Ctrl Pts',(33.4987128476622,66.0916996085245,0.));
#163488=CARTESIAN_POINT('Ctrl Pts',(33.4987128476622,66.0916996085245,12.));
#163489=CARTESIAN_POINT('Ctrl Pts',(33.4774434765745,66.0744231525415,0.));
#163490=CARTESIAN_POINT('Ctrl Pts',(33.4774434765745,66.0744231525415,12.));
#163491=CARTESIAN_POINT('Ctrl Pts',(33.4562173318025,66.0571497774434,0.));
#163492=CARTESIAN_POINT('Ctrl Pts',(33.4562173318025,66.0571497774434,12.));
#163493=CARTESIAN_POINT('Ctrl Pts',(33.43503445151,66.0398795737777,0.));
#163494=CARTESIAN_POINT('Ctrl Pts',(33.43503445151,66.0398795737777,12.));
#163495=CARTESIAN_POINT('Ctrl Pts',(33.4138948746388,66.0226126349446,0.));
#163496=CARTESIAN_POINT('Ctrl Pts',(33.4138948746388,66.0226126349446,12.));
#163497=CARTESIAN_POINT('Ctrl Pts',(33.3927986405605,66.0053490559812,0.));
#163498=CARTESIAN_POINT('Ctrl Pts',(33.3927986405605,66.0053490559812,12.));
#163499=CARTESIAN_POINT('Ctrl Pts',(33.37174578871,65.9880889322831,0.));
#163500=CARTESIAN_POINT('Ctrl Pts',(33.37174578871,65.9880889322831,12.));
#163501=CARTESIAN_POINT('Ctrl Pts',(33.3507363581592,65.970832358141,0.));
#163502=CARTESIAN_POINT('Ctrl Pts',(33.3507363581592,65.970832358141,12.));
#163503=CARTESIAN_POINT('Ctrl Pts',(33.3297703874265,65.9535794260831,0.));
#163504=CARTESIAN_POINT('Ctrl Pts',(33.3297703874265,65.9535794260831,12.));
#163505=CARTESIAN_POINT('Ctrl Pts',(33.3088479147164,65.9363302276846,0.));
#163506=CARTESIAN_POINT('Ctrl Pts',(33.3088479147164,65.9363302276846,12.));
#163507=CARTESIAN_POINT('Ctrl Pts',(33.2879689780572,65.9190848540433,0.));
#163508=CARTESIAN_POINT('Ctrl Pts',(33.2879689780572,65.9190848540433,12.));
#163509=CARTESIAN_POINT('Ctrl Pts',(33.2671336154753,65.9018433963889,0.));
#163510=CARTESIAN_POINT('Ctrl Pts',(33.2671336154753,65.9018433963889,12.));
#163511=CARTESIAN_POINT('Ctrl Pts',(33.2463418651492,65.8846059466372,0.));
#163512=CARTESIAN_POINT('Ctrl Pts',(33.2463418651492,65.8846059466372,12.));
#163513=CARTESIAN_POINT('Ctrl Pts',(33.2255937655649,65.8673725979578,0.));
#163514=CARTESIAN_POINT('Ctrl Pts',(33.2255937655649,65.8673725979578,12.));
#163515=CARTESIAN_POINT('Ctrl Pts',(33.2048893554491,65.8501434445164,0.));
#163516=CARTESIAN_POINT('Ctrl Pts',(33.2048893554491,65.8501434445164,12.));
#163517=CARTESIAN_POINT('Ctrl Pts',(33.1842286737051,65.8329185812375,0.));
#163518=CARTESIAN_POINT('Ctrl Pts',(33.1842286737051,65.8329185812375,12.));
#163519=CARTESIAN_POINT('Ctrl Pts',(33.16361175934,65.8156981035503,0.));
#163520=CARTESIAN_POINT('Ctrl Pts',(33.16361175934,65.8156981035503,12.));
#163521=CARTESIAN_POINT('Ctrl Pts',(33.1430386513976,65.7984821071623,0.));
#163522=CARTESIAN_POINT('Ctrl Pts',(33.1430386513976,65.7984821071623,12.));
#163523=CARTESIAN_POINT('Ctrl Pts',(33.1225093888672,65.7812706877697,0.));
#163524=CARTESIAN_POINT('Ctrl Pts',(33.1225093888672,65.7812706877697,12.));
#163525=CARTESIAN_POINT('Ctrl Pts',(33.1020240106884,65.7640639410661,0.));
#163526=CARTESIAN_POINT('Ctrl Pts',(33.1020240106884,65.7640639410661,12.));
#163527=CARTESIAN_POINT('Ctrl Pts',(33.081582555798,65.7468619628816,0.));
#163528=CARTESIAN_POINT('Ctrl Pts',(33.081582555798,65.7468619628816,12.));
#163529=CARTESIAN_POINT('Ctrl Pts',(33.0611850631582,65.7296648492825,0.));
#163530=CARTESIAN_POINT('Ctrl Pts',(33.0611850631582,65.7296648492825,12.));
#163531=CARTESIAN_POINT('Ctrl Pts',(33.0408315717873,65.7124726966802,0.));
#163532=CARTESIAN_POINT('Ctrl Pts',(33.0408315717873,65.7124726966802,12.));
#163533=CARTESIAN_POINT('Ctrl Pts',(33.0205221207873,65.6952856019533,0.));
#163534=CARTESIAN_POINT('Ctrl Pts',(33.0205221207873,65.6952856019533,12.));
#163535=CARTESIAN_POINT('Ctrl Pts',(33.0002567493573,65.6781036625027,0.));
#163536=CARTESIAN_POINT('Ctrl Pts',(33.0002567493573,65.6781036625027,12.));
#163537=CARTESIAN_POINT('Ctrl Pts',(32.980035496784,65.6609269761889,0.));
#163538=CARTESIAN_POINT('Ctrl Pts',(32.980035496784,65.6609269761889,12.));
#163539=CARTESIAN_POINT('Ctrl Pts',(32.9598584024312,65.6437556412947,0.));
#163540=CARTESIAN_POINT('Ctrl Pts',(32.9598584024312,65.6437556412947,12.));
#163541=CARTESIAN_POINT('Ctrl Pts',(32.9397255057274,65.6265897564783,0.));
#163542=CARTESIAN_POINT('Ctrl Pts',(32.9397255057274,65.6265897564783,12.));
#163543=CARTESIAN_POINT('Ctrl Pts',(32.9196368461463,65.6094294207276,0.));
#163544=CARTESIAN_POINT('Ctrl Pts',(32.9196368461463,65.6094294207276,12.));
#163545=CARTESIAN_POINT('Ctrl Pts',(32.8995924631898,65.5922747333194,0.));
#163546=CARTESIAN_POINT('Ctrl Pts',(32.8995924631898,65.5922747333194,12.));
#163547=CARTESIAN_POINT('Ctrl Pts',(32.879592396403,65.5751257938473,0.));
#163548=CARTESIAN_POINT('Ctrl Pts',(32.879592396403,65.5751257938473,12.));
#163549=CARTESIAN_POINT('Ctrl Pts',(32.8596366853832,65.5579827022421,0.));
#163550=CARTESIAN_POINT('Ctrl Pts',(32.8596366853832,65.5579827022421,12.));
#163551=CARTESIAN_POINT('Ctrl Pts',(32.8397253697865,65.5408455587965,0.));
#163552=CARTESIAN_POINT('Ctrl Pts',(32.8397253697865,65.5408455587965,12.));
#163553=CARTESIAN_POINT('Ctrl Pts',(32.8198584893315,65.5237144641858,0.));
#163554=CARTESIAN_POINT('Ctrl Pts',(32.8198584893315,65.5237144641858,12.));
#163555=CARTESIAN_POINT('Ctrl Pts',(32.8000360837975,65.5065895194928,0.));
#163556=CARTESIAN_POINT('Ctrl Pts',(32.8000360837975,65.5065895194928,12.));
#163557=CARTESIAN_POINT('Ctrl Pts',(32.7802581930287,65.4894708262061,0.));
#163558=CARTESIAN_POINT('Ctrl Pts',(32.7802581930287,65.4894708262061,12.));
#163559=CARTESIAN_POINT('Ctrl Pts',(32.7605248569378,65.4723584862122,0.));
#163560=CARTESIAN_POINT('Ctrl Pts',(32.7605248569378,65.4723584862122,12.));
#163561=CARTESIAN_POINT('Ctrl Pts',(32.7408361155037,65.4552526017905,0.));
#163562=CARTESIAN_POINT('Ctrl Pts',(32.7408361155037,65.4552526017905,12.));
#163563=CARTESIAN_POINT('Ctrl Pts',(32.7211920087684,65.4381532756065,0.));
#163564=CARTESIAN_POINT('Ctrl Pts',(32.7211920087684,65.4381532756065,12.));
#163565=CARTESIAN_POINT('Ctrl Pts',(32.7015925768265,65.4210606107035,0.));
#163566=CARTESIAN_POINT('Ctrl Pts',(32.7015925768265,65.4210606107035,12.));
#163567=CARTESIAN_POINT('Ctrl Pts',(32.6820378598267,65.4039747105038,0.));
#163568=CARTESIAN_POINT('Ctrl Pts',(32.6820378598267,65.4039747105038,12.));
#163569=CARTESIAN_POINT('Ctrl Pts',(32.662527897981,65.3868956788182,0.));
#163570=CARTESIAN_POINT('Ctrl Pts',(32.662527897981,65.3868956788182,12.));
#163571=CARTESIAN_POINT('Ctrl Pts',(32.6430627315674,65.3698236198513,0.));
#163572=CARTESIAN_POINT('Ctrl Pts',(32.6430627315674,65.3698236198513,12.));
#163573=CARTESIAN_POINT('Ctrl Pts',(32.6236424009301,65.3527586382081,0.));
#163574=CARTESIAN_POINT('Ctrl Pts',(32.6236424009301,65.3527586382081,12.));
#163575=CARTESIAN_POINT('Ctrl Pts',(32.6042669464751,65.3357008389004,0.));
#163576=CARTESIAN_POINT('Ctrl Pts',(32.6042669464751,65.3357008389004,12.));
#163577=CARTESIAN_POINT('Ctrl Pts',(32.5849364086678,65.31865032735,0.));
#163578=CARTESIAN_POINT('Ctrl Pts',(32.5849364086678,65.31865032735,12.));
#163579=CARTESIAN_POINT('Ctrl Pts',(32.5656508280421,65.3016072093912,0.));
#163580=CARTESIAN_POINT('Ctrl Pts',(32.5656508280421,65.3016072093912,12.));
#163581=CARTESIAN_POINT('Ctrl Pts',(32.5464102452014,65.2845715912721,0.));
#163582=CARTESIAN_POINT('Ctrl Pts',(32.5464102452014,65.2845715912721,12.));
#163583=CARTESIAN_POINT('Ctrl Pts',(32.5272147008191,65.2675435796558,0.));
#163584=CARTESIAN_POINT('Ctrl Pts',(32.5272147008191,65.2675435796558,12.));
#163585=CARTESIAN_POINT('Ctrl Pts',(32.5080642356328,65.2505232816209,0.));
#163586=CARTESIAN_POINT('Ctrl Pts',(32.5080642356328,65.2505232816209,12.));
#163587=CARTESIAN_POINT('Ctrl Pts',(32.4889588904392,65.2335108046614,0.));
#163588=CARTESIAN_POINT('Ctrl Pts',(32.4889588904392,65.2335108046614,12.));
#163589=CARTESIAN_POINT('Ctrl Pts',(32.4698987061032,65.2165062566924,0.));
#163590=CARTESIAN_POINT('Ctrl Pts',(32.4698987061032,65.2165062566924,12.));
#163591=CARTESIAN_POINT('Ctrl Pts',(32.450883723561,65.1995097460538,0.));
#163592=CARTESIAN_POINT('Ctrl Pts',(32.450883723561,65.1995097460538,12.));
#163593=CARTESIAN_POINT('Ctrl Pts',(32.4319139838212,65.182521381514,0.));
#163594=CARTESIAN_POINT('Ctrl Pts',(32.4319139838212,65.182521381514,12.));
#163595=CARTESIAN_POINT('Ctrl Pts',(32.4129895279615,65.1655412722726,0.));
#163596=CARTESIAN_POINT('Ctrl Pts',(32.4129895279615,65.1655412722726,12.));
#163597=CARTESIAN_POINT('Ctrl Pts',(32.3941103971221,65.1485695279635,0.));
#163598=CARTESIAN_POINT('Ctrl Pts',(32.3941103971221,65.1485695279635,12.));
#163599=CARTESIAN_POINT('Ctrl Pts',(32.3752766325136,65.1316062586588,0.));
#163600=CARTESIAN_POINT('Ctrl Pts',(32.3752766325136,65.1316062586588,12.));
#163601=CARTESIAN_POINT('Ctrl Pts',(32.3564882754212,65.1146515748722,0.));
#163602=CARTESIAN_POINT('Ctrl Pts',(32.3564882754212,65.1146515748722,12.));
#163603=CARTESIAN_POINT('Ctrl Pts',(32.3377453672051,65.0977055875608,0.));
#163604=CARTESIAN_POINT('Ctrl Pts',(32.3377453672051,65.0977055875608,12.));
#163605=CARTESIAN_POINT('Ctrl Pts',(32.3190479492987,65.0807684081282,0.));
#163606=CARTESIAN_POINT('Ctrl Pts',(32.3190479492987,65.0807684081282,12.));
#163607=CARTESIAN_POINT('Ctrl Pts',(32.3003960632006,65.0638401484257,0.));
#163608=CARTESIAN_POINT('Ctrl Pts',(32.3003960632006,65.0638401484257,12.));
#163609=CARTESIAN_POINT('Ctrl Pts',(32.2817897504807,65.0469209207563,0.));
#163610=CARTESIAN_POINT('Ctrl Pts',(32.2817897504807,65.0469209207563,12.));
#163611=CARTESIAN_POINT('Ctrl Pts',(32.2632290527862,65.03001083788,0.));
#163612=CARTESIAN_POINT('Ctrl Pts',(32.2632290527862,65.03001083788,12.));
#163613=CARTESIAN_POINT('Ctrl Pts',(32.2447140118422,65.0131100130158,0.));
#163614=CARTESIAN_POINT('Ctrl Pts',(32.2447140118422,65.0131100130158,12.));
#163615=CARTESIAN_POINT('Ctrl Pts',(32.2262446694512,64.9962185598462,0.));
#163616=CARTESIAN_POINT('Ctrl Pts',(32.2262446694512,64.9962185598462,12.));
#163617=CARTESIAN_POINT('Ctrl Pts',(32.207821067485,64.9793365925178,0.));
#163618=CARTESIAN_POINT('Ctrl Pts',(32.207821067485,64.9793365925178,12.));
#163619=CARTESIAN_POINT('Ctrl Pts',(32.189443247888,64.9624642256461,0.));
#163620=CARTESIAN_POINT('Ctrl Pts',(32.189443247888,64.9624642256461,12.));
#163621=CARTESIAN_POINT('Ctrl Pts',(32.1711112526854,64.9456015743193,0.));
#163622=CARTESIAN_POINT('Ctrl Pts',(32.1711112526854,64.9456015743193,12.));
#163623=CARTESIAN_POINT('Ctrl Pts',(32.152825123983,64.9287487541015,0.));
#163624=CARTESIAN_POINT('Ctrl Pts',(32.152825123983,64.9287487541015,12.));
#163625=CARTESIAN_POINT('Ctrl Pts',(32.1345849039674,64.9119058810367,0.));
#163626=CARTESIAN_POINT('Ctrl Pts',(32.1345849039674,64.9119058810367,12.));
#163627=CARTESIAN_POINT('Ctrl Pts',(32.1163906348983,64.8950730716501,0.));
#163628=CARTESIAN_POINT('Ctrl Pts',(32.1163906348983,64.8950730716501,12.));
#163629=CARTESIAN_POINT('Ctrl Pts',(32.0982423591112,64.8782504429527,0.));
#163630=CARTESIAN_POINT('Ctrl Pts',(32.0982423591112,64.8782504429527,12.));
#163631=CARTESIAN_POINT('Ctrl Pts',(32.0801401190244,64.8614381124455,0.));
#163632=CARTESIAN_POINT('Ctrl Pts',(32.0801401190244,64.8614381124455,12.));
#163633=CARTESIAN_POINT('Ctrl Pts',(32.0620839571409,64.8446361981234,0.));
#163634=CARTESIAN_POINT('Ctrl Pts',(32.0620839571409,64.8446361981234,12.));
#163635=CARTESIAN_POINT('Ctrl Pts',(32.0440739160476,64.8278448184785,0.));
#163636=CARTESIAN_POINT('Ctrl Pts',(32.0440739160476,64.8278448184785,12.));
#163637=CARTESIAN_POINT('Ctrl Pts',(32.0261100384092,64.811064092502,0.));
#163638=CARTESIAN_POINT('Ctrl Pts',(32.0261100384092,64.811064092502,12.));
#163639=CARTESIAN_POINT('Ctrl Pts',(32.0081923669677,64.7942941396883,0.));
#163640=CARTESIAN_POINT('Ctrl Pts',(32.0081923669677,64.7942941396883,12.));
#163641=CARTESIAN_POINT('Ctrl Pts',(31.9903209445521,64.7775350800404,0.));
#163642=CARTESIAN_POINT('Ctrl Pts',(31.9903209445521,64.7775350800404,12.));
#163643=CARTESIAN_POINT('Ctrl Pts',(31.972495814079,64.7607870340738,0.));
#163644=CARTESIAN_POINT('Ctrl Pts',(31.972495814079,64.7607870340738,12.));
#163645=CARTESIAN_POINT('Ctrl Pts',(31.9547170185533,64.7440501228201,0.));
#163646=CARTESIAN_POINT('Ctrl Pts',(31.9547170185533,64.7440501228201,12.));
#163647=CARTESIAN_POINT('Ctrl Pts',(31.9369846010613,64.727324467829,0.));
#163648=CARTESIAN_POINT('Ctrl Pts',(31.9369846010613,64.727324467829,12.));
#163649=CARTESIAN_POINT('Ctrl Pts',(31.9192986047702,64.7106101911723,0.));
#163650=CARTESIAN_POINT('Ctrl Pts',(31.9192986047702,64.7106101911723,12.));
#163651=CARTESIAN_POINT('Ctrl Pts',(31.9016590729371,64.6939074154491,0.));
#163652=CARTESIAN_POINT('Ctrl Pts',(31.9016590729371,64.6939074154491,12.));
#163653=CARTESIAN_POINT('Ctrl Pts',(31.8840660489106,64.6772162637905,0.));
#163654=CARTESIAN_POINT('Ctrl Pts',(31.8840660489106,64.6772162637905,12.));
#163655=CARTESIAN_POINT('Ctrl Pts',(31.8665195761312,64.6605368598631,0.));
#163656=CARTESIAN_POINT('Ctrl Pts',(31.8665195761312,64.6605368598631,12.));
#163657=CARTESIAN_POINT('Ctrl Pts',(31.849019698125,64.6438693278718,0.));
#163658=CARTESIAN_POINT('Ctrl Pts',(31.849019698125,64.6438693278718,12.));
#163659=CARTESIAN_POINT('Ctrl Pts',(31.8315664585027,64.627213792563,0.));
#163660=CARTESIAN_POINT('Ctrl Pts',(31.8315664585027,64.627213792563,12.));
#163661=CARTESIAN_POINT('Ctrl Pts',(31.8141599009684,64.6105703792311,0.));
#163662=CARTESIAN_POINT('Ctrl Pts',(31.8141599009684,64.6105703792311,12.));
#163663=CARTESIAN_POINT('Ctrl Pts',(31.7968000693218,64.5939392137233,0.));
#163664=CARTESIAN_POINT('Ctrl Pts',(31.7968000693218,64.5939392137233,12.));
#163665=CARTESIAN_POINT('Ctrl Pts',(31.7794870074583,64.5773204224429,0.));
#163666=CARTESIAN_POINT('Ctrl Pts',(31.7794870074583,64.5773204224429,12.));
#163667=CARTESIAN_POINT('Ctrl Pts',(31.7622207593637,64.5607141323527,0.));
#163668=CARTESIAN_POINT('Ctrl Pts',(31.7622207593637,64.5607141323527,12.));
#163669=CARTESIAN_POINT('Ctrl Pts',(31.7450013691117,64.544120470978,0.));
#163670=CARTESIAN_POINT('Ctrl Pts',(31.7450013691117,64.544120470978,12.));
#163671=CARTESIAN_POINT('Ctrl Pts',(31.7278288808736,64.5275395664134,0.));
#163672=CARTESIAN_POINT('Ctrl Pts',(31.7278288808736,64.5275395664134,12.));
#163673=CARTESIAN_POINT('Ctrl Pts',(31.7107033389204,64.5109715473277,0.));
#163674=CARTESIAN_POINT('Ctrl Pts',(31.7107033389204,64.5109715473277,12.));
#163675=CARTESIAN_POINT('Ctrl Pts',(31.6936247876228,64.4944165429672,0.));
#163676=CARTESIAN_POINT('Ctrl Pts',(31.6936247876228,64.4944165429672,12.));
#163677=CARTESIAN_POINT('Ctrl Pts',(31.6765932714456,64.4778746831598,0.));
#163678=CARTESIAN_POINT('Ctrl Pts',(31.6765932714456,64.4778746831598,12.));
#163679=CARTESIAN_POINT('Ctrl Pts',(31.6596088349468,64.4613460983186,0.));
#163680=CARTESIAN_POINT('Ctrl Pts',(31.6596088349468,64.4613460983186,12.));
#163681=CARTESIAN_POINT('Ctrl Pts',(31.6426715227865,64.4448309194499,0.));
#163682=CARTESIAN_POINT('Ctrl Pts',(31.6426715227865,64.4448309194499,12.));
#163683=CARTESIAN_POINT('Ctrl Pts',(31.6257813797281,64.4283292781553,0.));
#163684=CARTESIAN_POINT('Ctrl Pts',(31.6257813797281,64.4283292781553,12.));
#163685=CARTESIAN_POINT('Ctrl Pts',(31.6089384506399,64.4118413066386,0.));
#163686=CARTESIAN_POINT('Ctrl Pts',(31.6089384506399,64.4118413066386,12.));
#163687=CARTESIAN_POINT('Ctrl Pts',(31.5921427804879,64.3953671377071,0.));
#163688=CARTESIAN_POINT('Ctrl Pts',(31.5921427804879,64.3953671377071,12.));
#163689=CARTESIAN_POINT('Ctrl Pts',(31.5753944143355,64.3789069047768,0.));
#163690=CARTESIAN_POINT('Ctrl Pts',(31.5753944143355,64.3789069047768,12.));
#163691=CARTESIAN_POINT('Ctrl Pts',(31.5586933973531,64.3624607418798,0.));
#163692=CARTESIAN_POINT('Ctrl Pts',(31.5586933973531,64.3624607418798,12.));
#163693=CARTESIAN_POINT('Ctrl Pts',(31.5420397748198,64.34602878367,0.));
#163694=CARTESIAN_POINT('Ctrl Pts',(31.5420397748198,64.34602878367,12.));
#163695=CARTESIAN_POINT('Ctrl Pts',(31.5254335921239,64.3296111654273,0.));
#163696=CARTESIAN_POINT('Ctrl Pts',(31.5254335921239,64.3296111654273,12.));
#163697=CARTESIAN_POINT('Ctrl Pts',(31.5088748947565,64.3132080230603,0.));
#163698=CARTESIAN_POINT('Ctrl Pts',(31.5088748947565,64.3132080230603,12.));
#163699=CARTESIAN_POINT('Ctrl Pts',(31.4923637283109,64.2968194931113,0.));
#163700=CARTESIAN_POINT('Ctrl Pts',(31.4923637283109,64.2968194931113,12.));
#163701=CARTESIAN_POINT('Ctrl Pts',(31.4759001384922,64.2804457127633,0.));
#163702=CARTESIAN_POINT('Ctrl Pts',(31.4759001384922,64.2804457127633,12.));
#163703=CARTESIAN_POINT('Ctrl Pts',(31.4594841711188,64.264086819846,0.));
#163704=CARTESIAN_POINT('Ctrl Pts',(31.4594841711188,64.264086819846,12.));
#163705=CARTESIAN_POINT('Ctrl Pts',(31.4431158721229,64.2477429528408,0.));
#163706=CARTESIAN_POINT('Ctrl Pts',(31.4431158721229,64.2477429528408,12.));
#163707=CARTESIAN_POINT('Ctrl Pts',(31.426795287544,64.2314142508843,0.));
#163708=CARTESIAN_POINT('Ctrl Pts',(31.426795287544,64.2314142508843,12.));
#163709=CARTESIAN_POINT('Ctrl Pts',(31.4105224635298,64.2151008537733,0.));
#163710=CARTESIAN_POINT('Ctrl Pts',(31.4105224635298,64.2151008537733,12.));
#163711=CARTESIAN_POINT('Ctrl Pts',(31.3942974463458,64.1988029019733,0.));
#163712=CARTESIAN_POINT('Ctrl Pts',(31.3942974463458,64.1988029019733,12.));
#163713=CARTESIAN_POINT('Ctrl Pts',(31.3781202823758,64.1825205366231,0.));
#163714=CARTESIAN_POINT('Ctrl Pts',(31.3781202823758,64.1825205366231,12.));
#163715=CARTESIAN_POINT('Ctrl Pts',(31.3619910181222,64.1662538995407,0.));
#163716=CARTESIAN_POINT('Ctrl Pts',(31.3619910181222,64.1662538995407,12.));
#163717=CARTESIAN_POINT('Ctrl Pts',(31.3459097001995,64.150003133226,0.));
#163718=CARTESIAN_POINT('Ctrl Pts',(31.3459097001995,64.150003133226,12.));
#163719=CARTESIAN_POINT('Ctrl Pts',(31.3298763753366,64.1337683808667,0.));
#163720=CARTESIAN_POINT('Ctrl Pts',(31.3298763753366,64.1337683808667,12.));
#163721=CARTESIAN_POINT('Ctrl Pts',(31.3138910903852,64.1175497863475,0.));
#163722=CARTESIAN_POINT('Ctrl Pts',(31.3138910903852,64.1175497863475,12.));
#163723=CARTESIAN_POINT('Ctrl Pts',(31.2979538923213,64.1013474942554,0.));
#163724=CARTESIAN_POINT('Ctrl Pts',(31.2979538923213,64.1013474942554,12.));
#163725=CARTESIAN_POINT('Ctrl Pts',(31.2820648282451,64.0851616498861,0.));
#163726=CARTESIAN_POINT('Ctrl Pts',(31.2820648282451,64.0851616498861,12.));
#163727=CARTESIAN_POINT('Ctrl Pts',(31.2662239453734,64.0689923992475,0.));
#163728=CARTESIAN_POINT('Ctrl Pts',(31.2662239453734,64.0689923992475,12.));
#163729=CARTESIAN_POINT('Ctrl Pts',(31.2504312910457,64.0528398890671,0.));
#163730=CARTESIAN_POINT('Ctrl Pts',(31.2504312910457,64.0528398890671,12.));
#163731=CARTESIAN_POINT('Ctrl Pts',(31.23468691273,64.036704266799,0.));
#163732=CARTESIAN_POINT('Ctrl Pts',(31.23468691273,64.036704266799,12.));
#163733=CARTESIAN_POINT('Ctrl Pts',(31.2189908580245,64.0205856806298,0.));
#163734=CARTESIAN_POINT('Ctrl Pts',(31.2189908580245,64.0205856806298,12.));
#163735=CARTESIAN_POINT('Ctrl Pts',(31.2033431746558,64.004484279483,0.));
#163736=CARTESIAN_POINT('Ctrl Pts',(31.2033431746558,64.004484279483,12.));
#163737=CARTESIAN_POINT('Ctrl Pts',(31.1877439104717,63.9884002130209,0.));
#163738=CARTESIAN_POINT('Ctrl Pts',(31.1877439104717,63.9884002130209,12.));
#163739=CARTESIAN_POINT('Ctrl Pts',(31.1721931134488,63.972333631655,0.));
#163740=CARTESIAN_POINT('Ctrl Pts',(31.1721931134488,63.972333631655,12.));
#163741=CARTESIAN_POINT('Ctrl Pts',(31.1566908316992,63.9562846865566,0.));
#163742=CARTESIAN_POINT('Ctrl Pts',(31.1566908316992,63.9562846865566,12.));
#163743=CARTESIAN_POINT('Ctrl Pts',(31.1412371134727,63.9402535296651,0.));
#163744=CARTESIAN_POINT('Ctrl Pts',(31.1412371134727,63.9402535296651,12.));
#163745=CARTESIAN_POINT('Ctrl Pts',(31.1258320071545,63.9242403136954,0.));
#163746=CARTESIAN_POINT('Ctrl Pts',(31.1258320071545,63.9242403136954,12.));
#163747=CARTESIAN_POINT('Ctrl Pts',(31.1104755612606,63.9082451921447,0.));
#163748=CARTESIAN_POINT('Ctrl Pts',(31.1104755612606,63.9082451921447,12.));
#163749=CARTESIAN_POINT('Ctrl Pts',(31.0951678244454,63.8922683192963,0.));
#163750=CARTESIAN_POINT('Ctrl Pts',(31.0951678244454,63.8922683192963,12.));
#163751=CARTESIAN_POINT('Ctrl Pts',(31.079908845504,63.8763098502235,0.));
#163752=CARTESIAN_POINT('Ctrl Pts',(31.079908845504,63.8763098502235,12.));
#163753=CARTESIAN_POINT('Ctrl Pts',(31.0646986733723,63.8603699407922,0.));
#163754=CARTESIAN_POINT('Ctrl Pts',(31.0646986733723,63.8603699407922,12.));
#163755=CARTESIAN_POINT('Ctrl Pts',(31.0495373571217,63.8444487476615,0.));
#163756=CARTESIAN_POINT('Ctrl Pts',(31.0495373571217,63.8444487476615,12.));
#163757=CARTESIAN_POINT('Ctrl Pts',(31.0344249459544,63.8285464282857,0.));
#163758=CARTESIAN_POINT('Ctrl Pts',(31.0344249459544,63.8285464282857,12.));
#163759=CARTESIAN_POINT('Ctrl Pts',(31.0193614892177,63.8126631409376,0.));
#163760=CARTESIAN_POINT('Ctrl Pts',(31.0193614892177,63.8126631409376,12.));
#163761=CARTESIAN_POINT('Ctrl Pts',(31.0043470364112,63.7967990447288,0.));
#163762=CARTESIAN_POINT('Ctrl Pts',(31.0043470364112,63.7967990447288,12.));
#163763=CARTESIAN_POINT('Ctrl Pts',(30.9893816371907,63.7809542996258,0.));
#163764=CARTESIAN_POINT('Ctrl Pts',(30.9893816371907,63.7809542996258,12.));
#163765=CARTESIAN_POINT('Ctrl Pts',(30.9744653413679,63.7651290664713,0.));
#163766=CARTESIAN_POINT('Ctrl Pts',(30.9744653413679,63.7651290664713,12.));
#163767=CARTESIAN_POINT('Ctrl Pts',(30.9595981989091,63.7493235069844,0.));
#163768=CARTESIAN_POINT('Ctrl Pts',(30.9595981989091,63.7493235069844,12.));
#163769=CARTESIAN_POINT('Ctrl Pts',(30.9447802599345,63.733537783742,0.));
#163770=CARTESIAN_POINT('Ctrl Pts',(30.9447802599345,63.733537783742,12.));
#163771=CARTESIAN_POINT('Ctrl Pts',(30.9300115747113,63.7177720601604,0.));
#163772=CARTESIAN_POINT('Ctrl Pts',(30.9300115747113,63.7177720601604,12.));
#163773=CARTESIAN_POINT('Ctrl Pts',(30.9152921936471,63.7020265004805,0.));
#163774=CARTESIAN_POINT('Ctrl Pts',(30.9152921936471,63.7020265004805,12.));
#163775=CARTESIAN_POINT('Ctrl Pts',(30.9006221672703,63.6863012697354,0.));
#163776=CARTESIAN_POINT('Ctrl Pts',(30.9006221672703,63.6863012697354,12.));
#163777=CARTESIAN_POINT('Ctrl Pts',(30.8860015462488,63.6705965337996,0.));
#163778=CARTESIAN_POINT('Ctrl Pts',(30.8860015462488,63.6705965337996,12.));
#163779=CARTESIAN_POINT('Ctrl Pts',(30.8714303814202,63.6549124594681,0.));
#163780=CARTESIAN_POINT('Ctrl Pts',(30.8714303814202,63.6549124594681,12.));
#163781=CARTESIAN_POINT('Ctrl Pts',(30.8569087238131,63.6392492145233,0.));
#163782=CARTESIAN_POINT('Ctrl Pts',(30.8569087238131,63.6392492145233,12.));
#163783=CARTESIAN_POINT('Ctrl Pts',(30.8424366246665,63.6236069678041,0.));
#163784=CARTESIAN_POINT('Ctrl Pts',(30.8424366246665,63.6236069678041,12.));
#163785=CARTESIAN_POINT('Ctrl Pts',(30.8280141354447,63.6079858892747,0.));
#163786=CARTESIAN_POINT('Ctrl Pts',(30.8280141354447,63.6079858892747,12.));
#163787=CARTESIAN_POINT('Ctrl Pts',(30.8136413077999,63.5923861498964,0.));
#163788=CARTESIAN_POINT('Ctrl Pts',(30.8136413077999,63.5923861498964,12.));
#163789=CARTESIAN_POINT('Ctrl Pts',(30.7993181935265,63.5768079214868,0.));
#163790=CARTESIAN_POINT('Ctrl Pts',(30.7993181935265,63.5768079214868,12.));
#163791=CARTESIAN_POINT('Ctrl Pts',(30.7850448445207,63.5612513766005,0.));
#163792=CARTESIAN_POINT('Ctrl Pts',(30.7850448445207,63.5612513766005,12.));
#163793=CARTESIAN_POINT('Ctrl Pts',(30.7708213127169,63.5457166883558,0.));
#163794=CARTESIAN_POINT('Ctrl Pts',(30.7708213127169,63.5457166883558,12.));
#163795=CARTESIAN_POINT('Ctrl Pts',(30.7566476500772,63.5302040304173,0.));
#163796=CARTESIAN_POINT('Ctrl Pts',(30.7566476500772,63.5302040304173,12.));
#163797=CARTESIAN_POINT('Ctrl Pts',(30.7425239087294,63.514713577392,0.));
#163798=CARTESIAN_POINT('Ctrl Pts',(30.7425239087294,63.514713577392,12.));
#163799=CARTESIAN_POINT('Ctrl Pts',(30.7284501410827,63.4992455051805,0.));
#163800=CARTESIAN_POINT('Ctrl Pts',(30.7284501410827,63.4992455051805,12.));
#163801=CARTESIAN_POINT('Ctrl Pts',(30.7144263999259,63.4837999912758,0.));
#163802=CARTESIAN_POINT('Ctrl Pts',(30.7144263999259,63.4837999912758,12.));
#163803=CARTESIAN_POINT('Ctrl Pts',(30.7004527385806,63.4683772152497,0.));
#163804=CARTESIAN_POINT('Ctrl Pts',(30.7004527385806,63.4683772152497,12.));
#163805=CARTESIAN_POINT('Ctrl Pts',(30.686529210791,63.4529773584211,0.));
#163806=CARTESIAN_POINT('Ctrl Pts',(30.686529210791,63.4529773584211,12.));
#163807=CARTESIAN_POINT('Ctrl Pts',(30.6726558704301,63.4376006029575,0.));
#163808=CARTESIAN_POINT('Ctrl Pts',(30.6726558704301,63.4376006029575,12.));
#163809=CARTESIAN_POINT('Ctrl Pts',(30.6588327712482,63.4222471311236,0.));
#163810=CARTESIAN_POINT('Ctrl Pts',(30.6588327712482,63.4222471311236,12.));
#163811=CARTESIAN_POINT('Ctrl Pts',(30.6450599666135,63.4069171245094,0.));
#163812=CARTESIAN_POINT('Ctrl Pts',(30.6450599666135,63.4069171245094,12.));
#163813=CARTESIAN_POINT('Ctrl Pts',(30.6313375092084,63.3916107631421,0.));
#163814=CARTESIAN_POINT('Ctrl Pts',(30.6313375092084,63.3916107631421,12.));
#163815=CARTESIAN_POINT('Ctrl Pts',(30.6176654515988,63.3763282271838,0.));
#163816=CARTESIAN_POINT('Ctrl Pts',(30.6176654515988,63.3763282271838,12.));
#163817=CARTESIAN_POINT('Ctrl Pts',(30.6040438469089,63.3610696989599,0.));
#163818=CARTESIAN_POINT('Ctrl Pts',(30.6040438469089,63.3610696989599,12.));
#163819=CARTESIAN_POINT('Ctrl Pts',(30.5904727493707,63.3458353646144,0.));
#163820=CARTESIAN_POINT('Ctrl Pts',(30.5904727493707,63.3458353646144,12.));
#163821=CARTESIAN_POINT('Ctrl Pts',(30.5769522151147,63.330625416509,0.));
#163822=CARTESIAN_POINT('Ctrl Pts',(30.5769522151147,63.330625416509,12.));
#163823=CARTESIAN_POINT('Ctrl Pts',(30.5634823022358,63.315440053435,0.));
#163824=CARTESIAN_POINT('Ctrl Pts',(30.5634823022358,63.315440053435,12.));
#163825=CARTESIAN_POINT('Ctrl Pts',(30.5500630691342,63.300279475605,0.));
#163826=CARTESIAN_POINT('Ctrl Pts',(30.5500630691342,63.300279475605,12.));
#163827=CARTESIAN_POINT('Ctrl Pts',(30.5366945730503,63.2851438802462,0.));
#163828=CARTESIAN_POINT('Ctrl Pts',(30.5366945730503,63.2851438802462,12.));
#163829=CARTESIAN_POINT('Ctrl Pts',(30.5233768687875,63.2700334577661,0.));
#163830=CARTESIAN_POINT('Ctrl Pts',(30.5233768687875,63.2700334577661,12.));
#163831=CARTESIAN_POINT('Ctrl Pts',(30.5101100066683,63.2549483856268,0.));
#163832=CARTESIAN_POINT('Ctrl Pts',(30.5101100066683,63.2549483856268,12.));
#163833=CARTESIAN_POINT('Ctrl Pts',(30.4968940345027,63.2398888342612,0.));
#163834=CARTESIAN_POINT('Ctrl Pts',(30.4968940345027,63.2398888342612,12.));
#163835=CARTESIAN_POINT('Ctrl Pts',(30.4837290015011,63.2248549788272,0.));
#163836=CARTESIAN_POINT('Ctrl Pts',(30.4837290015011,63.2248549788272,12.));
#163837=CARTESIAN_POINT('Ctrl Pts',(30.470614961416,63.2098470086636,0.));
#163838=CARTESIAN_POINT('Ctrl Pts',(30.470614961416,63.2098470086636,12.));
#163839=CARTESIAN_POINT('Ctrl Pts',(30.4575519763305,63.1948651386868,0.));
#163840=CARTESIAN_POINT('Ctrl Pts',(30.4575519763305,63.1948651386868,12.));
#163841=CARTESIAN_POINT('Ctrl Pts',(30.4445401192324,63.1799096171757,0.));
#163842=CARTESIAN_POINT('Ctrl Pts',(30.4445401192324,63.1799096171757,12.));
#163843=CARTESIAN_POINT('Ctrl Pts',(30.431579465967,63.1649807016766,0.));
#163844=CARTESIAN_POINT('Ctrl Pts',(30.431579465967,63.1649807016766,12.));
#163845=CARTESIAN_POINT('Ctrl Pts',(30.4186700875598,63.1500786361382,0.));
#163846=CARTESIAN_POINT('Ctrl Pts',(30.4186700875598,63.1500786361382,12.));
#163847=CARTESIAN_POINT('Ctrl Pts',(30.4058120432259,63.1352036298512,0.));
#163848=CARTESIAN_POINT('Ctrl Pts',(30.4058120432259,63.1352036298512,12.));
#163849=CARTESIAN_POINT('Ctrl Pts',(30.3930053710592,63.1203558300911,0.));
#163850=CARTESIAN_POINT('Ctrl Pts',(30.3930053710592,63.1203558300911,12.));
#163851=CARTESIAN_POINT('Ctrl Pts',(30.3802500880565,63.1055353202641,0.));
#163852=CARTESIAN_POINT('Ctrl Pts',(30.3802500880565,63.1055353202641,12.));
#163853=CARTESIAN_POINT('Ctrl Pts',(30.3700869762658,63.0937007763826,0.));
#163854=CARTESIAN_POINT('Ctrl Pts',(30.3700869762658,63.0937007763826,12.));
#163855=CARTESIAN_POINT('Ctrl Pts',(30.3624877680747,63.0848371718274,0.));
#163856=CARTESIAN_POINT('Ctrl Pts',(30.3624877680747,63.0848371718274,12.));
#163857=CARTESIAN_POINT('Ctrl Pts',(30.3574319069365,63.0789335700774,0.));
#163858=CARTESIAN_POINT('Ctrl Pts',(30.3574319069365,63.0789335700774,12.));
#163859=CARTESIAN_POINT('Ctrl Pts',(30.3549065457811,63.0759831361898,0.));
#163860=CARTESIAN_POINT('Ctrl Pts',(30.3549065457811,63.0759831361898,12.));
#163861=CARTESIAN_POINT('',(30.3549065457811,63.0759831361898,12.));
#163862=CARTESIAN_POINT('Ctrl Pts',(30.3549065457811,63.0759831361898,12.));
#163863=CARTESIAN_POINT('Ctrl Pts',(30.3574319069365,63.0789335700774,12.));
#163864=CARTESIAN_POINT('Ctrl Pts',(30.3624877680747,63.0848371718274,12.));
#163865=CARTESIAN_POINT('Ctrl Pts',(30.3700869762658,63.0937007763826,12.));
#163866=CARTESIAN_POINT('Ctrl Pts',(30.3802500880565,63.1055353202641,12.));
#163867=CARTESIAN_POINT('Ctrl Pts',(30.3930053710592,63.1203558300911,12.));
#163868=CARTESIAN_POINT('Ctrl Pts',(30.4058120432259,63.1352036298512,12.));
#163869=CARTESIAN_POINT('Ctrl Pts',(30.4186700875598,63.1500786361382,12.));
#163870=CARTESIAN_POINT('Ctrl Pts',(30.431579465967,63.1649807016766,12.));
#163871=CARTESIAN_POINT('Ctrl Pts',(30.4445401192324,63.1799096171757,12.));
#163872=CARTESIAN_POINT('Ctrl Pts',(30.4575519763305,63.1948651386868,12.));
#163873=CARTESIAN_POINT('Ctrl Pts',(30.470614961416,63.2098470086636,12.));
#163874=CARTESIAN_POINT('Ctrl Pts',(30.4837290015011,63.2248549788272,12.));
#163875=CARTESIAN_POINT('Ctrl Pts',(30.4968940345027,63.2398888342612,12.));
#163876=CARTESIAN_POINT('Ctrl Pts',(30.5101100066683,63.2549483856268,12.));
#163877=CARTESIAN_POINT('Ctrl Pts',(30.5233768687875,63.2700334577661,12.));
#163878=CARTESIAN_POINT('Ctrl Pts',(30.5366945730503,63.2851438802462,12.));
#163879=CARTESIAN_POINT('Ctrl Pts',(30.5500630691342,63.300279475605,12.));
#163880=CARTESIAN_POINT('Ctrl Pts',(30.5634823022358,63.315440053435,12.));
#163881=CARTESIAN_POINT('Ctrl Pts',(30.5769522151147,63.330625416509,12.));
#163882=CARTESIAN_POINT('Ctrl Pts',(30.5904727493707,63.3458353646144,12.));
#163883=CARTESIAN_POINT('Ctrl Pts',(30.6040438469089,63.3610696989599,12.));
#163884=CARTESIAN_POINT('Ctrl Pts',(30.6176654515988,63.3763282271838,12.));
#163885=CARTESIAN_POINT('Ctrl Pts',(30.6313375092084,63.3916107631421,12.));
#163886=CARTESIAN_POINT('Ctrl Pts',(30.6450599666135,63.4069171245094,12.));
#163887=CARTESIAN_POINT('Ctrl Pts',(30.6588327712482,63.4222471311236,12.));
#163888=CARTESIAN_POINT('Ctrl Pts',(30.6726558704301,63.4376006029575,12.));
#163889=CARTESIAN_POINT('Ctrl Pts',(30.686529210791,63.4529773584211,12.));
#163890=CARTESIAN_POINT('Ctrl Pts',(30.7004527385806,63.4683772152497,12.));
#163891=CARTESIAN_POINT('Ctrl Pts',(30.7144263999259,63.4837999912758,12.));
#163892=CARTESIAN_POINT('Ctrl Pts',(30.7284501410827,63.4992455051805,12.));
#163893=CARTESIAN_POINT('Ctrl Pts',(30.7425239087294,63.514713577392,12.));
#163894=CARTESIAN_POINT('Ctrl Pts',(30.7566476500772,63.5302040304173,12.));
#163895=CARTESIAN_POINT('Ctrl Pts',(30.7708213127169,63.5457166883558,12.));
#163896=CARTESIAN_POINT('Ctrl Pts',(30.7850448445207,63.5612513766005,12.));
#163897=CARTESIAN_POINT('Ctrl Pts',(30.7993181935265,63.5768079214868,12.));
#163898=CARTESIAN_POINT('Ctrl Pts',(30.8136413077999,63.5923861498964,12.));
#163899=CARTESIAN_POINT('Ctrl Pts',(30.8280141354447,63.6079858892747,12.));
#163900=CARTESIAN_POINT('Ctrl Pts',(30.8424366246665,63.6236069678041,12.));
#163901=CARTESIAN_POINT('Ctrl Pts',(30.8569087238131,63.6392492145233,12.));
#163902=CARTESIAN_POINT('Ctrl Pts',(30.8714303814202,63.6549124594681,12.));
#163903=CARTESIAN_POINT('Ctrl Pts',(30.8860015462488,63.6705965337996,12.));
#163904=CARTESIAN_POINT('Ctrl Pts',(30.9006221672703,63.6863012697354,12.));
#163905=CARTESIAN_POINT('Ctrl Pts',(30.9152921936471,63.7020265004805,12.));
#163906=CARTESIAN_POINT('Ctrl Pts',(30.9300115747113,63.7177720601604,12.));
#163907=CARTESIAN_POINT('Ctrl Pts',(30.9447802599345,63.733537783742,12.));
#163908=CARTESIAN_POINT('Ctrl Pts',(30.9595981989091,63.7493235069844,12.));
#163909=CARTESIAN_POINT('Ctrl Pts',(30.9744653413679,63.7651290664713,12.));
#163910=CARTESIAN_POINT('Ctrl Pts',(30.9893816371907,63.7809542996258,12.));
#163911=CARTESIAN_POINT('Ctrl Pts',(31.0043470364112,63.7967990447288,12.));
#163912=CARTESIAN_POINT('Ctrl Pts',(31.0193614892177,63.8126631409376,12.));
#163913=CARTESIAN_POINT('Ctrl Pts',(31.0344249459544,63.8285464282857,12.));
#163914=CARTESIAN_POINT('Ctrl Pts',(31.0495373571217,63.8444487476615,12.));
#163915=CARTESIAN_POINT('Ctrl Pts',(31.0646986733723,63.8603699407922,12.));
#163916=CARTESIAN_POINT('Ctrl Pts',(31.079908845504,63.8763098502235,12.));
#163917=CARTESIAN_POINT('Ctrl Pts',(31.0951678244454,63.8922683192963,12.));
#163918=CARTESIAN_POINT('Ctrl Pts',(31.1104755612606,63.9082451921447,12.));
#163919=CARTESIAN_POINT('Ctrl Pts',(31.1258320071545,63.9242403136954,12.));
#163920=CARTESIAN_POINT('Ctrl Pts',(31.1412371134727,63.9402535296651,12.));
#163921=CARTESIAN_POINT('Ctrl Pts',(31.1566908316992,63.9562846865566,12.));
#163922=CARTESIAN_POINT('Ctrl Pts',(31.1721931134488,63.972333631655,12.));
#163923=CARTESIAN_POINT('Ctrl Pts',(31.1877439104717,63.9884002130209,12.));
#163924=CARTESIAN_POINT('Ctrl Pts',(31.2033431746558,64.004484279483,12.));
#163925=CARTESIAN_POINT('Ctrl Pts',(31.2189908580245,64.0205856806298,12.));
#163926=CARTESIAN_POINT('Ctrl Pts',(31.23468691273,64.036704266799,12.));
#163927=CARTESIAN_POINT('Ctrl Pts',(31.2504312910457,64.0528398890671,12.));
#163928=CARTESIAN_POINT('Ctrl Pts',(31.2662239453734,64.0689923992475,12.));
#163929=CARTESIAN_POINT('Ctrl Pts',(31.2820648282451,64.0851616498861,12.));
#163930=CARTESIAN_POINT('Ctrl Pts',(31.2979538923213,64.1013474942554,12.));
#163931=CARTESIAN_POINT('Ctrl Pts',(31.3138910903852,64.1175497863475,12.));
#163932=CARTESIAN_POINT('Ctrl Pts',(31.3298763753366,64.1337683808667,12.));
#163933=CARTESIAN_POINT('Ctrl Pts',(31.3459097001995,64.150003133226,12.));
#163934=CARTESIAN_POINT('Ctrl Pts',(31.3619910181222,64.1662538995407,12.));
#163935=CARTESIAN_POINT('Ctrl Pts',(31.3781202823758,64.1825205366231,12.));
#163936=CARTESIAN_POINT('Ctrl Pts',(31.3942974463458,64.1988029019733,12.));
#163937=CARTESIAN_POINT('Ctrl Pts',(31.4105224635298,64.2151008537733,12.));
#163938=CARTESIAN_POINT('Ctrl Pts',(31.426795287544,64.2314142508843,12.));
#163939=CARTESIAN_POINT('Ctrl Pts',(31.4431158721229,64.2477429528408,12.));
#163940=CARTESIAN_POINT('Ctrl Pts',(31.4594841711188,64.264086819846,12.));
#163941=CARTESIAN_POINT('Ctrl Pts',(31.4759001384922,64.2804457127633,12.));
#163942=CARTESIAN_POINT('Ctrl Pts',(31.4923637283109,64.2968194931113,12.));
#163943=CARTESIAN_POINT('Ctrl Pts',(31.5088748947565,64.3132080230603,12.));
#163944=CARTESIAN_POINT('Ctrl Pts',(31.5254335921239,64.3296111654273,12.));
#163945=CARTESIAN_POINT('Ctrl Pts',(31.5420397748198,64.34602878367,12.));
#163946=CARTESIAN_POINT('Ctrl Pts',(31.5586933973531,64.3624607418798,12.));
#163947=CARTESIAN_POINT('Ctrl Pts',(31.5753944143355,64.3789069047768,12.));
#163948=CARTESIAN_POINT('Ctrl Pts',(31.5921427804879,64.3953671377071,12.));
#163949=CARTESIAN_POINT('Ctrl Pts',(31.6089384506399,64.4118413066386,12.));
#163950=CARTESIAN_POINT('Ctrl Pts',(31.6257813797281,64.4283292781553,12.));
#163951=CARTESIAN_POINT('Ctrl Pts',(31.6426715227865,64.4448309194499,12.));
#163952=CARTESIAN_POINT('Ctrl Pts',(31.6596088349468,64.4613460983186,12.));
#163953=CARTESIAN_POINT('Ctrl Pts',(31.6765932714456,64.4778746831598,12.));
#163954=CARTESIAN_POINT('Ctrl Pts',(31.6936247876228,64.4944165429672,12.));
#163955=CARTESIAN_POINT('Ctrl Pts',(31.7107033389204,64.5109715473277,12.));
#163956=CARTESIAN_POINT('Ctrl Pts',(31.7278288808736,64.5275395664134,12.));
#163957=CARTESIAN_POINT('Ctrl Pts',(31.7450013691117,64.544120470978,12.));
#163958=CARTESIAN_POINT('Ctrl Pts',(31.7622207593637,64.5607141323527,12.));
#163959=CARTESIAN_POINT('Ctrl Pts',(31.7794870074583,64.5773204224429,12.));
#163960=CARTESIAN_POINT('Ctrl Pts',(31.7968000693218,64.5939392137233,12.));
#163961=CARTESIAN_POINT('Ctrl Pts',(31.8141599009684,64.6105703792311,12.));
#163962=CARTESIAN_POINT('Ctrl Pts',(31.8315664585027,64.627213792563,12.));
#163963=CARTESIAN_POINT('Ctrl Pts',(31.849019698125,64.6438693278718,12.));
#163964=CARTESIAN_POINT('Ctrl Pts',(31.8665195761312,64.6605368598631,12.));
#163965=CARTESIAN_POINT('Ctrl Pts',(31.8840660489106,64.6772162637905,12.));
#163966=CARTESIAN_POINT('Ctrl Pts',(31.9016590729371,64.6939074154491,12.));
#163967=CARTESIAN_POINT('Ctrl Pts',(31.9192986047702,64.7106101911723,12.));
#163968=CARTESIAN_POINT('Ctrl Pts',(31.9369846010613,64.727324467829,12.));
#163969=CARTESIAN_POINT('Ctrl Pts',(31.9547170185533,64.7440501228201,12.));
#163970=CARTESIAN_POINT('Ctrl Pts',(31.972495814079,64.7607870340738,12.));
#163971=CARTESIAN_POINT('Ctrl Pts',(31.9903209445521,64.7775350800404,12.));
#163972=CARTESIAN_POINT('Ctrl Pts',(32.0081923669677,64.7942941396883,12.));
#163973=CARTESIAN_POINT('Ctrl Pts',(32.0261100384092,64.811064092502,12.));
#163974=CARTESIAN_POINT('Ctrl Pts',(32.0440739160476,64.8278448184785,12.));
#163975=CARTESIAN_POINT('Ctrl Pts',(32.0620839571409,64.8446361981234,12.));
#163976=CARTESIAN_POINT('Ctrl Pts',(32.0801401190244,64.8614381124455,12.));
#163977=CARTESIAN_POINT('Ctrl Pts',(32.0982423591112,64.8782504429527,12.));
#163978=CARTESIAN_POINT('Ctrl Pts',(32.1163906348983,64.8950730716501,12.));
#163979=CARTESIAN_POINT('Ctrl Pts',(32.1345849039674,64.9119058810367,12.));
#163980=CARTESIAN_POINT('Ctrl Pts',(32.152825123983,64.9287487541015,12.));
#163981=CARTESIAN_POINT('Ctrl Pts',(32.1711112526854,64.9456015743193,12.));
#163982=CARTESIAN_POINT('Ctrl Pts',(32.189443247888,64.9624642256461,12.));
#163983=CARTESIAN_POINT('Ctrl Pts',(32.207821067485,64.9793365925178,12.));
#163984=CARTESIAN_POINT('Ctrl Pts',(32.2262446694512,64.9962185598462,12.));
#163985=CARTESIAN_POINT('Ctrl Pts',(32.2447140118422,65.0131100130158,12.));
#163986=CARTESIAN_POINT('Ctrl Pts',(32.2632290527862,65.03001083788,12.));
#163987=CARTESIAN_POINT('Ctrl Pts',(32.2817897504807,65.0469209207563,12.));
#163988=CARTESIAN_POINT('Ctrl Pts',(32.3003960632006,65.0638401484257,12.));
#163989=CARTESIAN_POINT('Ctrl Pts',(32.3190479492987,65.0807684081282,12.));
#163990=CARTESIAN_POINT('Ctrl Pts',(32.3377453672051,65.0977055875608,12.));
#163991=CARTESIAN_POINT('Ctrl Pts',(32.3564882754212,65.1146515748722,12.));
#163992=CARTESIAN_POINT('Ctrl Pts',(32.3752766325136,65.1316062586588,12.));
#163993=CARTESIAN_POINT('Ctrl Pts',(32.3941103971221,65.1485695279635,12.));
#163994=CARTESIAN_POINT('Ctrl Pts',(32.4129895279615,65.1655412722726,12.));
#163995=CARTESIAN_POINT('Ctrl Pts',(32.4319139838212,65.182521381514,12.));
#163996=CARTESIAN_POINT('Ctrl Pts',(32.450883723561,65.1995097460538,12.));
#163997=CARTESIAN_POINT('Ctrl Pts',(32.4698987061032,65.2165062566924,12.));
#163998=CARTESIAN_POINT('Ctrl Pts',(32.4889588904392,65.2335108046614,12.));
#163999=CARTESIAN_POINT('Ctrl Pts',(32.5080642356328,65.2505232816209,12.));
#164000=CARTESIAN_POINT('Ctrl Pts',(32.5272147008191,65.2675435796558,12.));
#164001=CARTESIAN_POINT('Ctrl Pts',(32.5464102452014,65.2845715912721,12.));
#164002=CARTESIAN_POINT('Ctrl Pts',(32.5656508280421,65.3016072093912,12.));
#164003=CARTESIAN_POINT('Ctrl Pts',(32.5849364086678,65.31865032735,12.));
#164004=CARTESIAN_POINT('Ctrl Pts',(32.6042669464751,65.3357008389004,12.));
#164005=CARTESIAN_POINT('Ctrl Pts',(32.6236424009301,65.3527586382081,12.));
#164006=CARTESIAN_POINT('Ctrl Pts',(32.6430627315674,65.3698236198513,12.));
#164007=CARTESIAN_POINT('Ctrl Pts',(32.662527897981,65.3868956788182,12.));
#164008=CARTESIAN_POINT('Ctrl Pts',(32.6820378598267,65.4039747105038,12.));
#164009=CARTESIAN_POINT('Ctrl Pts',(32.7015925768265,65.4210606107035,12.));
#164010=CARTESIAN_POINT('Ctrl Pts',(32.7211920087684,65.4381532756065,12.));
#164011=CARTESIAN_POINT('Ctrl Pts',(32.7408361155037,65.4552526017905,12.));
#164012=CARTESIAN_POINT('Ctrl Pts',(32.7605248569378,65.4723584862122,12.));
#164013=CARTESIAN_POINT('Ctrl Pts',(32.7802581930287,65.4894708262061,12.));
#164014=CARTESIAN_POINT('Ctrl Pts',(32.8000360837975,65.5065895194928,12.));
#164015=CARTESIAN_POINT('Ctrl Pts',(32.8198584893315,65.5237144641858,12.));
#164016=CARTESIAN_POINT('Ctrl Pts',(32.8397253697865,65.5408455587965,12.));
#164017=CARTESIAN_POINT('Ctrl Pts',(32.8596366853832,65.5579827022421,12.));
#164018=CARTESIAN_POINT('Ctrl Pts',(32.879592396403,65.5751257938473,12.));
#164019=CARTESIAN_POINT('Ctrl Pts',(32.8995924631898,65.5922747333194,12.));
#164020=CARTESIAN_POINT('Ctrl Pts',(32.9196368461463,65.6094294207276,12.));
#164021=CARTESIAN_POINT('Ctrl Pts',(32.9397255057274,65.6265897564783,12.));
#164022=CARTESIAN_POINT('Ctrl Pts',(32.9598584024312,65.6437556412947,12.));
#164023=CARTESIAN_POINT('Ctrl Pts',(32.980035496784,65.6609269761889,12.));
#164024=CARTESIAN_POINT('Ctrl Pts',(33.0002567493573,65.6781036625027,12.));
#164025=CARTESIAN_POINT('Ctrl Pts',(33.0205221207873,65.6952856019533,12.));
#164026=CARTESIAN_POINT('Ctrl Pts',(33.0408315717873,65.7124726966802,12.));
#164027=CARTESIAN_POINT('Ctrl Pts',(33.0611850631582,65.7296648492825,12.));
#164028=CARTESIAN_POINT('Ctrl Pts',(33.081582555798,65.7468619628816,12.));
#164029=CARTESIAN_POINT('Ctrl Pts',(33.1020240106884,65.7640639410661,12.));
#164030=CARTESIAN_POINT('Ctrl Pts',(33.1225093888672,65.7812706877697,12.));
#164031=CARTESIAN_POINT('Ctrl Pts',(33.1430386513976,65.7984821071623,12.));
#164032=CARTESIAN_POINT('Ctrl Pts',(33.16361175934,65.8156981035503,12.));
#164033=CARTESIAN_POINT('Ctrl Pts',(33.1842286737051,65.8329185812375,12.));
#164034=CARTESIAN_POINT('Ctrl Pts',(33.2048893554491,65.8501434445164,12.));
#164035=CARTESIAN_POINT('Ctrl Pts',(33.2255937655649,65.8673725979578,12.));
#164036=CARTESIAN_POINT('Ctrl Pts',(33.2463418651492,65.8846059466372,12.));
#164037=CARTESIAN_POINT('Ctrl Pts',(33.2671336154753,65.9018433963889,12.));
#164038=CARTESIAN_POINT('Ctrl Pts',(33.2879689780572,65.9190848540433,12.));
#164039=CARTESIAN_POINT('Ctrl Pts',(33.3088479147164,65.9363302276846,12.));
#164040=CARTESIAN_POINT('Ctrl Pts',(33.3297703874265,65.9535794260831,12.));
#164041=CARTESIAN_POINT('Ctrl Pts',(33.3507363581592,65.970832358141,12.));
#164042=CARTESIAN_POINT('Ctrl Pts',(33.37174578871,65.9880889322831,12.));
#164043=CARTESIAN_POINT('Ctrl Pts',(33.3927986405605,66.0053490559812,12.));
#164044=CARTESIAN_POINT('Ctrl Pts',(33.4138948746388,66.0226126349446,12.));
#164045=CARTESIAN_POINT('Ctrl Pts',(33.43503445151,66.0398795737777,12.));
#164046=CARTESIAN_POINT('Ctrl Pts',(33.4562173318025,66.0571497774434,12.));
#164047=CARTESIAN_POINT('Ctrl Pts',(33.4774434765745,66.0744231525415,12.));
#164048=CARTESIAN_POINT('Ctrl Pts',(33.4987128476622,66.0916996085245,12.));
#164049=CARTESIAN_POINT('Ctrl Pts',(33.5200254081243,66.1089790592729,12.));
#164050=CARTESIAN_POINT('Ctrl Pts',(33.541381122345,66.1262614234674,12.));
#164051=CARTESIAN_POINT('Ctrl Pts',(33.5597240685845,66.1410781873278,12.));
#164052=CARTESIAN_POINT('Ctrl Pts',(33.5738105077873,66.1524393974172,12.));
#164053=CARTESIAN_POINT('Ctrl Pts',(33.5836213514186,66.160343817752,12.));
#164054=CARTESIAN_POINT('Ctrl Pts',(33.5891439876489,66.1647906582654,12.));
#164055=CARTESIAN_POINT('Ctrl Pts',(33.5903722665274,66.1657795405958,12.));
#164056=CARTESIAN_POINT('',(30.3549065457811,63.0759831361898,0.));
#164057=CARTESIAN_POINT('',(30.3549065457811,63.0759831361898,0.));
#164058=CARTESIAN_POINT('Ctrl Pts',(33.5903722665274,66.1657795405958,0.));
#164059=CARTESIAN_POINT('Ctrl Pts',(33.5891439876489,66.1647906582654,0.));
#164060=CARTESIAN_POINT('Ctrl Pts',(33.5836213514186,66.160343817752,0.));
#164061=CARTESIAN_POINT('Ctrl Pts',(33.5738105077873,66.1524393974172,0.));
#164062=CARTESIAN_POINT('Ctrl Pts',(33.5597240685845,66.1410781873278,0.));
#164063=CARTESIAN_POINT('Ctrl Pts',(33.541381122345,66.1262614234674,0.));
#164064=CARTESIAN_POINT('Ctrl Pts',(33.5200254081243,66.1089790592729,0.));
#164065=CARTESIAN_POINT('Ctrl Pts',(33.4987128476622,66.0916996085245,0.));
#164066=CARTESIAN_POINT('Ctrl Pts',(33.4774434765745,66.0744231525415,0.));
#164067=CARTESIAN_POINT('Ctrl Pts',(33.4562173318025,66.0571497774434,0.));
#164068=CARTESIAN_POINT('Ctrl Pts',(33.43503445151,66.0398795737777,0.));
#164069=CARTESIAN_POINT('Ctrl Pts',(33.4138948746388,66.0226126349446,0.));
#164070=CARTESIAN_POINT('Ctrl Pts',(33.3927986405605,66.0053490559812,0.));
#164071=CARTESIAN_POINT('Ctrl Pts',(33.37174578871,65.9880889322831,0.));
#164072=CARTESIAN_POINT('Ctrl Pts',(33.3507363581592,65.970832358141,0.));
#164073=CARTESIAN_POINT('Ctrl Pts',(33.3297703874265,65.9535794260831,0.));
#164074=CARTESIAN_POINT('Ctrl Pts',(33.3088479147164,65.9363302276846,0.));
#164075=CARTESIAN_POINT('Ctrl Pts',(33.2879689780572,65.9190848540433,0.));
#164076=CARTESIAN_POINT('Ctrl Pts',(33.2671336154753,65.9018433963889,0.));
#164077=CARTESIAN_POINT('Ctrl Pts',(33.2463418651492,65.8846059466372,0.));
#164078=CARTESIAN_POINT('Ctrl Pts',(33.2255937655649,65.8673725979578,0.));
#164079=CARTESIAN_POINT('Ctrl Pts',(33.2048893554491,65.8501434445164,0.));
#164080=CARTESIAN_POINT('Ctrl Pts',(33.1842286737051,65.8329185812375,0.));
#164081=CARTESIAN_POINT('Ctrl Pts',(33.16361175934,65.8156981035503,0.));
#164082=CARTESIAN_POINT('Ctrl Pts',(33.1430386513976,65.7984821071623,0.));
#164083=CARTESIAN_POINT('Ctrl Pts',(33.1225093888672,65.7812706877697,0.));
#164084=CARTESIAN_POINT('Ctrl Pts',(33.1020240106884,65.7640639410661,0.));
#164085=CARTESIAN_POINT('Ctrl Pts',(33.081582555798,65.7468619628816,0.));
#164086=CARTESIAN_POINT('Ctrl Pts',(33.0611850631582,65.7296648492825,0.));
#164087=CARTESIAN_POINT('Ctrl Pts',(33.0408315717873,65.7124726966802,0.));
#164088=CARTESIAN_POINT('Ctrl Pts',(33.0205221207873,65.6952856019533,0.));
#164089=CARTESIAN_POINT('Ctrl Pts',(33.0002567493573,65.6781036625027,0.));
#164090=CARTESIAN_POINT('Ctrl Pts',(32.980035496784,65.6609269761889,0.));
#164091=CARTESIAN_POINT('Ctrl Pts',(32.9598584024312,65.6437556412947,0.));
#164092=CARTESIAN_POINT('Ctrl Pts',(32.9397255057274,65.6265897564783,0.));
#164093=CARTESIAN_POINT('Ctrl Pts',(32.9196368461463,65.6094294207276,0.));
#164094=CARTESIAN_POINT('Ctrl Pts',(32.8995924631898,65.5922747333194,0.));
#164095=CARTESIAN_POINT('Ctrl Pts',(32.879592396403,65.5751257938473,0.));
#164096=CARTESIAN_POINT('Ctrl Pts',(32.8596366853832,65.5579827022421,0.));
#164097=CARTESIAN_POINT('Ctrl Pts',(32.8397253697865,65.5408455587965,0.));
#164098=CARTESIAN_POINT('Ctrl Pts',(32.8198584893315,65.5237144641858,0.));
#164099=CARTESIAN_POINT('Ctrl Pts',(32.8000360837975,65.5065895194928,0.));
#164100=CARTESIAN_POINT('Ctrl Pts',(32.7802581930287,65.4894708262061,0.));
#164101=CARTESIAN_POINT('Ctrl Pts',(32.7605248569378,65.4723584862122,0.));
#164102=CARTESIAN_POINT('Ctrl Pts',(32.7408361155037,65.4552526017905,0.));
#164103=CARTESIAN_POINT('Ctrl Pts',(32.7211920087684,65.4381532756065,0.));
#164104=CARTESIAN_POINT('Ctrl Pts',(32.7015925768265,65.4210606107035,0.));
#164105=CARTESIAN_POINT('Ctrl Pts',(32.6820378598267,65.4039747105038,0.));
#164106=CARTESIAN_POINT('Ctrl Pts',(32.662527897981,65.3868956788182,0.));
#164107=CARTESIAN_POINT('Ctrl Pts',(32.6430627315674,65.3698236198513,0.));
#164108=CARTESIAN_POINT('Ctrl Pts',(32.6236424009301,65.3527586382081,0.));
#164109=CARTESIAN_POINT('Ctrl Pts',(32.6042669464751,65.3357008389004,0.));
#164110=CARTESIAN_POINT('Ctrl Pts',(32.5849364086678,65.31865032735,0.));
#164111=CARTESIAN_POINT('Ctrl Pts',(32.5656508280421,65.3016072093912,0.));
#164112=CARTESIAN_POINT('Ctrl Pts',(32.5464102452014,65.2845715912721,0.));
#164113=CARTESIAN_POINT('Ctrl Pts',(32.5272147008191,65.2675435796558,0.));
#164114=CARTESIAN_POINT('Ctrl Pts',(32.5080642356328,65.2505232816209,0.));
#164115=CARTESIAN_POINT('Ctrl Pts',(32.4889588904392,65.2335108046614,0.));
#164116=CARTESIAN_POINT('Ctrl Pts',(32.4698987061032,65.2165062566924,0.));
#164117=CARTESIAN_POINT('Ctrl Pts',(32.450883723561,65.1995097460538,0.));
#164118=CARTESIAN_POINT('Ctrl Pts',(32.4319139838212,65.182521381514,0.));
#164119=CARTESIAN_POINT('Ctrl Pts',(32.4129895279615,65.1655412722726,0.));
#164120=CARTESIAN_POINT('Ctrl Pts',(32.3941103971221,65.1485695279635,0.));
#164121=CARTESIAN_POINT('Ctrl Pts',(32.3752766325136,65.1316062586588,0.));
#164122=CARTESIAN_POINT('Ctrl Pts',(32.3564882754212,65.1146515748722,0.));
#164123=CARTESIAN_POINT('Ctrl Pts',(32.3377453672051,65.0977055875608,0.));
#164124=CARTESIAN_POINT('Ctrl Pts',(32.3190479492987,65.0807684081282,0.));
#164125=CARTESIAN_POINT('Ctrl Pts',(32.3003960632006,65.0638401484257,0.));
#164126=CARTESIAN_POINT('Ctrl Pts',(32.2817897504807,65.0469209207563,0.));
#164127=CARTESIAN_POINT('Ctrl Pts',(32.2632290527862,65.03001083788,0.));
#164128=CARTESIAN_POINT('Ctrl Pts',(32.2447140118422,65.0131100130158,0.));
#164129=CARTESIAN_POINT('Ctrl Pts',(32.2262446694512,64.9962185598462,0.));
#164130=CARTESIAN_POINT('Ctrl Pts',(32.207821067485,64.9793365925178,0.));
#164131=CARTESIAN_POINT('Ctrl Pts',(32.189443247888,64.9624642256461,0.));
#164132=CARTESIAN_POINT('Ctrl Pts',(32.1711112526854,64.9456015743193,0.));
#164133=CARTESIAN_POINT('Ctrl Pts',(32.152825123983,64.9287487541015,0.));
#164134=CARTESIAN_POINT('Ctrl Pts',(32.1345849039674,64.9119058810367,0.));
#164135=CARTESIAN_POINT('Ctrl Pts',(32.1163906348983,64.8950730716501,0.));
#164136=CARTESIAN_POINT('Ctrl Pts',(32.0982423591112,64.8782504429527,0.));
#164137=CARTESIAN_POINT('Ctrl Pts',(32.0801401190244,64.8614381124455,0.));
#164138=CARTESIAN_POINT('Ctrl Pts',(32.0620839571409,64.8446361981234,0.));
#164139=CARTESIAN_POINT('Ctrl Pts',(32.0440739160476,64.8278448184785,0.));
#164140=CARTESIAN_POINT('Ctrl Pts',(32.0261100384092,64.811064092502,0.));
#164141=CARTESIAN_POINT('Ctrl Pts',(32.0081923669677,64.7942941396883,0.));
#164142=CARTESIAN_POINT('Ctrl Pts',(31.9903209445521,64.7775350800404,0.));
#164143=CARTESIAN_POINT('Ctrl Pts',(31.972495814079,64.7607870340738,0.));
#164144=CARTESIAN_POINT('Ctrl Pts',(31.9547170185533,64.7440501228201,0.));
#164145=CARTESIAN_POINT('Ctrl Pts',(31.9369846010613,64.727324467829,0.));
#164146=CARTESIAN_POINT('Ctrl Pts',(31.9192986047702,64.7106101911723,0.));
#164147=CARTESIAN_POINT('Ctrl Pts',(31.9016590729371,64.6939074154491,0.));
#164148=CARTESIAN_POINT('Ctrl Pts',(31.8840660489106,64.6772162637905,0.));
#164149=CARTESIAN_POINT('Ctrl Pts',(31.8665195761312,64.6605368598631,0.));
#164150=CARTESIAN_POINT('Ctrl Pts',(31.849019698125,64.6438693278718,0.));
#164151=CARTESIAN_POINT('Ctrl Pts',(31.8315664585027,64.627213792563,0.));
#164152=CARTESIAN_POINT('Ctrl Pts',(31.8141599009684,64.6105703792311,0.));
#164153=CARTESIAN_POINT('Ctrl Pts',(31.7968000693218,64.5939392137233,0.));
#164154=CARTESIAN_POINT('Ctrl Pts',(31.7794870074583,64.5773204224429,0.));
#164155=CARTESIAN_POINT('Ctrl Pts',(31.7622207593637,64.5607141323527,0.));
#164156=CARTESIAN_POINT('Ctrl Pts',(31.7450013691117,64.544120470978,0.));
#164157=CARTESIAN_POINT('Ctrl Pts',(31.7278288808736,64.5275395664134,0.));
#164158=CARTESIAN_POINT('Ctrl Pts',(31.7107033389204,64.5109715473277,0.));
#164159=CARTESIAN_POINT('Ctrl Pts',(31.6936247876228,64.4944165429672,0.));
#164160=CARTESIAN_POINT('Ctrl Pts',(31.6765932714456,64.4778746831598,0.));
#164161=CARTESIAN_POINT('Ctrl Pts',(31.6596088349468,64.4613460983186,0.));
#164162=CARTESIAN_POINT('Ctrl Pts',(31.6426715227865,64.4448309194499,0.));
#164163=CARTESIAN_POINT('Ctrl Pts',(31.6257813797281,64.4283292781553,0.));
#164164=CARTESIAN_POINT('Ctrl Pts',(31.6089384506399,64.4118413066386,0.));
#164165=CARTESIAN_POINT('Ctrl Pts',(31.5921427804879,64.3953671377071,0.));
#164166=CARTESIAN_POINT('Ctrl Pts',(31.5753944143355,64.3789069047768,0.));
#164167=CARTESIAN_POINT('Ctrl Pts',(31.5586933973531,64.3624607418798,0.));
#164168=CARTESIAN_POINT('Ctrl Pts',(31.5420397748198,64.34602878367,0.));
#164169=CARTESIAN_POINT('Ctrl Pts',(31.5254335921239,64.3296111654273,0.));
#164170=CARTESIAN_POINT('Ctrl Pts',(31.5088748947565,64.3132080230603,0.));
#164171=CARTESIAN_POINT('Ctrl Pts',(31.4923637283109,64.2968194931113,0.));
#164172=CARTESIAN_POINT('Ctrl Pts',(31.4759001384922,64.2804457127633,0.));
#164173=CARTESIAN_POINT('Ctrl Pts',(31.4594841711188,64.264086819846,0.));
#164174=CARTESIAN_POINT('Ctrl Pts',(31.4431158721229,64.2477429528408,0.));
#164175=CARTESIAN_POINT('Ctrl Pts',(31.426795287544,64.2314142508843,0.));
#164176=CARTESIAN_POINT('Ctrl Pts',(31.4105224635298,64.2151008537733,0.));
#164177=CARTESIAN_POINT('Ctrl Pts',(31.3942974463458,64.1988029019733,0.));
#164178=CARTESIAN_POINT('Ctrl Pts',(31.3781202823758,64.1825205366231,0.));
#164179=CARTESIAN_POINT('Ctrl Pts',(31.3619910181222,64.1662538995407,0.));
#164180=CARTESIAN_POINT('Ctrl Pts',(31.3459097001995,64.150003133226,0.));
#164181=CARTESIAN_POINT('Ctrl Pts',(31.3298763753366,64.1337683808667,0.));
#164182=CARTESIAN_POINT('Ctrl Pts',(31.3138910903852,64.1175497863475,0.));
#164183=CARTESIAN_POINT('Ctrl Pts',(31.2979538923213,64.1013474942554,0.));
#164184=CARTESIAN_POINT('Ctrl Pts',(31.2820648282451,64.0851616498861,0.));
#164185=CARTESIAN_POINT('Ctrl Pts',(31.2662239453734,64.0689923992475,0.));
#164186=CARTESIAN_POINT('Ctrl Pts',(31.2504312910457,64.0528398890671,0.));
#164187=CARTESIAN_POINT('Ctrl Pts',(31.23468691273,64.036704266799,0.));
#164188=CARTESIAN_POINT('Ctrl Pts',(31.2189908580245,64.0205856806298,0.));
#164189=CARTESIAN_POINT('Ctrl Pts',(31.2033431746558,64.004484279483,0.));
#164190=CARTESIAN_POINT('Ctrl Pts',(31.1877439104717,63.9884002130209,0.));
#164191=CARTESIAN_POINT('Ctrl Pts',(31.1721931134488,63.972333631655,0.));
#164192=CARTESIAN_POINT('Ctrl Pts',(31.1566908316992,63.9562846865566,0.));
#164193=CARTESIAN_POINT('Ctrl Pts',(31.1412371134727,63.9402535296651,0.));
#164194=CARTESIAN_POINT('Ctrl Pts',(31.1258320071545,63.9242403136954,0.));
#164195=CARTESIAN_POINT('Ctrl Pts',(31.1104755612606,63.9082451921447,0.));
#164196=CARTESIAN_POINT('Ctrl Pts',(31.0951678244454,63.8922683192963,0.));
#164197=CARTESIAN_POINT('Ctrl Pts',(31.079908845504,63.8763098502235,0.));
#164198=CARTESIAN_POINT('Ctrl Pts',(31.0646986733723,63.8603699407922,0.));
#164199=CARTESIAN_POINT('Ctrl Pts',(31.0495373571217,63.8444487476615,0.));
#164200=CARTESIAN_POINT('Ctrl Pts',(31.0344249459544,63.8285464282857,0.));
#164201=CARTESIAN_POINT('Ctrl Pts',(31.0193614892177,63.8126631409376,0.));
#164202=CARTESIAN_POINT('Ctrl Pts',(31.0043470364112,63.7967990447288,0.));
#164203=CARTESIAN_POINT('Ctrl Pts',(30.9893816371907,63.7809542996258,0.));
#164204=CARTESIAN_POINT('Ctrl Pts',(30.9744653413679,63.7651290664713,0.));
#164205=CARTESIAN_POINT('Ctrl Pts',(30.9595981989091,63.7493235069844,0.));
#164206=CARTESIAN_POINT('Ctrl Pts',(30.9447802599345,63.733537783742,0.));
#164207=CARTESIAN_POINT('Ctrl Pts',(30.9300115747113,63.7177720601604,0.));
#164208=CARTESIAN_POINT('Ctrl Pts',(30.9152921936471,63.7020265004805,0.));
#164209=CARTESIAN_POINT('Ctrl Pts',(30.9006221672703,63.6863012697354,0.));
#164210=CARTESIAN_POINT('Ctrl Pts',(30.8860015462488,63.6705965337996,0.));
#164211=CARTESIAN_POINT('Ctrl Pts',(30.8714303814202,63.6549124594681,0.));
#164212=CARTESIAN_POINT('Ctrl Pts',(30.8569087238131,63.6392492145233,0.));
#164213=CARTESIAN_POINT('Ctrl Pts',(30.8424366246665,63.6236069678041,0.));
#164214=CARTESIAN_POINT('Ctrl Pts',(30.8280141354447,63.6079858892747,0.));
#164215=CARTESIAN_POINT('Ctrl Pts',(30.8136413077999,63.5923861498964,0.));
#164216=CARTESIAN_POINT('Ctrl Pts',(30.7993181935265,63.5768079214868,0.));
#164217=CARTESIAN_POINT('Ctrl Pts',(30.7850448445207,63.5612513766005,0.));
#164218=CARTESIAN_POINT('Ctrl Pts',(30.7708213127169,63.5457166883558,0.));
#164219=CARTESIAN_POINT('Ctrl Pts',(30.7566476500772,63.5302040304173,0.));
#164220=CARTESIAN_POINT('Ctrl Pts',(30.7425239087294,63.514713577392,0.));
#164221=CARTESIAN_POINT('Ctrl Pts',(30.7284501410827,63.4992455051805,0.));
#164222=CARTESIAN_POINT('Ctrl Pts',(30.7144263999259,63.4837999912758,0.));
#164223=CARTESIAN_POINT('Ctrl Pts',(30.7004527385806,63.4683772152497,0.));
#164224=CARTESIAN_POINT('Ctrl Pts',(30.686529210791,63.4529773584211,0.));
#164225=CARTESIAN_POINT('Ctrl Pts',(30.6726558704301,63.4376006029575,0.));
#164226=CARTESIAN_POINT('Ctrl Pts',(30.6588327712482,63.4222471311236,0.));
#164227=CARTESIAN_POINT('Ctrl Pts',(30.6450599666135,63.4069171245094,0.));
#164228=CARTESIAN_POINT('Ctrl Pts',(30.6313375092084,63.3916107631421,0.));
#164229=CARTESIAN_POINT('Ctrl Pts',(30.6176654515988,63.3763282271838,0.));
#164230=CARTESIAN_POINT('Ctrl Pts',(30.6040438469089,63.3610696989599,0.));
#164231=CARTESIAN_POINT('Ctrl Pts',(30.5904727493707,63.3458353646144,0.));
#164232=CARTESIAN_POINT('Ctrl Pts',(30.5769522151147,63.330625416509,0.));
#164233=CARTESIAN_POINT('Ctrl Pts',(30.5634823022358,63.315440053435,0.));
#164234=CARTESIAN_POINT('Ctrl Pts',(30.5500630691342,63.300279475605,0.));
#164235=CARTESIAN_POINT('Ctrl Pts',(30.5366945730503,63.2851438802462,0.));
#164236=CARTESIAN_POINT('Ctrl Pts',(30.5233768687875,63.2700334577661,0.));
#164237=CARTESIAN_POINT('Ctrl Pts',(30.5101100066683,63.2549483856268,0.));
#164238=CARTESIAN_POINT('Ctrl Pts',(30.4968940345027,63.2398888342612,0.));
#164239=CARTESIAN_POINT('Ctrl Pts',(30.4837290015011,63.2248549788272,0.));
#164240=CARTESIAN_POINT('Ctrl Pts',(30.470614961416,63.2098470086636,0.));
#164241=CARTESIAN_POINT('Ctrl Pts',(30.4575519763305,63.1948651386868,0.));
#164242=CARTESIAN_POINT('Ctrl Pts',(30.4445401192324,63.1799096171757,0.));
#164243=CARTESIAN_POINT('Ctrl Pts',(30.431579465967,63.1649807016766,0.));
#164244=CARTESIAN_POINT('Ctrl Pts',(30.4186700875598,63.1500786361382,0.));
#164245=CARTESIAN_POINT('Ctrl Pts',(30.4058120432259,63.1352036298512,0.));
#164246=CARTESIAN_POINT('Ctrl Pts',(30.3930053710592,63.1203558300911,0.));
#164247=CARTESIAN_POINT('Ctrl Pts',(30.3802500880565,63.1055353202641,0.));
#164248=CARTESIAN_POINT('Ctrl Pts',(30.3700869762658,63.0937007763826,0.));
#164249=CARTESIAN_POINT('Ctrl Pts',(30.3624877680747,63.0848371718274,0.));
#164250=CARTESIAN_POINT('Ctrl Pts',(30.3574319069365,63.0789335700774,0.));
#164251=CARTESIAN_POINT('Ctrl Pts',(30.3549065457811,63.0759831361898,0.));
#164252=CARTESIAN_POINT('Ctrl Pts',(39.5004851439258,63.1661434108059,0.));
#164253=CARTESIAN_POINT('Ctrl Pts',(39.5004851439258,63.1661434108059,12.));
#164254=CARTESIAN_POINT('Ctrl Pts',(39.4958045828135,63.1630766582788,0.));
#164255=CARTESIAN_POINT('Ctrl Pts',(39.4958045828135,63.1630766582788,12.));
#164256=CARTESIAN_POINT('Ctrl Pts',(39.4864477303823,63.1569429707875,0.));
#164257=CARTESIAN_POINT('Ctrl Pts',(39.4864477303823,63.1569429707875,12.));
#164258=CARTESIAN_POINT('Ctrl Pts',(39.4724252611155,63.1477418922406,0.));
#164259=CARTESIAN_POINT('Ctrl Pts',(39.4724252611155,63.1477418922406,12.));
#164260=CARTESIAN_POINT('Ctrl Pts',(39.4537542552268,63.1354726928398,0.));
#164261=CARTESIAN_POINT('Ctrl Pts',(39.4537542552268,63.1354726928398,12.));
#164262=CARTESIAN_POINT('Ctrl Pts',(39.4304582059864,63.1201343731172,0.));
#164263=CARTESIAN_POINT('Ctrl Pts',(39.4304582059864,63.1201343731172,12.));
#164264=CARTESIAN_POINT('Ctrl Pts',(39.4072048797615,63.10479424519,0.));
#164265=CARTESIAN_POINT('Ctrl Pts',(39.4072048797615,63.10479424519,12.));
#164266=CARTESIAN_POINT('Ctrl Pts',(39.3839942985739,63.0894523341314,0.));
#164267=CARTESIAN_POINT('Ctrl Pts',(39.3839942985739,63.0894523341314,12.));
#164268=CARTESIAN_POINT('Ctrl Pts',(39.3608264920409,63.0741086815841,0.));
#164269=CARTESIAN_POINT('Ctrl Pts',(39.3608264920409,63.0741086815841,12.));
#164270=CARTESIAN_POINT('Ctrl Pts',(39.3377014983609,63.0587633513774,0.));
#164271=CARTESIAN_POINT('Ctrl Pts',(39.3377014983609,63.0587633513774,12.));
#164272=CARTESIAN_POINT('Ctrl Pts',(39.3146193632392,63.0434164277992,0.));
#164273=CARTESIAN_POINT('Ctrl Pts',(39.3146193632392,63.0434164277992,12.));
#164274=CARTESIAN_POINT('Ctrl Pts',(39.2915801372354,63.0280680082353,0.));
#164275=CARTESIAN_POINT('Ctrl Pts',(39.2915801372354,63.0280680082353,12.));
#164276=CARTESIAN_POINT('Ctrl Pts',(39.2685838735361,63.0127181973628,0.));
#164277=CARTESIAN_POINT('Ctrl Pts',(39.2685838735361,63.0127181973628,12.));
#164278=CARTESIAN_POINT('Ctrl Pts',(39.2456306256104,62.9973671008704,0.));
#164279=CARTESIAN_POINT('Ctrl Pts',(39.2456306256104,62.9973671008704,12.));
#164280=CARTESIAN_POINT('Ctrl Pts',(39.2227204447638,62.9820148189929,0.));
#164281=CARTESIAN_POINT('Ctrl Pts',(39.2227204447638,62.9820148189929,12.));
#164282=CARTESIAN_POINT('Ctrl Pts',(39.199853378166,62.9666614412731,0.));
#164283=CARTESIAN_POINT('Ctrl Pts',(39.199853378166,62.9666614412731,12.));
#164284=CARTESIAN_POINT('Ctrl Pts',(39.1770294702428,62.9513070501867,0.));
#164285=CARTESIAN_POINT('Ctrl Pts',(39.1770294702428,62.9513070501867,12.));
#164286=CARTESIAN_POINT('Ctrl Pts',(39.1542487636743,62.9359517237404,0.));
#164287=CARTESIAN_POINT('Ctrl Pts',(39.1542487636743,62.9359517237404,12.));
#164288=CARTESIAN_POINT('Ctrl Pts',(39.131511300575,62.9205955385558,0.));
#164289=CARTESIAN_POINT('Ctrl Pts',(39.131511300575,62.9205955385558,12.));
#164290=CARTESIAN_POINT('Ctrl Pts',(39.1088171235125,62.9052385725388,0.));
#164291=CARTESIAN_POINT('Ctrl Pts',(39.1088171235125,62.9052385725388,12.));
#164292=CARTESIAN_POINT('Ctrl Pts',(39.0861662767932,62.8898809082612,0.));
#164293=CARTESIAN_POINT('Ctrl Pts',(39.0861662767932,62.8898809082612,12.));
#164294=CARTESIAN_POINT('Ctrl Pts',(39.0635588063276,62.8745226325998,0.));
#164295=CARTESIAN_POINT('Ctrl Pts',(39.0635588063276,62.8745226325998,12.));
#164296=CARTESIAN_POINT('Ctrl Pts',(39.0409947590496,62.8591638352056,0.));
#164297=CARTESIAN_POINT('Ctrl Pts',(39.0409947590496,62.8591638352056,12.));
#164298=CARTESIAN_POINT('Ctrl Pts',(39.0184741824641,62.8438046073224,0.));
#164299=CARTESIAN_POINT('Ctrl Pts',(39.0184741824641,62.8438046073224,12.));
#164300=CARTESIAN_POINT('Ctrl Pts',(38.9959971241701,62.8284450405459,0.));
#164301=CARTESIAN_POINT('Ctrl Pts',(38.9959971241701,62.8284450405459,12.));
#164302=CARTESIAN_POINT('Ctrl Pts',(38.9735636313088,62.8130852254027,0.));
#164303=CARTESIAN_POINT('Ctrl Pts',(38.9735636313088,62.8130852254027,12.));
#164304=CARTESIAN_POINT('Ctrl Pts',(38.9511737503165,62.7977252507118,0.));
#164305=CARTESIAN_POINT('Ctrl Pts',(38.9511737503165,62.7977252507118,12.));
#164306=CARTESIAN_POINT('Ctrl Pts',(38.9288275272335,62.78236520437,0.));
#164307=CARTESIAN_POINT('Ctrl Pts',(38.9288275272335,62.78236520437,12.));
#164308=CARTESIAN_POINT('Ctrl Pts',(38.9065250078832,62.7670051738143,0.));
#164309=CARTESIAN_POINT('Ctrl Pts',(38.9065250078832,62.7670051738143,12.));
#164310=CARTESIAN_POINT('Ctrl Pts',(38.8842662380984,62.7516452466128,0.));
#164311=CARTESIAN_POINT('Ctrl Pts',(38.8842662380984,62.7516452466128,12.));
#164312=CARTESIAN_POINT('Ctrl Pts',(38.8620512639232,62.7362855110042,0.));
#164313=CARTESIAN_POINT('Ctrl Pts',(38.8620512639232,62.7362855110042,12.));
#164314=CARTESIAN_POINT('Ctrl Pts',(38.8398801318176,62.7209260564493,0.));
#164315=CARTESIAN_POINT('Ctrl Pts',(38.8398801318176,62.7209260564493,12.));
#164316=CARTESIAN_POINT('Ctrl Pts',(38.8177528885681,62.7055669733802,0.));
#164317=CARTESIAN_POINT('Ctrl Pts',(38.8177528885681,62.7055669733802,12.));
#164318=CARTESIAN_POINT('Ctrl Pts',(38.795669581203,62.6902083529695,0.));
#164319=CARTESIAN_POINT('Ctrl Pts',(38.795669581203,62.6902083529695,12.));
#164320=CARTESIAN_POINT('Ctrl Pts',(38.7736302568982,62.6748502868835,0.));
#164321=CARTESIAN_POINT('Ctrl Pts',(38.7736302568982,62.6748502868835,12.));
#164322=CARTESIAN_POINT('Ctrl Pts',(38.7516349628903,62.6594928670628,0.));
#164323=CARTESIAN_POINT('Ctrl Pts',(38.7516349628903,62.6594928670628,12.));
#164324=CARTESIAN_POINT('Ctrl Pts',(38.7296837463608,62.6441361854411,0.));
#164325=CARTESIAN_POINT('Ctrl Pts',(38.7296837463608,62.6441361854411,12.));
#164326=CARTESIAN_POINT('Ctrl Pts',(38.7077766544416,62.6287803339542,0.));
#164327=CARTESIAN_POINT('Ctrl Pts',(38.7077766544416,62.6287803339542,12.));
#164328=CARTESIAN_POINT('Ctrl Pts',(38.685913734273,62.6134254046739,0.));
#164329=CARTESIAN_POINT('Ctrl Pts',(38.685913734273,62.6134254046739,12.));
#164330=CARTESIAN_POINT('Ctrl Pts',(38.6640950330421,62.5980714899052,0.));
#164331=CARTESIAN_POINT('Ctrl Pts',(38.6640950330421,62.5980714899052,12.));
#164332=CARTESIAN_POINT('Ctrl Pts',(38.6423205980213,62.5827186822921,0.));
#164333=CARTESIAN_POINT('Ctrl Pts',(38.6423205980213,62.5827186822921,12.));
#164334=CARTESIAN_POINT('Ctrl Pts',(38.6205904766072,62.5673670749362,0.));
#164335=CARTESIAN_POINT('Ctrl Pts',(38.6205904766072,62.5673670749362,12.));
#164336=CARTESIAN_POINT('Ctrl Pts',(38.5989047163393,62.5520167614516,0.));
#164337=CARTESIAN_POINT('Ctrl Pts',(38.5989047163393,62.5520167614516,12.));
#164338=CARTESIAN_POINT('Ctrl Pts',(38.5772633648832,62.5366678359023,0.));
#164339=CARTESIAN_POINT('Ctrl Pts',(38.5772633648832,62.5366678359023,12.));
#164340=CARTESIAN_POINT('Ctrl Pts',(38.5556664700195,62.5213203927663,0.));
#164341=CARTESIAN_POINT('Ctrl Pts',(38.5556664700195,62.5213203927663,12.));
#164342=CARTESIAN_POINT('Ctrl Pts',(38.5341140796248,62.5059745268901,0.));
#164343=CARTESIAN_POINT('Ctrl Pts',(38.5341140796248,62.5059745268901,12.));
#164344=CARTESIAN_POINT('Ctrl Pts',(38.5126062416502,62.4906303334443,0.));
#164345=CARTESIAN_POINT('Ctrl Pts',(38.5126062416502,62.4906303334443,12.));
#164346=CARTESIAN_POINT('Ctrl Pts',(38.4911430040997,62.4752879078854,0.));
#164347=CARTESIAN_POINT('Ctrl Pts',(38.4911430040997,62.4752879078854,12.));
#164348=CARTESIAN_POINT('Ctrl Pts',(38.4697244150482,62.4599473459811,0.));
#164349=CARTESIAN_POINT('Ctrl Pts',(38.4697244150482,62.4599473459811,12.));
#164350=CARTESIAN_POINT('Ctrl Pts',(38.4483505226518,62.4446087438312,0.));
#164351=CARTESIAN_POINT('Ctrl Pts',(38.4483505226518,62.4446087438312,12.));
#164352=CARTESIAN_POINT('Ctrl Pts',(38.4270213751568,62.4292721978901,0.));
#164353=CARTESIAN_POINT('Ctrl Pts',(38.4270213751568,62.4292721978901,12.));
#164354=CARTESIAN_POINT('Ctrl Pts',(38.405737020905,62.4139378049886,0.));
#164355=CARTESIAN_POINT('Ctrl Pts',(38.405737020905,62.4139378049886,12.));
#164356=CARTESIAN_POINT('Ctrl Pts',(38.3844975083343,62.3986056623577,0.));
#164357=CARTESIAN_POINT('Ctrl Pts',(38.3844975083343,62.3986056623577,12.));
#164358=CARTESIAN_POINT('Ctrl Pts',(38.3633028859828,62.3832758676271,0.));
#164359=CARTESIAN_POINT('Ctrl Pts',(38.3633028859828,62.3832758676271,12.));
#164360=CARTESIAN_POINT('Ctrl Pts',(38.342153202491,62.3679485188172,0.));
#164361=CARTESIAN_POINT('Ctrl Pts',(38.342153202491,62.3679485188172,12.));
#164362=CARTESIAN_POINT('Ctrl Pts',(38.3210485066001,62.3526237143336,0.));
#164363=CARTESIAN_POINT('Ctrl Pts',(38.3210485066001,62.3526237143336,12.));
#164364=CARTESIAN_POINT('Ctrl Pts',(38.2999888471476,62.3373015529613,0.));
#164365=CARTESIAN_POINT('Ctrl Pts',(38.2999888471476,62.3373015529613,12.));
#164366=CARTESIAN_POINT('Ctrl Pts',(38.2789742730563,62.3219821338569,0.));
#164367=CARTESIAN_POINT('Ctrl Pts',(38.2789742730563,62.3219821338569,12.));
#164368=CARTESIAN_POINT('Ctrl Pts',(38.258004833336,62.3066655565503,0.));
#164369=CARTESIAN_POINT('Ctrl Pts',(38.258004833336,62.3066655565503,12.));
#164370=CARTESIAN_POINT('Ctrl Pts',(38.2370805770935,62.2913519209521,0.));
#164371=CARTESIAN_POINT('Ctrl Pts',(38.2370805770935,62.2913519209521,12.));
#164372=CARTESIAN_POINT('Ctrl Pts',(38.2162015535352,62.2760413273602,0.));
#164373=CARTESIAN_POINT('Ctrl Pts',(38.2162015535352,62.2760413273602,12.));
#164374=CARTESIAN_POINT('Ctrl Pts',(38.1953678119691,62.2607338764654,0.));
#164375=CARTESIAN_POINT('Ctrl Pts',(38.1953678119691,62.2607338764654,12.));
#164376=CARTESIAN_POINT('Ctrl Pts',(38.1745794017995,62.245429669358,0.));
#164377=CARTESIAN_POINT('Ctrl Pts',(38.1745794017995,62.245429669358,12.));
#164378=CARTESIAN_POINT('Ctrl Pts',(38.1538363725263,62.2301288075321,0.));
#164379=CARTESIAN_POINT('Ctrl Pts',(38.1538363725263,62.2301288075321,12.));
#164380=CARTESIAN_POINT('Ctrl Pts',(38.1331387737529,62.2148313928863,0.));
#164381=CARTESIAN_POINT('Ctrl Pts',(38.1331387737529,62.2148313928863,12.));
#164382=CARTESIAN_POINT('Ctrl Pts',(38.1124866551885,62.1995375277257,0.));
#164383=CARTESIAN_POINT('Ctrl Pts',(38.1124866551885,62.1995375277257,12.));
#164384=CARTESIAN_POINT('Ctrl Pts',(38.0918800666479,62.1842473147626,0.));
#164385=CARTESIAN_POINT('Ctrl Pts',(38.0918800666479,62.1842473147626,12.));
#164386=CARTESIAN_POINT('Ctrl Pts',(38.0713190580463,62.1689608571176,0.));
#164387=CARTESIAN_POINT('Ctrl Pts',(38.0713190580463,62.1689608571176,12.));
#164388=CARTESIAN_POINT('Ctrl Pts',(38.0508036793939,62.1536782583199,0.));
#164389=CARTESIAN_POINT('Ctrl Pts',(38.0508036793939,62.1536782583199,12.));
#164390=CARTESIAN_POINT('Ctrl Pts',(38.0303339808053,62.1383996223125,0.));
#164391=CARTESIAN_POINT('Ctrl Pts',(38.0303339808053,62.1383996223125,12.));
#164392=CARTESIAN_POINT('Ctrl Pts',(38.0099100125037,62.123125053455,0.));
#164393=CARTESIAN_POINT('Ctrl Pts',(38.0099100125037,62.123125053455,12.));
#164394=CARTESIAN_POINT('Ctrl Pts',(37.9895318248212,62.107854656528,0.));
#164395=CARTESIAN_POINT('Ctrl Pts',(37.9895318248212,62.107854656528,12.));
#164396=CARTESIAN_POINT('Ctrl Pts',(37.9691994681966,62.0925885367352,0.));
#164397=CARTESIAN_POINT('Ctrl Pts',(37.9691994681966,62.0925885367352,12.));
#164398=CARTESIAN_POINT('Ctrl Pts',(37.9489129931688,62.0773267997079,0.));
#164399=CARTESIAN_POINT('Ctrl Pts',(37.9489129931688,62.0773267997079,12.));
#164400=CARTESIAN_POINT('Ctrl Pts',(37.9286724503851,62.0620695515075,0.));
#164401=CARTESIAN_POINT('Ctrl Pts',(37.9286724503851,62.0620695515075,12.));
#164402=CARTESIAN_POINT('Ctrl Pts',(37.9084778906053,62.0468168986288,0.));
#164403=CARTESIAN_POINT('Ctrl Pts',(37.9084778906053,62.0468168986288,12.));
#164404=CARTESIAN_POINT('Ctrl Pts',(37.8883293647029,62.031568948002,0.));
#164405=CARTESIAN_POINT('Ctrl Pts',(37.8883293647029,62.031568948002,12.));
#164406=CARTESIAN_POINT('Ctrl Pts',(37.868226923663,62.0163258069957,0.));
#164407=CARTESIAN_POINT('Ctrl Pts',(37.868226923663,62.0163258069957,12.));
#164408=CARTESIAN_POINT('Ctrl Pts',(37.8481706185749,62.0010875834187,0.));
#164409=CARTESIAN_POINT('Ctrl Pts',(37.8481706185749,62.0010875834187,12.));
#164410=CARTESIAN_POINT('Ctrl Pts',(37.828160500638,61.9858543855236,0.));
#164411=CARTESIAN_POINT('Ctrl Pts',(37.828160500638,61.9858543855236,12.));
#164412=CARTESIAN_POINT('Ctrl Pts',(37.8081966211688,61.9706263220114,0.));
#164413=CARTESIAN_POINT('Ctrl Pts',(37.8081966211688,61.9706263220114,12.));
#164414=CARTESIAN_POINT('Ctrl Pts',(37.7882790316014,61.9554035020338,0.));
#164415=CARTESIAN_POINT('Ctrl Pts',(37.7882790316014,61.9554035020338,12.));
#164416=CARTESIAN_POINT('Ctrl Pts',(37.7684077834872,61.9401860351973,0.));
#164417=CARTESIAN_POINT('Ctrl Pts',(37.7684077834872,61.9401860351973,12.));
#164418=CARTESIAN_POINT('Ctrl Pts',(37.7485829284871,61.9249740315649,0.));
#164419=CARTESIAN_POINT('Ctrl Pts',(37.7485829284871,61.9249740315649,12.));
#164420=CARTESIAN_POINT('Ctrl Pts',(37.7288045183756,61.9097676016601,0.));
#164421=CARTESIAN_POINT('Ctrl Pts',(37.7288045183756,61.9097676016601,12.));
#164422=CARTESIAN_POINT('Ctrl Pts',(37.7090726050482,61.8945668564704,0.));
#164423=CARTESIAN_POINT('Ctrl Pts',(37.7090726050482,61.8945668564704,12.));
#164424=CARTESIAN_POINT('Ctrl Pts',(37.6893872405228,61.8793719074507,0.));
#164425=CARTESIAN_POINT('Ctrl Pts',(37.6893872405228,61.8793719074507,12.));
#164426=CARTESIAN_POINT('Ctrl Pts',(37.6697484769392,61.8641828665262,0.));
#164427=CARTESIAN_POINT('Ctrl Pts',(37.6697484769392,61.8641828665262,12.));
#164428=CARTESIAN_POINT('Ctrl Pts',(37.6501563665523,61.8489998460957,0.));
#164429=CARTESIAN_POINT('Ctrl Pts',(37.6501563665523,61.8489998460957,12.));
#164430=CARTESIAN_POINT('Ctrl Pts',(37.6306109617346,61.8338229590353,0.));
#164431=CARTESIAN_POINT('Ctrl Pts',(37.6306109617346,61.8338229590353,12.));
#164432=CARTESIAN_POINT('Ctrl Pts',(37.6111123149839,61.8186523187015,0.));
#164433=CARTESIAN_POINT('Ctrl Pts',(37.6111123149839,61.8186523187015,12.));
#164434=CARTESIAN_POINT('Ctrl Pts',(37.5916604789253,61.8034880389363,0.));
#164435=CARTESIAN_POINT('Ctrl Pts',(37.5916604789253,61.8034880389363,12.));
#164436=CARTESIAN_POINT('Ctrl Pts',(37.5722555063111,61.7883302340687,0.));
#164437=CARTESIAN_POINT('Ctrl Pts',(37.5722555063111,61.7883302340687,12.));
#164438=CARTESIAN_POINT('Ctrl Pts',(37.5528974500141,61.7731790189191,0.));
#164439=CARTESIAN_POINT('Ctrl Pts',(37.5528974500141,61.7731790189191,12.));
#164440=CARTESIAN_POINT('Ctrl Pts',(37.5335863630287,61.7580345088016,0.));
#164441=CARTESIAN_POINT('Ctrl Pts',(37.5335863630287,61.7580345088016,12.));
#164442=CARTESIAN_POINT('Ctrl Pts',(37.5143222984795,61.7428968195299,0.));
#164443=CARTESIAN_POINT('Ctrl Pts',(37.5143222984795,61.7428968195299,12.));
#164444=CARTESIAN_POINT('Ctrl Pts',(37.4951053096237,61.7277660674205,0.));
#164445=CARTESIAN_POINT('Ctrl Pts',(37.4951053096237,61.7277660674205,12.));
#164446=CARTESIAN_POINT('Ctrl Pts',(37.4759354498509,61.7126423692963,0.));
#164447=CARTESIAN_POINT('Ctrl Pts',(37.4759354498509,61.7126423692963,12.));
#164448=CARTESIAN_POINT('Ctrl Pts',(37.4568127726773,61.6975258424894,0.));
#164449=CARTESIAN_POINT('Ctrl Pts',(37.4568127726773,61.6975258424894,12.));
#164450=CARTESIAN_POINT('Ctrl Pts',(37.4377373317451,61.6824166048444,0.));
#164451=CARTESIAN_POINT('Ctrl Pts',(37.4377373317451,61.6824166048444,12.));
#164452=CARTESIAN_POINT('Ctrl Pts',(37.418709180832,61.6673147747242,0.));
#164453=CARTESIAN_POINT('Ctrl Pts',(37.418709180832,61.6673147747242,12.));
#164454=CARTESIAN_POINT('Ctrl Pts',(37.3997283738533,61.6522204710131,0.));
#164455=CARTESIAN_POINT('Ctrl Pts',(37.3997283738533,61.6522204710131,12.));
#164456=CARTESIAN_POINT('Ctrl Pts',(37.3807949648624,61.637133813121,0.));
#164457=CARTESIAN_POINT('Ctrl Pts',(37.3807949648624,61.637133813121,12.));
#164458=CARTESIAN_POINT('Ctrl Pts',(37.3619090080449,61.6220549209866,0.));
#164459=CARTESIAN_POINT('Ctrl Pts',(37.3619090080449,61.6220549209866,12.));
#164460=CARTESIAN_POINT('Ctrl Pts',(37.343070557718,61.6069839150807,0.));
#164461=CARTESIAN_POINT('Ctrl Pts',(37.343070557718,61.6069839150807,12.));
#164462=CARTESIAN_POINT('Ctrl Pts',(37.3242796683395,61.591920916412,0.));
#164463=CARTESIAN_POINT('Ctrl Pts',(37.3242796683395,61.591920916412,12.));
#164464=CARTESIAN_POINT('Ctrl Pts',(37.3055363945107,61.5768660465311,0.));
#164465=CARTESIAN_POINT('Ctrl Pts',(37.3055363945107,61.5768660465311,12.));
#164466=CARTESIAN_POINT('Ctrl Pts',(37.286840790977,61.5618194275348,0.));
#164467=CARTESIAN_POINT('Ctrl Pts',(37.286840790977,61.5618194275348,12.));
#164468=CARTESIAN_POINT('Ctrl Pts',(37.2681929126221,61.5467811820691,0.));
#164469=CARTESIAN_POINT('Ctrl Pts',(37.2681929126221,61.5467811820691,12.));
#164470=CARTESIAN_POINT('Ctrl Pts',(37.2495928144666,61.5317514333328,0.));
#164471=CARTESIAN_POINT('Ctrl Pts',(37.2495928144666,61.5317514333328,12.));
#164472=CARTESIAN_POINT('Ctrl Pts',(37.2310405516781,61.5167303050832,0.));
#164473=CARTESIAN_POINT('Ctrl Pts',(37.2310405516781,61.5167303050832,12.));
#164474=CARTESIAN_POINT('Ctrl Pts',(37.2125361795731,61.501717921641,0.));
#164475=CARTESIAN_POINT('Ctrl Pts',(37.2125361795731,61.501717921641,12.));
#164476=CARTESIAN_POINT('Ctrl Pts',(37.1940797536181,61.4867144078937,0.));
#164477=CARTESIAN_POINT('Ctrl Pts',(37.1940797536181,61.4867144078937,12.));
#164478=CARTESIAN_POINT('Ctrl Pts',(37.175671329424,61.4717198892994,0.));
#164479=CARTESIAN_POINT('Ctrl Pts',(37.175671329424,61.4717198892994,12.));
#164480=CARTESIAN_POINT('Ctrl Pts',(37.1573109627454,61.456734491892,0.));
#164481=CARTESIAN_POINT('Ctrl Pts',(37.1573109627454,61.456734491892,12.));
#164482=CARTESIAN_POINT('Ctrl Pts',(37.1389987094904,61.4417583422863,0.));
#164483=CARTESIAN_POINT('Ctrl Pts',(37.1389987094904,61.4417583422863,12.));
#164484=CARTESIAN_POINT('Ctrl Pts',(37.1207346257221,61.4267915676822,0.));
#164485=CARTESIAN_POINT('Ctrl Pts',(37.1207346257221,61.4267915676822,12.));
#164486=CARTESIAN_POINT('Ctrl Pts',(37.1025187676602,61.4118342958697,0.));
#164487=CARTESIAN_POINT('Ctrl Pts',(37.1025187676602,61.4118342958697,12.));
#164488=CARTESIAN_POINT('Ctrl Pts',(37.0843511916744,61.3968866552318,0.));
#164489=CARTESIAN_POINT('Ctrl Pts',(37.0843511916744,61.3968866552318,12.));
#164490=CARTESIAN_POINT('Ctrl Pts',(37.0662319542849,61.381948774749,0.));
#164491=CARTESIAN_POINT('Ctrl Pts',(37.0662319542849,61.381948774749,12.));
#164492=CARTESIAN_POINT('Ctrl Pts',(37.0481611121717,61.3670207840069,0.));
#164493=CARTESIAN_POINT('Ctrl Pts',(37.0481611121717,61.3670207840069,12.));
#164494=CARTESIAN_POINT('Ctrl Pts',(37.0301387221774,61.3521028132003,0.));
#164495=CARTESIAN_POINT('Ctrl Pts',(37.0301387221774,61.3521028132003,12.));
#164496=CARTESIAN_POINT('Ctrl Pts',(37.0121648413081,61.3371949931387,0.));
#164497=CARTESIAN_POINT('Ctrl Pts',(37.0121648413081,61.3371949931387,12.));
#164498=CARTESIAN_POINT('Ctrl Pts',(36.994239526727,61.3222974552487,0.));
#164499=CARTESIAN_POINT('Ctrl Pts',(36.994239526727,61.3222974552487,12.));
#164500=CARTESIAN_POINT('Ctrl Pts',(36.9763628357544,61.3074103315792,0.));
#164501=CARTESIAN_POINT('Ctrl Pts',(36.9763628357544,61.3074103315792,12.));
#164502=CARTESIAN_POINT('Ctrl Pts',(36.9585348258776,61.2925337548077,0.));
#164503=CARTESIAN_POINT('Ctrl Pts',(36.9585348258776,61.2925337548077,12.));
#164504=CARTESIAN_POINT('Ctrl Pts',(36.9407555547534,61.2776678582461,0.));
#164505=CARTESIAN_POINT('Ctrl Pts',(36.9407555547534,61.2776678582461,12.));
#164506=CARTESIAN_POINT('Ctrl Pts',(36.9230250802087,61.2628127758457,0.));
#164507=CARTESIAN_POINT('Ctrl Pts',(36.9230250802087,61.2628127758457,12.));
#164508=CARTESIAN_POINT('Ctrl Pts',(36.9053434602343,61.247968642201,0.));
#164509=CARTESIAN_POINT('Ctrl Pts',(36.9053434602343,61.247968642201,12.));
#164510=CARTESIAN_POINT('Ctrl Pts',(36.8877107529865,61.2331355925547,0.));
#164511=CARTESIAN_POINT('Ctrl Pts',(36.8877107529865,61.2331355925547,12.));
#164512=CARTESIAN_POINT('Ctrl Pts',(36.8701270167969,61.2183137628056,0.));
#164513=CARTESIAN_POINT('Ctrl Pts',(36.8701270167969,61.2183137628056,12.));
#164514=CARTESIAN_POINT('Ctrl Pts',(36.852592310174,61.2035032895127,0.));
#164515=CARTESIAN_POINT('Ctrl Pts',(36.852592310174,61.2035032895127,12.));
#164516=CARTESIAN_POINT('Ctrl Pts',(36.8351066918036,61.1887043099014,0.));
#164517=CARTESIAN_POINT('Ctrl Pts',(36.8351066918036,61.1887043099014,12.));
#164518=CARTESIAN_POINT('Ctrl Pts',(36.8176702205423,61.1739169618667,0.));
#164519=CARTESIAN_POINT('Ctrl Pts',(36.8176702205423,61.1739169618667,12.));
#164520=CARTESIAN_POINT('Ctrl Pts',(36.8002829554209,61.1591413839787,0.));
#164521=CARTESIAN_POINT('Ctrl Pts',(36.8002829554209,61.1591413839787,12.));
#164522=CARTESIAN_POINT('Ctrl Pts',(36.7829449556532,61.1443777154911,0.));
#164523=CARTESIAN_POINT('Ctrl Pts',(36.7829449556532,61.1443777154911,12.));
#164524=CARTESIAN_POINT('Ctrl Pts',(36.765656280638,61.1296260963466,0.));
#164525=CARTESIAN_POINT('Ctrl Pts',(36.765656280638,61.1296260963466,12.));
#164526=CARTESIAN_POINT('Ctrl Pts',(36.7484169899596,61.1148866671829,0.));
#164527=CARTESIAN_POINT('Ctrl Pts',(36.7484169899596,61.1148866671829,12.));
#164528=CARTESIAN_POINT('Ctrl Pts',(36.7312271433807,61.100159569337,0.));
#164529=CARTESIAN_POINT('Ctrl Pts',(36.7312271433807,61.100159569337,12.));
#164530=CARTESIAN_POINT('Ctrl Pts',(36.7140868008486,61.0854449448524,0.));
#164531=CARTESIAN_POINT('Ctrl Pts',(36.7140868008486,61.0854449448524,12.));
#164532=CARTESIAN_POINT('Ctrl Pts',(36.6969960225022,61.0707429364847,0.));
#164533=CARTESIAN_POINT('Ctrl Pts',(36.6969960225022,61.0707429364847,12.));
#164534=CARTESIAN_POINT('Ctrl Pts',(36.679954868674,61.0560536877083,0.));
#164535=CARTESIAN_POINT('Ctrl Pts',(36.679954868674,61.0560536877083,12.));
#164536=CARTESIAN_POINT('Ctrl Pts',(36.6629633998886,61.0413773427203,0.));
#164537=CARTESIAN_POINT('Ctrl Pts',(36.6629633998886,61.0413773427203,12.));
#164538=CARTESIAN_POINT('Ctrl Pts',(36.6460216768553,61.0267140464432,0.));
#164539=CARTESIAN_POINT('Ctrl Pts',(36.6460216768553,61.0267140464432,12.));
#164540=CARTESIAN_POINT('Ctrl Pts',(36.6291297604776,61.0120639445349,0.));
#164541=CARTESIAN_POINT('Ctrl Pts',(36.6291297604776,61.0120639445349,12.));
#164542=CARTESIAN_POINT('Ctrl Pts',(36.61228771186,60.9974271833981,0.));
#164543=CARTESIAN_POINT('Ctrl Pts',(36.61228771186,60.9974271833981,12.));
#164544=CARTESIAN_POINT('Ctrl Pts',(36.5954955923109,60.9828039101887,0.));
#164545=CARTESIAN_POINT('Ctrl Pts',(36.5954955923109,60.9828039101887,12.));
#164546=CARTESIAN_POINT('Ctrl Pts',(36.5787534633415,60.9681942728237,0.));
#164547=CARTESIAN_POINT('Ctrl Pts',(36.5787534633415,60.9681942728237,12.));
#164548=CARTESIAN_POINT('Ctrl Pts',(36.5620613866614,60.9535984199873,0.));
#164549=CARTESIAN_POINT('Ctrl Pts',(36.5620613866614,60.9535984199873,12.));
#164550=CARTESIAN_POINT('Ctrl Pts',(36.5454194241865,60.9390165011355,0.));
#164551=CARTESIAN_POINT('Ctrl Pts',(36.5454194241865,60.9390165011355,12.));
#164552=CARTESIAN_POINT('Ctrl Pts',(36.5288276380416,60.9244486664988,0.));
#164553=CARTESIAN_POINT('Ctrl Pts',(36.5288276380416,60.9244486664988,12.));
#164554=CARTESIAN_POINT('Ctrl Pts',(36.5122860905612,60.9098950670847,0.));
#164555=CARTESIAN_POINT('Ctrl Pts',(36.5122860905612,60.9098950670847,12.));
#164556=CARTESIAN_POINT('Ctrl Pts',(36.4957948442835,60.8953558546795,0.));
#164557=CARTESIAN_POINT('Ctrl Pts',(36.4957948442835,60.8953558546795,12.));
#164558=CARTESIAN_POINT('Ctrl Pts',(36.4793539619466,60.8808311818499,0.));
#164559=CARTESIAN_POINT('Ctrl Pts',(36.4793539619466,60.8808311818499,12.));
#164560=CARTESIAN_POINT('Ctrl Pts',(36.4629635065045,60.8663212019657,0.));
#164561=CARTESIAN_POINT('Ctrl Pts',(36.4629635065045,60.8663212019657,12.));
#164562=CARTESIAN_POINT('Ctrl Pts',(36.4466235411358,60.8518260692188,0.));
#164563=CARTESIAN_POINT('Ctrl Pts',(36.4466235411358,60.8518260692188,12.));
#164564=CARTESIAN_POINT('Ctrl Pts',(36.4303341292494,60.8373459386392,0.));
#164565=CARTESIAN_POINT('Ctrl Pts',(36.4303341292494,60.8373459386392,12.));
#164566=CARTESIAN_POINT('Ctrl Pts',(36.4140953344858,60.8228809661161,0.));
#164567=CARTESIAN_POINT('Ctrl Pts',(36.4140953344858,60.8228809661161,12.));
#164568=CARTESIAN_POINT('Ctrl Pts',(36.397907220716,60.8084313083984,0.));
#164569=CARTESIAN_POINT('Ctrl Pts',(36.397907220716,60.8084313083984,12.));
#164570=CARTESIAN_POINT('Ctrl Pts',(36.3817698520388,60.7939971230761,0.));
#164571=CARTESIAN_POINT('Ctrl Pts',(36.3817698520388,60.7939971230761,12.));
#164572=CARTESIAN_POINT('Ctrl Pts',(36.365683292773,60.7795785685625,0.));
#164573=CARTESIAN_POINT('Ctrl Pts',(36.365683292773,60.7795785685625,12.));
#164574=CARTESIAN_POINT('Ctrl Pts',(36.3496476074488,60.7651758040804,0.));
#164575=CARTESIAN_POINT('Ctrl Pts',(36.3496476074488,60.7651758040804,12.));
#164576=CARTESIAN_POINT('Ctrl Pts',(36.3336628607858,60.7507889896308,0.));
#164577=CARTESIAN_POINT('Ctrl Pts',(36.3336628607858,60.7507889896308,12.));
#164578=CARTESIAN_POINT('Ctrl Pts',(36.3177291177163,60.7364182860412,0.));
#164579=CARTESIAN_POINT('Ctrl Pts',(36.3177291177163,60.7364182860412,12.));
#164580=CARTESIAN_POINT('Ctrl Pts',(36.3018464434213,60.722063855041,0.));
#164581=CARTESIAN_POINT('Ctrl Pts',(36.3018464434213,60.722063855041,12.));
#164582=CARTESIAN_POINT('Ctrl Pts',(36.2860149033587,60.7077258593268,0.));
#164583=CARTESIAN_POINT('Ctrl Pts',(36.2860149033587,60.7077258593268,12.));
#164584=CARTESIAN_POINT('Ctrl Pts',(36.2702345632875,60.6934044626291,0.));
#164585=CARTESIAN_POINT('Ctrl Pts',(36.2702345632875,60.6934044626291,12.));
#164586=CARTESIAN_POINT('Ctrl Pts',(36.2545054892897,60.67909982978,0.));
#164587=CARTESIAN_POINT('Ctrl Pts',(36.2545054892897,60.67909982978,12.));
#164588=CARTESIAN_POINT('Ctrl Pts',(36.2388277477212,60.6648121265885,0.));
#164589=CARTESIAN_POINT('Ctrl Pts',(36.2388277477212,60.6648121265885,12.));
#164590=CARTESIAN_POINT('Ctrl Pts',(36.2232014051541,60.6505415197042,0.));
#164591=CARTESIAN_POINT('Ctrl Pts',(36.2232014051541,60.6505415197042,12.));
#164592=CARTESIAN_POINT('Ctrl Pts',(36.2076265283264,60.6362881765019,0.));
#164593=CARTESIAN_POINT('Ctrl Pts',(36.2076265283264,60.6362881765019,12.));
#164594=CARTESIAN_POINT('Ctrl Pts',(36.1921031840629,60.6220522649149,0.));
#164595=CARTESIAN_POINT('Ctrl Pts',(36.1921031840629,60.6220522649149,12.));
#164596=CARTESIAN_POINT('Ctrl Pts',(36.1766314392641,60.6078339534181,0.));
#164597=CARTESIAN_POINT('Ctrl Pts',(36.1766314392641,60.6078339534181,12.));
#164598=CARTESIAN_POINT('Ctrl Pts',(36.1612113610773,60.5936334114108,0.));
#164599=CARTESIAN_POINT('Ctrl Pts',(36.1612113610773,60.5936334114108,12.));
#164600=CARTESIAN_POINT('Ctrl Pts',(36.145843017043,60.5794508095565,0.));
#164601=CARTESIAN_POINT('Ctrl Pts',(36.145843017043,60.5794508095565,12.));
#164602=CARTESIAN_POINT('Ctrl Pts',(36.1305264752187,60.565286320072,0.));
#164603=CARTESIAN_POINT('Ctrl Pts',(36.1305264752187,60.565286320072,12.));
#164604=CARTESIAN_POINT('Ctrl Pts',(36.1152618043738,60.5511401171984,0.));
#164605=CARTESIAN_POINT('Ctrl Pts',(36.1152618043738,60.5511401171984,12.));
#164606=CARTESIAN_POINT('Ctrl Pts',(36.100049073851,60.5370123768804,0.));
#164607=CARTESIAN_POINT('Ctrl Pts',(36.100049073851,60.5370123768804,12.));
#164608=CARTESIAN_POINT('Ctrl Pts',(36.0848883531952,60.5229032758974,0.));
#164609=CARTESIAN_POINT('Ctrl Pts',(36.0848883531952,60.5229032758974,12.));
#164610=CARTESIAN_POINT('Ctrl Pts',(36.0697797118375,60.5088129911354,0.));
#164611=CARTESIAN_POINT('Ctrl Pts',(36.0697797118375,60.5088129911354,12.));
#164612=CARTESIAN_POINT('Ctrl Pts',(36.0547232187697,60.4947416988422,0.));
#164613=CARTESIAN_POINT('Ctrl Pts',(36.0547232187697,60.4947416988422,12.));
#164614=CARTESIAN_POINT('Ctrl Pts',(36.0397189421644,60.4806895737686,0.));
#164615=CARTESIAN_POINT('Ctrl Pts',(36.0397189421644,60.4806895737686,12.));
#164616=CARTESIAN_POINT('Ctrl Pts',(36.0247669500891,60.4666567908093,0.));
#164617=CARTESIAN_POINT('Ctrl Pts',(36.0247669500891,60.4666567908093,12.));
#164618=CARTESIAN_POINT('Ctrl Pts',(36.009867311357,60.4526435269662,0.));
#164619=CARTESIAN_POINT('Ctrl Pts',(36.009867311357,60.4526435269662,12.));
#164620=CARTESIAN_POINT('Ctrl Pts',(35.995020096217,60.4386499629481,0.));
#164621=CARTESIAN_POINT('Ctrl Pts',(35.995020096217,60.4386499629481,12.));
#164622=CARTESIAN_POINT('Ctrl Pts',(35.9802253773514,60.4246762854926,0.));
#164623=CARTESIAN_POINT('Ctrl Pts',(35.9802253773514,60.4246762854926,12.));
#164624=CARTESIAN_POINT('Ctrl Pts',(35.9654832299601,60.4107226875714,0.));
#164625=CARTESIAN_POINT('Ctrl Pts',(35.9654832299601,60.4107226875714,12.));
#164626=CARTESIAN_POINT('Ctrl Pts',(35.9507937296706,60.3967893635452,0.));
#164627=CARTESIAN_POINT('Ctrl Pts',(35.9507937296706,60.3967893635452,12.));
#164628=CARTESIAN_POINT('Ctrl Pts',(35.9361569506949,60.3828765049019,0.));
#164629=CARTESIAN_POINT('Ctrl Pts',(35.9361569506949,60.3828765049019,12.));
#164630=CARTESIAN_POINT('Ctrl Pts',(35.9215729642231,60.3689842965481,0.));
#164631=CARTESIAN_POINT('Ctrl Pts',(35.9215729642231,60.3689842965481,12.));
#164632=CARTESIAN_POINT('Ctrl Pts',(35.907041835853,60.3551129108845,0.));
#164633=CARTESIAN_POINT('Ctrl Pts',(35.907041835853,60.3551129108845,12.));
#164634=CARTESIAN_POINT('Ctrl Pts',(35.8925636280668,60.3412625135287,0.));
#164635=CARTESIAN_POINT('Ctrl Pts',(35.8925636280668,60.3412625135287,12.));
#164636=CARTESIAN_POINT('Ctrl Pts',(35.8781384051536,60.327433274683,0.));
#164637=CARTESIAN_POINT('Ctrl Pts',(35.8781384051536,60.327433274683,12.));
#164638=CARTESIAN_POINT('Ctrl Pts',(35.8637662371635,60.313625378281,0.));
#164639=CARTESIAN_POINT('Ctrl Pts',(35.8637662371635,60.313625378281,12.));
#164640=CARTESIAN_POINT('Ctrl Pts',(35.8494472046745,60.2998390330102,0.));
#164641=CARTESIAN_POINT('Ctrl Pts',(35.8494472046745,60.2998390330102,12.));
#164642=CARTESIAN_POINT('Ctrl Pts',(35.8351814020356,60.2860744798436,0.));
#164643=CARTESIAN_POINT('Ctrl Pts',(35.8351814020356,60.2860744798436,12.));
#164644=CARTESIAN_POINT('Ctrl Pts',(35.82096892725,60.2723319687369,0.));
#164645=CARTESIAN_POINT('Ctrl Pts',(35.82096892725,60.2723319687369,12.));
#164646=CARTESIAN_POINT('Ctrl Pts',(35.8068098723347,60.2586117365205,0.));
#164647=CARTESIAN_POINT('Ctrl Pts',(35.8068098723347,60.2586117365205,12.));
#164648=CARTESIAN_POINT('Ctrl Pts',(35.7927043145201,60.2449139865275,0.));
#164649=CARTESIAN_POINT('Ctrl Pts',(35.7927043145201,60.2449139865275,12.));
#164650=CARTESIAN_POINT('Ctrl Pts',(35.7786523045911,60.2312388621529,0.));
#164651=CARTESIAN_POINT('Ctrl Pts',(35.7786523045911,60.2312388621529,12.));
#164652=CARTESIAN_POINT('Ctrl Pts',(35.7646538667493,60.2175864450043,0.));
#164653=CARTESIAN_POINT('Ctrl Pts',(35.7646538667493,60.2175864450043,12.));
#164654=CARTESIAN_POINT('Ctrl Pts',(35.7534979802053,60.206682708692,0.));
#164655=CARTESIAN_POINT('Ctrl Pts',(35.7534979802053,60.206682708692,12.));
#164656=CARTESIAN_POINT('Ctrl Pts',(35.7451551752572,60.1985151474623,0.));
#164657=CARTESIAN_POINT('Ctrl Pts',(35.7451551752572,60.1985151474623,12.));
#164658=CARTESIAN_POINT('Ctrl Pts',(35.7396040204017,60.193074658032,0.));
#164659=CARTESIAN_POINT('Ctrl Pts',(35.7396040204017,60.193074658032,12.));
#164660=CARTESIAN_POINT('Ctrl Pts',(35.7368311217509,60.1903555511633,0.));
#164661=CARTESIAN_POINT('Ctrl Pts',(35.7368311217509,60.1903555511633,12.));
#164662=CARTESIAN_POINT('',(35.7368311217509,60.1903555511633,12.));
#164663=CARTESIAN_POINT('Ctrl Pts',(35.7368311217509,60.1903555511633,12.));
#164664=CARTESIAN_POINT('Ctrl Pts',(35.7396040204017,60.193074658032,12.));
#164665=CARTESIAN_POINT('Ctrl Pts',(35.7451551752572,60.1985151474623,12.));
#164666=CARTESIAN_POINT('Ctrl Pts',(35.7534979802053,60.206682708692,12.));
#164667=CARTESIAN_POINT('Ctrl Pts',(35.7646538667493,60.2175864450043,12.));
#164668=CARTESIAN_POINT('Ctrl Pts',(35.7786523045911,60.2312388621529,12.));
#164669=CARTESIAN_POINT('Ctrl Pts',(35.7927043145201,60.2449139865275,12.));
#164670=CARTESIAN_POINT('Ctrl Pts',(35.8068098723347,60.2586117365205,12.));
#164671=CARTESIAN_POINT('Ctrl Pts',(35.82096892725,60.2723319687369,12.));
#164672=CARTESIAN_POINT('Ctrl Pts',(35.8351814020356,60.2860744798436,12.));
#164673=CARTESIAN_POINT('Ctrl Pts',(35.8494472046745,60.2998390330102,12.));
#164674=CARTESIAN_POINT('Ctrl Pts',(35.8637662371635,60.313625378281,12.));
#164675=CARTESIAN_POINT('Ctrl Pts',(35.8781384051536,60.327433274683,12.));
#164676=CARTESIAN_POINT('Ctrl Pts',(35.8925636280668,60.3412625135287,12.));
#164677=CARTESIAN_POINT('Ctrl Pts',(35.907041835853,60.3551129108845,12.));
#164678=CARTESIAN_POINT('Ctrl Pts',(35.9215729642231,60.3689842965481,12.));
#164679=CARTESIAN_POINT('Ctrl Pts',(35.9361569506949,60.3828765049019,12.));
#164680=CARTESIAN_POINT('Ctrl Pts',(35.9507937296706,60.3967893635452,12.));
#164681=CARTESIAN_POINT('Ctrl Pts',(35.9654832299601,60.4107226875714,12.));
#164682=CARTESIAN_POINT('Ctrl Pts',(35.9802253773514,60.4246762854926,12.));
#164683=CARTESIAN_POINT('Ctrl Pts',(35.995020096217,60.4386499629481,12.));
#164684=CARTESIAN_POINT('Ctrl Pts',(36.009867311357,60.4526435269662,12.));
#164685=CARTESIAN_POINT('Ctrl Pts',(36.0247669500891,60.4666567908093,12.));
#164686=CARTESIAN_POINT('Ctrl Pts',(36.0397189421644,60.4806895737686,12.));
#164687=CARTESIAN_POINT('Ctrl Pts',(36.0547232187697,60.4947416988422,12.));
#164688=CARTESIAN_POINT('Ctrl Pts',(36.0697797118375,60.5088129911354,12.));
#164689=CARTESIAN_POINT('Ctrl Pts',(36.0848883531952,60.5229032758974,12.));
#164690=CARTESIAN_POINT('Ctrl Pts',(36.100049073851,60.5370123768804,12.));
#164691=CARTESIAN_POINT('Ctrl Pts',(36.1152618043738,60.5511401171984,12.));
#164692=CARTESIAN_POINT('Ctrl Pts',(36.1305264752187,60.565286320072,12.));
#164693=CARTESIAN_POINT('Ctrl Pts',(36.145843017043,60.5794508095565,12.));
#164694=CARTESIAN_POINT('Ctrl Pts',(36.1612113610773,60.5936334114108,12.));
#164695=CARTESIAN_POINT('Ctrl Pts',(36.1766314392641,60.6078339534181,12.));
#164696=CARTESIAN_POINT('Ctrl Pts',(36.1921031840629,60.6220522649149,12.));
#164697=CARTESIAN_POINT('Ctrl Pts',(36.2076265283264,60.6362881765019,12.));
#164698=CARTESIAN_POINT('Ctrl Pts',(36.2232014051541,60.6505415197042,12.));
#164699=CARTESIAN_POINT('Ctrl Pts',(36.2388277477212,60.6648121265885,12.));
#164700=CARTESIAN_POINT('Ctrl Pts',(36.2545054892897,60.67909982978,12.));
#164701=CARTESIAN_POINT('Ctrl Pts',(36.2702345632875,60.6934044626291,12.));
#164702=CARTESIAN_POINT('Ctrl Pts',(36.2860149033587,60.7077258593268,12.));
#164703=CARTESIAN_POINT('Ctrl Pts',(36.3018464434213,60.722063855041,12.));
#164704=CARTESIAN_POINT('Ctrl Pts',(36.3177291177163,60.7364182860412,12.));
#164705=CARTESIAN_POINT('Ctrl Pts',(36.3336628607858,60.7507889896308,12.));
#164706=CARTESIAN_POINT('Ctrl Pts',(36.3496476074488,60.7651758040804,12.));
#164707=CARTESIAN_POINT('Ctrl Pts',(36.365683292773,60.7795785685625,12.));
#164708=CARTESIAN_POINT('Ctrl Pts',(36.3817698520388,60.7939971230761,12.));
#164709=CARTESIAN_POINT('Ctrl Pts',(36.397907220716,60.8084313083984,12.));
#164710=CARTESIAN_POINT('Ctrl Pts',(36.4140953344858,60.8228809661161,12.));
#164711=CARTESIAN_POINT('Ctrl Pts',(36.4303341292494,60.8373459386392,12.));
#164712=CARTESIAN_POINT('Ctrl Pts',(36.4466235411358,60.8518260692188,12.));
#164713=CARTESIAN_POINT('Ctrl Pts',(36.4629635065045,60.8663212019657,12.));
#164714=CARTESIAN_POINT('Ctrl Pts',(36.4793539619466,60.8808311818499,12.));
#164715=CARTESIAN_POINT('Ctrl Pts',(36.4957948442835,60.8953558546795,12.));
#164716=CARTESIAN_POINT('Ctrl Pts',(36.5122860905612,60.9098950670847,12.));
#164717=CARTESIAN_POINT('Ctrl Pts',(36.5288276380416,60.9244486664988,12.));
#164718=CARTESIAN_POINT('Ctrl Pts',(36.5454194241865,60.9390165011355,12.));
#164719=CARTESIAN_POINT('Ctrl Pts',(36.5620613866614,60.9535984199873,12.));
#164720=CARTESIAN_POINT('Ctrl Pts',(36.5787534633415,60.9681942728237,12.));
#164721=CARTESIAN_POINT('Ctrl Pts',(36.5954955923109,60.9828039101887,12.));
#164722=CARTESIAN_POINT('Ctrl Pts',(36.61228771186,60.9974271833981,12.));
#164723=CARTESIAN_POINT('Ctrl Pts',(36.6291297604776,61.0120639445349,12.));
#164724=CARTESIAN_POINT('Ctrl Pts',(36.6460216768553,61.0267140464432,12.));
#164725=CARTESIAN_POINT('Ctrl Pts',(36.6629633998886,61.0413773427203,12.));
#164726=CARTESIAN_POINT('Ctrl Pts',(36.679954868674,61.0560536877083,12.));
#164727=CARTESIAN_POINT('Ctrl Pts',(36.6969960225022,61.0707429364847,12.));
#164728=CARTESIAN_POINT('Ctrl Pts',(36.7140868008486,61.0854449448524,12.));
#164729=CARTESIAN_POINT('Ctrl Pts',(36.7312271433807,61.100159569337,12.));
#164730=CARTESIAN_POINT('Ctrl Pts',(36.7484169899596,61.1148866671829,12.));
#164731=CARTESIAN_POINT('Ctrl Pts',(36.765656280638,61.1296260963466,12.));
#164732=CARTESIAN_POINT('Ctrl Pts',(36.7829449556532,61.1443777154911,12.));
#164733=CARTESIAN_POINT('Ctrl Pts',(36.8002829554209,61.1591413839787,12.));
#164734=CARTESIAN_POINT('Ctrl Pts',(36.8176702205423,61.1739169618667,12.));
#164735=CARTESIAN_POINT('Ctrl Pts',(36.8351066918036,61.1887043099014,12.));
#164736=CARTESIAN_POINT('Ctrl Pts',(36.852592310174,61.2035032895127,12.));
#164737=CARTESIAN_POINT('Ctrl Pts',(36.8701270167969,61.2183137628056,12.));
#164738=CARTESIAN_POINT('Ctrl Pts',(36.8877107529865,61.2331355925547,12.));
#164739=CARTESIAN_POINT('Ctrl Pts',(36.9053434602343,61.247968642201,12.));
#164740=CARTESIAN_POINT('Ctrl Pts',(36.9230250802087,61.2628127758457,12.));
#164741=CARTESIAN_POINT('Ctrl Pts',(36.9407555547534,61.2776678582461,12.));
#164742=CARTESIAN_POINT('Ctrl Pts',(36.9585348258776,61.2925337548077,12.));
#164743=CARTESIAN_POINT('Ctrl Pts',(36.9763628357544,61.3074103315792,12.));
#164744=CARTESIAN_POINT('Ctrl Pts',(36.994239526727,61.3222974552487,12.));
#164745=CARTESIAN_POINT('Ctrl Pts',(37.0121648413081,61.3371949931387,12.));
#164746=CARTESIAN_POINT('Ctrl Pts',(37.0301387221774,61.3521028132003,12.));
#164747=CARTESIAN_POINT('Ctrl Pts',(37.0481611121717,61.3670207840069,12.));
#164748=CARTESIAN_POINT('Ctrl Pts',(37.0662319542849,61.381948774749,12.));
#164749=CARTESIAN_POINT('Ctrl Pts',(37.0843511916744,61.3968866552318,12.));
#164750=CARTESIAN_POINT('Ctrl Pts',(37.1025187676602,61.4118342958697,12.));
#164751=CARTESIAN_POINT('Ctrl Pts',(37.1207346257221,61.4267915676822,12.));
#164752=CARTESIAN_POINT('Ctrl Pts',(37.1389987094904,61.4417583422863,12.));
#164753=CARTESIAN_POINT('Ctrl Pts',(37.1573109627454,61.456734491892,12.));
#164754=CARTESIAN_POINT('Ctrl Pts',(37.175671329424,61.4717198892994,12.));
#164755=CARTESIAN_POINT('Ctrl Pts',(37.1940797536181,61.4867144078937,12.));
#164756=CARTESIAN_POINT('Ctrl Pts',(37.2125361795731,61.501717921641,12.));
#164757=CARTESIAN_POINT('Ctrl Pts',(37.2310405516781,61.5167303050832,12.));
#164758=CARTESIAN_POINT('Ctrl Pts',(37.2495928144666,61.5317514333328,12.));
#164759=CARTESIAN_POINT('Ctrl Pts',(37.2681929126221,61.5467811820691,12.));
#164760=CARTESIAN_POINT('Ctrl Pts',(37.286840790977,61.5618194275348,12.));
#164761=CARTESIAN_POINT('Ctrl Pts',(37.3055363945107,61.5768660465311,12.));
#164762=CARTESIAN_POINT('Ctrl Pts',(37.3242796683395,61.591920916412,12.));
#164763=CARTESIAN_POINT('Ctrl Pts',(37.343070557718,61.6069839150807,12.));
#164764=CARTESIAN_POINT('Ctrl Pts',(37.3619090080449,61.6220549209866,12.));
#164765=CARTESIAN_POINT('Ctrl Pts',(37.3807949648624,61.637133813121,12.));
#164766=CARTESIAN_POINT('Ctrl Pts',(37.3997283738533,61.6522204710131,12.));
#164767=CARTESIAN_POINT('Ctrl Pts',(37.418709180832,61.6673147747242,12.));
#164768=CARTESIAN_POINT('Ctrl Pts',(37.4377373317451,61.6824166048444,12.));
#164769=CARTESIAN_POINT('Ctrl Pts',(37.4568127726773,61.6975258424894,12.));
#164770=CARTESIAN_POINT('Ctrl Pts',(37.4759354498509,61.7126423692963,12.));
#164771=CARTESIAN_POINT('Ctrl Pts',(37.4951053096237,61.7277660674205,12.));
#164772=CARTESIAN_POINT('Ctrl Pts',(37.5143222984795,61.7428968195299,12.));
#164773=CARTESIAN_POINT('Ctrl Pts',(37.5335863630287,61.7580345088016,12.));
#164774=CARTESIAN_POINT('Ctrl Pts',(37.5528974500141,61.7731790189191,12.));
#164775=CARTESIAN_POINT('Ctrl Pts',(37.5722555063111,61.7883302340687,12.));
#164776=CARTESIAN_POINT('Ctrl Pts',(37.5916604789253,61.8034880389363,12.));
#164777=CARTESIAN_POINT('Ctrl Pts',(37.6111123149839,61.8186523187015,12.));
#164778=CARTESIAN_POINT('Ctrl Pts',(37.6306109617346,61.8338229590353,12.));
#164779=CARTESIAN_POINT('Ctrl Pts',(37.6501563665523,61.8489998460957,12.));
#164780=CARTESIAN_POINT('Ctrl Pts',(37.6697484769392,61.8641828665262,12.));
#164781=CARTESIAN_POINT('Ctrl Pts',(37.6893872405228,61.8793719074507,12.));
#164782=CARTESIAN_POINT('Ctrl Pts',(37.7090726050482,61.8945668564704,12.));
#164783=CARTESIAN_POINT('Ctrl Pts',(37.7288045183756,61.9097676016601,12.));
#164784=CARTESIAN_POINT('Ctrl Pts',(37.7485829284871,61.9249740315649,12.));
#164785=CARTESIAN_POINT('Ctrl Pts',(37.7684077834872,61.9401860351973,12.));
#164786=CARTESIAN_POINT('Ctrl Pts',(37.7882790316014,61.9554035020338,12.));
#164787=CARTESIAN_POINT('Ctrl Pts',(37.8081966211688,61.9706263220114,12.));
#164788=CARTESIAN_POINT('Ctrl Pts',(37.828160500638,61.9858543855236,12.));
#164789=CARTESIAN_POINT('Ctrl Pts',(37.8481706185749,62.0010875834187,12.));
#164790=CARTESIAN_POINT('Ctrl Pts',(37.868226923663,62.0163258069957,12.));
#164791=CARTESIAN_POINT('Ctrl Pts',(37.8883293647029,62.031568948002,12.));
#164792=CARTESIAN_POINT('Ctrl Pts',(37.9084778906053,62.0468168986288,12.));
#164793=CARTESIAN_POINT('Ctrl Pts',(37.9286724503851,62.0620695515075,12.));
#164794=CARTESIAN_POINT('Ctrl Pts',(37.9489129931688,62.0773267997079,12.));
#164795=CARTESIAN_POINT('Ctrl Pts',(37.9691994681966,62.0925885367352,12.));
#164796=CARTESIAN_POINT('Ctrl Pts',(37.9895318248212,62.107854656528,12.));
#164797=CARTESIAN_POINT('Ctrl Pts',(38.0099100125037,62.123125053455,12.));
#164798=CARTESIAN_POINT('Ctrl Pts',(38.0303339808053,62.1383996223125,12.));
#164799=CARTESIAN_POINT('Ctrl Pts',(38.0508036793939,62.1536782583199,12.));
#164800=CARTESIAN_POINT('Ctrl Pts',(38.0713190580463,62.1689608571176,12.));
#164801=CARTESIAN_POINT('Ctrl Pts',(38.0918800666479,62.1842473147626,12.));
#164802=CARTESIAN_POINT('Ctrl Pts',(38.1124866551885,62.1995375277257,12.));
#164803=CARTESIAN_POINT('Ctrl Pts',(38.1331387737529,62.2148313928863,12.));
#164804=CARTESIAN_POINT('Ctrl Pts',(38.1538363725263,62.2301288075321,12.));
#164805=CARTESIAN_POINT('Ctrl Pts',(38.1745794017995,62.245429669358,12.));
#164806=CARTESIAN_POINT('Ctrl Pts',(38.1953678119691,62.2607338764654,12.));
#164807=CARTESIAN_POINT('Ctrl Pts',(38.2162015535352,62.2760413273602,12.));
#164808=CARTESIAN_POINT('Ctrl Pts',(38.2370805770935,62.2913519209521,12.));
#164809=CARTESIAN_POINT('Ctrl Pts',(38.258004833336,62.3066655565503,12.));
#164810=CARTESIAN_POINT('Ctrl Pts',(38.2789742730563,62.3219821338569,12.));
#164811=CARTESIAN_POINT('Ctrl Pts',(38.2999888471476,62.3373015529613,12.));
#164812=CARTESIAN_POINT('Ctrl Pts',(38.3210485066001,62.3526237143336,12.));
#164813=CARTESIAN_POINT('Ctrl Pts',(38.342153202491,62.3679485188172,12.));
#164814=CARTESIAN_POINT('Ctrl Pts',(38.3633028859828,62.3832758676271,12.));
#164815=CARTESIAN_POINT('Ctrl Pts',(38.3844975083343,62.3986056623577,12.));
#164816=CARTESIAN_POINT('Ctrl Pts',(38.405737020905,62.4139378049886,12.));
#164817=CARTESIAN_POINT('Ctrl Pts',(38.4270213751568,62.4292721978901,12.));
#164818=CARTESIAN_POINT('Ctrl Pts',(38.4483505226518,62.4446087438312,12.));
#164819=CARTESIAN_POINT('Ctrl Pts',(38.4697244150482,62.4599473459811,12.));
#164820=CARTESIAN_POINT('Ctrl Pts',(38.4911430040997,62.4752879078854,12.));
#164821=CARTESIAN_POINT('Ctrl Pts',(38.5126062416502,62.4906303334443,12.));
#164822=CARTESIAN_POINT('Ctrl Pts',(38.5341140796248,62.5059745268901,12.));
#164823=CARTESIAN_POINT('Ctrl Pts',(38.5556664700195,62.5213203927663,12.));
#164824=CARTESIAN_POINT('Ctrl Pts',(38.5772633648832,62.5366678359023,12.));
#164825=CARTESIAN_POINT('Ctrl Pts',(38.5989047163393,62.5520167614516,12.));
#164826=CARTESIAN_POINT('Ctrl Pts',(38.6205904766072,62.5673670749362,12.));
#164827=CARTESIAN_POINT('Ctrl Pts',(38.6423205980213,62.5827186822921,12.));
#164828=CARTESIAN_POINT('Ctrl Pts',(38.6640950330421,62.5980714899052,12.));
#164829=CARTESIAN_POINT('Ctrl Pts',(38.685913734273,62.6134254046739,12.));
#164830=CARTESIAN_POINT('Ctrl Pts',(38.7077766544416,62.6287803339542,12.));
#164831=CARTESIAN_POINT('Ctrl Pts',(38.7296837463608,62.6441361854411,12.));
#164832=CARTESIAN_POINT('Ctrl Pts',(38.7516349628903,62.6594928670628,12.));
#164833=CARTESIAN_POINT('Ctrl Pts',(38.7736302568982,62.6748502868835,12.));
#164834=CARTESIAN_POINT('Ctrl Pts',(38.795669581203,62.6902083529695,12.));
#164835=CARTESIAN_POINT('Ctrl Pts',(38.8177528885681,62.7055669733802,12.));
#164836=CARTESIAN_POINT('Ctrl Pts',(38.8398801318176,62.7209260564493,12.));
#164837=CARTESIAN_POINT('Ctrl Pts',(38.8620512639232,62.7362855110042,12.));
#164838=CARTESIAN_POINT('Ctrl Pts',(38.8842662380984,62.7516452466128,12.));
#164839=CARTESIAN_POINT('Ctrl Pts',(38.9065250078832,62.7670051738143,12.));
#164840=CARTESIAN_POINT('Ctrl Pts',(38.9288275272335,62.78236520437,12.));
#164841=CARTESIAN_POINT('Ctrl Pts',(38.9511737503165,62.7977252507118,12.));
#164842=CARTESIAN_POINT('Ctrl Pts',(38.9735636313088,62.8130852254027,12.));
#164843=CARTESIAN_POINT('Ctrl Pts',(38.9959971241701,62.8284450405459,12.));
#164844=CARTESIAN_POINT('Ctrl Pts',(39.0184741824641,62.8438046073224,12.));
#164845=CARTESIAN_POINT('Ctrl Pts',(39.0409947590496,62.8591638352056,12.));
#164846=CARTESIAN_POINT('Ctrl Pts',(39.0635588063276,62.8745226325998,12.));
#164847=CARTESIAN_POINT('Ctrl Pts',(39.0861662767932,62.8898809082612,12.));
#164848=CARTESIAN_POINT('Ctrl Pts',(39.1088171235125,62.9052385725388,12.));
#164849=CARTESIAN_POINT('Ctrl Pts',(39.131511300575,62.9205955385558,12.));
#164850=CARTESIAN_POINT('Ctrl Pts',(39.1542487636743,62.9359517237404,12.));
#164851=CARTESIAN_POINT('Ctrl Pts',(39.1770294702428,62.9513070501867,12.));
#164852=CARTESIAN_POINT('Ctrl Pts',(39.1965939820933,62.9644687386836,12.));
#164853=CARTESIAN_POINT('Ctrl Pts',(39.2116170128461,62.9745590018673,12.));
#164854=CARTESIAN_POINT('Ctrl Pts',(39.2220794388807,62.9815782721326,12.));
#164855=CARTESIAN_POINT('Ctrl Pts',(39.2279686275008,62.9855268616129,12.));
#164856=CARTESIAN_POINT('Ctrl Pts',(39.2292784191814,62.9864049293895,12.));
#164857=CARTESIAN_POINT('',(35.7368311217509,60.1903555511633,0.));
#164858=CARTESIAN_POINT('',(35.7368311217509,60.1903555511633,0.));
#164859=CARTESIAN_POINT('Ctrl Pts',(39.2292784191814,62.9864049293895,0.));
#164860=CARTESIAN_POINT('Ctrl Pts',(39.2279686275008,62.9855268616129,0.));
#164861=CARTESIAN_POINT('Ctrl Pts',(39.2220794388807,62.9815782721326,0.));
#164862=CARTESIAN_POINT('Ctrl Pts',(39.2116170128461,62.9745590018673,0.));
#164863=CARTESIAN_POINT('Ctrl Pts',(39.1965939820933,62.9644687386836,0.));
#164864=CARTESIAN_POINT('Ctrl Pts',(39.1770294702428,62.9513070501867,0.));
#164865=CARTESIAN_POINT('Ctrl Pts',(39.1542487636743,62.9359517237404,0.));
#164866=CARTESIAN_POINT('Ctrl Pts',(39.131511300575,62.9205955385558,0.));
#164867=CARTESIAN_POINT('Ctrl Pts',(39.1088171235125,62.9052385725388,0.));
#164868=CARTESIAN_POINT('Ctrl Pts',(39.0861662767932,62.8898809082612,0.));
#164869=CARTESIAN_POINT('Ctrl Pts',(39.0635588063276,62.8745226325998,0.));
#164870=CARTESIAN_POINT('Ctrl Pts',(39.0409947590496,62.8591638352056,0.));
#164871=CARTESIAN_POINT('Ctrl Pts',(39.0184741824641,62.8438046073224,0.));
#164872=CARTESIAN_POINT('Ctrl Pts',(38.9959971241701,62.8284450405459,0.));
#164873=CARTESIAN_POINT('Ctrl Pts',(38.9735636313088,62.8130852254027,0.));
#164874=CARTESIAN_POINT('Ctrl Pts',(38.9511737503165,62.7977252507118,0.));
#164875=CARTESIAN_POINT('Ctrl Pts',(38.9288275272335,62.78236520437,0.));
#164876=CARTESIAN_POINT('Ctrl Pts',(38.9065250078832,62.7670051738143,0.));
#164877=CARTESIAN_POINT('Ctrl Pts',(38.8842662380984,62.7516452466128,0.));
#164878=CARTESIAN_POINT('Ctrl Pts',(38.8620512639232,62.7362855110042,0.));
#164879=CARTESIAN_POINT('Ctrl Pts',(38.8398801318176,62.7209260564493,0.));
#164880=CARTESIAN_POINT('Ctrl Pts',(38.8177528885681,62.7055669733802,0.));
#164881=CARTESIAN_POINT('Ctrl Pts',(38.795669581203,62.6902083529695,0.));
#164882=CARTESIAN_POINT('Ctrl Pts',(38.7736302568982,62.6748502868835,0.));
#164883=CARTESIAN_POINT('Ctrl Pts',(38.7516349628903,62.6594928670628,0.));
#164884=CARTESIAN_POINT('Ctrl Pts',(38.7296837463608,62.6441361854411,0.));
#164885=CARTESIAN_POINT('Ctrl Pts',(38.7077766544416,62.6287803339542,0.));
#164886=CARTESIAN_POINT('Ctrl Pts',(38.685913734273,62.6134254046739,0.));
#164887=CARTESIAN_POINT('Ctrl Pts',(38.6640950330421,62.5980714899052,0.));
#164888=CARTESIAN_POINT('Ctrl Pts',(38.6423205980213,62.5827186822921,0.));
#164889=CARTESIAN_POINT('Ctrl Pts',(38.6205904766072,62.5673670749362,0.));
#164890=CARTESIAN_POINT('Ctrl Pts',(38.5989047163393,62.5520167614516,0.));
#164891=CARTESIAN_POINT('Ctrl Pts',(38.5772633648832,62.5366678359023,0.));
#164892=CARTESIAN_POINT('Ctrl Pts',(38.5556664700195,62.5213203927663,0.));
#164893=CARTESIAN_POINT('Ctrl Pts',(38.5341140796248,62.5059745268901,0.));
#164894=CARTESIAN_POINT('Ctrl Pts',(38.5126062416502,62.4906303334443,0.));
#164895=CARTESIAN_POINT('Ctrl Pts',(38.4911430040997,62.4752879078854,0.));
#164896=CARTESIAN_POINT('Ctrl Pts',(38.4697244150482,62.4599473459811,0.));
#164897=CARTESIAN_POINT('Ctrl Pts',(38.4483505226518,62.4446087438312,0.));
#164898=CARTESIAN_POINT('Ctrl Pts',(38.4270213751568,62.4292721978901,0.));
#164899=CARTESIAN_POINT('Ctrl Pts',(38.405737020905,62.4139378049886,0.));
#164900=CARTESIAN_POINT('Ctrl Pts',(38.3844975083343,62.3986056623577,0.));
#164901=CARTESIAN_POINT('Ctrl Pts',(38.3633028859828,62.3832758676271,0.));
#164902=CARTESIAN_POINT('Ctrl Pts',(38.342153202491,62.3679485188172,0.));
#164903=CARTESIAN_POINT('Ctrl Pts',(38.3210485066001,62.3526237143336,0.));
#164904=CARTESIAN_POINT('Ctrl Pts',(38.2999888471476,62.3373015529613,0.));
#164905=CARTESIAN_POINT('Ctrl Pts',(38.2789742730563,62.3219821338569,0.));
#164906=CARTESIAN_POINT('Ctrl Pts',(38.258004833336,62.3066655565503,0.));
#164907=CARTESIAN_POINT('Ctrl Pts',(38.2370805770935,62.2913519209521,0.));
#164908=CARTESIAN_POINT('Ctrl Pts',(38.2162015535352,62.2760413273602,0.));
#164909=CARTESIAN_POINT('Ctrl Pts',(38.1953678119691,62.2607338764654,0.));
#164910=CARTESIAN_POINT('Ctrl Pts',(38.1745794017995,62.245429669358,0.));
#164911=CARTESIAN_POINT('Ctrl Pts',(38.1538363725263,62.2301288075321,0.));
#164912=CARTESIAN_POINT('Ctrl Pts',(38.1331387737529,62.2148313928863,0.));
#164913=CARTESIAN_POINT('Ctrl Pts',(38.1124866551885,62.1995375277257,0.));
#164914=CARTESIAN_POINT('Ctrl Pts',(38.0918800666479,62.1842473147626,0.));
#164915=CARTESIAN_POINT('Ctrl Pts',(38.0713190580463,62.1689608571176,0.));
#164916=CARTESIAN_POINT('Ctrl Pts',(38.0508036793939,62.1536782583199,0.));
#164917=CARTESIAN_POINT('Ctrl Pts',(38.0303339808053,62.1383996223125,0.));
#164918=CARTESIAN_POINT('Ctrl Pts',(38.0099100125037,62.123125053455,0.));
#164919=CARTESIAN_POINT('Ctrl Pts',(37.9895318248212,62.107854656528,0.));
#164920=CARTESIAN_POINT('Ctrl Pts',(37.9691994681966,62.0925885367352,0.));
#164921=CARTESIAN_POINT('Ctrl Pts',(37.9489129931688,62.0773267997079,0.));
#164922=CARTESIAN_POINT('Ctrl Pts',(37.9286724503851,62.0620695515075,0.));
#164923=CARTESIAN_POINT('Ctrl Pts',(37.9084778906053,62.0468168986288,0.));
#164924=CARTESIAN_POINT('Ctrl Pts',(37.8883293647029,62.031568948002,0.));
#164925=CARTESIAN_POINT('Ctrl Pts',(37.868226923663,62.0163258069957,0.));
#164926=CARTESIAN_POINT('Ctrl Pts',(37.8481706185749,62.0010875834187,0.));
#164927=CARTESIAN_POINT('Ctrl Pts',(37.828160500638,61.9858543855236,0.));
#164928=CARTESIAN_POINT('Ctrl Pts',(37.8081966211688,61.9706263220114,0.));
#164929=CARTESIAN_POINT('Ctrl Pts',(37.7882790316014,61.9554035020338,0.));
#164930=CARTESIAN_POINT('Ctrl Pts',(37.7684077834872,61.9401860351973,0.));
#164931=CARTESIAN_POINT('Ctrl Pts',(37.7485829284871,61.9249740315649,0.));
#164932=CARTESIAN_POINT('Ctrl Pts',(37.7288045183756,61.9097676016601,0.));
#164933=CARTESIAN_POINT('Ctrl Pts',(37.7090726050482,61.8945668564704,0.));
#164934=CARTESIAN_POINT('Ctrl Pts',(37.6893872405228,61.8793719074507,0.));
#164935=CARTESIAN_POINT('Ctrl Pts',(37.6697484769392,61.8641828665262,0.));
#164936=CARTESIAN_POINT('Ctrl Pts',(37.6501563665523,61.8489998460957,0.));
#164937=CARTESIAN_POINT('Ctrl Pts',(37.6306109617346,61.8338229590353,0.));
#164938=CARTESIAN_POINT('Ctrl Pts',(37.6111123149839,61.8186523187015,0.));
#164939=CARTESIAN_POINT('Ctrl Pts',(37.5916604789253,61.8034880389363,0.));
#164940=CARTESIAN_POINT('Ctrl Pts',(37.5722555063111,61.7883302340687,0.));
#164941=CARTESIAN_POINT('Ctrl Pts',(37.5528974500141,61.7731790189191,0.));
#164942=CARTESIAN_POINT('Ctrl Pts',(37.5335863630287,61.7580345088016,0.));
#164943=CARTESIAN_POINT('Ctrl Pts',(37.5143222984795,61.7428968195299,0.));
#164944=CARTESIAN_POINT('Ctrl Pts',(37.4951053096237,61.7277660674205,0.));
#164945=CARTESIAN_POINT('Ctrl Pts',(37.4759354498509,61.7126423692963,0.));
#164946=CARTESIAN_POINT('Ctrl Pts',(37.4568127726773,61.6975258424894,0.));
#164947=CARTESIAN_POINT('Ctrl Pts',(37.4377373317451,61.6824166048444,0.));
#164948=CARTESIAN_POINT('Ctrl Pts',(37.418709180832,61.6673147747242,0.));
#164949=CARTESIAN_POINT('Ctrl Pts',(37.3997283738533,61.6522204710131,0.));
#164950=CARTESIAN_POINT('Ctrl Pts',(37.3807949648624,61.637133813121,0.));
#164951=CARTESIAN_POINT('Ctrl Pts',(37.3619090080449,61.6220549209866,0.));
#164952=CARTESIAN_POINT('Ctrl Pts',(37.343070557718,61.6069839150807,0.));
#164953=CARTESIAN_POINT('Ctrl Pts',(37.3242796683395,61.591920916412,0.));
#164954=CARTESIAN_POINT('Ctrl Pts',(37.3055363945107,61.5768660465311,0.));
#164955=CARTESIAN_POINT('Ctrl Pts',(37.286840790977,61.5618194275348,0.));
#164956=CARTESIAN_POINT('Ctrl Pts',(37.2681929126221,61.5467811820691,0.));
#164957=CARTESIAN_POINT('Ctrl Pts',(37.2495928144666,61.5317514333328,0.));
#164958=CARTESIAN_POINT('Ctrl Pts',(37.2310405516781,61.5167303050832,0.));
#164959=CARTESIAN_POINT('Ctrl Pts',(37.2125361795731,61.501717921641,0.));
#164960=CARTESIAN_POINT('Ctrl Pts',(37.1940797536181,61.4867144078937,0.));
#164961=CARTESIAN_POINT('Ctrl Pts',(37.175671329424,61.4717198892994,0.));
#164962=CARTESIAN_POINT('Ctrl Pts',(37.1573109627454,61.456734491892,0.));
#164963=CARTESIAN_POINT('Ctrl Pts',(37.1389987094904,61.4417583422863,0.));
#164964=CARTESIAN_POINT('Ctrl Pts',(37.1207346257221,61.4267915676822,0.));
#164965=CARTESIAN_POINT('Ctrl Pts',(37.1025187676602,61.4118342958697,0.));
#164966=CARTESIAN_POINT('Ctrl Pts',(37.0843511916744,61.3968866552318,0.));
#164967=CARTESIAN_POINT('Ctrl Pts',(37.0662319542849,61.381948774749,0.));
#164968=CARTESIAN_POINT('Ctrl Pts',(37.0481611121717,61.3670207840069,0.));
#164969=CARTESIAN_POINT('Ctrl Pts',(37.0301387221774,61.3521028132003,0.));
#164970=CARTESIAN_POINT('Ctrl Pts',(37.0121648413081,61.3371949931387,0.));
#164971=CARTESIAN_POINT('Ctrl Pts',(36.994239526727,61.3222974552487,0.));
#164972=CARTESIAN_POINT('Ctrl Pts',(36.9763628357544,61.3074103315792,0.));
#164973=CARTESIAN_POINT('Ctrl Pts',(36.9585348258776,61.2925337548077,0.));
#164974=CARTESIAN_POINT('Ctrl Pts',(36.9407555547534,61.2776678582461,0.));
#164975=CARTESIAN_POINT('Ctrl Pts',(36.9230250802087,61.2628127758457,0.));
#164976=CARTESIAN_POINT('Ctrl Pts',(36.9053434602343,61.247968642201,0.));
#164977=CARTESIAN_POINT('Ctrl Pts',(36.8877107529865,61.2331355925547,0.));
#164978=CARTESIAN_POINT('Ctrl Pts',(36.8701270167969,61.2183137628056,0.));
#164979=CARTESIAN_POINT('Ctrl Pts',(36.852592310174,61.2035032895127,0.));
#164980=CARTESIAN_POINT('Ctrl Pts',(36.8351066918036,61.1887043099014,0.));
#164981=CARTESIAN_POINT('Ctrl Pts',(36.8176702205423,61.1739169618667,0.));
#164982=CARTESIAN_POINT('Ctrl Pts',(36.8002829554209,61.1591413839787,0.));
#164983=CARTESIAN_POINT('Ctrl Pts',(36.7829449556532,61.1443777154911,0.));
#164984=CARTESIAN_POINT('Ctrl Pts',(36.765656280638,61.1296260963466,0.));
#164985=CARTESIAN_POINT('Ctrl Pts',(36.7484169899596,61.1148866671829,0.));
#164986=CARTESIAN_POINT('Ctrl Pts',(36.7312271433807,61.100159569337,0.));
#164987=CARTESIAN_POINT('Ctrl Pts',(36.7140868008486,61.0854449448524,0.));
#164988=CARTESIAN_POINT('Ctrl Pts',(36.6969960225022,61.0707429364847,0.));
#164989=CARTESIAN_POINT('Ctrl Pts',(36.679954868674,61.0560536877083,0.));
#164990=CARTESIAN_POINT('Ctrl Pts',(36.6629633998886,61.0413773427203,0.));
#164991=CARTESIAN_POINT('Ctrl Pts',(36.6460216768553,61.0267140464432,0.));
#164992=CARTESIAN_POINT('Ctrl Pts',(36.6291297604776,61.0120639445349,0.));
#164993=CARTESIAN_POINT('Ctrl Pts',(36.61228771186,60.9974271833981,0.));
#164994=CARTESIAN_POINT('Ctrl Pts',(36.5954955923109,60.9828039101887,0.));
#164995=CARTESIAN_POINT('Ctrl Pts',(36.5787534633415,60.9681942728237,0.));
#164996=CARTESIAN_POINT('Ctrl Pts',(36.5620613866614,60.9535984199873,0.));
#164997=CARTESIAN_POINT('Ctrl Pts',(36.5454194241865,60.9390165011355,0.));
#164998=CARTESIAN_POINT('Ctrl Pts',(36.5288276380416,60.9244486664988,0.));
#164999=CARTESIAN_POINT('Ctrl Pts',(36.5122860905612,60.9098950670847,0.));
#165000=CARTESIAN_POINT('Ctrl Pts',(36.4957948442835,60.8953558546795,0.));
#165001=CARTESIAN_POINT('Ctrl Pts',(36.4793539619466,60.8808311818499,0.));
#165002=CARTESIAN_POINT('Ctrl Pts',(36.4629635065045,60.8663212019657,0.));
#165003=CARTESIAN_POINT('Ctrl Pts',(36.4466235411358,60.8518260692188,0.));
#165004=CARTESIAN_POINT('Ctrl Pts',(36.4303341292494,60.8373459386392,0.));
#165005=CARTESIAN_POINT('Ctrl Pts',(36.4140953344858,60.8228809661161,0.));
#165006=CARTESIAN_POINT('Ctrl Pts',(36.397907220716,60.8084313083984,0.));
#165007=CARTESIAN_POINT('Ctrl Pts',(36.3817698520388,60.7939971230761,0.));
#165008=CARTESIAN_POINT('Ctrl Pts',(36.365683292773,60.7795785685625,0.));
#165009=CARTESIAN_POINT('Ctrl Pts',(36.3496476074488,60.7651758040804,0.));
#165010=CARTESIAN_POINT('Ctrl Pts',(36.3336628607858,60.7507889896308,0.));
#165011=CARTESIAN_POINT('Ctrl Pts',(36.3177291177163,60.7364182860412,0.));
#165012=CARTESIAN_POINT('Ctrl Pts',(36.3018464434213,60.722063855041,0.));
#165013=CARTESIAN_POINT('Ctrl Pts',(36.2860149033587,60.7077258593268,0.));
#165014=CARTESIAN_POINT('Ctrl Pts',(36.2702345632875,60.6934044626291,0.));
#165015=CARTESIAN_POINT('Ctrl Pts',(36.2545054892897,60.67909982978,0.));
#165016=CARTESIAN_POINT('Ctrl Pts',(36.2388277477212,60.6648121265885,0.));
#165017=CARTESIAN_POINT('Ctrl Pts',(36.2232014051541,60.6505415197042,0.));
#165018=CARTESIAN_POINT('Ctrl Pts',(36.2076265283264,60.6362881765019,0.));
#165019=CARTESIAN_POINT('Ctrl Pts',(36.1921031840629,60.6220522649149,0.));
#165020=CARTESIAN_POINT('Ctrl Pts',(36.1766314392641,60.6078339534181,0.));
#165021=CARTESIAN_POINT('Ctrl Pts',(36.1612113610773,60.5936334114108,0.));
#165022=CARTESIAN_POINT('Ctrl Pts',(36.145843017043,60.5794508095565,0.));
#165023=CARTESIAN_POINT('Ctrl Pts',(36.1305264752187,60.565286320072,0.));
#165024=CARTESIAN_POINT('Ctrl Pts',(36.1152618043738,60.5511401171984,0.));
#165025=CARTESIAN_POINT('Ctrl Pts',(36.100049073851,60.5370123768804,0.));
#165026=CARTESIAN_POINT('Ctrl Pts',(36.0848883531952,60.5229032758974,0.));
#165027=CARTESIAN_POINT('Ctrl Pts',(36.0697797118375,60.5088129911354,0.));
#165028=CARTESIAN_POINT('Ctrl Pts',(36.0547232187697,60.4947416988422,0.));
#165029=CARTESIAN_POINT('Ctrl Pts',(36.0397189421644,60.4806895737686,0.));
#165030=CARTESIAN_POINT('Ctrl Pts',(36.0247669500891,60.4666567908093,0.));
#165031=CARTESIAN_POINT('Ctrl Pts',(36.009867311357,60.4526435269662,0.));
#165032=CARTESIAN_POINT('Ctrl Pts',(35.995020096217,60.4386499629481,0.));
#165033=CARTESIAN_POINT('Ctrl Pts',(35.9802253773514,60.4246762854926,0.));
#165034=CARTESIAN_POINT('Ctrl Pts',(35.9654832299601,60.4107226875714,0.));
#165035=CARTESIAN_POINT('Ctrl Pts',(35.9507937296706,60.3967893635452,0.));
#165036=CARTESIAN_POINT('Ctrl Pts',(35.9361569506949,60.3828765049019,0.));
#165037=CARTESIAN_POINT('Ctrl Pts',(35.9215729642231,60.3689842965481,0.));
#165038=CARTESIAN_POINT('Ctrl Pts',(35.907041835853,60.3551129108845,0.));
#165039=CARTESIAN_POINT('Ctrl Pts',(35.8925636280668,60.3412625135287,0.));
#165040=CARTESIAN_POINT('Ctrl Pts',(35.8781384051536,60.327433274683,0.));
#165041=CARTESIAN_POINT('Ctrl Pts',(35.8637662371635,60.313625378281,0.));
#165042=CARTESIAN_POINT('Ctrl Pts',(35.8494472046745,60.2998390330102,0.));
#165043=CARTESIAN_POINT('Ctrl Pts',(35.8351814020356,60.2860744798436,0.));
#165044=CARTESIAN_POINT('Ctrl Pts',(35.82096892725,60.2723319687369,0.));
#165045=CARTESIAN_POINT('Ctrl Pts',(35.8068098723347,60.2586117365205,0.));
#165046=CARTESIAN_POINT('Ctrl Pts',(35.7927043145201,60.2449139865275,0.));
#165047=CARTESIAN_POINT('Ctrl Pts',(35.7786523045911,60.2312388621529,0.));
#165048=CARTESIAN_POINT('Ctrl Pts',(35.7646538667493,60.2175864450043,0.));
#165049=CARTESIAN_POINT('Ctrl Pts',(35.7534979802053,60.206682708692,0.));
#165050=CARTESIAN_POINT('Ctrl Pts',(35.7451551752572,60.1985151474623,0.));
#165051=CARTESIAN_POINT('Ctrl Pts',(35.7396040204017,60.193074658032,0.));
#165052=CARTESIAN_POINT('Ctrl Pts',(35.7368311217509,60.1903555511633,0.));
#165053=CARTESIAN_POINT('Ctrl Pts',(44.8554660179045,59.483083043136,0.));
#165054=CARTESIAN_POINT('Ctrl Pts',(44.8554660179045,59.483083043136,12.));
#165055=CARTESIAN_POINT('Ctrl Pts',(44.850535982646,59.4804358983083,0.));
#165056=CARTESIAN_POINT('Ctrl Pts',(44.850535982646,59.4804358983083,12.));
#165057=CARTESIAN_POINT('Ctrl Pts',(44.8406801497742,59.4751410547732,0.));
#165058=CARTESIAN_POINT('Ctrl Pts',(44.8406801497742,59.4751410547732,12.));
#165059=CARTESIAN_POINT('Ctrl Pts',(44.8259091134015,59.4671971278321,0.));
#165060=CARTESIAN_POINT('Ctrl Pts',(44.8259091134015,59.4671971278321,12.));
#165061=CARTESIAN_POINT('Ctrl Pts',(44.8062398251406,59.4566019018254,0.));
#165062=CARTESIAN_POINT('Ctrl Pts',(44.8062398251406,59.4566019018254,12.));
#165063=CARTESIAN_POINT('Ctrl Pts',(44.7816956017528,59.4433523335147,0.));
#165064=CARTESIAN_POINT('Ctrl Pts',(44.7816956017528,59.4433523335147,12.));
#165065=CARTESIAN_POINT('Ctrl Pts',(44.7571937812113,59.4300972403241,0.));
#165066=CARTESIAN_POINT('Ctrl Pts',(44.7571937812113,59.4300972403241,12.));
#165067=CARTESIAN_POINT('Ctrl Pts',(44.7327343876391,59.4168366453118,0.));
#165068=CARTESIAN_POINT('Ctrl Pts',(44.7327343876391,59.4168366453118,12.));
#165069=CARTESIAN_POINT('Ctrl Pts',(44.7083174541702,59.4035705873811,0.));
#165070=CARTESIAN_POINT('Ctrl Pts',(44.7083174541702,59.4035705873811,12.));
#165071=CARTESIAN_POINT('Ctrl Pts',(44.683943024421,59.3902991267889,0.));
#165072=CARTESIAN_POINT('Ctrl Pts',(44.683943024421,59.3902991267889,12.));
#165073=CARTESIAN_POINT('Ctrl Pts',(44.6596111512687,59.377022343519,0.));
#165074=CARTESIAN_POINT('Ctrl Pts',(44.6596111512687,59.377022343519,12.));
#165075=CARTESIAN_POINT('Ctrl Pts',(44.6353218935685,59.3637403301801,0.));
#165076=CARTESIAN_POINT('Ctrl Pts',(44.6353218935685,59.3637403301801,12.));
#165077=CARTESIAN_POINT('Ctrl Pts',(44.6110753134277,59.3504531864154,0.));
#165078=CARTESIAN_POINT('Ctrl Pts',(44.6110753134277,59.3504531864154,12.));
#165079=CARTESIAN_POINT('Ctrl Pts',(44.5868714733234,59.3371610128511,0.));
#165080=CARTESIAN_POINT('Ctrl Pts',(44.5868714733234,59.3371610128511,12.));
#165081=CARTESIAN_POINT('Ctrl Pts',(44.5627104331017,59.3238639048694,0.));
#165082=CARTESIAN_POINT('Ctrl Pts',(44.5627104331017,59.3238639048694,12.));
#165083=CARTESIAN_POINT('Ctrl Pts',(44.5385922475573,59.3105619475609,0.));
#165084=CARTESIAN_POINT('Ctrl Pts',(44.5385922475573,59.3105619475609,12.));
#165085=CARTESIAN_POINT('Ctrl Pts',(44.5145169681349,59.2972552192156,0.));
#165086=CARTESIAN_POINT('Ctrl Pts',(44.5145169681349,59.2972552192156,12.));
#165087=CARTESIAN_POINT('Ctrl Pts',(44.490484644151,59.2839437938237,0.));
#165088=CARTESIAN_POINT('Ctrl Pts',(44.490484644151,59.2839437938237,12.));
#165089=CARTESIAN_POINT('Ctrl Pts',(44.4664953242378,59.2706277440445,0.));
#165090=CARTESIAN_POINT('Ctrl Pts',(44.4664953242378,59.2706277440445,12.));
#165091=CARTESIAN_POINT('Ctrl Pts',(44.4425490575911,59.2573071437774,0.));
#165092=CARTESIAN_POINT('Ctrl Pts',(44.4425490575911,59.2573071437774,12.));
#165093=CARTESIAN_POINT('Ctrl Pts',(44.418645895545,59.2439820714187,0.));
#165094=CARTESIAN_POINT('Ctrl Pts',(44.418645895545,59.2439820714187,12.));
#165095=CARTESIAN_POINT('Ctrl Pts',(44.3947858914074,59.2306526095131,0.));
#165096=CARTESIAN_POINT('Ctrl Pts',(44.3947858914074,59.2306526095131,12.));
#165097=CARTESIAN_POINT('Ctrl Pts',(44.3709690997469,59.2173188432798,0.));
#165098=CARTESIAN_POINT('Ctrl Pts',(44.3709690997469,59.2173188432798,12.));
#165099=CARTESIAN_POINT('Ctrl Pts',(44.3471955758402,59.2039808594752,0.));
#165100=CARTESIAN_POINT('Ctrl Pts',(44.3471955758402,59.2039808594752,12.));
#165101=CARTESIAN_POINT('Ctrl Pts',(44.3234653750884,59.1906387451979,0.));
#165102=CARTESIAN_POINT('Ctrl Pts',(44.3234653750884,59.1906387451979,12.));
#165103=CARTESIAN_POINT('Ctrl Pts',(44.2997785523431,59.1772925865213,0.));
#165104=CARTESIAN_POINT('Ctrl Pts',(44.2997785523431,59.1772925865213,12.));
#165105=CARTESIAN_POINT('Ctrl Pts',(44.2761351616048,59.1639424678793,0.));
#165106=CARTESIAN_POINT('Ctrl Pts',(44.2761351616048,59.1639424678793,12.));
#165107=CARTESIAN_POINT('Ctrl Pts',(44.2525352563996,59.1505884728215,0.));
#165108=CARTESIAN_POINT('Ctrl Pts',(44.2525352563996,59.1505884728215,12.));
#165109=CARTESIAN_POINT('Ctrl Pts',(44.228978889997,59.1372306844586,0.));
#165110=CARTESIAN_POINT('Ctrl Pts',(44.228978889997,59.1372306844586,12.));
#165111=CARTESIAN_POINT('Ctrl Pts',(44.2054661156875,59.1238691860306,0.));
#165112=CARTESIAN_POINT('Ctrl Pts',(44.2054661156875,59.1238691860306,12.));
#165113=CARTESIAN_POINT('Ctrl Pts',(44.1819969870307,59.1105040614276,0.));
#165114=CARTESIAN_POINT('Ctrl Pts',(44.1819969870307,59.1105040614276,12.));
#165115=CARTESIAN_POINT('Ctrl Pts',(44.1585715581064,59.0971353957206,0.));
#165116=CARTESIAN_POINT('Ctrl Pts',(44.1585715581064,59.0971353957206,12.));
#165117=CARTESIAN_POINT('Ctrl Pts',(44.1351898834051,59.08376327492,0.));
#165118=CARTESIAN_POINT('Ctrl Pts',(44.1351898834051,59.08376327492,12.));
#165119=CARTESIAN_POINT('Ctrl Pts',(44.1118520177221,59.0703877857526,0.));
#165120=CARTESIAN_POINT('Ctrl Pts',(44.1118520177221,59.0703877857526,12.));
#165121=CARTESIAN_POINT('Ctrl Pts',(44.0885580160432,59.0570090154242,0.));
#165122=CARTESIAN_POINT('Ctrl Pts',(44.0885580160432,59.0570090154242,12.));
#165123=CARTESIAN_POINT('Ctrl Pts',(44.0653079334385,59.0436270514087,0.));
#165124=CARTESIAN_POINT('Ctrl Pts',(44.0653079334385,59.0436270514087,12.));
#165125=CARTESIAN_POINT('Ctrl Pts',(44.0421018249223,59.0302419811777,0.));
#165126=CARTESIAN_POINT('Ctrl Pts',(44.0421018249223,59.0302419811777,12.));
#165127=CARTESIAN_POINT('Ctrl Pts',(44.0189397454599,59.0168538922095,0.));
#165128=CARTESIAN_POINT('Ctrl Pts',(44.0189397454599,59.0168538922095,12.));
#165129=CARTESIAN_POINT('Ctrl Pts',(43.9958217500369,59.0034628721168,0.));
#165130=CARTESIAN_POINT('Ctrl Pts',(43.9958217500369,59.0034628721168,12.));
#165131=CARTESIAN_POINT('Ctrl Pts',(43.9727478937056,58.9900690087408,0.));
#165132=CARTESIAN_POINT('Ctrl Pts',(43.9727478937056,58.9900690087408,12.));
#165133=CARTESIAN_POINT('Ctrl Pts',(43.9497182316331,58.9766723902529,0.));
#165134=CARTESIAN_POINT('Ctrl Pts',(43.9497182316331,58.9766723902529,12.));
#165135=CARTESIAN_POINT('Ctrl Pts',(43.9267328191501,58.9632731052696,0.));
#165136=CARTESIAN_POINT('Ctrl Pts',(43.9267328191501,58.9632731052696,12.));
#165137=CARTESIAN_POINT('Ctrl Pts',(43.9037917117739,58.9498712429054,0.));
#165138=CARTESIAN_POINT('Ctrl Pts',(43.9037917117739,58.9498712429054,12.));
#165139=CARTESIAN_POINT('Ctrl Pts',(43.8808949651872,58.936466892712,0.));
#165140=CARTESIAN_POINT('Ctrl Pts',(43.8808949651872,58.936466892712,12.));
#165141=CARTESIAN_POINT('Ctrl Pts',(43.858042635223,58.9230601446436,0.));
#165142=CARTESIAN_POINT('Ctrl Pts',(43.858042635223,58.9230601446436,12.));
#165143=CARTESIAN_POINT('Ctrl Pts',(43.835234777842,58.9096510890129,0.));
#165144=CARTESIAN_POINT('Ctrl Pts',(43.835234777842,58.9096510890129,12.));
#165145=CARTESIAN_POINT('Ctrl Pts',(43.8124714491076,58.8962398164493,0.));
#165146=CARTESIAN_POINT('Ctrl Pts',(43.8124714491076,58.8962398164493,12.));
#165147=CARTESIAN_POINT('Ctrl Pts',(43.7897527051609,58.8828264178621,0.));
#165148=CARTESIAN_POINT('Ctrl Pts',(43.7897527051609,58.8828264178621,12.));
#165149=CARTESIAN_POINT('Ctrl Pts',(43.7670786022402,58.8694109844648,0.));
#165150=CARTESIAN_POINT('Ctrl Pts',(43.7670786022402,58.8694109844648,12.));
#165151=CARTESIAN_POINT('Ctrl Pts',(43.7444491966942,58.8559936077941,0.));
#165152=CARTESIAN_POINT('Ctrl Pts',(43.7444491966942,58.8559936077941,12.));
#165153=CARTESIAN_POINT('Ctrl Pts',(43.7218645449922,58.8425743797326,0.));
#165154=CARTESIAN_POINT('Ctrl Pts',(43.7218645449922,58.8425743797326,12.));
#165155=CARTESIAN_POINT('Ctrl Pts',(43.6993247037314,58.8291533925293,0.));
#165156=CARTESIAN_POINT('Ctrl Pts',(43.6993247037314,58.8291533925293,12.));
#165157=CARTESIAN_POINT('Ctrl Pts',(43.6768297296395,58.8157307388238,0.));
#165158=CARTESIAN_POINT('Ctrl Pts',(43.6768297296395,58.8157307388238,12.));
#165159=CARTESIAN_POINT('Ctrl Pts',(43.6543796795789,58.8023065116436,0.));
#165160=CARTESIAN_POINT('Ctrl Pts',(43.6543796795789,58.8023065116436,12.));
#165161=CARTESIAN_POINT('Ctrl Pts',(43.6319746105482,58.788880804397,0.));
#165162=CARTESIAN_POINT('Ctrl Pts',(43.6319746105482,58.788880804397,12.));
#165163=CARTESIAN_POINT('Ctrl Pts',(43.6096145796796,58.775453710867,0.));
#165164=CARTESIAN_POINT('Ctrl Pts',(43.6096145796796,58.775453710867,12.));
#165165=CARTESIAN_POINT('Ctrl Pts',(43.5872996442345,58.7620253252062,0.));
#165166=CARTESIAN_POINT('Ctrl Pts',(43.5872996442345,58.7620253252062,12.));
#165167=CARTESIAN_POINT('Ctrl Pts',(43.5650298615916,58.74859574193,0.));
#165168=CARTESIAN_POINT('Ctrl Pts',(43.5650298615916,58.74859574193,12.));
#165169=CARTESIAN_POINT('Ctrl Pts',(43.5428052892488,58.7351650559181,0.));
#165170=CARTESIAN_POINT('Ctrl Pts',(43.5428052892488,58.7351650559181,12.));
#165171=CARTESIAN_POINT('Ctrl Pts',(43.5206259848337,58.7217333624209,0.));
#165172=CARTESIAN_POINT('Ctrl Pts',(43.5206259848337,58.7217333624209,12.));
#165173=CARTESIAN_POINT('Ctrl Pts',(43.4984920061073,58.7083007570661,0.));
#165174=CARTESIAN_POINT('Ctrl Pts',(43.4984920061073,58.7083007570661,12.));
#165175=CARTESIAN_POINT('Ctrl Pts',(43.4764034109654,58.6948673358638,0.));
#165176=CARTESIAN_POINT('Ctrl Pts',(43.4764034109654,58.6948673358638,12.));
#165177=CARTESIAN_POINT('Ctrl Pts',(43.4543602574351,58.6814331952138,0.));
#165178=CARTESIAN_POINT('Ctrl Pts',(43.4543602574351,58.6814331952138,12.));
#165179=CARTESIAN_POINT('Ctrl Pts',(43.4323626036736,58.6679984319097,0.));
#165180=CARTESIAN_POINT('Ctrl Pts',(43.4323626036736,58.6679984319097,12.));
#165181=CARTESIAN_POINT('Ctrl Pts',(43.4104105079768,58.6545631431393,0.));
#165182=CARTESIAN_POINT('Ctrl Pts',(43.4104105079768,58.6545631431393,12.));
#165183=CARTESIAN_POINT('Ctrl Pts',(43.388504028781,58.6411274264857,0.));
#165184=CARTESIAN_POINT('Ctrl Pts',(43.388504028781,58.6411274264857,12.));
#165185=CARTESIAN_POINT('Ctrl Pts',(43.3666432246635,58.627691379929,0.));
#165186=CARTESIAN_POINT('Ctrl Pts',(43.3666432246635,58.627691379929,12.));
#165187=CARTESIAN_POINT('Ctrl Pts',(43.3448281543371,58.6142551018467,0.));
#165188=CARTESIAN_POINT('Ctrl Pts',(43.3448281543371,58.6142551018467,12.));
#165189=CARTESIAN_POINT('Ctrl Pts',(43.3230588766449,58.6008186910156,0.));
#165190=CARTESIAN_POINT('Ctrl Pts',(43.3230588766449,58.6008186910156,12.));
#165191=CARTESIAN_POINT('Ctrl Pts',(43.3013354505701,58.5873822466152,0.));
#165192=CARTESIAN_POINT('Ctrl Pts',(43.3013354505701,58.5873822466152,12.));
#165193=CARTESIAN_POINT('Ctrl Pts',(43.27965793524,58.573945868231,0.));
#165194=CARTESIAN_POINT('Ctrl Pts',(43.27965793524,58.573945868231,12.));
#165195=CARTESIAN_POINT('Ctrl Pts',(43.2580263899278,58.5605096558578,0.));
#165196=CARTESIAN_POINT('Ctrl Pts',(43.2580263899278,58.5605096558578,12.));
#165197=CARTESIAN_POINT('Ctrl Pts',(43.2364408740493,58.5470737099032,0.));
#165198=CARTESIAN_POINT('Ctrl Pts',(43.2364408740493,58.5470737099032,12.));
#165199=CARTESIAN_POINT('Ctrl Pts',(43.2149014471574,58.5336381311917,0.));
#165200=CARTESIAN_POINT('Ctrl Pts',(43.2149014471574,58.5336381311917,12.));
#165201=CARTESIAN_POINT('Ctrl Pts',(43.1934081689505,58.5202030209669,0.));
#165202=CARTESIAN_POINT('Ctrl Pts',(43.1934081689505,58.5202030209669,12.));
#165203=CARTESIAN_POINT('Ctrl Pts',(43.1719610992771,58.5067684808944,0.));
#165204=CARTESIAN_POINT('Ctrl Pts',(43.1719610992771,58.5067684808944,12.));
#165205=CARTESIAN_POINT('Ctrl Pts',(43.1505602981365,58.4933346130636,0.));
#165206=CARTESIAN_POINT('Ctrl Pts',(43.1505602981365,58.4933346130636,12.));
#165207=CARTESIAN_POINT('Ctrl Pts',(43.1292058256776,58.4799015199907,0.));
#165208=CARTESIAN_POINT('Ctrl Pts',(43.1292058256776,58.4799015199907,12.));
#165209=CARTESIAN_POINT('Ctrl Pts',(43.1078977421916,58.4664693046217,0.));
#165210=CARTESIAN_POINT('Ctrl Pts',(43.1078977421916,58.4664693046217,12.));
#165211=CARTESIAN_POINT('Ctrl Pts',(43.0866361081177,58.4530380703349,0.));
#165212=CARTESIAN_POINT('Ctrl Pts',(43.0866361081177,58.4530380703349,12.));
#165213=CARTESIAN_POINT('Ctrl Pts',(43.0654209840511,58.4396079209451,0.));
#165214=CARTESIAN_POINT('Ctrl Pts',(43.0654209840511,58.4396079209451,12.));
#165215=CARTESIAN_POINT('Ctrl Pts',(43.0442524307434,58.4261789607058,0.));
#165216=CARTESIAN_POINT('Ctrl Pts',(43.0442524307434,58.4261789607058,12.));
#165217=CARTESIAN_POINT('Ctrl Pts',(43.0231305091027,58.4127512943136,0.));
#165218=CARTESIAN_POINT('Ctrl Pts',(43.0231305091027,58.4127512943136,12.));
#165219=CARTESIAN_POINT('Ctrl Pts',(43.0020552801859,58.3993250269101,0.));
#165220=CARTESIAN_POINT('Ctrl Pts',(43.0020552801859,58.3993250269101,12.));
#165221=CARTESIAN_POINT('Ctrl Pts',(42.9810268052032,58.3859002640857,0.));
#165222=CARTESIAN_POINT('Ctrl Pts',(42.9810268052032,58.3859002640857,12.));
#165223=CARTESIAN_POINT('Ctrl Pts',(42.960045145526,58.3724771118826,0.));
#165224=CARTESIAN_POINT('Ctrl Pts',(42.960045145526,58.3724771118826,12.));
#165225=CARTESIAN_POINT('Ctrl Pts',(42.9391103626879,58.3590556767978,0.));
#165226=CARTESIAN_POINT('Ctrl Pts',(42.9391103626879,58.3590556767978,12.));
#165227=CARTESIAN_POINT('Ctrl Pts',(42.9182225183854,58.3456360657865,0.));
#165228=CARTESIAN_POINT('Ctrl Pts',(42.9182225183854,58.3456360657865,12.));
#165229=CARTESIAN_POINT('Ctrl Pts',(42.8973816744709,58.3322183862654,0.));
#165230=CARTESIAN_POINT('Ctrl Pts',(42.8973816744709,58.3322183862654,12.));
#165231=CARTESIAN_POINT('Ctrl Pts',(42.8765878929551,58.3188027461164,0.));
#165232=CARTESIAN_POINT('Ctrl Pts',(42.8765878929551,58.3188027461164,12.));
#165233=CARTESIAN_POINT('Ctrl Pts',(42.8558412360158,58.3053892536894,0.));
#165234=CARTESIAN_POINT('Ctrl Pts',(42.8558412360158,58.3053892536894,12.));
#165235=CARTESIAN_POINT('Ctrl Pts',(42.8351417659999,58.2919780178064,0.));
#165236=CARTESIAN_POINT('Ctrl Pts',(42.8351417659999,58.2919780178064,12.));
#165237=CARTESIAN_POINT('Ctrl Pts',(42.8144895454233,58.2785691477638,0.));
#165238=CARTESIAN_POINT('Ctrl Pts',(42.8144895454233,58.2785691477638,12.));
#165239=CARTESIAN_POINT('Ctrl Pts',(42.7938846369651,58.2651627533368,0.));
#165240=CARTESIAN_POINT('Ctrl Pts',(42.7938846369651,58.2651627533368,12.));
#165241=CARTESIAN_POINT('Ctrl Pts',(42.7733271034679,58.2517589447821,0.));
#165242=CARTESIAN_POINT('Ctrl Pts',(42.7733271034679,58.2517589447821,12.));
#165243=CARTESIAN_POINT('Ctrl Pts',(42.7528170079484,58.2383578328424,0.));
#165244=CARTESIAN_POINT('Ctrl Pts',(42.7528170079484,58.2383578328424,12.));
#165245=CARTESIAN_POINT('Ctrl Pts',(42.7323544135985,58.22495952875,0.));
#165246=CARTESIAN_POINT('Ctrl Pts',(42.7323544135985,58.22495952875,12.));
#165247=CARTESIAN_POINT('Ctrl Pts',(42.7119393837866,58.21156414423,0.));
#165248=CARTESIAN_POINT('Ctrl Pts',(42.7119393837866,58.21156414423,12.));
#165249=CARTESIAN_POINT('Ctrl Pts',(42.6915719820513,58.1981717915037,0.));
#165250=CARTESIAN_POINT('Ctrl Pts',(42.6915719820513,58.1981717915037,12.));
#165251=CARTESIAN_POINT('Ctrl Pts',(42.6712522721016,58.1847825832923,0.));
#165252=CARTESIAN_POINT('Ctrl Pts',(42.6712522721016,58.1847825832923,12.));
#165253=CARTESIAN_POINT('Ctrl Pts',(42.6509803178265,58.171396632821,0.));
#165254=CARTESIAN_POINT('Ctrl Pts',(42.6509803178265,58.171396632821,12.));
#165255=CARTESIAN_POINT('Ctrl Pts',(42.6307561832976,58.1580140538228,0.));
#165256=CARTESIAN_POINT('Ctrl Pts',(42.6307561832976,58.1580140538228,12.));
#165257=CARTESIAN_POINT('Ctrl Pts',(42.6105799327699,58.1446349605421,0.));
#165258=CARTESIAN_POINT('Ctrl Pts',(42.6105799327699,58.1446349605421,12.));
#165259=CARTESIAN_POINT('Ctrl Pts',(42.5904516306762,58.1312594677386,0.));
#165260=CARTESIAN_POINT('Ctrl Pts',(42.5904516306762,58.1312594677386,12.));
#165261=CARTESIAN_POINT('Ctrl Pts',(42.5703713416265,58.1178876906907,0.));
#165262=CARTESIAN_POINT('Ctrl Pts',(42.5703713416265,58.1178876906907,12.));
#165263=CARTESIAN_POINT('Ctrl Pts',(42.5503391304183,58.1045197452003,0.));
#165264=CARTESIAN_POINT('Ctrl Pts',(42.5503391304183,58.1045197452003,12.));
#165265=CARTESIAN_POINT('Ctrl Pts',(42.5303550620387,58.0911557475965,0.));
#165266=CARTESIAN_POINT('Ctrl Pts',(42.5303550620387,58.0911557475965,12.));
#165267=CARTESIAN_POINT('Ctrl Pts',(42.5104192016664,58.0777958147403,0.));
#165268=CARTESIAN_POINT('Ctrl Pts',(42.5104192016664,58.0777958147403,12.));
#165269=CARTESIAN_POINT('Ctrl Pts',(42.4905316146653,58.0644400640275,0.));
#165270=CARTESIAN_POINT('Ctrl Pts',(42.4905316146653,58.0644400640275,12.));
#165271=CARTESIAN_POINT('Ctrl Pts',(42.4706923665845,58.0510886133926,0.));
#165272=CARTESIAN_POINT('Ctrl Pts',(42.4706923665845,58.0510886133926,12.));
#165273=CARTESIAN_POINT('Ctrl Pts',(42.4509015231674,58.037741581314,0.));
#165274=CARTESIAN_POINT('Ctrl Pts',(42.4509015231674,58.037741581314,12.));
#165275=CARTESIAN_POINT('Ctrl Pts',(42.4311591503555,58.0243990868181,0.));
#165276=CARTESIAN_POINT('Ctrl Pts',(42.4311591503555,58.0243990868181,12.));
#165277=CARTESIAN_POINT('Ctrl Pts',(42.411465314289,58.0110612494828,0.));
#165278=CARTESIAN_POINT('Ctrl Pts',(42.411465314289,58.0110612494828,12.));
#165279=CARTESIAN_POINT('Ctrl Pts',(42.3918200813014,57.9977281894422,0.));
#165280=CARTESIAN_POINT('Ctrl Pts',(42.3918200813014,57.9977281894422,12.));
#165281=CARTESIAN_POINT('Ctrl Pts',(42.3722235179197,57.9844000273911,0.));
#165282=CARTESIAN_POINT('Ctrl Pts',(42.3722235179197,57.9844000273911,12.));
#165283=CARTESIAN_POINT('Ctrl Pts',(42.3526756908746,57.9710768845899,0.));
#165284=CARTESIAN_POINT('Ctrl Pts',(42.3526756908746,57.9710768845899,12.));
#165285=CARTESIAN_POINT('Ctrl Pts',(42.333176667102,57.9577588828683,0.));
#165286=CARTESIAN_POINT('Ctrl Pts',(42.333176667102,57.9577588828683,12.));
#165287=CARTESIAN_POINT('Ctrl Pts',(42.3137265137452,57.9444461446299,0.));
#165288=CARTESIAN_POINT('Ctrl Pts',(42.3137265137452,57.9444461446299,12.));
#165289=CARTESIAN_POINT('Ctrl Pts',(42.2943252981489,57.9311387928563,0.));
#165290=CARTESIAN_POINT('Ctrl Pts',(42.2943252981489,57.9311387928563,12.));
#165291=CARTESIAN_POINT('Ctrl Pts',(42.2749730878594,57.9178369511114,0.));
#165292=CARTESIAN_POINT('Ctrl Pts',(42.2749730878594,57.9178369511114,12.));
#165293=CARTESIAN_POINT('Ctrl Pts',(42.2556699506353,57.9045407435474,0.));
#165294=CARTESIAN_POINT('Ctrl Pts',(42.2556699506353,57.9045407435474,12.));
#165295=CARTESIAN_POINT('Ctrl Pts',(42.2364159544501,57.8912502949096,0.));
#165296=CARTESIAN_POINT('Ctrl Pts',(42.2364159544501,57.8912502949096,12.));
#165297=CARTESIAN_POINT('Ctrl Pts',(42.2172111674938,57.8779657305413,0.));
#165298=CARTESIAN_POINT('Ctrl Pts',(42.2172111674938,57.8779657305413,12.));
#165299=CARTESIAN_POINT('Ctrl Pts',(42.1980556581665,57.864687176387,0.));
#165300=CARTESIAN_POINT('Ctrl Pts',(42.1980556581665,57.864687176387,12.));
#165301=CARTESIAN_POINT('Ctrl Pts',(42.1789494950794,57.8514147589972,0.));
#165302=CARTESIAN_POINT('Ctrl Pts',(42.1789494950794,57.8514147589972,12.));
#165303=CARTESIAN_POINT('Ctrl Pts',(42.1598927470646,57.8381486055342,0.));
#165304=CARTESIAN_POINT('Ctrl Pts',(42.1598927470646,57.8381486055342,12.));
#165305=CARTESIAN_POINT('Ctrl Pts',(42.1408854831783,57.8248888437775,0.));
#165306=CARTESIAN_POINT('Ctrl Pts',(42.1408854831783,57.8248888437775,12.));
#165307=CARTESIAN_POINT('Ctrl Pts',(42.121927772702,57.8116356021288,0.));
#165308=CARTESIAN_POINT('Ctrl Pts',(42.121927772702,57.8116356021288,12.));
#165309=CARTESIAN_POINT('Ctrl Pts',(42.1030196851366,57.798389009616,0.));
#165310=CARTESIAN_POINT('Ctrl Pts',(42.1030196851366,57.798389009616,12.));
#165311=CARTESIAN_POINT('Ctrl Pts',(42.0841612902042,57.7851491958987,0.));
#165312=CARTESIAN_POINT('Ctrl Pts',(42.0841612902042,57.7851491958987,12.));
#165313=CARTESIAN_POINT('Ctrl Pts',(42.0653526578588,57.7719162912744,0.));
#165314=CARTESIAN_POINT('Ctrl Pts',(42.0653526578588,57.7719162912744,12.));
#165315=CARTESIAN_POINT('Ctrl Pts',(42.0465938582882,57.7586904266834,0.));
#165316=CARTESIAN_POINT('Ctrl Pts',(42.0465938582882,57.7586904266834,12.));
#165317=CARTESIAN_POINT('Ctrl Pts',(42.0278849619148,57.745471733714,0.));
#165318=CARTESIAN_POINT('Ctrl Pts',(42.0278849619148,57.745471733714,12.));
#165319=CARTESIAN_POINT('Ctrl Pts',(42.0092260393897,57.7322603446066,0.));
#165320=CARTESIAN_POINT('Ctrl Pts',(42.0092260393897,57.7322603446066,12.));
#165321=CARTESIAN_POINT('Ctrl Pts',(41.990617161596,57.7190563922593,0.));
#165322=CARTESIAN_POINT('Ctrl Pts',(41.990617161596,57.7190563922593,12.));
#165323=CARTESIAN_POINT('Ctrl Pts',(41.9720583996592,57.7058600102351,0.));
#165324=CARTESIAN_POINT('Ctrl Pts',(41.9720583996592,57.7058600102351,12.));
#165325=CARTESIAN_POINT('Ctrl Pts',(41.9535498249488,57.6926713327672,0.));
#165326=CARTESIAN_POINT('Ctrl Pts',(41.9535498249488,57.6926713327672,12.));
#165327=CARTESIAN_POINT('Ctrl Pts',(41.9350915090796,57.6794904947649,0.));
#165328=CARTESIAN_POINT('Ctrl Pts',(41.9350915090796,57.6794904947649,12.));
#165329=CARTESIAN_POINT('Ctrl Pts',(41.9166835239054,57.6663176318189,0.));
#165330=CARTESIAN_POINT('Ctrl Pts',(41.9166835239054,57.6663176318189,12.));
#165331=CARTESIAN_POINT('Ctrl Pts',(41.8983259415253,57.6531528802072,0.));
#165332=CARTESIAN_POINT('Ctrl Pts',(41.8983259415253,57.6531528802072,12.));
#165333=CARTESIAN_POINT('Ctrl Pts',(41.8800188342912,57.6399963769009,0.));
#165334=CARTESIAN_POINT('Ctrl Pts',(41.8800188342912,57.6399963769009,12.));
#165335=CARTESIAN_POINT('Ctrl Pts',(41.8617622748107,57.6268482595701,0.));
#165336=CARTESIAN_POINT('Ctrl Pts',(41.8617622748107,57.6268482595701,12.));
#165337=CARTESIAN_POINT('Ctrl Pts',(41.8435563359456,57.613708666588,0.));
#165338=CARTESIAN_POINT('Ctrl Pts',(41.8435563359456,57.613708666588,12.));
#165339=CARTESIAN_POINT('Ctrl Pts',(41.8254010908051,57.6005777370347,0.));
#165340=CARTESIAN_POINT('Ctrl Pts',(41.8254010908051,57.6005777370347,12.));
#165341=CARTESIAN_POINT('Ctrl Pts',(41.8072966127559,57.5874556107054,0.));
#165342=CARTESIAN_POINT('Ctrl Pts',(41.8072966127559,57.5874556107054,12.));
#165343=CARTESIAN_POINT('Ctrl Pts',(41.7892429754298,57.5743424281204,0.));
#165344=CARTESIAN_POINT('Ctrl Pts',(41.7892429754298,57.5743424281204,12.));
#165345=CARTESIAN_POINT('Ctrl Pts',(41.7712402527273,57.561238330532,0.));
#165346=CARTESIAN_POINT('Ctrl Pts',(41.7712402527273,57.561238330532,12.));
#165347=CARTESIAN_POINT('Ctrl Pts',(41.7532885188174,57.5481434599334,0.));
#165348=CARTESIAN_POINT('Ctrl Pts',(41.7532885188174,57.5481434599334,12.));
#165349=CARTESIAN_POINT('Ctrl Pts',(41.7353878481335,57.5350579590648,0.));
#165350=CARTESIAN_POINT('Ctrl Pts',(41.7353878481335,57.5350579590648,12.));
#165351=CARTESIAN_POINT('Ctrl Pts',(41.7175383153819,57.5219819714169,0.));
#165352=CARTESIAN_POINT('Ctrl Pts',(41.7175383153819,57.5219819714169,12.));
#165353=CARTESIAN_POINT('Ctrl Pts',(41.6997399955445,57.5089156412341,0.));
#165354=CARTESIAN_POINT('Ctrl Pts',(41.6997399955445,57.5089156412341,12.));
#165355=CARTESIAN_POINT('Ctrl Pts',(41.6819929638797,57.4958591135165,0.));
#165356=CARTESIAN_POINT('Ctrl Pts',(41.6819929638797,57.4958591135165,12.));
#165357=CARTESIAN_POINT('Ctrl Pts',(41.6642972959168,57.4828125340222,0.));
#165358=CARTESIAN_POINT('Ctrl Pts',(41.6642972959168,57.4828125340222,12.));
#165359=CARTESIAN_POINT('Ctrl Pts',(41.6466530674522,57.4697760492693,0.));
#165360=CARTESIAN_POINT('Ctrl Pts',(41.6466530674522,57.4697760492693,12.));
#165361=CARTESIAN_POINT('Ctrl Pts',(41.6290603545674,57.4567498065573,0.));
#165362=CARTESIAN_POINT('Ctrl Pts',(41.6290603545674,57.4567498065573,12.));
#165363=CARTESIAN_POINT('Ctrl Pts',(41.6115192336393,57.4437339539848,0.));
#165364=CARTESIAN_POINT('Ctrl Pts',(41.6115192336393,57.4437339539848,12.));
#165365=CARTESIAN_POINT('Ctrl Pts',(41.5940297813473,57.4307286404657,0.));
#165366=CARTESIAN_POINT('Ctrl Pts',(41.5940297813473,57.4307286404657,12.));
#165367=CARTESIAN_POINT('Ctrl Pts',(41.5765920746764,57.417734015749,0.));
#165368=CARTESIAN_POINT('Ctrl Pts',(41.5765920746764,57.417734015749,12.));
#165369=CARTESIAN_POINT('Ctrl Pts',(41.5592061909159,57.4047502304207,0.));
#165370=CARTESIAN_POINT('Ctrl Pts',(41.5592061909159,57.4047502304207,12.));
#165371=CARTESIAN_POINT('Ctrl Pts',(41.5418722076558,57.3917774358844,0.));
#165372=CARTESIAN_POINT('Ctrl Pts',(41.5418722076558,57.3917774358844,12.));
#165373=CARTESIAN_POINT('Ctrl Pts',(41.5245902027767,57.378815784345,0.));
#165374=CARTESIAN_POINT('Ctrl Pts',(41.5245902027767,57.378815784345,12.));
#165375=CARTESIAN_POINT('Ctrl Pts',(41.5073602544404,57.3658654287948,0.));
#165376=CARTESIAN_POINT('Ctrl Pts',(41.5073602544404,57.3658654287948,12.));
#165377=CARTESIAN_POINT('Ctrl Pts',(41.4901824410654,57.3529265229858,0.));
#165378=CARTESIAN_POINT('Ctrl Pts',(41.4901824410654,57.3529265229858,12.));
#165379=CARTESIAN_POINT('Ctrl Pts',(41.4730568413535,57.339999221474,0.));
#165380=CARTESIAN_POINT('Ctrl Pts',(41.4730568413535,57.339999221474,12.));
#165381=CARTESIAN_POINT('Ctrl Pts',(41.4559835343338,57.3270836796925,0.));
#165382=CARTESIAN_POINT('Ctrl Pts',(41.4559835343338,57.3270836796925,12.));
#165383=CARTESIAN_POINT('Ctrl Pts',(41.4389625993948,57.3141800540137,0.));
#165384=CARTESIAN_POINT('Ctrl Pts',(41.4389625993948,57.3141800540137,12.));
#165385=CARTESIAN_POINT('Ctrl Pts',(41.4219941163154,57.3012885018139,0.));
#165386=CARTESIAN_POINT('Ctrl Pts',(41.4219941163154,57.3012885018139,12.));
#165387=CARTESIAN_POINT('Ctrl Pts',(41.4050781652923,57.2884091815385,0.));
#165388=CARTESIAN_POINT('Ctrl Pts',(41.4050781652923,57.2884091815385,12.));
#165389=CARTESIAN_POINT('Ctrl Pts',(41.3882148268798,57.2755422525822,0.));
#165390=CARTESIAN_POINT('Ctrl Pts',(41.3882148268798,57.2755422525822,12.));
#165391=CARTESIAN_POINT('Ctrl Pts',(41.3714041819215,57.2626878751584,0.));
#165392=CARTESIAN_POINT('Ctrl Pts',(41.3714041819215,57.2626878751584,12.));
#165393=CARTESIAN_POINT('Ctrl Pts',(41.3546463114889,57.2498462101883,0.));
#165394=CARTESIAN_POINT('Ctrl Pts',(41.3546463114889,57.2498462101883,12.));
#165395=CARTESIAN_POINT('Ctrl Pts',(41.3379412967889,57.237017419142,0.));
#165396=CARTESIAN_POINT('Ctrl Pts',(41.3379412967889,57.237017419142,12.));
#165397=CARTESIAN_POINT('Ctrl Pts',(41.321289219151,57.2242016640226,0.));
#165398=CARTESIAN_POINT('Ctrl Pts',(41.321289219151,57.2242016640226,12.));
#165399=CARTESIAN_POINT('Ctrl Pts',(41.304690160231,57.2113991077325,0.));
#165400=CARTESIAN_POINT('Ctrl Pts',(41.304690160231,57.2113991077325,12.));
#165401=CARTESIAN_POINT('Ctrl Pts',(41.2881442021869,57.1986099143992,0.));
#165402=CARTESIAN_POINT('Ctrl Pts',(41.2881442021869,57.1986099143992,12.));
#165403=CARTESIAN_POINT('Ctrl Pts',(41.2716514278268,57.1858342496526,0.));
#165404=CARTESIAN_POINT('Ctrl Pts',(41.2716514278268,57.1858342496526,12.));
#165405=CARTESIAN_POINT('Ctrl Pts',(41.2552119208445,57.1730722810771,0.));
#165406=CARTESIAN_POINT('Ctrl Pts',(41.2552119208445,57.1730722810771,12.));
#165407=CARTESIAN_POINT('Ctrl Pts',(41.2388257656534,57.1603241779043,0.));
#165408=CARTESIAN_POINT('Ctrl Pts',(41.2388257656534,57.1603241779043,12.));
#165409=CARTESIAN_POINT('Ctrl Pts',(41.2224930469412,57.1475901101795,0.));
#165410=CARTESIAN_POINT('Ctrl Pts',(41.2224930469412,57.1475901101795,12.));
#165411=CARTESIAN_POINT('Ctrl Pts',(41.2062138492913,57.1348702480644,0.));
#165412=CARTESIAN_POINT('Ctrl Pts',(41.2062138492913,57.1348702480644,12.));
#165413=CARTESIAN_POINT('Ctrl Pts',(41.1899882567941,57.1221647611232,0.));
#165414=CARTESIAN_POINT('Ctrl Pts',(41.1899882567941,57.1221647611232,12.));
#165415=CARTESIAN_POINT('Ctrl Pts',(41.1738163525931,57.1094738174998,0.));
#165416=CARTESIAN_POINT('Ctrl Pts',(41.1738163525931,57.1094738174998,12.));
#165417=CARTESIAN_POINT('Ctrl Pts',(41.1576982197402,57.0967975854912,0.));
#165418=CARTESIAN_POINT('Ctrl Pts',(41.1576982197402,57.0967975854912,12.));
#165419=CARTESIAN_POINT('Ctrl Pts',(41.1416339422132,57.0841362354281,0.));
#165420=CARTESIAN_POINT('Ctrl Pts',(41.1416339422132,57.0841362354281,12.));
#165421=CARTESIAN_POINT('Ctrl Pts',(41.1256236057436,57.0714899412091,0.));
#165422=CARTESIAN_POINT('Ctrl Pts',(41.1256236057436,57.0714899412091,12.));
#165423=CARTESIAN_POINT('Ctrl Pts',(41.1096672990125,57.0588588825266,0.));
#165424=CARTESIAN_POINT('Ctrl Pts',(41.1096672990125,57.0588588825266,12.));
#165425=CARTESIAN_POINT('Ctrl Pts',(41.0937651137519,57.0462432450637,0.));
#165426=CARTESIAN_POINT('Ctrl Pts',(41.0937651137519,57.0462432450637,12.));
#165427=CARTESIAN_POINT('Ctrl Pts',(41.0779171422415,57.0336432158504,0.));
#165428=CARTESIAN_POINT('Ctrl Pts',(41.0779171422415,57.0336432158504,12.));
#165429=CARTESIAN_POINT('Ctrl Pts',(41.0621234751,57.0210589791777,0.));
#165430=CARTESIAN_POINT('Ctrl Pts',(41.0621234751,57.0210589791777,12.));
#165431=CARTESIAN_POINT('Ctrl Pts',(41.0463841993622,57.008490713044,0.));
#165432=CARTESIAN_POINT('Ctrl Pts',(41.0463841993622,57.008490713044,12.));
#165433=CARTESIAN_POINT('Ctrl Pts',(41.0306993954021,56.9959385834768,0.));
#165434=CARTESIAN_POINT('Ctrl Pts',(41.0306993954021,56.9959385834768,12.));
#165435=CARTESIAN_POINT('Ctrl Pts',(41.0150691398988,56.9834027500178,0.));
#165436=CARTESIAN_POINT('Ctrl Pts',(41.0150691398988,56.9834027500178,12.));
#165437=CARTESIAN_POINT('Ctrl Pts',(40.9994935117307,56.9708833766184,0.));
#165438=CARTESIAN_POINT('Ctrl Pts',(40.9994935117307,56.9708833766184,12.));
#165439=CARTESIAN_POINT('Ctrl Pts',(40.9839725967121,56.9583806404069,0.));
#165440=CARTESIAN_POINT('Ctrl Pts',(40.9839725967121,56.9583806404069,12.));
#165441=CARTESIAN_POINT('Ctrl Pts',(40.968506493303,56.9458947422541,0.));
#165442=CARTESIAN_POINT('Ctrl Pts',(40.968506493303,56.9458947422541,12.));
#165443=CARTESIAN_POINT('Ctrl Pts',(40.9530953164952,56.9334259139928,0.));
#165444=CARTESIAN_POINT('Ctrl Pts',(40.9530953164952,56.9334259139928,12.));
#165445=CARTESIAN_POINT('Ctrl Pts',(40.9377391857043,56.9209743960861,0.));
#165446=CARTESIAN_POINT('Ctrl Pts',(40.9377391857043,56.9209743960861,12.));
#165447=CARTESIAN_POINT('Ctrl Pts',(40.9224382132382,56.9085404164432,0.));
#165448=CARTESIAN_POINT('Ctrl Pts',(40.9224382132382,56.9085404164432,12.));
#165449=CARTESIAN_POINT('Ctrl Pts',(40.907192493755,56.8961241708926,0.));
#165450=CARTESIAN_POINT('Ctrl Pts',(40.907192493755,56.8961241708926,12.));
#165451=CARTESIAN_POINT('Ctrl Pts',(40.8920020903443,56.8837257978574,0.));
#165452=CARTESIAN_POINT('Ctrl Pts',(40.8920020903443,56.8837257978574,12.));
#165453=CARTESIAN_POINT('Ctrl Pts',(40.8768670342278,56.8713453765253,0.));
#165454=CARTESIAN_POINT('Ctrl Pts',(40.8768670342278,56.8713453765253,12.));
#165455=CARTESIAN_POINT('Ctrl Pts',(40.8648032759631,56.8614554317993,0.));
#165456=CARTESIAN_POINT('Ctrl Pts',(40.8648032759631,56.8614554317993,12.));
#165457=CARTESIAN_POINT('Ctrl Pts',(40.8557803680411,56.8540460739677,0.));
#165458=CARTESIAN_POINT('Ctrl Pts',(40.8557803680411,56.8540460739677,12.));
#165459=CARTESIAN_POINT('Ctrl Pts',(40.8497761671086,56.8491101022668,0.));
#165460=CARTESIAN_POINT('Ctrl Pts',(40.8497761671086,56.8491101022668,12.));
#165461=CARTESIAN_POINT('Ctrl Pts',(40.8467768343956,56.8466430164621,0.));
#165462=CARTESIAN_POINT('Ctrl Pts',(40.8467768343956,56.8466430164621,12.));
#165463=CARTESIAN_POINT('',(40.8467768343956,56.8466430164621,12.));
#165464=CARTESIAN_POINT('Ctrl Pts',(40.8467768343956,56.8466430164621,12.));
#165465=CARTESIAN_POINT('Ctrl Pts',(40.8497761671086,56.8491101022668,12.));
#165466=CARTESIAN_POINT('Ctrl Pts',(40.8557803680411,56.8540460739677,12.));
#165467=CARTESIAN_POINT('Ctrl Pts',(40.8648032759631,56.8614554317993,12.));
#165468=CARTESIAN_POINT('Ctrl Pts',(40.8768670342278,56.8713453765253,12.));
#165469=CARTESIAN_POINT('Ctrl Pts',(40.8920020903443,56.8837257978574,12.));
#165470=CARTESIAN_POINT('Ctrl Pts',(40.907192493755,56.8961241708926,12.));
#165471=CARTESIAN_POINT('Ctrl Pts',(40.9224382132382,56.9085404164432,12.));
#165472=CARTESIAN_POINT('Ctrl Pts',(40.9377391857043,56.9209743960861,12.));
#165473=CARTESIAN_POINT('Ctrl Pts',(40.9530953164952,56.9334259139928,12.));
#165474=CARTESIAN_POINT('Ctrl Pts',(40.968506493303,56.9458947422541,12.));
#165475=CARTESIAN_POINT('Ctrl Pts',(40.9839725967121,56.9583806404069,12.));
#165476=CARTESIAN_POINT('Ctrl Pts',(40.9994935117307,56.9708833766184,12.));
#165477=CARTESIAN_POINT('Ctrl Pts',(41.0150691398988,56.9834027500178,12.));
#165478=CARTESIAN_POINT('Ctrl Pts',(41.0306993954021,56.9959385834768,12.));
#165479=CARTESIAN_POINT('Ctrl Pts',(41.0463841993622,57.008490713044,12.));
#165480=CARTESIAN_POINT('Ctrl Pts',(41.0621234751,57.0210589791777,12.));
#165481=CARTESIAN_POINT('Ctrl Pts',(41.0779171422415,57.0336432158504,12.));
#165482=CARTESIAN_POINT('Ctrl Pts',(41.0937651137519,57.0462432450637,12.));
#165483=CARTESIAN_POINT('Ctrl Pts',(41.1096672990125,57.0588588825266,12.));
#165484=CARTESIAN_POINT('Ctrl Pts',(41.1256236057436,57.0714899412091,12.));
#165485=CARTESIAN_POINT('Ctrl Pts',(41.1416339422132,57.0841362354281,12.));
#165486=CARTESIAN_POINT('Ctrl Pts',(41.1576982197402,57.0967975854912,12.));
#165487=CARTESIAN_POINT('Ctrl Pts',(41.1738163525931,57.1094738174998,12.));
#165488=CARTESIAN_POINT('Ctrl Pts',(41.1899882567941,57.1221647611232,12.));
#165489=CARTESIAN_POINT('Ctrl Pts',(41.2062138492913,57.1348702480644,12.));
#165490=CARTESIAN_POINT('Ctrl Pts',(41.2224930469412,57.1475901101795,12.));
#165491=CARTESIAN_POINT('Ctrl Pts',(41.2388257656534,57.1603241779043,12.));
#165492=CARTESIAN_POINT('Ctrl Pts',(41.2552119208445,57.1730722810771,12.));
#165493=CARTESIAN_POINT('Ctrl Pts',(41.2716514278268,57.1858342496526,12.));
#165494=CARTESIAN_POINT('Ctrl Pts',(41.2881442021869,57.1986099143992,12.));
#165495=CARTESIAN_POINT('Ctrl Pts',(41.304690160231,57.2113991077325,12.));
#165496=CARTESIAN_POINT('Ctrl Pts',(41.321289219151,57.2242016640226,12.));
#165497=CARTESIAN_POINT('Ctrl Pts',(41.3379412967889,57.237017419142,12.));
#165498=CARTESIAN_POINT('Ctrl Pts',(41.3546463114889,57.2498462101883,12.));
#165499=CARTESIAN_POINT('Ctrl Pts',(41.3714041819215,57.2626878751584,12.));
#165500=CARTESIAN_POINT('Ctrl Pts',(41.3882148268798,57.2755422525822,12.));
#165501=CARTESIAN_POINT('Ctrl Pts',(41.4050781652923,57.2884091815385,12.));
#165502=CARTESIAN_POINT('Ctrl Pts',(41.4219941163154,57.3012885018139,12.));
#165503=CARTESIAN_POINT('Ctrl Pts',(41.4389625993948,57.3141800540137,12.));
#165504=CARTESIAN_POINT('Ctrl Pts',(41.4559835343338,57.3270836796925,12.));
#165505=CARTESIAN_POINT('Ctrl Pts',(41.4730568413535,57.339999221474,12.));
#165506=CARTESIAN_POINT('Ctrl Pts',(41.4901824410654,57.3529265229858,12.));
#165507=CARTESIAN_POINT('Ctrl Pts',(41.5073602544404,57.3658654287948,12.));
#165508=CARTESIAN_POINT('Ctrl Pts',(41.5245902027767,57.378815784345,12.));
#165509=CARTESIAN_POINT('Ctrl Pts',(41.5418722076558,57.3917774358844,12.));
#165510=CARTESIAN_POINT('Ctrl Pts',(41.5592061909159,57.4047502304207,12.));
#165511=CARTESIAN_POINT('Ctrl Pts',(41.5765920746764,57.417734015749,12.));
#165512=CARTESIAN_POINT('Ctrl Pts',(41.5940297813473,57.4307286404657,12.));
#165513=CARTESIAN_POINT('Ctrl Pts',(41.6115192336393,57.4437339539848,12.));
#165514=CARTESIAN_POINT('Ctrl Pts',(41.6290603545674,57.4567498065573,12.));
#165515=CARTESIAN_POINT('Ctrl Pts',(41.6466530674522,57.4697760492693,12.));
#165516=CARTESIAN_POINT('Ctrl Pts',(41.6642972959168,57.4828125340222,12.));
#165517=CARTESIAN_POINT('Ctrl Pts',(41.6819929638797,57.4958591135165,12.));
#165518=CARTESIAN_POINT('Ctrl Pts',(41.6997399955445,57.5089156412341,12.));
#165519=CARTESIAN_POINT('Ctrl Pts',(41.7175383153819,57.5219819714169,12.));
#165520=CARTESIAN_POINT('Ctrl Pts',(41.7353878481335,57.5350579590648,12.));
#165521=CARTESIAN_POINT('Ctrl Pts',(41.7532885188174,57.5481434599334,12.));
#165522=CARTESIAN_POINT('Ctrl Pts',(41.7712402527273,57.561238330532,12.));
#165523=CARTESIAN_POINT('Ctrl Pts',(41.7892429754298,57.5743424281204,12.));
#165524=CARTESIAN_POINT('Ctrl Pts',(41.8072966127559,57.5874556107054,12.));
#165525=CARTESIAN_POINT('Ctrl Pts',(41.8254010908051,57.6005777370347,12.));
#165526=CARTESIAN_POINT('Ctrl Pts',(41.8435563359456,57.613708666588,12.));
#165527=CARTESIAN_POINT('Ctrl Pts',(41.8617622748107,57.6268482595701,12.));
#165528=CARTESIAN_POINT('Ctrl Pts',(41.8800188342912,57.6399963769009,12.));
#165529=CARTESIAN_POINT('Ctrl Pts',(41.8983259415253,57.6531528802072,12.));
#165530=CARTESIAN_POINT('Ctrl Pts',(41.9166835239054,57.6663176318189,12.));
#165531=CARTESIAN_POINT('Ctrl Pts',(41.9350915090796,57.6794904947649,12.));
#165532=CARTESIAN_POINT('Ctrl Pts',(41.9535498249488,57.6926713327672,12.));
#165533=CARTESIAN_POINT('Ctrl Pts',(41.9720583996592,57.7058600102351,12.));
#165534=CARTESIAN_POINT('Ctrl Pts',(41.990617161596,57.7190563922593,12.));
#165535=CARTESIAN_POINT('Ctrl Pts',(42.0092260393897,57.7322603446066,12.));
#165536=CARTESIAN_POINT('Ctrl Pts',(42.0278849619148,57.745471733714,12.));
#165537=CARTESIAN_POINT('Ctrl Pts',(42.0465938582882,57.7586904266834,12.));
#165538=CARTESIAN_POINT('Ctrl Pts',(42.0653526578588,57.7719162912744,12.));
#165539=CARTESIAN_POINT('Ctrl Pts',(42.0841612902042,57.7851491958987,12.));
#165540=CARTESIAN_POINT('Ctrl Pts',(42.1030196851366,57.798389009616,12.));
#165541=CARTESIAN_POINT('Ctrl Pts',(42.121927772702,57.8116356021288,12.));
#165542=CARTESIAN_POINT('Ctrl Pts',(42.1408854831783,57.8248888437775,12.));
#165543=CARTESIAN_POINT('Ctrl Pts',(42.1598927470646,57.8381486055342,12.));
#165544=CARTESIAN_POINT('Ctrl Pts',(42.1789494950794,57.8514147589972,12.));
#165545=CARTESIAN_POINT('Ctrl Pts',(42.1980556581665,57.864687176387,12.));
#165546=CARTESIAN_POINT('Ctrl Pts',(42.2172111674938,57.8779657305413,12.));
#165547=CARTESIAN_POINT('Ctrl Pts',(42.2364159544501,57.8912502949096,12.));
#165548=CARTESIAN_POINT('Ctrl Pts',(42.2556699506353,57.9045407435474,12.));
#165549=CARTESIAN_POINT('Ctrl Pts',(42.2749730878594,57.9178369511114,12.));
#165550=CARTESIAN_POINT('Ctrl Pts',(42.2943252981489,57.9311387928563,12.));
#165551=CARTESIAN_POINT('Ctrl Pts',(42.3137265137452,57.9444461446299,12.));
#165552=CARTESIAN_POINT('Ctrl Pts',(42.333176667102,57.9577588828683,12.));
#165553=CARTESIAN_POINT('Ctrl Pts',(42.3526756908746,57.9710768845899,12.));
#165554=CARTESIAN_POINT('Ctrl Pts',(42.3722235179197,57.9844000273911,12.));
#165555=CARTESIAN_POINT('Ctrl Pts',(42.3918200813014,57.9977281894422,12.));
#165556=CARTESIAN_POINT('Ctrl Pts',(42.411465314289,58.0110612494828,12.));
#165557=CARTESIAN_POINT('Ctrl Pts',(42.4311591503555,58.0243990868181,12.));
#165558=CARTESIAN_POINT('Ctrl Pts',(42.4509015231674,58.037741581314,12.));
#165559=CARTESIAN_POINT('Ctrl Pts',(42.4706923665845,58.0510886133926,12.));
#165560=CARTESIAN_POINT('Ctrl Pts',(42.4905316146653,58.0644400640275,12.));
#165561=CARTESIAN_POINT('Ctrl Pts',(42.5104192016664,58.0777958147403,12.));
#165562=CARTESIAN_POINT('Ctrl Pts',(42.5303550620387,58.0911557475965,12.));
#165563=CARTESIAN_POINT('Ctrl Pts',(42.5503391304183,58.1045197452003,12.));
#165564=CARTESIAN_POINT('Ctrl Pts',(42.5703713416265,58.1178876906907,12.));
#165565=CARTESIAN_POINT('Ctrl Pts',(42.5904516306762,58.1312594677386,12.));
#165566=CARTESIAN_POINT('Ctrl Pts',(42.6105799327699,58.1446349605421,12.));
#165567=CARTESIAN_POINT('Ctrl Pts',(42.6307561832976,58.1580140538228,12.));
#165568=CARTESIAN_POINT('Ctrl Pts',(42.6509803178265,58.171396632821,12.));
#165569=CARTESIAN_POINT('Ctrl Pts',(42.6712522721016,58.1847825832923,12.));
#165570=CARTESIAN_POINT('Ctrl Pts',(42.6915719820513,58.1981717915037,12.));
#165571=CARTESIAN_POINT('Ctrl Pts',(42.7119393837866,58.21156414423,12.));
#165572=CARTESIAN_POINT('Ctrl Pts',(42.7323544135985,58.22495952875,12.));
#165573=CARTESIAN_POINT('Ctrl Pts',(42.7528170079484,58.2383578328424,12.));
#165574=CARTESIAN_POINT('Ctrl Pts',(42.7733271034679,58.2517589447821,12.));
#165575=CARTESIAN_POINT('Ctrl Pts',(42.7938846369651,58.2651627533368,12.));
#165576=CARTESIAN_POINT('Ctrl Pts',(42.8144895454233,58.2785691477638,12.));
#165577=CARTESIAN_POINT('Ctrl Pts',(42.8351417659999,58.2919780178064,12.));
#165578=CARTESIAN_POINT('Ctrl Pts',(42.8558412360158,58.3053892536894,12.));
#165579=CARTESIAN_POINT('Ctrl Pts',(42.8765878929551,58.3188027461164,12.));
#165580=CARTESIAN_POINT('Ctrl Pts',(42.8973816744709,58.3322183862654,12.));
#165581=CARTESIAN_POINT('Ctrl Pts',(42.9182225183854,58.3456360657865,12.));
#165582=CARTESIAN_POINT('Ctrl Pts',(42.9391103626879,58.3590556767978,12.));
#165583=CARTESIAN_POINT('Ctrl Pts',(42.960045145526,58.3724771118826,12.));
#165584=CARTESIAN_POINT('Ctrl Pts',(42.9810268052032,58.3859002640857,12.));
#165585=CARTESIAN_POINT('Ctrl Pts',(43.0020552801859,58.3993250269101,12.));
#165586=CARTESIAN_POINT('Ctrl Pts',(43.0231305091027,58.4127512943136,12.));
#165587=CARTESIAN_POINT('Ctrl Pts',(43.0442524307434,58.4261789607058,12.));
#165588=CARTESIAN_POINT('Ctrl Pts',(43.0654209840511,58.4396079209451,12.));
#165589=CARTESIAN_POINT('Ctrl Pts',(43.0866361081177,58.4530380703349,12.));
#165590=CARTESIAN_POINT('Ctrl Pts',(43.1078977421916,58.4664693046217,12.));
#165591=CARTESIAN_POINT('Ctrl Pts',(43.1292058256776,58.4799015199907,12.));
#165592=CARTESIAN_POINT('Ctrl Pts',(43.1505602981365,58.4933346130636,12.));
#165593=CARTESIAN_POINT('Ctrl Pts',(43.1719610992771,58.5067684808944,12.));
#165594=CARTESIAN_POINT('Ctrl Pts',(43.1934081689505,58.5202030209669,12.));
#165595=CARTESIAN_POINT('Ctrl Pts',(43.2149014471574,58.5336381311917,12.));
#165596=CARTESIAN_POINT('Ctrl Pts',(43.2364408740493,58.5470737099032,12.));
#165597=CARTESIAN_POINT('Ctrl Pts',(43.2580263899278,58.5605096558578,12.));
#165598=CARTESIAN_POINT('Ctrl Pts',(43.27965793524,58.573945868231,12.));
#165599=CARTESIAN_POINT('Ctrl Pts',(43.3013354505701,58.5873822466152,12.));
#165600=CARTESIAN_POINT('Ctrl Pts',(43.3230588766449,58.6008186910156,12.));
#165601=CARTESIAN_POINT('Ctrl Pts',(43.3448281543371,58.6142551018467,12.));
#165602=CARTESIAN_POINT('Ctrl Pts',(43.3666432246635,58.627691379929,12.));
#165603=CARTESIAN_POINT('Ctrl Pts',(43.388504028781,58.6411274264857,12.));
#165604=CARTESIAN_POINT('Ctrl Pts',(43.4104105079768,58.6545631431393,12.));
#165605=CARTESIAN_POINT('Ctrl Pts',(43.4323626036736,58.6679984319097,12.));
#165606=CARTESIAN_POINT('Ctrl Pts',(43.4543602574351,58.6814331952138,12.));
#165607=CARTESIAN_POINT('Ctrl Pts',(43.4764034109654,58.6948673358638,12.));
#165608=CARTESIAN_POINT('Ctrl Pts',(43.4984920061073,58.7083007570661,12.));
#165609=CARTESIAN_POINT('Ctrl Pts',(43.5206259848337,58.7217333624209,12.));
#165610=CARTESIAN_POINT('Ctrl Pts',(43.5428052892488,58.7351650559181,12.));
#165611=CARTESIAN_POINT('Ctrl Pts',(43.5650298615916,58.74859574193,12.));
#165612=CARTESIAN_POINT('Ctrl Pts',(43.5872996442345,58.7620253252062,12.));
#165613=CARTESIAN_POINT('Ctrl Pts',(43.6096145796796,58.775453710867,12.));
#165614=CARTESIAN_POINT('Ctrl Pts',(43.6319746105482,58.788880804397,12.));
#165615=CARTESIAN_POINT('Ctrl Pts',(43.6543796795789,58.8023065116436,12.));
#165616=CARTESIAN_POINT('Ctrl Pts',(43.6768297296395,58.8157307388238,12.));
#165617=CARTESIAN_POINT('Ctrl Pts',(43.6993247037314,58.8291533925293,12.));
#165618=CARTESIAN_POINT('Ctrl Pts',(43.7218645449922,58.8425743797326,12.));
#165619=CARTESIAN_POINT('Ctrl Pts',(43.7444491966942,58.8559936077941,12.));
#165620=CARTESIAN_POINT('Ctrl Pts',(43.7670786022402,58.8694109844648,12.));
#165621=CARTESIAN_POINT('Ctrl Pts',(43.7897527051609,58.8828264178621,12.));
#165622=CARTESIAN_POINT('Ctrl Pts',(43.8124714491076,58.8962398164493,12.));
#165623=CARTESIAN_POINT('Ctrl Pts',(43.835234777842,58.9096510890129,12.));
#165624=CARTESIAN_POINT('Ctrl Pts',(43.858042635223,58.9230601446436,12.));
#165625=CARTESIAN_POINT('Ctrl Pts',(43.8808949651872,58.936466892712,12.));
#165626=CARTESIAN_POINT('Ctrl Pts',(43.9037917117739,58.9498712429054,12.));
#165627=CARTESIAN_POINT('Ctrl Pts',(43.9267328191501,58.9632731052696,12.));
#165628=CARTESIAN_POINT('Ctrl Pts',(43.9497182316331,58.9766723902529,12.));
#165629=CARTESIAN_POINT('Ctrl Pts',(43.9727478937056,58.9900690087408,12.));
#165630=CARTESIAN_POINT('Ctrl Pts',(43.9958217500369,59.0034628721168,12.));
#165631=CARTESIAN_POINT('Ctrl Pts',(44.0189397454599,59.0168538922095,12.));
#165632=CARTESIAN_POINT('Ctrl Pts',(44.0421018249223,59.0302419811777,12.));
#165633=CARTESIAN_POINT('Ctrl Pts',(44.0653079334385,59.0436270514087,12.));
#165634=CARTESIAN_POINT('Ctrl Pts',(44.0885580160432,59.0570090154242,12.));
#165635=CARTESIAN_POINT('Ctrl Pts',(44.1118520177221,59.0703877857526,12.));
#165636=CARTESIAN_POINT('Ctrl Pts',(44.1351898834051,59.08376327492,12.));
#165637=CARTESIAN_POINT('Ctrl Pts',(44.1585715581064,59.0971353957206,12.));
#165638=CARTESIAN_POINT('Ctrl Pts',(44.1819969870307,59.1105040614276,12.));
#165639=CARTESIAN_POINT('Ctrl Pts',(44.2054661156875,59.1238691860306,12.));
#165640=CARTESIAN_POINT('Ctrl Pts',(44.228978889997,59.1372306844586,12.));
#165641=CARTESIAN_POINT('Ctrl Pts',(44.2525352563996,59.1505884728215,12.));
#165642=CARTESIAN_POINT('Ctrl Pts',(44.2761351616048,59.1639424678793,12.));
#165643=CARTESIAN_POINT('Ctrl Pts',(44.2997785523431,59.1772925865213,12.));
#165644=CARTESIAN_POINT('Ctrl Pts',(44.3234653750884,59.1906387451979,12.));
#165645=CARTESIAN_POINT('Ctrl Pts',(44.3471955758402,59.2039808594752,12.));
#165646=CARTESIAN_POINT('Ctrl Pts',(44.3709690997469,59.2173188432798,12.));
#165647=CARTESIAN_POINT('Ctrl Pts',(44.3947858914074,59.2306526095131,12.));
#165648=CARTESIAN_POINT('Ctrl Pts',(44.418645895545,59.2439820714187,12.));
#165649=CARTESIAN_POINT('Ctrl Pts',(44.4425490575911,59.2573071437774,12.));
#165650=CARTESIAN_POINT('Ctrl Pts',(44.4664953242378,59.2706277440445,12.));
#165651=CARTESIAN_POINT('Ctrl Pts',(44.490484644151,59.2839437938237,12.));
#165652=CARTESIAN_POINT('Ctrl Pts',(44.5145169681349,59.2972552192156,12.));
#165653=CARTESIAN_POINT('Ctrl Pts',(44.535154147848,59.3086616639524,12.));
#165654=CARTESIAN_POINT('Ctrl Pts',(44.5509994358156,59.3174041872348,12.));
#165655=CARTESIAN_POINT('Ctrl Pts',(44.5620338188741,59.3234848865457,12.));
#165656=CARTESIAN_POINT('Ctrl Pts',(44.5682447396025,59.3269051738425,12.));
#165657=CARTESIAN_POINT('Ctrl Pts',(44.5696260757798,59.3276657444395,12.));
#165658=CARTESIAN_POINT('',(40.8467768343956,56.8466430164621,0.));
#165659=CARTESIAN_POINT('',(40.8467768343956,56.8466430164621,0.));
#165660=CARTESIAN_POINT('Ctrl Pts',(44.5696260757798,59.3276657444395,0.));
#165661=CARTESIAN_POINT('Ctrl Pts',(44.5682447396025,59.3269051738425,0.));
#165662=CARTESIAN_POINT('Ctrl Pts',(44.5620338188741,59.3234848865457,0.));
#165663=CARTESIAN_POINT('Ctrl Pts',(44.5509994358156,59.3174041872348,0.));
#165664=CARTESIAN_POINT('Ctrl Pts',(44.535154147848,59.3086616639524,0.));
#165665=CARTESIAN_POINT('Ctrl Pts',(44.5145169681349,59.2972552192156,0.));
#165666=CARTESIAN_POINT('Ctrl Pts',(44.490484644151,59.2839437938237,0.));
#165667=CARTESIAN_POINT('Ctrl Pts',(44.4664953242378,59.2706277440445,0.));
#165668=CARTESIAN_POINT('Ctrl Pts',(44.4425490575911,59.2573071437774,0.));
#165669=CARTESIAN_POINT('Ctrl Pts',(44.418645895545,59.2439820714187,0.));
#165670=CARTESIAN_POINT('Ctrl Pts',(44.3947858914074,59.2306526095131,0.));
#165671=CARTESIAN_POINT('Ctrl Pts',(44.3709690997469,59.2173188432798,0.));
#165672=CARTESIAN_POINT('Ctrl Pts',(44.3471955758402,59.2039808594752,0.));
#165673=CARTESIAN_POINT('Ctrl Pts',(44.3234653750884,59.1906387451979,0.));
#165674=CARTESIAN_POINT('Ctrl Pts',(44.2997785523431,59.1772925865213,0.));
#165675=CARTESIAN_POINT('Ctrl Pts',(44.2761351616048,59.1639424678793,0.));
#165676=CARTESIAN_POINT('Ctrl Pts',(44.2525352563996,59.1505884728215,0.));
#165677=CARTESIAN_POINT('Ctrl Pts',(44.228978889997,59.1372306844586,0.));
#165678=CARTESIAN_POINT('Ctrl Pts',(44.2054661156875,59.1238691860306,0.));
#165679=CARTESIAN_POINT('Ctrl Pts',(44.1819969870307,59.1105040614276,0.));
#165680=CARTESIAN_POINT('Ctrl Pts',(44.1585715581064,59.0971353957206,0.));
#165681=CARTESIAN_POINT('Ctrl Pts',(44.1351898834051,59.08376327492,0.));
#165682=CARTESIAN_POINT('Ctrl Pts',(44.1118520177221,59.0703877857526,0.));
#165683=CARTESIAN_POINT('Ctrl Pts',(44.0885580160432,59.0570090154242,0.));
#165684=CARTESIAN_POINT('Ctrl Pts',(44.0653079334385,59.0436270514087,0.));
#165685=CARTESIAN_POINT('Ctrl Pts',(44.0421018249223,59.0302419811777,0.));
#165686=CARTESIAN_POINT('Ctrl Pts',(44.0189397454599,59.0168538922095,0.));
#165687=CARTESIAN_POINT('Ctrl Pts',(43.9958217500369,59.0034628721168,0.));
#165688=CARTESIAN_POINT('Ctrl Pts',(43.9727478937056,58.9900690087408,0.));
#165689=CARTESIAN_POINT('Ctrl Pts',(43.9497182316331,58.9766723902529,0.));
#165690=CARTESIAN_POINT('Ctrl Pts',(43.9267328191501,58.9632731052696,0.));
#165691=CARTESIAN_POINT('Ctrl Pts',(43.9037917117739,58.9498712429054,0.));
#165692=CARTESIAN_POINT('Ctrl Pts',(43.8808949651872,58.936466892712,0.));
#165693=CARTESIAN_POINT('Ctrl Pts',(43.858042635223,58.9230601446436,0.));
#165694=CARTESIAN_POINT('Ctrl Pts',(43.835234777842,58.9096510890129,0.));
#165695=CARTESIAN_POINT('Ctrl Pts',(43.8124714491076,58.8962398164493,0.));
#165696=CARTESIAN_POINT('Ctrl Pts',(43.7897527051609,58.8828264178621,0.));
#165697=CARTESIAN_POINT('Ctrl Pts',(43.7670786022402,58.8694109844648,0.));
#165698=CARTESIAN_POINT('Ctrl Pts',(43.7444491966942,58.8559936077941,0.));
#165699=CARTESIAN_POINT('Ctrl Pts',(43.7218645449922,58.8425743797326,0.));
#165700=CARTESIAN_POINT('Ctrl Pts',(43.6993247037314,58.8291533925293,0.));
#165701=CARTESIAN_POINT('Ctrl Pts',(43.6768297296395,58.8157307388238,0.));
#165702=CARTESIAN_POINT('Ctrl Pts',(43.6543796795789,58.8023065116436,0.));
#165703=CARTESIAN_POINT('Ctrl Pts',(43.6319746105482,58.788880804397,0.));
#165704=CARTESIAN_POINT('Ctrl Pts',(43.6096145796796,58.775453710867,0.));
#165705=CARTESIAN_POINT('Ctrl Pts',(43.5872996442345,58.7620253252062,0.));
#165706=CARTESIAN_POINT('Ctrl Pts',(43.5650298615916,58.74859574193,0.));
#165707=CARTESIAN_POINT('Ctrl Pts',(43.5428052892488,58.7351650559181,0.));
#165708=CARTESIAN_POINT('Ctrl Pts',(43.5206259848337,58.7217333624209,0.));
#165709=CARTESIAN_POINT('Ctrl Pts',(43.4984920061073,58.7083007570661,0.));
#165710=CARTESIAN_POINT('Ctrl Pts',(43.4764034109654,58.6948673358638,0.));
#165711=CARTESIAN_POINT('Ctrl Pts',(43.4543602574351,58.6814331952138,0.));
#165712=CARTESIAN_POINT('Ctrl Pts',(43.4323626036736,58.6679984319097,0.));
#165713=CARTESIAN_POINT('Ctrl Pts',(43.4104105079768,58.6545631431393,0.));
#165714=CARTESIAN_POINT('Ctrl Pts',(43.388504028781,58.6411274264857,0.));
#165715=CARTESIAN_POINT('Ctrl Pts',(43.3666432246635,58.627691379929,0.));
#165716=CARTESIAN_POINT('Ctrl Pts',(43.3448281543371,58.6142551018467,0.));
#165717=CARTESIAN_POINT('Ctrl Pts',(43.3230588766449,58.6008186910156,0.));
#165718=CARTESIAN_POINT('Ctrl Pts',(43.3013354505701,58.5873822466152,0.));
#165719=CARTESIAN_POINT('Ctrl Pts',(43.27965793524,58.573945868231,0.));
#165720=CARTESIAN_POINT('Ctrl Pts',(43.2580263899278,58.5605096558578,0.));
#165721=CARTESIAN_POINT('Ctrl Pts',(43.2364408740493,58.5470737099032,0.));
#165722=CARTESIAN_POINT('Ctrl Pts',(43.2149014471574,58.5336381311917,0.));
#165723=CARTESIAN_POINT('Ctrl Pts',(43.1934081689505,58.5202030209669,0.));
#165724=CARTESIAN_POINT('Ctrl Pts',(43.1719610992771,58.5067684808944,0.));
#165725=CARTESIAN_POINT('Ctrl Pts',(43.1505602981365,58.4933346130636,0.));
#165726=CARTESIAN_POINT('Ctrl Pts',(43.1292058256776,58.4799015199907,0.));
#165727=CARTESIAN_POINT('Ctrl Pts',(43.1078977421916,58.4664693046217,0.));
#165728=CARTESIAN_POINT('Ctrl Pts',(43.0866361081177,58.4530380703349,0.));
#165729=CARTESIAN_POINT('Ctrl Pts',(43.0654209840511,58.4396079209451,0.));
#165730=CARTESIAN_POINT('Ctrl Pts',(43.0442524307434,58.4261789607058,0.));
#165731=CARTESIAN_POINT('Ctrl Pts',(43.0231305091027,58.4127512943136,0.));
#165732=CARTESIAN_POINT('Ctrl Pts',(43.0020552801859,58.3993250269101,0.));
#165733=CARTESIAN_POINT('Ctrl Pts',(42.9810268052032,58.3859002640857,0.));
#165734=CARTESIAN_POINT('Ctrl Pts',(42.960045145526,58.3724771118826,0.));
#165735=CARTESIAN_POINT('Ctrl Pts',(42.9391103626879,58.3590556767978,0.));
#165736=CARTESIAN_POINT('Ctrl Pts',(42.9182225183854,58.3456360657865,0.));
#165737=CARTESIAN_POINT('Ctrl Pts',(42.8973816744709,58.3322183862654,0.));
#165738=CARTESIAN_POINT('Ctrl Pts',(42.8765878929551,58.3188027461164,0.));
#165739=CARTESIAN_POINT('Ctrl Pts',(42.8558412360158,58.3053892536894,0.));
#165740=CARTESIAN_POINT('Ctrl Pts',(42.8351417659999,58.2919780178064,0.));
#165741=CARTESIAN_POINT('Ctrl Pts',(42.8144895454233,58.2785691477638,0.));
#165742=CARTESIAN_POINT('Ctrl Pts',(42.7938846369651,58.2651627533368,0.));
#165743=CARTESIAN_POINT('Ctrl Pts',(42.7733271034679,58.2517589447821,0.));
#165744=CARTESIAN_POINT('Ctrl Pts',(42.7528170079484,58.2383578328424,0.));
#165745=CARTESIAN_POINT('Ctrl Pts',(42.7323544135985,58.22495952875,0.));
#165746=CARTESIAN_POINT('Ctrl Pts',(42.7119393837866,58.21156414423,0.));
#165747=CARTESIAN_POINT('Ctrl Pts',(42.6915719820513,58.1981717915037,0.));
#165748=CARTESIAN_POINT('Ctrl Pts',(42.6712522721016,58.1847825832923,0.));
#165749=CARTESIAN_POINT('Ctrl Pts',(42.6509803178265,58.171396632821,0.));
#165750=CARTESIAN_POINT('Ctrl Pts',(42.6307561832976,58.1580140538228,0.));
#165751=CARTESIAN_POINT('Ctrl Pts',(42.6105799327699,58.1446349605421,0.));
#165752=CARTESIAN_POINT('Ctrl Pts',(42.5904516306762,58.1312594677386,0.));
#165753=CARTESIAN_POINT('Ctrl Pts',(42.5703713416265,58.1178876906907,0.));
#165754=CARTESIAN_POINT('Ctrl Pts',(42.5503391304183,58.1045197452003,0.));
#165755=CARTESIAN_POINT('Ctrl Pts',(42.5303550620387,58.0911557475965,0.));
#165756=CARTESIAN_POINT('Ctrl Pts',(42.5104192016664,58.0777958147403,0.));
#165757=CARTESIAN_POINT('Ctrl Pts',(42.4905316146653,58.0644400640275,0.));
#165758=CARTESIAN_POINT('Ctrl Pts',(42.4706923665845,58.0510886133926,0.));
#165759=CARTESIAN_POINT('Ctrl Pts',(42.4509015231674,58.037741581314,0.));
#165760=CARTESIAN_POINT('Ctrl Pts',(42.4311591503555,58.0243990868181,0.));
#165761=CARTESIAN_POINT('Ctrl Pts',(42.411465314289,58.0110612494828,0.));
#165762=CARTESIAN_POINT('Ctrl Pts',(42.3918200813014,57.9977281894422,0.));
#165763=CARTESIAN_POINT('Ctrl Pts',(42.3722235179197,57.9844000273911,0.));
#165764=CARTESIAN_POINT('Ctrl Pts',(42.3526756908746,57.9710768845899,0.));
#165765=CARTESIAN_POINT('Ctrl Pts',(42.333176667102,57.9577588828683,0.));
#165766=CARTESIAN_POINT('Ctrl Pts',(42.3137265137452,57.9444461446299,0.));
#165767=CARTESIAN_POINT('Ctrl Pts',(42.2943252981489,57.9311387928563,0.));
#165768=CARTESIAN_POINT('Ctrl Pts',(42.2749730878594,57.9178369511114,0.));
#165769=CARTESIAN_POINT('Ctrl Pts',(42.2556699506353,57.9045407435474,0.));
#165770=CARTESIAN_POINT('Ctrl Pts',(42.2364159544501,57.8912502949096,0.));
#165771=CARTESIAN_POINT('Ctrl Pts',(42.2172111674938,57.8779657305413,0.));
#165772=CARTESIAN_POINT('Ctrl Pts',(42.1980556581665,57.864687176387,0.));
#165773=CARTESIAN_POINT('Ctrl Pts',(42.1789494950794,57.8514147589972,0.));
#165774=CARTESIAN_POINT('Ctrl Pts',(42.1598927470646,57.8381486055342,0.));
#165775=CARTESIAN_POINT('Ctrl Pts',(42.1408854831783,57.8248888437775,0.));
#165776=CARTESIAN_POINT('Ctrl Pts',(42.121927772702,57.8116356021288,0.));
#165777=CARTESIAN_POINT('Ctrl Pts',(42.1030196851366,57.798389009616,0.));
#165778=CARTESIAN_POINT('Ctrl Pts',(42.0841612902042,57.7851491958987,0.));
#165779=CARTESIAN_POINT('Ctrl Pts',(42.0653526578588,57.7719162912744,0.));
#165780=CARTESIAN_POINT('Ctrl Pts',(42.0465938582882,57.7586904266834,0.));
#165781=CARTESIAN_POINT('Ctrl Pts',(42.0278849619148,57.745471733714,0.));
#165782=CARTESIAN_POINT('Ctrl Pts',(42.0092260393897,57.7322603446066,0.));
#165783=CARTESIAN_POINT('Ctrl Pts',(41.990617161596,57.7190563922593,0.));
#165784=CARTESIAN_POINT('Ctrl Pts',(41.9720583996592,57.7058600102351,0.));
#165785=CARTESIAN_POINT('Ctrl Pts',(41.9535498249488,57.6926713327672,0.));
#165786=CARTESIAN_POINT('Ctrl Pts',(41.9350915090796,57.6794904947649,0.));
#165787=CARTESIAN_POINT('Ctrl Pts',(41.9166835239054,57.6663176318189,0.));
#165788=CARTESIAN_POINT('Ctrl Pts',(41.8983259415253,57.6531528802072,0.));
#165789=CARTESIAN_POINT('Ctrl Pts',(41.8800188342912,57.6399963769009,0.));
#165790=CARTESIAN_POINT('Ctrl Pts',(41.8617622748107,57.6268482595701,0.));
#165791=CARTESIAN_POINT('Ctrl Pts',(41.8435563359456,57.613708666588,0.));
#165792=CARTESIAN_POINT('Ctrl Pts',(41.8254010908051,57.6005777370347,0.));
#165793=CARTESIAN_POINT('Ctrl Pts',(41.8072966127559,57.5874556107054,0.));
#165794=CARTESIAN_POINT('Ctrl Pts',(41.7892429754298,57.5743424281204,0.));
#165795=CARTESIAN_POINT('Ctrl Pts',(41.7712402527273,57.561238330532,0.));
#165796=CARTESIAN_POINT('Ctrl Pts',(41.7532885188174,57.5481434599334,0.));
#165797=CARTESIAN_POINT('Ctrl Pts',(41.7353878481335,57.5350579590648,0.));
#165798=CARTESIAN_POINT('Ctrl Pts',(41.7175383153819,57.5219819714169,0.));
#165799=CARTESIAN_POINT('Ctrl Pts',(41.6997399955445,57.5089156412341,0.));
#165800=CARTESIAN_POINT('Ctrl Pts',(41.6819929638797,57.4958591135165,0.));
#165801=CARTESIAN_POINT('Ctrl Pts',(41.6642972959168,57.4828125340222,0.));
#165802=CARTESIAN_POINT('Ctrl Pts',(41.6466530674522,57.4697760492693,0.));
#165803=CARTESIAN_POINT('Ctrl Pts',(41.6290603545674,57.4567498065573,0.));
#165804=CARTESIAN_POINT('Ctrl Pts',(41.6115192336393,57.4437339539848,0.));
#165805=CARTESIAN_POINT('Ctrl Pts',(41.5940297813473,57.4307286404657,0.));
#165806=CARTESIAN_POINT('Ctrl Pts',(41.5765920746764,57.417734015749,0.));
#165807=CARTESIAN_POINT('Ctrl Pts',(41.5592061909159,57.4047502304207,0.));
#165808=CARTESIAN_POINT('Ctrl Pts',(41.5418722076558,57.3917774358844,0.));
#165809=CARTESIAN_POINT('Ctrl Pts',(41.5245902027767,57.378815784345,0.));
#165810=CARTESIAN_POINT('Ctrl Pts',(41.5073602544404,57.3658654287948,0.));
#165811=CARTESIAN_POINT('Ctrl Pts',(41.4901824410654,57.3529265229858,0.));
#165812=CARTESIAN_POINT('Ctrl Pts',(41.4730568413535,57.339999221474,0.));
#165813=CARTESIAN_POINT('Ctrl Pts',(41.4559835343338,57.3270836796925,0.));
#165814=CARTESIAN_POINT('Ctrl Pts',(41.4389625993948,57.3141800540137,0.));
#165815=CARTESIAN_POINT('Ctrl Pts',(41.4219941163154,57.3012885018139,0.));
#165816=CARTESIAN_POINT('Ctrl Pts',(41.4050781652923,57.2884091815385,0.));
#165817=CARTESIAN_POINT('Ctrl Pts',(41.3882148268798,57.2755422525822,0.));
#165818=CARTESIAN_POINT('Ctrl Pts',(41.3714041819215,57.2626878751584,0.));
#165819=CARTESIAN_POINT('Ctrl Pts',(41.3546463114889,57.2498462101883,0.));
#165820=CARTESIAN_POINT('Ctrl Pts',(41.3379412967889,57.237017419142,0.));
#165821=CARTESIAN_POINT('Ctrl Pts',(41.321289219151,57.2242016640226,0.));
#165822=CARTESIAN_POINT('Ctrl Pts',(41.304690160231,57.2113991077325,0.));
#165823=CARTESIAN_POINT('Ctrl Pts',(41.2881442021869,57.1986099143992,0.));
#165824=CARTESIAN_POINT('Ctrl Pts',(41.2716514278268,57.1858342496526,0.));
#165825=CARTESIAN_POINT('Ctrl Pts',(41.2552119208445,57.1730722810771,0.));
#165826=CARTESIAN_POINT('Ctrl Pts',(41.2388257656534,57.1603241779043,0.));
#165827=CARTESIAN_POINT('Ctrl Pts',(41.2224930469412,57.1475901101795,0.));
#165828=CARTESIAN_POINT('Ctrl Pts',(41.2062138492913,57.1348702480644,0.));
#165829=CARTESIAN_POINT('Ctrl Pts',(41.1899882567941,57.1221647611232,0.));
#165830=CARTESIAN_POINT('Ctrl Pts',(41.1738163525931,57.1094738174998,0.));
#165831=CARTESIAN_POINT('Ctrl Pts',(41.1576982197402,57.0967975854912,0.));
#165832=CARTESIAN_POINT('Ctrl Pts',(41.1416339422132,57.0841362354281,0.));
#165833=CARTESIAN_POINT('Ctrl Pts',(41.1256236057436,57.0714899412091,0.));
#165834=CARTESIAN_POINT('Ctrl Pts',(41.1096672990125,57.0588588825266,0.));
#165835=CARTESIAN_POINT('Ctrl Pts',(41.0937651137519,57.0462432450637,0.));
#165836=CARTESIAN_POINT('Ctrl Pts',(41.0779171422415,57.0336432158504,0.));
#165837=CARTESIAN_POINT('Ctrl Pts',(41.0621234751,57.0210589791777,0.));
#165838=CARTESIAN_POINT('Ctrl Pts',(41.0463841993622,57.008490713044,0.));
#165839=CARTESIAN_POINT('Ctrl Pts',(41.0306993954021,56.9959385834768,0.));
#165840=CARTESIAN_POINT('Ctrl Pts',(41.0150691398988,56.9834027500178,0.));
#165841=CARTESIAN_POINT('Ctrl Pts',(40.9994935117307,56.9708833766184,0.));
#165842=CARTESIAN_POINT('Ctrl Pts',(40.9839725967121,56.9583806404069,0.));
#165843=CARTESIAN_POINT('Ctrl Pts',(40.968506493303,56.9458947422541,0.));
#165844=CARTESIAN_POINT('Ctrl Pts',(40.9530953164952,56.9334259139928,0.));
#165845=CARTESIAN_POINT('Ctrl Pts',(40.9377391857043,56.9209743960861,0.));
#165846=CARTESIAN_POINT('Ctrl Pts',(40.9224382132382,56.9085404164432,0.));
#165847=CARTESIAN_POINT('Ctrl Pts',(40.907192493755,56.8961241708926,0.));
#165848=CARTESIAN_POINT('Ctrl Pts',(40.8920020903443,56.8837257978574,0.));
#165849=CARTESIAN_POINT('Ctrl Pts',(40.8768670342278,56.8713453765253,0.));
#165850=CARTESIAN_POINT('Ctrl Pts',(40.8648032759631,56.8614554317993,0.));
#165851=CARTESIAN_POINT('Ctrl Pts',(40.8557803680411,56.8540460739677,0.));
#165852=CARTESIAN_POINT('Ctrl Pts',(40.8497761671086,56.8491101022668,0.));
#165853=CARTESIAN_POINT('Ctrl Pts',(40.8467768343956,56.8466430164621,0.));
#165854=CARTESIAN_POINT('Ctrl Pts',(49.8690697110161,55.3473204966403,0.));
#165855=CARTESIAN_POINT('Ctrl Pts',(49.8690697110161,55.3473204966403,12.));
#165856=CARTESIAN_POINT('Ctrl Pts',(49.8639277221566,55.3451131058826,0.));
#165857=CARTESIAN_POINT('Ctrl Pts',(49.8639277221566,55.3451131058826,12.));
#165858=CARTESIAN_POINT('Ctrl Pts',(49.8536479176833,55.34069740326,0.));
#165859=CARTESIAN_POINT('Ctrl Pts',(49.8536479176833,55.34069740326,12.));
#165860=CARTESIAN_POINT('Ctrl Pts',(49.8382407307107,55.3340710860055,0.));
#165861=CARTESIAN_POINT('Ctrl Pts',(49.8382407307107,55.3340710860055,12.));
#165862=CARTESIAN_POINT('Ctrl Pts',(49.8177228552376,55.3252304694602,0.));
#165863=CARTESIAN_POINT('Ctrl Pts',(49.8177228552376,55.3252304694602,12.));
#165864=CARTESIAN_POINT('Ctrl Pts',(49.7921172540628,55.3141704897766,0.));
#165865=CARTESIAN_POINT('Ctrl Pts',(49.7921172540628,55.3141704897766,12.));
#165866=CARTESIAN_POINT('Ctrl Pts',(49.7665534128535,55.3031013105853,0.));
#165867=CARTESIAN_POINT('Ctrl Pts',(49.7665534128535,55.3031013105853,12.));
#165868=CARTESIAN_POINT('Ctrl Pts',(49.7410313576508,55.2920229527546,0.));
#165869=CARTESIAN_POINT('Ctrl Pts',(49.7410313576508,55.2920229527546,12.));
#165870=CARTESIAN_POINT('Ctrl Pts',(49.7155511248531,55.2809354521515,0.));
#165871=CARTESIAN_POINT('Ctrl Pts',(49.7155511248531,55.2809354521515,12.));
#165872=CARTESIAN_POINT('Ctrl Pts',(49.6901127631627,55.2698388650025,0.));
#165873=CARTESIAN_POINT('Ctrl Pts',(49.6901127631627,55.2698388650025,12.));
#165874=CARTESIAN_POINT('Ctrl Pts',(49.6647163322266,55.2587332663783,0.));
#165875=CARTESIAN_POINT('Ctrl Pts',(49.6647163322266,55.2587332663783,12.));
#165876=CARTESIAN_POINT('Ctrl Pts',(49.6393618987473,55.2476187434057,0.));
#165877=CARTESIAN_POINT('Ctrl Pts',(49.6393618987473,55.2476187434057,12.));
#165878=CARTESIAN_POINT('Ctrl Pts',(49.6140495332803,55.2364953899358,0.));
#165879=CARTESIAN_POINT('Ctrl Pts',(49.6140495332803,55.2364953899358,12.));
#165880=CARTESIAN_POINT('Ctrl Pts',(49.5887793068352,55.2253633007666,0.));
#165881=CARTESIAN_POINT('Ctrl Pts',(49.5887793068352,55.2253633007666,12.));
#165882=CARTESIAN_POINT('Ctrl Pts',(49.5635512873435,55.2142225657013,0.));
#165883=CARTESIAN_POINT('Ctrl Pts',(49.5635512873435,55.2142225657013,12.));
#165884=CARTESIAN_POINT('Ctrl Pts',(49.5383655368073,55.2030732647312,0.));
#165885=CARTESIAN_POINT('Ctrl Pts',(49.5383655368073,55.2030732647312,12.));
#165886=CARTESIAN_POINT('Ctrl Pts',(49.5132221132992,55.1919154713647,0.));
#165887=CARTESIAN_POINT('Ctrl Pts',(49.5132221132992,55.1919154713647,12.));
#165888=CARTESIAN_POINT('Ctrl Pts',(49.4881210723966,55.1807492550119,0.));
#165889=CARTESIAN_POINT('Ctrl Pts',(49.4881210723966,55.1807492550119,12.));
#165890=CARTESIAN_POINT('Ctrl Pts',(49.4630624688793,55.1695746838174,0.));
#165891=CARTESIAN_POINT('Ctrl Pts',(49.4630624688793,55.1695746838174,12.));
#165892=CARTESIAN_POINT('Ctrl Pts',(49.4380463581965,55.1583918271116,0.));
#165893=CARTESIAN_POINT('Ctrl Pts',(49.4380463581965,55.1583918271116,12.));
#165894=CARTESIAN_POINT('Ctrl Pts',(49.4130727983201,55.1472007585183,0.));
#165895=CARTESIAN_POINT('Ctrl Pts',(49.4130727983201,55.1472007585183,12.));
#165896=CARTESIAN_POINT('Ctrl Pts',(49.3881418495489,55.1360015556221,0.));
#165897=CARTESIAN_POINT('Ctrl Pts',(49.3881418495489,55.1360015556221,12.));
#165898=CARTESIAN_POINT('Ctrl Pts',(49.3632535736715,55.1247942985619,0.));
#165899=CARTESIAN_POINT('Ctrl Pts',(49.3632535736715,55.1247942985619,12.));
#165900=CARTESIAN_POINT('Ctrl Pts',(49.3384080333155,55.1135790689464,0.));
#165901=CARTESIAN_POINT('Ctrl Pts',(49.3384080333155,55.1135790689464,12.));
#165902=CARTESIAN_POINT('Ctrl Pts',(49.3136052912621,55.102355948714,0.));
#165903=CARTESIAN_POINT('Ctrl Pts',(49.3136052912621,55.102355948714,12.));
#165904=CARTESIAN_POINT('Ctrl Pts',(49.2888454096563,55.0911250188302,0.));
#165905=CARTESIAN_POINT('Ctrl Pts',(49.2888454096563,55.0911250188302,12.));
#165906=CARTESIAN_POINT('Ctrl Pts',(49.264128449652,55.079886358701,0.));
#165907=CARTESIAN_POINT('Ctrl Pts',(49.264128449652,55.079886358701,12.));
#165908=CARTESIAN_POINT('Ctrl Pts',(49.2394544718531,55.0686400468931,0.));
#165909=CARTESIAN_POINT('Ctrl Pts',(49.2394544718531,55.0686400468931,12.));
#165910=CARTESIAN_POINT('Ctrl Pts',(49.2148235365703,55.0573861615579,0.));
#165911=CARTESIAN_POINT('Ctrl Pts',(49.2148235365703,55.0573861615579,12.));
#165912=CARTESIAN_POINT('Ctrl Pts',(49.1902357041461,55.0461247809744,0.));
#165913=CARTESIAN_POINT('Ctrl Pts',(49.1902357041461,55.0461247809744,12.));
#165914=CARTESIAN_POINT('Ctrl Pts',(49.1656910352476,55.0348559840453,0.));
#165915=CARTESIAN_POINT('Ctrl Pts',(49.1656910352476,55.0348559840453,12.));
#165916=CARTESIAN_POINT('Ctrl Pts',(49.1411895911635,55.0235798508045,0.));
#165917=CARTESIAN_POINT('Ctrl Pts',(49.1411895911635,55.0235798508045,12.));
#165918=CARTESIAN_POINT('Ctrl Pts',(49.116731433673,55.012296462186,0.));
#165919=CARTESIAN_POINT('Ctrl Pts',(49.116731433673,55.012296462186,12.));
#165920=CARTESIAN_POINT('Ctrl Pts',(49.0923166249219,55.0010058998107,0.));
#165921=CARTESIAN_POINT('Ctrl Pts',(49.0923166249219,55.0010058998107,12.));
#165922=CARTESIAN_POINT('Ctrl Pts',(49.067945227287,54.9897082457606,0.));
#165923=CARTESIAN_POINT('Ctrl Pts',(49.067945227287,54.9897082457606,12.));
#165924=CARTESIAN_POINT('Ctrl Pts',(49.0436173032528,54.9784035823766,0.));
#165925=CARTESIAN_POINT('Ctrl Pts',(49.0436173032528,54.9784035823766,12.));
#165926=CARTESIAN_POINT('Ctrl Pts',(49.0193329152479,54.9670919920029,0.));
#165927=CARTESIAN_POINT('Ctrl Pts',(49.0193329152479,54.9670919920029,12.));
#165928=CARTESIAN_POINT('Ctrl Pts',(48.9950921256526,54.9557735569943,0.));
#165929=CARTESIAN_POINT('Ctrl Pts',(48.9950921256526,54.9557735569943,12.));
#165930=CARTESIAN_POINT('Ctrl Pts',(48.9708949968795,54.9444483598378,0.));
#165931=CARTESIAN_POINT('Ctrl Pts',(48.9708949968795,54.9444483598378,12.));
#165932=CARTESIAN_POINT('Ctrl Pts',(48.9467415914269,54.9331164832424,0.));
#165933=CARTESIAN_POINT('Ctrl Pts',(48.9467415914269,54.9331164832424,12.));
#165934=CARTESIAN_POINT('Ctrl Pts',(48.9226319719368,54.9217780102355,0.));
#165935=CARTESIAN_POINT('Ctrl Pts',(48.9226319719368,54.9217780102355,12.));
#165936=CARTESIAN_POINT('Ctrl Pts',(48.8985662012528,54.9104330242742,0.));
#165937=CARTESIAN_POINT('Ctrl Pts',(48.8985662012528,54.9104330242742,12.));
#165938=CARTESIAN_POINT('Ctrl Pts',(48.8745443424477,54.8990816092953,0.));
#165939=CARTESIAN_POINT('Ctrl Pts',(48.8745443424477,54.8990816092953,12.));
#165940=CARTESIAN_POINT('Ctrl Pts',(48.8505664587974,54.8877238496566,0.));
#165941=CARTESIAN_POINT('Ctrl Pts',(48.8505664587974,54.8877238496566,12.));
#165942=CARTESIAN_POINT('Ctrl Pts',(48.8266326137622,54.8763598301037,0.));
#165943=CARTESIAN_POINT('Ctrl Pts',(48.8266326137622,54.8763598301037,12.));
#165944=CARTESIAN_POINT('Ctrl Pts',(48.8027428709614,54.8649896357285,0.));
#165945=CARTESIAN_POINT('Ctrl Pts',(48.8027428709614,54.8649896357285,12.));
#165946=CARTESIAN_POINT('Ctrl Pts',(48.7788972941438,54.8536133519292,0.));
#165947=CARTESIAN_POINT('Ctrl Pts',(48.7788972941438,54.8536133519292,12.));
#165948=CARTESIAN_POINT('Ctrl Pts',(48.7550959471601,54.8422310643763,0.));
#165949=CARTESIAN_POINT('Ctrl Pts',(48.7550959471601,54.8422310643763,12.));
#165950=CARTESIAN_POINT('Ctrl Pts',(48.7313388939845,54.8308428590344,0.));
#165951=CARTESIAN_POINT('Ctrl Pts',(48.7313388939845,54.8308428590344,12.));
#165952=CARTESIAN_POINT('Ctrl Pts',(48.7076261987292,54.819448822181,0.));
#165953=CARTESIAN_POINT('Ctrl Pts',(48.7076261987292,54.819448822181,12.));
#165954=CARTESIAN_POINT('Ctrl Pts',(48.6839579256566,54.8080490404275,0.));
#165955=CARTESIAN_POINT('Ctrl Pts',(48.6839579256566,54.8080490404275,12.));
#165956=CARTESIAN_POINT('Ctrl Pts',(48.6603341391886,54.796643600739,0.));
#165957=CARTESIAN_POINT('Ctrl Pts',(48.6603341391886,54.796643600739,12.));
#165958=CARTESIAN_POINT('Ctrl Pts',(48.6367549039112,54.7852325904583,0.));
#165959=CARTESIAN_POINT('Ctrl Pts',(48.6367549039112,54.7852325904583,12.));
#165960=CARTESIAN_POINT('Ctrl Pts',(48.6132202845783,54.7738160973031,0.));
#165961=CARTESIAN_POINT('Ctrl Pts',(48.6132202845783,54.7738160973031,12.));
#165962=CARTESIAN_POINT('Ctrl Pts',(48.5897303461125,54.7623942093586,0.));
#165963=CARTESIAN_POINT('Ctrl Pts',(48.5897303461125,54.7623942093586,12.));
#165964=CARTESIAN_POINT('Ctrl Pts',(48.5662851536026,54.7509670150714,0.));
#165965=CARTESIAN_POINT('Ctrl Pts',(48.5662851536026,54.7509670150714,12.));
#165966=CARTESIAN_POINT('Ctrl Pts',(48.5428847722977,54.7395346032453,0.));
#165967=CARTESIAN_POINT('Ctrl Pts',(48.5428847722977,54.7395346032453,12.));
#165968=CARTESIAN_POINT('Ctrl Pts',(48.519529267596,54.7280970630351,0.));
#165969=CARTESIAN_POINT('Ctrl Pts',(48.519529267596,54.7280970630351,12.));
#165970=CARTESIAN_POINT('Ctrl Pts',(48.4962187050457,54.716654483948,0.));
#165971=CARTESIAN_POINT('Ctrl Pts',(48.4962187050457,54.716654483948,12.));
#165972=CARTESIAN_POINT('Ctrl Pts',(48.472953150357,54.7052069558497,0.));
#165973=CARTESIAN_POINT('Ctrl Pts',(48.472953150357,54.7052069558497,12.));
#165974=CARTESIAN_POINT('Ctrl Pts',(48.4497326694052,54.6937545689695,0.));
#165975=CARTESIAN_POINT('Ctrl Pts',(48.4497326694052,54.6937545689695,12.));
#165976=CARTESIAN_POINT('Ctrl Pts',(48.426557328234,54.6822974139064,0.));
#165977=CARTESIAN_POINT('Ctrl Pts',(48.426557328234,54.6822974139064,12.));
#165978=CARTESIAN_POINT('Ctrl Pts',(48.4034271930514,54.6708355816358,0.));
#165979=CARTESIAN_POINT('Ctrl Pts',(48.4034271930514,54.6708355816358,12.));
#165980=CARTESIAN_POINT('Ctrl Pts',(48.3803423302294,54.6593691635145,0.));
#165981=CARTESIAN_POINT('Ctrl Pts',(48.3803423302294,54.6593691635145,12.));
#165982=CARTESIAN_POINT('Ctrl Pts',(48.3573028063124,54.6478982512794,0.));
#165983=CARTESIAN_POINT('Ctrl Pts',(48.3573028063124,54.6478982512794,12.));
#165984=CARTESIAN_POINT('Ctrl Pts',(48.3343086880194,54.6364229370494,0.));
#165985=CARTESIAN_POINT('Ctrl Pts',(48.3343086880194,54.6364229370494,12.));
#165986=CARTESIAN_POINT('Ctrl Pts',(48.3113600422443,54.6249433133261,0.));
#165987=CARTESIAN_POINT('Ctrl Pts',(48.3113600422443,54.6249433133261,12.));
#165988=CARTESIAN_POINT('Ctrl Pts',(48.2884569360506,54.6134594729959,0.));
#165989=CARTESIAN_POINT('Ctrl Pts',(48.2884569360506,54.6134594729959,12.));
#165990=CARTESIAN_POINT('Ctrl Pts',(48.2655994366665,54.6019715093309,0.));
#165991=CARTESIAN_POINT('Ctrl Pts',(48.2655994366665,54.6019715093309,12.));
#165992=CARTESIAN_POINT('Ctrl Pts',(48.2427876114947,54.5904795159926,0.));
#165993=CARTESIAN_POINT('Ctrl Pts',(48.2427876114947,54.5904795159926,12.));
#165994=CARTESIAN_POINT('Ctrl Pts',(48.2200215281173,54.5789835870342,0.));
#165995=CARTESIAN_POINT('Ctrl Pts',(48.2200215281173,54.5789835870342,12.));
#165996=CARTESIAN_POINT('Ctrl Pts',(48.1973012542966,54.5674838169041,0.));
#165997=CARTESIAN_POINT('Ctrl Pts',(48.1973012542966,54.5674838169041,12.));
#165998=CARTESIAN_POINT('Ctrl Pts',(48.1746268579736,54.5559803004492,0.));
#165999=CARTESIAN_POINT('Ctrl Pts',(48.1746268579736,54.5559803004492,12.));
#166000=CARTESIAN_POINT('Ctrl Pts',(48.1519984072622,54.5444731329201,0.));
#166001=CARTESIAN_POINT('Ctrl Pts',(48.1519984072622,54.5444731329201,12.));
#166002=CARTESIAN_POINT('Ctrl Pts',(48.1294159704573,54.5329624099721,0.));
#166003=CARTESIAN_POINT('Ctrl Pts',(48.1294159704573,54.5329624099721,12.));
#166004=CARTESIAN_POINT('Ctrl Pts',(48.1068796160405,54.5214482276678,0.));
#166005=CARTESIAN_POINT('Ctrl Pts',(48.1068796160405,54.5214482276678,12.));
#166006=CARTESIAN_POINT('Ctrl Pts',(48.0843894126806,54.5099306824786,0.));
#166007=CARTESIAN_POINT('Ctrl Pts',(48.0843894126806,54.5099306824786,12.));
#166008=CARTESIAN_POINT('Ctrl Pts',(48.0619454292324,54.4984098712886,0.));
#166009=CARTESIAN_POINT('Ctrl Pts',(48.0619454292324,54.4984098712886,12.));
#166010=CARTESIAN_POINT('Ctrl Pts',(48.0395477347298,54.4868858913971,0.));
#166011=CARTESIAN_POINT('Ctrl Pts',(48.0395477347298,54.4868858913971,12.));
#166012=CARTESIAN_POINT('Ctrl Pts',(48.0171963983924,54.4753588405215,0.));
#166013=CARTESIAN_POINT('Ctrl Pts',(48.0171963983924,54.4753588405215,12.));
#166014=CARTESIAN_POINT('Ctrl Pts',(47.9948914896326,54.4638288168003,0.));
#166015=CARTESIAN_POINT('Ctrl Pts',(47.9948914896326,54.4638288168003,12.));
#166016=CARTESIAN_POINT('Ctrl Pts',(47.9726330780572,54.4522959187955,0.));
#166017=CARTESIAN_POINT('Ctrl Pts',(47.9726330780572,54.4522959187955,12.));
#166018=CARTESIAN_POINT('Ctrl Pts',(47.9504212334675,54.4407602454967,0.));
#166019=CARTESIAN_POINT('Ctrl Pts',(47.9504212334675,54.4407602454967,12.));
#166020=CARTESIAN_POINT('Ctrl Pts',(47.9282560258516,54.429221896324,0.));
#166021=CARTESIAN_POINT('Ctrl Pts',(47.9282560258516,54.429221896324,12.));
#166022=CARTESIAN_POINT('Ctrl Pts',(47.9061375253897,54.4176809711311,0.));
#166023=CARTESIAN_POINT('Ctrl Pts',(47.9061375253897,54.4176809711311,12.));
#166024=CARTESIAN_POINT('Ctrl Pts',(47.8840658024618,54.4061375702079,0.));
#166025=CARTESIAN_POINT('Ctrl Pts',(47.8840658024618,54.4061375702079,12.));
#166026=CARTESIAN_POINT('Ctrl Pts',(47.8620409276493,54.3945917942832,0.));
#166027=CARTESIAN_POINT('Ctrl Pts',(47.8620409276493,54.3945917942832,12.));
#166028=CARTESIAN_POINT('Ctrl Pts',(47.8400629717355,54.3830437445279,0.));
#166029=CARTESIAN_POINT('Ctrl Pts',(47.8400629717355,54.3830437445279,12.));
#166030=CARTESIAN_POINT('Ctrl Pts',(47.8181320056995,54.3714935225591,0.));
#166031=CARTESIAN_POINT('Ctrl Pts',(47.8181320056995,54.3714935225591,12.));
#166032=CARTESIAN_POINT('Ctrl Pts',(47.7962481007185,54.3599412304437,0.));
#166033=CARTESIAN_POINT('Ctrl Pts',(47.7962481007185,54.3599412304437,12.));
#166034=CARTESIAN_POINT('Ctrl Pts',(47.7744113281771,54.3483869707002,0.));
#166035=CARTESIAN_POINT('Ctrl Pts',(47.7744113281771,54.3483869707002,12.));
#166036=CARTESIAN_POINT('Ctrl Pts',(47.7526217596694,54.3368308463023,0.));
#166037=CARTESIAN_POINT('Ctrl Pts',(47.7526217596694,54.3368308463023,12.));
#166038=CARTESIAN_POINT('Ctrl Pts',(47.7308794669993,54.3252729606823,0.));
#166039=CARTESIAN_POINT('Ctrl Pts',(47.7308794669993,54.3252729606823,12.));
#166040=CARTESIAN_POINT('Ctrl Pts',(47.7091845221747,54.3137134177345,0.));
#166041=CARTESIAN_POINT('Ctrl Pts',(47.7091845221747,54.3137134177345,12.));
#166042=CARTESIAN_POINT('Ctrl Pts',(47.6875369974087,54.302152321819,0.));
#166043=CARTESIAN_POINT('Ctrl Pts',(47.6875369974087,54.302152321819,12.));
#166044=CARTESIAN_POINT('Ctrl Pts',(47.6659369651301,54.290589777765,0.));
#166045=CARTESIAN_POINT('Ctrl Pts',(47.6659369651301,54.290589777765,12.));
#166046=CARTESIAN_POINT('Ctrl Pts',(47.6443844979847,54.2790258908738,0.));
#166047=CARTESIAN_POINT('Ctrl Pts',(47.6443844979847,54.2790258908738,12.));
#166048=CARTESIAN_POINT('Ctrl Pts',(47.6228796688375,54.2674607669226,0.));
#166049=CARTESIAN_POINT('Ctrl Pts',(47.6228796688375,54.2674607669226,12.));
#166050=CARTESIAN_POINT('Ctrl Pts',(47.6014225507659,54.2558945121678,0.));
#166051=CARTESIAN_POINT('Ctrl Pts',(47.6014225507659,54.2558945121678,12.));
#166052=CARTESIAN_POINT('Ctrl Pts',(47.5800132170608,54.244327233349,0.));
#166053=CARTESIAN_POINT('Ctrl Pts',(47.5800132170608,54.244327233349,12.));
#166054=CARTESIAN_POINT('Ctrl Pts',(47.5586517412363,54.2327590376924,0.));
#166055=CARTESIAN_POINT('Ctrl Pts',(47.5586517412363,54.2327590376924,12.));
#166056=CARTESIAN_POINT('Ctrl Pts',(47.5373381970326,54.2211900329138,0.));
#166057=CARTESIAN_POINT('Ctrl Pts',(47.5373381970326,54.2211900329138,12.));
#166058=CARTESIAN_POINT('Ctrl Pts',(47.5160726584174,54.209620327223,0.));
#166059=CARTESIAN_POINT('Ctrl Pts',(47.5160726584174,54.209620327223,12.));
#166060=CARTESIAN_POINT('Ctrl Pts',(47.4948551995801,54.198050029327,0.));
#166061=CARTESIAN_POINT('Ctrl Pts',(47.4948551995801,54.198050029327,12.));
#166062=CARTESIAN_POINT('Ctrl Pts',(47.4736858949322,54.1864792484345,0.));
#166063=CARTESIAN_POINT('Ctrl Pts',(47.4736858949322,54.1864792484345,12.));
#166064=CARTESIAN_POINT('Ctrl Pts',(47.4525648191173,54.1749080942593,0.));
#166065=CARTESIAN_POINT('Ctrl Pts',(47.4525648191173,54.1749080942593,12.));
#166066=CARTESIAN_POINT('Ctrl Pts',(47.4314920470141,54.1633366770239,0.));
#166067=CARTESIAN_POINT('Ctrl Pts',(47.4314920470141,54.1633366770239,12.));
#166068=CARTESIAN_POINT('Ctrl Pts',(47.4104676537381,54.1517651074637,0.));
#166069=CARTESIAN_POINT('Ctrl Pts',(47.4104676537381,54.1517651074637,12.));
#166070=CARTESIAN_POINT('Ctrl Pts',(47.3894917146365,54.1401934968311,0.));
#166071=CARTESIAN_POINT('Ctrl Pts',(47.3894917146365,54.1401934968311,12.));
#166072=CARTESIAN_POINT('Ctrl Pts',(47.3685643052874,54.1286219568989,0.));
#166073=CARTESIAN_POINT('Ctrl Pts',(47.3685643052874,54.1286219568989,12.));
#166074=CARTESIAN_POINT('Ctrl Pts',(47.3476855015102,54.1170505999645,0.));
#166075=CARTESIAN_POINT('Ctrl Pts',(47.3476855015102,54.1170505999645,12.));
#166076=CARTESIAN_POINT('Ctrl Pts',(47.3268553793694,54.1054795388543,0.));
#166077=CARTESIAN_POINT('Ctrl Pts',(47.3268553793694,54.1054795388543,12.));
#166078=CARTESIAN_POINT('Ctrl Pts',(47.3060740151752,54.0939088869269,0.));
#166079=CARTESIAN_POINT('Ctrl Pts',(47.3060740151752,54.0939088869269,12.));
#166080=CARTESIAN_POINT('Ctrl Pts',(47.2853414854793,54.0823387580776,0.));
#166081=CARTESIAN_POINT('Ctrl Pts',(47.2853414854793,54.0823387580776,12.));
#166082=CARTESIAN_POINT('Ctrl Pts',(47.2646578670746,54.0707692667438,0.));
#166083=CARTESIAN_POINT('Ctrl Pts',(47.2646578670746,54.0707692667438,12.));
#166084=CARTESIAN_POINT('Ctrl Pts',(47.2440232370065,54.0592005279086,0.));
#166085=CARTESIAN_POINT('Ctrl Pts',(47.2440232370065,54.0592005279086,12.));
#166086=CARTESIAN_POINT('Ctrl Pts',(47.2234376725743,54.047632657104,0.));
#166087=CARTESIAN_POINT('Ctrl Pts',(47.2234376725743,54.047632657104,12.));
#166088=CARTESIAN_POINT('Ctrl Pts',(47.202901251334,54.0360657704163,0.));
#166089=CARTESIAN_POINT('Ctrl Pts',(47.202901251334,54.0360657704163,12.));
#166090=CARTESIAN_POINT('Ctrl Pts',(47.1824140510926,54.0244999844893,0.));
#166091=CARTESIAN_POINT('Ctrl Pts',(47.1824140510926,54.0244999844893,12.));
#166092=CARTESIAN_POINT('Ctrl Pts',(47.1619761499087,54.0129354165297,0.));
#166093=CARTESIAN_POINT('Ctrl Pts',(47.1619761499087,54.0129354165297,12.));
#166094=CARTESIAN_POINT('Ctrl Pts',(47.1415876261035,54.0013721843118,0.));
#166095=CARTESIAN_POINT('Ctrl Pts',(47.1415876261035,54.0013721843118,12.));
#166096=CARTESIAN_POINT('Ctrl Pts',(47.1212485582643,53.989810406182,0.));
#166097=CARTESIAN_POINT('Ctrl Pts',(47.1212485582643,53.989810406182,12.));
#166098=CARTESIAN_POINT('Ctrl Pts',(47.1009590252458,53.9782502010634,0.));
#166099=CARTESIAN_POINT('Ctrl Pts',(47.1009590252458,53.9782502010634,12.));
#166100=CARTESIAN_POINT('Ctrl Pts',(47.0807191061648,53.9666916884596,0.));
#166101=CARTESIAN_POINT('Ctrl Pts',(47.0807191061648,53.9666916884596,12.));
#166102=CARTESIAN_POINT('Ctrl Pts',(47.0605288804008,53.95513498846,0.));
#166103=CARTESIAN_POINT('Ctrl Pts',(47.0605288804008,53.95513498846,12.));
#166104=CARTESIAN_POINT('Ctrl Pts',(47.0403884276071,53.9435802217436,0.));
#166105=CARTESIAN_POINT('Ctrl Pts',(47.0403884276071,53.9435802217436,12.));
#166106=CARTESIAN_POINT('Ctrl Pts',(47.0202978277138,53.9320275095853,0.));
#166107=CARTESIAN_POINT('Ctrl Pts',(47.0202978277138,53.9320275095853,12.));
#166108=CARTESIAN_POINT('Ctrl Pts',(47.0002571609297,53.9204769738596,0.));
#166109=CARTESIAN_POINT('Ctrl Pts',(47.0002571609297,53.9204769738596,12.));
#166110=CARTESIAN_POINT('Ctrl Pts',(46.9802665077366,53.9089287370463,0.));
#166111=CARTESIAN_POINT('Ctrl Pts',(46.9802665077366,53.9089287370463,12.));
#166112=CARTESIAN_POINT('Ctrl Pts',(46.960325948892,53.8973829222348,0.));
#166113=CARTESIAN_POINT('Ctrl Pts',(46.960325948892,53.8973829222348,12.));
#166114=CARTESIAN_POINT('Ctrl Pts',(46.94043556544,53.8858396531298,0.));
#166115=CARTESIAN_POINT('Ctrl Pts',(46.94043556544,53.8858396531298,12.));
#166116=CARTESIAN_POINT('Ctrl Pts',(46.9205954387133,53.8742990540563,0.));
#166117=CARTESIAN_POINT('Ctrl Pts',(46.9205954387133,53.8742990540563,12.));
#166118=CARTESIAN_POINT('Ctrl Pts',(46.9008056503351,53.8627612499638,0.));
#166119=CARTESIAN_POINT('Ctrl Pts',(46.9008056503351,53.8627612499638,12.));
#166120=CARTESIAN_POINT('Ctrl Pts',(46.881066282213,53.8512263664321,0.));
#166121=CARTESIAN_POINT('Ctrl Pts',(46.881066282213,53.8512263664321,12.));
#166122=CARTESIAN_POINT('Ctrl Pts',(46.8613774165435,53.8396945296757,0.));
#166123=CARTESIAN_POINT('Ctrl Pts',(46.8613774165435,53.8396945296757,12.));
#166124=CARTESIAN_POINT('Ctrl Pts',(46.841739135822,53.8281658665503,0.));
#166125=CARTESIAN_POINT('Ctrl Pts',(46.841739135822,53.8281658665503,12.));
#166126=CARTESIAN_POINT('Ctrl Pts',(46.8221515228457,53.816640504558,0.));
#166127=CARTESIAN_POINT('Ctrl Pts',(46.8221515228457,53.816640504558,12.));
#166128=CARTESIAN_POINT('Ctrl Pts',(46.802614660715,53.8051185718532,0.));
#166129=CARTESIAN_POINT('Ctrl Pts',(46.802614660715,53.8051185718532,12.));
#166130=CARTESIAN_POINT('Ctrl Pts',(46.7831286328278,53.793600197248,0.));
#166131=CARTESIAN_POINT('Ctrl Pts',(46.7831286328278,53.793600197248,12.));
#166132=CARTESIAN_POINT('Ctrl Pts',(46.763693522886,53.7820855102182,0.));
#166133=CARTESIAN_POINT('Ctrl Pts',(46.763693522886,53.7820855102182,12.));
#166134=CARTESIAN_POINT('Ctrl Pts',(46.7443094149045,53.7705746409076,0.));
#166135=CARTESIAN_POINT('Ctrl Pts',(46.7443094149045,53.7705746409076,12.));
#166136=CARTESIAN_POINT('Ctrl Pts',(46.7249763932129,53.7590677201342,0.));
#166137=CARTESIAN_POINT('Ctrl Pts',(46.7249763932129,53.7590677201342,12.));
#166138=CARTESIAN_POINT('Ctrl Pts',(46.7056945424559,53.7475648793946,0.));
#166139=CARTESIAN_POINT('Ctrl Pts',(46.7056945424559,53.7475648793946,12.));
#166140=CARTESIAN_POINT('Ctrl Pts',(46.6864639475862,53.7360662508675,0.));
#166141=CARTESIAN_POINT('Ctrl Pts',(46.6864639475862,53.7360662508675,12.));
#166142=CARTESIAN_POINT('Ctrl Pts',(46.6672846938752,53.7245719674221,0.));
#166143=CARTESIAN_POINT('Ctrl Pts',(46.6672846938752,53.7245719674221,12.));
#166144=CARTESIAN_POINT('Ctrl Pts',(46.6481568669217,53.7130821626262,0.));
#166145=CARTESIAN_POINT('Ctrl Pts',(46.6481568669217,53.7130821626262,12.));
#166146=CARTESIAN_POINT('Ctrl Pts',(46.6290805526559,53.7015969707541,0.));
#166147=CARTESIAN_POINT('Ctrl Pts',(46.6290805526559,53.7015969707541,12.));
#166148=CARTESIAN_POINT('Ctrl Pts',(46.6100558373401,53.690116526794,0.));
#166149=CARTESIAN_POINT('Ctrl Pts',(46.6100558373401,53.690116526794,12.));
#166150=CARTESIAN_POINT('Ctrl Pts',(46.5910828075652,53.678640966456,0.));
#166151=CARTESIAN_POINT('Ctrl Pts',(46.5910828075652,53.678640966456,12.));
#166152=CARTESIAN_POINT('Ctrl Pts',(46.5721615502589,53.6671704261735,0.));
#166153=CARTESIAN_POINT('Ctrl Pts',(46.5721615502589,53.6671704261735,12.));
#166154=CARTESIAN_POINT('Ctrl Pts',(46.5532921526899,53.6557050431069,0.));
#166155=CARTESIAN_POINT('Ctrl Pts',(46.5532921526899,53.6557050431069,12.));
#166156=CARTESIAN_POINT('Ctrl Pts',(46.5344747024677,53.6442449551455,0.));
#166157=CARTESIAN_POINT('Ctrl Pts',(46.5344747024677,53.6442449551455,12.));
#166158=CARTESIAN_POINT('Ctrl Pts',(46.5157092875377,53.6327903009098,0.));
#166159=CARTESIAN_POINT('Ctrl Pts',(46.5157092875377,53.6327903009098,12.));
#166160=CARTESIAN_POINT('Ctrl Pts',(46.4969959961779,53.6213412197542,0.));
#166161=CARTESIAN_POINT('Ctrl Pts',(46.4969959961779,53.6213412197542,12.));
#166162=CARTESIAN_POINT('Ctrl Pts',(46.4783349170182,53.6098978517869,0.));
#166163=CARTESIAN_POINT('Ctrl Pts',(46.4783349170182,53.6098978517869,12.));
#166164=CARTESIAN_POINT('Ctrl Pts',(46.4597261390526,53.5984603378862,0.));
#166165=CARTESIAN_POINT('Ctrl Pts',(46.4597261390526,53.5984603378862,12.));
#166166=CARTESIAN_POINT('Ctrl Pts',(46.4411697516474,53.5870288197161,0.));
#166167=CARTESIAN_POINT('Ctrl Pts',(46.4411697516474,53.5870288197161,12.));
#166168=CARTESIAN_POINT('Ctrl Pts',(46.422665844546,53.5756034397464,0.));
#166169=CARTESIAN_POINT('Ctrl Pts',(46.422665844546,53.5756034397464,12.));
#166170=CARTESIAN_POINT('Ctrl Pts',(46.4042145078682,53.5641843412537,0.));
#166171=CARTESIAN_POINT('Ctrl Pts',(46.4042145078682,53.5641843412537,12.));
#166172=CARTESIAN_POINT('Ctrl Pts',(46.3858158321044,53.552771668303,0.));
#166173=CARTESIAN_POINT('Ctrl Pts',(46.3858158321044,53.552771668303,12.));
#166174=CARTESIAN_POINT('Ctrl Pts',(46.3674699081043,53.5413655657323,0.));
#166175=CARTESIAN_POINT('Ctrl Pts',(46.3674699081043,53.5413655657323,12.));
#166176=CARTESIAN_POINT('Ctrl Pts',(46.3491768270664,53.5299661791396,0.));
#166177=CARTESIAN_POINT('Ctrl Pts',(46.3491768270664,53.5299661791396,12.));
#166178=CARTESIAN_POINT('Ctrl Pts',(46.3309366805112,53.518573654857,0.));
#166179=CARTESIAN_POINT('Ctrl Pts',(46.3309366805112,53.518573654857,12.));
#166180=CARTESIAN_POINT('Ctrl Pts',(46.3127495603117,53.5071881399932,0.));
#166181=CARTESIAN_POINT('Ctrl Pts',(46.3127495603117,53.5071881399932,12.));
#166182=CARTESIAN_POINT('Ctrl Pts',(46.2946155587428,53.4958097825019,0.));
#166183=CARTESIAN_POINT('Ctrl Pts',(46.2946155587428,53.4958097825019,12.));
#166184=CARTESIAN_POINT('Ctrl Pts',(46.2765347685198,53.4844387312414,0.));
#166185=CARTESIAN_POINT('Ctrl Pts',(46.2765347685198,53.4844387312414,12.));
#166186=CARTESIAN_POINT('Ctrl Pts',(46.2585072828343,53.4730751360359,0.));
#166187=CARTESIAN_POINT('Ctrl Pts',(46.2585072828343,53.4730751360359,12.));
#166188=CARTESIAN_POINT('Ctrl Pts',(46.2405331953872,53.4617191477382,0.));
#166189=CARTESIAN_POINT('Ctrl Pts',(46.2405331953872,53.4617191477382,12.));
#166190=CARTESIAN_POINT('Ctrl Pts',(46.2226126003185,53.4503709181158,0.));
#166191=CARTESIAN_POINT('Ctrl Pts',(46.2226126003185,53.4503709181158,12.));
#166192=CARTESIAN_POINT('Ctrl Pts',(46.2047455921276,53.4390305997263,0.));
#166193=CARTESIAN_POINT('Ctrl Pts',(46.2047455921276,53.4390305997263,12.));
#166194=CARTESIAN_POINT('Ctrl Pts',(46.1869322656027,53.4276983458129,0.));
#166195=CARTESIAN_POINT('Ctrl Pts',(46.1869322656027,53.4276983458129,12.));
#166196=CARTESIAN_POINT('Ctrl Pts',(46.1691727157149,53.4163743101535,0.));
#166197=CARTESIAN_POINT('Ctrl Pts',(46.1691727157149,53.4163743101535,12.));
#166198=CARTESIAN_POINT('Ctrl Pts',(46.1514670376035,53.4050586470463,0.));
#166199=CARTESIAN_POINT('Ctrl Pts',(46.1514670376035,53.4050586470463,12.));
#166200=CARTESIAN_POINT('Ctrl Pts',(46.1338153268116,53.3937515116572,0.));
#166201=CARTESIAN_POINT('Ctrl Pts',(46.1338153268116,53.3937515116572,12.));
#166202=CARTESIAN_POINT('Ctrl Pts',(46.1162176794891,53.3824530603284,0.));
#166203=CARTESIAN_POINT('Ctrl Pts',(46.1162176794891,53.3824530603284,12.));
#166204=CARTESIAN_POINT('Ctrl Pts',(46.0986741925646,53.3711634508426,0.));
#166205=CARTESIAN_POINT('Ctrl Pts',(46.0986741925646,53.3711634508426,12.));
#166206=CARTESIAN_POINT('Ctrl Pts',(46.0811849640195,53.3598828428519,0.));
#166207=CARTESIAN_POINT('Ctrl Pts',(46.0811849640195,53.3598828428519,12.));
#166208=CARTESIAN_POINT('Ctrl Pts',(46.0637500926954,53.3486113975868,0.));
#166209=CARTESIAN_POINT('Ctrl Pts',(46.0637500926954,53.3486113975868,12.));
#166210=CARTESIAN_POINT('Ctrl Pts',(46.046369677778,53.3373492770647,0.));
#166211=CARTESIAN_POINT('Ctrl Pts',(46.046369677778,53.3373492770647,12.));
#166212=CARTESIAN_POINT('Ctrl Pts',(46.0290438183598,53.3260966434277,0.));
#166213=CARTESIAN_POINT('Ctrl Pts',(46.0290438183598,53.3260966434277,12.));
#166214=CARTESIAN_POINT('Ctrl Pts',(46.0117726129893,53.3148536582658,0.));
#166215=CARTESIAN_POINT('Ctrl Pts',(46.0117726129893,53.3148536582658,12.));
#166216=CARTESIAN_POINT('Ctrl Pts',(45.9945561591486,53.3036204818367,0.));
#166217=CARTESIAN_POINT('Ctrl Pts',(45.9945561591486,53.3036204818367,12.));
#166218=CARTESIAN_POINT('Ctrl Pts',(45.9773945542415,53.2923972745585,0.));
#166219=CARTESIAN_POINT('Ctrl Pts',(45.9773945542415,53.2923972745585,12.));
#166220=CARTESIAN_POINT('Ctrl Pts',(45.9602878967714,53.2811841987945,0.));
#166221=CARTESIAN_POINT('Ctrl Pts',(45.9602878967714,53.2811841987945,12.));
#166222=CARTESIAN_POINT('Ctrl Pts',(45.9432362873001,53.2699814203097,0.));
#166223=CARTESIAN_POINT('Ctrl Pts',(45.9432362873001,53.2699814203097,12.));
#166224=CARTESIAN_POINT('Ctrl Pts',(45.9262398298323,53.2587891103835,0.));
#166225=CARTESIAN_POINT('Ctrl Pts',(45.9262398298323,53.2587891103835,12.));
#166226=CARTESIAN_POINT('Ctrl Pts',(45.9092986319343,53.2476074459977,0.));
#166227=CARTESIAN_POINT('Ctrl Pts',(45.9092986319343,53.2476074459977,12.));
#166228=CARTESIAN_POINT('Ctrl Pts',(45.8924128018354,53.2364366054276,0.));
#166229=CARTESIAN_POINT('Ctrl Pts',(45.8924128018354,53.2364366054276,12.));
#166230=CARTESIAN_POINT('Ctrl Pts',(45.8755824458715,53.2252767643652,0.));
#166231=CARTESIAN_POINT('Ctrl Pts',(45.8755824458715,53.2252767643652,12.));
#166232=CARTESIAN_POINT('Ctrl Pts',(45.8588076662598,53.2141280925458,0.));
#166233=CARTESIAN_POINT('Ctrl Pts',(45.8588076662598,53.2141280925458,12.));
#166234=CARTESIAN_POINT('Ctrl Pts',(45.8420885575386,53.2029907483602,0.));
#166235=CARTESIAN_POINT('Ctrl Pts',(45.8420885575386,53.2029907483602,12.));
#166236=CARTESIAN_POINT('Ctrl Pts',(45.8254252100003,53.1918648840598,0.));
#166237=CARTESIAN_POINT('Ctrl Pts',(45.8254252100003,53.1918648840598,12.));
#166238=CARTESIAN_POINT('Ctrl Pts',(45.8088177165124,53.1807506560977,0.));
#166239=CARTESIAN_POINT('Ctrl Pts',(45.8088177165124,53.1807506560977,12.));
#166240=CARTESIAN_POINT('Ctrl Pts',(45.7922661780005,53.1696482334487,0.));
#166241=CARTESIAN_POINT('Ctrl Pts',(45.7922661780005,53.1696482334487,12.));
#166242=CARTESIAN_POINT('Ctrl Pts',(45.7757707100568,53.158557807638,0.));
#166243=CARTESIAN_POINT('Ctrl Pts',(45.7757707100568,53.158557807638,12.));
#166244=CARTESIAN_POINT('Ctrl Pts',(45.7593314474412,53.147479599594,0.));
#166245=CARTESIAN_POINT('Ctrl Pts',(45.7593314474412,53.147479599594,12.));
#166246=CARTESIAN_POINT('Ctrl Pts',(45.7429485300727,53.136413838457,0.));
#166247=CARTESIAN_POINT('Ctrl Pts',(45.7429485300727,53.136413838457,12.));
#166248=CARTESIAN_POINT('Ctrl Pts',(45.7266220896951,53.1253607414806,0.));
#166249=CARTESIAN_POINT('Ctrl Pts',(45.7266220896951,53.1253607414806,12.));
#166250=CARTESIAN_POINT('Ctrl Pts',(45.7103522376744,53.1143204954981,0.));
#166251=CARTESIAN_POINT('Ctrl Pts',(45.7103522376744,53.1143204954981,12.));
#166252=CARTESIAN_POINT('Ctrl Pts',(45.6941390489239,53.1032932329074,0.));
#166253=CARTESIAN_POINT('Ctrl Pts',(45.6941390489239,53.1032932329074,12.));
#166254=CARTESIAN_POINT('Ctrl Pts',(45.6779825614486,53.0922790298736,0.));
#166255=CARTESIAN_POINT('Ctrl Pts',(45.6779825614486,53.0922790298736,12.));
#166256=CARTESIAN_POINT('Ctrl Pts',(45.6651027439479,53.083478145185,0.));
#166257=CARTESIAN_POINT('Ctrl Pts',(45.6651027439479,53.083478145185,12.));
#166258=CARTESIAN_POINT('Ctrl Pts',(45.6554684028296,53.0768833804386,0.));
#166259=CARTESIAN_POINT('Ctrl Pts',(45.6554684028296,53.0768833804386,12.));
#166260=CARTESIAN_POINT('Ctrl Pts',(45.6490568514146,53.0724894921921,0.));
#166261=CARTESIAN_POINT('Ctrl Pts',(45.6490568514146,53.0724894921921,12.));
#166262=CARTESIAN_POINT('Ctrl Pts',(45.6458539113724,53.0702932034641,0.));
#166263=CARTESIAN_POINT('Ctrl Pts',(45.6458539113724,53.0702932034641,12.));
#166264=CARTESIAN_POINT('',(45.6458539113724,53.0702932034641,12.));
#166265=CARTESIAN_POINT('Ctrl Pts',(45.6458539113724,53.0702932034641,12.));
#166266=CARTESIAN_POINT('Ctrl Pts',(45.6490568514146,53.0724894921921,12.));
#166267=CARTESIAN_POINT('Ctrl Pts',(45.6554684028296,53.0768833804386,12.));
#166268=CARTESIAN_POINT('Ctrl Pts',(45.6651027439479,53.083478145185,12.));
#166269=CARTESIAN_POINT('Ctrl Pts',(45.6779825614486,53.0922790298736,12.));
#166270=CARTESIAN_POINT('Ctrl Pts',(45.6941390489239,53.1032932329074,12.));
#166271=CARTESIAN_POINT('Ctrl Pts',(45.7103522376744,53.1143204954981,12.));
#166272=CARTESIAN_POINT('Ctrl Pts',(45.7266220896951,53.1253607414806,12.));
#166273=CARTESIAN_POINT('Ctrl Pts',(45.7429485300727,53.136413838457,12.));
#166274=CARTESIAN_POINT('Ctrl Pts',(45.7593314474412,53.147479599594,12.));
#166275=CARTESIAN_POINT('Ctrl Pts',(45.7757707100568,53.158557807638,12.));
#166276=CARTESIAN_POINT('Ctrl Pts',(45.7922661780005,53.1696482334487,12.));
#166277=CARTESIAN_POINT('Ctrl Pts',(45.8088177165124,53.1807506560977,12.));
#166278=CARTESIAN_POINT('Ctrl Pts',(45.8254252100003,53.1918648840598,12.));
#166279=CARTESIAN_POINT('Ctrl Pts',(45.8420885575386,53.2029907483602,12.));
#166280=CARTESIAN_POINT('Ctrl Pts',(45.8588076662598,53.2141280925458,12.));
#166281=CARTESIAN_POINT('Ctrl Pts',(45.8755824458715,53.2252767643652,12.));
#166282=CARTESIAN_POINT('Ctrl Pts',(45.8924128018354,53.2364366054276,12.));
#166283=CARTESIAN_POINT('Ctrl Pts',(45.9092986319343,53.2476074459977,12.));
#166284=CARTESIAN_POINT('Ctrl Pts',(45.9262398298323,53.2587891103835,12.));
#166285=CARTESIAN_POINT('Ctrl Pts',(45.9432362873001,53.2699814203097,12.));
#166286=CARTESIAN_POINT('Ctrl Pts',(45.9602878967714,53.2811841987945,12.));
#166287=CARTESIAN_POINT('Ctrl Pts',(45.9773945542415,53.2923972745585,12.));
#166288=CARTESIAN_POINT('Ctrl Pts',(45.9945561591486,53.3036204818367,12.));
#166289=CARTESIAN_POINT('Ctrl Pts',(46.0117726129893,53.3148536582658,12.));
#166290=CARTESIAN_POINT('Ctrl Pts',(46.0290438183598,53.3260966434277,12.));
#166291=CARTESIAN_POINT('Ctrl Pts',(46.046369677778,53.3373492770647,12.));
#166292=CARTESIAN_POINT('Ctrl Pts',(46.0637500926954,53.3486113975868,12.));
#166293=CARTESIAN_POINT('Ctrl Pts',(46.0811849640195,53.3598828428519,12.));
#166294=CARTESIAN_POINT('Ctrl Pts',(46.0986741925646,53.3711634508426,12.));
#166295=CARTESIAN_POINT('Ctrl Pts',(46.1162176794891,53.3824530603284,12.));
#166296=CARTESIAN_POINT('Ctrl Pts',(46.1338153268116,53.3937515116572,12.));
#166297=CARTESIAN_POINT('Ctrl Pts',(46.1514670376035,53.4050586470463,12.));
#166298=CARTESIAN_POINT('Ctrl Pts',(46.1691727157149,53.4163743101535,12.));
#166299=CARTESIAN_POINT('Ctrl Pts',(46.1869322656027,53.4276983458129,12.));
#166300=CARTESIAN_POINT('Ctrl Pts',(46.2047455921276,53.4390305997263,12.));
#166301=CARTESIAN_POINT('Ctrl Pts',(46.2226126003185,53.4503709181158,12.));
#166302=CARTESIAN_POINT('Ctrl Pts',(46.2405331953872,53.4617191477382,12.));
#166303=CARTESIAN_POINT('Ctrl Pts',(46.2585072828343,53.4730751360359,12.));
#166304=CARTESIAN_POINT('Ctrl Pts',(46.2765347685198,53.4844387312414,12.));
#166305=CARTESIAN_POINT('Ctrl Pts',(46.2946155587428,53.4958097825019,12.));
#166306=CARTESIAN_POINT('Ctrl Pts',(46.3127495603117,53.5071881399932,12.));
#166307=CARTESIAN_POINT('Ctrl Pts',(46.3309366805112,53.518573654857,12.));
#166308=CARTESIAN_POINT('Ctrl Pts',(46.3491768270664,53.5299661791396,12.));
#166309=CARTESIAN_POINT('Ctrl Pts',(46.3674699081043,53.5413655657323,12.));
#166310=CARTESIAN_POINT('Ctrl Pts',(46.3858158321044,53.552771668303,12.));
#166311=CARTESIAN_POINT('Ctrl Pts',(46.4042145078682,53.5641843412537,12.));
#166312=CARTESIAN_POINT('Ctrl Pts',(46.422665844546,53.5756034397464,12.));
#166313=CARTESIAN_POINT('Ctrl Pts',(46.4411697516474,53.5870288197161,12.));
#166314=CARTESIAN_POINT('Ctrl Pts',(46.4597261390526,53.5984603378862,12.));
#166315=CARTESIAN_POINT('Ctrl Pts',(46.4783349170182,53.6098978517869,12.));
#166316=CARTESIAN_POINT('Ctrl Pts',(46.4969959961779,53.6213412197542,12.));
#166317=CARTESIAN_POINT('Ctrl Pts',(46.5157092875377,53.6327903009098,12.));
#166318=CARTESIAN_POINT('Ctrl Pts',(46.5344747024677,53.6442449551455,12.));
#166319=CARTESIAN_POINT('Ctrl Pts',(46.5532921526899,53.6557050431069,12.));
#166320=CARTESIAN_POINT('Ctrl Pts',(46.5721615502589,53.6671704261735,12.));
#166321=CARTESIAN_POINT('Ctrl Pts',(46.5910828075652,53.678640966456,12.));
#166322=CARTESIAN_POINT('Ctrl Pts',(46.6100558373401,53.690116526794,12.));
#166323=CARTESIAN_POINT('Ctrl Pts',(46.6290805526559,53.7015969707541,12.));
#166324=CARTESIAN_POINT('Ctrl Pts',(46.6481568669217,53.7130821626262,12.));
#166325=CARTESIAN_POINT('Ctrl Pts',(46.6672846938752,53.7245719674221,12.));
#166326=CARTESIAN_POINT('Ctrl Pts',(46.6864639475862,53.7360662508675,12.));
#166327=CARTESIAN_POINT('Ctrl Pts',(46.7056945424559,53.7475648793946,12.));
#166328=CARTESIAN_POINT('Ctrl Pts',(46.7249763932129,53.7590677201342,12.));
#166329=CARTESIAN_POINT('Ctrl Pts',(46.7443094149045,53.7705746409076,12.));
#166330=CARTESIAN_POINT('Ctrl Pts',(46.763693522886,53.7820855102182,12.));
#166331=CARTESIAN_POINT('Ctrl Pts',(46.7831286328278,53.793600197248,12.));
#166332=CARTESIAN_POINT('Ctrl Pts',(46.802614660715,53.8051185718532,12.));
#166333=CARTESIAN_POINT('Ctrl Pts',(46.8221515228457,53.816640504558,12.));
#166334=CARTESIAN_POINT('Ctrl Pts',(46.841739135822,53.8281658665503,12.));
#166335=CARTESIAN_POINT('Ctrl Pts',(46.8613774165435,53.8396945296757,12.));
#166336=CARTESIAN_POINT('Ctrl Pts',(46.881066282213,53.8512263664321,12.));
#166337=CARTESIAN_POINT('Ctrl Pts',(46.9008056503351,53.8627612499638,12.));
#166338=CARTESIAN_POINT('Ctrl Pts',(46.9205954387133,53.8742990540563,12.));
#166339=CARTESIAN_POINT('Ctrl Pts',(46.94043556544,53.8858396531298,12.));
#166340=CARTESIAN_POINT('Ctrl Pts',(46.960325948892,53.8973829222348,12.));
#166341=CARTESIAN_POINT('Ctrl Pts',(46.9802665077366,53.9089287370463,12.));
#166342=CARTESIAN_POINT('Ctrl Pts',(47.0002571609297,53.9204769738596,12.));
#166343=CARTESIAN_POINT('Ctrl Pts',(47.0202978277138,53.9320275095853,12.));
#166344=CARTESIAN_POINT('Ctrl Pts',(47.0403884276071,53.9435802217436,12.));
#166345=CARTESIAN_POINT('Ctrl Pts',(47.0605288804008,53.95513498846,12.));
#166346=CARTESIAN_POINT('Ctrl Pts',(47.0807191061648,53.9666916884596,12.));
#166347=CARTESIAN_POINT('Ctrl Pts',(47.1009590252458,53.9782502010634,12.));
#166348=CARTESIAN_POINT('Ctrl Pts',(47.1212485582643,53.989810406182,12.));
#166349=CARTESIAN_POINT('Ctrl Pts',(47.1415876261035,54.0013721843118,12.));
#166350=CARTESIAN_POINT('Ctrl Pts',(47.1619761499087,54.0129354165297,12.));
#166351=CARTESIAN_POINT('Ctrl Pts',(47.1824140510926,54.0244999844893,12.));
#166352=CARTESIAN_POINT('Ctrl Pts',(47.202901251334,54.0360657704163,12.));
#166353=CARTESIAN_POINT('Ctrl Pts',(47.2234376725743,54.047632657104,12.));
#166354=CARTESIAN_POINT('Ctrl Pts',(47.2440232370065,54.0592005279086,12.));
#166355=CARTESIAN_POINT('Ctrl Pts',(47.2646578670746,54.0707692667438,12.));
#166356=CARTESIAN_POINT('Ctrl Pts',(47.2853414854793,54.0823387580776,12.));
#166357=CARTESIAN_POINT('Ctrl Pts',(47.3060740151752,54.0939088869269,12.));
#166358=CARTESIAN_POINT('Ctrl Pts',(47.3268553793694,54.1054795388543,12.));
#166359=CARTESIAN_POINT('Ctrl Pts',(47.3476855015102,54.1170505999645,12.));
#166360=CARTESIAN_POINT('Ctrl Pts',(47.3685643052874,54.1286219568989,12.));
#166361=CARTESIAN_POINT('Ctrl Pts',(47.3894917146365,54.1401934968311,12.));
#166362=CARTESIAN_POINT('Ctrl Pts',(47.4104676537381,54.1517651074637,12.));
#166363=CARTESIAN_POINT('Ctrl Pts',(47.4314920470141,54.1633366770239,12.));
#166364=CARTESIAN_POINT('Ctrl Pts',(47.4525648191173,54.1749080942593,12.));
#166365=CARTESIAN_POINT('Ctrl Pts',(47.4736858949322,54.1864792484345,12.));
#166366=CARTESIAN_POINT('Ctrl Pts',(47.4948551995801,54.198050029327,12.));
#166367=CARTESIAN_POINT('Ctrl Pts',(47.5160726584174,54.209620327223,12.));
#166368=CARTESIAN_POINT('Ctrl Pts',(47.5373381970326,54.2211900329138,12.));
#166369=CARTESIAN_POINT('Ctrl Pts',(47.5586517412363,54.2327590376924,12.));
#166370=CARTESIAN_POINT('Ctrl Pts',(47.5800132170608,54.244327233349,12.));
#166371=CARTESIAN_POINT('Ctrl Pts',(47.6014225507659,54.2558945121678,12.));
#166372=CARTESIAN_POINT('Ctrl Pts',(47.6228796688375,54.2674607669226,12.));
#166373=CARTESIAN_POINT('Ctrl Pts',(47.6443844979847,54.2790258908738,12.));
#166374=CARTESIAN_POINT('Ctrl Pts',(47.6659369651301,54.290589777765,12.));
#166375=CARTESIAN_POINT('Ctrl Pts',(47.6875369974087,54.302152321819,12.));
#166376=CARTESIAN_POINT('Ctrl Pts',(47.7091845221747,54.3137134177345,12.));
#166377=CARTESIAN_POINT('Ctrl Pts',(47.7308794669993,54.3252729606823,12.));
#166378=CARTESIAN_POINT('Ctrl Pts',(47.7526217596694,54.3368308463023,12.));
#166379=CARTESIAN_POINT('Ctrl Pts',(47.7744113281771,54.3483869707002,12.));
#166380=CARTESIAN_POINT('Ctrl Pts',(47.7962481007185,54.3599412304437,12.));
#166381=CARTESIAN_POINT('Ctrl Pts',(47.8181320056995,54.3714935225591,12.));
#166382=CARTESIAN_POINT('Ctrl Pts',(47.8400629717355,54.3830437445279,12.));
#166383=CARTESIAN_POINT('Ctrl Pts',(47.8620409276493,54.3945917942832,12.));
#166384=CARTESIAN_POINT('Ctrl Pts',(47.8840658024618,54.4061375702079,12.));
#166385=CARTESIAN_POINT('Ctrl Pts',(47.9061375253897,54.4176809711311,12.));
#166386=CARTESIAN_POINT('Ctrl Pts',(47.9282560258516,54.429221896324,12.));
#166387=CARTESIAN_POINT('Ctrl Pts',(47.9504212334675,54.4407602454967,12.));
#166388=CARTESIAN_POINT('Ctrl Pts',(47.9726330780572,54.4522959187955,12.));
#166389=CARTESIAN_POINT('Ctrl Pts',(47.9948914896326,54.4638288168003,12.));
#166390=CARTESIAN_POINT('Ctrl Pts',(48.0171963983924,54.4753588405215,12.));
#166391=CARTESIAN_POINT('Ctrl Pts',(48.0395477347298,54.4868858913971,12.));
#166392=CARTESIAN_POINT('Ctrl Pts',(48.0619454292324,54.4984098712886,12.));
#166393=CARTESIAN_POINT('Ctrl Pts',(48.0843894126806,54.5099306824786,12.));
#166394=CARTESIAN_POINT('Ctrl Pts',(48.1068796160405,54.5214482276678,12.));
#166395=CARTESIAN_POINT('Ctrl Pts',(48.1294159704573,54.5329624099721,12.));
#166396=CARTESIAN_POINT('Ctrl Pts',(48.1519984072622,54.5444731329201,12.));
#166397=CARTESIAN_POINT('Ctrl Pts',(48.1746268579736,54.5559803004492,12.));
#166398=CARTESIAN_POINT('Ctrl Pts',(48.1973012542966,54.5674838169041,12.));
#166399=CARTESIAN_POINT('Ctrl Pts',(48.2200215281173,54.5789835870342,12.));
#166400=CARTESIAN_POINT('Ctrl Pts',(48.2427876114947,54.5904795159926,12.));
#166401=CARTESIAN_POINT('Ctrl Pts',(48.2655994366665,54.6019715093309,12.));
#166402=CARTESIAN_POINT('Ctrl Pts',(48.2884569360506,54.6134594729959,12.));
#166403=CARTESIAN_POINT('Ctrl Pts',(48.3113600422443,54.6249433133261,12.));
#166404=CARTESIAN_POINT('Ctrl Pts',(48.3343086880194,54.6364229370494,12.));
#166405=CARTESIAN_POINT('Ctrl Pts',(48.3573028063124,54.6478982512794,12.));
#166406=CARTESIAN_POINT('Ctrl Pts',(48.3803423302294,54.6593691635145,12.));
#166407=CARTESIAN_POINT('Ctrl Pts',(48.4034271930514,54.6708355816358,12.));
#166408=CARTESIAN_POINT('Ctrl Pts',(48.426557328234,54.6822974139064,12.));
#166409=CARTESIAN_POINT('Ctrl Pts',(48.4497326694052,54.6937545689695,12.));
#166410=CARTESIAN_POINT('Ctrl Pts',(48.472953150357,54.7052069558497,12.));
#166411=CARTESIAN_POINT('Ctrl Pts',(48.4962187050457,54.716654483948,12.));
#166412=CARTESIAN_POINT('Ctrl Pts',(48.519529267596,54.7280970630351,12.));
#166413=CARTESIAN_POINT('Ctrl Pts',(48.5428847722977,54.7395346032453,12.));
#166414=CARTESIAN_POINT('Ctrl Pts',(48.5662851536026,54.7509670150714,12.));
#166415=CARTESIAN_POINT('Ctrl Pts',(48.5897303461125,54.7623942093586,12.));
#166416=CARTESIAN_POINT('Ctrl Pts',(48.6132202845783,54.7738160973031,12.));
#166417=CARTESIAN_POINT('Ctrl Pts',(48.6367549039112,54.7852325904583,12.));
#166418=CARTESIAN_POINT('Ctrl Pts',(48.6603341391886,54.796643600739,12.));
#166419=CARTESIAN_POINT('Ctrl Pts',(48.6839579256566,54.8080490404275,12.));
#166420=CARTESIAN_POINT('Ctrl Pts',(48.7076261987292,54.819448822181,12.));
#166421=CARTESIAN_POINT('Ctrl Pts',(48.7313388939845,54.8308428590344,12.));
#166422=CARTESIAN_POINT('Ctrl Pts',(48.7550959471601,54.8422310643763,12.));
#166423=CARTESIAN_POINT('Ctrl Pts',(48.7788972941438,54.8536133519292,12.));
#166424=CARTESIAN_POINT('Ctrl Pts',(48.8027428709614,54.8649896357285,12.));
#166425=CARTESIAN_POINT('Ctrl Pts',(48.8266326137622,54.8763598301037,12.));
#166426=CARTESIAN_POINT('Ctrl Pts',(48.8505664587974,54.8877238496566,12.));
#166427=CARTESIAN_POINT('Ctrl Pts',(48.8745443424477,54.8990816092953,12.));
#166428=CARTESIAN_POINT('Ctrl Pts',(48.8985662012528,54.9104330242742,12.));
#166429=CARTESIAN_POINT('Ctrl Pts',(48.9226319719368,54.9217780102355,12.));
#166430=CARTESIAN_POINT('Ctrl Pts',(48.9467415914269,54.9331164832424,12.));
#166431=CARTESIAN_POINT('Ctrl Pts',(48.9708949968795,54.9444483598378,12.));
#166432=CARTESIAN_POINT('Ctrl Pts',(48.9950921256526,54.9557735569943,12.));
#166433=CARTESIAN_POINT('Ctrl Pts',(49.0193329152479,54.9670919920029,12.));
#166434=CARTESIAN_POINT('Ctrl Pts',(49.0436173032528,54.9784035823766,12.));
#166435=CARTESIAN_POINT('Ctrl Pts',(49.067945227287,54.9897082457606,12.));
#166436=CARTESIAN_POINT('Ctrl Pts',(49.0923166249219,55.0010058998107,12.));
#166437=CARTESIAN_POINT('Ctrl Pts',(49.116731433673,55.012296462186,12.));
#166438=CARTESIAN_POINT('Ctrl Pts',(49.1411895911635,55.0235798508045,12.));
#166439=CARTESIAN_POINT('Ctrl Pts',(49.1656910352476,55.0348559840453,12.));
#166440=CARTESIAN_POINT('Ctrl Pts',(49.1902357041461,55.0461247809744,12.));
#166441=CARTESIAN_POINT('Ctrl Pts',(49.2148235365703,55.0573861615579,12.));
#166442=CARTESIAN_POINT('Ctrl Pts',(49.2394544718531,55.0686400468931,12.));
#166443=CARTESIAN_POINT('Ctrl Pts',(49.264128449652,55.079886358701,12.));
#166444=CARTESIAN_POINT('Ctrl Pts',(49.2888454096563,55.0911250188302,12.));
#166445=CARTESIAN_POINT('Ctrl Pts',(49.3136052912621,55.102355948714,12.));
#166446=CARTESIAN_POINT('Ctrl Pts',(49.3384080333155,55.1135790689464,12.));
#166447=CARTESIAN_POINT('Ctrl Pts',(49.3632535736715,55.1247942985619,12.));
#166448=CARTESIAN_POINT('Ctrl Pts',(49.3881418495489,55.1360015556221,12.));
#166449=CARTESIAN_POINT('Ctrl Pts',(49.4130727983201,55.1472007585183,12.));
#166450=CARTESIAN_POINT('Ctrl Pts',(49.4380463581965,55.1583918271116,12.));
#166451=CARTESIAN_POINT('Ctrl Pts',(49.4630624688793,55.1695746838174,12.));
#166452=CARTESIAN_POINT('Ctrl Pts',(49.4881210723966,55.1807492550119,12.));
#166453=CARTESIAN_POINT('Ctrl Pts',(49.5132221132992,55.1919154713647,12.));
#166454=CARTESIAN_POINT('Ctrl Pts',(49.5347748994759,55.2014798624093,12.));
#166455=CARTESIAN_POINT('Ctrl Pts',(49.551321852449,55.2088081099093,12.));
#166456=CARTESIAN_POINT('Ctrl Pts',(49.5628442142133,55.2139039604722,12.));
#166457=CARTESIAN_POINT('Ctrl Pts',(49.5693295981928,55.2167699151339,12.));
#166458=CARTESIAN_POINT('Ctrl Pts',(49.5707719660639,55.2174072001495,12.));
#166459=CARTESIAN_POINT('',(45.6458539113724,53.0702932034641,0.));
#166460=CARTESIAN_POINT('',(45.6458539113724,53.0702932034641,0.));
#166461=CARTESIAN_POINT('Ctrl Pts',(49.5707719660639,55.2174072001495,0.));
#166462=CARTESIAN_POINT('Ctrl Pts',(49.5693295981928,55.2167699151339,0.));
#166463=CARTESIAN_POINT('Ctrl Pts',(49.5628442142133,55.2139039604722,0.));
#166464=CARTESIAN_POINT('Ctrl Pts',(49.551321852449,55.2088081099093,0.));
#166465=CARTESIAN_POINT('Ctrl Pts',(49.5347748994759,55.2014798624093,0.));
#166466=CARTESIAN_POINT('Ctrl Pts',(49.5132221132992,55.1919154713647,0.));
#166467=CARTESIAN_POINT('Ctrl Pts',(49.4881210723966,55.1807492550119,0.));
#166468=CARTESIAN_POINT('Ctrl Pts',(49.4630624688793,55.1695746838174,0.));
#166469=CARTESIAN_POINT('Ctrl Pts',(49.4380463581965,55.1583918271116,0.));
#166470=CARTESIAN_POINT('Ctrl Pts',(49.4130727983201,55.1472007585183,0.));
#166471=CARTESIAN_POINT('Ctrl Pts',(49.3881418495489,55.1360015556221,0.));
#166472=CARTESIAN_POINT('Ctrl Pts',(49.3632535736715,55.1247942985619,0.));
#166473=CARTESIAN_POINT('Ctrl Pts',(49.3384080333155,55.1135790689464,0.));
#166474=CARTESIAN_POINT('Ctrl Pts',(49.3136052912621,55.102355948714,0.));
#166475=CARTESIAN_POINT('Ctrl Pts',(49.2888454096563,55.0911250188302,0.));
#166476=CARTESIAN_POINT('Ctrl Pts',(49.264128449652,55.079886358701,0.));
#166477=CARTESIAN_POINT('Ctrl Pts',(49.2394544718531,55.0686400468931,0.));
#166478=CARTESIAN_POINT('Ctrl Pts',(49.2148235365703,55.0573861615579,0.));
#166479=CARTESIAN_POINT('Ctrl Pts',(49.1902357041461,55.0461247809744,0.));
#166480=CARTESIAN_POINT('Ctrl Pts',(49.1656910352476,55.0348559840453,0.));
#166481=CARTESIAN_POINT('Ctrl Pts',(49.1411895911635,55.0235798508045,0.));
#166482=CARTESIAN_POINT('Ctrl Pts',(49.116731433673,55.012296462186,0.));
#166483=CARTESIAN_POINT('Ctrl Pts',(49.0923166249219,55.0010058998107,0.));
#166484=CARTESIAN_POINT('Ctrl Pts',(49.067945227287,54.9897082457606,0.));
#166485=CARTESIAN_POINT('Ctrl Pts',(49.0436173032528,54.9784035823766,0.));
#166486=CARTESIAN_POINT('Ctrl Pts',(49.0193329152479,54.9670919920029,0.));
#166487=CARTESIAN_POINT('Ctrl Pts',(48.9950921256526,54.9557735569943,0.));
#166488=CARTESIAN_POINT('Ctrl Pts',(48.9708949968795,54.9444483598378,0.));
#166489=CARTESIAN_POINT('Ctrl Pts',(48.9467415914269,54.9331164832424,0.));
#166490=CARTESIAN_POINT('Ctrl Pts',(48.9226319719368,54.9217780102355,0.));
#166491=CARTESIAN_POINT('Ctrl Pts',(48.8985662012528,54.9104330242742,0.));
#166492=CARTESIAN_POINT('Ctrl Pts',(48.8745443424477,54.8990816092953,0.));
#166493=CARTESIAN_POINT('Ctrl Pts',(48.8505664587974,54.8877238496566,0.));
#166494=CARTESIAN_POINT('Ctrl Pts',(48.8266326137622,54.8763598301037,0.));
#166495=CARTESIAN_POINT('Ctrl Pts',(48.8027428709614,54.8649896357285,0.));
#166496=CARTESIAN_POINT('Ctrl Pts',(48.7788972941438,54.8536133519292,0.));
#166497=CARTESIAN_POINT('Ctrl Pts',(48.7550959471601,54.8422310643763,0.));
#166498=CARTESIAN_POINT('Ctrl Pts',(48.7313388939845,54.8308428590344,0.));
#166499=CARTESIAN_POINT('Ctrl Pts',(48.7076261987292,54.819448822181,0.));
#166500=CARTESIAN_POINT('Ctrl Pts',(48.6839579256566,54.8080490404275,0.));
#166501=CARTESIAN_POINT('Ctrl Pts',(48.6603341391886,54.796643600739,0.));
#166502=CARTESIAN_POINT('Ctrl Pts',(48.6367549039112,54.7852325904583,0.));
#166503=CARTESIAN_POINT('Ctrl Pts',(48.6132202845783,54.7738160973031,0.));
#166504=CARTESIAN_POINT('Ctrl Pts',(48.5897303461125,54.7623942093586,0.));
#166505=CARTESIAN_POINT('Ctrl Pts',(48.5662851536026,54.7509670150714,0.));
#166506=CARTESIAN_POINT('Ctrl Pts',(48.5428847722977,54.7395346032453,0.));
#166507=CARTESIAN_POINT('Ctrl Pts',(48.519529267596,54.7280970630351,0.));
#166508=CARTESIAN_POINT('Ctrl Pts',(48.4962187050457,54.716654483948,0.));
#166509=CARTESIAN_POINT('Ctrl Pts',(48.472953150357,54.7052069558497,0.));
#166510=CARTESIAN_POINT('Ctrl Pts',(48.4497326694052,54.6937545689695,0.));
#166511=CARTESIAN_POINT('Ctrl Pts',(48.426557328234,54.6822974139064,0.));
#166512=CARTESIAN_POINT('Ctrl Pts',(48.4034271930514,54.6708355816358,0.));
#166513=CARTESIAN_POINT('Ctrl Pts',(48.3803423302294,54.6593691635145,0.));
#166514=CARTESIAN_POINT('Ctrl Pts',(48.3573028063124,54.6478982512794,0.));
#166515=CARTESIAN_POINT('Ctrl Pts',(48.3343086880194,54.6364229370494,0.));
#166516=CARTESIAN_POINT('Ctrl Pts',(48.3113600422443,54.6249433133261,0.));
#166517=CARTESIAN_POINT('Ctrl Pts',(48.2884569360506,54.6134594729959,0.));
#166518=CARTESIAN_POINT('Ctrl Pts',(48.2655994366665,54.6019715093309,0.));
#166519=CARTESIAN_POINT('Ctrl Pts',(48.2427876114947,54.5904795159926,0.));
#166520=CARTESIAN_POINT('Ctrl Pts',(48.2200215281173,54.5789835870342,0.));
#166521=CARTESIAN_POINT('Ctrl Pts',(48.1973012542966,54.5674838169041,0.));
#166522=CARTESIAN_POINT('Ctrl Pts',(48.1746268579736,54.5559803004492,0.));
#166523=CARTESIAN_POINT('Ctrl Pts',(48.1519984072622,54.5444731329201,0.));
#166524=CARTESIAN_POINT('Ctrl Pts',(48.1294159704573,54.5329624099721,0.));
#166525=CARTESIAN_POINT('Ctrl Pts',(48.1068796160405,54.5214482276678,0.));
#166526=CARTESIAN_POINT('Ctrl Pts',(48.0843894126806,54.5099306824786,0.));
#166527=CARTESIAN_POINT('Ctrl Pts',(48.0619454292324,54.4984098712886,0.));
#166528=CARTESIAN_POINT('Ctrl Pts',(48.0395477347298,54.4868858913971,0.));
#166529=CARTESIAN_POINT('Ctrl Pts',(48.0171963983924,54.4753588405215,0.));
#166530=CARTESIAN_POINT('Ctrl Pts',(47.9948914896326,54.4638288168003,0.));
#166531=CARTESIAN_POINT('Ctrl Pts',(47.9726330780572,54.4522959187955,0.));
#166532=CARTESIAN_POINT('Ctrl Pts',(47.9504212334675,54.4407602454967,0.));
#166533=CARTESIAN_POINT('Ctrl Pts',(47.9282560258516,54.429221896324,0.));
#166534=CARTESIAN_POINT('Ctrl Pts',(47.9061375253897,54.4176809711311,0.));
#166535=CARTESIAN_POINT('Ctrl Pts',(47.8840658024618,54.4061375702079,0.));
#166536=CARTESIAN_POINT('Ctrl Pts',(47.8620409276493,54.3945917942832,0.));
#166537=CARTESIAN_POINT('Ctrl Pts',(47.8400629717355,54.3830437445279,0.));
#166538=CARTESIAN_POINT('Ctrl Pts',(47.8181320056995,54.3714935225591,0.));
#166539=CARTESIAN_POINT('Ctrl Pts',(47.7962481007185,54.3599412304437,0.));
#166540=CARTESIAN_POINT('Ctrl Pts',(47.7744113281771,54.3483869707002,0.));
#166541=CARTESIAN_POINT('Ctrl Pts',(47.7526217596694,54.3368308463023,0.));
#166542=CARTESIAN_POINT('Ctrl Pts',(47.7308794669993,54.3252729606823,0.));
#166543=CARTESIAN_POINT('Ctrl Pts',(47.7091845221747,54.3137134177345,0.));
#166544=CARTESIAN_POINT('Ctrl Pts',(47.6875369974087,54.302152321819,0.));
#166545=CARTESIAN_POINT('Ctrl Pts',(47.6659369651301,54.290589777765,0.));
#166546=CARTESIAN_POINT('Ctrl Pts',(47.6443844979847,54.2790258908738,0.));
#166547=CARTESIAN_POINT('Ctrl Pts',(47.6228796688375,54.2674607669226,0.));
#166548=CARTESIAN_POINT('Ctrl Pts',(47.6014225507659,54.2558945121678,0.));
#166549=CARTESIAN_POINT('Ctrl Pts',(47.5800132170608,54.244327233349,0.));
#166550=CARTESIAN_POINT('Ctrl Pts',(47.5586517412363,54.2327590376924,0.));
#166551=CARTESIAN_POINT('Ctrl Pts',(47.5373381970326,54.2211900329138,0.));
#166552=CARTESIAN_POINT('Ctrl Pts',(47.5160726584174,54.209620327223,0.));
#166553=CARTESIAN_POINT('Ctrl Pts',(47.4948551995801,54.198050029327,0.));
#166554=CARTESIAN_POINT('Ctrl Pts',(47.4736858949322,54.1864792484345,0.));
#166555=CARTESIAN_POINT('Ctrl Pts',(47.4525648191173,54.1749080942593,0.));
#166556=CARTESIAN_POINT('Ctrl Pts',(47.4314920470141,54.1633366770239,0.));
#166557=CARTESIAN_POINT('Ctrl Pts',(47.4104676537381,54.1517651074637,0.));
#166558=CARTESIAN_POINT('Ctrl Pts',(47.3894917146365,54.1401934968311,0.));
#166559=CARTESIAN_POINT('Ctrl Pts',(47.3685643052874,54.1286219568989,0.));
#166560=CARTESIAN_POINT('Ctrl Pts',(47.3476855015102,54.1170505999645,0.));
#166561=CARTESIAN_POINT('Ctrl Pts',(47.3268553793694,54.1054795388543,0.));
#166562=CARTESIAN_POINT('Ctrl Pts',(47.3060740151752,54.0939088869269,0.));
#166563=CARTESIAN_POINT('Ctrl Pts',(47.2853414854793,54.0823387580776,0.));
#166564=CARTESIAN_POINT('Ctrl Pts',(47.2646578670746,54.0707692667438,0.));
#166565=CARTESIAN_POINT('Ctrl Pts',(47.2440232370065,54.0592005279086,0.));
#166566=CARTESIAN_POINT('Ctrl Pts',(47.2234376725743,54.047632657104,0.));
#166567=CARTESIAN_POINT('Ctrl Pts',(47.202901251334,54.0360657704163,0.));
#166568=CARTESIAN_POINT('Ctrl Pts',(47.1824140510926,54.0244999844893,0.));
#166569=CARTESIAN_POINT('Ctrl Pts',(47.1619761499087,54.0129354165297,0.));
#166570=CARTESIAN_POINT('Ctrl Pts',(47.1415876261035,54.0013721843118,0.));
#166571=CARTESIAN_POINT('Ctrl Pts',(47.1212485582643,53.989810406182,0.));
#166572=CARTESIAN_POINT('Ctrl Pts',(47.1009590252458,53.9782502010634,0.));
#166573=CARTESIAN_POINT('Ctrl Pts',(47.0807191061648,53.9666916884596,0.));
#166574=CARTESIAN_POINT('Ctrl Pts',(47.0605288804008,53.95513498846,0.));
#166575=CARTESIAN_POINT('Ctrl Pts',(47.0403884276071,53.9435802217436,0.));
#166576=CARTESIAN_POINT('Ctrl Pts',(47.0202978277138,53.9320275095853,0.));
#166577=CARTESIAN_POINT('Ctrl Pts',(47.0002571609297,53.9204769738596,0.));
#166578=CARTESIAN_POINT('Ctrl Pts',(46.9802665077366,53.9089287370463,0.));
#166579=CARTESIAN_POINT('Ctrl Pts',(46.960325948892,53.8973829222348,0.));
#166580=CARTESIAN_POINT('Ctrl Pts',(46.94043556544,53.8858396531298,0.));
#166581=CARTESIAN_POINT('Ctrl Pts',(46.9205954387133,53.8742990540563,0.));
#166582=CARTESIAN_POINT('Ctrl Pts',(46.9008056503351,53.8627612499638,0.));
#166583=CARTESIAN_POINT('Ctrl Pts',(46.881066282213,53.8512263664321,0.));
#166584=CARTESIAN_POINT('Ctrl Pts',(46.8613774165435,53.8396945296757,0.));
#166585=CARTESIAN_POINT('Ctrl Pts',(46.841739135822,53.8281658665503,0.));
#166586=CARTESIAN_POINT('Ctrl Pts',(46.8221515228457,53.816640504558,0.));
#166587=CARTESIAN_POINT('Ctrl Pts',(46.802614660715,53.8051185718532,0.));
#166588=CARTESIAN_POINT('Ctrl Pts',(46.7831286328278,53.793600197248,0.));
#166589=CARTESIAN_POINT('Ctrl Pts',(46.763693522886,53.7820855102182,0.));
#166590=CARTESIAN_POINT('Ctrl Pts',(46.7443094149045,53.7705746409076,0.));
#166591=CARTESIAN_POINT('Ctrl Pts',(46.7249763932129,53.7590677201342,0.));
#166592=CARTESIAN_POINT('Ctrl Pts',(46.7056945424559,53.7475648793946,0.));
#166593=CARTESIAN_POINT('Ctrl Pts',(46.6864639475862,53.7360662508675,0.));
#166594=CARTESIAN_POINT('Ctrl Pts',(46.6672846938752,53.7245719674221,0.));
#166595=CARTESIAN_POINT('Ctrl Pts',(46.6481568669217,53.7130821626262,0.));
#166596=CARTESIAN_POINT('Ctrl Pts',(46.6290805526559,53.7015969707541,0.));
#166597=CARTESIAN_POINT('Ctrl Pts',(46.6100558373401,53.690116526794,0.));
#166598=CARTESIAN_POINT('Ctrl Pts',(46.5910828075652,53.678640966456,0.));
#166599=CARTESIAN_POINT('Ctrl Pts',(46.5721615502589,53.6671704261735,0.));
#166600=CARTESIAN_POINT('Ctrl Pts',(46.5532921526899,53.6557050431069,0.));
#166601=CARTESIAN_POINT('Ctrl Pts',(46.5344747024677,53.6442449551455,0.));
#166602=CARTESIAN_POINT('Ctrl Pts',(46.5157092875377,53.6327903009098,0.));
#166603=CARTESIAN_POINT('Ctrl Pts',(46.4969959961779,53.6213412197542,0.));
#166604=CARTESIAN_POINT('Ctrl Pts',(46.4783349170182,53.6098978517869,0.));
#166605=CARTESIAN_POINT('Ctrl Pts',(46.4597261390526,53.5984603378862,0.));
#166606=CARTESIAN_POINT('Ctrl Pts',(46.4411697516474,53.5870288197161,0.));
#166607=CARTESIAN_POINT('Ctrl Pts',(46.422665844546,53.5756034397464,0.));
#166608=CARTESIAN_POINT('Ctrl Pts',(46.4042145078682,53.5641843412537,0.));
#166609=CARTESIAN_POINT('Ctrl Pts',(46.3858158321044,53.552771668303,0.));
#166610=CARTESIAN_POINT('Ctrl Pts',(46.3674699081043,53.5413655657323,0.));
#166611=CARTESIAN_POINT('Ctrl Pts',(46.3491768270664,53.5299661791396,0.));
#166612=CARTESIAN_POINT('Ctrl Pts',(46.3309366805112,53.518573654857,0.));
#166613=CARTESIAN_POINT('Ctrl Pts',(46.3127495603117,53.5071881399932,0.));
#166614=CARTESIAN_POINT('Ctrl Pts',(46.2946155587428,53.4958097825019,0.));
#166615=CARTESIAN_POINT('Ctrl Pts',(46.2765347685198,53.4844387312414,0.));
#166616=CARTESIAN_POINT('Ctrl Pts',(46.2585072828343,53.4730751360359,0.));
#166617=CARTESIAN_POINT('Ctrl Pts',(46.2405331953872,53.4617191477382,0.));
#166618=CARTESIAN_POINT('Ctrl Pts',(46.2226126003185,53.4503709181158,0.));
#166619=CARTESIAN_POINT('Ctrl Pts',(46.2047455921276,53.4390305997263,0.));
#166620=CARTESIAN_POINT('Ctrl Pts',(46.1869322656027,53.4276983458129,0.));
#166621=CARTESIAN_POINT('Ctrl Pts',(46.1691727157149,53.4163743101535,0.));
#166622=CARTESIAN_POINT('Ctrl Pts',(46.1514670376035,53.4050586470463,0.));
#166623=CARTESIAN_POINT('Ctrl Pts',(46.1338153268116,53.3937515116572,0.));
#166624=CARTESIAN_POINT('Ctrl Pts',(46.1162176794891,53.3824530603284,0.));
#166625=CARTESIAN_POINT('Ctrl Pts',(46.0986741925646,53.3711634508426,0.));
#166626=CARTESIAN_POINT('Ctrl Pts',(46.0811849640195,53.3598828428519,0.));
#166627=CARTESIAN_POINT('Ctrl Pts',(46.0637500926954,53.3486113975868,0.));
#166628=CARTESIAN_POINT('Ctrl Pts',(46.046369677778,53.3373492770647,0.));
#166629=CARTESIAN_POINT('Ctrl Pts',(46.0290438183598,53.3260966434277,0.));
#166630=CARTESIAN_POINT('Ctrl Pts',(46.0117726129893,53.3148536582658,0.));
#166631=CARTESIAN_POINT('Ctrl Pts',(45.9945561591486,53.3036204818367,0.));
#166632=CARTESIAN_POINT('Ctrl Pts',(45.9773945542415,53.2923972745585,0.));
#166633=CARTESIAN_POINT('Ctrl Pts',(45.9602878967714,53.2811841987945,0.));
#166634=CARTESIAN_POINT('Ctrl Pts',(45.9432362873001,53.2699814203097,0.));
#166635=CARTESIAN_POINT('Ctrl Pts',(45.9262398298323,53.2587891103835,0.));
#166636=CARTESIAN_POINT('Ctrl Pts',(45.9092986319343,53.2476074459977,0.));
#166637=CARTESIAN_POINT('Ctrl Pts',(45.8924128018354,53.2364366054276,0.));
#166638=CARTESIAN_POINT('Ctrl Pts',(45.8755824458715,53.2252767643652,0.));
#166639=CARTESIAN_POINT('Ctrl Pts',(45.8588076662598,53.2141280925458,0.));
#166640=CARTESIAN_POINT('Ctrl Pts',(45.8420885575386,53.2029907483602,0.));
#166641=CARTESIAN_POINT('Ctrl Pts',(45.8254252100003,53.1918648840598,0.));
#166642=CARTESIAN_POINT('Ctrl Pts',(45.8088177165124,53.1807506560977,0.));
#166643=CARTESIAN_POINT('Ctrl Pts',(45.7922661780005,53.1696482334487,0.));
#166644=CARTESIAN_POINT('Ctrl Pts',(45.7757707100568,53.158557807638,0.));
#166645=CARTESIAN_POINT('Ctrl Pts',(45.7593314474412,53.147479599594,0.));
#166646=CARTESIAN_POINT('Ctrl Pts',(45.7429485300727,53.136413838457,0.));
#166647=CARTESIAN_POINT('Ctrl Pts',(45.7266220896951,53.1253607414806,0.));
#166648=CARTESIAN_POINT('Ctrl Pts',(45.7103522376744,53.1143204954981,0.));
#166649=CARTESIAN_POINT('Ctrl Pts',(45.6941390489239,53.1032932329074,0.));
#166650=CARTESIAN_POINT('Ctrl Pts',(45.6779825614486,53.0922790298736,0.));
#166651=CARTESIAN_POINT('Ctrl Pts',(45.6651027439479,53.083478145185,0.));
#166652=CARTESIAN_POINT('Ctrl Pts',(45.6554684028296,53.0768833804386,0.));
#166653=CARTESIAN_POINT('Ctrl Pts',(45.6490568514146,53.0724894921921,0.));
#166654=CARTESIAN_POINT('Ctrl Pts',(45.6458539113724,53.0702932034641,0.));
#166655=CARTESIAN_POINT('Ctrl Pts',(54.5031396718592,50.7903314215393,0.));
#166656=CARTESIAN_POINT('Ctrl Pts',(54.5031396718592,50.7903314215393,12.));
#166657=CARTESIAN_POINT('Ctrl Pts',(54.4978248630387,50.7885805844281,0.));
#166658=CARTESIAN_POINT('Ctrl Pts',(54.4978248630387,50.7885805844281,12.));
#166659=CARTESIAN_POINT('Ctrl Pts',(54.4871993224832,50.7850776288814,0.));
#166660=CARTESIAN_POINT('Ctrl Pts',(54.4871993224832,50.7850776288814,12.));
#166661=CARTESIAN_POINT('Ctrl Pts',(54.4712732429066,50.7798193515888,0.));
#166662=CARTESIAN_POINT('Ctrl Pts',(54.4712732429066,50.7798193515888,12.));
#166663=CARTESIAN_POINT('Ctrl Pts',(54.4500629336429,50.7728006269349,0.));
#166664=CARTESIAN_POINT('Ctrl Pts',(54.4500629336429,50.7728006269349,12.));
#166665=CARTESIAN_POINT('Ctrl Pts',(54.423590828767,50.764014409002,0.));
#166666=CARTESIAN_POINT('Ctrl Pts',(54.423590828767,50.764014409002,12.));
#166667=CARTESIAN_POINT('Ctrl Pts',(54.3971595231574,50.7552153869475,0.));
#166668=CARTESIAN_POINT('Ctrl Pts',(54.3971595231574,50.7552153869475,12.));
#166669=CARTESIAN_POINT('Ctrl Pts',(54.3707690445749,50.7464035792906,0.));
#166670=CARTESIAN_POINT('Ctrl Pts',(54.3707690445749,50.7464035792906,12.));
#166671=CARTESIAN_POINT('Ctrl Pts',(54.3444194324054,50.7375790185896,0.));
#166672=CARTESIAN_POINT('Ctrl Pts',(54.3444194324054,50.7375790185896,12.));
#166673=CARTESIAN_POINT('Ctrl Pts',(54.3181107400663,50.7287417566123,0.));
#166674=CARTESIAN_POINT('Ctrl Pts',(54.3181107400663,50.7287417566123,12.));
#166675=CARTESIAN_POINT('Ctrl Pts',(54.2918430335206,50.7198918629451,0.));
#166676=CARTESIAN_POINT('Ctrl Pts',(54.2918430335206,50.7198918629451,12.));
#166677=CARTESIAN_POINT('Ctrl Pts',(54.2656163868104,50.7110294185698,0.));
#166678=CARTESIAN_POINT('Ctrl Pts',(54.2656163868104,50.7110294185698,12.));
#166679=CARTESIAN_POINT('Ctrl Pts',(54.2394308784026,50.7021545108311,0.));
#166680=CARTESIAN_POINT('Ctrl Pts',(54.2394308784026,50.7021545108311,12.));
#166681=CARTESIAN_POINT('Ctrl Pts',(54.2132865872985,50.6932672279772,0.));
#166682=CARTESIAN_POINT('Ctrl Pts',(54.2132865872985,50.6932672279772,12.));
#166683=CARTESIAN_POINT('Ctrl Pts',(54.1871835889981,50.6843676535492,0.));
#166684=CARTESIAN_POINT('Ctrl Pts',(54.1871835889981,50.6843676535492,12.));
#166685=CARTESIAN_POINT('Ctrl Pts',(54.1611219522394,50.67545586183,0.));
#166686=CARTESIAN_POINT('Ctrl Pts',(54.1611219522394,50.67545586183,12.));
#166687=CARTESIAN_POINT('Ctrl Pts',(54.1351017412804,50.6665319209869,0.));
#166688=CARTESIAN_POINT('Ctrl Pts',(54.1351017412804,50.6665319209869,12.));
#166689=CARTESIAN_POINT('Ctrl Pts',(54.1091230175367,50.6575958953221,0.));
#166690=CARTESIAN_POINT('Ctrl Pts',(54.1091230175367,50.6575958953221,12.));
#166691=CARTESIAN_POINT('Ctrl Pts',(54.0831858415189,50.6486478479465,0.));
#166692=CARTESIAN_POINT('Ctrl Pts',(54.0831858415189,50.6486478479465,12.));
#166693=CARTESIAN_POINT('Ctrl Pts',(54.0572902745076,50.6396878430939,0.));
#166694=CARTESIAN_POINT('Ctrl Pts',(54.0572902745076,50.6396878430939,12.));
#166695=CARTESIAN_POINT('Ctrl Pts',(54.0314363806708,50.6307159490553,0.));
#166696=CARTESIAN_POINT('Ctrl Pts',(54.0314363806708,50.6307159490553,12.));
#166697=CARTESIAN_POINT('Ctrl Pts',(54.0056242268399,50.6217322378648,0.));
#166698=CARTESIAN_POINT('Ctrl Pts',(54.0056242268399,50.6217322378648,12.));
#166699=CARTESIAN_POINT('Ctrl Pts',(53.979853881553,50.6127367839711,0.));
#166700=CARTESIAN_POINT('Ctrl Pts',(53.979853881553,50.6127367839711,12.));
#166701=CARTESIAN_POINT('Ctrl Pts',(53.9541254143119,50.603729663214,0.));
#166702=CARTESIAN_POINT('Ctrl Pts',(53.9541254143119,50.603729663214,12.));
#166703=CARTESIAN_POINT('Ctrl Pts',(53.9284388948004,50.5947109517483,0.));
#166704=CARTESIAN_POINT('Ctrl Pts',(53.9284388948004,50.5947109517483,12.));
#166705=CARTESIAN_POINT('Ctrl Pts',(53.9027943919836,50.5856807248151,0.));
#166706=CARTESIAN_POINT('Ctrl Pts',(53.9027943919836,50.5856807248151,12.));
#166707=CARTESIAN_POINT('Ctrl Pts',(53.8771919737032,50.5766390561884,0.));
#166708=CARTESIAN_POINT('Ctrl Pts',(53.8771919737032,50.5766390561884,12.));
#166709=CARTESIAN_POINT('Ctrl Pts',(53.8516317071804,50.5675860188538,0.));
#166710=CARTESIAN_POINT('Ctrl Pts',(53.8516317071804,50.5675860188538,12.));
#166711=CARTESIAN_POINT('Ctrl Pts',(53.8261136593075,50.5585216854091,0.));
#166712=CARTESIAN_POINT('Ctrl Pts',(53.8261136593075,50.5585216854091,12.));
#166713=CARTESIAN_POINT('Ctrl Pts',(53.8006378970197,50.5494461285761,0.));
#166714=CARTESIAN_POINT('Ctrl Pts',(53.8006378970197,50.5494461285761,12.));
#166715=CARTESIAN_POINT('Ctrl Pts',(53.7752044876304,50.5403594216698,0.));
#166716=CARTESIAN_POINT('Ctrl Pts',(53.7752044876304,50.5403594216698,12.));
#166717=CARTESIAN_POINT('Ctrl Pts',(53.7498134991703,50.5312616390779,0.));
#166718=CARTESIAN_POINT('Ctrl Pts',(53.7498134991703,50.5312616390779,12.));
#166719=CARTESIAN_POINT('Ctrl Pts',(53.7244650002374,50.522152856042,0.));
#166720=CARTESIAN_POINT('Ctrl Pts',(53.7244650002374,50.522152856042,12.));
#166721=CARTESIAN_POINT('Ctrl Pts',(53.6991590598548,50.513033148456,0.));
#166722=CARTESIAN_POINT('Ctrl Pts',(53.6991590598548,50.513033148456,12.));
#166723=CARTESIAN_POINT('Ctrl Pts',(53.6738957473158,50.503902592653,0.));
#166724=CARTESIAN_POINT('Ctrl Pts',(53.6738957473158,50.503902592653,12.));
#166725=CARTESIAN_POINT('Ctrl Pts',(53.6486751320436,50.4947612652149,0.));
#166726=CARTESIAN_POINT('Ctrl Pts',(53.6486751320436,50.4947612652149,12.));
#166727=CARTESIAN_POINT('Ctrl Pts',(53.623497283406,50.4856092427314,0.));
#166728=CARTESIAN_POINT('Ctrl Pts',(53.623497283406,50.4856092427314,12.));
#166729=CARTESIAN_POINT('Ctrl Pts',(53.5983622707238,50.4764466018071,0.));
#166730=CARTESIAN_POINT('Ctrl Pts',(53.5983622707238,50.4764466018071,12.));
#166731=CARTESIAN_POINT('Ctrl Pts',(53.5732701633609,50.4672734191756,0.));
#166732=CARTESIAN_POINT('Ctrl Pts',(53.5732701633609,50.4672734191756,12.));
#166733=CARTESIAN_POINT('Ctrl Pts',(53.5482210307868,50.4580897717838,0.));
#166734=CARTESIAN_POINT('Ctrl Pts',(53.5482210307868,50.4580897717838,12.));
#166735=CARTESIAN_POINT('Ctrl Pts',(53.5232149426413,50.4488957368839,0.));
#166736=CARTESIAN_POINT('Ctrl Pts',(53.5232149426413,50.4488957368839,12.));
#166737=CARTESIAN_POINT('Ctrl Pts',(53.4982519688024,50.4396913921382,0.));
#166738=CARTESIAN_POINT('Ctrl Pts',(53.4982519688024,50.4396913921382,12.));
#166739=CARTESIAN_POINT('Ctrl Pts',(53.4733321794188,50.4304768156667,0.));
#166740=CARTESIAN_POINT('Ctrl Pts',(53.4733321794188,50.4304768156667,12.));
#166741=CARTESIAN_POINT('Ctrl Pts',(53.4484556448776,50.4212520859914,0.));
#166742=CARTESIAN_POINT('Ctrl Pts',(53.4484556448776,50.4212520859914,12.));
#166743=CARTESIAN_POINT('Ctrl Pts',(53.4236224357838,50.4120172820047,0.));
#166744=CARTESIAN_POINT('Ctrl Pts',(53.4236224357838,50.4120172820047,12.));
#166745=CARTESIAN_POINT('Ctrl Pts',(53.398832622931,50.4027724829297,0.));
#166746=CARTESIAN_POINT('Ctrl Pts',(53.398832622931,50.4027724829297,12.));
#166747=CARTESIAN_POINT('Ctrl Pts',(53.3740862772681,50.3935177682837,0.));
#166748=CARTESIAN_POINT('Ctrl Pts',(53.3740862772681,50.3935177682837,12.));
#166749=CARTESIAN_POINT('Ctrl Pts',(53.3493834698697,50.384253217846,0.));
#166750=CARTESIAN_POINT('Ctrl Pts',(53.3493834698697,50.384253217846,12.));
#166751=CARTESIAN_POINT('Ctrl Pts',(53.3247242719587,50.3749789116786,0.));
#166752=CARTESIAN_POINT('Ctrl Pts',(53.3247242719587,50.3749789116786,12.));
#166753=CARTESIAN_POINT('Ctrl Pts',(53.300108754923,50.365694930143,0.));
#166754=CARTESIAN_POINT('Ctrl Pts',(53.300108754923,50.365694930143,12.));
#166755=CARTESIAN_POINT('Ctrl Pts',(53.2755369903293,50.3564013539199,0.));
#166756=CARTESIAN_POINT('Ctrl Pts',(53.2755369903293,50.3564013539199,12.));
#166757=CARTESIAN_POINT('Ctrl Pts',(53.2510090499336,50.3470982640289,0.));
#166758=CARTESIAN_POINT('Ctrl Pts',(53.2510090499336,50.3470982640289,12.));
#166759=CARTESIAN_POINT('Ctrl Pts',(53.2265250056887,50.3377857418515,0.));
#166760=CARTESIAN_POINT('Ctrl Pts',(53.2265250056887,50.3377857418515,12.));
#166761=CARTESIAN_POINT('Ctrl Pts',(53.2020849297471,50.3284638691278,0.));
#166762=CARTESIAN_POINT('Ctrl Pts',(53.2020849297471,50.3284638691278,12.));
#166763=CARTESIAN_POINT('Ctrl Pts',(53.1776888944616,50.3191327279493,0.));
#166764=CARTESIAN_POINT('Ctrl Pts',(53.1776888944616,50.3191327279493,12.));
#166765=CARTESIAN_POINT('Ctrl Pts',(53.1533369723818,50.3097924007534,0.));
#166766=CARTESIAN_POINT('Ctrl Pts',(53.1533369723818,50.3097924007534,12.));
#166767=CARTESIAN_POINT('Ctrl Pts',(53.1290292362485,50.300442970319,0.));
#166768=CARTESIAN_POINT('Ctrl Pts',(53.1290292362485,50.300442970319,12.));
#166769=CARTESIAN_POINT('Ctrl Pts',(53.1047657589812,50.2910845197619,0.));
#166770=CARTESIAN_POINT('Ctrl Pts',(53.1047657589812,50.2910845197619,12.));
#166771=CARTESIAN_POINT('Ctrl Pts',(53.0805466136798,50.2817171325358,0.));
#166772=CARTESIAN_POINT('Ctrl Pts',(53.0805466136798,50.2817171325358,12.));
#166773=CARTESIAN_POINT('Ctrl Pts',(53.0563718736366,50.2723408924373,0.));
#166774=CARTESIAN_POINT('Ctrl Pts',(53.0563718736366,50.2723408924373,12.));
#166775=CARTESIAN_POINT('Ctrl Pts',(53.0322416123406,50.2629558836111,0.));
#166776=CARTESIAN_POINT('Ctrl Pts',(53.0322416123406,50.2629558836111,12.));
#166777=CARTESIAN_POINT('Ctrl Pts',(53.0081559034801,50.2535621905552,0.));
#166778=CARTESIAN_POINT('Ctrl Pts',(53.0081559034801,50.2535621905552,12.));
#166779=CARTESIAN_POINT('Ctrl Pts',(52.9841148209402,50.2441598981286,0.));
#166780=CARTESIAN_POINT('Ctrl Pts',(52.9841148209402,50.2441598981286,12.));
#166781=CARTESIAN_POINT('Ctrl Pts',(52.9601184388028,50.2347490915555,0.));
#166782=CARTESIAN_POINT('Ctrl Pts',(52.9601184388028,50.2347490915555,12.));
#166783=CARTESIAN_POINT('Ctrl Pts',(52.9361668313542,50.2253298564241,0.));
#166784=CARTESIAN_POINT('Ctrl Pts',(52.9361668313542,50.2253298564241,12.));
#166785=CARTESIAN_POINT('Ctrl Pts',(52.9122600730884,50.2159022786879,0.));
#166786=CARTESIAN_POINT('Ctrl Pts',(52.9122600730884,50.2159022786879,12.));
#166787=CARTESIAN_POINT('Ctrl Pts',(52.8883982387068,50.2064664446663,0.));
#166788=CARTESIAN_POINT('Ctrl Pts',(52.8883982387068,50.2064664446663,12.));
#166789=CARTESIAN_POINT('Ctrl Pts',(52.8645814031133,50.1970224410471,0.));
#166790=CARTESIAN_POINT('Ctrl Pts',(52.8645814031133,50.1970224410471,12.));
#166791=CARTESIAN_POINT('Ctrl Pts',(52.8408096414093,50.1875703548884,0.));
#166792=CARTESIAN_POINT('Ctrl Pts',(52.8408096414093,50.1875703548884,12.));
#166793=CARTESIAN_POINT('Ctrl Pts',(52.8170830289044,50.1781102736205,0.));
#166794=CARTESIAN_POINT('Ctrl Pts',(52.8170830289044,50.1781102736205,12.));
#166795=CARTESIAN_POINT('Ctrl Pts',(52.7934016411205,50.1686422850488,0.));
#166796=CARTESIAN_POINT('Ctrl Pts',(52.7934016411205,50.1686422850488,12.));
#166797=CARTESIAN_POINT('Ctrl Pts',(52.769765553794,50.1591664773561,0.));
#166798=CARTESIAN_POINT('Ctrl Pts',(52.769765553794,50.1591664773561,12.));
#166799=CARTESIAN_POINT('Ctrl Pts',(52.7461748428738,50.1496829391073,0.));
#166800=CARTESIAN_POINT('Ctrl Pts',(52.7461748428738,50.1496829391073,12.));
#166801=CARTESIAN_POINT('Ctrl Pts',(52.7226295845161,50.1401917592537,0.));
#166802=CARTESIAN_POINT('Ctrl Pts',(52.7226295845161,50.1401917592537,12.));
#166803=CARTESIAN_POINT('Ctrl Pts',(52.699129855093,50.1306930271345,0.));
#166804=CARTESIAN_POINT('Ctrl Pts',(52.699129855093,50.1306930271345,12.));
#166805=CARTESIAN_POINT('Ctrl Pts',(52.6756757311978,50.1211868324781,0.));
#166806=CARTESIAN_POINT('Ctrl Pts',(52.6756757311978,50.1211868324781,12.));
#166807=CARTESIAN_POINT('Ctrl Pts',(52.652267289646,50.111673265404,0.));
#166808=CARTESIAN_POINT('Ctrl Pts',(52.652267289646,50.111673265404,12.));
#166809=CARTESIAN_POINT('Ctrl Pts',(52.6289046074746,50.1021524164264,0.));
#166810=CARTESIAN_POINT('Ctrl Pts',(52.6289046074746,50.1021524164264,12.));
#166811=CARTESIAN_POINT('Ctrl Pts',(52.6055877619348,50.0926243764578,0.));
#166812=CARTESIAN_POINT('Ctrl Pts',(52.6055877619348,50.0926243764578,12.));
#166813=CARTESIAN_POINT('Ctrl Pts',(52.5823168304994,50.0830892368107,0.));
#166814=CARTESIAN_POINT('Ctrl Pts',(52.5823168304994,50.0830892368107,12.));
#166815=CARTESIAN_POINT('Ctrl Pts',(52.5590918908702,50.0735470892007,0.));
#166816=CARTESIAN_POINT('Ctrl Pts',(52.5590918908702,50.0735470892007,12.));
#166817=CARTESIAN_POINT('Ctrl Pts',(52.5359130209792,50.0639980257479,0.));
#166818=CARTESIAN_POINT('Ctrl Pts',(52.5359130209792,50.0639980257479,12.));
#166819=CARTESIAN_POINT('Ctrl Pts',(52.5127802989896,50.0544421389818,0.));
#166820=CARTESIAN_POINT('Ctrl Pts',(52.5127802989896,50.0544421389818,12.));
#166821=CARTESIAN_POINT('Ctrl Pts',(52.4896938032884,50.0448795218441,0.));
#166822=CARTESIAN_POINT('Ctrl Pts',(52.4896938032884,50.0448795218441,12.));
#166823=CARTESIAN_POINT('Ctrl Pts',(52.4666536124913,50.0353102676921,0.));
#166824=CARTESIAN_POINT('Ctrl Pts',(52.4666536124913,50.0353102676921,12.));
#166825=CARTESIAN_POINT('Ctrl Pts',(52.4436598054515,50.0257344703,0.));
#166826=CARTESIAN_POINT('Ctrl Pts',(52.4436598054515,50.0257344703,12.));
#166827=CARTESIAN_POINT('Ctrl Pts',(52.4207124612608,50.0161522238616,0.));
#166828=CARTESIAN_POINT('Ctrl Pts',(52.4207124612608,50.0161522238616,12.));
#166829=CARTESIAN_POINT('Ctrl Pts',(52.3978116592509,50.0065636229938,0.));
#166830=CARTESIAN_POINT('Ctrl Pts',(52.3978116592509,50.0065636229938,12.));
#166831=CARTESIAN_POINT('Ctrl Pts',(52.3749574789871,49.9969687627408,0.));
#166832=CARTESIAN_POINT('Ctrl Pts',(52.3749574789871,49.9969687627408,12.));
#166833=CARTESIAN_POINT('Ctrl Pts',(52.3521500002718,49.9873677385775,0.));
#166834=CARTESIAN_POINT('Ctrl Pts',(52.3521500002718,49.9873677385775,12.));
#166835=CARTESIAN_POINT('Ctrl Pts',(52.3293893031528,49.9777606464106,0.));
#166836=CARTESIAN_POINT('Ctrl Pts',(52.3293893031528,49.9777606464106,12.));
#166837=CARTESIAN_POINT('Ctrl Pts',(52.3066754679265,49.9681475825824,0.));
#166838=CARTESIAN_POINT('Ctrl Pts',(52.3066754679265,49.9681475825824,12.));
#166839=CARTESIAN_POINT('Ctrl Pts',(52.2840085751384,49.9585286438733,0.));
#166840=CARTESIAN_POINT('Ctrl Pts',(52.2840085751384,49.9585286438733,12.));
#166841=CARTESIAN_POINT('Ctrl Pts',(52.2613887055773,49.9489039275064,0.));
#166842=CARTESIAN_POINT('Ctrl Pts',(52.2613887055773,49.9489039275064,12.));
#166843=CARTESIAN_POINT('Ctrl Pts',(52.2388159402771,49.9392735311509,0.));
#166844=CARTESIAN_POINT('Ctrl Pts',(52.2388159402771,49.9392735311509,12.));
#166845=CARTESIAN_POINT('Ctrl Pts',(52.2162903605275,49.9296375529245,0.));
#166846=CARTESIAN_POINT('Ctrl Pts',(52.2162903605275,49.9296375529245,12.));
#166847=CARTESIAN_POINT('Ctrl Pts',(52.1938120478754,49.9199960913962,0.));
#166848=CARTESIAN_POINT('Ctrl Pts',(52.1938120478754,49.9199960913962,12.));
#166849=CARTESIAN_POINT('Ctrl Pts',(52.1713810841276,49.9103492455902,0.));
#166850=CARTESIAN_POINT('Ctrl Pts',(52.1713810841276,49.9103492455902,12.));
#166851=CARTESIAN_POINT('Ctrl Pts',(52.1489975513445,49.9006971149895,0.));
#166852=CARTESIAN_POINT('Ctrl Pts',(52.1489975513445,49.9006971149895,12.));
#166853=CARTESIAN_POINT('Ctrl Pts',(52.1266615318407,49.8910397995397,0.));
#166854=CARTESIAN_POINT('Ctrl Pts',(52.1266615318407,49.8910397995397,12.));
#166855=CARTESIAN_POINT('Ctrl Pts',(52.1043731081962,49.8813773996517,0.));
#166856=CARTESIAN_POINT('Ctrl Pts',(52.1043731081962,49.8813773996517,12.));
#166857=CARTESIAN_POINT('Ctrl Pts',(52.0821323632587,49.8717100162048,0.));
#166858=CARTESIAN_POINT('Ctrl Pts',(52.0821323632587,49.8717100162048,12.));
#166859=CARTESIAN_POINT('Ctrl Pts',(52.0599393801452,49.86203775055,0.));
#166860=CARTESIAN_POINT('Ctrl Pts',(52.0599393801452,49.86203775055,12.));
#166861=CARTESIAN_POINT('Ctrl Pts',(52.0377942422376,49.8523607045149,0.));
#166862=CARTESIAN_POINT('Ctrl Pts',(52.0377942422376,49.8523607045149,12.));
#166863=CARTESIAN_POINT('Ctrl Pts',(52.0156970331823,49.8426789804071,0.));
#166864=CARTESIAN_POINT('Ctrl Pts',(52.0156970331823,49.8426789804071,12.));
#166865=CARTESIAN_POINT('Ctrl Pts',(51.9936478369008,49.8329926810172,0.));
#166866=CARTESIAN_POINT('Ctrl Pts',(51.9936478369008,49.8329926810172,12.));
#166867=CARTESIAN_POINT('Ctrl Pts',(51.9716467375937,49.8233019096222,0.));
#166868=CARTESIAN_POINT('Ctrl Pts',(51.9716467375937,49.8233019096222,12.));
#166869=CARTESIAN_POINT('Ctrl Pts',(51.9496938197418,49.8136067699896,0.));
#166870=CARTESIAN_POINT('Ctrl Pts',(51.9496938197418,49.8136067699896,12.));
#166871=CARTESIAN_POINT('Ctrl Pts',(51.9277891681018,49.8039073663812,0.));
#166872=CARTESIAN_POINT('Ctrl Pts',(51.9277891681018,49.8039073663812,12.));
#166873=CARTESIAN_POINT('Ctrl Pts',(51.9059328677059,49.7942038035576,0.));
#166874=CARTESIAN_POINT('Ctrl Pts',(51.9059328677059,49.7942038035576,12.));
#166875=CARTESIAN_POINT('Ctrl Pts',(51.8841250038724,49.7844961867808,0.));
#166876=CARTESIAN_POINT('Ctrl Pts',(51.8841250038724,49.7844961867808,12.));
#166877=CARTESIAN_POINT('Ctrl Pts',(51.8623656622097,49.7747846218182,0.));
#166878=CARTESIAN_POINT('Ctrl Pts',(51.8623656622097,49.7747846218182,12.));
#166879=CARTESIAN_POINT('Ctrl Pts',(51.8406549286175,49.7650692149462,0.));
#166880=CARTESIAN_POINT('Ctrl Pts',(51.8406549286175,49.7650692149462,12.));
#166881=CARTESIAN_POINT('Ctrl Pts',(51.8189928892828,49.755350072955,0.));
#166882=CARTESIAN_POINT('Ctrl Pts',(51.8189928892828,49.755350072955,12.));
#166883=CARTESIAN_POINT('Ctrl Pts',(51.7973796306803,49.7456273031534,0.));
#166884=CARTESIAN_POINT('Ctrl Pts',(51.7973796306803,49.7456273031534,12.));
#166885=CARTESIAN_POINT('Ctrl Pts',(51.7758152395836,49.7359010133721,0.));
#166886=CARTESIAN_POINT('Ctrl Pts',(51.7758152395836,49.7359010133721,12.));
#166887=CARTESIAN_POINT('Ctrl Pts',(51.754299803067,49.7261713119663,0.));
#166888=CARTESIAN_POINT('Ctrl Pts',(51.754299803067,49.7261713119663,12.));
#166889=CARTESIAN_POINT('Ctrl Pts',(51.7328334085091,49.7164383078212,0.));
#166890=CARTESIAN_POINT('Ctrl Pts',(51.7328334085091,49.7164383078212,12.));
#166891=CARTESIAN_POINT('Ctrl Pts',(51.7114161435869,49.7067021103553,0.));
#166892=CARTESIAN_POINT('Ctrl Pts',(51.7114161435869,49.7067021103553,12.));
#166893=CARTESIAN_POINT('Ctrl Pts',(51.6900480962773,49.6969628295262,0.));
#166894=CARTESIAN_POINT('Ctrl Pts',(51.6900480962773,49.6969628295262,12.));
#166895=CARTESIAN_POINT('Ctrl Pts',(51.6687293548682,49.6872205758336,0.));
#166896=CARTESIAN_POINT('Ctrl Pts',(51.6687293548682,49.6872205758336,12.));
#166897=CARTESIAN_POINT('Ctrl Pts',(51.6474600079622,49.6774754603245,0.));
#166898=CARTESIAN_POINT('Ctrl Pts',(51.6474600079622,49.6774754603245,12.));
#166899=CARTESIAN_POINT('Ctrl Pts',(51.626240144479,49.6677275945967,0.));
#166900=CARTESIAN_POINT('Ctrl Pts',(51.626240144479,49.6677275945967,12.));
#166901=CARTESIAN_POINT('Ctrl Pts',(51.6050698536496,49.6579770908037,0.));
#166902=CARTESIAN_POINT('Ctrl Pts',(51.6050698536496,49.6579770908037,12.));
#166903=CARTESIAN_POINT('Ctrl Pts',(51.5839492250181,49.6482240616593,0.));
#166904=CARTESIAN_POINT('Ctrl Pts',(51.5839492250181,49.6482240616593,12.));
#166905=CARTESIAN_POINT('Ctrl Pts',(51.5628783484525,49.6384686204413,0.));
#166906=CARTESIAN_POINT('Ctrl Pts',(51.5628783484525,49.6384686204413,12.));
#166907=CARTESIAN_POINT('Ctrl Pts',(51.5418573141484,49.6287108809966,0.));
#166908=CARTESIAN_POINT('Ctrl Pts',(51.5418573141484,49.6287108809966,12.));
#166909=CARTESIAN_POINT('Ctrl Pts',(51.5208862126315,49.6189509577452,0.));
#166910=CARTESIAN_POINT('Ctrl Pts',(51.5208862126315,49.6189509577452,12.));
#166911=CARTESIAN_POINT('Ctrl Pts',(51.4999651347523,49.6091889656866,0.));
#166912=CARTESIAN_POINT('Ctrl Pts',(51.4999651347523,49.6091889656866,12.));
#166913=CARTESIAN_POINT('Ctrl Pts',(51.4790941716888,49.5994250204031,0.));
#166914=CARTESIAN_POINT('Ctrl Pts',(51.4790941716888,49.5994250204031,12.));
#166915=CARTESIAN_POINT('Ctrl Pts',(51.4582734149583,49.5896592380654,0.));
#166916=CARTESIAN_POINT('Ctrl Pts',(51.4582734149583,49.5896592380654,12.));
#166917=CARTESIAN_POINT('Ctrl Pts',(51.4375029564197,49.5798917354366,0.));
#166918=CARTESIAN_POINT('Ctrl Pts',(51.4375029564197,49.5798917354366,12.));
#166919=CARTESIAN_POINT('Ctrl Pts',(51.4167828882756,49.5701226298769,0.));
#166920=CARTESIAN_POINT('Ctrl Pts',(51.4167828882756,49.5701226298769,12.));
#166921=CARTESIAN_POINT('Ctrl Pts',(51.396113303067,49.5603520393496,0.));
#166922=CARTESIAN_POINT('Ctrl Pts',(51.396113303067,49.5603520393496,12.));
#166923=CARTESIAN_POINT('Ctrl Pts',(51.3754942936778,49.550580082425,0.));
#166924=CARTESIAN_POINT('Ctrl Pts',(51.3754942936778,49.550580082425,12.));
#166925=CARTESIAN_POINT('Ctrl Pts',(51.3549259533458,49.5408068782859,0.));
#166926=CARTESIAN_POINT('Ctrl Pts',(51.3549259533458,49.5408068782859,12.));
#166927=CARTESIAN_POINT('Ctrl Pts',(51.3344083756657,49.5310325467332,0.));
#166928=CARTESIAN_POINT('Ctrl Pts',(51.3344083756657,49.5310325467332,12.));
#166929=CARTESIAN_POINT('Ctrl Pts',(51.313941654591,49.5212572081908,0.));
#166930=CARTESIAN_POINT('Ctrl Pts',(51.313941654591,49.5212572081908,12.));
#166931=CARTESIAN_POINT('Ctrl Pts',(51.2935258844289,49.5114809837122,0.));
#166932=CARTESIAN_POINT('Ctrl Pts',(51.2935258844289,49.5114809837122,12.));
#166933=CARTESIAN_POINT('Ctrl Pts',(51.2731611598475,49.5017039949852,0.));
#166934=CARTESIAN_POINT('Ctrl Pts',(51.2731611598475,49.5017039949852,12.));
#166935=CARTESIAN_POINT('Ctrl Pts',(51.2528475758846,49.4919263643362,0.));
#166936=CARTESIAN_POINT('Ctrl Pts',(51.2528475758846,49.4919263643362,12.));
#166937=CARTESIAN_POINT('Ctrl Pts',(51.2325852279506,49.4821482147356,0.));
#166938=CARTESIAN_POINT('Ctrl Pts',(51.2325852279506,49.4821482147356,12.));
#166939=CARTESIAN_POINT('Ctrl Pts',(51.2123742118287,49.4723696698021,0.));
#166940=CARTESIAN_POINT('Ctrl Pts',(51.2123742118287,49.4723696698021,12.));
#166941=CARTESIAN_POINT('Ctrl Pts',(51.1922146236686,49.4625908538074,0.));
#166942=CARTESIAN_POINT('Ctrl Pts',(51.1922146236686,49.4625908538074,12.));
#166943=CARTESIAN_POINT('Ctrl Pts',(51.1721065599973,49.4528118916832,0.));
#166944=CARTESIAN_POINT('Ctrl Pts',(51.1721065599973,49.4528118916832,12.));
#166945=CARTESIAN_POINT('Ctrl Pts',(51.1520501177291,49.4430329090287,0.));
#166946=CARTESIAN_POINT('Ctrl Pts',(51.1520501177291,49.4430329090287,12.));
#166947=CARTESIAN_POINT('Ctrl Pts',(51.1320453941702,49.4332540321178,0.));
#166948=CARTESIAN_POINT('Ctrl Pts',(51.1320453941702,49.4332540321178,12.));
#166949=CARTESIAN_POINT('Ctrl Pts',(51.1120924870195,49.423475387907,0.));
#166950=CARTESIAN_POINT('Ctrl Pts',(51.1120924870195,49.423475387907,12.));
#166951=CARTESIAN_POINT('Ctrl Pts',(51.0921914943662,49.4136971040428,0.));
#166952=CARTESIAN_POINT('Ctrl Pts',(51.0921914943662,49.4136971040428,12.));
#166953=CARTESIAN_POINT('Ctrl Pts',(51.0723425146985,49.4039193088634,0.));
#166954=CARTESIAN_POINT('Ctrl Pts',(51.0723425146985,49.4039193088634,12.));
#166955=CARTESIAN_POINT('Ctrl Pts',(51.052545646907,49.3941421314013,0.));
#166956=CARTESIAN_POINT('Ctrl Pts',(51.052545646907,49.3941421314013,12.));
#166957=CARTESIAN_POINT('Ctrl Pts',(51.0328009902858,49.3843657013852,0.));
#166958=CARTESIAN_POINT('Ctrl Pts',(51.0328009902858,49.3843657013852,12.));
#166959=CARTESIAN_POINT('Ctrl Pts',(51.0131086445272,49.3745901492432,0.));
#166960=CARTESIAN_POINT('Ctrl Pts',(51.0131086445272,49.3745901492432,12.));
#166961=CARTESIAN_POINT('Ctrl Pts',(50.9934687097188,49.3648156061058,0.));
#166962=CARTESIAN_POINT('Ctrl Pts',(50.9934687097188,49.3648156061058,12.));
#166963=CARTESIAN_POINT('Ctrl Pts',(50.9738812863646,49.355042203823,0.));
#166964=CARTESIAN_POINT('Ctrl Pts',(50.9738812863646,49.355042203823,12.));
#166965=CARTESIAN_POINT('Ctrl Pts',(50.9543464753981,49.345270074981,0.));
#166966=CARTESIAN_POINT('Ctrl Pts',(50.9543464753981,49.345270074981,12.));
#166967=CARTESIAN_POINT('Ctrl Pts',(50.9348643781924,49.3354993529159,0.));
#166968=CARTESIAN_POINT('Ctrl Pts',(50.9348643781924,49.3354993529159,12.));
#166969=CARTESIAN_POINT('Ctrl Pts',(50.9154350965666,49.3257301717335,0.));
#166970=CARTESIAN_POINT('Ctrl Pts',(50.9154350965666,49.3257301717335,12.));
#166971=CARTESIAN_POINT('Ctrl Pts',(50.8960587327848,49.3159626663109,0.));
#166972=CARTESIAN_POINT('Ctrl Pts',(50.8960587327848,49.3159626663109,12.));
#166973=CARTESIAN_POINT('Ctrl Pts',(50.8767353895492,49.3061969722781,0.));
#166974=CARTESIAN_POINT('Ctrl Pts',(50.8767353895492,49.3061969722781,12.));
#166975=CARTESIAN_POINT('Ctrl Pts',(50.8574651699873,49.2964332260039,0.));
#166976=CARTESIAN_POINT('Ctrl Pts',(50.8574651699873,49.2964332260039,12.));
#166977=CARTESIAN_POINT('Ctrl Pts',(50.8382481776403,49.2866715645838,0.));
#166978=CARTESIAN_POINT('Ctrl Pts',(50.8382481776403,49.2866715645838,12.));
#166979=CARTESIAN_POINT('Ctrl Pts',(50.819084516434,49.2769121258164,0.));
#166980=CARTESIAN_POINT('Ctrl Pts',(50.819084516434,49.2769121258164,12.));
#166981=CARTESIAN_POINT('Ctrl Pts',(50.7999742907131,49.2671550482435,0.));
#166982=CARTESIAN_POINT('Ctrl Pts',(50.7999742907131,49.2671550482435,12.));
#166983=CARTESIAN_POINT('Ctrl Pts',(50.7809176052966,49.2574004712134,0.));
#166984=CARTESIAN_POINT('Ctrl Pts',(50.7809176052966,49.2574004712134,12.));
#166985=CARTESIAN_POINT('Ctrl Pts',(50.7619145655207,49.2476485349373,0.));
#166986=CARTESIAN_POINT('Ctrl Pts',(50.7619145655207,49.2476485349373,12.));
#166987=CARTESIAN_POINT('Ctrl Pts',(50.7429652772805,49.2378993805471,0.));
#166988=CARTESIAN_POINT('Ctrl Pts',(50.7429652772805,49.2378993805471,12.));
#166989=CARTESIAN_POINT('Ctrl Pts',(50.7240698470679,49.228153150155,0.));
#166990=CARTESIAN_POINT('Ctrl Pts',(50.7240698470679,49.228153150155,12.));
#166991=CARTESIAN_POINT('Ctrl Pts',(50.7052283818922,49.2184099867461,0.));
#166992=CARTESIAN_POINT('Ctrl Pts',(50.7052283818922,49.2184099867461,12.));
#166993=CARTESIAN_POINT('Ctrl Pts',(50.6864409891895,49.2086700340614,0.));
#166994=CARTESIAN_POINT('Ctrl Pts',(50.6864409891895,49.2086700340614,12.));
#166995=CARTESIAN_POINT('Ctrl Pts',(50.6677077767432,49.1989334364996,0.));
#166996=CARTESIAN_POINT('Ctrl Pts',(50.6677077767432,49.1989334364996,12.));
#166997=CARTESIAN_POINT('Ctrl Pts',(50.6490288525656,49.189200338976,0.));
#166998=CARTESIAN_POINT('Ctrl Pts',(50.6490288525656,49.189200338976,12.));
#166999=CARTESIAN_POINT('Ctrl Pts',(50.6304043248821,49.1794708869099,0.));
#167000=CARTESIAN_POINT('Ctrl Pts',(50.6304043248821,49.1794708869099,12.));
#167001=CARTESIAN_POINT('Ctrl Pts',(50.6118343023958,49.1697452265494,0.));
#167002=CARTESIAN_POINT('Ctrl Pts',(50.6118343023958,49.1697452265494,12.));
#167003=CARTESIAN_POINT('Ctrl Pts',(50.5933188945168,49.1600235052621,0.));
#167004=CARTESIAN_POINT('Ctrl Pts',(50.5933188945168,49.1600235052621,12.));
#167005=CARTESIAN_POINT('Ctrl Pts',(50.5748582115565,49.1503058717821,0.));
#167006=CARTESIAN_POINT('Ctrl Pts',(50.5748582115565,49.1503058717821,12.));
#167007=CARTESIAN_POINT('Ctrl Pts',(50.556452365038,49.1405924766144,0.));
#167008=CARTESIAN_POINT('Ctrl Pts',(50.556452365038,49.1405924766144,12.));
#167009=CARTESIAN_POINT('Ctrl Pts',(50.5381014674791,49.1308834717615,0.));
#167010=CARTESIAN_POINT('Ctrl Pts',(50.5381014674791,49.1308834717615,12.));
#167011=CARTESIAN_POINT('Ctrl Pts',(50.5198056318089,49.1211790099795,0.));
#167012=CARTESIAN_POINT('Ctrl Pts',(50.5198056318089,49.1211790099795,12.));
#167013=CARTESIAN_POINT('Ctrl Pts',(50.501564970874,49.1114792441571,0.));
#167014=CARTESIAN_POINT('Ctrl Pts',(50.501564970874,49.1114792441571,12.));
#167015=CARTESIAN_POINT('Ctrl Pts',(50.4833795969318,49.1017843266803,0.));
#167016=CARTESIAN_POINT('Ctrl Pts',(50.4833795969318,49.1017843266803,12.));
#167017=CARTESIAN_POINT('Ctrl Pts',(50.4652496210607,49.0920944087008,0.));
#167018=CARTESIAN_POINT('Ctrl Pts',(50.4652496210607,49.0920944087008,12.));
#167019=CARTESIAN_POINT('Ctrl Pts',(50.4471751542751,49.0824096415371,0.));
#167020=CARTESIAN_POINT('Ctrl Pts',(50.4471751542751,49.0824096415371,12.));
#167021=CARTESIAN_POINT('Ctrl Pts',(50.4291563088547,49.0727301783494,0.));
#167022=CARTESIAN_POINT('Ctrl Pts',(50.4291563088547,49.0727301783494,12.));
#167023=CARTESIAN_POINT('Ctrl Pts',(50.4111931994257,49.0630561755075,0.));
#167024=CARTESIAN_POINT('Ctrl Pts',(50.4111931994257,49.0630561755075,12.));
#167025=CARTESIAN_POINT('Ctrl Pts',(50.3932859445252,49.0533877945744,0.));
#167026=CARTESIAN_POINT('Ctrl Pts',(50.3932859445252,49.0533877945744,12.));
#167027=CARTESIAN_POINT('Ctrl Pts',(50.3754346667353,49.0437252024832,0.));
#167028=CARTESIAN_POINT('Ctrl Pts',(50.3754346667353,49.0437252024832,12.));
#167029=CARTESIAN_POINT('Ctrl Pts',(50.3576394894108,49.0340685673982,0.));
#167030=CARTESIAN_POINT('Ctrl Pts',(50.3576394894108,49.0340685673982,12.));
#167031=CARTESIAN_POINT('Ctrl Pts',(50.3399005337958,49.024418055075,0.));
#167032=CARTESIAN_POINT('Ctrl Pts',(50.3399005337958,49.024418055075,12.));
#167033=CARTESIAN_POINT('Ctrl Pts',(50.3222179165119,49.0147738256942,0.));
#167034=CARTESIAN_POINT('Ctrl Pts',(50.3222179165119,49.0147738256942,12.));
#167035=CARTESIAN_POINT('Ctrl Pts',(50.3045917455424,49.0051360288044,0.));
#167036=CARTESIAN_POINT('Ctrl Pts',(50.3045917455424,49.0051360288044,12.));
#167037=CARTESIAN_POINT('Ctrl Pts',(50.2870221241054,48.9955048082081,0.));
#167038=CARTESIAN_POINT('Ctrl Pts',(50.2870221241054,48.9955048082081,12.));
#167039=CARTESIAN_POINT('Ctrl Pts',(50.2695091583511,48.9858803116689,0.));
#167040=CARTESIAN_POINT('Ctrl Pts',(50.2695091583511,48.9858803116689,12.));
#167041=CARTESIAN_POINT('Ctrl Pts',(50.252052963548,48.9762626987227,0.));
#167042=CARTESIAN_POINT('Ctrl Pts',(50.252052963548,48.9762626987227,12.));
#167043=CARTESIAN_POINT('Ctrl Pts',(50.234653671541,48.9666521500911,0.));
#167044=CARTESIAN_POINT('Ctrl Pts',(50.234653671541,48.9666521500911,12.));
#167045=CARTESIAN_POINT('Ctrl Pts',(50.2173114358325,48.9570488741167,0.));
#167046=CARTESIAN_POINT('Ctrl Pts',(50.2173114358325,48.9570488741167,12.));
#167047=CARTESIAN_POINT('Ctrl Pts',(50.2000264157797,48.9474530868733,0.));
#167048=CARTESIAN_POINT('Ctrl Pts',(50.2000264157797,48.9474530868733,12.));
#167049=CARTESIAN_POINT('Ctrl Pts',(50.1827987615602,48.9378649933055,0.));
#167050=CARTESIAN_POINT('Ctrl Pts',(50.1827987615602,48.9378649933055,12.));
#167051=CARTESIAN_POINT('Ctrl Pts',(50.1656286003997,48.9282847698294,0.));
#167052=CARTESIAN_POINT('Ctrl Pts',(50.1656286003997,48.9282847698294,12.));
#167053=CARTESIAN_POINT('Ctrl Pts',(50.1485160184657,48.9187125418099,0.));
#167054=CARTESIAN_POINT('Ctrl Pts',(50.1485160184657,48.9187125418099,12.));
#167055=CARTESIAN_POINT('Ctrl Pts',(50.1314610602569,48.90914838181,0.));
#167056=CARTESIAN_POINT('Ctrl Pts',(50.1314610602569,48.90914838181,12.));
#167057=CARTESIAN_POINT('Ctrl Pts',(50.1178632067084,48.9015035372055,0.));
#167058=CARTESIAN_POINT('Ctrl Pts',(50.1178632067084,48.9015035372055,12.));
#167059=CARTESIAN_POINT('Ctrl Pts',(50.1076907555471,48.895773555686,0.));
#167060=CARTESIAN_POINT('Ctrl Pts',(50.1076907555471,48.895773555686,12.));
#167061=CARTESIAN_POINT('Ctrl Pts',(50.1009206494272,48.8919551910366,0.));
#167062=CARTESIAN_POINT('Ctrl Pts',(50.1009206494272,48.8919551910366,12.));
#167063=CARTESIAN_POINT('Ctrl Pts',(50.0975384783635,48.8900464144686,0.));
#167064=CARTESIAN_POINT('Ctrl Pts',(50.0975384783635,48.8900464144686,12.));
#167065=CARTESIAN_POINT('',(50.0975384783635,48.8900464144686,12.));
#167066=CARTESIAN_POINT('Ctrl Pts',(50.0975384783635,48.8900464144686,12.));
#167067=CARTESIAN_POINT('Ctrl Pts',(50.1009206494272,48.8919551910366,12.));
#167068=CARTESIAN_POINT('Ctrl Pts',(50.1076907555471,48.895773555686,12.));
#167069=CARTESIAN_POINT('Ctrl Pts',(50.1178632067084,48.9015035372055,12.));
#167070=CARTESIAN_POINT('Ctrl Pts',(50.1314610602569,48.90914838181,12.));
#167071=CARTESIAN_POINT('Ctrl Pts',(50.1485160184657,48.9187125418099,12.));
#167072=CARTESIAN_POINT('Ctrl Pts',(50.1656286003997,48.9282847698294,12.));
#167073=CARTESIAN_POINT('Ctrl Pts',(50.1827987615602,48.9378649933055,12.));
#167074=CARTESIAN_POINT('Ctrl Pts',(50.2000264157797,48.9474530868733,12.));
#167075=CARTESIAN_POINT('Ctrl Pts',(50.2173114358325,48.9570488741167,12.));
#167076=CARTESIAN_POINT('Ctrl Pts',(50.234653671541,48.9666521500911,12.));
#167077=CARTESIAN_POINT('Ctrl Pts',(50.252052963548,48.9762626987227,12.));
#167078=CARTESIAN_POINT('Ctrl Pts',(50.2695091583511,48.9858803116689,12.));
#167079=CARTESIAN_POINT('Ctrl Pts',(50.2870221241054,48.9955048082081,12.));
#167080=CARTESIAN_POINT('Ctrl Pts',(50.3045917455424,49.0051360288044,12.));
#167081=CARTESIAN_POINT('Ctrl Pts',(50.3222179165119,49.0147738256942,12.));
#167082=CARTESIAN_POINT('Ctrl Pts',(50.3399005337958,49.024418055075,12.));
#167083=CARTESIAN_POINT('Ctrl Pts',(50.3576394894108,49.0340685673982,12.));
#167084=CARTESIAN_POINT('Ctrl Pts',(50.3754346667353,49.0437252024832,12.));
#167085=CARTESIAN_POINT('Ctrl Pts',(50.3932859445252,49.0533877945744,12.));
#167086=CARTESIAN_POINT('Ctrl Pts',(50.4111931994257,49.0630561755075,12.));
#167087=CARTESIAN_POINT('Ctrl Pts',(50.4291563088547,49.0727301783494,12.));
#167088=CARTESIAN_POINT('Ctrl Pts',(50.4471751542751,49.0824096415371,12.));
#167089=CARTESIAN_POINT('Ctrl Pts',(50.4652496210607,49.0920944087008,12.));
#167090=CARTESIAN_POINT('Ctrl Pts',(50.4833795969318,49.1017843266803,12.));
#167091=CARTESIAN_POINT('Ctrl Pts',(50.501564970874,49.1114792441571,12.));
#167092=CARTESIAN_POINT('Ctrl Pts',(50.5198056318089,49.1211790099795,12.));
#167093=CARTESIAN_POINT('Ctrl Pts',(50.5381014674791,49.1308834717615,12.));
#167094=CARTESIAN_POINT('Ctrl Pts',(50.556452365038,49.1405924766144,12.));
#167095=CARTESIAN_POINT('Ctrl Pts',(50.5748582115565,49.1503058717821,12.));
#167096=CARTESIAN_POINT('Ctrl Pts',(50.5933188945168,49.1600235052621,12.));
#167097=CARTESIAN_POINT('Ctrl Pts',(50.6118343023958,49.1697452265494,12.));
#167098=CARTESIAN_POINT('Ctrl Pts',(50.6304043248821,49.1794708869099,12.));
#167099=CARTESIAN_POINT('Ctrl Pts',(50.6490288525656,49.189200338976,12.));
#167100=CARTESIAN_POINT('Ctrl Pts',(50.6677077767432,49.1989334364996,12.));
#167101=CARTESIAN_POINT('Ctrl Pts',(50.6864409891895,49.2086700340614,12.));
#167102=CARTESIAN_POINT('Ctrl Pts',(50.7052283818922,49.2184099867461,12.));
#167103=CARTESIAN_POINT('Ctrl Pts',(50.7240698470679,49.228153150155,12.));
#167104=CARTESIAN_POINT('Ctrl Pts',(50.7429652772805,49.2378993805471,12.));
#167105=CARTESIAN_POINT('Ctrl Pts',(50.7619145655207,49.2476485349373,12.));
#167106=CARTESIAN_POINT('Ctrl Pts',(50.7809176052966,49.2574004712134,12.));
#167107=CARTESIAN_POINT('Ctrl Pts',(50.7999742907131,49.2671550482435,12.));
#167108=CARTESIAN_POINT('Ctrl Pts',(50.819084516434,49.2769121258164,12.));
#167109=CARTESIAN_POINT('Ctrl Pts',(50.8382481776403,49.2866715645838,12.));
#167110=CARTESIAN_POINT('Ctrl Pts',(50.8574651699873,49.2964332260039,12.));
#167111=CARTESIAN_POINT('Ctrl Pts',(50.8767353895492,49.3061969722781,12.));
#167112=CARTESIAN_POINT('Ctrl Pts',(50.8960587327848,49.3159626663109,12.));
#167113=CARTESIAN_POINT('Ctrl Pts',(50.9154350965666,49.3257301717335,12.));
#167114=CARTESIAN_POINT('Ctrl Pts',(50.9348643781924,49.3354993529159,12.));
#167115=CARTESIAN_POINT('Ctrl Pts',(50.9543464753981,49.345270074981,12.));
#167116=CARTESIAN_POINT('Ctrl Pts',(50.9738812863646,49.355042203823,12.));
#167117=CARTESIAN_POINT('Ctrl Pts',(50.9934687097188,49.3648156061058,12.));
#167118=CARTESIAN_POINT('Ctrl Pts',(51.0131086445272,49.3745901492432,12.));
#167119=CARTESIAN_POINT('Ctrl Pts',(51.0328009902858,49.3843657013852,12.));
#167120=CARTESIAN_POINT('Ctrl Pts',(51.052545646907,49.3941421314013,12.));
#167121=CARTESIAN_POINT('Ctrl Pts',(51.0723425146985,49.4039193088634,12.));
#167122=CARTESIAN_POINT('Ctrl Pts',(51.0921914943662,49.4136971040428,12.));
#167123=CARTESIAN_POINT('Ctrl Pts',(51.1120924870195,49.423475387907,12.));
#167124=CARTESIAN_POINT('Ctrl Pts',(51.1320453941702,49.4332540321178,12.));
#167125=CARTESIAN_POINT('Ctrl Pts',(51.1520501177291,49.4430329090287,12.));
#167126=CARTESIAN_POINT('Ctrl Pts',(51.1721065599973,49.4528118916832,12.));
#167127=CARTESIAN_POINT('Ctrl Pts',(51.1922146236686,49.4625908538074,12.));
#167128=CARTESIAN_POINT('Ctrl Pts',(51.2123742118287,49.4723696698021,12.));
#167129=CARTESIAN_POINT('Ctrl Pts',(51.2325852279506,49.4821482147356,12.));
#167130=CARTESIAN_POINT('Ctrl Pts',(51.2528475758846,49.4919263643362,12.));
#167131=CARTESIAN_POINT('Ctrl Pts',(51.2731611598475,49.5017039949852,12.));
#167132=CARTESIAN_POINT('Ctrl Pts',(51.2935258844289,49.5114809837122,12.));
#167133=CARTESIAN_POINT('Ctrl Pts',(51.313941654591,49.5212572081908,12.));
#167134=CARTESIAN_POINT('Ctrl Pts',(51.3344083756657,49.5310325467332,12.));
#167135=CARTESIAN_POINT('Ctrl Pts',(51.3549259533458,49.5408068782859,12.));
#167136=CARTESIAN_POINT('Ctrl Pts',(51.3754942936778,49.550580082425,12.));
#167137=CARTESIAN_POINT('Ctrl Pts',(51.396113303067,49.5603520393496,12.));
#167138=CARTESIAN_POINT('Ctrl Pts',(51.4167828882756,49.5701226298769,12.));
#167139=CARTESIAN_POINT('Ctrl Pts',(51.4375029564197,49.5798917354366,12.));
#167140=CARTESIAN_POINT('Ctrl Pts',(51.4582734149583,49.5896592380654,12.));
#167141=CARTESIAN_POINT('Ctrl Pts',(51.4790941716888,49.5994250204031,12.));
#167142=CARTESIAN_POINT('Ctrl Pts',(51.4999651347523,49.6091889656866,12.));
#167143=CARTESIAN_POINT('Ctrl Pts',(51.5208862126315,49.6189509577452,12.));
#167144=CARTESIAN_POINT('Ctrl Pts',(51.5418573141484,49.6287108809966,12.));
#167145=CARTESIAN_POINT('Ctrl Pts',(51.5628783484525,49.6384686204413,12.));
#167146=CARTESIAN_POINT('Ctrl Pts',(51.5839492250181,49.6482240616593,12.));
#167147=CARTESIAN_POINT('Ctrl Pts',(51.6050698536496,49.6579770908037,12.));
#167148=CARTESIAN_POINT('Ctrl Pts',(51.626240144479,49.6677275945967,12.));
#167149=CARTESIAN_POINT('Ctrl Pts',(51.6474600079622,49.6774754603245,12.));
#167150=CARTESIAN_POINT('Ctrl Pts',(51.6687293548682,49.6872205758336,12.));
#167151=CARTESIAN_POINT('Ctrl Pts',(51.6900480962773,49.6969628295262,12.));
#167152=CARTESIAN_POINT('Ctrl Pts',(51.7114161435869,49.7067021103553,12.));
#167153=CARTESIAN_POINT('Ctrl Pts',(51.7328334085091,49.7164383078212,12.));
#167154=CARTESIAN_POINT('Ctrl Pts',(51.754299803067,49.7261713119663,12.));
#167155=CARTESIAN_POINT('Ctrl Pts',(51.7758152395836,49.7359010133721,12.));
#167156=CARTESIAN_POINT('Ctrl Pts',(51.7973796306803,49.7456273031534,12.));
#167157=CARTESIAN_POINT('Ctrl Pts',(51.8189928892828,49.755350072955,12.));
#167158=CARTESIAN_POINT('Ctrl Pts',(51.8406549286175,49.7650692149462,12.));
#167159=CARTESIAN_POINT('Ctrl Pts',(51.8623656622097,49.7747846218182,12.));
#167160=CARTESIAN_POINT('Ctrl Pts',(51.8841250038724,49.7844961867808,12.));
#167161=CARTESIAN_POINT('Ctrl Pts',(51.9059328677059,49.7942038035576,12.));
#167162=CARTESIAN_POINT('Ctrl Pts',(51.9277891681018,49.8039073663812,12.));
#167163=CARTESIAN_POINT('Ctrl Pts',(51.9496938197418,49.8136067699896,12.));
#167164=CARTESIAN_POINT('Ctrl Pts',(51.9716467375937,49.8233019096222,12.));
#167165=CARTESIAN_POINT('Ctrl Pts',(51.9936478369008,49.8329926810172,12.));
#167166=CARTESIAN_POINT('Ctrl Pts',(52.0156970331823,49.8426789804071,12.));
#167167=CARTESIAN_POINT('Ctrl Pts',(52.0377942422376,49.8523607045149,12.));
#167168=CARTESIAN_POINT('Ctrl Pts',(52.0599393801452,49.86203775055,12.));
#167169=CARTESIAN_POINT('Ctrl Pts',(52.0821323632587,49.8717100162048,12.));
#167170=CARTESIAN_POINT('Ctrl Pts',(52.1043731081962,49.8813773996517,12.));
#167171=CARTESIAN_POINT('Ctrl Pts',(52.1266615318407,49.8910397995397,12.));
#167172=CARTESIAN_POINT('Ctrl Pts',(52.1489975513445,49.9006971149895,12.));
#167173=CARTESIAN_POINT('Ctrl Pts',(52.1713810841276,49.9103492455902,12.));
#167174=CARTESIAN_POINT('Ctrl Pts',(52.1938120478754,49.9199960913962,12.));
#167175=CARTESIAN_POINT('Ctrl Pts',(52.2162903605275,49.9296375529245,12.));
#167176=CARTESIAN_POINT('Ctrl Pts',(52.2388159402771,49.9392735311509,12.));
#167177=CARTESIAN_POINT('Ctrl Pts',(52.2613887055773,49.9489039275064,12.));
#167178=CARTESIAN_POINT('Ctrl Pts',(52.2840085751384,49.9585286438733,12.));
#167179=CARTESIAN_POINT('Ctrl Pts',(52.3066754679265,49.9681475825824,12.));
#167180=CARTESIAN_POINT('Ctrl Pts',(52.3293893031528,49.9777606464106,12.));
#167181=CARTESIAN_POINT('Ctrl Pts',(52.3521500002718,49.9873677385775,12.));
#167182=CARTESIAN_POINT('Ctrl Pts',(52.3749574789871,49.9969687627408,12.));
#167183=CARTESIAN_POINT('Ctrl Pts',(52.3978116592509,50.0065636229938,12.));
#167184=CARTESIAN_POINT('Ctrl Pts',(52.4207124612608,50.0161522238616,12.));
#167185=CARTESIAN_POINT('Ctrl Pts',(52.4436598054515,50.0257344703,12.));
#167186=CARTESIAN_POINT('Ctrl Pts',(52.4666536124913,50.0353102676921,12.));
#167187=CARTESIAN_POINT('Ctrl Pts',(52.4896938032884,50.0448795218441,12.));
#167188=CARTESIAN_POINT('Ctrl Pts',(52.5127802989896,50.0544421389818,12.));
#167189=CARTESIAN_POINT('Ctrl Pts',(52.5359130209792,50.0639980257479,12.));
#167190=CARTESIAN_POINT('Ctrl Pts',(52.5590918908702,50.0735470892007,12.));
#167191=CARTESIAN_POINT('Ctrl Pts',(52.5823168304994,50.0830892368107,12.));
#167192=CARTESIAN_POINT('Ctrl Pts',(52.6055877619348,50.0926243764578,12.));
#167193=CARTESIAN_POINT('Ctrl Pts',(52.6289046074746,50.1021524164264,12.));
#167194=CARTESIAN_POINT('Ctrl Pts',(52.652267289646,50.111673265404,12.));
#167195=CARTESIAN_POINT('Ctrl Pts',(52.6756757311978,50.1211868324781,12.));
#167196=CARTESIAN_POINT('Ctrl Pts',(52.699129855093,50.1306930271345,12.));
#167197=CARTESIAN_POINT('Ctrl Pts',(52.7226295845161,50.1401917592537,12.));
#167198=CARTESIAN_POINT('Ctrl Pts',(52.7461748428738,50.1496829391073,12.));
#167199=CARTESIAN_POINT('Ctrl Pts',(52.769765553794,50.1591664773561,12.));
#167200=CARTESIAN_POINT('Ctrl Pts',(52.7934016411205,50.1686422850488,12.));
#167201=CARTESIAN_POINT('Ctrl Pts',(52.8170830289044,50.1781102736205,12.));
#167202=CARTESIAN_POINT('Ctrl Pts',(52.8408096414093,50.1875703548884,12.));
#167203=CARTESIAN_POINT('Ctrl Pts',(52.8645814031133,50.1970224410471,12.));
#167204=CARTESIAN_POINT('Ctrl Pts',(52.8883982387068,50.2064664446663,12.));
#167205=CARTESIAN_POINT('Ctrl Pts',(52.9122600730884,50.2159022786879,12.));
#167206=CARTESIAN_POINT('Ctrl Pts',(52.9361668313542,50.2253298564241,12.));
#167207=CARTESIAN_POINT('Ctrl Pts',(52.9601184388028,50.2347490915555,12.));
#167208=CARTESIAN_POINT('Ctrl Pts',(52.9841148209402,50.2441598981286,12.));
#167209=CARTESIAN_POINT('Ctrl Pts',(53.0081559034801,50.2535621905552,12.));
#167210=CARTESIAN_POINT('Ctrl Pts',(53.0322416123406,50.2629558836111,12.));
#167211=CARTESIAN_POINT('Ctrl Pts',(53.0563718736366,50.2723408924373,12.));
#167212=CARTESIAN_POINT('Ctrl Pts',(53.0805466136798,50.2817171325358,12.));
#167213=CARTESIAN_POINT('Ctrl Pts',(53.1047657589812,50.2910845197619,12.));
#167214=CARTESIAN_POINT('Ctrl Pts',(53.1290292362485,50.300442970319,12.));
#167215=CARTESIAN_POINT('Ctrl Pts',(53.1533369723818,50.3097924007534,12.));
#167216=CARTESIAN_POINT('Ctrl Pts',(53.1776888944616,50.3191327279493,12.));
#167217=CARTESIAN_POINT('Ctrl Pts',(53.2020849297471,50.3284638691278,12.));
#167218=CARTESIAN_POINT('Ctrl Pts',(53.2265250056887,50.3377857418515,12.));
#167219=CARTESIAN_POINT('Ctrl Pts',(53.2510090499336,50.3470982640289,12.));
#167220=CARTESIAN_POINT('Ctrl Pts',(53.2755369903293,50.3564013539199,12.));
#167221=CARTESIAN_POINT('Ctrl Pts',(53.300108754923,50.365694930143,12.));
#167222=CARTESIAN_POINT('Ctrl Pts',(53.3247242719587,50.3749789116786,12.));
#167223=CARTESIAN_POINT('Ctrl Pts',(53.3493834698697,50.384253217846,12.));
#167224=CARTESIAN_POINT('Ctrl Pts',(53.3740862772681,50.3935177682837,12.));
#167225=CARTESIAN_POINT('Ctrl Pts',(53.398832622931,50.4027724829297,12.));
#167226=CARTESIAN_POINT('Ctrl Pts',(53.4236224357838,50.4120172820047,12.));
#167227=CARTESIAN_POINT('Ctrl Pts',(53.4484556448776,50.4212520859914,12.));
#167228=CARTESIAN_POINT('Ctrl Pts',(53.4733321794188,50.4304768156667,12.));
#167229=CARTESIAN_POINT('Ctrl Pts',(53.4982519688024,50.4396913921382,12.));
#167230=CARTESIAN_POINT('Ctrl Pts',(53.5232149426413,50.4488957368839,12.));
#167231=CARTESIAN_POINT('Ctrl Pts',(53.5482210307868,50.4580897717838,12.));
#167232=CARTESIAN_POINT('Ctrl Pts',(53.5732701633609,50.4672734191756,12.));
#167233=CARTESIAN_POINT('Ctrl Pts',(53.5983622707238,50.4764466018071,12.));
#167234=CARTESIAN_POINT('Ctrl Pts',(53.623497283406,50.4856092427314,12.));
#167235=CARTESIAN_POINT('Ctrl Pts',(53.6486751320436,50.4947612652149,12.));
#167236=CARTESIAN_POINT('Ctrl Pts',(53.6738957473158,50.503902592653,12.));
#167237=CARTESIAN_POINT('Ctrl Pts',(53.6991590598548,50.513033148456,12.));
#167238=CARTESIAN_POINT('Ctrl Pts',(53.7244650002374,50.522152856042,12.));
#167239=CARTESIAN_POINT('Ctrl Pts',(53.7498134991703,50.5312616390779,12.));
#167240=CARTESIAN_POINT('Ctrl Pts',(53.7752044876304,50.5403594216698,12.));
#167241=CARTESIAN_POINT('Ctrl Pts',(53.8006378970197,50.5494461285761,12.));
#167242=CARTESIAN_POINT('Ctrl Pts',(53.8261136593075,50.5585216854091,12.));
#167243=CARTESIAN_POINT('Ctrl Pts',(53.8516317071804,50.5675860188538,12.));
#167244=CARTESIAN_POINT('Ctrl Pts',(53.8771919737032,50.5766390561884,12.));
#167245=CARTESIAN_POINT('Ctrl Pts',(53.9027943919836,50.5856807248151,12.));
#167246=CARTESIAN_POINT('Ctrl Pts',(53.9284388948004,50.5947109517483,12.));
#167247=CARTESIAN_POINT('Ctrl Pts',(53.9541254143119,50.603729663214,12.));
#167248=CARTESIAN_POINT('Ctrl Pts',(53.979853881553,50.6127367839711,12.));
#167249=CARTESIAN_POINT('Ctrl Pts',(54.0056242268399,50.6217322378648,12.));
#167250=CARTESIAN_POINT('Ctrl Pts',(54.0314363806708,50.6307159490553,12.));
#167251=CARTESIAN_POINT('Ctrl Pts',(54.0572902745076,50.6396878430939,12.));
#167252=CARTESIAN_POINT('Ctrl Pts',(54.0831858415189,50.6486478479465,12.));
#167253=CARTESIAN_POINT('Ctrl Pts',(54.1091230175367,50.6575958953221,12.));
#167254=CARTESIAN_POINT('Ctrl Pts',(54.1351017412804,50.6665319209869,12.));
#167255=CARTESIAN_POINT('Ctrl Pts',(54.1574061042043,50.6741814675486,12.));
#167256=CARTESIAN_POINT('Ctrl Pts',(54.1745287898797,50.6800396668778,12.));
#167257=CARTESIAN_POINT('Ctrl Pts',(54.1864514382196,50.6841118861931,12.));
#167258=CARTESIAN_POINT('Ctrl Pts',(54.1931619277624,50.6864016965744,12.));
#167259=CARTESIAN_POINT('Ctrl Pts',(54.1946543500373,50.6869108458851,12.));
#167260=CARTESIAN_POINT('',(50.0975384783635,48.8900464144686,0.));
#167261=CARTESIAN_POINT('',(50.0975384783634,48.8900464144686,0.));
#167262=CARTESIAN_POINT('Ctrl Pts',(54.1946543500373,50.6869108458851,0.));
#167263=CARTESIAN_POINT('Ctrl Pts',(54.1931619277624,50.6864016965744,0.));
#167264=CARTESIAN_POINT('Ctrl Pts',(54.1864514382196,50.6841118861931,0.));
#167265=CARTESIAN_POINT('Ctrl Pts',(54.1745287898797,50.6800396668778,0.));
#167266=CARTESIAN_POINT('Ctrl Pts',(54.1574061042043,50.6741814675486,0.));
#167267=CARTESIAN_POINT('Ctrl Pts',(54.1351017412804,50.6665319209869,0.));
#167268=CARTESIAN_POINT('Ctrl Pts',(54.1091230175367,50.6575958953221,0.));
#167269=CARTESIAN_POINT('Ctrl Pts',(54.0831858415189,50.6486478479465,0.));
#167270=CARTESIAN_POINT('Ctrl Pts',(54.0572902745076,50.6396878430939,0.));
#167271=CARTESIAN_POINT('Ctrl Pts',(54.0314363806708,50.6307159490553,0.));
#167272=CARTESIAN_POINT('Ctrl Pts',(54.0056242268399,50.6217322378648,0.));
#167273=CARTESIAN_POINT('Ctrl Pts',(53.979853881553,50.6127367839711,0.));
#167274=CARTESIAN_POINT('Ctrl Pts',(53.9541254143119,50.603729663214,0.));
#167275=CARTESIAN_POINT('Ctrl Pts',(53.9284388948004,50.5947109517483,0.));
#167276=CARTESIAN_POINT('Ctrl Pts',(53.9027943919836,50.5856807248151,0.));
#167277=CARTESIAN_POINT('Ctrl Pts',(53.8771919737032,50.5766390561884,0.));
#167278=CARTESIAN_POINT('Ctrl Pts',(53.8516317071804,50.5675860188538,0.));
#167279=CARTESIAN_POINT('Ctrl Pts',(53.8261136593075,50.5585216854091,0.));
#167280=CARTESIAN_POINT('Ctrl Pts',(53.8006378970197,50.5494461285761,0.));
#167281=CARTESIAN_POINT('Ctrl Pts',(53.7752044876304,50.5403594216698,0.));
#167282=CARTESIAN_POINT('Ctrl Pts',(53.7498134991703,50.5312616390779,0.));
#167283=CARTESIAN_POINT('Ctrl Pts',(53.7244650002374,50.522152856042,0.));
#167284=CARTESIAN_POINT('Ctrl Pts',(53.6991590598548,50.513033148456,0.));
#167285=CARTESIAN_POINT('Ctrl Pts',(53.6738957473158,50.503902592653,0.));
#167286=CARTESIAN_POINT('Ctrl Pts',(53.6486751320436,50.4947612652149,0.));
#167287=CARTESIAN_POINT('Ctrl Pts',(53.623497283406,50.4856092427314,0.));
#167288=CARTESIAN_POINT('Ctrl Pts',(53.5983622707238,50.4764466018071,0.));
#167289=CARTESIAN_POINT('Ctrl Pts',(53.5732701633609,50.4672734191756,0.));
#167290=CARTESIAN_POINT('Ctrl Pts',(53.5482210307868,50.4580897717838,0.));
#167291=CARTESIAN_POINT('Ctrl Pts',(53.5232149426413,50.4488957368839,0.));
#167292=CARTESIAN_POINT('Ctrl Pts',(53.4982519688024,50.4396913921382,0.));
#167293=CARTESIAN_POINT('Ctrl Pts',(53.4733321794188,50.4304768156667,0.));
#167294=CARTESIAN_POINT('Ctrl Pts',(53.4484556448776,50.4212520859914,0.));
#167295=CARTESIAN_POINT('Ctrl Pts',(53.4236224357838,50.4120172820047,0.));
#167296=CARTESIAN_POINT('Ctrl Pts',(53.398832622931,50.4027724829297,0.));
#167297=CARTESIAN_POINT('Ctrl Pts',(53.3740862772681,50.3935177682837,0.));
#167298=CARTESIAN_POINT('Ctrl Pts',(53.3493834698697,50.384253217846,0.));
#167299=CARTESIAN_POINT('Ctrl Pts',(53.3247242719587,50.3749789116786,0.));
#167300=CARTESIAN_POINT('Ctrl Pts',(53.300108754923,50.365694930143,0.));
#167301=CARTESIAN_POINT('Ctrl Pts',(53.2755369903293,50.3564013539199,0.));
#167302=CARTESIAN_POINT('Ctrl Pts',(53.2510090499336,50.3470982640289,0.));
#167303=CARTESIAN_POINT('Ctrl Pts',(53.2265250056887,50.3377857418515,0.));
#167304=CARTESIAN_POINT('Ctrl Pts',(53.2020849297471,50.3284638691278,0.));
#167305=CARTESIAN_POINT('Ctrl Pts',(53.1776888944616,50.3191327279493,0.));
#167306=CARTESIAN_POINT('Ctrl Pts',(53.1533369723818,50.3097924007534,0.));
#167307=CARTESIAN_POINT('Ctrl Pts',(53.1290292362485,50.300442970319,0.));
#167308=CARTESIAN_POINT('Ctrl Pts',(53.1047657589812,50.2910845197619,0.));
#167309=CARTESIAN_POINT('Ctrl Pts',(53.0805466136798,50.2817171325358,0.));
#167310=CARTESIAN_POINT('Ctrl Pts',(53.0563718736366,50.2723408924373,0.));
#167311=CARTESIAN_POINT('Ctrl Pts',(53.0322416123406,50.2629558836111,0.));
#167312=CARTESIAN_POINT('Ctrl Pts',(53.0081559034801,50.2535621905552,0.));
#167313=CARTESIAN_POINT('Ctrl Pts',(52.9841148209402,50.2441598981286,0.));
#167314=CARTESIAN_POINT('Ctrl Pts',(52.9601184388028,50.2347490915555,0.));
#167315=CARTESIAN_POINT('Ctrl Pts',(52.9361668313542,50.2253298564241,0.));
#167316=CARTESIAN_POINT('Ctrl Pts',(52.9122600730884,50.2159022786879,0.));
#167317=CARTESIAN_POINT('Ctrl Pts',(52.8883982387068,50.2064664446663,0.));
#167318=CARTESIAN_POINT('Ctrl Pts',(52.8645814031133,50.1970224410471,0.));
#167319=CARTESIAN_POINT('Ctrl Pts',(52.8408096414093,50.1875703548884,0.));
#167320=CARTESIAN_POINT('Ctrl Pts',(52.8170830289044,50.1781102736205,0.));
#167321=CARTESIAN_POINT('Ctrl Pts',(52.7934016411205,50.1686422850488,0.));
#167322=CARTESIAN_POINT('Ctrl Pts',(52.769765553794,50.1591664773561,0.));
#167323=CARTESIAN_POINT('Ctrl Pts',(52.7461748428738,50.1496829391073,0.));
#167324=CARTESIAN_POINT('Ctrl Pts',(52.7226295845161,50.1401917592537,0.));
#167325=CARTESIAN_POINT('Ctrl Pts',(52.699129855093,50.1306930271345,0.));
#167326=CARTESIAN_POINT('Ctrl Pts',(52.6756757311978,50.1211868324781,0.));
#167327=CARTESIAN_POINT('Ctrl Pts',(52.652267289646,50.111673265404,0.));
#167328=CARTESIAN_POINT('Ctrl Pts',(52.6289046074746,50.1021524164264,0.));
#167329=CARTESIAN_POINT('Ctrl Pts',(52.6055877619348,50.0926243764578,0.));
#167330=CARTESIAN_POINT('Ctrl Pts',(52.5823168304994,50.0830892368107,0.));
#167331=CARTESIAN_POINT('Ctrl Pts',(52.5590918908702,50.0735470892007,0.));
#167332=CARTESIAN_POINT('Ctrl Pts',(52.5359130209792,50.0639980257479,0.));
#167333=CARTESIAN_POINT('Ctrl Pts',(52.5127802989896,50.0544421389818,0.));
#167334=CARTESIAN_POINT('Ctrl Pts',(52.4896938032884,50.0448795218441,0.));
#167335=CARTESIAN_POINT('Ctrl Pts',(52.4666536124913,50.0353102676921,0.));
#167336=CARTESIAN_POINT('Ctrl Pts',(52.4436598054515,50.0257344703,0.));
#167337=CARTESIAN_POINT('Ctrl Pts',(52.4207124612608,50.0161522238616,0.));
#167338=CARTESIAN_POINT('Ctrl Pts',(52.3978116592509,50.0065636229938,0.));
#167339=CARTESIAN_POINT('Ctrl Pts',(52.3749574789871,49.9969687627408,0.));
#167340=CARTESIAN_POINT('Ctrl Pts',(52.3521500002718,49.9873677385775,0.));
#167341=CARTESIAN_POINT('Ctrl Pts',(52.3293893031528,49.9777606464106,0.));
#167342=CARTESIAN_POINT('Ctrl Pts',(52.3066754679265,49.9681475825824,0.));
#167343=CARTESIAN_POINT('Ctrl Pts',(52.2840085751384,49.9585286438733,0.));
#167344=CARTESIAN_POINT('Ctrl Pts',(52.2613887055773,49.9489039275064,0.));
#167345=CARTESIAN_POINT('Ctrl Pts',(52.2388159402771,49.9392735311509,0.));
#167346=CARTESIAN_POINT('Ctrl Pts',(52.2162903605275,49.9296375529245,0.));
#167347=CARTESIAN_POINT('Ctrl Pts',(52.1938120478754,49.9199960913962,0.));
#167348=CARTESIAN_POINT('Ctrl Pts',(52.1713810841276,49.9103492455902,0.));
#167349=CARTESIAN_POINT('Ctrl Pts',(52.1489975513445,49.9006971149895,0.));
#167350=CARTESIAN_POINT('Ctrl Pts',(52.1266615318407,49.8910397995397,0.));
#167351=CARTESIAN_POINT('Ctrl Pts',(52.1043731081962,49.8813773996517,0.));
#167352=CARTESIAN_POINT('Ctrl Pts',(52.0821323632587,49.8717100162048,0.));
#167353=CARTESIAN_POINT('Ctrl Pts',(52.0599393801452,49.86203775055,0.));
#167354=CARTESIAN_POINT('Ctrl Pts',(52.0377942422376,49.8523607045149,0.));
#167355=CARTESIAN_POINT('Ctrl Pts',(52.0156970331823,49.8426789804071,0.));
#167356=CARTESIAN_POINT('Ctrl Pts',(51.9936478369008,49.8329926810172,0.));
#167357=CARTESIAN_POINT('Ctrl Pts',(51.9716467375937,49.8233019096222,0.));
#167358=CARTESIAN_POINT('Ctrl Pts',(51.9496938197418,49.8136067699896,0.));
#167359=CARTESIAN_POINT('Ctrl Pts',(51.9277891681018,49.8039073663812,0.));
#167360=CARTESIAN_POINT('Ctrl Pts',(51.9059328677059,49.7942038035576,0.));
#167361=CARTESIAN_POINT('Ctrl Pts',(51.8841250038724,49.7844961867808,0.));
#167362=CARTESIAN_POINT('Ctrl Pts',(51.8623656622097,49.7747846218182,0.));
#167363=CARTESIAN_POINT('Ctrl Pts',(51.8406549286175,49.7650692149462,0.));
#167364=CARTESIAN_POINT('Ctrl Pts',(51.8189928892828,49.755350072955,0.));
#167365=CARTESIAN_POINT('Ctrl Pts',(51.7973796306803,49.7456273031534,0.));
#167366=CARTESIAN_POINT('Ctrl Pts',(51.7758152395836,49.7359010133721,0.));
#167367=CARTESIAN_POINT('Ctrl Pts',(51.754299803067,49.7261713119663,0.));
#167368=CARTESIAN_POINT('Ctrl Pts',(51.7328334085091,49.7164383078212,0.));
#167369=CARTESIAN_POINT('Ctrl Pts',(51.7114161435869,49.7067021103553,0.));
#167370=CARTESIAN_POINT('Ctrl Pts',(51.6900480962773,49.6969628295262,0.));
#167371=CARTESIAN_POINT('Ctrl Pts',(51.6687293548682,49.6872205758336,0.));
#167372=CARTESIAN_POINT('Ctrl Pts',(51.6474600079622,49.6774754603245,0.));
#167373=CARTESIAN_POINT('Ctrl Pts',(51.626240144479,49.6677275945967,0.));
#167374=CARTESIAN_POINT('Ctrl Pts',(51.6050698536496,49.6579770908037,0.));
#167375=CARTESIAN_POINT('Ctrl Pts',(51.5839492250181,49.6482240616593,0.));
#167376=CARTESIAN_POINT('Ctrl Pts',(51.5628783484525,49.6384686204413,0.));
#167377=CARTESIAN_POINT('Ctrl Pts',(51.5418573141484,49.6287108809966,0.));
#167378=CARTESIAN_POINT('Ctrl Pts',(51.5208862126315,49.6189509577452,0.));
#167379=CARTESIAN_POINT('Ctrl Pts',(51.4999651347523,49.6091889656866,0.));
#167380=CARTESIAN_POINT('Ctrl Pts',(51.4790941716888,49.5994250204031,0.));
#167381=CARTESIAN_POINT('Ctrl Pts',(51.4582734149583,49.5896592380654,0.));
#167382=CARTESIAN_POINT('Ctrl Pts',(51.4375029564197,49.5798917354366,0.));
#167383=CARTESIAN_POINT('Ctrl Pts',(51.4167828882756,49.5701226298769,0.));
#167384=CARTESIAN_POINT('Ctrl Pts',(51.396113303067,49.5603520393496,0.));
#167385=CARTESIAN_POINT('Ctrl Pts',(51.3754942936778,49.550580082425,0.));
#167386=CARTESIAN_POINT('Ctrl Pts',(51.3549259533458,49.5408068782859,0.));
#167387=CARTESIAN_POINT('Ctrl Pts',(51.3344083756657,49.5310325467332,0.));
#167388=CARTESIAN_POINT('Ctrl Pts',(51.313941654591,49.5212572081908,0.));
#167389=CARTESIAN_POINT('Ctrl Pts',(51.2935258844289,49.5114809837122,0.));
#167390=CARTESIAN_POINT('Ctrl Pts',(51.2731611598475,49.5017039949852,0.));
#167391=CARTESIAN_POINT('Ctrl Pts',(51.2528475758846,49.4919263643362,0.));
#167392=CARTESIAN_POINT('Ctrl Pts',(51.2325852279506,49.4821482147356,0.));
#167393=CARTESIAN_POINT('Ctrl Pts',(51.2123742118287,49.4723696698021,0.));
#167394=CARTESIAN_POINT('Ctrl Pts',(51.1922146236686,49.4625908538074,0.));
#167395=CARTESIAN_POINT('Ctrl Pts',(51.1721065599973,49.4528118916832,0.));
#167396=CARTESIAN_POINT('Ctrl Pts',(51.1520501177291,49.4430329090287,0.));
#167397=CARTESIAN_POINT('Ctrl Pts',(51.1320453941702,49.4332540321178,0.));
#167398=CARTESIAN_POINT('Ctrl Pts',(51.1120924870195,49.423475387907,0.));
#167399=CARTESIAN_POINT('Ctrl Pts',(51.0921914943662,49.4136971040428,0.));
#167400=CARTESIAN_POINT('Ctrl Pts',(51.0723425146985,49.4039193088634,0.));
#167401=CARTESIAN_POINT('Ctrl Pts',(51.052545646907,49.3941421314013,0.));
#167402=CARTESIAN_POINT('Ctrl Pts',(51.0328009902858,49.3843657013852,0.));
#167403=CARTESIAN_POINT('Ctrl Pts',(51.0131086445272,49.3745901492432,0.));
#167404=CARTESIAN_POINT('Ctrl Pts',(50.9934687097188,49.3648156061058,0.));
#167405=CARTESIAN_POINT('Ctrl Pts',(50.9738812863646,49.355042203823,0.));
#167406=CARTESIAN_POINT('Ctrl Pts',(50.9543464753981,49.345270074981,0.));
#167407=CARTESIAN_POINT('Ctrl Pts',(50.9348643781924,49.3354993529159,0.));
#167408=CARTESIAN_POINT('Ctrl Pts',(50.9154350965666,49.3257301717335,0.));
#167409=CARTESIAN_POINT('Ctrl Pts',(50.8960587327848,49.3159626663109,0.));
#167410=CARTESIAN_POINT('Ctrl Pts',(50.8767353895492,49.3061969722781,0.));
#167411=CARTESIAN_POINT('Ctrl Pts',(50.8574651699873,49.2964332260039,0.));
#167412=CARTESIAN_POINT('Ctrl Pts',(50.8382481776403,49.2866715645838,0.));
#167413=CARTESIAN_POINT('Ctrl Pts',(50.819084516434,49.2769121258164,0.));
#167414=CARTESIAN_POINT('Ctrl Pts',(50.7999742907131,49.2671550482435,0.));
#167415=CARTESIAN_POINT('Ctrl Pts',(50.7809176052966,49.2574004712134,0.));
#167416=CARTESIAN_POINT('Ctrl Pts',(50.7619145655207,49.2476485349373,0.));
#167417=CARTESIAN_POINT('Ctrl Pts',(50.7429652772805,49.2378993805471,0.));
#167418=CARTESIAN_POINT('Ctrl Pts',(50.7240698470679,49.228153150155,0.));
#167419=CARTESIAN_POINT('Ctrl Pts',(50.7052283818922,49.2184099867461,0.));
#167420=CARTESIAN_POINT('Ctrl Pts',(50.6864409891895,49.2086700340614,0.));
#167421=CARTESIAN_POINT('Ctrl Pts',(50.6677077767432,49.1989334364996,0.));
#167422=CARTESIAN_POINT('Ctrl Pts',(50.6490288525656,49.189200338976,0.));
#167423=CARTESIAN_POINT('Ctrl Pts',(50.6304043248821,49.1794708869099,0.));
#167424=CARTESIAN_POINT('Ctrl Pts',(50.6118343023958,49.1697452265494,0.));
#167425=CARTESIAN_POINT('Ctrl Pts',(50.5933188945168,49.1600235052621,0.));
#167426=CARTESIAN_POINT('Ctrl Pts',(50.5748582115565,49.1503058717821,0.));
#167427=CARTESIAN_POINT('Ctrl Pts',(50.556452365038,49.1405924766144,0.));
#167428=CARTESIAN_POINT('Ctrl Pts',(50.5381014674791,49.1308834717615,0.));
#167429=CARTESIAN_POINT('Ctrl Pts',(50.5198056318089,49.1211790099795,0.));
#167430=CARTESIAN_POINT('Ctrl Pts',(50.501564970874,49.1114792441571,0.));
#167431=CARTESIAN_POINT('Ctrl Pts',(50.4833795969318,49.1017843266803,0.));
#167432=CARTESIAN_POINT('Ctrl Pts',(50.4652496210607,49.0920944087008,0.));
#167433=CARTESIAN_POINT('Ctrl Pts',(50.4471751542751,49.0824096415371,0.));
#167434=CARTESIAN_POINT('Ctrl Pts',(50.4291563088547,49.0727301783494,0.));
#167435=CARTESIAN_POINT('Ctrl Pts',(50.4111931994257,49.0630561755075,0.));
#167436=CARTESIAN_POINT('Ctrl Pts',(50.3932859445252,49.0533877945744,0.));
#167437=CARTESIAN_POINT('Ctrl Pts',(50.3754346667353,49.0437252024832,0.));
#167438=CARTESIAN_POINT('Ctrl Pts',(50.3576394894108,49.0340685673982,0.));
#167439=CARTESIAN_POINT('Ctrl Pts',(50.3399005337958,49.024418055075,0.));
#167440=CARTESIAN_POINT('Ctrl Pts',(50.3222179165119,49.0147738256942,0.));
#167441=CARTESIAN_POINT('Ctrl Pts',(50.3045917455424,49.0051360288044,0.));
#167442=CARTESIAN_POINT('Ctrl Pts',(50.2870221241054,48.9955048082081,0.));
#167443=CARTESIAN_POINT('Ctrl Pts',(50.2695091583511,48.9858803116689,0.));
#167444=CARTESIAN_POINT('Ctrl Pts',(50.252052963548,48.9762626987227,0.));
#167445=CARTESIAN_POINT('Ctrl Pts',(50.234653671541,48.9666521500911,0.));
#167446=CARTESIAN_POINT('Ctrl Pts',(50.2173114358325,48.9570488741167,0.));
#167447=CARTESIAN_POINT('Ctrl Pts',(50.2000264157797,48.9474530868733,0.));
#167448=CARTESIAN_POINT('Ctrl Pts',(50.1827987615602,48.9378649933055,0.));
#167449=CARTESIAN_POINT('Ctrl Pts',(50.1656286003997,48.9282847698294,0.));
#167450=CARTESIAN_POINT('Ctrl Pts',(50.1485160184657,48.9187125418099,0.));
#167451=CARTESIAN_POINT('Ctrl Pts',(50.1314610602569,48.90914838181,0.));
#167452=CARTESIAN_POINT('Ctrl Pts',(50.1178632067084,48.9015035372055,0.));
#167453=CARTESIAN_POINT('Ctrl Pts',(50.1076907555471,48.895773555686,0.));
#167454=CARTESIAN_POINT('Ctrl Pts',(50.1009206494272,48.8919551910366,0.));
#167455=CARTESIAN_POINT('Ctrl Pts',(50.0975384783635,48.8900464144686,0.));
#167456=CARTESIAN_POINT('Ctrl Pts',(58.722407829904,45.8467972562798,0.));
#167457=CARTESIAN_POINT('Ctrl Pts',(58.722407829904,45.8467972562798,12.));
#167458=CARTESIAN_POINT('Ctrl Pts',(58.7169606500268,45.8455162977427,0.));
#167459=CARTESIAN_POINT('Ctrl Pts',(58.7169606500268,45.8455162977427,12.));
#167460=CARTESIAN_POINT('Ctrl Pts',(58.7060702401686,45.8429527488786,0.));
#167461=CARTESIAN_POINT('Ctrl Pts',(58.7060702401686,45.8429527488786,12.));
#167462=CARTESIAN_POINT('Ctrl Pts',(58.6897464750699,45.8391025302132,0.));
#167463=CARTESIAN_POINT('Ctrl Pts',(58.6897464750699,45.8391025302132,12.));
#167464=CARTESIAN_POINT('Ctrl Pts',(58.6680051552762,45.8339591141834,0.));
#167465=CARTESIAN_POINT('Ctrl Pts',(58.6680051552762,45.8339591141834,12.));
#167466=CARTESIAN_POINT('Ctrl Pts',(58.6408680154016,45.827513526425,0.));
#167467=CARTESIAN_POINT('Ctrl Pts',(58.6408680154016,45.827513526425,12.));
#167468=CARTESIAN_POINT('Ctrl Pts',(58.6137704035871,45.8210516273781,0.));
#167469=CARTESIAN_POINT('Ctrl Pts',(58.6137704035871,45.8210516273781,12.));
#167470=CARTESIAN_POINT('Ctrl Pts',(58.5867123491018,45.814573433072,0.));
#167471=CARTESIAN_POINT('Ctrl Pts',(58.5867123491018,45.814573433072,12.));
#167472=CARTESIAN_POINT('Ctrl Pts',(58.5596938940195,45.8080789725084,0.));
#167473=CARTESIAN_POINT('Ctrl Pts',(58.5596938940195,45.8080789725084,12.));
#167474=CARTESIAN_POINT('Ctrl Pts',(58.5327150960661,45.8015682926025,0.));
#167475=CARTESIAN_POINT('Ctrl Pts',(58.5327150960661,45.8015682926025,12.));
#167476=CARTESIAN_POINT('Ctrl Pts',(58.5057760270184,45.7950414569268,0.));
#167477=CARTESIAN_POINT('Ctrl Pts',(58.5057760270184,45.7950414569268,12.));
#167478=CARTESIAN_POINT('Ctrl Pts',(58.4788767676949,45.7884985397018,0.));
#167479=CARTESIAN_POINT('Ctrl Pts',(58.4788767676949,45.7884985397018,12.));
#167480=CARTESIAN_POINT('Ctrl Pts',(58.4520174038764,45.7819396211009,0.));
#167481=CARTESIAN_POINT('Ctrl Pts',(58.4520174038764,45.7819396211009,12.));
#167482=CARTESIAN_POINT('Ctrl Pts',(58.425198021955,45.7753647821513,0.));
#167483=CARTESIAN_POINT('Ctrl Pts',(58.425198021955,45.7753647821513,12.));
#167484=CARTESIAN_POINT('Ctrl Pts',(58.3984187044245,45.7687740994957,0.));
#167485=CARTESIAN_POINT('Ctrl Pts',(58.3984187044245,45.7687740994957,12.));
#167486=CARTESIAN_POINT('Ctrl Pts',(58.3716795262353,45.7621676411434,0.));
#167487=CARTESIAN_POINT('Ctrl Pts',(58.3716795262353,45.7621676411434,12.));
#167488=CARTESIAN_POINT('Ctrl Pts',(58.3449805573423,45.755545469402,0.));
#167489=CARTESIAN_POINT('Ctrl Pts',(58.3449805573423,45.755545469402,12.));
#167490=CARTESIAN_POINT('Ctrl Pts',(58.3183218645316,45.7489076429763,0.));
#167491=CARTESIAN_POINT('Ctrl Pts',(58.3183218645316,45.7489076429763,12.));
#167492=CARTESIAN_POINT('Ctrl Pts',(58.291703513584,45.742254219463,0.));
#167493=CARTESIAN_POINT('Ctrl Pts',(58.291703513584,45.742254219463,12.));
#167494=CARTESIAN_POINT('Ctrl Pts',(58.2651255711453,45.7355852575107,0.));
#167495=CARTESIAN_POINT('Ctrl Pts',(58.2651255711453,45.7355852575107,12.));
#167496=CARTESIAN_POINT('Ctrl Pts',(58.2385881070913,45.7289008195579,0.));
#167497=CARTESIAN_POINT('Ctrl Pts',(58.2385881070913,45.7289008195579,12.));
#167498=CARTESIAN_POINT('Ctrl Pts',(58.2120911942772,45.7222009715397,0.));
#167499=CARTESIAN_POINT('Ctrl Pts',(58.2120911942772,45.7222009715397,12.));
#167500=CARTESIAN_POINT('Ctrl Pts',(58.185634907469,45.7154857816483,0.));
#167501=CARTESIAN_POINT('Ctrl Pts',(58.185634907469,45.7154857816483,12.));
#167502=CARTESIAN_POINT('Ctrl Pts',(58.1592193225137,45.7087553193771,0.));
#167503=CARTESIAN_POINT('Ctrl Pts',(58.1592193225137,45.7087553193771,12.));
#167504=CARTESIAN_POINT('Ctrl Pts',(58.1328445154676,45.702009654518,0.));
#167505=CARTESIAN_POINT('Ctrl Pts',(58.1328445154676,45.702009654518,12.));
#167506=CARTESIAN_POINT('Ctrl Pts',(58.1065105615907,45.695248856015,0.));
#167507=CARTESIAN_POINT('Ctrl Pts',(58.1065105615907,45.695248856015,12.));
#167508=CARTESIAN_POINT('Ctrl Pts',(58.0802175348966,45.6884729914485,0.));
#167509=CARTESIAN_POINT('Ctrl Pts',(58.0802175348966,45.6884729914485,12.));
#167510=CARTESIAN_POINT('Ctrl Pts',(58.0539655087117,45.6816821276678,0.));
#167511=CARTESIAN_POINT('Ctrl Pts',(58.0539655087117,45.6816821276678,12.));
#167512=CARTESIAN_POINT('Ctrl Pts',(58.0277545560012,45.6748763311643,0.));
#167513=CARTESIAN_POINT('Ctrl Pts',(58.0277545560012,45.6748763311643,12.));
#167514=CARTESIAN_POINT('Ctrl Pts',(58.0015847497837,45.6680556685493,0.));
#167515=CARTESIAN_POINT('Ctrl Pts',(58.0015847497837,45.6680556685493,12.));
#167516=CARTESIAN_POINT('Ctrl Pts',(57.9754561635061,45.661220206992,0.));
#167517=CARTESIAN_POINT('Ctrl Pts',(57.9754561635061,45.661220206992,12.));
#167518=CARTESIAN_POINT('Ctrl Pts',(57.9493688714237,45.6543700146679,0.));
#167519=CARTESIAN_POINT('Ctrl Pts',(57.9493688714237,45.6543700146679,12.));
#167520=CARTESIAN_POINT('Ctrl Pts',(57.9233229484311,45.6475051605535,0.));
#167521=CARTESIAN_POINT('Ctrl Pts',(57.9233229484311,45.6475051605535,12.));
#167522=CARTESIAN_POINT('Ctrl Pts',(57.8973184699034,45.6406257142382,0.));
#167523=CARTESIAN_POINT('Ctrl Pts',(57.8973184699034,45.6406257142382,12.));
#167524=CARTESIAN_POINT('Ctrl Pts',(57.8713555115232,45.6337317457252,0.));
#167525=CARTESIAN_POINT('Ctrl Pts',(57.8713555115232,45.6337317457252,12.));
#167526=CARTESIAN_POINT('Ctrl Pts',(57.8454341491238,45.6268233252544,0.));
#167527=CARTESIAN_POINT('Ctrl Pts',(57.8454341491238,45.6268233252544,12.));
#167528=CARTESIAN_POINT('Ctrl Pts',(57.8195544584845,45.6199005230784,0.));
#167529=CARTESIAN_POINT('Ctrl Pts',(57.8195544584845,45.6199005230784,12.));
#167530=CARTESIAN_POINT('Ctrl Pts',(57.7937165153387,45.6129634094683,0.));
#167531=CARTESIAN_POINT('Ctrl Pts',(57.7937165153387,45.6129634094683,12.));
#167532=CARTESIAN_POINT('Ctrl Pts',(57.7679203954742,45.6060120548205,0.));
#167533=CARTESIAN_POINT('Ctrl Pts',(57.7679203954742,45.6060120548205,12.));
#167534=CARTESIAN_POINT('Ctrl Pts',(57.7421661748026,45.5990465297344,0.));
#167535=CARTESIAN_POINT('Ctrl Pts',(57.7421661748026,45.5990465297344,12.));
#167536=CARTESIAN_POINT('Ctrl Pts',(57.7164539294314,45.5920669050986,0.));
#167537=CARTESIAN_POINT('Ctrl Pts',(57.7164539294314,45.5920669050986,12.));
#167538=CARTESIAN_POINT('Ctrl Pts',(57.6907837357417,45.5850732521896,0.));
#167539=CARTESIAN_POINT('Ctrl Pts',(57.6907837357417,45.5850732521896,12.));
#167540=CARTESIAN_POINT('Ctrl Pts',(57.6651556704237,45.5780656427163,0.));
#167541=CARTESIAN_POINT('Ctrl Pts',(57.6651556704237,45.5780656427163,12.));
#167542=CARTESIAN_POINT('Ctrl Pts',(57.6395698104404,45.5710441487674,0.));
#167543=CARTESIAN_POINT('Ctrl Pts',(57.6395698104404,45.5710441487674,12.));
#167544=CARTESIAN_POINT('Ctrl Pts',(57.614026233004,45.5640088427813,0.));
#167545=CARTESIAN_POINT('Ctrl Pts',(57.614026233004,45.5640088427813,12.));
#167546=CARTESIAN_POINT('Ctrl Pts',(57.5885250155433,45.5569597975096,0.));
#167547=CARTESIAN_POINT('Ctrl Pts',(57.5885250155433,45.5569597975096,12.));
#167548=CARTESIAN_POINT('Ctrl Pts',(57.563066235668,45.5498970859835,0.));
#167549=CARTESIAN_POINT('Ctrl Pts',(57.563066235668,45.5498970859835,12.));
#167550=CARTESIAN_POINT('Ctrl Pts',(57.537649971135,45.542820781484,0.));
#167551=CARTESIAN_POINT('Ctrl Pts',(57.537649971135,45.542820781484,12.));
#167552=CARTESIAN_POINT('Ctrl Pts',(57.5122762998745,45.5357309575611,0.));
#167553=CARTESIAN_POINT('Ctrl Pts',(57.5122762998745,45.5357309575611,12.));
#167554=CARTESIAN_POINT('Ctrl Pts',(57.4869453000063,45.5286276880485,0.));
#167555=CARTESIAN_POINT('Ctrl Pts',(57.4869453000063,45.5286276880485,12.));
#167556=CARTESIAN_POINT('Ctrl Pts',(57.4616570498568,45.5215110470825,0.));
#167557=CARTESIAN_POINT('Ctrl Pts',(57.4616570498568,45.5215110470825,12.));
#167558=CARTESIAN_POINT('Ctrl Pts',(57.4364116279702,45.5143811091205,0.));
#167559=CARTESIAN_POINT('Ctrl Pts',(57.4364116279702,45.5143811091205,12.));
#167560=CARTESIAN_POINT('Ctrl Pts',(57.4112091131183,45.5072379489631,0.));
#167561=CARTESIAN_POINT('Ctrl Pts',(57.4112091131183,45.5072379489631,12.));
#167562=CARTESIAN_POINT('Ctrl Pts',(57.3860495843033,45.500081641751,0.));
#167563=CARTESIAN_POINT('Ctrl Pts',(57.3860495843033,45.500081641751,12.));
#167564=CARTESIAN_POINT('Ctrl Pts',(57.3609331207574,45.4929122629572,0.));
#167565=CARTESIAN_POINT('Ctrl Pts',(57.3609331207574,45.4929122629572,12.));
#167566=CARTESIAN_POINT('Ctrl Pts',(57.3358598019389,45.4857298883824,0.));
#167567=CARTESIAN_POINT('Ctrl Pts',(57.3358598019389,45.4857298883824,12.));
#167568=CARTESIAN_POINT('Ctrl Pts',(57.3108297075265,45.4785345941507,0.));
#167569=CARTESIAN_POINT('Ctrl Pts',(57.3108297075265,45.4785345941507,12.));
#167570=CARTESIAN_POINT('Ctrl Pts',(57.2858429174062,45.4713264567063,0.));
#167571=CARTESIAN_POINT('Ctrl Pts',(57.2858429174062,45.4713264567063,12.));
#167572=CARTESIAN_POINT('Ctrl Pts',(57.2608995116733,45.4641055528141,0.));
#167573=CARTESIAN_POINT('Ctrl Pts',(57.2608995116733,45.4641055528141,12.));
#167574=CARTESIAN_POINT('Ctrl Pts',(57.2359995706447,45.4568719595642,0.));
#167575=CARTESIAN_POINT('Ctrl Pts',(57.2359995706447,45.4568719595642,12.));
#167576=CARTESIAN_POINT('Ctrl Pts',(57.2111431748631,45.4496257543759,0.));
#167577=CARTESIAN_POINT('Ctrl Pts',(57.2111431748631,45.4496257543759,12.));
#167578=CARTESIAN_POINT('Ctrl Pts',(57.186330405101,45.4423670150034,0.));
#167579=CARTESIAN_POINT('Ctrl Pts',(57.186330405101,45.4423670150034,12.));
#167580=CARTESIAN_POINT('Ctrl Pts',(57.1615613423584,45.4350958195434,0.));
#167581=CARTESIAN_POINT('Ctrl Pts',(57.1615613423584,45.4350958195434,12.));
#167582=CARTESIAN_POINT('Ctrl Pts',(57.136836067863,45.4278122464389,0.));
#167583=CARTESIAN_POINT('Ctrl Pts',(57.136836067863,45.4278122464389,12.));
#167584=CARTESIAN_POINT('Ctrl Pts',(57.112154663078,45.4205163744782,0.));
#167585=CARTESIAN_POINT('Ctrl Pts',(57.112154663078,45.4205163744782,12.));
#167586=CARTESIAN_POINT('Ctrl Pts',(57.0875172097051,45.4132082827948,0.));
#167587=CARTESIAN_POINT('Ctrl Pts',(57.0875172097051,45.4132082827948,12.));
#167588=CARTESIAN_POINT('Ctrl Pts',(57.0629237896848,45.4058880508693,0.));
#167589=CARTESIAN_POINT('Ctrl Pts',(57.0629237896848,45.4058880508693,12.));
#167590=CARTESIAN_POINT('Ctrl Pts',(57.0383744851913,45.3985557585311,0.));
#167591=CARTESIAN_POINT('Ctrl Pts',(57.0383744851913,45.3985557585311,12.));
#167592=CARTESIAN_POINT('Ctrl Pts',(57.0138693786278,45.3912114859616,0.));
#167593=CARTESIAN_POINT('Ctrl Pts',(57.0138693786278,45.3912114859616,12.));
#167594=CARTESIAN_POINT('Ctrl Pts',(56.9894085526373,45.3838553136948,0.));
#167595=CARTESIAN_POINT('Ctrl Pts',(56.9894085526373,45.3838553136948,12.));
#167596=CARTESIAN_POINT('Ctrl Pts',(56.9649920901073,45.3764873226196,0.));
#167597=CARTESIAN_POINT('Ctrl Pts',(56.9649920901073,45.3764873226196,12.));
#167598=CARTESIAN_POINT('Ctrl Pts',(56.9406200741714,45.3691075939827,0.));
#167599=CARTESIAN_POINT('Ctrl Pts',(56.9406200741714,45.3691075939827,12.));
#167600=CARTESIAN_POINT('Ctrl Pts',(56.9162925882085,45.3617162093923,0.));
#167601=CARTESIAN_POINT('Ctrl Pts',(56.9162925882085,45.3617162093923,12.));
#167602=CARTESIAN_POINT('Ctrl Pts',(56.8920097158377,45.3543132508239,0.));
#167603=CARTESIAN_POINT('Ctrl Pts',(56.8920097158377,45.3543132508239,12.));
#167604=CARTESIAN_POINT('Ctrl Pts',(56.8677715409268,45.3468988006203,0.));
#167605=CARTESIAN_POINT('Ctrl Pts',(56.8677715409268,45.3468988006203,12.));
#167606=CARTESIAN_POINT('Ctrl Pts',(56.8435781475981,45.3394729414931,0.));
#167607=CARTESIAN_POINT('Ctrl Pts',(56.8435781475981,45.3394729414931,12.));
#167608=CARTESIAN_POINT('Ctrl Pts',(56.8194296202291,45.332035756524,0.));
#167609=CARTESIAN_POINT('Ctrl Pts',(56.8194296202291,45.332035756524,12.));
#167610=CARTESIAN_POINT('Ctrl Pts',(56.7953260434524,45.3245873291684,0.));
#167611=CARTESIAN_POINT('Ctrl Pts',(56.7953260434524,45.3245873291684,12.));
#167612=CARTESIAN_POINT('Ctrl Pts',(56.7712675021491,45.31712774326,0.));
#167613=CARTESIAN_POINT('Ctrl Pts',(56.7712675021491,45.31712774326,12.));
#167614=CARTESIAN_POINT('Ctrl Pts',(56.7472540814553,45.3096570830118,0.));
#167615=CARTESIAN_POINT('Ctrl Pts',(56.7472540814553,45.3096570830118,12.));
#167616=CARTESIAN_POINT('Ctrl Pts',(56.7232858667709,45.3021754330179,0.));
#167617=CARTESIAN_POINT('Ctrl Pts',(56.7232858667709,45.3021754330179,12.));
#167618=CARTESIAN_POINT('Ctrl Pts',(56.69936294376,45.2946828782559,0.));
#167619=CARTESIAN_POINT('Ctrl Pts',(56.69936294376,45.2946828782559,12.));
#167620=CARTESIAN_POINT('Ctrl Pts',(56.6754853983528,45.2871795040906,0.));
#167621=CARTESIAN_POINT('Ctrl Pts',(56.6754853983528,45.2871795040906,12.));
#167622=CARTESIAN_POINT('Ctrl Pts',(56.6516533167384,45.2796653962785,0.));
#167623=CARTESIAN_POINT('Ctrl Pts',(56.6516533167384,45.2796653962785,12.));
#167624=CARTESIAN_POINT('Ctrl Pts',(56.6278667853702,45.2721406409695,0.));
#167625=CARTESIAN_POINT('Ctrl Pts',(56.6278667853702,45.2721406409695,12.));
#167626=CARTESIAN_POINT('Ctrl Pts',(56.6041258909741,45.2646053247087,0.));
#167627=CARTESIAN_POINT('Ctrl Pts',(56.6041258909741,45.2646053247087,12.));
#167628=CARTESIAN_POINT('Ctrl Pts',(56.5804307205505,45.257059534438,0.));
#167629=CARTESIAN_POINT('Ctrl Pts',(56.5804307205505,45.257059534438,12.));
#167630=CARTESIAN_POINT('Ctrl Pts',(56.5567813613756,45.2495033575,0.));
#167631=CARTESIAN_POINT('Ctrl Pts',(56.5567813613756,45.2495033575,12.));
#167632=CARTESIAN_POINT('Ctrl Pts',(56.5331779009958,45.2419368816429,0.));
#167633=CARTESIAN_POINT('Ctrl Pts',(56.5331779009958,45.2419368816429,12.));
#167634=CARTESIAN_POINT('Ctrl Pts',(56.5096204272306,45.2343601950228,0.));
#167635=CARTESIAN_POINT('Ctrl Pts',(56.5096204272306,45.2343601950228,12.));
#167636=CARTESIAN_POINT('Ctrl Pts',(56.4861090281823,45.2267733862049,0.));
#167637=CARTESIAN_POINT('Ctrl Pts',(56.4861090281823,45.2267733862049,12.));
#167638=CARTESIAN_POINT('Ctrl Pts',(56.4626437922386,45.2191765441667,0.));
#167639=CARTESIAN_POINT('Ctrl Pts',(56.4626437922386,45.2191765441667,12.));
#167640=CARTESIAN_POINT('Ctrl Pts',(56.4392248080732,45.2115697583001,0.));
#167641=CARTESIAN_POINT('Ctrl Pts',(56.4392248080732,45.2115697583001,12.));
#167642=CARTESIAN_POINT('Ctrl Pts',(56.4158521646411,45.2039531184172,0.));
#167643=CARTESIAN_POINT('Ctrl Pts',(56.4158521646411,45.2039531184172,12.));
#167644=CARTESIAN_POINT('Ctrl Pts',(56.3925259511806,45.1963267147529,0.));
#167645=CARTESIAN_POINT('Ctrl Pts',(56.3925259511806,45.1963267147529,12.));
#167646=CARTESIAN_POINT('Ctrl Pts',(56.3692462572231,45.1886906379667,0.));
#167647=CARTESIAN_POINT('Ctrl Pts',(56.3692462572231,45.1886906379667,12.));
#167648=CARTESIAN_POINT('Ctrl Pts',(56.3460131725964,45.1810449791453,0.));
#167649=CARTESIAN_POINT('Ctrl Pts',(56.3460131725964,45.1810449791453,12.));
#167650=CARTESIAN_POINT('Ctrl Pts',(56.3228267874264,45.1733898298061,0.));
#167651=CARTESIAN_POINT('Ctrl Pts',(56.3228267874264,45.1733898298061,12.));
#167652=CARTESIAN_POINT('Ctrl Pts',(56.2996871921316,45.1657252819013,0.));
#167653=CARTESIAN_POINT('Ctrl Pts',(56.2996871921316,45.1657252819013,12.));
#167654=CARTESIAN_POINT('Ctrl Pts',(56.2765944774245,45.1580514278223,0.));
#167655=CARTESIAN_POINT('Ctrl Pts',(56.2765944774245,45.1580514278223,12.));
#167656=CARTESIAN_POINT('Ctrl Pts',(56.2535487343221,45.1503683604005,0.));
#167657=CARTESIAN_POINT('Ctrl Pts',(56.2535487343221,45.1503683604005,12.));
#167658=CARTESIAN_POINT('Ctrl Pts',(56.2305500541489,45.1426761729105,0.));
#167659=CARTESIAN_POINT('Ctrl Pts',(56.2305500541489,45.1426761729105,12.));
#167660=CARTESIAN_POINT('Ctrl Pts',(56.2075985285393,45.1349749590738,0.));
#167661=CARTESIAN_POINT('Ctrl Pts',(56.2075985285393,45.1349749590738,12.));
#167662=CARTESIAN_POINT('Ctrl Pts',(56.1846942494325,45.127264813063,0.));
#167663=CARTESIAN_POINT('Ctrl Pts',(56.1846942494325,45.127264813063,12.));
#167664=CARTESIAN_POINT('Ctrl Pts',(56.1618373090732,45.1195458295063,0.));
#167665=CARTESIAN_POINT('Ctrl Pts',(56.1618373090732,45.1195458295063,12.));
#167666=CARTESIAN_POINT('Ctrl Pts',(56.1390278000226,45.1118181034888,0.));
#167667=CARTESIAN_POINT('Ctrl Pts',(56.1390278000226,45.1118181034888,12.));
#167668=CARTESIAN_POINT('Ctrl Pts',(56.116265815162,45.1040817305561,0.));
#167669=CARTESIAN_POINT('Ctrl Pts',(56.116265815162,45.1040817305561,12.));
#167670=CARTESIAN_POINT('Ctrl Pts',(56.0935514476945,45.0963368067177,0.));
#167671=CARTESIAN_POINT('Ctrl Pts',(56.0935514476945,45.0963368067177,12.));
#167672=CARTESIAN_POINT('Ctrl Pts',(56.0708847911416,45.0885834284517,0.));
#167673=CARTESIAN_POINT('Ctrl Pts',(56.0708847911416,45.0885834284517,12.));
#167674=CARTESIAN_POINT('Ctrl Pts',(56.048265939342,45.0808216927089,0.));
#167675=CARTESIAN_POINT('Ctrl Pts',(56.048265939342,45.0808216927089,12.));
#167676=CARTESIAN_POINT('Ctrl Pts',(56.0256949864639,45.0730516969149,0.));
#167677=CARTESIAN_POINT('Ctrl Pts',(56.0256949864639,45.0730516969149,12.));
#167678=CARTESIAN_POINT('Ctrl Pts',(56.003172027008,45.0652735389733,0.));
#167679=CARTESIAN_POINT('Ctrl Pts',(56.003172027008,45.0652735389733,12.));
#167680=CARTESIAN_POINT('Ctrl Pts',(55.9806971558097,45.0574873172695,0.));
#167681=CARTESIAN_POINT('Ctrl Pts',(55.9806971558097,45.0574873172695,12.));
#167682=CARTESIAN_POINT('Ctrl Pts',(55.9582704680356,45.0496931306755,0.));
#167683=CARTESIAN_POINT('Ctrl Pts',(55.9582704680356,45.0496931306755,12.));
#167684=CARTESIAN_POINT('Ctrl Pts',(55.9358920591837,45.0418910785551,0.));
#167685=CARTESIAN_POINT('Ctrl Pts',(55.9358920591837,45.0418910785551,12.));
#167686=CARTESIAN_POINT('Ctrl Pts',(55.9135620250954,45.0340812607657,0.));
#167687=CARTESIAN_POINT('Ctrl Pts',(55.9135620250954,45.0340812607657,12.));
#167688=CARTESIAN_POINT('Ctrl Pts',(55.8912804619577,45.0262637776615,0.));
#167689=CARTESIAN_POINT('Ctrl Pts',(55.8912804619577,45.0262637776615,12.));
#167690=CARTESIAN_POINT('Ctrl Pts',(55.8690474663065,45.0184387300973,0.));
#167691=CARTESIAN_POINT('Ctrl Pts',(55.8690474663065,45.0184387300973,12.));
#167692=CARTESIAN_POINT('Ctrl Pts',(55.8468631350218,45.0106062194342,0.));
#167693=CARTESIAN_POINT('Ctrl Pts',(55.8468631350218,45.0106062194342,12.));
#167694=CARTESIAN_POINT('Ctrl Pts',(55.8247275653289,45.0027663475433,0.));
#167695=CARTESIAN_POINT('Ctrl Pts',(55.8247275653289,45.0027663475433,12.));
#167696=CARTESIAN_POINT('Ctrl Pts',(55.8026408548105,44.9949192168093,0.));
#167697=CARTESIAN_POINT('Ctrl Pts',(55.8026408548105,44.9949192168093,12.));
#167698=CARTESIAN_POINT('Ctrl Pts',(55.7806031014106,44.9870649301342,0.));
#167699=CARTESIAN_POINT('Ctrl Pts',(55.7806031014106,44.9870649301342,12.));
#167700=CARTESIAN_POINT('Ctrl Pts',(55.7586144034367,44.9792035909413,0.));
#167701=CARTESIAN_POINT('Ctrl Pts',(55.7586144034367,44.9792035909413,12.));
#167702=CARTESIAN_POINT('Ctrl Pts',(55.7366748595551,44.9713353031804,0.));
#167703=CARTESIAN_POINT('Ctrl Pts',(55.7366748595551,44.9713353031804,12.));
#167704=CARTESIAN_POINT('Ctrl Pts',(55.714784568793,44.9634601713321,0.));
#167705=CARTESIAN_POINT('Ctrl Pts',(55.714784568793,44.9634601713321,12.));
#167706=CARTESIAN_POINT('Ctrl Pts',(55.6929436305489,44.9555783004106,0.));
#167707=CARTESIAN_POINT('Ctrl Pts',(55.6929436305489,44.9555783004106,12.));
#167708=CARTESIAN_POINT('Ctrl Pts',(55.6711521445979,44.9476897959685,0.));
#167709=CARTESIAN_POINT('Ctrl Pts',(55.6711521445979,44.9476897959685,12.));
#167710=CARTESIAN_POINT('Ctrl Pts',(55.6494102110935,44.9397947641007,0.));
#167711=CARTESIAN_POINT('Ctrl Pts',(55.6494102110935,44.9397947641007,12.));
#167712=CARTESIAN_POINT('Ctrl Pts',(55.6277179305633,44.9318933114507,0.));
#167713=CARTESIAN_POINT('Ctrl Pts',(55.6277179305633,44.9318933114507,12.));
#167714=CARTESIAN_POINT('Ctrl Pts',(55.6060754039121,44.9239855452144,0.));
#167715=CARTESIAN_POINT('Ctrl Pts',(55.6060754039121,44.9239855452144,12.));
#167716=CARTESIAN_POINT('Ctrl Pts',(55.5844827324338,44.9160715731443,0.));
#167717=CARTESIAN_POINT('Ctrl Pts',(55.5844827324338,44.9160715731443,12.));
#167718=CARTESIAN_POINT('Ctrl Pts',(55.5629400178142,44.908151503553,0.));
#167719=CARTESIAN_POINT('Ctrl Pts',(55.5629400178142,44.908151503553,12.));
#167720=CARTESIAN_POINT('Ctrl Pts',(55.541447362134,44.9002254453183,0.));
#167721=CARTESIAN_POINT('Ctrl Pts',(55.541447362134,44.9002254453183,12.));
#167722=CARTESIAN_POINT('Ctrl Pts',(55.5200048678629,44.8922935078889,0.));
#167723=CARTESIAN_POINT('Ctrl Pts',(55.5200048678629,44.8922935078889,12.));
#167724=CARTESIAN_POINT('Ctrl Pts',(55.4986126378656,44.8843558012886,0.));
#167725=CARTESIAN_POINT('Ctrl Pts',(55.4986126378656,44.8843558012886,12.));
#167726=CARTESIAN_POINT('Ctrl Pts',(55.4772707754126,44.8764124361207,0.));
#167727=CARTESIAN_POINT('Ctrl Pts',(55.4772707754126,44.8764124361207,12.));
#167728=CARTESIAN_POINT('Ctrl Pts',(55.4559793841836,44.8684635235725,0.));
#167729=CARTESIAN_POINT('Ctrl Pts',(55.4559793841836,44.8684635235725,12.));
#167730=CARTESIAN_POINT('Ctrl Pts',(55.4347385682704,44.8605091754214,0.));
#167731=CARTESIAN_POINT('Ctrl Pts',(55.4347385682704,44.8605091754214,12.));
#167732=CARTESIAN_POINT('Ctrl Pts',(55.4135484321718,44.8525495040408,0.));
#167733=CARTESIAN_POINT('Ctrl Pts',(55.4135484321718,44.8525495040408,12.));
#167734=CARTESIAN_POINT('Ctrl Pts',(55.3924090808014,44.8445846224044,0.));
#167735=CARTESIAN_POINT('Ctrl Pts',(55.3924090808014,44.8445846224044,12.));
#167736=CARTESIAN_POINT('Ctrl Pts',(55.3713206194967,44.8366146440901,0.));
#167737=CARTESIAN_POINT('Ctrl Pts',(55.3713206194967,44.8366146440901,12.));
#167738=CARTESIAN_POINT('Ctrl Pts',(55.3502831540228,44.8286396832848,0.));
#167739=CARTESIAN_POINT('Ctrl Pts',(55.3502831540228,44.8286396832848,12.));
#167740=CARTESIAN_POINT('Ctrl Pts',(55.3292967905725,44.8206598547888,0.));
#167741=CARTESIAN_POINT('Ctrl Pts',(55.3292967905725,44.8206598547888,12.));
#167742=CARTESIAN_POINT('Ctrl Pts',(55.3083616357605,44.8126752740208,0.));
#167743=CARTESIAN_POINT('Ctrl Pts',(55.3083616357605,44.8126752740208,12.));
#167744=CARTESIAN_POINT('Ctrl Pts',(55.287477796635,44.8046860570244,0.));
#167745=CARTESIAN_POINT('Ctrl Pts',(55.287477796635,44.8046860570244,12.));
#167746=CARTESIAN_POINT('Ctrl Pts',(55.2666453806883,44.796692320474,0.));
#167747=CARTESIAN_POINT('Ctrl Pts',(55.2666453806883,44.796692320474,12.));
#167748=CARTESIAN_POINT('Ctrl Pts',(55.2458644958617,44.7886941816823,0.));
#167749=CARTESIAN_POINT('Ctrl Pts',(55.2458644958617,44.7886941816823,12.));
#167750=CARTESIAN_POINT('Ctrl Pts',(55.2251352505474,44.7806917586077,0.));
#167751=CARTESIAN_POINT('Ctrl Pts',(55.2251352505474,44.7806917586077,12.));
#167752=CARTESIAN_POINT('Ctrl Pts',(55.2044577535865,44.7726851698618,0.));
#167753=CARTESIAN_POINT('Ctrl Pts',(55.2044577535865,44.7726851698618,12.));
#167754=CARTESIAN_POINT('Ctrl Pts',(55.1838321142777,44.7646745347108,0.));
#167755=CARTESIAN_POINT('Ctrl Pts',(55.1838321142777,44.7646745347108,12.));
#167756=CARTESIAN_POINT('Ctrl Pts',(55.1632584423813,44.7566599730771,0.));
#167757=CARTESIAN_POINT('Ctrl Pts',(55.1632584423813,44.7566599730771,12.));
#167758=CARTESIAN_POINT('Ctrl Pts',(55.1427368481201,44.748641605542,0.));
#167759=CARTESIAN_POINT('Ctrl Pts',(55.1427368481201,44.748641605542,12.));
#167760=CARTESIAN_POINT('Ctrl Pts',(55.1222674421747,44.7406195533483,0.));
#167761=CARTESIAN_POINT('Ctrl Pts',(55.1222674421747,44.7406195533483,12.));
#167762=CARTESIAN_POINT('Ctrl Pts',(55.1018503356806,44.7325939384042,0.));
#167763=CARTESIAN_POINT('Ctrl Pts',(55.1018503356806,44.7325939384042,12.));
#167764=CARTESIAN_POINT('Ctrl Pts',(55.0814856402507,44.7245648832988,0.));
#167765=CARTESIAN_POINT('Ctrl Pts',(55.0814856402507,44.7245648832988,12.));
#167766=CARTESIAN_POINT('Ctrl Pts',(55.0611734679902,44.7165325113165,0.));
#167767=CARTESIAN_POINT('Ctrl Pts',(55.0611734679902,44.7165325113165,12.));
#167768=CARTESIAN_POINT('Ctrl Pts',(55.0409139315074,44.7084969464509,0.));
#167769=CARTESIAN_POINT('Ctrl Pts',(55.0409139315074,44.7084969464509,12.));
#167770=CARTESIAN_POINT('Ctrl Pts',(55.020707143922,44.7004583134235,0.));
#167771=CARTESIAN_POINT('Ctrl Pts',(55.020707143922,44.7004583134235,12.));
#167772=CARTESIAN_POINT('Ctrl Pts',(55.0005532188644,44.6924167376851,0.));
#167773=CARTESIAN_POINT('Ctrl Pts',(55.0005532188644,44.6924167376851,12.));
#167774=CARTESIAN_POINT('Ctrl Pts',(54.9804522704668,44.6843723453985,0.));
#167775=CARTESIAN_POINT('Ctrl Pts',(54.9804522704668,44.6843723453985,12.));
#167776=CARTESIAN_POINT('Ctrl Pts',(54.9604044133497,44.6763252634255,0.));
#167777=CARTESIAN_POINT('Ctrl Pts',(54.9604044133497,44.6763252634255,12.));
#167778=CARTESIAN_POINT('Ctrl Pts',(54.9404097626088,44.6682756193156,0.));
#167779=CARTESIAN_POINT('Ctrl Pts',(54.9404097626088,44.6682756193156,12.));
#167780=CARTESIAN_POINT('Ctrl Pts',(54.9204684337845,44.6602235412854,0.));
#167781=CARTESIAN_POINT('Ctrl Pts',(54.9204684337845,44.6602235412854,12.));
#167782=CARTESIAN_POINT('Ctrl Pts',(54.9005805428991,44.6521691582551,0.));
#167783=CARTESIAN_POINT('Ctrl Pts',(54.9005805428991,44.6521691582551,12.));
#167784=CARTESIAN_POINT('Ctrl Pts',(54.8807462065177,44.6441125999074,0.));
#167785=CARTESIAN_POINT('Ctrl Pts',(54.8807462065177,44.6441125999074,12.));
#167786=CARTESIAN_POINT('Ctrl Pts',(54.860965541796,44.6360539967392,0.));
#167787=CARTESIAN_POINT('Ctrl Pts',(54.860965541796,44.6360539967392,12.));
#167788=CARTESIAN_POINT('Ctrl Pts',(54.8412386665264,44.6279934801159,0.));
#167789=CARTESIAN_POINT('Ctrl Pts',(54.8412386665264,44.6279934801159,12.));
#167790=CARTESIAN_POINT('Ctrl Pts',(54.8215656991817,44.6199311823276,0.));
#167791=CARTESIAN_POINT('Ctrl Pts',(54.8215656991817,44.6199311823276,12.));
#167792=CARTESIAN_POINT('Ctrl Pts',(54.8019467588257,44.6118672364889,0.));
#167793=CARTESIAN_POINT('Ctrl Pts',(54.8019467588257,44.6118672364889,12.));
#167794=CARTESIAN_POINT('Ctrl Pts',(54.7823819650137,44.60380177643,0.));
#167795=CARTESIAN_POINT('Ctrl Pts',(54.7823819650137,44.60380177643,12.));
#167796=CARTESIAN_POINT('Ctrl Pts',(54.7628714377041,44.5957349366062,0.));
#167797=CARTESIAN_POINT('Ctrl Pts',(54.7628714377041,44.5957349366062,12.));
#167798=CARTESIAN_POINT('Ctrl Pts',(54.7434152971285,44.5876668519676,0.));
#167799=CARTESIAN_POINT('Ctrl Pts',(54.7434152971285,44.5876668519676,12.));
#167800=CARTESIAN_POINT('Ctrl Pts',(54.7240136637744,44.5795976579476,0.));
#167801=CARTESIAN_POINT('Ctrl Pts',(54.7240136637744,44.5795976579476,12.));
#167802=CARTESIAN_POINT('Ctrl Pts',(54.7046666586776,44.5715274907637,0.));
#167803=CARTESIAN_POINT('Ctrl Pts',(54.7046666586776,44.5715274907637,12.));
#167804=CARTESIAN_POINT('Ctrl Pts',(54.685374403676,44.563456487687,0.));
#167805=CARTESIAN_POINT('Ctrl Pts',(54.685374403676,44.563456487687,12.));
#167806=CARTESIAN_POINT('Ctrl Pts',(54.6661370216242,44.5553847872712,0.));
#167807=CARTESIAN_POINT('Ctrl Pts',(54.6661370216242,44.5553847872712,12.));
#167808=CARTESIAN_POINT('Ctrl Pts',(54.6469546367381,44.5473125297289,0.));
#167809=CARTESIAN_POINT('Ctrl Pts',(54.6469546367381,44.5473125297289,12.));
#167810=CARTESIAN_POINT('Ctrl Pts',(54.6278273743554,44.5392398566775,0.));
#167811=CARTESIAN_POINT('Ctrl Pts',(54.6278273743554,44.5392398566775,12.));
#167812=CARTESIAN_POINT('Ctrl Pts',(54.6087553602889,44.5311669104495,0.));
#167813=CARTESIAN_POINT('Ctrl Pts',(54.6087553602889,44.5311669104495,12.));
#167814=CARTESIAN_POINT('Ctrl Pts',(54.5897387202812,44.5230938335165,0.));
#167815=CARTESIAN_POINT('Ctrl Pts',(54.5897387202812,44.5230938335165,12.));
#167816=CARTESIAN_POINT('Ctrl Pts',(54.5707775794436,44.5150207679007,0.));
#167817=CARTESIAN_POINT('Ctrl Pts',(54.5707775794436,44.5150207679007,12.));
#167818=CARTESIAN_POINT('Ctrl Pts',(54.5518720616056,44.5069478544977,0.));
#167819=CARTESIAN_POINT('Ctrl Pts',(54.5518720616056,44.5069478544977,12.));
#167820=CARTESIAN_POINT('Ctrl Pts',(54.5330222905475,44.4988752343744,0.));
#167821=CARTESIAN_POINT('Ctrl Pts',(54.5330222905475,44.4988752343744,12.));
#167822=CARTESIAN_POINT('Ctrl Pts',(54.5142283914704,44.4908030503225,0.));
#167823=CARTESIAN_POINT('Ctrl Pts',(54.5142283914704,44.4908030503225,12.));
#167824=CARTESIAN_POINT('Ctrl Pts',(54.495490492193,44.4827314481264,0.));
#167825=CARTESIAN_POINT('Ctrl Pts',(54.495490492193,44.4827314481264,12.));
#167826=CARTESIAN_POINT('Ctrl Pts',(54.4768087248824,44.4746605784031,0.));
#167827=CARTESIAN_POINT('Ctrl Pts',(54.4768087248824,44.4746605784031,12.));
#167828=CARTESIAN_POINT('Ctrl Pts',(54.4581832262033,44.4665905967668,0.));
#167829=CARTESIAN_POINT('Ctrl Pts',(54.4581832262033,44.4665905967668,12.));
#167830=CARTESIAN_POINT('Ctrl Pts',(54.4396141336978,44.4585216599908,0.));
#167831=CARTESIAN_POINT('Ctrl Pts',(54.4396141336978,44.4585216599908,12.));
#167832=CARTESIAN_POINT('Ctrl Pts',(54.421101582595,44.4504539226328,0.));
#167833=CARTESIAN_POINT('Ctrl Pts',(54.421101582595,44.4504539226328,12.));
#167834=CARTESIAN_POINT('Ctrl Pts',(54.4026457030335,44.4423875340996,0.));
#167835=CARTESIAN_POINT('Ctrl Pts',(54.4026457030335,44.4423875340996,12.));
#167836=CARTESIAN_POINT('Ctrl Pts',(54.3842466156196,44.4343226339593,0.));
#167837=CARTESIAN_POINT('Ctrl Pts',(54.3842466156196,44.4343226339593,12.));
#167838=CARTESIAN_POINT('Ctrl Pts',(54.3659044357119,44.4262593564712,0.));
#167839=CARTESIAN_POINT('Ctrl Pts',(54.3659044357119,44.4262593564712,12.));
#167840=CARTESIAN_POINT('Ctrl Pts',(54.3476192819352,44.4181978395851,0.));
#167841=CARTESIAN_POINT('Ctrl Pts',(54.3476192819352,44.4181978395851,12.));
#167842=CARTESIAN_POINT('Ctrl Pts',(54.3293912830237,44.4101382321834,0.));
#167843=CARTESIAN_POINT('Ctrl Pts',(54.3293912830237,44.4101382321834,12.));
#167844=CARTESIAN_POINT('Ctrl Pts',(54.3112205860716,44.402080702809,0.));
#167845=CARTESIAN_POINT('Ctrl Pts',(54.3112205860716,44.402080702809,12.));
#167846=CARTESIAN_POINT('Ctrl Pts',(54.2931073621553,44.3940254456331,0.));
#167847=CARTESIAN_POINT('Ctrl Pts',(54.2931073621553,44.3940254456331,12.));
#167848=CARTESIAN_POINT('Ctrl Pts',(54.2750517888579,44.3859726620183,0.));
#167849=CARTESIAN_POINT('Ctrl Pts',(54.2750517888579,44.3859726620183,12.));
#167850=CARTESIAN_POINT('Ctrl Pts',(54.2570540336475,44.3779225430406,0.));
#167851=CARTESIAN_POINT('Ctrl Pts',(54.2570540336475,44.3779225430406,12.));
#167852=CARTESIAN_POINT('Ctrl Pts',(54.2391142386412,44.3698752533562,0.));
#167853=CARTESIAN_POINT('Ctrl Pts',(54.2391142386412,44.3698752533562,12.));
#167854=CARTESIAN_POINT('Ctrl Pts',(54.2212325006052,44.361830910343,0.));
#167855=CARTESIAN_POINT('Ctrl Pts',(54.2212325006052,44.361830910343,12.));
#167856=CARTESIAN_POINT('Ctrl Pts',(54.2034088701928,44.3537895824096,0.));
#167857=CARTESIAN_POINT('Ctrl Pts',(54.2034088701928,44.3537895824096,12.));
#167858=CARTESIAN_POINT('Ctrl Pts',(54.1891964684727,44.3473589597726,0.));
#167859=CARTESIAN_POINT('Ctrl Pts',(54.1891964684727,44.3473589597726,12.));
#167860=CARTESIAN_POINT('Ctrl Pts',(54.1785633257639,44.3425373700993,0.));
#167861=CARTESIAN_POINT('Ctrl Pts',(54.1785633257639,44.3425373700993,12.));
#167862=CARTESIAN_POINT('Ctrl Pts',(54.1714861895346,44.3393235891075,0.));
#167863=CARTESIAN_POINT('Ctrl Pts',(54.1714861895346,44.3393235891075,12.));
#167864=CARTESIAN_POINT('Ctrl Pts',(54.1679505278134,44.3377168516418,0.));
#167865=CARTESIAN_POINT('Ctrl Pts',(54.1679505278134,44.3377168516418,12.));
#167866=CARTESIAN_POINT('',(54.1679505278134,44.3377168516418,12.));
#167867=CARTESIAN_POINT('Ctrl Pts',(54.1679505278134,44.3377168516418,12.));
#167868=CARTESIAN_POINT('Ctrl Pts',(54.1714861895346,44.3393235891075,12.));
#167869=CARTESIAN_POINT('Ctrl Pts',(54.1785633257639,44.3425373700993,12.));
#167870=CARTESIAN_POINT('Ctrl Pts',(54.1891964684727,44.3473589597726,12.));
#167871=CARTESIAN_POINT('Ctrl Pts',(54.2034088701928,44.3537895824096,12.));
#167872=CARTESIAN_POINT('Ctrl Pts',(54.2212325006052,44.361830910343,12.));
#167873=CARTESIAN_POINT('Ctrl Pts',(54.2391142386412,44.3698752533562,12.));
#167874=CARTESIAN_POINT('Ctrl Pts',(54.2570540336475,44.3779225430406,12.));
#167875=CARTESIAN_POINT('Ctrl Pts',(54.2750517888579,44.3859726620183,12.));
#167876=CARTESIAN_POINT('Ctrl Pts',(54.2931073621553,44.3940254456331,12.));
#167877=CARTESIAN_POINT('Ctrl Pts',(54.3112205860716,44.402080702809,12.));
#167878=CARTESIAN_POINT('Ctrl Pts',(54.3293912830237,44.4101382321834,12.));
#167879=CARTESIAN_POINT('Ctrl Pts',(54.3476192819352,44.4181978395851,12.));
#167880=CARTESIAN_POINT('Ctrl Pts',(54.3659044357119,44.4262593564712,12.));
#167881=CARTESIAN_POINT('Ctrl Pts',(54.3842466156196,44.4343226339593,12.));
#167882=CARTESIAN_POINT('Ctrl Pts',(54.4026457030335,44.4423875340996,12.));
#167883=CARTESIAN_POINT('Ctrl Pts',(54.421101582595,44.4504539226328,12.));
#167884=CARTESIAN_POINT('Ctrl Pts',(54.4396141336978,44.4585216599908,12.));
#167885=CARTESIAN_POINT('Ctrl Pts',(54.4581832262033,44.4665905967668,12.));
#167886=CARTESIAN_POINT('Ctrl Pts',(54.4768087248824,44.4746605784031,12.));
#167887=CARTESIAN_POINT('Ctrl Pts',(54.495490492193,44.4827314481264,12.));
#167888=CARTESIAN_POINT('Ctrl Pts',(54.5142283914704,44.4908030503225,12.));
#167889=CARTESIAN_POINT('Ctrl Pts',(54.5330222905475,44.4988752343744,12.));
#167890=CARTESIAN_POINT('Ctrl Pts',(54.5518720616056,44.5069478544977,12.));
#167891=CARTESIAN_POINT('Ctrl Pts',(54.5707775794436,44.5150207679007,12.));
#167892=CARTESIAN_POINT('Ctrl Pts',(54.5897387202812,44.5230938335165,12.));
#167893=CARTESIAN_POINT('Ctrl Pts',(54.6087553602889,44.5311669104495,12.));
#167894=CARTESIAN_POINT('Ctrl Pts',(54.6278273743554,44.5392398566775,12.));
#167895=CARTESIAN_POINT('Ctrl Pts',(54.6469546367381,44.5473125297289,12.));
#167896=CARTESIAN_POINT('Ctrl Pts',(54.6661370216242,44.5553847872712,12.));
#167897=CARTESIAN_POINT('Ctrl Pts',(54.685374403676,44.563456487687,12.));
#167898=CARTESIAN_POINT('Ctrl Pts',(54.7046666586776,44.5715274907637,12.));
#167899=CARTESIAN_POINT('Ctrl Pts',(54.7240136637744,44.5795976579476,12.));
#167900=CARTESIAN_POINT('Ctrl Pts',(54.7434152971285,44.5876668519676,12.));
#167901=CARTESIAN_POINT('Ctrl Pts',(54.7628714377041,44.5957349366062,12.));
#167902=CARTESIAN_POINT('Ctrl Pts',(54.7823819650137,44.60380177643,12.));
#167903=CARTESIAN_POINT('Ctrl Pts',(54.8019467588257,44.6118672364889,12.));
#167904=CARTESIAN_POINT('Ctrl Pts',(54.8215656991817,44.6199311823276,12.));
#167905=CARTESIAN_POINT('Ctrl Pts',(54.8412386665264,44.6279934801159,12.));
#167906=CARTESIAN_POINT('Ctrl Pts',(54.860965541796,44.6360539967392,12.));
#167907=CARTESIAN_POINT('Ctrl Pts',(54.8807462065177,44.6441125999074,12.));
#167908=CARTESIAN_POINT('Ctrl Pts',(54.9005805428991,44.6521691582551,12.));
#167909=CARTESIAN_POINT('Ctrl Pts',(54.9204684337845,44.6602235412854,12.));
#167910=CARTESIAN_POINT('Ctrl Pts',(54.9404097626088,44.6682756193156,12.));
#167911=CARTESIAN_POINT('Ctrl Pts',(54.9604044133497,44.6763252634255,12.));
#167912=CARTESIAN_POINT('Ctrl Pts',(54.9804522704668,44.6843723453985,12.));
#167913=CARTESIAN_POINT('Ctrl Pts',(55.0005532188644,44.6924167376851,12.));
#167914=CARTESIAN_POINT('Ctrl Pts',(55.020707143922,44.7004583134235,12.));
#167915=CARTESIAN_POINT('Ctrl Pts',(55.0409139315074,44.7084969464509,12.));
#167916=CARTESIAN_POINT('Ctrl Pts',(55.0611734679902,44.7165325113165,12.));
#167917=CARTESIAN_POINT('Ctrl Pts',(55.0814856402507,44.7245648832988,12.));
#167918=CARTESIAN_POINT('Ctrl Pts',(55.1018503356806,44.7325939384042,12.));
#167919=CARTESIAN_POINT('Ctrl Pts',(55.1222674421747,44.7406195533483,12.));
#167920=CARTESIAN_POINT('Ctrl Pts',(55.1427368481201,44.748641605542,12.));
#167921=CARTESIAN_POINT('Ctrl Pts',(55.1632584423813,44.7566599730771,12.));
#167922=CARTESIAN_POINT('Ctrl Pts',(55.1838321142777,44.7646745347108,12.));
#167923=CARTESIAN_POINT('Ctrl Pts',(55.2044577535865,44.7726851698618,12.));
#167924=CARTESIAN_POINT('Ctrl Pts',(55.2251352505474,44.7806917586077,12.));
#167925=CARTESIAN_POINT('Ctrl Pts',(55.2458644958617,44.7886941816823,12.));
#167926=CARTESIAN_POINT('Ctrl Pts',(55.2666453806883,44.796692320474,12.));
#167927=CARTESIAN_POINT('Ctrl Pts',(55.287477796635,44.8046860570244,12.));
#167928=CARTESIAN_POINT('Ctrl Pts',(55.3083616357605,44.8126752740208,12.));
#167929=CARTESIAN_POINT('Ctrl Pts',(55.3292967905725,44.8206598547888,12.));
#167930=CARTESIAN_POINT('Ctrl Pts',(55.3502831540228,44.8286396832848,12.));
#167931=CARTESIAN_POINT('Ctrl Pts',(55.3713206194967,44.8366146440901,12.));
#167932=CARTESIAN_POINT('Ctrl Pts',(55.3924090808014,44.8445846224044,12.));
#167933=CARTESIAN_POINT('Ctrl Pts',(55.4135484321718,44.8525495040408,12.));
#167934=CARTESIAN_POINT('Ctrl Pts',(55.4347385682704,44.8605091754214,12.));
#167935=CARTESIAN_POINT('Ctrl Pts',(55.4559793841836,44.8684635235725,12.));
#167936=CARTESIAN_POINT('Ctrl Pts',(55.4772707754126,44.8764124361207,12.));
#167937=CARTESIAN_POINT('Ctrl Pts',(55.4986126378656,44.8843558012886,12.));
#167938=CARTESIAN_POINT('Ctrl Pts',(55.5200048678629,44.8922935078889,12.));
#167939=CARTESIAN_POINT('Ctrl Pts',(55.541447362134,44.9002254453183,12.));
#167940=CARTESIAN_POINT('Ctrl Pts',(55.5629400178142,44.908151503553,12.));
#167941=CARTESIAN_POINT('Ctrl Pts',(55.5844827324338,44.9160715731443,12.));
#167942=CARTESIAN_POINT('Ctrl Pts',(55.6060754039121,44.9239855452144,12.));
#167943=CARTESIAN_POINT('Ctrl Pts',(55.6277179305633,44.9318933114507,12.));
#167944=CARTESIAN_POINT('Ctrl Pts',(55.6494102110935,44.9397947641007,12.));
#167945=CARTESIAN_POINT('Ctrl Pts',(55.6711521445979,44.9476897959685,12.));
#167946=CARTESIAN_POINT('Ctrl Pts',(55.6929436305489,44.9555783004106,12.));
#167947=CARTESIAN_POINT('Ctrl Pts',(55.714784568793,44.9634601713321,12.));
#167948=CARTESIAN_POINT('Ctrl Pts',(55.7366748595551,44.9713353031804,12.));
#167949=CARTESIAN_POINT('Ctrl Pts',(55.7586144034367,44.9792035909413,12.));
#167950=CARTESIAN_POINT('Ctrl Pts',(55.7806031014106,44.9870649301342,12.));
#167951=CARTESIAN_POINT('Ctrl Pts',(55.8026408548105,44.9949192168093,12.));
#167952=CARTESIAN_POINT('Ctrl Pts',(55.8247275653289,45.0027663475433,12.));
#167953=CARTESIAN_POINT('Ctrl Pts',(55.8468631350218,45.0106062194342,12.));
#167954=CARTESIAN_POINT('Ctrl Pts',(55.8690474663065,45.0184387300973,12.));
#167955=CARTESIAN_POINT('Ctrl Pts',(55.8912804619577,45.0262637776615,12.));
#167956=CARTESIAN_POINT('Ctrl Pts',(55.9135620250954,45.0340812607657,12.));
#167957=CARTESIAN_POINT('Ctrl Pts',(55.9358920591837,45.0418910785551,12.));
#167958=CARTESIAN_POINT('Ctrl Pts',(55.9582704680356,45.0496931306755,12.));
#167959=CARTESIAN_POINT('Ctrl Pts',(55.9806971558097,45.0574873172695,12.));
#167960=CARTESIAN_POINT('Ctrl Pts',(56.003172027008,45.0652735389733,12.));
#167961=CARTESIAN_POINT('Ctrl Pts',(56.0256949864639,45.0730516969149,12.));
#167962=CARTESIAN_POINT('Ctrl Pts',(56.048265939342,45.0808216927089,12.));
#167963=CARTESIAN_POINT('Ctrl Pts',(56.0708847911416,45.0885834284517,12.));
#167964=CARTESIAN_POINT('Ctrl Pts',(56.0935514476945,45.0963368067177,12.));
#167965=CARTESIAN_POINT('Ctrl Pts',(56.116265815162,45.1040817305561,12.));
#167966=CARTESIAN_POINT('Ctrl Pts',(56.1390278000226,45.1118181034888,12.));
#167967=CARTESIAN_POINT('Ctrl Pts',(56.1618373090732,45.1195458295063,12.));
#167968=CARTESIAN_POINT('Ctrl Pts',(56.1846942494325,45.127264813063,12.));
#167969=CARTESIAN_POINT('Ctrl Pts',(56.2075985285393,45.1349749590738,12.));
#167970=CARTESIAN_POINT('Ctrl Pts',(56.2305500541489,45.1426761729105,12.));
#167971=CARTESIAN_POINT('Ctrl Pts',(56.2535487343221,45.1503683604005,12.));
#167972=CARTESIAN_POINT('Ctrl Pts',(56.2765944774245,45.1580514278223,12.));
#167973=CARTESIAN_POINT('Ctrl Pts',(56.2996871921316,45.1657252819013,12.));
#167974=CARTESIAN_POINT('Ctrl Pts',(56.3228267874264,45.1733898298061,12.));
#167975=CARTESIAN_POINT('Ctrl Pts',(56.3460131725964,45.1810449791453,12.));
#167976=CARTESIAN_POINT('Ctrl Pts',(56.3692462572231,45.1886906379667,12.));
#167977=CARTESIAN_POINT('Ctrl Pts',(56.3925259511806,45.1963267147529,12.));
#167978=CARTESIAN_POINT('Ctrl Pts',(56.4158521646411,45.2039531184172,12.));
#167979=CARTESIAN_POINT('Ctrl Pts',(56.4392248080732,45.2115697583001,12.));
#167980=CARTESIAN_POINT('Ctrl Pts',(56.4626437922386,45.2191765441667,12.));
#167981=CARTESIAN_POINT('Ctrl Pts',(56.4861090281823,45.2267733862049,12.));
#167982=CARTESIAN_POINT('Ctrl Pts',(56.5096204272306,45.2343601950228,12.));
#167983=CARTESIAN_POINT('Ctrl Pts',(56.5331779009958,45.2419368816429,12.));
#167984=CARTESIAN_POINT('Ctrl Pts',(56.5567813613756,45.2495033575,12.));
#167985=CARTESIAN_POINT('Ctrl Pts',(56.5804307205505,45.257059534438,12.));
#167986=CARTESIAN_POINT('Ctrl Pts',(56.6041258909741,45.2646053247087,12.));
#167987=CARTESIAN_POINT('Ctrl Pts',(56.6278667853702,45.2721406409695,12.));
#167988=CARTESIAN_POINT('Ctrl Pts',(56.6516533167384,45.2796653962785,12.));
#167989=CARTESIAN_POINT('Ctrl Pts',(56.6754853983528,45.2871795040906,12.));
#167990=CARTESIAN_POINT('Ctrl Pts',(56.69936294376,45.2946828782559,12.));
#167991=CARTESIAN_POINT('Ctrl Pts',(56.7232858667709,45.3021754330179,12.));
#167992=CARTESIAN_POINT('Ctrl Pts',(56.7472540814553,45.3096570830118,12.));
#167993=CARTESIAN_POINT('Ctrl Pts',(56.7712675021491,45.31712774326,12.));
#167994=CARTESIAN_POINT('Ctrl Pts',(56.7953260434524,45.3245873291684,12.));
#167995=CARTESIAN_POINT('Ctrl Pts',(56.8194296202291,45.332035756524,12.));
#167996=CARTESIAN_POINT('Ctrl Pts',(56.8435781475981,45.3394729414931,12.));
#167997=CARTESIAN_POINT('Ctrl Pts',(56.8677715409268,45.3468988006203,12.));
#167998=CARTESIAN_POINT('Ctrl Pts',(56.8920097158377,45.3543132508239,12.));
#167999=CARTESIAN_POINT('Ctrl Pts',(56.9162925882085,45.3617162093923,12.));
#168000=CARTESIAN_POINT('Ctrl Pts',(56.9406200741714,45.3691075939827,12.));
#168001=CARTESIAN_POINT('Ctrl Pts',(56.9649920901073,45.3764873226196,12.));
#168002=CARTESIAN_POINT('Ctrl Pts',(56.9894085526373,45.3838553136948,12.));
#168003=CARTESIAN_POINT('Ctrl Pts',(57.0138693786278,45.3912114859616,12.));
#168004=CARTESIAN_POINT('Ctrl Pts',(57.0383744851913,45.3985557585311,12.));
#168005=CARTESIAN_POINT('Ctrl Pts',(57.0629237896848,45.4058880508693,12.));
#168006=CARTESIAN_POINT('Ctrl Pts',(57.0875172097051,45.4132082827948,12.));
#168007=CARTESIAN_POINT('Ctrl Pts',(57.112154663078,45.4205163744782,12.));
#168008=CARTESIAN_POINT('Ctrl Pts',(57.136836067863,45.4278122464389,12.));
#168009=CARTESIAN_POINT('Ctrl Pts',(57.1615613423584,45.4350958195434,12.));
#168010=CARTESIAN_POINT('Ctrl Pts',(57.186330405101,45.4423670150034,12.));
#168011=CARTESIAN_POINT('Ctrl Pts',(57.2111431748631,45.4496257543759,12.));
#168012=CARTESIAN_POINT('Ctrl Pts',(57.2359995706447,45.4568719595642,12.));
#168013=CARTESIAN_POINT('Ctrl Pts',(57.2608995116733,45.4641055528141,12.));
#168014=CARTESIAN_POINT('Ctrl Pts',(57.2858429174062,45.4713264567063,12.));
#168015=CARTESIAN_POINT('Ctrl Pts',(57.3108297075265,45.4785345941507,12.));
#168016=CARTESIAN_POINT('Ctrl Pts',(57.3358598019389,45.4857298883824,12.));
#168017=CARTESIAN_POINT('Ctrl Pts',(57.3609331207574,45.4929122629572,12.));
#168018=CARTESIAN_POINT('Ctrl Pts',(57.3860495843033,45.500081641751,12.));
#168019=CARTESIAN_POINT('Ctrl Pts',(57.4112091131183,45.5072379489631,12.));
#168020=CARTESIAN_POINT('Ctrl Pts',(57.4364116279702,45.5143811091205,12.));
#168021=CARTESIAN_POINT('Ctrl Pts',(57.4616570498568,45.5215110470825,12.));
#168022=CARTESIAN_POINT('Ctrl Pts',(57.4869453000063,45.5286276880485,12.));
#168023=CARTESIAN_POINT('Ctrl Pts',(57.5122762998745,45.5357309575611,12.));
#168024=CARTESIAN_POINT('Ctrl Pts',(57.537649971135,45.542820781484,12.));
#168025=CARTESIAN_POINT('Ctrl Pts',(57.563066235668,45.5498970859835,12.));
#168026=CARTESIAN_POINT('Ctrl Pts',(57.5885250155433,45.5569597975096,12.));
#168027=CARTESIAN_POINT('Ctrl Pts',(57.614026233004,45.5640088427813,12.));
#168028=CARTESIAN_POINT('Ctrl Pts',(57.6395698104404,45.5710441487674,12.));
#168029=CARTESIAN_POINT('Ctrl Pts',(57.6651556704237,45.5780656427163,12.));
#168030=CARTESIAN_POINT('Ctrl Pts',(57.6907837357417,45.5850732521896,12.));
#168031=CARTESIAN_POINT('Ctrl Pts',(57.7164539294314,45.5920669050986,12.));
#168032=CARTESIAN_POINT('Ctrl Pts',(57.7421661748026,45.5990465297344,12.));
#168033=CARTESIAN_POINT('Ctrl Pts',(57.7679203954742,45.6060120548205,12.));
#168034=CARTESIAN_POINT('Ctrl Pts',(57.7937165153387,45.6129634094683,12.));
#168035=CARTESIAN_POINT('Ctrl Pts',(57.8195544584845,45.6199005230784,12.));
#168036=CARTESIAN_POINT('Ctrl Pts',(57.8454341491238,45.6268233252544,12.));
#168037=CARTESIAN_POINT('Ctrl Pts',(57.8713555115232,45.6337317457252,12.));
#168038=CARTESIAN_POINT('Ctrl Pts',(57.8973184699034,45.6406257142382,12.));
#168039=CARTESIAN_POINT('Ctrl Pts',(57.9233229484311,45.6475051605535,12.));
#168040=CARTESIAN_POINT('Ctrl Pts',(57.9493688714237,45.6543700146679,12.));
#168041=CARTESIAN_POINT('Ctrl Pts',(57.9754561635061,45.661220206992,12.));
#168042=CARTESIAN_POINT('Ctrl Pts',(58.0015847497837,45.6680556685493,12.));
#168043=CARTESIAN_POINT('Ctrl Pts',(58.0277545560012,45.6748763311643,12.));
#168044=CARTESIAN_POINT('Ctrl Pts',(58.0539655087117,45.6816821276678,12.));
#168045=CARTESIAN_POINT('Ctrl Pts',(58.0802175348966,45.6884729914485,12.));
#168046=CARTESIAN_POINT('Ctrl Pts',(58.1065105615907,45.695248856015,12.));
#168047=CARTESIAN_POINT('Ctrl Pts',(58.1328445154676,45.702009654518,12.));
#168048=CARTESIAN_POINT('Ctrl Pts',(58.1592193225137,45.7087553193771,12.));
#168049=CARTESIAN_POINT('Ctrl Pts',(58.185634907469,45.7154857816483,12.));
#168050=CARTESIAN_POINT('Ctrl Pts',(58.2120911942772,45.7222009715397,12.));
#168051=CARTESIAN_POINT('Ctrl Pts',(58.2385881070913,45.7289008195579,12.));
#168052=CARTESIAN_POINT('Ctrl Pts',(58.2651255711453,45.7355852575107,12.));
#168053=CARTESIAN_POINT('Ctrl Pts',(58.291703513584,45.742254219463,12.));
#168054=CARTESIAN_POINT('Ctrl Pts',(58.3183218645316,45.7489076429763,12.));
#168055=CARTESIAN_POINT('Ctrl Pts',(58.3449805573423,45.755545469402,12.));
#168056=CARTESIAN_POINT('Ctrl Pts',(58.3678667473437,45.7612219538124,12.));
#168057=CARTESIAN_POINT('Ctrl Pts',(58.3854348517442,45.7655655205367,12.));
#168058=CARTESIAN_POINT('Ctrl Pts',(58.3976670481067,45.7685831165564,12.));
#168059=CARTESIAN_POINT('Ctrl Pts',(58.4045515723353,45.7702793558176,12.));
#168060=CARTESIAN_POINT('Ctrl Pts',(58.4060826907792,45.7706564944895,12.));
#168061=CARTESIAN_POINT('',(54.1679505278134,44.3377168516418,0.));
#168062=CARTESIAN_POINT('',(54.1679505278134,44.3377168516418,0.));
#168063=CARTESIAN_POINT('Ctrl Pts',(58.4060826907792,45.7706564944895,0.));
#168064=CARTESIAN_POINT('Ctrl Pts',(58.4045515723353,45.7702793558176,0.));
#168065=CARTESIAN_POINT('Ctrl Pts',(58.3976670481067,45.7685831165564,0.));
#168066=CARTESIAN_POINT('Ctrl Pts',(58.3854348517442,45.7655655205367,0.));
#168067=CARTESIAN_POINT('Ctrl Pts',(58.3678667473437,45.7612219538124,0.));
#168068=CARTESIAN_POINT('Ctrl Pts',(58.3449805573423,45.755545469402,0.));
#168069=CARTESIAN_POINT('Ctrl Pts',(58.3183218645316,45.7489076429763,0.));
#168070=CARTESIAN_POINT('Ctrl Pts',(58.291703513584,45.742254219463,0.));
#168071=CARTESIAN_POINT('Ctrl Pts',(58.2651255711453,45.7355852575107,0.));
#168072=CARTESIAN_POINT('Ctrl Pts',(58.2385881070913,45.7289008195579,0.));
#168073=CARTESIAN_POINT('Ctrl Pts',(58.2120911942772,45.7222009715397,0.));
#168074=CARTESIAN_POINT('Ctrl Pts',(58.185634907469,45.7154857816483,0.));
#168075=CARTESIAN_POINT('Ctrl Pts',(58.1592193225137,45.7087553193771,0.));
#168076=CARTESIAN_POINT('Ctrl Pts',(58.1328445154676,45.702009654518,0.));
#168077=CARTESIAN_POINT('Ctrl Pts',(58.1065105615907,45.695248856015,0.));
#168078=CARTESIAN_POINT('Ctrl Pts',(58.0802175348966,45.6884729914485,0.));
#168079=CARTESIAN_POINT('Ctrl Pts',(58.0539655087117,45.6816821276678,0.));
#168080=CARTESIAN_POINT('Ctrl Pts',(58.0277545560012,45.6748763311643,0.));
#168081=CARTESIAN_POINT('Ctrl Pts',(58.0015847497837,45.6680556685493,0.));
#168082=CARTESIAN_POINT('Ctrl Pts',(57.9754561635061,45.661220206992,0.));
#168083=CARTESIAN_POINT('Ctrl Pts',(57.9493688714237,45.6543700146679,0.));
#168084=CARTESIAN_POINT('Ctrl Pts',(57.9233229484311,45.6475051605535,0.));
#168085=CARTESIAN_POINT('Ctrl Pts',(57.8973184699034,45.6406257142382,0.));
#168086=CARTESIAN_POINT('Ctrl Pts',(57.8713555115232,45.6337317457252,0.));
#168087=CARTESIAN_POINT('Ctrl Pts',(57.8454341491238,45.6268233252544,0.));
#168088=CARTESIAN_POINT('Ctrl Pts',(57.8195544584845,45.6199005230784,0.));
#168089=CARTESIAN_POINT('Ctrl Pts',(57.7937165153387,45.6129634094683,0.));
#168090=CARTESIAN_POINT('Ctrl Pts',(57.7679203954742,45.6060120548205,0.));
#168091=CARTESIAN_POINT('Ctrl Pts',(57.7421661748026,45.5990465297344,0.));
#168092=CARTESIAN_POINT('Ctrl Pts',(57.7164539294314,45.5920669050986,0.));
#168093=CARTESIAN_POINT('Ctrl Pts',(57.6907837357417,45.5850732521896,0.));
#168094=CARTESIAN_POINT('Ctrl Pts',(57.6651556704237,45.5780656427163,0.));
#168095=CARTESIAN_POINT('Ctrl Pts',(57.6395698104404,45.5710441487674,0.));
#168096=CARTESIAN_POINT('Ctrl Pts',(57.614026233004,45.5640088427813,0.));
#168097=CARTESIAN_POINT('Ctrl Pts',(57.5885250155433,45.5569597975096,0.));
#168098=CARTESIAN_POINT('Ctrl Pts',(57.563066235668,45.5498970859835,0.));
#168099=CARTESIAN_POINT('Ctrl Pts',(57.537649971135,45.542820781484,0.));
#168100=CARTESIAN_POINT('Ctrl Pts',(57.5122762998745,45.5357309575611,0.));
#168101=CARTESIAN_POINT('Ctrl Pts',(57.4869453000063,45.5286276880485,0.));
#168102=CARTESIAN_POINT('Ctrl Pts',(57.4616570498568,45.5215110470825,0.));
#168103=CARTESIAN_POINT('Ctrl Pts',(57.4364116279702,45.5143811091205,0.));
#168104=CARTESIAN_POINT('Ctrl Pts',(57.4112091131183,45.5072379489631,0.));
#168105=CARTESIAN_POINT('Ctrl Pts',(57.3860495843033,45.500081641751,0.));
#168106=CARTESIAN_POINT('Ctrl Pts',(57.3609331207574,45.4929122629572,0.));
#168107=CARTESIAN_POINT('Ctrl Pts',(57.3358598019389,45.4857298883824,0.));
#168108=CARTESIAN_POINT('Ctrl Pts',(57.3108297075265,45.4785345941507,0.));
#168109=CARTESIAN_POINT('Ctrl Pts',(57.2858429174062,45.4713264567063,0.));
#168110=CARTESIAN_POINT('Ctrl Pts',(57.2608995116733,45.4641055528141,0.));
#168111=CARTESIAN_POINT('Ctrl Pts',(57.2359995706447,45.4568719595642,0.));
#168112=CARTESIAN_POINT('Ctrl Pts',(57.2111431748631,45.4496257543759,0.));
#168113=CARTESIAN_POINT('Ctrl Pts',(57.186330405101,45.4423670150034,0.));
#168114=CARTESIAN_POINT('Ctrl Pts',(57.1615613423584,45.4350958195434,0.));
#168115=CARTESIAN_POINT('Ctrl Pts',(57.136836067863,45.4278122464389,0.));
#168116=CARTESIAN_POINT('Ctrl Pts',(57.112154663078,45.4205163744782,0.));
#168117=CARTESIAN_POINT('Ctrl Pts',(57.0875172097051,45.4132082827948,0.));
#168118=CARTESIAN_POINT('Ctrl Pts',(57.0629237896848,45.4058880508693,0.));
#168119=CARTESIAN_POINT('Ctrl Pts',(57.0383744851913,45.3985557585311,0.));
#168120=CARTESIAN_POINT('Ctrl Pts',(57.0138693786278,45.3912114859616,0.));
#168121=CARTESIAN_POINT('Ctrl Pts',(56.9894085526373,45.3838553136948,0.));
#168122=CARTESIAN_POINT('Ctrl Pts',(56.9649920901073,45.3764873226196,0.));
#168123=CARTESIAN_POINT('Ctrl Pts',(56.9406200741714,45.3691075939827,0.));
#168124=CARTESIAN_POINT('Ctrl Pts',(56.9162925882085,45.3617162093923,0.));
#168125=CARTESIAN_POINT('Ctrl Pts',(56.8920097158377,45.3543132508239,0.));
#168126=CARTESIAN_POINT('Ctrl Pts',(56.8677715409268,45.3468988006203,0.));
#168127=CARTESIAN_POINT('Ctrl Pts',(56.8435781475981,45.3394729414931,0.));
#168128=CARTESIAN_POINT('Ctrl Pts',(56.8194296202291,45.332035756524,0.));
#168129=CARTESIAN_POINT('Ctrl Pts',(56.7953260434524,45.3245873291684,0.));
#168130=CARTESIAN_POINT('Ctrl Pts',(56.7712675021491,45.31712774326,0.));
#168131=CARTESIAN_POINT('Ctrl Pts',(56.7472540814553,45.3096570830118,0.));
#168132=CARTESIAN_POINT('Ctrl Pts',(56.7232858667709,45.3021754330179,0.));
#168133=CARTESIAN_POINT('Ctrl Pts',(56.69936294376,45.2946828782559,0.));
#168134=CARTESIAN_POINT('Ctrl Pts',(56.6754853983528,45.2871795040906,0.));
#168135=CARTESIAN_POINT('Ctrl Pts',(56.6516533167384,45.2796653962785,0.));
#168136=CARTESIAN_POINT('Ctrl Pts',(56.6278667853702,45.2721406409695,0.));
#168137=CARTESIAN_POINT('Ctrl Pts',(56.6041258909741,45.2646053247087,0.));
#168138=CARTESIAN_POINT('Ctrl Pts',(56.5804307205505,45.257059534438,0.));
#168139=CARTESIAN_POINT('Ctrl Pts',(56.5567813613756,45.2495033575,0.));
#168140=CARTESIAN_POINT('Ctrl Pts',(56.5331779009958,45.2419368816429,0.));
#168141=CARTESIAN_POINT('Ctrl Pts',(56.5096204272306,45.2343601950228,0.));
#168142=CARTESIAN_POINT('Ctrl Pts',(56.4861090281823,45.2267733862049,0.));
#168143=CARTESIAN_POINT('Ctrl Pts',(56.4626437922386,45.2191765441667,0.));
#168144=CARTESIAN_POINT('Ctrl Pts',(56.4392248080732,45.2115697583001,0.));
#168145=CARTESIAN_POINT('Ctrl Pts',(56.4158521646411,45.2039531184172,0.));
#168146=CARTESIAN_POINT('Ctrl Pts',(56.3925259511806,45.1963267147529,0.));
#168147=CARTESIAN_POINT('Ctrl Pts',(56.3692462572231,45.1886906379667,0.));
#168148=CARTESIAN_POINT('Ctrl Pts',(56.3460131725964,45.1810449791453,0.));
#168149=CARTESIAN_POINT('Ctrl Pts',(56.3228267874264,45.1733898298061,0.));
#168150=CARTESIAN_POINT('Ctrl Pts',(56.2996871921316,45.1657252819013,0.));
#168151=CARTESIAN_POINT('Ctrl Pts',(56.2765944774245,45.1580514278223,0.));
#168152=CARTESIAN_POINT('Ctrl Pts',(56.2535487343221,45.1503683604005,0.));
#168153=CARTESIAN_POINT('Ctrl Pts',(56.2305500541489,45.1426761729105,0.));
#168154=CARTESIAN_POINT('Ctrl Pts',(56.2075985285393,45.1349749590738,0.));
#168155=CARTESIAN_POINT('Ctrl Pts',(56.1846942494325,45.127264813063,0.));
#168156=CARTESIAN_POINT('Ctrl Pts',(56.1618373090732,45.1195458295063,0.));
#168157=CARTESIAN_POINT('Ctrl Pts',(56.1390278000226,45.1118181034888,0.));
#168158=CARTESIAN_POINT('Ctrl Pts',(56.116265815162,45.1040817305561,0.));
#168159=CARTESIAN_POINT('Ctrl Pts',(56.0935514476945,45.0963368067177,0.));
#168160=CARTESIAN_POINT('Ctrl Pts',(56.0708847911416,45.0885834284517,0.));
#168161=CARTESIAN_POINT('Ctrl Pts',(56.048265939342,45.0808216927089,0.));
#168162=CARTESIAN_POINT('Ctrl Pts',(56.0256949864639,45.0730516969149,0.));
#168163=CARTESIAN_POINT('Ctrl Pts',(56.003172027008,45.0652735389733,0.));
#168164=CARTESIAN_POINT('Ctrl Pts',(55.9806971558097,45.0574873172695,0.));
#168165=CARTESIAN_POINT('Ctrl Pts',(55.9582704680356,45.0496931306755,0.));
#168166=CARTESIAN_POINT('Ctrl Pts',(55.9358920591837,45.0418910785551,0.));
#168167=CARTESIAN_POINT('Ctrl Pts',(55.9135620250954,45.0340812607657,0.));
#168168=CARTESIAN_POINT('Ctrl Pts',(55.8912804619577,45.0262637776615,0.));
#168169=CARTESIAN_POINT('Ctrl Pts',(55.8690474663065,45.0184387300973,0.));
#168170=CARTESIAN_POINT('Ctrl Pts',(55.8468631350218,45.0106062194342,0.));
#168171=CARTESIAN_POINT('Ctrl Pts',(55.8247275653289,45.0027663475433,0.));
#168172=CARTESIAN_POINT('Ctrl Pts',(55.8026408548105,44.9949192168093,0.));
#168173=CARTESIAN_POINT('Ctrl Pts',(55.7806031014106,44.9870649301342,0.));
#168174=CARTESIAN_POINT('Ctrl Pts',(55.7586144034367,44.9792035909413,0.));
#168175=CARTESIAN_POINT('Ctrl Pts',(55.7366748595551,44.9713353031804,0.));
#168176=CARTESIAN_POINT('Ctrl Pts',(55.714784568793,44.9634601713321,0.));
#168177=CARTESIAN_POINT('Ctrl Pts',(55.6929436305489,44.9555783004106,0.));
#168178=CARTESIAN_POINT('Ctrl Pts',(55.6711521445979,44.9476897959685,0.));
#168179=CARTESIAN_POINT('Ctrl Pts',(55.6494102110935,44.9397947641007,0.));
#168180=CARTESIAN_POINT('Ctrl Pts',(55.6277179305633,44.9318933114507,0.));
#168181=CARTESIAN_POINT('Ctrl Pts',(55.6060754039121,44.9239855452144,0.));
#168182=CARTESIAN_POINT('Ctrl Pts',(55.5844827324338,44.9160715731443,0.));
#168183=CARTESIAN_POINT('Ctrl Pts',(55.5629400178142,44.908151503553,0.));
#168184=CARTESIAN_POINT('Ctrl Pts',(55.541447362134,44.9002254453183,0.));
#168185=CARTESIAN_POINT('Ctrl Pts',(55.5200048678629,44.8922935078889,0.));
#168186=CARTESIAN_POINT('Ctrl Pts',(55.4986126378656,44.8843558012886,0.));
#168187=CARTESIAN_POINT('Ctrl Pts',(55.4772707754126,44.8764124361207,0.));
#168188=CARTESIAN_POINT('Ctrl Pts',(55.4559793841836,44.8684635235725,0.));
#168189=CARTESIAN_POINT('Ctrl Pts',(55.4347385682704,44.8605091754214,0.));
#168190=CARTESIAN_POINT('Ctrl Pts',(55.4135484321718,44.8525495040408,0.));
#168191=CARTESIAN_POINT('Ctrl Pts',(55.3924090808014,44.8445846224044,0.));
#168192=CARTESIAN_POINT('Ctrl Pts',(55.3713206194967,44.8366146440901,0.));
#168193=CARTESIAN_POINT('Ctrl Pts',(55.3502831540228,44.8286396832848,0.));
#168194=CARTESIAN_POINT('Ctrl Pts',(55.3292967905725,44.8206598547888,0.));
#168195=CARTESIAN_POINT('Ctrl Pts',(55.3083616357605,44.8126752740208,0.));
#168196=CARTESIAN_POINT('Ctrl Pts',(55.287477796635,44.8046860570244,0.));
#168197=CARTESIAN_POINT('Ctrl Pts',(55.2666453806883,44.796692320474,0.));
#168198=CARTESIAN_POINT('Ctrl Pts',(55.2458644958617,44.7886941816823,0.));
#168199=CARTESIAN_POINT('Ctrl Pts',(55.2251352505474,44.7806917586077,0.));
#168200=CARTESIAN_POINT('Ctrl Pts',(55.2044577535865,44.7726851698618,0.));
#168201=CARTESIAN_POINT('Ctrl Pts',(55.1838321142777,44.7646745347108,0.));
#168202=CARTESIAN_POINT('Ctrl Pts',(55.1632584423813,44.7566599730771,0.));
#168203=CARTESIAN_POINT('Ctrl Pts',(55.1427368481201,44.748641605542,0.));
#168204=CARTESIAN_POINT('Ctrl Pts',(55.1222674421747,44.7406195533483,0.));
#168205=CARTESIAN_POINT('Ctrl Pts',(55.1018503356806,44.7325939384042,0.));
#168206=CARTESIAN_POINT('Ctrl Pts',(55.0814856402507,44.7245648832988,0.));
#168207=CARTESIAN_POINT('Ctrl Pts',(55.0611734679902,44.7165325113165,0.));
#168208=CARTESIAN_POINT('Ctrl Pts',(55.0409139315074,44.7084969464509,0.));
#168209=CARTESIAN_POINT('Ctrl Pts',(55.020707143922,44.7004583134235,0.));
#168210=CARTESIAN_POINT('Ctrl Pts',(55.0005532188644,44.6924167376851,0.));
#168211=CARTESIAN_POINT('Ctrl Pts',(54.9804522704668,44.6843723453985,0.));
#168212=CARTESIAN_POINT('Ctrl Pts',(54.9604044133497,44.6763252634255,0.));
#168213=CARTESIAN_POINT('Ctrl Pts',(54.9404097626088,44.6682756193156,0.));
#168214=CARTESIAN_POINT('Ctrl Pts',(54.9204684337845,44.6602235412854,0.));
#168215=CARTESIAN_POINT('Ctrl Pts',(54.9005805428991,44.6521691582551,0.));
#168216=CARTESIAN_POINT('Ctrl Pts',(54.8807462065177,44.6441125999074,0.));
#168217=CARTESIAN_POINT('Ctrl Pts',(54.860965541796,44.6360539967392,0.));
#168218=CARTESIAN_POINT('Ctrl Pts',(54.8412386665264,44.6279934801159,0.));
#168219=CARTESIAN_POINT('Ctrl Pts',(54.8215656991817,44.6199311823276,0.));
#168220=CARTESIAN_POINT('Ctrl Pts',(54.8019467588257,44.6118672364889,0.));
#168221=CARTESIAN_POINT('Ctrl Pts',(54.7823819650137,44.60380177643,0.));
#168222=CARTESIAN_POINT('Ctrl Pts',(54.7628714377041,44.5957349366062,0.));
#168223=CARTESIAN_POINT('Ctrl Pts',(54.7434152971285,44.5876668519676,0.));
#168224=CARTESIAN_POINT('Ctrl Pts',(54.7240136637744,44.5795976579476,0.));
#168225=CARTESIAN_POINT('Ctrl Pts',(54.7046666586776,44.5715274907637,0.));
#168226=CARTESIAN_POINT('Ctrl Pts',(54.685374403676,44.563456487687,0.));
#168227=CARTESIAN_POINT('Ctrl Pts',(54.6661370216242,44.5553847872712,0.));
#168228=CARTESIAN_POINT('Ctrl Pts',(54.6469546367381,44.5473125297289,0.));
#168229=CARTESIAN_POINT('Ctrl Pts',(54.6278273743554,44.5392398566775,0.));
#168230=CARTESIAN_POINT('Ctrl Pts',(54.6087553602889,44.5311669104495,0.));
#168231=CARTESIAN_POINT('Ctrl Pts',(54.5897387202812,44.5230938335165,0.));
#168232=CARTESIAN_POINT('Ctrl Pts',(54.5707775794436,44.5150207679007,0.));
#168233=CARTESIAN_POINT('Ctrl Pts',(54.5518720616056,44.5069478544977,0.));
#168234=CARTESIAN_POINT('Ctrl Pts',(54.5330222905475,44.4988752343744,0.));
#168235=CARTESIAN_POINT('Ctrl Pts',(54.5142283914704,44.4908030503225,0.));
#168236=CARTESIAN_POINT('Ctrl Pts',(54.495490492193,44.4827314481264,0.));
#168237=CARTESIAN_POINT('Ctrl Pts',(54.4768087248824,44.4746605784031,0.));
#168238=CARTESIAN_POINT('Ctrl Pts',(54.4581832262033,44.4665905967668,0.));
#168239=CARTESIAN_POINT('Ctrl Pts',(54.4396141336978,44.4585216599908,0.));
#168240=CARTESIAN_POINT('Ctrl Pts',(54.421101582595,44.4504539226328,0.));
#168241=CARTESIAN_POINT('Ctrl Pts',(54.4026457030335,44.4423875340996,0.));
#168242=CARTESIAN_POINT('Ctrl Pts',(54.3842466156196,44.4343226339593,0.));
#168243=CARTESIAN_POINT('Ctrl Pts',(54.3659044357119,44.4262593564712,0.));
#168244=CARTESIAN_POINT('Ctrl Pts',(54.3476192819352,44.4181978395851,0.));
#168245=CARTESIAN_POINT('Ctrl Pts',(54.3293912830237,44.4101382321834,0.));
#168246=CARTESIAN_POINT('Ctrl Pts',(54.3112205860716,44.402080702809,0.));
#168247=CARTESIAN_POINT('Ctrl Pts',(54.2931073621553,44.3940254456331,0.));
#168248=CARTESIAN_POINT('Ctrl Pts',(54.2750517888579,44.3859726620183,0.));
#168249=CARTESIAN_POINT('Ctrl Pts',(54.2570540336475,44.3779225430406,0.));
#168250=CARTESIAN_POINT('Ctrl Pts',(54.2391142386412,44.3698752533562,0.));
#168251=CARTESIAN_POINT('Ctrl Pts',(54.2212325006052,44.361830910343,0.));
#168252=CARTESIAN_POINT('Ctrl Pts',(54.2034088701928,44.3537895824096,0.));
#168253=CARTESIAN_POINT('Ctrl Pts',(54.1891964684727,44.3473589597726,0.));
#168254=CARTESIAN_POINT('Ctrl Pts',(54.1785633257639,44.3425373700993,0.));
#168255=CARTESIAN_POINT('Ctrl Pts',(54.1714861895346,44.3393235891075,0.));
#168256=CARTESIAN_POINT('Ctrl Pts',(54.1679505278134,44.3377168516418,0.));
#168257=CARTESIAN_POINT('Ctrl Pts',(62.494763006804,40.554341280847,0.));
#168258=CARTESIAN_POINT('Ctrl Pts',(62.494763006804,40.554341280847,12.));
#168259=CARTESIAN_POINT('Ctrl Pts',(62.489224912198,40.5535399497519,0.));
#168260=CARTESIAN_POINT('Ctrl Pts',(62.489224912198,40.5535399497519,12.));
#168261=CARTESIAN_POINT('Ctrl Pts',(62.4781525156318,40.5519353177252,0.));
#168262=CARTESIAN_POINT('Ctrl Pts',(62.4781525156318,40.5519353177252,12.));
#168263=CARTESIAN_POINT('Ctrl Pts',(62.4615552987202,40.5495224601758,0.));
#168264=CARTESIAN_POINT('Ctrl Pts',(62.4615552987202,40.5495224601758,12.));
#168265=CARTESIAN_POINT('Ctrl Pts',(62.4394484329678,40.5462934972718,0.));
#168266=CARTESIAN_POINT('Ctrl Pts',(62.4394484329678,40.5462934972718,12.));
#168267=CARTESIAN_POINT('Ctrl Pts',(62.4118527881148,40.5422375945026,0.));
#168268=CARTESIAN_POINT('Ctrl Pts',(62.4118527881148,40.5422375945026,12.));
#168269=CARTESIAN_POINT('Ctrl Pts',(62.3842950992833,40.5381619974169,0.));
#168270=CARTESIAN_POINT('Ctrl Pts',(62.3842950992833,40.5381619974169,12.));
#168271=CARTESIAN_POINT('Ctrl Pts',(62.3567753970279,40.5340667194319,0.));
#168272=CARTESIAN_POINT('Ctrl Pts',(62.3567753970279,40.5340667194319,12.));
#168273=CARTESIAN_POINT('Ctrl Pts',(62.3292937257901,40.5299517857721,0.));
#168274=CARTESIAN_POINT('Ctrl Pts',(62.3292937257901,40.5299517857721,12.));
#168275=CARTESIAN_POINT('Ctrl Pts',(62.301850147165,40.5258172381428,0.));
#168276=CARTESIAN_POINT('Ctrl Pts',(62.301850147165,40.5258172381428,12.));
#168277=CARTESIAN_POINT('Ctrl Pts',(62.2744447381971,40.5216631336193,0.));
#168278=CARTESIAN_POINT('Ctrl Pts',(62.2744447381971,40.5216631336193,12.));
#168279=CARTESIAN_POINT('Ctrl Pts',(62.247077585866,40.5174895390954,0.));
#168280=CARTESIAN_POINT('Ctrl Pts',(62.247077585866,40.5174895390954,12.));
#168281=CARTESIAN_POINT('Ctrl Pts',(62.2197487826136,40.5132965269633,0.));
#168282=CARTESIAN_POINT('Ctrl Pts',(62.2197487826136,40.5132965269633,12.));
#168283=CARTESIAN_POINT('Ctrl Pts',(62.1924584215653,40.5090841704122,0.));
#168284=CARTESIAN_POINT('Ctrl Pts',(62.1924584215653,40.5090841704122,12.));
#168285=CARTESIAN_POINT('Ctrl Pts',(62.1652065915808,40.5048525386035,0.));
#168286=CARTESIAN_POINT('Ctrl Pts',(62.1652065915808,40.5048525386035,12.));
#168287=CARTESIAN_POINT('Ctrl Pts',(62.1379933732528,40.5006016927554,0.));
#168288=CARTESIAN_POINT('Ctrl Pts',(62.1379933732528,40.5006016927554,12.));
#168289=CARTESIAN_POINT('Ctrl Pts',(62.1108188417003,40.4963316888412,0.));
#168290=CARTESIAN_POINT('Ctrl Pts',(62.1108188417003,40.4963316888412,12.));
#168291=CARTESIAN_POINT('Ctrl Pts',(62.0836830685719,40.4920425795217,0.));
#168292=CARTESIAN_POINT('Ctrl Pts',(62.0836830685719,40.4920425795217,12.));
#168293=CARTESIAN_POINT('Ctrl Pts',(62.0565861244179,40.4877344164411,0.));
#168294=CARTESIAN_POINT('Ctrl Pts',(62.0565861244179,40.4877344164411,12.));
#168295=CARTESIAN_POINT('Ctrl Pts',(62.029528080742,40.4834072522164,0.));
#168296=CARTESIAN_POINT('Ctrl Pts',(62.029528080742,40.4834072522164,12.));
#168297=CARTESIAN_POINT('Ctrl Pts',(62.0025090125959,40.4790611429583,0.));
#168298=CARTESIAN_POINT('Ctrl Pts',(62.0025090125959,40.4790611429583,12.));
#168299=CARTESIAN_POINT('Ctrl Pts',(61.9755289983044,40.4746961480015,0.));
#168300=CARTESIAN_POINT('Ctrl Pts',(61.9755289983044,40.4746961480015,12.));
#168301=CARTESIAN_POINT('Ctrl Pts',(61.9485881182921,40.4703123287621,0.));
#168302=CARTESIAN_POINT('Ctrl Pts',(61.9485881182921,40.4703123287621,12.));
#168303=CARTESIAN_POINT('Ctrl Pts',(61.9216864541744,40.4659097478587,0.));
#168304=CARTESIAN_POINT('Ctrl Pts',(61.9216864541744,40.4659097478587,12.));
#168305=CARTESIAN_POINT('Ctrl Pts',(61.8948240878008,40.4614884681889,0.));
#168306=CARTESIAN_POINT('Ctrl Pts',(61.8948240878008,40.4614884681889,12.));
#168307=CARTESIAN_POINT('Ctrl Pts',(61.8680011001537,40.4570485518749,0.));
#168308=CARTESIAN_POINT('Ctrl Pts',(61.8680011001537,40.4570485518749,12.));
#168309=CARTESIAN_POINT('Ctrl Pts',(61.8412175708552,40.4525900597894,0.));
#168310=CARTESIAN_POINT('Ctrl Pts',(61.8412175708552,40.4525900597894,12.));
#168311=CARTESIAN_POINT('Ctrl Pts',(61.814473578779,40.4481130521364,0.));
#168312=CARTESIAN_POINT('Ctrl Pts',(61.814473578779,40.4481130521364,12.));
#168313=CARTESIAN_POINT('Ctrl Pts',(61.7877692024076,40.4436175887949,0.));
#168314=CARTESIAN_POINT('Ctrl Pts',(61.7877692024076,40.4436175887949,12.));
#168315=CARTESIAN_POINT('Ctrl Pts',(61.7611045202874,40.4391037297589,0.));
#168316=CARTESIAN_POINT('Ctrl Pts',(61.7611045202874,40.4391037297589,12.));
#168317=CARTESIAN_POINT('Ctrl Pts',(61.7344796114399,40.4345715355405,0.));
#168318=CARTESIAN_POINT('Ctrl Pts',(61.7344796114399,40.4345715355405,12.));
#168319=CARTESIAN_POINT('Ctrl Pts',(61.7078945557799,40.430021067584,0.));
#168320=CARTESIAN_POINT('Ctrl Pts',(61.7078945557799,40.430021067584,12.));
#168321=CARTESIAN_POINT('Ctrl Pts',(61.6813494339286,40.425452388076,0.));
#168322=CARTESIAN_POINT('Ctrl Pts',(61.6813494339286,40.425452388076,12.));
#168323=CARTESIAN_POINT('Ctrl Pts',(61.6548443270394,40.4208655597717,0.));
#168324=CARTESIAN_POINT('Ctrl Pts',(61.6548443270394,40.4208655597717,12.));
#168325=CARTESIAN_POINT('Ctrl Pts',(61.628379316608,40.4162606458119,0.));
#168326=CARTESIAN_POINT('Ctrl Pts',(61.628379316608,40.4162606458119,12.));
#168327=CARTESIAN_POINT('Ctrl Pts',(61.601954484301,40.4116377095596,0.));
#168328=CARTESIAN_POINT('Ctrl Pts',(61.601954484301,40.4116377095596,12.));
#168329=CARTESIAN_POINT('Ctrl Pts',(61.5755699117324,40.4069968143956,0.));
#168330=CARTESIAN_POINT('Ctrl Pts',(61.5755699117324,40.4069968143956,12.));
#168331=CARTESIAN_POINT('Ctrl Pts',(61.5492256804717,40.4023380237232,0.));
#168332=CARTESIAN_POINT('Ctrl Pts',(61.5492256804717,40.4023380237232,12.));
#168333=CARTESIAN_POINT('Ctrl Pts',(61.522921872154,40.3976614010652,0.));
#168334=CARTESIAN_POINT('Ctrl Pts',(61.522921872154,40.3976614010652,12.));
#168335=CARTESIAN_POINT('Ctrl Pts',(61.4966585685549,40.3929670101366,0.));
#168336=CARTESIAN_POINT('Ctrl Pts',(61.4966585685549,40.3929670101366,12.));
#168337=CARTESIAN_POINT('Ctrl Pts',(61.4704358516709,40.3882549149228,0.));
#168338=CARTESIAN_POINT('Ctrl Pts',(61.4704358516709,40.3882549149228,12.));
#168339=CARTESIAN_POINT('Ctrl Pts',(61.4442538038044,40.383525179772,0.));
#168340=CARTESIAN_POINT('Ctrl Pts',(61.4442538038044,40.383525179772,12.));
#168341=CARTESIAN_POINT('Ctrl Pts',(61.4181125076037,40.3787778694364,0.));
#168342=CARTESIAN_POINT('Ctrl Pts',(61.4181125076037,40.3787778694364,12.));
#168343=CARTESIAN_POINT('Ctrl Pts',(61.3920120460219,40.3740130490225,0.));
#168344=CARTESIAN_POINT('Ctrl Pts',(61.3920120460219,40.3740130490225,12.));
#168345=CARTESIAN_POINT('Ctrl Pts',(61.3659525022908,40.3692307839636,0.));
#168346=CARTESIAN_POINT('Ctrl Pts',(61.3659525022908,40.3692307839636,12.));
#168347=CARTESIAN_POINT('Ctrl Pts',(61.3399339598853,40.3644311399861,0.));
#168348=CARTESIAN_POINT('Ctrl Pts',(61.3399339598853,40.3644311399861,12.));
#168349=CARTESIAN_POINT('Ctrl Pts',(61.3139565024847,40.3596141830791,0.));
#168350=CARTESIAN_POINT('Ctrl Pts',(61.3139565024847,40.3596141830791,12.));
#168351=CARTESIAN_POINT('Ctrl Pts',(61.2880202139371,40.3547799794679,0.));
#168352=CARTESIAN_POINT('Ctrl Pts',(61.2880202139371,40.3547799794679,12.));
#168353=CARTESIAN_POINT('Ctrl Pts',(61.2621251782863,40.3499285956304,0.));
#168354=CARTESIAN_POINT('Ctrl Pts',(61.2621251782863,40.3499285956304,12.));
#168355=CARTESIAN_POINT('Ctrl Pts',(61.23627147979,40.3450600983109,0.));
#168356=CARTESIAN_POINT('Ctrl Pts',(61.23627147979,40.3450600983109,12.));
#168357=CARTESIAN_POINT('Ctrl Pts',(61.2104592029377,40.340174554537,0.));
#168358=CARTESIAN_POINT('Ctrl Pts',(61.2104592029377,40.340174554537,12.));
#168359=CARTESIAN_POINT('Ctrl Pts',(61.1846884324644,40.335272031637,0.));
#168360=CARTESIAN_POINT('Ctrl Pts',(61.1846884324644,40.335272031637,12.));
#168361=CARTESIAN_POINT('Ctrl Pts',(61.1589592533613,40.3303525972615,0.));
#168362=CARTESIAN_POINT('Ctrl Pts',(61.1589592533613,40.3303525972615,12.));
#168363=CARTESIAN_POINT('Ctrl Pts',(61.1332717508789,40.32541631938,0.));
#168364=CARTESIAN_POINT('Ctrl Pts',(61.1332717508789,40.32541631938,12.));
#168365=CARTESIAN_POINT('Ctrl Pts',(61.1076260105258,40.3204632662725,0.));
#168366=CARTESIAN_POINT('Ctrl Pts',(61.1076260105258,40.3204632662725,12.));
#168367=CARTESIAN_POINT('Ctrl Pts',(61.0820221180645,40.3154935065262,0.));
#168368=CARTESIAN_POINT('Ctrl Pts',(61.0820221180645,40.3154935065262,12.));
#168369=CARTESIAN_POINT('Ctrl Pts',(61.056460159505,40.310507109031,0.));
#168370=CARTESIAN_POINT('Ctrl Pts',(61.056460159505,40.310507109031,12.));
#168371=CARTESIAN_POINT('Ctrl Pts',(61.0309402210921,40.3055041429775,0.));
#168372=CARTESIAN_POINT('Ctrl Pts',(61.0309402210921,40.3055041429775,12.));
#168373=CARTESIAN_POINT('Ctrl Pts',(61.0054623893066,40.300484677858,0.));
#168374=CARTESIAN_POINT('Ctrl Pts',(61.0054623893066,40.300484677858,12.));
#168375=CARTESIAN_POINT('Ctrl Pts',(60.9800267508786,40.295448783469,0.));
#168376=CARTESIAN_POINT('Ctrl Pts',(60.9800267508786,40.295448783469,12.));
#168377=CARTESIAN_POINT('Ctrl Pts',(60.9546333927921,40.2903965299155,0.));
#168378=CARTESIAN_POINT('Ctrl Pts',(60.9546333927921,40.2903965299155,12.));
#168379=CARTESIAN_POINT('Ctrl Pts',(60.9292824022887,40.2853279876161,0.));
#168380=CARTESIAN_POINT('Ctrl Pts',(60.9292824022887,40.2853279876161,12.));
#168381=CARTESIAN_POINT('Ctrl Pts',(60.9039738668669,40.2802432273104,0.));
#168382=CARTESIAN_POINT('Ctrl Pts',(60.9039738668669,40.2802432273104,12.));
#168383=CARTESIAN_POINT('Ctrl Pts',(60.8787078742818,40.2751423200639,0.));
#168384=CARTESIAN_POINT('Ctrl Pts',(60.8787078742818,40.2751423200639,12.));
#168385=CARTESIAN_POINT('Ctrl Pts',(60.8534845125538,40.2700253372648,0.));
#168386=CARTESIAN_POINT('Ctrl Pts',(60.8534845125538,40.2700253372648,12.));
#168387=CARTESIAN_POINT('Ctrl Pts',(60.8283038699706,40.2648923506248,0.));
#168388=CARTESIAN_POINT('Ctrl Pts',(60.8283038699706,40.2648923506248,12.));
#168389=CARTESIAN_POINT('Ctrl Pts',(60.8031660350879,40.2597434321803,0.));
#168390=CARTESIAN_POINT('Ctrl Pts',(60.8031660350879,40.2597434321803,12.));
#168391=CARTESIAN_POINT('Ctrl Pts',(60.7780710967248,40.2545786542953,0.));
#168392=CARTESIAN_POINT('Ctrl Pts',(60.7780710967248,40.2545786542953,12.));
#168393=CARTESIAN_POINT('Ctrl Pts',(60.7530191439593,40.2493980896638,0.));
#168394=CARTESIAN_POINT('Ctrl Pts',(60.7530191439593,40.2493980896638,12.));
#168395=CARTESIAN_POINT('Ctrl Pts',(60.728010266139,40.2442018113108,0.));
#168396=CARTESIAN_POINT('Ctrl Pts',(60.728010266139,40.2442018113108,12.));
#168397=CARTESIAN_POINT('Ctrl Pts',(60.7030445528857,40.2389898925932,0.));
#168398=CARTESIAN_POINT('Ctrl Pts',(60.7030445528857,40.2389898925932,12.));
#168399=CARTESIAN_POINT('Ctrl Pts',(60.678122094098,40.2337624072029,0.));
#168400=CARTESIAN_POINT('Ctrl Pts',(60.678122094098,40.2337624072029,12.));
#168401=CARTESIAN_POINT('Ctrl Pts',(60.6532429799499,40.2285194291706,0.));
#168402=CARTESIAN_POINT('Ctrl Pts',(60.6532429799499,40.2285194291706,12.));
#168403=CARTESIAN_POINT('Ctrl Pts',(60.6284073008871,40.2232610328721,0.));
#168404=CARTESIAN_POINT('Ctrl Pts',(60.6284073008871,40.2232610328721,12.));
#168405=CARTESIAN_POINT('Ctrl Pts',(60.6036151476349,40.2179872930273,0.));
#168406=CARTESIAN_POINT('Ctrl Pts',(60.6036151476349,40.2179872930273,12.));
#168407=CARTESIAN_POINT('Ctrl Pts',(60.5788666112042,40.2126982847011,0.));
#168408=CARTESIAN_POINT('Ctrl Pts',(60.5788666112042,40.2126982847011,12.));
#168409=CARTESIAN_POINT('Ctrl Pts',(60.5541617828925,40.2073940833053,0.));
#168410=CARTESIAN_POINT('Ctrl Pts',(60.5541617828925,40.2073940833053,12.));
#168411=CARTESIAN_POINT('Ctrl Pts',(60.5295007542841,40.2020747646014,0.));
#168412=CARTESIAN_POINT('Ctrl Pts',(60.5295007542841,40.2020747646014,12.));
#168413=CARTESIAN_POINT('Ctrl Pts',(60.5048836172435,40.1967404047062,0.));
#168414=CARTESIAN_POINT('Ctrl Pts',(60.5048836172435,40.1967404047062,12.));
#168415=CARTESIAN_POINT('Ctrl Pts',(60.4803104639225,40.1913910800921,0.));
#168416=CARTESIAN_POINT('Ctrl Pts',(60.4803104639225,40.1913910800921,12.));
#168417=CARTESIAN_POINT('Ctrl Pts',(60.455781386769,40.1860268675884,0.));
#168418=CARTESIAN_POINT('Ctrl Pts',(60.455781386769,40.1860268675884,12.));
#168419=CARTESIAN_POINT('Ctrl Pts',(60.4312964785273,40.180647844383,0.));
#168420=CARTESIAN_POINT('Ctrl Pts',(60.4312964785273,40.180647844383,12.));
#168421=CARTESIAN_POINT('Ctrl Pts',(60.4068558322407,40.1752540880268,0.));
#168422=CARTESIAN_POINT('Ctrl Pts',(60.4068558322407,40.1752540880268,12.));
#168423=CARTESIAN_POINT('Ctrl Pts',(60.3824595412445,40.1698456764377,0.));
#168424=CARTESIAN_POINT('Ctrl Pts',(60.3824595412445,40.1698456764377,12.));
#168425=CARTESIAN_POINT('Ctrl Pts',(60.3581076991716,40.1644226879033,0.));
#168426=CARTESIAN_POINT('Ctrl Pts',(60.3581076991716,40.1644226879033,12.));
#168427=CARTESIAN_POINT('Ctrl Pts',(60.3338003999607,40.1589852010804,0.));
#168428=CARTESIAN_POINT('Ctrl Pts',(60.3338003999607,40.1589852010804,12.));
#168429=CARTESIAN_POINT('Ctrl Pts',(60.3095377378586,40.1535332949976,0.));
#168430=CARTESIAN_POINT('Ctrl Pts',(60.3095377378586,40.1535332949976,12.));
#168431=CARTESIAN_POINT('Ctrl Pts',(60.285319807422,40.1480670490586,0.));
#168432=CARTESIAN_POINT('Ctrl Pts',(60.285319807422,40.1480670490586,12.));
#168433=CARTESIAN_POINT('Ctrl Pts',(60.2611467035116,40.1425865430472,0.));
#168434=CARTESIAN_POINT('Ctrl Pts',(60.2611467035116,40.1425865430472,12.));
#168435=CARTESIAN_POINT('Ctrl Pts',(60.2370185212964,40.1370918571304,0.));
#168436=CARTESIAN_POINT('Ctrl Pts',(60.2370185212964,40.1370918571304,12.));
#168437=CARTESIAN_POINT('Ctrl Pts',(60.2129353562622,40.1315830718577,0.));
#168438=CARTESIAN_POINT('Ctrl Pts',(60.2129353562622,40.1315830718577,12.));
#168439=CARTESIAN_POINT('Ctrl Pts',(60.1888973042152,40.1260602681644,0.));
#168440=CARTESIAN_POINT('Ctrl Pts',(60.1888973042152,40.1260602681644,12.));
#168441=CARTESIAN_POINT('Ctrl Pts',(60.1649044612828,40.1205235273739,0.));
#168442=CARTESIAN_POINT('Ctrl Pts',(60.1649044612828,40.1205235273739,12.));
#168443=CARTESIAN_POINT('Ctrl Pts',(60.1409569239092,40.1149729312036,0.));
#168444=CARTESIAN_POINT('Ctrl Pts',(60.1409569239092,40.1149729312036,12.));
#168445=CARTESIAN_POINT('Ctrl Pts',(60.1170547888574,40.1094085617674,0.));
#168446=CARTESIAN_POINT('Ctrl Pts',(60.1170547888574,40.1094085617674,12.));
#168447=CARTESIAN_POINT('Ctrl Pts',(60.0931981532198,40.1038305015766,0.));
#168448=CARTESIAN_POINT('Ctrl Pts',(60.0931981532198,40.1038305015766,12.));
#168449=CARTESIAN_POINT('Ctrl Pts',(60.069387114421,40.0982388335423,0.));
#168450=CARTESIAN_POINT('Ctrl Pts',(60.069387114421,40.0982388335423,12.));
#168451=CARTESIAN_POINT('Ctrl Pts',(60.0456217702202,40.0926336409785,0.));
#168452=CARTESIAN_POINT('Ctrl Pts',(60.0456217702202,40.0926336409785,12.));
#168453=CARTESIAN_POINT('Ctrl Pts',(60.021902218706,40.0870150076074,0.));
#168454=CARTESIAN_POINT('Ctrl Pts',(60.021902218706,40.0870150076074,12.));
#168455=CARTESIAN_POINT('Ctrl Pts',(59.9982285582983,40.0813830175623,0.));
#168456=CARTESIAN_POINT('Ctrl Pts',(59.9982285582983,40.0813830175623,12.));
#168457=CARTESIAN_POINT('Ctrl Pts',(59.9746008877584,40.0757377553888,0.));
#168458=CARTESIAN_POINT('Ctrl Pts',(59.9746008877584,40.0757377553888,12.));
#168459=CARTESIAN_POINT('Ctrl Pts',(59.9510193061927,40.0700793060473,0.));
#168460=CARTESIAN_POINT('Ctrl Pts',(59.9510193061927,40.0700793060473,12.));
#168461=CARTESIAN_POINT('Ctrl Pts',(59.9274839130553,40.0644077549159,0.));
#168462=CARTESIAN_POINT('Ctrl Pts',(59.9274839130553,40.0644077549159,12.));
#168463=CARTESIAN_POINT('Ctrl Pts',(59.9039948081432,40.0587231877961,0.));
#168464=CARTESIAN_POINT('Ctrl Pts',(59.9039948081432,40.0587231877961,12.));
#168465=CARTESIAN_POINT('Ctrl Pts',(59.8805520915975,40.0530256909162,0.));
#168466=CARTESIAN_POINT('Ctrl Pts',(59.8805520915975,40.0530256909162,12.));
#168467=CARTESIAN_POINT('Ctrl Pts',(59.8571558639145,40.0473153509323,0.));
#168468=CARTESIAN_POINT('Ctrl Pts',(59.8571558639145,40.0473153509323,12.));
#168469=CARTESIAN_POINT('Ctrl Pts',(59.8338062259491,40.0415922549313,0.));
#168470=CARTESIAN_POINT('Ctrl Pts',(59.8338062259491,40.0415922549313,12.));
#168471=CARTESIAN_POINT('Ctrl Pts',(59.8105032789179,40.035856490434,0.));
#168472=CARTESIAN_POINT('Ctrl Pts',(59.8105032789179,40.035856490434,12.));
#168473=CARTESIAN_POINT('Ctrl Pts',(59.7872471243948,40.0301081454006,0.));
#168474=CARTESIAN_POINT('Ctrl Pts',(59.7872471243948,40.0301081454006,12.));
#168475=CARTESIAN_POINT('Ctrl Pts',(59.7640378643115,40.0243473082343,0.));
#168476=CARTESIAN_POINT('Ctrl Pts',(59.7640378643115,40.0243473082343,12.));
#168477=CARTESIAN_POINT('Ctrl Pts',(59.7408756009688,40.0185740677827,0.));
#168478=CARTESIAN_POINT('Ctrl Pts',(59.7408756009688,40.0185740677827,12.));
#168479=CARTESIAN_POINT('Ctrl Pts',(59.7177604370409,40.0127885133407,0.));
#168480=CARTESIAN_POINT('Ctrl Pts',(59.7177604370409,40.0127885133407,12.));
#168481=CARTESIAN_POINT('Ctrl Pts',(59.6946924755771,40.0069907346536,0.));
#168482=CARTESIAN_POINT('Ctrl Pts',(59.6946924755771,40.0069907346536,12.));
#168483=CARTESIAN_POINT('Ctrl Pts',(59.671671819999,40.0011808219231,0.));
#168484=CARTESIAN_POINT('Ctrl Pts',(59.671671819999,40.0011808219231,12.));
#168485=CARTESIAN_POINT('Ctrl Pts',(59.6486985741015,39.9953588658114,0.));
#168486=CARTESIAN_POINT('Ctrl Pts',(59.6486985741015,39.9953588658114,12.));
#168487=CARTESIAN_POINT('Ctrl Pts',(59.6257728420644,39.9895249574432,0.));
#168488=CARTESIAN_POINT('Ctrl Pts',(59.6257728420644,39.9895249574432,12.));
#168489=CARTESIAN_POINT('Ctrl Pts',(59.6028947284551,39.9836791884071,0.));
#168490=CARTESIAN_POINT('Ctrl Pts',(59.6028947284551,39.9836791884071,12.));
#168491=CARTESIAN_POINT('Ctrl Pts',(59.5800643382322,39.9778216507609,0.));
#168492=CARTESIAN_POINT('Ctrl Pts',(59.5800643382322,39.9778216507609,12.));
#168493=CARTESIAN_POINT('Ctrl Pts',(59.5572817767412,39.971952437036,0.));
#168494=CARTESIAN_POINT('Ctrl Pts',(59.5572817767412,39.971952437036,12.));
#168495=CARTESIAN_POINT('Ctrl Pts',(59.5345471497162,39.9660716402423,0.));
#168496=CARTESIAN_POINT('Ctrl Pts',(59.5345471497162,39.9660716402423,12.));
#168497=CARTESIAN_POINT('Ctrl Pts',(59.511860563292,39.96017935387,0.));
#168498=CARTESIAN_POINT('Ctrl Pts',(59.511860563292,39.96017935387,12.));
#168499=CARTESIAN_POINT('Ctrl Pts',(59.4892221240081,39.954275671893,0.));
#168500=CARTESIAN_POINT('Ctrl Pts',(59.4892221240081,39.954275671893,12.));
#168501=CARTESIAN_POINT('Ctrl Pts',(59.4666319388123,39.9483606887731,0.));
#168502=CARTESIAN_POINT('Ctrl Pts',(59.4666319388123,39.9483606887731,12.));
#168503=CARTESIAN_POINT('Ctrl Pts',(59.444090115055,39.9424344994652,0.));
#168504=CARTESIAN_POINT('Ctrl Pts',(59.444090115055,39.9424344994652,12.));
#168505=CARTESIAN_POINT('Ctrl Pts',(59.4215967604925,39.9364971994215,0.));
#168506=CARTESIAN_POINT('Ctrl Pts',(59.4215967604925,39.9364971994215,12.));
#168507=CARTESIAN_POINT('Ctrl Pts',(59.3991519832981,39.9305488845934,0.));
#168508=CARTESIAN_POINT('Ctrl Pts',(59.3991519832981,39.9305488845934,12.));
#168509=CARTESIAN_POINT('Ctrl Pts',(59.3767558920663,39.9245896514359,0.));
#168510=CARTESIAN_POINT('Ctrl Pts',(59.3767558920663,39.9245896514359,12.));
#168511=CARTESIAN_POINT('Ctrl Pts',(59.3544085958165,39.9186195969113,0.));
#168512=CARTESIAN_POINT('Ctrl Pts',(59.3544085958165,39.9186195969113,12.));
#168513=CARTESIAN_POINT('Ctrl Pts',(59.3321102039883,39.9126388184956,0.));
#168514=CARTESIAN_POINT('Ctrl Pts',(59.3321102039883,39.9126388184956,12.));
#168515=CARTESIAN_POINT('Ctrl Pts',(59.3098608264452,39.9066474141826,0.));
#168516=CARTESIAN_POINT('Ctrl Pts',(59.3098608264452,39.9066474141826,12.));
#168517=CARTESIAN_POINT('Ctrl Pts',(59.2876605734871,39.9006454824861,0.));
#168518=CARTESIAN_POINT('Ctrl Pts',(59.2876605734871,39.9006454824861,12.));
#168519=CARTESIAN_POINT('Ctrl Pts',(59.2655095558527,39.8946331224442,0.));
#168520=CARTESIAN_POINT('Ctrl Pts',(59.2655095558527,39.8946331224442,12.));
#168521=CARTESIAN_POINT('Ctrl Pts',(59.2434078847236,39.8886104336234,0.));
#168522=CARTESIAN_POINT('Ctrl Pts',(59.2434078847236,39.8886104336234,12.));
#168523=CARTESIAN_POINT('Ctrl Pts',(59.2213556717189,39.8825775161252,0.));
#168524=CARTESIAN_POINT('Ctrl Pts',(59.2213556717189,39.8825775161252,12.));
#168525=CARTESIAN_POINT('Ctrl Pts',(59.1993530289008,39.8765344705895,0.));
#168526=CARTESIAN_POINT('Ctrl Pts',(59.1993530289008,39.8765344705895,12.));
#168527=CARTESIAN_POINT('Ctrl Pts',(59.1774000687865,39.8704813981978,0.));
#168528=CARTESIAN_POINT('Ctrl Pts',(59.1774000687865,39.8704813981978,12.));
#168529=CARTESIAN_POINT('Ctrl Pts',(59.155496904352,39.8644184006785,0.));
#168530=CARTESIAN_POINT('Ctrl Pts',(59.155496904352,39.8644184006785,12.));
#168531=CARTESIAN_POINT('Ctrl Pts',(59.133643649035,39.8583455803111,0.));
#168532=CARTESIAN_POINT('Ctrl Pts',(59.133643649035,39.8583455803111,12.));
#168533=CARTESIAN_POINT('Ctrl Pts',(59.1118404167304,39.8522630399337,0.));
#168534=CARTESIAN_POINT('Ctrl Pts',(59.1118404167304,39.8522630399337,12.));
#168535=CARTESIAN_POINT('Ctrl Pts',(59.0900873217992,39.8461708829465,0.));
#168536=CARTESIAN_POINT('Ctrl Pts',(59.0900873217992,39.8461708829465,12.));
#168537=CARTESIAN_POINT('Ctrl Pts',(59.068384479077,39.8400692133143,0.));
#168538=CARTESIAN_POINT('Ctrl Pts',(59.068384479077,39.8400692133143,12.));
#168539=CARTESIAN_POINT('Ctrl Pts',(59.0467320038782,39.8339581355715,0.));
#168540=CARTESIAN_POINT('Ctrl Pts',(59.0467320038782,39.8339581355715,12.));
#168541=CARTESIAN_POINT('Ctrl Pts',(59.0251300119972,39.8278377548261,0.));
#168542=CARTESIAN_POINT('Ctrl Pts',(59.0251300119972,39.8278377548261,12.));
#168543=CARTESIAN_POINT('Ctrl Pts',(59.0035786197024,39.8217081767658,0.));
#168544=CARTESIAN_POINT('Ctrl Pts',(59.0035786197024,39.8217081767658,12.));
#168545=CARTESIAN_POINT('Ctrl Pts',(58.9820779437485,39.8155695076625,0.));
#168546=CARTESIAN_POINT('Ctrl Pts',(58.9820779437485,39.8155695076625,12.));
#168547=CARTESIAN_POINT('Ctrl Pts',(58.9606281013876,39.8094218543781,0.));
#168548=CARTESIAN_POINT('Ctrl Pts',(58.9606281013876,39.8094218543781,12.));
#168549=CARTESIAN_POINT('Ctrl Pts',(58.9392292103747,39.8032653243712,0.));
#168550=CARTESIAN_POINT('Ctrl Pts',(58.9392292103747,39.8032653243712,12.));
#168551=CARTESIAN_POINT('Ctrl Pts',(58.9178813889703,39.7971000257044,0.));
#168552=CARTESIAN_POINT('Ctrl Pts',(58.9178813889703,39.7971000257044,12.));
#168553=CARTESIAN_POINT('Ctrl Pts',(58.896584755939,39.7909260670517,0.));
#168554=CARTESIAN_POINT('Ctrl Pts',(58.896584755939,39.7909260670517,12.));
#168555=CARTESIAN_POINT('Ctrl Pts',(58.8753394305583,39.7847435576995,0.));
#168556=CARTESIAN_POINT('Ctrl Pts',(58.8753394305583,39.7847435576995,12.));
#168557=CARTESIAN_POINT('Ctrl Pts',(58.8541455326229,39.7785526075477,0.));
#168558=CARTESIAN_POINT('Ctrl Pts',(58.8541455326229,39.7785526075477,12.));
#168559=CARTESIAN_POINT('Ctrl Pts',(58.8330031824453,39.772353327112,0.));
#168560=CARTESIAN_POINT('Ctrl Pts',(58.8330031824453,39.772353327112,12.));
#168561=CARTESIAN_POINT('Ctrl Pts',(58.8119125008521,39.7661458275276,0.));
#168562=CARTESIAN_POINT('Ctrl Pts',(58.8119125008521,39.7661458275276,12.));
#168563=CARTESIAN_POINT('Ctrl Pts',(58.7908736091808,39.7599302205527,0.));
#168564=CARTESIAN_POINT('Ctrl Pts',(58.7908736091808,39.7599302205527,12.));
#168565=CARTESIAN_POINT('Ctrl Pts',(58.769886629304,39.753706618582,0.));
#168566=CARTESIAN_POINT('Ctrl Pts',(58.769886629304,39.753706618582,12.));
#168567=CARTESIAN_POINT('Ctrl Pts',(58.7489516836453,39.7474751346603,0.));
#168568=CARTESIAN_POINT('Ctrl Pts',(58.7489516836453,39.7474751346603,12.));
#168569=CARTESIAN_POINT('Ctrl Pts',(58.7280688951911,39.7412358824949,0.));
#168570=CARTESIAN_POINT('Ctrl Pts',(58.7280688951911,39.7412358824949,12.));
#168571=CARTESIAN_POINT('Ctrl Pts',(58.7072383875009,39.7349889764737,0.));
#168572=CARTESIAN_POINT('Ctrl Pts',(58.7072383875009,39.7349889764737,12.));
#168573=CARTESIAN_POINT('Ctrl Pts',(58.6864602847064,39.7287345316664,0.));
#168574=CARTESIAN_POINT('Ctrl Pts',(58.6864602847064,39.7287345316664,12.));
#168575=CARTESIAN_POINT('Ctrl Pts',(58.6657347115014,39.7224726638087,0.));
#168576=CARTESIAN_POINT('Ctrl Pts',(58.6657347115014,39.7224726638087,12.));
#168577=CARTESIAN_POINT('Ctrl Pts',(58.6450617931269,39.7162034892896,0.));
#168578=CARTESIAN_POINT('Ctrl Pts',(58.6450617931269,39.7162034892896,12.));
#168579=CARTESIAN_POINT('Ctrl Pts',(58.6244416553574,39.7099271251421,0.));
#168580=CARTESIAN_POINT('Ctrl Pts',(58.6244416553574,39.7099271251421,12.));
#168581=CARTESIAN_POINT('Ctrl Pts',(58.6038744244683,39.7036436890248,0.));
#168582=CARTESIAN_POINT('Ctrl Pts',(58.6038744244683,39.7036436890248,12.));
#168583=CARTESIAN_POINT('Ctrl Pts',(58.5833602272767,39.6973532992555,0.));
#168584=CARTESIAN_POINT('Ctrl Pts',(58.5833602272767,39.6973532992555,12.));
#168585=CARTESIAN_POINT('Ctrl Pts',(58.5628991912067,39.6910560748639,0.));
#168586=CARTESIAN_POINT('Ctrl Pts',(58.5628991912067,39.6910560748639,12.));
#168587=CARTESIAN_POINT('Ctrl Pts',(58.5424914443415,39.6847521356395,0.));
#168588=CARTESIAN_POINT('Ctrl Pts',(58.5424914443415,39.6847521356395,12.));
#168589=CARTESIAN_POINT('Ctrl Pts',(58.5221371154748,39.6784416021817,0.));
#168590=CARTESIAN_POINT('Ctrl Pts',(58.5221371154748,39.6784416021817,12.));
#168591=CARTESIAN_POINT('Ctrl Pts',(58.5018363341582,39.6721245959516,0.));
#168592=CARTESIAN_POINT('Ctrl Pts',(58.5018363341582,39.6721245959516,12.));
#168593=CARTESIAN_POINT('Ctrl Pts',(58.4815892306044,39.66580123918,0.));
#168594=CARTESIAN_POINT('Ctrl Pts',(58.4815892306044,39.66580123918,12.));
#168595=CARTESIAN_POINT('Ctrl Pts',(58.4613959355776,39.6594716547681,0.));
#168596=CARTESIAN_POINT('Ctrl Pts',(58.4613959355776,39.6594716547681,12.));
#168597=CARTESIAN_POINT('Ctrl Pts',(58.4412565802984,39.6531359662043,0.));
#168598=CARTESIAN_POINT('Ctrl Pts',(58.4412565802984,39.6531359662043,12.));
#168599=CARTESIAN_POINT('Ctrl Pts',(58.4211712963023,39.6467942974465,0.));
#168600=CARTESIAN_POINT('Ctrl Pts',(58.4211712963023,39.6467942974465,12.));
#168601=CARTESIAN_POINT('Ctrl Pts',(58.4011402154225,39.6404467729113,0.));
#168602=CARTESIAN_POINT('Ctrl Pts',(58.4011402154225,39.6404467729113,12.));
#168603=CARTESIAN_POINT('Ctrl Pts',(58.3811634701061,39.6340935177492,0.));
#168604=CARTESIAN_POINT('Ctrl Pts',(58.3811634701061,39.6340935177492,12.));
#168605=CARTESIAN_POINT('Ctrl Pts',(58.3612411936914,39.6277346580898,0.));
#168606=CARTESIAN_POINT('Ctrl Pts',(58.3612411936914,39.6277346580898,12.));
#168607=CARTESIAN_POINT('Ctrl Pts',(58.3413735206412,39.6213703212523,0.));
#168608=CARTESIAN_POINT('Ctrl Pts',(58.3413735206412,39.6213703212523,12.));
#168609=CARTESIAN_POINT('Ctrl Pts',(58.3215605869192,39.6150006360894,0.));
#168610=CARTESIAN_POINT('Ctrl Pts',(58.3215605869192,39.6150006360894,12.));
#168611=CARTESIAN_POINT('Ctrl Pts',(58.3018025297288,39.6086257327559,0.));
#168612=CARTESIAN_POINT('Ctrl Pts',(58.3018025297288,39.6086257327559,12.));
#168613=CARTESIAN_POINT('Ctrl Pts',(58.2820994868092,39.6022457420772,0.));
#168614=CARTESIAN_POINT('Ctrl Pts',(58.2820994868092,39.6022457420772,12.));
#168615=CARTESIAN_POINT('Ctrl Pts',(58.2624515958416,39.5958607950237,0.));
#168616=CARTESIAN_POINT('Ctrl Pts',(58.2624515958416,39.5958607950237,12.));
#168617=CARTESIAN_POINT('Ctrl Pts',(58.2428589938394,39.589471022173,0.));
#168618=CARTESIAN_POINT('Ctrl Pts',(58.2428589938394,39.589471022173,12.));
#168619=CARTESIAN_POINT('Ctrl Pts',(58.2233218164407,39.5830765530919,0.));
#168620=CARTESIAN_POINT('Ctrl Pts',(58.2233218164407,39.5830765530919,12.));
#168621=CARTESIAN_POINT('Ctrl Pts',(58.2038401992496,39.5766775175226,0.));
#168622=CARTESIAN_POINT('Ctrl Pts',(58.2038401992496,39.5766775175226,12.));
#168623=CARTESIAN_POINT('Ctrl Pts',(58.1844142794359,39.5702740468013,0.));
#168624=CARTESIAN_POINT('Ctrl Pts',(58.1844142794359,39.5702740468013,12.));
#168625=CARTESIAN_POINT('Ctrl Pts',(58.1650441970379,39.5638662750174,0.));
#168626=CARTESIAN_POINT('Ctrl Pts',(58.1650441970379,39.5638662750174,12.));
#168627=CARTESIAN_POINT('Ctrl Pts',(58.1457300968467,39.5574543406959,0.));
#168628=CARTESIAN_POINT('Ctrl Pts',(58.1457300968467,39.5574543406959,12.));
#168629=CARTESIAN_POINT('Ctrl Pts',(58.1264721285698,39.5510383869476,0.));
#168630=CARTESIAN_POINT('Ctrl Pts',(58.1264721285698,39.5510383869476,12.));
#168631=CARTESIAN_POINT('Ctrl Pts',(58.1072704428895,39.5446185579615,0.));
#168632=CARTESIAN_POINT('Ctrl Pts',(58.1072704428895,39.5446185579615,12.));
#168633=CARTESIAN_POINT('Ctrl Pts',(58.088125187991,39.5381949959214,0.));
#168634=CARTESIAN_POINT('Ctrl Pts',(58.088125187991,39.5381949959214,12.));
#168635=CARTESIAN_POINT('Ctrl Pts',(58.0690365065393,39.5317678383231,0.));
#168636=CARTESIAN_POINT('Ctrl Pts',(58.0690365065393,39.5317678383231,12.));
#168637=CARTESIAN_POINT('Ctrl Pts',(58.050004530846,39.5253372136921,0.));
#168638=CARTESIAN_POINT('Ctrl Pts',(58.050004530846,39.5253372136921,12.));
#168639=CARTESIAN_POINT('Ctrl Pts',(58.0310293875321,39.5189032457227,0.));
#168640=CARTESIAN_POINT('Ctrl Pts',(58.0310293875321,39.5189032457227,12.));
#168641=CARTESIAN_POINT('Ctrl Pts',(58.012111206794,39.5124660615009,0.));
#168642=CARTESIAN_POINT('Ctrl Pts',(58.012111206794,39.5124660615009,12.));
#168643=CARTESIAN_POINT('Ctrl Pts',(57.9932501298522,39.5060257981225,0.));
#168644=CARTESIAN_POINT('Ctrl Pts',(57.9932501298522,39.5060257981225,12.));
#168645=CARTESIAN_POINT('Ctrl Pts',(57.9744463179305,39.4995826106691,0.));
#168646=CARTESIAN_POINT('Ctrl Pts',(57.9744463179305,39.4995826106691,12.));
#168647=CARTESIAN_POINT('Ctrl Pts',(57.9556999583777,39.4931366776627,0.));
#168648=CARTESIAN_POINT('Ctrl Pts',(57.9556999583777,39.4931366776627,12.));
#168649=CARTESIAN_POINT('Ctrl Pts',(57.9370112456506,39.4866881842223,0.));
#168650=CARTESIAN_POINT('Ctrl Pts',(57.9370112456506,39.4866881842223,12.));
#168651=CARTESIAN_POINT('Ctrl Pts',(57.9183803632337,39.4802373061008,0.));
#168652=CARTESIAN_POINT('Ctrl Pts',(57.9183803632337,39.4802373061008,12.));
#168653=CARTESIAN_POINT('Ctrl Pts',(57.8998074670541,39.4737841949417,0.));
#168654=CARTESIAN_POINT('Ctrl Pts',(57.8998074670541,39.4737841949417,12.));
#168655=CARTESIAN_POINT('Ctrl Pts',(57.8812926637397,39.4673289592425,0.));
#168656=CARTESIAN_POINT('Ctrl Pts',(57.8812926637397,39.4673289592425,12.));
#168657=CARTESIAN_POINT('Ctrl Pts',(57.8628360097134,39.4608716627367,0.));
#168658=CARTESIAN_POINT('Ctrl Pts',(57.8628360097134,39.4608716627367,12.));
#168659=CARTESIAN_POINT('Ctrl Pts',(57.8481172247805,39.4557042029884,0.));
#168660=CARTESIAN_POINT('Ctrl Pts',(57.8481172247805,39.4557042029884,12.));
#168661=CARTESIAN_POINT('Ctrl Pts',(57.8371043151607,39.45182770037,0.));
#168662=CARTESIAN_POINT('Ctrl Pts',(57.8371043151607,39.45182770037,12.));
#168663=CARTESIAN_POINT('Ctrl Pts',(57.829774010102,39.4492429618498,0.));
#168664=CARTESIAN_POINT('Ctrl Pts',(57.829774010102,39.4492429618498,12.));
#168665=CARTESIAN_POINT('Ctrl Pts',(57.8261117662439,39.4479504917286,0.));
#168666=CARTESIAN_POINT('Ctrl Pts',(57.8261117662439,39.4479504917286,12.));
#168667=CARTESIAN_POINT('',(57.8261117662439,39.4479504917286,12.));
#168668=CARTESIAN_POINT('Ctrl Pts',(57.8261117662439,39.4479504917286,12.));
#168669=CARTESIAN_POINT('Ctrl Pts',(57.829774010102,39.4492429618498,12.));
#168670=CARTESIAN_POINT('Ctrl Pts',(57.8371043151607,39.45182770037,12.));
#168671=CARTESIAN_POINT('Ctrl Pts',(57.8481172247805,39.4557042029884,12.));
#168672=CARTESIAN_POINT('Ctrl Pts',(57.8628360097134,39.4608716627367,12.));
#168673=CARTESIAN_POINT('Ctrl Pts',(57.8812926637397,39.4673289592425,12.));
#168674=CARTESIAN_POINT('Ctrl Pts',(57.8998074670541,39.4737841949417,12.));
#168675=CARTESIAN_POINT('Ctrl Pts',(57.9183803632337,39.4802373061008,12.));
#168676=CARTESIAN_POINT('Ctrl Pts',(57.9370112456506,39.4866881842223,12.));
#168677=CARTESIAN_POINT('Ctrl Pts',(57.9556999583777,39.4931366776627,12.));
#168678=CARTESIAN_POINT('Ctrl Pts',(57.9744463179305,39.4995826106691,12.));
#168679=CARTESIAN_POINT('Ctrl Pts',(57.9932501298522,39.5060257981225,12.));
#168680=CARTESIAN_POINT('Ctrl Pts',(58.012111206794,39.5124660615009,12.));
#168681=CARTESIAN_POINT('Ctrl Pts',(58.0310293875321,39.5189032457227,12.));
#168682=CARTESIAN_POINT('Ctrl Pts',(58.050004530846,39.5253372136921,12.));
#168683=CARTESIAN_POINT('Ctrl Pts',(58.0690365065393,39.5317678383231,12.));
#168684=CARTESIAN_POINT('Ctrl Pts',(58.088125187991,39.5381949959214,12.));
#168685=CARTESIAN_POINT('Ctrl Pts',(58.1072704428895,39.5446185579615,12.));
#168686=CARTESIAN_POINT('Ctrl Pts',(58.1264721285698,39.5510383869476,12.));
#168687=CARTESIAN_POINT('Ctrl Pts',(58.1457300968467,39.5574543406959,12.));
#168688=CARTESIAN_POINT('Ctrl Pts',(58.1650441970379,39.5638662750174,12.));
#168689=CARTESIAN_POINT('Ctrl Pts',(58.1844142794359,39.5702740468013,12.));
#168690=CARTESIAN_POINT('Ctrl Pts',(58.2038401992496,39.5766775175226,12.));
#168691=CARTESIAN_POINT('Ctrl Pts',(58.2233218164407,39.5830765530919,12.));
#168692=CARTESIAN_POINT('Ctrl Pts',(58.2428589938394,39.589471022173,12.));
#168693=CARTESIAN_POINT('Ctrl Pts',(58.2624515958416,39.5958607950237,12.));
#168694=CARTESIAN_POINT('Ctrl Pts',(58.2820994868092,39.6022457420772,12.));
#168695=CARTESIAN_POINT('Ctrl Pts',(58.3018025297288,39.6086257327559,12.));
#168696=CARTESIAN_POINT('Ctrl Pts',(58.3215605869192,39.6150006360894,12.));
#168697=CARTESIAN_POINT('Ctrl Pts',(58.3413735206412,39.6213703212523,12.));
#168698=CARTESIAN_POINT('Ctrl Pts',(58.3612411936914,39.6277346580898,12.));
#168699=CARTESIAN_POINT('Ctrl Pts',(58.3811634701061,39.6340935177492,12.));
#168700=CARTESIAN_POINT('Ctrl Pts',(58.4011402154225,39.6404467729113,12.));
#168701=CARTESIAN_POINT('Ctrl Pts',(58.4211712963023,39.6467942974465,12.));
#168702=CARTESIAN_POINT('Ctrl Pts',(58.4412565802984,39.6531359662043,12.));
#168703=CARTESIAN_POINT('Ctrl Pts',(58.4613959355776,39.6594716547681,12.));
#168704=CARTESIAN_POINT('Ctrl Pts',(58.4815892306044,39.66580123918,12.));
#168705=CARTESIAN_POINT('Ctrl Pts',(58.5018363341582,39.6721245959516,12.));
#168706=CARTESIAN_POINT('Ctrl Pts',(58.5221371154748,39.6784416021817,12.));
#168707=CARTESIAN_POINT('Ctrl Pts',(58.5424914443415,39.6847521356395,12.));
#168708=CARTESIAN_POINT('Ctrl Pts',(58.5628991912067,39.6910560748639,12.));
#168709=CARTESIAN_POINT('Ctrl Pts',(58.5833602272767,39.6973532992555,12.));
#168710=CARTESIAN_POINT('Ctrl Pts',(58.6038744244683,39.7036436890248,12.));
#168711=CARTESIAN_POINT('Ctrl Pts',(58.6244416553574,39.7099271251421,12.));
#168712=CARTESIAN_POINT('Ctrl Pts',(58.6450617931269,39.7162034892896,12.));
#168713=CARTESIAN_POINT('Ctrl Pts',(58.6657347115014,39.7224726638087,12.));
#168714=CARTESIAN_POINT('Ctrl Pts',(58.6864602847064,39.7287345316664,12.));
#168715=CARTESIAN_POINT('Ctrl Pts',(58.7072383875009,39.7349889764737,12.));
#168716=CARTESIAN_POINT('Ctrl Pts',(58.7280688951911,39.7412358824949,12.));
#168717=CARTESIAN_POINT('Ctrl Pts',(58.7489516836453,39.7474751346603,12.));
#168718=CARTESIAN_POINT('Ctrl Pts',(58.769886629304,39.753706618582,12.));
#168719=CARTESIAN_POINT('Ctrl Pts',(58.7908736091808,39.7599302205527,12.));
#168720=CARTESIAN_POINT('Ctrl Pts',(58.8119125008521,39.7661458275276,12.));
#168721=CARTESIAN_POINT('Ctrl Pts',(58.8330031824453,39.772353327112,12.));
#168722=CARTESIAN_POINT('Ctrl Pts',(58.8541455326229,39.7785526075477,12.));
#168723=CARTESIAN_POINT('Ctrl Pts',(58.8753394305583,39.7847435576995,12.));
#168724=CARTESIAN_POINT('Ctrl Pts',(58.896584755939,39.7909260670517,12.));
#168725=CARTESIAN_POINT('Ctrl Pts',(58.9178813889703,39.7971000257044,12.));
#168726=CARTESIAN_POINT('Ctrl Pts',(58.9392292103747,39.8032653243712,12.));
#168727=CARTESIAN_POINT('Ctrl Pts',(58.9606281013876,39.8094218543781,12.));
#168728=CARTESIAN_POINT('Ctrl Pts',(58.9820779437485,39.8155695076625,12.));
#168729=CARTESIAN_POINT('Ctrl Pts',(59.0035786197024,39.8217081767658,12.));
#168730=CARTESIAN_POINT('Ctrl Pts',(59.0251300119972,39.8278377548261,12.));
#168731=CARTESIAN_POINT('Ctrl Pts',(59.0467320038782,39.8339581355715,12.));
#168732=CARTESIAN_POINT('Ctrl Pts',(59.068384479077,39.8400692133143,12.));
#168733=CARTESIAN_POINT('Ctrl Pts',(59.0900873217992,39.8461708829465,12.));
#168734=CARTESIAN_POINT('Ctrl Pts',(59.1118404167304,39.8522630399337,12.));
#168735=CARTESIAN_POINT('Ctrl Pts',(59.133643649035,39.8583455803111,12.));
#168736=CARTESIAN_POINT('Ctrl Pts',(59.155496904352,39.8644184006785,12.));
#168737=CARTESIAN_POINT('Ctrl Pts',(59.1774000687865,39.8704813981978,12.));
#168738=CARTESIAN_POINT('Ctrl Pts',(59.1993530289008,39.8765344705895,12.));
#168739=CARTESIAN_POINT('Ctrl Pts',(59.2213556717189,39.8825775161252,12.));
#168740=CARTESIAN_POINT('Ctrl Pts',(59.2434078847236,39.8886104336234,12.));
#168741=CARTESIAN_POINT('Ctrl Pts',(59.2655095558527,39.8946331224442,12.));
#168742=CARTESIAN_POINT('Ctrl Pts',(59.2876605734871,39.9006454824861,12.));
#168743=CARTESIAN_POINT('Ctrl Pts',(59.3098608264452,39.9066474141826,12.));
#168744=CARTESIAN_POINT('Ctrl Pts',(59.3321102039883,39.9126388184956,12.));
#168745=CARTESIAN_POINT('Ctrl Pts',(59.3544085958165,39.9186195969113,12.));
#168746=CARTESIAN_POINT('Ctrl Pts',(59.3767558920663,39.9245896514359,12.));
#168747=CARTESIAN_POINT('Ctrl Pts',(59.3991519832981,39.9305488845934,12.));
#168748=CARTESIAN_POINT('Ctrl Pts',(59.4215967604925,39.9364971994215,12.));
#168749=CARTESIAN_POINT('Ctrl Pts',(59.444090115055,39.9424344994652,12.));
#168750=CARTESIAN_POINT('Ctrl Pts',(59.4666319388123,39.9483606887731,12.));
#168751=CARTESIAN_POINT('Ctrl Pts',(59.4892221240081,39.954275671893,12.));
#168752=CARTESIAN_POINT('Ctrl Pts',(59.511860563292,39.96017935387,12.));
#168753=CARTESIAN_POINT('Ctrl Pts',(59.5345471497162,39.9660716402423,12.));
#168754=CARTESIAN_POINT('Ctrl Pts',(59.5572817767412,39.971952437036,12.));
#168755=CARTESIAN_POINT('Ctrl Pts',(59.5800643382322,39.9778216507609,12.));
#168756=CARTESIAN_POINT('Ctrl Pts',(59.6028947284551,39.9836791884071,12.));
#168757=CARTESIAN_POINT('Ctrl Pts',(59.6257728420644,39.9895249574432,12.));
#168758=CARTESIAN_POINT('Ctrl Pts',(59.6486985741015,39.9953588658114,12.));
#168759=CARTESIAN_POINT('Ctrl Pts',(59.671671819999,40.0011808219231,12.));
#168760=CARTESIAN_POINT('Ctrl Pts',(59.6946924755771,40.0069907346536,12.));
#168761=CARTESIAN_POINT('Ctrl Pts',(59.7177604370409,40.0127885133407,12.));
#168762=CARTESIAN_POINT('Ctrl Pts',(59.7408756009688,40.0185740677827,12.));
#168763=CARTESIAN_POINT('Ctrl Pts',(59.7640378643115,40.0243473082343,12.));
#168764=CARTESIAN_POINT('Ctrl Pts',(59.7872471243948,40.0301081454006,12.));
#168765=CARTESIAN_POINT('Ctrl Pts',(59.8105032789179,40.035856490434,12.));
#168766=CARTESIAN_POINT('Ctrl Pts',(59.8338062259491,40.0415922549313,12.));
#168767=CARTESIAN_POINT('Ctrl Pts',(59.8571558639145,40.0473153509323,12.));
#168768=CARTESIAN_POINT('Ctrl Pts',(59.8805520915975,40.0530256909162,12.));
#168769=CARTESIAN_POINT('Ctrl Pts',(59.9039948081432,40.0587231877961,12.));
#168770=CARTESIAN_POINT('Ctrl Pts',(59.9274839130553,40.0644077549159,12.));
#168771=CARTESIAN_POINT('Ctrl Pts',(59.9510193061927,40.0700793060473,12.));
#168772=CARTESIAN_POINT('Ctrl Pts',(59.9746008877584,40.0757377553888,12.));
#168773=CARTESIAN_POINT('Ctrl Pts',(59.9982285582983,40.0813830175623,12.));
#168774=CARTESIAN_POINT('Ctrl Pts',(60.021902218706,40.0870150076074,12.));
#168775=CARTESIAN_POINT('Ctrl Pts',(60.0456217702202,40.0926336409785,12.));
#168776=CARTESIAN_POINT('Ctrl Pts',(60.069387114421,40.0982388335423,12.));
#168777=CARTESIAN_POINT('Ctrl Pts',(60.0931981532198,40.1038305015766,12.));
#168778=CARTESIAN_POINT('Ctrl Pts',(60.1170547888574,40.1094085617674,12.));
#168779=CARTESIAN_POINT('Ctrl Pts',(60.1409569239092,40.1149729312036,12.));
#168780=CARTESIAN_POINT('Ctrl Pts',(60.1649044612828,40.1205235273739,12.));
#168781=CARTESIAN_POINT('Ctrl Pts',(60.1888973042152,40.1260602681644,12.));
#168782=CARTESIAN_POINT('Ctrl Pts',(60.2129353562622,40.1315830718577,12.));
#168783=CARTESIAN_POINT('Ctrl Pts',(60.2370185212964,40.1370918571304,12.));
#168784=CARTESIAN_POINT('Ctrl Pts',(60.2611467035116,40.1425865430472,12.));
#168785=CARTESIAN_POINT('Ctrl Pts',(60.285319807422,40.1480670490586,12.));
#168786=CARTESIAN_POINT('Ctrl Pts',(60.3095377378586,40.1535332949976,12.));
#168787=CARTESIAN_POINT('Ctrl Pts',(60.3338003999607,40.1589852010804,12.));
#168788=CARTESIAN_POINT('Ctrl Pts',(60.3581076991716,40.1644226879033,12.));
#168789=CARTESIAN_POINT('Ctrl Pts',(60.3824595412445,40.1698456764377,12.));
#168790=CARTESIAN_POINT('Ctrl Pts',(60.4068558322407,40.1752540880268,12.));
#168791=CARTESIAN_POINT('Ctrl Pts',(60.4312964785273,40.180647844383,12.));
#168792=CARTESIAN_POINT('Ctrl Pts',(60.455781386769,40.1860268675884,12.));
#168793=CARTESIAN_POINT('Ctrl Pts',(60.4803104639225,40.1913910800921,12.));
#168794=CARTESIAN_POINT('Ctrl Pts',(60.5048836172435,40.1967404047062,12.));
#168795=CARTESIAN_POINT('Ctrl Pts',(60.5295007542841,40.2020747646014,12.));
#168796=CARTESIAN_POINT('Ctrl Pts',(60.5541617828925,40.2073940833053,12.));
#168797=CARTESIAN_POINT('Ctrl Pts',(60.5788666112042,40.2126982847011,12.));
#168798=CARTESIAN_POINT('Ctrl Pts',(60.6036151476349,40.2179872930273,12.));
#168799=CARTESIAN_POINT('Ctrl Pts',(60.6284073008871,40.2232610328721,12.));
#168800=CARTESIAN_POINT('Ctrl Pts',(60.6532429799499,40.2285194291706,12.));
#168801=CARTESIAN_POINT('Ctrl Pts',(60.678122094098,40.2337624072029,12.));
#168802=CARTESIAN_POINT('Ctrl Pts',(60.7030445528857,40.2389898925932,12.));
#168803=CARTESIAN_POINT('Ctrl Pts',(60.728010266139,40.2442018113108,12.));
#168804=CARTESIAN_POINT('Ctrl Pts',(60.7530191439593,40.2493980896638,12.));
#168805=CARTESIAN_POINT('Ctrl Pts',(60.7780710967248,40.2545786542953,12.));
#168806=CARTESIAN_POINT('Ctrl Pts',(60.8031660350879,40.2597434321803,12.));
#168807=CARTESIAN_POINT('Ctrl Pts',(60.8283038699706,40.2648923506248,12.));
#168808=CARTESIAN_POINT('Ctrl Pts',(60.8534845125538,40.2700253372648,12.));
#168809=CARTESIAN_POINT('Ctrl Pts',(60.8787078742818,40.2751423200639,12.));
#168810=CARTESIAN_POINT('Ctrl Pts',(60.9039738668669,40.2802432273104,12.));
#168811=CARTESIAN_POINT('Ctrl Pts',(60.9292824022887,40.2853279876161,12.));
#168812=CARTESIAN_POINT('Ctrl Pts',(60.9546333927921,40.2903965299155,12.));
#168813=CARTESIAN_POINT('Ctrl Pts',(60.9800267508786,40.295448783469,12.));
#168814=CARTESIAN_POINT('Ctrl Pts',(61.0054623893066,40.300484677858,12.));
#168815=CARTESIAN_POINT('Ctrl Pts',(61.0309402210921,40.3055041429775,12.));
#168816=CARTESIAN_POINT('Ctrl Pts',(61.056460159505,40.310507109031,12.));
#168817=CARTESIAN_POINT('Ctrl Pts',(61.0820221180645,40.3154935065262,12.));
#168818=CARTESIAN_POINT('Ctrl Pts',(61.1076260105258,40.3204632662725,12.));
#168819=CARTESIAN_POINT('Ctrl Pts',(61.1332717508789,40.32541631938,12.));
#168820=CARTESIAN_POINT('Ctrl Pts',(61.1589592533613,40.3303525972615,12.));
#168821=CARTESIAN_POINT('Ctrl Pts',(61.1846884324644,40.335272031637,12.));
#168822=CARTESIAN_POINT('Ctrl Pts',(61.2104592029377,40.340174554537,12.));
#168823=CARTESIAN_POINT('Ctrl Pts',(61.23627147979,40.3450600983109,12.));
#168824=CARTESIAN_POINT('Ctrl Pts',(61.2621251782863,40.3499285956304,12.));
#168825=CARTESIAN_POINT('Ctrl Pts',(61.2880202139371,40.3547799794679,12.));
#168826=CARTESIAN_POINT('Ctrl Pts',(61.3139565024847,40.3596141830791,12.));
#168827=CARTESIAN_POINT('Ctrl Pts',(61.3399339598853,40.3644311399861,12.));
#168828=CARTESIAN_POINT('Ctrl Pts',(61.3659525022908,40.3692307839636,12.));
#168829=CARTESIAN_POINT('Ctrl Pts',(61.3920120460219,40.3740130490225,12.));
#168830=CARTESIAN_POINT('Ctrl Pts',(61.4181125076037,40.3787778694364,12.));
#168831=CARTESIAN_POINT('Ctrl Pts',(61.4442538038044,40.383525179772,12.));
#168832=CARTESIAN_POINT('Ctrl Pts',(61.4704358516709,40.3882549149228,12.));
#168833=CARTESIAN_POINT('Ctrl Pts',(61.4966585685549,40.3929670101366,12.));
#168834=CARTESIAN_POINT('Ctrl Pts',(61.522921872154,40.3976614010652,12.));
#168835=CARTESIAN_POINT('Ctrl Pts',(61.5492256804717,40.4023380237232,12.));
#168836=CARTESIAN_POINT('Ctrl Pts',(61.5755699117324,40.4069968143956,12.));
#168837=CARTESIAN_POINT('Ctrl Pts',(61.601954484301,40.4116377095596,12.));
#168838=CARTESIAN_POINT('Ctrl Pts',(61.628379316608,40.4162606458119,12.));
#168839=CARTESIAN_POINT('Ctrl Pts',(61.6548443270394,40.4208655597717,12.));
#168840=CARTESIAN_POINT('Ctrl Pts',(61.6813494339286,40.425452388076,12.));
#168841=CARTESIAN_POINT('Ctrl Pts',(61.7078945557799,40.430021067584,12.));
#168842=CARTESIAN_POINT('Ctrl Pts',(61.7344796114399,40.4345715355405,12.));
#168843=CARTESIAN_POINT('Ctrl Pts',(61.7611045202874,40.4391037297589,12.));
#168844=CARTESIAN_POINT('Ctrl Pts',(61.7877692024076,40.4436175887949,12.));
#168845=CARTESIAN_POINT('Ctrl Pts',(61.814473578779,40.4481130521364,12.));
#168846=CARTESIAN_POINT('Ctrl Pts',(61.8412175708552,40.4525900597894,12.));
#168847=CARTESIAN_POINT('Ctrl Pts',(61.8680011001537,40.4570485518749,12.));
#168848=CARTESIAN_POINT('Ctrl Pts',(61.8948240878008,40.4614884681889,12.));
#168849=CARTESIAN_POINT('Ctrl Pts',(61.9216864541744,40.4659097478587,12.));
#168850=CARTESIAN_POINT('Ctrl Pts',(61.9485881182921,40.4703123287621,12.));
#168851=CARTESIAN_POINT('Ctrl Pts',(61.9755289983044,40.4746961480015,12.));
#168852=CARTESIAN_POINT('Ctrl Pts',(62.0025090125959,40.4790611429583,12.));
#168853=CARTESIAN_POINT('Ctrl Pts',(62.029528080742,40.4834072522164,12.));
#168854=CARTESIAN_POINT('Ctrl Pts',(62.0565861244179,40.4877344164411,12.));
#168855=CARTESIAN_POINT('Ctrl Pts',(62.0836830685719,40.4920425795217,12.));
#168856=CARTESIAN_POINT('Ctrl Pts',(62.1108188417003,40.4963316888412,12.));
#168857=CARTESIAN_POINT('Ctrl Pts',(62.1341126810541,40.4999919096264,12.));
#168858=CARTESIAN_POINT('Ctrl Pts',(62.1519925002974,40.5027877865802,12.));
#168859=CARTESIAN_POINT('Ctrl Pts',(62.1644411502821,40.5047277935767,12.));
#168860=CARTESIAN_POINT('Ctrl Pts',(62.1714473138102,40.5058175523127,12.));
#168861=CARTESIAN_POINT('Ctrl Pts',(62.1730054756871,40.5060598100929,12.));
#168862=CARTESIAN_POINT('',(57.8261117662439,39.4479504917286,0.));
#168863=CARTESIAN_POINT('',(57.8261117662439,39.4479504917286,0.));
#168864=CARTESIAN_POINT('Ctrl Pts',(62.1730054756871,40.5060598100929,0.));
#168865=CARTESIAN_POINT('Ctrl Pts',(62.1714473138102,40.5058175523127,0.));
#168866=CARTESIAN_POINT('Ctrl Pts',(62.1644411502821,40.5047277935767,0.));
#168867=CARTESIAN_POINT('Ctrl Pts',(62.1519925002974,40.5027877865802,0.));
#168868=CARTESIAN_POINT('Ctrl Pts',(62.1341126810541,40.4999919096264,0.));
#168869=CARTESIAN_POINT('Ctrl Pts',(62.1108188417003,40.4963316888412,0.));
#168870=CARTESIAN_POINT('Ctrl Pts',(62.0836830685719,40.4920425795217,0.));
#168871=CARTESIAN_POINT('Ctrl Pts',(62.0565861244179,40.4877344164411,0.));
#168872=CARTESIAN_POINT('Ctrl Pts',(62.029528080742,40.4834072522164,0.));
#168873=CARTESIAN_POINT('Ctrl Pts',(62.0025090125959,40.4790611429583,0.));
#168874=CARTESIAN_POINT('Ctrl Pts',(61.9755289983044,40.4746961480015,0.));
#168875=CARTESIAN_POINT('Ctrl Pts',(61.9485881182921,40.4703123287621,0.));
#168876=CARTESIAN_POINT('Ctrl Pts',(61.9216864541744,40.4659097478587,0.));
#168877=CARTESIAN_POINT('Ctrl Pts',(61.8948240878008,40.4614884681889,0.));
#168878=CARTESIAN_POINT('Ctrl Pts',(61.8680011001537,40.4570485518749,0.));
#168879=CARTESIAN_POINT('Ctrl Pts',(61.8412175708552,40.4525900597894,0.));
#168880=CARTESIAN_POINT('Ctrl Pts',(61.814473578779,40.4481130521364,0.));
#168881=CARTESIAN_POINT('Ctrl Pts',(61.7877692024076,40.4436175887949,0.));
#168882=CARTESIAN_POINT('Ctrl Pts',(61.7611045202874,40.4391037297589,0.));
#168883=CARTESIAN_POINT('Ctrl Pts',(61.7344796114399,40.4345715355405,0.));
#168884=CARTESIAN_POINT('Ctrl Pts',(61.7078945557799,40.430021067584,0.));
#168885=CARTESIAN_POINT('Ctrl Pts',(61.6813494339286,40.425452388076,0.));
#168886=CARTESIAN_POINT('Ctrl Pts',(61.6548443270394,40.4208655597717,0.));
#168887=CARTESIAN_POINT('Ctrl Pts',(61.628379316608,40.4162606458119,0.));
#168888=CARTESIAN_POINT('Ctrl Pts',(61.601954484301,40.4116377095596,0.));
#168889=CARTESIAN_POINT('Ctrl Pts',(61.5755699117324,40.4069968143956,0.));
#168890=CARTESIAN_POINT('Ctrl Pts',(61.5492256804717,40.4023380237232,0.));
#168891=CARTESIAN_POINT('Ctrl Pts',(61.522921872154,40.3976614010652,0.));
#168892=CARTESIAN_POINT('Ctrl Pts',(61.4966585685549,40.3929670101366,0.));
#168893=CARTESIAN_POINT('Ctrl Pts',(61.4704358516709,40.3882549149228,0.));
#168894=CARTESIAN_POINT('Ctrl Pts',(61.4442538038044,40.383525179772,0.));
#168895=CARTESIAN_POINT('Ctrl Pts',(61.4181125076037,40.3787778694364,0.));
#168896=CARTESIAN_POINT('Ctrl Pts',(61.3920120460219,40.3740130490225,0.));
#168897=CARTESIAN_POINT('Ctrl Pts',(61.3659525022908,40.3692307839636,0.));
#168898=CARTESIAN_POINT('Ctrl Pts',(61.3399339598853,40.3644311399861,0.));
#168899=CARTESIAN_POINT('Ctrl Pts',(61.3139565024847,40.3596141830791,0.));
#168900=CARTESIAN_POINT('Ctrl Pts',(61.2880202139371,40.3547799794679,0.));
#168901=CARTESIAN_POINT('Ctrl Pts',(61.2621251782863,40.3499285956304,0.));
#168902=CARTESIAN_POINT('Ctrl Pts',(61.23627147979,40.3450600983109,0.));
#168903=CARTESIAN_POINT('Ctrl Pts',(61.2104592029377,40.340174554537,0.));
#168904=CARTESIAN_POINT('Ctrl Pts',(61.1846884324644,40.335272031637,0.));
#168905=CARTESIAN_POINT('Ctrl Pts',(61.1589592533613,40.3303525972615,0.));
#168906=CARTESIAN_POINT('Ctrl Pts',(61.1332717508789,40.32541631938,0.));
#168907=CARTESIAN_POINT('Ctrl Pts',(61.1076260105258,40.3204632662725,0.));
#168908=CARTESIAN_POINT('Ctrl Pts',(61.0820221180645,40.3154935065262,0.));
#168909=CARTESIAN_POINT('Ctrl Pts',(61.056460159505,40.310507109031,0.));
#168910=CARTESIAN_POINT('Ctrl Pts',(61.0309402210921,40.3055041429775,0.));
#168911=CARTESIAN_POINT('Ctrl Pts',(61.0054623893066,40.300484677858,0.));
#168912=CARTESIAN_POINT('Ctrl Pts',(60.9800267508786,40.295448783469,0.));
#168913=CARTESIAN_POINT('Ctrl Pts',(60.9546333927921,40.2903965299155,0.));
#168914=CARTESIAN_POINT('Ctrl Pts',(60.9292824022887,40.2853279876161,0.));
#168915=CARTESIAN_POINT('Ctrl Pts',(60.9039738668669,40.2802432273104,0.));
#168916=CARTESIAN_POINT('Ctrl Pts',(60.8787078742818,40.2751423200639,0.));
#168917=CARTESIAN_POINT('Ctrl Pts',(60.8534845125538,40.2700253372648,0.));
#168918=CARTESIAN_POINT('Ctrl Pts',(60.8283038699706,40.2648923506248,0.));
#168919=CARTESIAN_POINT('Ctrl Pts',(60.8031660350879,40.2597434321803,0.));
#168920=CARTESIAN_POINT('Ctrl Pts',(60.7780710967248,40.2545786542953,0.));
#168921=CARTESIAN_POINT('Ctrl Pts',(60.7530191439593,40.2493980896638,0.));
#168922=CARTESIAN_POINT('Ctrl Pts',(60.728010266139,40.2442018113108,0.));
#168923=CARTESIAN_POINT('Ctrl Pts',(60.7030445528857,40.2389898925932,0.));
#168924=CARTESIAN_POINT('Ctrl Pts',(60.678122094098,40.2337624072029,0.));
#168925=CARTESIAN_POINT('Ctrl Pts',(60.6532429799499,40.2285194291706,0.));
#168926=CARTESIAN_POINT('Ctrl Pts',(60.6284073008871,40.2232610328721,0.));
#168927=CARTESIAN_POINT('Ctrl Pts',(60.6036151476349,40.2179872930273,0.));
#168928=CARTESIAN_POINT('Ctrl Pts',(60.5788666112042,40.2126982847011,0.));
#168929=CARTESIAN_POINT('Ctrl Pts',(60.5541617828925,40.2073940833053,0.));
#168930=CARTESIAN_POINT('Ctrl Pts',(60.5295007542841,40.2020747646014,0.));
#168931=CARTESIAN_POINT('Ctrl Pts',(60.5048836172435,40.1967404047062,0.));
#168932=CARTESIAN_POINT('Ctrl Pts',(60.4803104639225,40.1913910800921,0.));
#168933=CARTESIAN_POINT('Ctrl Pts',(60.455781386769,40.1860268675884,0.));
#168934=CARTESIAN_POINT('Ctrl Pts',(60.4312964785273,40.180647844383,0.));
#168935=CARTESIAN_POINT('Ctrl Pts',(60.4068558322407,40.1752540880268,0.));
#168936=CARTESIAN_POINT('Ctrl Pts',(60.3824595412445,40.1698456764377,0.));
#168937=CARTESIAN_POINT('Ctrl Pts',(60.3581076991716,40.1644226879033,0.));
#168938=CARTESIAN_POINT('Ctrl Pts',(60.3338003999607,40.1589852010804,0.));
#168939=CARTESIAN_POINT('Ctrl Pts',(60.3095377378586,40.1535332949976,0.));
#168940=CARTESIAN_POINT('Ctrl Pts',(60.285319807422,40.1480670490586,0.));
#168941=CARTESIAN_POINT('Ctrl Pts',(60.2611467035116,40.1425865430472,0.));
#168942=CARTESIAN_POINT('Ctrl Pts',(60.2370185212964,40.1370918571304,0.));
#168943=CARTESIAN_POINT('Ctrl Pts',(60.2129353562622,40.1315830718577,0.));
#168944=CARTESIAN_POINT('Ctrl Pts',(60.1888973042152,40.1260602681644,0.));
#168945=CARTESIAN_POINT('Ctrl Pts',(60.1649044612828,40.1205235273739,0.));
#168946=CARTESIAN_POINT('Ctrl Pts',(60.1409569239092,40.1149729312036,0.));
#168947=CARTESIAN_POINT('Ctrl Pts',(60.1170547888574,40.1094085617674,0.));
#168948=CARTESIAN_POINT('Ctrl Pts',(60.0931981532198,40.1038305015766,0.));
#168949=CARTESIAN_POINT('Ctrl Pts',(60.069387114421,40.0982388335423,0.));
#168950=CARTESIAN_POINT('Ctrl Pts',(60.0456217702202,40.0926336409785,0.));
#168951=CARTESIAN_POINT('Ctrl Pts',(60.021902218706,40.0870150076074,0.));
#168952=CARTESIAN_POINT('Ctrl Pts',(59.9982285582983,40.0813830175623,0.));
#168953=CARTESIAN_POINT('Ctrl Pts',(59.9746008877584,40.0757377553888,0.));
#168954=CARTESIAN_POINT('Ctrl Pts',(59.9510193061927,40.0700793060473,0.));
#168955=CARTESIAN_POINT('Ctrl Pts',(59.9274839130553,40.0644077549159,0.));
#168956=CARTESIAN_POINT('Ctrl Pts',(59.9039948081432,40.0587231877961,0.));
#168957=CARTESIAN_POINT('Ctrl Pts',(59.8805520915975,40.0530256909162,0.));
#168958=CARTESIAN_POINT('Ctrl Pts',(59.8571558639145,40.0473153509323,0.));
#168959=CARTESIAN_POINT('Ctrl Pts',(59.8338062259491,40.0415922549313,0.));
#168960=CARTESIAN_POINT('Ctrl Pts',(59.8105032789179,40.035856490434,0.));
#168961=CARTESIAN_POINT('Ctrl Pts',(59.7872471243948,40.0301081454006,0.));
#168962=CARTESIAN_POINT('Ctrl Pts',(59.7640378643115,40.0243473082343,0.));
#168963=CARTESIAN_POINT('Ctrl Pts',(59.7408756009688,40.0185740677827,0.));
#168964=CARTESIAN_POINT('Ctrl Pts',(59.7177604370409,40.0127885133407,0.));
#168965=CARTESIAN_POINT('Ctrl Pts',(59.6946924755771,40.0069907346536,0.));
#168966=CARTESIAN_POINT('Ctrl Pts',(59.671671819999,40.0011808219231,0.));
#168967=CARTESIAN_POINT('Ctrl Pts',(59.6486985741015,39.9953588658114,0.));
#168968=CARTESIAN_POINT('Ctrl Pts',(59.6257728420644,39.9895249574432,0.));
#168969=CARTESIAN_POINT('Ctrl Pts',(59.6028947284551,39.9836791884071,0.));
#168970=CARTESIAN_POINT('Ctrl Pts',(59.5800643382322,39.9778216507609,0.));
#168971=CARTESIAN_POINT('Ctrl Pts',(59.5572817767412,39.971952437036,0.));
#168972=CARTESIAN_POINT('Ctrl Pts',(59.5345471497162,39.9660716402423,0.));
#168973=CARTESIAN_POINT('Ctrl Pts',(59.511860563292,39.96017935387,0.));
#168974=CARTESIAN_POINT('Ctrl Pts',(59.4892221240081,39.954275671893,0.));
#168975=CARTESIAN_POINT('Ctrl Pts',(59.4666319388123,39.9483606887731,0.));
#168976=CARTESIAN_POINT('Ctrl Pts',(59.444090115055,39.9424344994652,0.));
#168977=CARTESIAN_POINT('Ctrl Pts',(59.4215967604925,39.9364971994215,0.));
#168978=CARTESIAN_POINT('Ctrl Pts',(59.3991519832981,39.9305488845934,0.));
#168979=CARTESIAN_POINT('Ctrl Pts',(59.3767558920663,39.9245896514359,0.));
#168980=CARTESIAN_POINT('Ctrl Pts',(59.3544085958165,39.9186195969113,0.));
#168981=CARTESIAN_POINT('Ctrl Pts',(59.3321102039883,39.9126388184956,0.));
#168982=CARTESIAN_POINT('Ctrl Pts',(59.3098608264452,39.9066474141826,0.));
#168983=CARTESIAN_POINT('Ctrl Pts',(59.2876605734871,39.9006454824861,0.));
#168984=CARTESIAN_POINT('Ctrl Pts',(59.2655095558527,39.8946331224442,0.));
#168985=CARTESIAN_POINT('Ctrl Pts',(59.2434078847236,39.8886104336234,0.));
#168986=CARTESIAN_POINT('Ctrl Pts',(59.2213556717189,39.8825775161252,0.));
#168987=CARTESIAN_POINT('Ctrl Pts',(59.1993530289008,39.8765344705895,0.));
#168988=CARTESIAN_POINT('Ctrl Pts',(59.1774000687865,39.8704813981978,0.));
#168989=CARTESIAN_POINT('Ctrl Pts',(59.155496904352,39.8644184006785,0.));
#168990=CARTESIAN_POINT('Ctrl Pts',(59.133643649035,39.8583455803111,0.));
#168991=CARTESIAN_POINT('Ctrl Pts',(59.1118404167304,39.8522630399337,0.));
#168992=CARTESIAN_POINT('Ctrl Pts',(59.0900873217992,39.8461708829465,0.));
#168993=CARTESIAN_POINT('Ctrl Pts',(59.068384479077,39.8400692133143,0.));
#168994=CARTESIAN_POINT('Ctrl Pts',(59.0467320038782,39.8339581355715,0.));
#168995=CARTESIAN_POINT('Ctrl Pts',(59.0251300119972,39.8278377548261,0.));
#168996=CARTESIAN_POINT('Ctrl Pts',(59.0035786197024,39.8217081767658,0.));
#168997=CARTESIAN_POINT('Ctrl Pts',(58.9820779437485,39.8155695076625,0.));
#168998=CARTESIAN_POINT('Ctrl Pts',(58.9606281013876,39.8094218543781,0.));
#168999=CARTESIAN_POINT('Ctrl Pts',(58.9392292103747,39.8032653243712,0.));
#169000=CARTESIAN_POINT('Ctrl Pts',(58.9178813889703,39.7971000257044,0.));
#169001=CARTESIAN_POINT('Ctrl Pts',(58.896584755939,39.7909260670517,0.));
#169002=CARTESIAN_POINT('Ctrl Pts',(58.8753394305583,39.7847435576995,0.));
#169003=CARTESIAN_POINT('Ctrl Pts',(58.8541455326229,39.7785526075477,0.));
#169004=CARTESIAN_POINT('Ctrl Pts',(58.8330031824453,39.772353327112,0.));
#169005=CARTESIAN_POINT('Ctrl Pts',(58.8119125008521,39.7661458275276,0.));
#169006=CARTESIAN_POINT('Ctrl Pts',(58.7908736091808,39.7599302205527,0.));
#169007=CARTESIAN_POINT('Ctrl Pts',(58.769886629304,39.753706618582,0.));
#169008=CARTESIAN_POINT('Ctrl Pts',(58.7489516836453,39.7474751346603,0.));
#169009=CARTESIAN_POINT('Ctrl Pts',(58.7280688951911,39.7412358824949,0.));
#169010=CARTESIAN_POINT('Ctrl Pts',(58.7072383875009,39.7349889764737,0.));
#169011=CARTESIAN_POINT('Ctrl Pts',(58.6864602847064,39.7287345316664,0.));
#169012=CARTESIAN_POINT('Ctrl Pts',(58.6657347115014,39.7224726638087,0.));
#169013=CARTESIAN_POINT('Ctrl Pts',(58.6450617931269,39.7162034892896,0.));
#169014=CARTESIAN_POINT('Ctrl Pts',(58.6244416553574,39.7099271251421,0.));
#169015=CARTESIAN_POINT('Ctrl Pts',(58.6038744244683,39.7036436890248,0.));
#169016=CARTESIAN_POINT('Ctrl Pts',(58.5833602272767,39.6973532992555,0.));
#169017=CARTESIAN_POINT('Ctrl Pts',(58.5628991912067,39.6910560748639,0.));
#169018=CARTESIAN_POINT('Ctrl Pts',(58.5424914443415,39.6847521356395,0.));
#169019=CARTESIAN_POINT('Ctrl Pts',(58.5221371154748,39.6784416021817,0.));
#169020=CARTESIAN_POINT('Ctrl Pts',(58.5018363341582,39.6721245959516,0.));
#169021=CARTESIAN_POINT('Ctrl Pts',(58.4815892306044,39.66580123918,0.));
#169022=CARTESIAN_POINT('Ctrl Pts',(58.4613959355776,39.6594716547681,0.));
#169023=CARTESIAN_POINT('Ctrl Pts',(58.4412565802984,39.6531359662043,0.));
#169024=CARTESIAN_POINT('Ctrl Pts',(58.4211712963023,39.6467942974465,0.));
#169025=CARTESIAN_POINT('Ctrl Pts',(58.4011402154225,39.6404467729113,0.));
#169026=CARTESIAN_POINT('Ctrl Pts',(58.3811634701061,39.6340935177492,0.));
#169027=CARTESIAN_POINT('Ctrl Pts',(58.3612411936914,39.6277346580898,0.));
#169028=CARTESIAN_POINT('Ctrl Pts',(58.3413735206412,39.6213703212523,0.));
#169029=CARTESIAN_POINT('Ctrl Pts',(58.3215605869192,39.6150006360894,0.));
#169030=CARTESIAN_POINT('Ctrl Pts',(58.3018025297288,39.6086257327559,0.));
#169031=CARTESIAN_POINT('Ctrl Pts',(58.2820994868092,39.6022457420772,0.));
#169032=CARTESIAN_POINT('Ctrl Pts',(58.2624515958416,39.5958607950237,0.));
#169033=CARTESIAN_POINT('Ctrl Pts',(58.2428589938394,39.589471022173,0.));
#169034=CARTESIAN_POINT('Ctrl Pts',(58.2233218164407,39.5830765530919,0.));
#169035=CARTESIAN_POINT('Ctrl Pts',(58.2038401992496,39.5766775175226,0.));
#169036=CARTESIAN_POINT('Ctrl Pts',(58.1844142794359,39.5702740468013,0.));
#169037=CARTESIAN_POINT('Ctrl Pts',(58.1650441970379,39.5638662750174,0.));
#169038=CARTESIAN_POINT('Ctrl Pts',(58.1457300968467,39.5574543406959,0.));
#169039=CARTESIAN_POINT('Ctrl Pts',(58.1264721285698,39.5510383869476,0.));
#169040=CARTESIAN_POINT('Ctrl Pts',(58.1072704428895,39.5446185579615,0.));
#169041=CARTESIAN_POINT('Ctrl Pts',(58.088125187991,39.5381949959214,0.));
#169042=CARTESIAN_POINT('Ctrl Pts',(58.0690365065393,39.5317678383231,0.));
#169043=CARTESIAN_POINT('Ctrl Pts',(58.050004530846,39.5253372136921,0.));
#169044=CARTESIAN_POINT('Ctrl Pts',(58.0310293875321,39.5189032457227,0.));
#169045=CARTESIAN_POINT('Ctrl Pts',(58.012111206794,39.5124660615009,0.));
#169046=CARTESIAN_POINT('Ctrl Pts',(57.9932501298522,39.5060257981225,0.));
#169047=CARTESIAN_POINT('Ctrl Pts',(57.9744463179305,39.4995826106691,0.));
#169048=CARTESIAN_POINT('Ctrl Pts',(57.9556999583777,39.4931366776627,0.));
#169049=CARTESIAN_POINT('Ctrl Pts',(57.9370112456506,39.4866881842223,0.));
#169050=CARTESIAN_POINT('Ctrl Pts',(57.9183803632337,39.4802373061008,0.));
#169051=CARTESIAN_POINT('Ctrl Pts',(57.8998074670541,39.4737841949417,0.));
#169052=CARTESIAN_POINT('Ctrl Pts',(57.8812926637397,39.4673289592425,0.));
#169053=CARTESIAN_POINT('Ctrl Pts',(57.8628360097134,39.4608716627367,0.));
#169054=CARTESIAN_POINT('Ctrl Pts',(57.8481172247805,39.4557042029884,0.));
#169055=CARTESIAN_POINT('Ctrl Pts',(57.8371043151607,39.45182770037,0.));
#169056=CARTESIAN_POINT('Ctrl Pts',(57.829774010102,39.4492429618498,0.));
#169057=CARTESIAN_POINT('Ctrl Pts',(57.8261117662439,39.4479504917286,0.));
#169058=CARTESIAN_POINT('Ctrl Pts',(65.7914953018525,34.9532422808861,0.));
#169059=CARTESIAN_POINT('Ctrl Pts',(65.7914953018525,34.9532422808861,12.));
#169060=CARTESIAN_POINT('Ctrl Pts',(65.7859084407617,34.9529266758466,0.));
#169061=CARTESIAN_POINT('Ctrl Pts',(65.7859084407617,34.9529266758466,12.));
#169062=CARTESIAN_POINT('Ctrl Pts',(65.7747383251112,34.9522931728759,0.));
#169063=CARTESIAN_POINT('Ctrl Pts',(65.7747383251112,34.9522931728759,12.));
#169064=CARTESIAN_POINT('Ctrl Pts',(65.7579939712289,34.9513360397454,0.));
#169065=CARTESIAN_POINT('Ctrl Pts',(65.7579939712289,34.9513360397454,12.));
#169066=CARTESIAN_POINT('Ctrl Pts',(65.7356898061147,34.9500461043246,0.));
#169067=CARTESIAN_POINT('Ctrl Pts',(65.7356898061147,34.9500461043246,12.));
#169068=CARTESIAN_POINT('Ctrl Pts',(65.7078456758034,34.9484107544137,0.));
#169069=CARTESIAN_POINT('Ctrl Pts',(65.7078456758034,34.9484107544137,12.));
#169070=CARTESIAN_POINT('Ctrl Pts',(65.6800376406066,34.9467524770439,0.));
#169071=CARTESIAN_POINT('Ctrl Pts',(65.6800376406066,34.9467524770439,12.));
#169072=CARTESIAN_POINT('Ctrl Pts',(65.6522657321322,34.9450712829183,0.));
#169073=CARTESIAN_POINT('Ctrl Pts',(65.6522657321322,34.9450712829183,12.));
#169074=CARTESIAN_POINT('Ctrl Pts',(65.624529996851,34.943367193292,0.));
#169075=CARTESIAN_POINT('Ctrl Pts',(65.624529996851,34.943367193292,12.));
#169076=CARTESIAN_POINT('Ctrl Pts',(65.5968304997584,34.9416402443435,0.));
#169077=CARTESIAN_POINT('Ctrl Pts',(65.5968304997584,34.9416402443435,12.));
#169078=CARTESIAN_POINT('Ctrl Pts',(65.5691673225803,34.9398904862157,0.));
#169079=CARTESIAN_POINT('Ctrl Pts',(65.5691673225803,34.9398904862157,12.));
#169080=CARTESIAN_POINT('Ctrl Pts',(65.5415405577955,34.9381179779673,0.));
#169081=CARTESIAN_POINT('Ctrl Pts',(65.5415405577955,34.9381179779673,12.));
#169082=CARTESIAN_POINT('Ctrl Pts',(65.5139503038036,34.9363227836582,0.));
#169083=CARTESIAN_POINT('Ctrl Pts',(65.5139503038036,34.9363227836582,12.));
#169084=CARTESIAN_POINT('Ctrl Pts',(65.4863966597544,34.9345049680826,0.));
#169085=CARTESIAN_POINT('Ctrl Pts',(65.4863966597544,34.9345049680826,12.));
#169086=CARTESIAN_POINT('Ctrl Pts',(65.4588797201972,34.932664592394,0.));
#169087=CARTESIAN_POINT('Ctrl Pts',(65.4588797201972,34.932664592394,12.));
#169088=CARTESIAN_POINT('Ctrl Pts',(65.4313995707536,34.9308017105536,0.));
#169089=CARTESIAN_POINT('Ctrl Pts',(65.4313995707536,34.9308017105536,12.));
#169090=CARTESIAN_POINT('Ctrl Pts',(65.4039562911352,34.9289163717747,0.));
#169091=CARTESIAN_POINT('Ctrl Pts',(65.4039562911352,34.9289163717747,12.));
#169092=CARTESIAN_POINT('Ctrl Pts',(65.3765499573077,34.9270086222731,0.));
#169093=CARTESIAN_POINT('Ctrl Pts',(65.3765499573077,34.9270086222731,12.));
#169094=CARTESIAN_POINT('Ctrl Pts',(65.3491806440537,34.9250785073477,0.));
#169095=CARTESIAN_POINT('Ctrl Pts',(65.3491806440537,34.9250785073477,12.));
#169096=CARTESIAN_POINT('Ctrl Pts',(65.321848427191,34.9231260731831,0.));
#169097=CARTESIAN_POINT('Ctrl Pts',(65.321848427191,34.9231260731831,12.));
#169098=CARTESIAN_POINT('Ctrl Pts',(65.2945533863761,34.9211513691355,0.));
#169099=CARTESIAN_POINT('Ctrl Pts',(65.2945533863761,34.9211513691355,12.));
#169100=CARTESIAN_POINT('Ctrl Pts',(65.2672956048069,34.9191544474872,0.));
#169101=CARTESIAN_POINT('Ctrl Pts',(65.2672956048069,34.9191544474872,12.));
#169102=CARTESIAN_POINT('Ctrl Pts',(65.2400751679549,34.9171353624113,0.));
#169103=CARTESIAN_POINT('Ctrl Pts',(65.2400751679549,34.9171353624113,12.));
#169104=CARTESIAN_POINT('Ctrl Pts',(65.2128921625823,34.9150941691747,0.));
#169105=CARTESIAN_POINT('Ctrl Pts',(65.2128921625823,34.9150941691747,12.));
#169106=CARTESIAN_POINT('Ctrl Pts',(65.1857466757092,34.9130309233022,0.));
#169107=CARTESIAN_POINT('Ctrl Pts',(65.1857466757092,34.9130309233022,12.));
#169108=CARTESIAN_POINT('Ctrl Pts',(65.1586387934241,34.9109456796213,0.));
#169109=CARTESIAN_POINT('Ctrl Pts',(65.1586387934241,34.9109456796213,12.));
#169110=CARTESIAN_POINT('Ctrl Pts',(65.1315686003516,34.9088384918336,0.));
#169111=CARTESIAN_POINT('Ctrl Pts',(65.1315686003516,34.9088384918336,12.));
#169112=CARTESIAN_POINT('Ctrl Pts',(65.1045361803121,34.9067094130399,0.));
#169113=CARTESIAN_POINT('Ctrl Pts',(65.1045361803121,34.9067094130399,12.));
#169114=CARTESIAN_POINT('Ctrl Pts',(65.0775416167085,34.9045584960509,0.));
#169115=CARTESIAN_POINT('Ctrl Pts',(65.0775416167085,34.9045584960509,12.));
#169116=CARTESIAN_POINT('Ctrl Pts',(65.0505849930171,34.9023857937865,0.));
#169117=CARTESIAN_POINT('Ctrl Pts',(65.0505849930171,34.9023857937865,12.));
#169118=CARTESIAN_POINT('Ctrl Pts',(65.0236663932328,34.9001913596416,0.));
#169119=CARTESIAN_POINT('Ctrl Pts',(65.0236663932328,34.9001913596416,12.));
#169120=CARTESIAN_POINT('Ctrl Pts',(64.9967859023212,34.8979752478616,0.));
#169121=CARTESIAN_POINT('Ctrl Pts',(64.9967859023212,34.8979752478616,12.));
#169122=CARTESIAN_POINT('Ctrl Pts',(64.9699436060169,34.8957375133697,0.));
#169123=CARTESIAN_POINT('Ctrl Pts',(64.9699436060169,34.8957375133697,12.));
#169124=CARTESIAN_POINT('Ctrl Pts',(64.9431395906337,34.8934782116095,0.));
#169125=CARTESIAN_POINT('Ctrl Pts',(64.9431395906337,34.8934782116095,12.));
#169126=CARTESIAN_POINT('Ctrl Pts',(64.9163739428605,34.8911973983785,0.));
#169127=CARTESIAN_POINT('Ctrl Pts',(64.9163739428605,34.8911973983785,12.));
#169128=CARTESIAN_POINT('Ctrl Pts',(64.8896467495757,34.888895129681,0.));
#169129=CARTESIAN_POINT('Ctrl Pts',(64.8896467495757,34.888895129681,12.));
#169130=CARTESIAN_POINT('Ctrl Pts',(64.8629580976063,34.8865714615436,0.));
#169131=CARTESIAN_POINT('Ctrl Pts',(64.8629580976063,34.8865714615436,12.));
#169132=CARTESIAN_POINT('Ctrl Pts',(64.8363080737377,34.8842264500188,0.));
#169133=CARTESIAN_POINT('Ctrl Pts',(64.8363080737377,34.8842264500188,12.));
#169134=CARTESIAN_POINT('Ctrl Pts',(64.8096967648307,34.881860151273,0.));
#169135=CARTESIAN_POINT('Ctrl Pts',(64.8096967648307,34.881860151273,12.));
#169136=CARTESIAN_POINT('Ctrl Pts',(64.7831242579028,34.8794726216513,0.));
#169137=CARTESIAN_POINT('Ctrl Pts',(64.7831242579028,34.8794726216513,12.));
#169138=CARTESIAN_POINT('Ctrl Pts',(64.7565906402151,34.8770639177493,0.));
#169139=CARTESIAN_POINT('Ctrl Pts',(64.7565906402151,34.8770639177493,12.));
#169140=CARTESIAN_POINT('Ctrl Pts',(64.7300959993653,34.8746340964972,0.));
#169141=CARTESIAN_POINT('Ctrl Pts',(64.7300959993653,34.8746340964972,12.));
#169142=CARTESIAN_POINT('Ctrl Pts',(64.7036404233306,34.8721832151975,0.));
#169143=CARTESIAN_POINT('Ctrl Pts',(64.7036404233306,34.8721832151975,12.));
#169144=CARTESIAN_POINT('Ctrl Pts',(64.6772240004228,34.869711331479,0.));
#169145=CARTESIAN_POINT('Ctrl Pts',(64.6772240004228,34.869711331479,12.));
#169146=CARTESIAN_POINT('Ctrl Pts',(64.6508468192599,34.867218503272,0.));
#169147=CARTESIAN_POINT('Ctrl Pts',(64.6508468192599,34.867218503272,12.));
#169148=CARTESIAN_POINT('Ctrl Pts',(64.6245089687277,34.8647047887774,0.));
#169149=CARTESIAN_POINT('Ctrl Pts',(64.6245089687277,34.8647047887774,12.));
#169150=CARTESIAN_POINT('Ctrl Pts',(64.5982105379383,34.8621702464401,0.));
#169151=CARTESIAN_POINT('Ctrl Pts',(64.5982105379383,34.8621702464401,12.));
#169152=CARTESIAN_POINT('Ctrl Pts',(64.5719516161927,34.8596149349257,0.));
#169153=CARTESIAN_POINT('Ctrl Pts',(64.5719516161927,34.8596149349257,12.));
#169154=CARTESIAN_POINT('Ctrl Pts',(64.5457322930088,34.857038913134,0.));
#169155=CARTESIAN_POINT('Ctrl Pts',(64.5457322930088,34.857038913134,12.));
#169156=CARTESIAN_POINT('Ctrl Pts',(64.5195526581407,34.8544422402118,0.));
#169157=CARTESIAN_POINT('Ctrl Pts',(64.5195526581407,34.8544422402118,12.));
#169158=CARTESIAN_POINT('Ctrl Pts',(64.4934128015985,34.851824975568,0.));
#169159=CARTESIAN_POINT('Ctrl Pts',(64.4934128015985,34.851824975568,12.));
#169160=CARTESIAN_POINT('Ctrl Pts',(64.4673128136625,34.8491871788896,0.));
#169161=CARTESIAN_POINT('Ctrl Pts',(64.4673128136625,34.8491871788896,12.));
#169162=CARTESIAN_POINT('Ctrl Pts',(64.4412527848969,34.8465289101622,0.));
#169163=CARTESIAN_POINT('Ctrl Pts',(64.4412527848969,34.8465289101622,12.));
#169164=CARTESIAN_POINT('Ctrl Pts',(64.4152328061515,34.8438502296664,0.));
#169165=CARTESIAN_POINT('Ctrl Pts',(64.4152328061515,34.8438502296664,12.));
#169166=CARTESIAN_POINT('Ctrl Pts',(64.3892529685607,34.8411511979702,0.));
#169167=CARTESIAN_POINT('Ctrl Pts',(64.3892529685607,34.8411511979702,12.));
#169168=CARTESIAN_POINT('Ctrl Pts',(64.3633133635382,34.8384318759248,0.));
#169169=CARTESIAN_POINT('Ctrl Pts',(64.3633133635382,34.8384318759248,12.));
#169170=CARTESIAN_POINT('Ctrl Pts',(64.3374140827711,34.8356923246618,0.));
#169171=CARTESIAN_POINT('Ctrl Pts',(64.3374140827711,34.8356923246618,12.));
#169172=CARTESIAN_POINT('Ctrl Pts',(64.3115552182062,34.8329326055919,0.));
#169173=CARTESIAN_POINT('Ctrl Pts',(64.3115552182062,34.8329326055919,12.));
#169174=CARTESIAN_POINT('Ctrl Pts',(64.285736862052,34.8301527804054,0.));
#169175=CARTESIAN_POINT('Ctrl Pts',(64.285736862052,34.8301527804054,12.));
#169176=CARTESIAN_POINT('Ctrl Pts',(64.2599591067916,34.8273529110744,0.));
#169177=CARTESIAN_POINT('Ctrl Pts',(64.2599591067916,34.8273529110744,12.));
#169178=CARTESIAN_POINT('Ctrl Pts',(64.234222045188,34.8245330598559,0.));
#169179=CARTESIAN_POINT('Ctrl Pts',(64.234222045188,34.8245330598559,12.));
#169180=CARTESIAN_POINT('Ctrl Pts',(64.2085257702884,34.8216932892969,0.));
#169181=CARTESIAN_POINT('Ctrl Pts',(64.2085257702884,34.8216932892969,12.));
#169182=CARTESIAN_POINT('Ctrl Pts',(64.1828703754236,34.8188336622419,0.));
#169183=CARTESIAN_POINT('Ctrl Pts',(64.1828703754236,34.8188336622419,12.));
#169184=CARTESIAN_POINT('Ctrl Pts',(64.1572559542086,34.8159542418374,0.));
#169185=CARTESIAN_POINT('Ctrl Pts',(64.1572559542086,34.8159542418374,12.));
#169186=CARTESIAN_POINT('Ctrl Pts',(64.1316826005506,34.8130550915287,0.));
#169187=CARTESIAN_POINT('Ctrl Pts',(64.1316826005506,34.8130550915287,12.));
#169188=CARTESIAN_POINT('Ctrl Pts',(64.1061504086515,34.8101362750597,0.));
#169189=CARTESIAN_POINT('Ctrl Pts',(64.1061504086515,34.8101362750597,12.));
#169190=CARTESIAN_POINT('Ctrl Pts',(64.0806594730085,34.8071978564748,0.));
#169191=CARTESIAN_POINT('Ctrl Pts',(64.0806594730085,34.8071978564748,12.));
#169192=CARTESIAN_POINT('Ctrl Pts',(64.0552098884095,34.8042399001211,0.));
#169193=CARTESIAN_POINT('Ctrl Pts',(64.0552098884095,34.8042399001211,12.));
#169194=CARTESIAN_POINT('Ctrl Pts',(64.0298017499294,34.8012624706527,0.));
#169195=CARTESIAN_POINT('Ctrl Pts',(64.0298017499294,34.8012624706527,12.));
#169196=CARTESIAN_POINT('Ctrl Pts',(64.0044351529402,34.7982656330293,0.));
#169197=CARTESIAN_POINT('Ctrl Pts',(64.0044351529402,34.7982656330293,12.));
#169198=CARTESIAN_POINT('Ctrl Pts',(63.9791101931162,34.7952494525178,0.));
#169199=CARTESIAN_POINT('Ctrl Pts',(63.9791101931162,34.7952494525178,12.));
#169200=CARTESIAN_POINT('Ctrl Pts',(63.9538269664366,34.7922139946943,0.));
#169201=CARTESIAN_POINT('Ctrl Pts',(63.9538269664366,34.7922139946943,12.));
#169202=CARTESIAN_POINT('Ctrl Pts',(63.9285855691845,34.7891593254488,0.));
#169203=CARTESIAN_POINT('Ctrl Pts',(63.9285855691845,34.7891593254488,12.));
#169204=CARTESIAN_POINT('Ctrl Pts',(63.9033860979435,34.7860855109911,0.));
#169205=CARTESIAN_POINT('Ctrl Pts',(63.9033860979435,34.7860855109911,12.));
#169206=CARTESIAN_POINT('Ctrl Pts',(63.8782286496062,34.7829926178496,0.));
#169207=CARTESIAN_POINT('Ctrl Pts',(63.8782286496062,34.7829926178496,12.));
#169208=CARTESIAN_POINT('Ctrl Pts',(63.8531133213793,34.7798807128715,0.));
#169209=CARTESIAN_POINT('Ctrl Pts',(63.8531133213793,34.7798807128715,12.));
#169210=CARTESIAN_POINT('Ctrl Pts',(63.8280402107856,34.7767498632243,0.));
#169211=CARTESIAN_POINT('Ctrl Pts',(63.8280402107856,34.7767498632243,12.));
#169212=CARTESIAN_POINT('Ctrl Pts',(63.8030094156639,34.7736001363993,0.));
#169213=CARTESIAN_POINT('Ctrl Pts',(63.8030094156639,34.7736001363993,12.));
#169214=CARTESIAN_POINT('Ctrl Pts',(63.778021034163,34.7704316002171,0.));
#169215=CARTESIAN_POINT('Ctrl Pts',(63.778021034163,34.7704316002171,12.));
#169216=CARTESIAN_POINT('Ctrl Pts',(63.7530751647494,34.7672443228275,0.));
#169217=CARTESIAN_POINT('Ctrl Pts',(63.7530751647494,34.7672443228275,12.));
#169218=CARTESIAN_POINT('Ctrl Pts',(63.7281719062149,34.7640383727101,0.));
#169219=CARTESIAN_POINT('Ctrl Pts',(63.7281719062149,34.7640383727101,12.));
#169220=CARTESIAN_POINT('Ctrl Pts',(63.7033113576785,34.7608138186759,0.));
#169221=CARTESIAN_POINT('Ctrl Pts',(63.7033113576785,34.7608138186759,12.));
#169222=CARTESIAN_POINT('Ctrl Pts',(63.6784936185885,34.7575707298713,0.));
#169223=CARTESIAN_POINT('Ctrl Pts',(63.6784936185885,34.7575707298713,12.));
#169224=CARTESIAN_POINT('Ctrl Pts',(63.6537187887159,34.7543091757833,0.));
#169225=CARTESIAN_POINT('Ctrl Pts',(63.6537187887159,34.7543091757833,12.));
#169226=CARTESIAN_POINT('Ctrl Pts',(63.6289869681604,34.7510292262406,0.));
#169227=CARTESIAN_POINT('Ctrl Pts',(63.6289869681604,34.7510292262406,12.));
#169228=CARTESIAN_POINT('Ctrl Pts',(63.6042982573588,34.7477309514136,0.));
#169229=CARTESIAN_POINT('Ctrl Pts',(63.6042982573588,34.7477309514136,12.));
#169230=CARTESIAN_POINT('Ctrl Pts',(63.5796527570871,34.744414421816,0.));
#169231=CARTESIAN_POINT('Ctrl Pts',(63.5796527570871,34.744414421816,12.));
#169232=CARTESIAN_POINT('Ctrl Pts',(63.5550505684626,34.7410797083081,0.));
#169233=CARTESIAN_POINT('Ctrl Pts',(63.5550505684626,34.7410797083081,12.));
#169234=CARTESIAN_POINT('Ctrl Pts',(63.5304917929386,34.7377268821026,0.));
#169235=CARTESIAN_POINT('Ctrl Pts',(63.5304917929386,34.7377268821026,12.));
#169236=CARTESIAN_POINT('Ctrl Pts',(63.505976532309,34.7343560147667,0.));
#169237=CARTESIAN_POINT('Ctrl Pts',(63.505976532309,34.7343560147667,12.));
#169238=CARTESIAN_POINT('Ctrl Pts',(63.4815048887165,34.7309671782214,0.));
#169239=CARTESIAN_POINT('Ctrl Pts',(63.4815048887165,34.7309671782214,12.));
#169240=CARTESIAN_POINT('Ctrl Pts',(63.4570769646569,34.7275604447439,0.));
#169241=CARTESIAN_POINT('Ctrl Pts',(63.4570769646569,34.7275604447439,12.));
#169242=CARTESIAN_POINT('Ctrl Pts',(63.4326928629795,34.7241358869701,0.));
#169243=CARTESIAN_POINT('Ctrl Pts',(63.4326928629795,34.7241358869701,12.));
#169244=CARTESIAN_POINT('Ctrl Pts',(63.4083526868836,34.7206935779007,0.));
#169245=CARTESIAN_POINT('Ctrl Pts',(63.4083526868836,34.7206935779007,12.));
#169246=CARTESIAN_POINT('Ctrl Pts',(63.3840565399208,34.7172335909038,0.));
#169247=CARTESIAN_POINT('Ctrl Pts',(63.3840565399208,34.7172335909038,12.));
#169248=CARTESIAN_POINT('Ctrl Pts',(63.3598045260053,34.7137559997146,0.));
#169249=CARTESIAN_POINT('Ctrl Pts',(63.3598045260053,34.7137559997146,12.));
#169250=CARTESIAN_POINT('Ctrl Pts',(63.3355967494171,34.7102608784374,0.));
#169251=CARTESIAN_POINT('Ctrl Pts',(63.3355967494171,34.7102608784374,12.));
#169252=CARTESIAN_POINT('Ctrl Pts',(63.3114333148048,34.7067483015491,0.));
#169253=CARTESIAN_POINT('Ctrl Pts',(63.3114333148048,34.7067483015491,12.));
#169254=CARTESIAN_POINT('Ctrl Pts',(63.2873143271806,34.7032183439041,0.));
#169255=CARTESIAN_POINT('Ctrl Pts',(63.2873143271806,34.7032183439041,12.));
#169256=CARTESIAN_POINT('Ctrl Pts',(63.2632398919225,34.6996710807378,0.));
#169257=CARTESIAN_POINT('Ctrl Pts',(63.2632398919225,34.6996710807378,12.));
#169258=CARTESIAN_POINT('Ctrl Pts',(63.2392101147847,34.6961065876666,0.));
#169259=CARTESIAN_POINT('Ctrl Pts',(63.2392101147847,34.6961065876666,12.));
#169260=CARTESIAN_POINT('Ctrl Pts',(63.2152251019012,34.6925249406897,0.));
#169261=CARTESIAN_POINT('Ctrl Pts',(63.2152251019012,34.6925249406897,12.));
#169262=CARTESIAN_POINT('Ctrl Pts',(63.1912849597887,34.6889262161924,0.));
#169263=CARTESIAN_POINT('Ctrl Pts',(63.1912849597887,34.6889262161924,12.));
#169264=CARTESIAN_POINT('Ctrl Pts',(63.1673897953429,34.6853104909518,0.));
#169265=CARTESIAN_POINT('Ctrl Pts',(63.1673897953429,34.6853104909518,12.));
#169266=CARTESIAN_POINT('Ctrl Pts',(63.1435397158388,34.6816778421402,0.));
#169267=CARTESIAN_POINT('Ctrl Pts',(63.1435397158388,34.6816778421402,12.));
#169268=CARTESIAN_POINT('Ctrl Pts',(63.119734828943,34.6780283473252,0.));
#169269=CARTESIAN_POINT('Ctrl Pts',(63.119734828943,34.6780283473252,12.));
#169270=CARTESIAN_POINT('Ctrl Pts',(63.0959752427168,34.674362084472,0.));
#169271=CARTESIAN_POINT('Ctrl Pts',(63.0959752427168,34.674362084472,12.));
#169272=CARTESIAN_POINT('Ctrl Pts',(63.0722610656194,34.670679131947,0.));
#169273=CARTESIAN_POINT('Ctrl Pts',(63.0722610656194,34.670679131947,12.));
#169274=CARTESIAN_POINT('Ctrl Pts',(63.0485924065045,34.6669795685229,0.));
#169275=CARTESIAN_POINT('Ctrl Pts',(63.0485924065045,34.6669795685229,12.));
#169276=CARTESIAN_POINT('Ctrl Pts',(63.0249693746208,34.6632634733824,0.));
#169277=CARTESIAN_POINT('Ctrl Pts',(63.0249693746208,34.6632634733824,12.));
#169278=CARTESIAN_POINT('Ctrl Pts',(63.0013920796235,34.6595309261191,0.));
#169279=CARTESIAN_POINT('Ctrl Pts',(63.0013920796235,34.6595309261191,12.));
#169280=CARTESIAN_POINT('Ctrl Pts',(62.9778606315783,34.6557820067393,0.));
#169281=CARTESIAN_POINT('Ctrl Pts',(62.9778606315783,34.6557820067393,12.));
#169282=CARTESIAN_POINT('Ctrl Pts',(62.9543751409645,34.6520167956655,0.));
#169283=CARTESIAN_POINT('Ctrl Pts',(62.9543751409645,34.6520167956655,12.));
#169284=CARTESIAN_POINT('Ctrl Pts',(62.9309357186717,34.6482353737424,0.));
#169285=CARTESIAN_POINT('Ctrl Pts',(62.9309357186717,34.6482353737424,12.));
#169286=CARTESIAN_POINT('Ctrl Pts',(62.9075424760015,34.6444378222411,0.));
#169287=CARTESIAN_POINT('Ctrl Pts',(62.9075424760015,34.6444378222411,12.));
#169288=CARTESIAN_POINT('Ctrl Pts',(62.8841955246794,34.6406242228592,0.));
#169289=CARTESIAN_POINT('Ctrl Pts',(62.8841955246794,34.6406242228592,12.));
#169290=CARTESIAN_POINT('Ctrl Pts',(62.8608949768571,34.6367946577235,0.));
#169291=CARTESIAN_POINT('Ctrl Pts',(62.8608949768571,34.6367946577235,12.));
#169292=CARTESIAN_POINT('Ctrl Pts',(62.8376409451175,34.6329492093935,0.));
#169293=CARTESIAN_POINT('Ctrl Pts',(62.8376409451175,34.6329492093935,12.));
#169294=CARTESIAN_POINT('Ctrl Pts',(62.8144335424697,34.6290879608673,0.));
#169295=CARTESIAN_POINT('Ctrl Pts',(62.8144335424697,34.6290879608673,12.));
#169296=CARTESIAN_POINT('Ctrl Pts',(62.7912728823518,34.6252109955853,0.));
#169297=CARTESIAN_POINT('Ctrl Pts',(62.7912728823518,34.6252109955853,12.));
#169298=CARTESIAN_POINT('Ctrl Pts',(62.7681590786429,34.6213183974317,0.));
#169299=CARTESIAN_POINT('Ctrl Pts',(62.7681590786429,34.6213183974317,12.));
#169300=CARTESIAN_POINT('Ctrl Pts',(62.7450922456676,34.6174102507375,0.));
#169301=CARTESIAN_POINT('Ctrl Pts',(62.7450922456676,34.6174102507375,12.));
#169302=CARTESIAN_POINT('Ctrl Pts',(62.7220724981994,34.6134866402837,0.));
#169303=CARTESIAN_POINT('Ctrl Pts',(62.7220724981994,34.6134866402837,12.));
#169304=CARTESIAN_POINT('Ctrl Pts',(62.6990999514563,34.6095476513077,0.));
#169305=CARTESIAN_POINT('Ctrl Pts',(62.6990999514563,34.6095476513077,12.));
#169306=CARTESIAN_POINT('Ctrl Pts',(62.6761747211037,34.6055933695069,0.));
#169307=CARTESIAN_POINT('Ctrl Pts',(62.6761747211037,34.6055933695069,12.));
#169308=CARTESIAN_POINT('Ctrl Pts',(62.6532969232657,34.6016238810399,0.));
#169309=CARTESIAN_POINT('Ctrl Pts',(62.6532969232657,34.6016238810399,12.));
#169310=CARTESIAN_POINT('Ctrl Pts',(62.6304666745306,34.5976392725296,0.));
#169311=CARTESIAN_POINT('Ctrl Pts',(62.6304666745306,34.5976392725296,12.));
#169312=CARTESIAN_POINT('Ctrl Pts',(62.6076840919536,34.5936396310679,0.));
#169313=CARTESIAN_POINT('Ctrl Pts',(62.6076840919536,34.5936396310679,12.));
#169314=CARTESIAN_POINT('Ctrl Pts',(62.5849492930533,34.5896250442216,0.));
#169315=CARTESIAN_POINT('Ctrl Pts',(62.5849492930533,34.5896250442216,12.));
#169316=CARTESIAN_POINT('Ctrl Pts',(62.562262395816,34.5855956000363,0.));
#169317=CARTESIAN_POINT('Ctrl Pts',(62.562262395816,34.5855956000363,12.));
#169318=CARTESIAN_POINT('Ctrl Pts',(62.5396235187079,34.5815513870377,0.));
#169319=CARTESIAN_POINT('Ctrl Pts',(62.5396235187079,34.5815513870377,12.));
#169320=CARTESIAN_POINT('Ctrl Pts',(62.5170327806781,34.5774924942355,0.));
#169321=CARTESIAN_POINT('Ctrl Pts',(62.5170327806781,34.5774924942355,12.));
#169322=CARTESIAN_POINT('Ctrl Pts',(62.4944903011628,34.5734190111272,0.));
#169323=CARTESIAN_POINT('Ctrl Pts',(62.4944903011628,34.5734190111272,12.));
#169324=CARTESIAN_POINT('Ctrl Pts',(62.4719962000808,34.5693310277051,0.));
#169325=CARTESIAN_POINT('Ctrl Pts',(62.4719962000808,34.5693310277051,12.));
#169326=CARTESIAN_POINT('Ctrl Pts',(62.4495505978393,34.5652286344593,0.));
#169327=CARTESIAN_POINT('Ctrl Pts',(62.4495505978393,34.5652286344593,12.));
#169328=CARTESIAN_POINT('Ctrl Pts',(62.4271536153459,34.5611119223799,0.));
#169329=CARTESIAN_POINT('Ctrl Pts',(62.4271536153459,34.5611119223799,12.));
#169330=CARTESIAN_POINT('Ctrl Pts',(62.4048053740127,34.5569809829613,0.));
#169331=CARTESIAN_POINT('Ctrl Pts',(62.4048053740127,34.5569809829613,12.));
#169332=CARTESIAN_POINT('Ctrl Pts',(62.3825059957601,34.5528359082075,0.));
#169333=CARTESIAN_POINT('Ctrl Pts',(62.3825059957601,34.5528359082075,12.));
#169334=CARTESIAN_POINT('Ctrl Pts',(62.3602556030127,34.5486767906384,0.));
#169335=CARTESIAN_POINT('Ctrl Pts',(62.3602556030127,34.5486767906384,12.));
#169336=CARTESIAN_POINT('Ctrl Pts',(62.338054318708,34.5445037232936,0.));
#169337=CARTESIAN_POINT('Ctrl Pts',(62.338054318708,34.5445037232936,12.));
#169338=CARTESIAN_POINT('Ctrl Pts',(62.3159022663058,34.5403167997337,0.));
#169339=CARTESIAN_POINT('Ctrl Pts',(62.3159022663058,34.5403167997337,12.));
#169340=CARTESIAN_POINT('Ctrl Pts',(62.2937995697925,34.5361161140449,0.));
#169341=CARTESIAN_POINT('Ctrl Pts',(62.2937995697925,34.5361161140449,12.));
#169342=CARTESIAN_POINT('Ctrl Pts',(62.2717463536827,34.5319017608433,0.));
#169343=CARTESIAN_POINT('Ctrl Pts',(62.2717463536827,34.5319017608433,12.));
#169344=CARTESIAN_POINT('Ctrl Pts',(62.2497427430135,34.5276738352808,0.));
#169345=CARTESIAN_POINT('Ctrl Pts',(62.2497427430135,34.5276738352808,12.));
#169346=CARTESIAN_POINT('Ctrl Pts',(62.2277888633576,34.5234324330491,0.));
#169347=CARTESIAN_POINT('Ctrl Pts',(62.2277888633576,34.5234324330491,12.));
#169348=CARTESIAN_POINT('Ctrl Pts',(62.2058848408347,34.5191776503842,0.));
#169349=CARTESIAN_POINT('Ctrl Pts',(62.2058848408347,34.5191776503842,12.));
#169350=CARTESIAN_POINT('Ctrl Pts',(62.1840308021171,34.514909584073,0.));
#169351=CARTESIAN_POINT('Ctrl Pts',(62.1840308021171,34.514909584073,12.));
#169352=CARTESIAN_POINT('Ctrl Pts',(62.1622268744336,34.5106283314594,0.));
#169353=CARTESIAN_POINT('Ctrl Pts',(62.1622268744336,34.5106283314594,12.));
#169354=CARTESIAN_POINT('Ctrl Pts',(62.1404731855686,34.5063339904533,0.));
#169355=CARTESIAN_POINT('Ctrl Pts',(62.1404731855686,34.5063339904533,12.));
#169356=CARTESIAN_POINT('Ctrl Pts',(62.1187698638705,34.5020266595292,0.));
#169357=CARTESIAN_POINT('Ctrl Pts',(62.1187698638705,34.5020266595292,12.));
#169358=CARTESIAN_POINT('Ctrl Pts',(62.0971170382565,34.4977064377281,0.));
#169359=CARTESIAN_POINT('Ctrl Pts',(62.0971170382565,34.4977064377281,12.));
#169360=CARTESIAN_POINT('Ctrl Pts',(62.0755148382136,34.4933734246593,0.));
#169361=CARTESIAN_POINT('Ctrl Pts',(62.0755148382136,34.4933734246593,12.));
#169362=CARTESIAN_POINT('Ctrl Pts',(62.0539633937944,34.4890277205042,0.));
#169363=CARTESIAN_POINT('Ctrl Pts',(62.0539633937944,34.4890277205042,12.));
#169364=CARTESIAN_POINT('Ctrl Pts',(62.0324628356152,34.4846694260205,0.));
#169365=CARTESIAN_POINT('Ctrl Pts',(62.0324628356152,34.4846694260205,12.));
#169366=CARTESIAN_POINT('Ctrl Pts',(62.0110132948807,34.4802986425535,0.));
#169367=CARTESIAN_POINT('Ctrl Pts',(62.0110132948807,34.4802986425535,12.));
#169368=CARTESIAN_POINT('Ctrl Pts',(61.9896149034009,34.4759154720477,0.));
#169369=CARTESIAN_POINT('Ctrl Pts',(61.9896149034009,34.4759154720477,12.));
#169370=CARTESIAN_POINT('Ctrl Pts',(61.9682677936048,34.4715200170589,0.));
#169371=CARTESIAN_POINT('Ctrl Pts',(61.9682677936048,34.4715200170589,12.));
#169372=CARTESIAN_POINT('Ctrl Pts',(61.9469720985512,34.4671123807706,0.));
#169373=CARTESIAN_POINT('Ctrl Pts',(61.9469720985512,34.4671123807706,12.));
#169374=CARTESIAN_POINT('Ctrl Pts',(61.9257279519283,34.462692666996,0.));
#169375=CARTESIAN_POINT('Ctrl Pts',(61.9257279519283,34.462692666996,12.));
#169376=CARTESIAN_POINT('Ctrl Pts',(61.9045354880424,34.4582609801625,0.));
#169377=CARTESIAN_POINT('Ctrl Pts',(61.9045354880424,34.4582609801625,12.));
#169378=CARTESIAN_POINT('Ctrl Pts',(61.883394841802,34.4538174253009,0.));
#169379=CARTESIAN_POINT('Ctrl Pts',(61.883394841802,34.4538174253009,12.));
#169380=CARTESIAN_POINT('Ctrl Pts',(61.862306148703,34.4493621080367,0.));
#169381=CARTESIAN_POINT('Ctrl Pts',(61.862306148703,34.4493621080367,12.));
#169382=CARTESIAN_POINT('Ctrl Pts',(61.8412695447951,34.4448951345753,0.));
#169383=CARTESIAN_POINT('Ctrl Pts',(61.8412695447951,34.4448951345753,12.));
#169384=CARTESIAN_POINT('Ctrl Pts',(61.8202851667247,34.4404166117313,0.));
#169385=CARTESIAN_POINT('Ctrl Pts',(61.8202851667247,34.4404166117313,12.));
#169386=CARTESIAN_POINT('Ctrl Pts',(61.7993531518052,34.4359266469757,0.));
#169387=CARTESIAN_POINT('Ctrl Pts',(61.7993531518052,34.4359266469757,12.));
#169388=CARTESIAN_POINT('Ctrl Pts',(61.7784736380727,34.4314253484792,0.));
#169389=CARTESIAN_POINT('Ctrl Pts',(61.7784736380727,34.4314253484792,12.));
#169390=CARTESIAN_POINT('Ctrl Pts',(61.7576467643419,34.4269128251569,0.));
#169391=CARTESIAN_POINT('Ctrl Pts',(61.7576467643419,34.4269128251569,12.));
#169392=CARTESIAN_POINT('Ctrl Pts',(61.7368726702573,34.4223891867166,0.));
#169393=CARTESIAN_POINT('Ctrl Pts',(61.7368726702573,34.4223891867166,12.));
#169394=CARTESIAN_POINT('Ctrl Pts',(61.7161514961892,34.4178545435753,0.));
#169395=CARTESIAN_POINT('Ctrl Pts',(61.7161514961892,34.4178545435753,12.));
#169396=CARTESIAN_POINT('Ctrl Pts',(61.6954833831157,34.4133090067696,0.));
#169397=CARTESIAN_POINT('Ctrl Pts',(61.6954833831157,34.4133090067696,12.));
#169398=CARTESIAN_POINT('Ctrl Pts',(61.674868472521,34.4087526878815,0.));
#169399=CARTESIAN_POINT('Ctrl Pts',(61.674868472521,34.4087526878815,12.));
#169400=CARTESIAN_POINT('Ctrl Pts',(61.6543069062436,34.4041856989328,0.));
#169401=CARTESIAN_POINT('Ctrl Pts',(61.6543069062436,34.4041856989328,12.));
#169402=CARTESIAN_POINT('Ctrl Pts',(61.6337988264586,34.399608152377,0.));
#169403=CARTESIAN_POINT('Ctrl Pts',(61.6337988264586,34.399608152377,12.));
#169404=CARTESIAN_POINT('Ctrl Pts',(61.6133443760168,34.3950201613446,0.));
#169405=CARTESIAN_POINT('Ctrl Pts',(61.6133443760168,34.3950201613446,12.));
#169406=CARTESIAN_POINT('Ctrl Pts',(61.5929436987419,34.3904218398642,0.));
#169407=CARTESIAN_POINT('Ctrl Pts',(61.5929436987419,34.3904218398642,12.));
#169408=CARTESIAN_POINT('Ctrl Pts',(61.5725969396817,34.3858133030511,0.));
#169409=CARTESIAN_POINT('Ctrl Pts',(61.5725969396817,34.3858133030511,12.));
#169410=CARTESIAN_POINT('Ctrl Pts',(61.5523042455127,34.3811946674179,0.));
#169411=CARTESIAN_POINT('Ctrl Pts',(61.5523042455127,34.3811946674179,12.));
#169412=CARTESIAN_POINT('Ctrl Pts',(61.5320657642601,34.3765660506659,0.));
#169413=CARTESIAN_POINT('Ctrl Pts',(61.5320657642601,34.3765660506659,12.));
#169414=CARTESIAN_POINT('Ctrl Pts',(61.511881644541,34.3719275711179,0.));
#169415=CARTESIAN_POINT('Ctrl Pts',(61.511881644541,34.3719275711179,12.));
#169416=CARTESIAN_POINT('Ctrl Pts',(61.4917520349276,34.3672793472464,0.));
#169417=CARTESIAN_POINT('Ctrl Pts',(61.4917520349276,34.3672793472464,12.));
#169418=CARTESIAN_POINT('Ctrl Pts',(61.4716770832924,34.3626214971903,0.));
#169419=CARTESIAN_POINT('Ctrl Pts',(61.4716770832924,34.3626214971903,12.));
#169420=CARTESIAN_POINT('Ctrl Pts',(61.4516569360499,34.357954138202,0.));
#169421=CARTESIAN_POINT('Ctrl Pts',(61.4516569360499,34.357954138202,12.));
#169422=CARTESIAN_POINT('Ctrl Pts',(61.4316917395959,34.3532773877112,0.));
#169423=CARTESIAN_POINT('Ctrl Pts',(61.4316917395959,34.3532773877112,12.));
#169424=CARTESIAN_POINT('Ctrl Pts',(61.4117816420251,34.3485913645991,0.));
#169425=CARTESIAN_POINT('Ctrl Pts',(61.4117816420251,34.3485913645991,12.));
#169426=CARTESIAN_POINT('Ctrl Pts',(61.3919267945293,34.34389619024,0.));
#169427=CARTESIAN_POINT('Ctrl Pts',(61.3919267945293,34.34389619024,12.));
#169428=CARTESIAN_POINT('Ctrl Pts',(61.3721273534222,34.339191990012,0.));
#169429=CARTESIAN_POINT('Ctrl Pts',(61.3721273534222,34.339191990012,12.));
#169430=CARTESIAN_POINT('Ctrl Pts',(61.3523834803144,34.3344788934337,0.));
#169431=CARTESIAN_POINT('Ctrl Pts',(61.3523834803144,34.3344788934337,12.));
#169432=CARTESIAN_POINT('Ctrl Pts',(61.3326953378817,34.3297570310126,0.));
#169433=CARTESIAN_POINT('Ctrl Pts',(61.3326953378817,34.3297570310126,12.));
#169434=CARTESIAN_POINT('Ctrl Pts',(61.3130630861375,34.3250265314761,0.));
#169435=CARTESIAN_POINT('Ctrl Pts',(61.3130630861375,34.3250265314761,12.));
#169436=CARTESIAN_POINT('Ctrl Pts',(61.2934868791875,34.3202875193629,0.));
#169437=CARTESIAN_POINT('Ctrl Pts',(61.2934868791875,34.3202875193629,12.));
#169438=CARTESIAN_POINT('Ctrl Pts',(61.2739668600415,34.3155401111777,0.));
#169439=CARTESIAN_POINT('Ctrl Pts',(61.2739668600415,34.3155401111777,12.));
#169440=CARTESIAN_POINT('Ctrl Pts',(61.2545031656196,34.3107844191081,0.));
#169441=CARTESIAN_POINT('Ctrl Pts',(61.2545031656196,34.3107844191081,12.));
#169442=CARTESIAN_POINT('Ctrl Pts',(61.2350959366987,34.3060205584093,0.));
#169443=CARTESIAN_POINT('Ctrl Pts',(61.2350959366987,34.3060205584093,12.));
#169444=CARTESIAN_POINT('Ctrl Pts',(61.2157453259107,34.3012486533474,0.));
#169445=CARTESIAN_POINT('Ctrl Pts',(61.2157453259107,34.3012486533474,12.));
#169446=CARTESIAN_POINT('Ctrl Pts',(61.1964515073823,34.296468844362,0.));
#169447=CARTESIAN_POINT('Ctrl Pts',(61.1964515073823,34.296468844362,12.));
#169448=CARTESIAN_POINT('Ctrl Pts',(61.1772146833083,34.2916812929675,0.));
#169449=CARTESIAN_POINT('Ctrl Pts',(61.1772146833083,34.2916812929675,12.));
#169450=CARTESIAN_POINT('Ctrl Pts',(61.15803506354,34.2868861666301,0.));
#169451=CARTESIAN_POINT('Ctrl Pts',(61.15803506354,34.2868861666301,12.));
#169452=CARTESIAN_POINT('Ctrl Pts',(61.1389128461815,34.2820836244425,0.));
#169453=CARTESIAN_POINT('Ctrl Pts',(61.1389128461815,34.2820836244425,12.));
#169454=CARTESIAN_POINT('Ctrl Pts',(61.119848199783,34.2772738038812,0.));
#169455=CARTESIAN_POINT('Ctrl Pts',(61.119848199783,34.2772738038812,12.));
#169456=CARTESIAN_POINT('Ctrl Pts',(61.100841240023,34.2724568037374,0.));
#169457=CARTESIAN_POINT('Ctrl Pts',(61.100841240023,34.2724568037374,12.));
#169458=CARTESIAN_POINT('Ctrl Pts',(61.0818920286644,34.2676326825846,0.));
#169459=CARTESIAN_POINT('Ctrl Pts',(61.0818920286644,34.2676326825846,12.));
#169460=CARTESIAN_POINT('Ctrl Pts',(61.0667788793594,34.2637677132139,0.));
#169461=CARTESIAN_POINT('Ctrl Pts',(61.0667788793594,34.2637677132139,12.));
#169462=CARTESIAN_POINT('Ctrl Pts',(61.0554700177206,34.2608658001761,0.));
#169463=CARTESIAN_POINT('Ctrl Pts',(61.0554700177206,34.2608658001761,12.));
#169464=CARTESIAN_POINT('Ctrl Pts',(61.0479423318803,34.2589297755482,0.));
#169465=CARTESIAN_POINT('Ctrl Pts',(61.0479423318803,34.2589297755482,12.));
#169466=CARTESIAN_POINT('Ctrl Pts',(61.0441813777723,34.2579614092497,0.));
#169467=CARTESIAN_POINT('Ctrl Pts',(61.0441813777723,34.2579614092497,12.));
#169468=CARTESIAN_POINT('',(61.0441813777723,34.2579614092497,12.));
#169469=CARTESIAN_POINT('Ctrl Pts',(61.0441813777723,34.2579614092497,12.));
#169470=CARTESIAN_POINT('Ctrl Pts',(61.0479423318803,34.2589297755482,12.));
#169471=CARTESIAN_POINT('Ctrl Pts',(61.0554700177206,34.2608658001761,12.));
#169472=CARTESIAN_POINT('Ctrl Pts',(61.0667788793594,34.2637677132139,12.));
#169473=CARTESIAN_POINT('Ctrl Pts',(61.0818920286644,34.2676326825846,12.));
#169474=CARTESIAN_POINT('Ctrl Pts',(61.100841240023,34.2724568037374,12.));
#169475=CARTESIAN_POINT('Ctrl Pts',(61.119848199783,34.2772738038812,12.));
#169476=CARTESIAN_POINT('Ctrl Pts',(61.1389128461815,34.2820836244425,12.));
#169477=CARTESIAN_POINT('Ctrl Pts',(61.15803506354,34.2868861666301,12.));
#169478=CARTESIAN_POINT('Ctrl Pts',(61.1772146833083,34.2916812929675,12.));
#169479=CARTESIAN_POINT('Ctrl Pts',(61.1964515073823,34.296468844362,12.));
#169480=CARTESIAN_POINT('Ctrl Pts',(61.2157453259107,34.3012486533474,12.));
#169481=CARTESIAN_POINT('Ctrl Pts',(61.2350959366987,34.3060205584093,12.));
#169482=CARTESIAN_POINT('Ctrl Pts',(61.2545031656196,34.3107844191081,12.));
#169483=CARTESIAN_POINT('Ctrl Pts',(61.2739668600415,34.3155401111777,12.));
#169484=CARTESIAN_POINT('Ctrl Pts',(61.2934868791875,34.3202875193629,12.));
#169485=CARTESIAN_POINT('Ctrl Pts',(61.3130630861375,34.3250265314761,12.));
#169486=CARTESIAN_POINT('Ctrl Pts',(61.3326953378817,34.3297570310126,12.));
#169487=CARTESIAN_POINT('Ctrl Pts',(61.3523834803144,34.3344788934337,12.));
#169488=CARTESIAN_POINT('Ctrl Pts',(61.3721273534222,34.339191990012,12.));
#169489=CARTESIAN_POINT('Ctrl Pts',(61.3919267945293,34.34389619024,12.));
#169490=CARTESIAN_POINT('Ctrl Pts',(61.4117816420251,34.3485913645991,12.));
#169491=CARTESIAN_POINT('Ctrl Pts',(61.4316917395959,34.3532773877112,12.));
#169492=CARTESIAN_POINT('Ctrl Pts',(61.4516569360499,34.357954138202,12.));
#169493=CARTESIAN_POINT('Ctrl Pts',(61.4716770832924,34.3626214971903,12.));
#169494=CARTESIAN_POINT('Ctrl Pts',(61.4917520349276,34.3672793472464,12.));
#169495=CARTESIAN_POINT('Ctrl Pts',(61.511881644541,34.3719275711179,12.));
#169496=CARTESIAN_POINT('Ctrl Pts',(61.5320657642601,34.3765660506659,12.));
#169497=CARTESIAN_POINT('Ctrl Pts',(61.5523042455127,34.3811946674179,12.));
#169498=CARTESIAN_POINT('Ctrl Pts',(61.5725969396817,34.3858133030511,12.));
#169499=CARTESIAN_POINT('Ctrl Pts',(61.5929436987419,34.3904218398642,12.));
#169500=CARTESIAN_POINT('Ctrl Pts',(61.6133443760168,34.3950201613446,12.));
#169501=CARTESIAN_POINT('Ctrl Pts',(61.6337988264586,34.399608152377,12.));
#169502=CARTESIAN_POINT('Ctrl Pts',(61.6543069062436,34.4041856989328,12.));
#169503=CARTESIAN_POINT('Ctrl Pts',(61.674868472521,34.4087526878815,12.));
#169504=CARTESIAN_POINT('Ctrl Pts',(61.6954833831157,34.4133090067696,12.));
#169505=CARTESIAN_POINT('Ctrl Pts',(61.7161514961892,34.4178545435753,12.));
#169506=CARTESIAN_POINT('Ctrl Pts',(61.7368726702573,34.4223891867166,12.));
#169507=CARTESIAN_POINT('Ctrl Pts',(61.7576467643419,34.4269128251569,12.));
#169508=CARTESIAN_POINT('Ctrl Pts',(61.7784736380727,34.4314253484792,12.));
#169509=CARTESIAN_POINT('Ctrl Pts',(61.7993531518052,34.4359266469757,12.));
#169510=CARTESIAN_POINT('Ctrl Pts',(61.8202851667247,34.4404166117313,12.));
#169511=CARTESIAN_POINT('Ctrl Pts',(61.8412695447951,34.4448951345753,12.));
#169512=CARTESIAN_POINT('Ctrl Pts',(61.862306148703,34.4493621080367,12.));
#169513=CARTESIAN_POINT('Ctrl Pts',(61.883394841802,34.4538174253009,12.));
#169514=CARTESIAN_POINT('Ctrl Pts',(61.9045354880424,34.4582609801625,12.));
#169515=CARTESIAN_POINT('Ctrl Pts',(61.9257279519283,34.462692666996,12.));
#169516=CARTESIAN_POINT('Ctrl Pts',(61.9469720985512,34.4671123807706,12.));
#169517=CARTESIAN_POINT('Ctrl Pts',(61.9682677936048,34.4715200170589,12.));
#169518=CARTESIAN_POINT('Ctrl Pts',(61.9896149034009,34.4759154720477,12.));
#169519=CARTESIAN_POINT('Ctrl Pts',(62.0110132948807,34.4802986425535,12.));
#169520=CARTESIAN_POINT('Ctrl Pts',(62.0324628356152,34.4846694260205,12.));
#169521=CARTESIAN_POINT('Ctrl Pts',(62.0539633937944,34.4890277205042,12.));
#169522=CARTESIAN_POINT('Ctrl Pts',(62.0755148382136,34.4933734246593,12.));
#169523=CARTESIAN_POINT('Ctrl Pts',(62.0971170382565,34.4977064377281,12.));
#169524=CARTESIAN_POINT('Ctrl Pts',(62.1187698638705,34.5020266595292,12.));
#169525=CARTESIAN_POINT('Ctrl Pts',(62.1404731855686,34.5063339904533,12.));
#169526=CARTESIAN_POINT('Ctrl Pts',(62.1622268744336,34.5106283314594,12.));
#169527=CARTESIAN_POINT('Ctrl Pts',(62.1840308021171,34.514909584073,12.));
#169528=CARTESIAN_POINT('Ctrl Pts',(62.2058848408347,34.5191776503842,12.));
#169529=CARTESIAN_POINT('Ctrl Pts',(62.2277888633576,34.5234324330491,12.));
#169530=CARTESIAN_POINT('Ctrl Pts',(62.2497427430135,34.5276738352808,12.));
#169531=CARTESIAN_POINT('Ctrl Pts',(62.2717463536827,34.5319017608433,12.));
#169532=CARTESIAN_POINT('Ctrl Pts',(62.2937995697925,34.5361161140449,12.));
#169533=CARTESIAN_POINT('Ctrl Pts',(62.3159022663058,34.5403167997337,12.));
#169534=CARTESIAN_POINT('Ctrl Pts',(62.338054318708,34.5445037232936,12.));
#169535=CARTESIAN_POINT('Ctrl Pts',(62.3602556030127,34.5486767906384,12.));
#169536=CARTESIAN_POINT('Ctrl Pts',(62.3825059957601,34.5528359082075,12.));
#169537=CARTESIAN_POINT('Ctrl Pts',(62.4048053740127,34.5569809829613,12.));
#169538=CARTESIAN_POINT('Ctrl Pts',(62.4271536153459,34.5611119223799,12.));
#169539=CARTESIAN_POINT('Ctrl Pts',(62.4495505978393,34.5652286344593,12.));
#169540=CARTESIAN_POINT('Ctrl Pts',(62.4719962000808,34.5693310277051,12.));
#169541=CARTESIAN_POINT('Ctrl Pts',(62.4944903011628,34.5734190111272,12.));
#169542=CARTESIAN_POINT('Ctrl Pts',(62.5170327806781,34.5774924942355,12.));
#169543=CARTESIAN_POINT('Ctrl Pts',(62.5396235187079,34.5815513870377,12.));
#169544=CARTESIAN_POINT('Ctrl Pts',(62.562262395816,34.5855956000363,12.));
#169545=CARTESIAN_POINT('Ctrl Pts',(62.5849492930533,34.5896250442216,12.));
#169546=CARTESIAN_POINT('Ctrl Pts',(62.6076840919536,34.5936396310679,12.));
#169547=CARTESIAN_POINT('Ctrl Pts',(62.6304666745306,34.5976392725296,12.));
#169548=CARTESIAN_POINT('Ctrl Pts',(62.6532969232657,34.6016238810399,12.));
#169549=CARTESIAN_POINT('Ctrl Pts',(62.6761747211037,34.6055933695069,12.));
#169550=CARTESIAN_POINT('Ctrl Pts',(62.6990999514563,34.6095476513077,12.));
#169551=CARTESIAN_POINT('Ctrl Pts',(62.7220724981994,34.6134866402837,12.));
#169552=CARTESIAN_POINT('Ctrl Pts',(62.7450922456676,34.6174102507375,12.));
#169553=CARTESIAN_POINT('Ctrl Pts',(62.7681590786429,34.6213183974317,12.));
#169554=CARTESIAN_POINT('Ctrl Pts',(62.7912728823518,34.6252109955853,12.));
#169555=CARTESIAN_POINT('Ctrl Pts',(62.8144335424697,34.6290879608673,12.));
#169556=CARTESIAN_POINT('Ctrl Pts',(62.8376409451175,34.6329492093935,12.));
#169557=CARTESIAN_POINT('Ctrl Pts',(62.8608949768571,34.6367946577235,12.));
#169558=CARTESIAN_POINT('Ctrl Pts',(62.8841955246794,34.6406242228592,12.));
#169559=CARTESIAN_POINT('Ctrl Pts',(62.9075424760015,34.6444378222411,12.));
#169560=CARTESIAN_POINT('Ctrl Pts',(62.9309357186717,34.6482353737424,12.));
#169561=CARTESIAN_POINT('Ctrl Pts',(62.9543751409645,34.6520167956655,12.));
#169562=CARTESIAN_POINT('Ctrl Pts',(62.9778606315783,34.6557820067393,12.));
#169563=CARTESIAN_POINT('Ctrl Pts',(63.0013920796235,34.6595309261191,12.));
#169564=CARTESIAN_POINT('Ctrl Pts',(63.0249693746208,34.6632634733824,12.));
#169565=CARTESIAN_POINT('Ctrl Pts',(63.0485924065045,34.6669795685229,12.));
#169566=CARTESIAN_POINT('Ctrl Pts',(63.0722610656194,34.670679131947,12.));
#169567=CARTESIAN_POINT('Ctrl Pts',(63.0959752427168,34.674362084472,12.));
#169568=CARTESIAN_POINT('Ctrl Pts',(63.119734828943,34.6780283473252,12.));
#169569=CARTESIAN_POINT('Ctrl Pts',(63.1435397158388,34.6816778421402,12.));
#169570=CARTESIAN_POINT('Ctrl Pts',(63.1673897953429,34.6853104909518,12.));
#169571=CARTESIAN_POINT('Ctrl Pts',(63.1912849597887,34.6889262161924,12.));
#169572=CARTESIAN_POINT('Ctrl Pts',(63.2152251019012,34.6925249406897,12.));
#169573=CARTESIAN_POINT('Ctrl Pts',(63.2392101147847,34.6961065876666,12.));
#169574=CARTESIAN_POINT('Ctrl Pts',(63.2632398919225,34.6996710807378,12.));
#169575=CARTESIAN_POINT('Ctrl Pts',(63.2873143271806,34.7032183439041,12.));
#169576=CARTESIAN_POINT('Ctrl Pts',(63.3114333148048,34.7067483015491,12.));
#169577=CARTESIAN_POINT('Ctrl Pts',(63.3355967494171,34.7102608784374,12.));
#169578=CARTESIAN_POINT('Ctrl Pts',(63.3598045260053,34.7137559997146,12.));
#169579=CARTESIAN_POINT('Ctrl Pts',(63.3840565399208,34.7172335909038,12.));
#169580=CARTESIAN_POINT('Ctrl Pts',(63.4083526868836,34.7206935779007,12.));
#169581=CARTESIAN_POINT('Ctrl Pts',(63.4326928629795,34.7241358869701,12.));
#169582=CARTESIAN_POINT('Ctrl Pts',(63.4570769646569,34.7275604447439,12.));
#169583=CARTESIAN_POINT('Ctrl Pts',(63.4815048887165,34.7309671782214,12.));
#169584=CARTESIAN_POINT('Ctrl Pts',(63.505976532309,34.7343560147667,12.));
#169585=CARTESIAN_POINT('Ctrl Pts',(63.5304917929386,34.7377268821026,12.));
#169586=CARTESIAN_POINT('Ctrl Pts',(63.5550505684626,34.7410797083081,12.));
#169587=CARTESIAN_POINT('Ctrl Pts',(63.5796527570871,34.744414421816,12.));
#169588=CARTESIAN_POINT('Ctrl Pts',(63.6042982573588,34.7477309514136,12.));
#169589=CARTESIAN_POINT('Ctrl Pts',(63.6289869681604,34.7510292262406,12.));
#169590=CARTESIAN_POINT('Ctrl Pts',(63.6537187887159,34.7543091757833,12.));
#169591=CARTESIAN_POINT('Ctrl Pts',(63.6784936185885,34.7575707298713,12.));
#169592=CARTESIAN_POINT('Ctrl Pts',(63.7033113576785,34.7608138186759,12.));
#169593=CARTESIAN_POINT('Ctrl Pts',(63.7281719062149,34.7640383727101,12.));
#169594=CARTESIAN_POINT('Ctrl Pts',(63.7530751647494,34.7672443228275,12.));
#169595=CARTESIAN_POINT('Ctrl Pts',(63.778021034163,34.7704316002171,12.));
#169596=CARTESIAN_POINT('Ctrl Pts',(63.8030094156639,34.7736001363993,12.));
#169597=CARTESIAN_POINT('Ctrl Pts',(63.8280402107856,34.7767498632243,12.));
#169598=CARTESIAN_POINT('Ctrl Pts',(63.8531133213793,34.7798807128715,12.));
#169599=CARTESIAN_POINT('Ctrl Pts',(63.8782286496062,34.7829926178496,12.));
#169600=CARTESIAN_POINT('Ctrl Pts',(63.9033860979435,34.7860855109911,12.));
#169601=CARTESIAN_POINT('Ctrl Pts',(63.9285855691845,34.7891593254488,12.));
#169602=CARTESIAN_POINT('Ctrl Pts',(63.9538269664366,34.7922139946943,12.));
#169603=CARTESIAN_POINT('Ctrl Pts',(63.9791101931162,34.7952494525178,12.));
#169604=CARTESIAN_POINT('Ctrl Pts',(64.0044351529402,34.7982656330293,12.));
#169605=CARTESIAN_POINT('Ctrl Pts',(64.0298017499294,34.8012624706527,12.));
#169606=CARTESIAN_POINT('Ctrl Pts',(64.0552098884095,34.8042399001211,12.));
#169607=CARTESIAN_POINT('Ctrl Pts',(64.0806594730085,34.8071978564748,12.));
#169608=CARTESIAN_POINT('Ctrl Pts',(64.1061504086515,34.8101362750597,12.));
#169609=CARTESIAN_POINT('Ctrl Pts',(64.1316826005506,34.8130550915287,12.));
#169610=CARTESIAN_POINT('Ctrl Pts',(64.1572559542086,34.8159542418374,12.));
#169611=CARTESIAN_POINT('Ctrl Pts',(64.1828703754236,34.8188336622419,12.));
#169612=CARTESIAN_POINT('Ctrl Pts',(64.2085257702884,34.8216932892969,12.));
#169613=CARTESIAN_POINT('Ctrl Pts',(64.234222045188,34.8245330598559,12.));
#169614=CARTESIAN_POINT('Ctrl Pts',(64.2599591067916,34.8273529110744,12.));
#169615=CARTESIAN_POINT('Ctrl Pts',(64.285736862052,34.8301527804054,12.));
#169616=CARTESIAN_POINT('Ctrl Pts',(64.3115552182062,34.8329326055919,12.));
#169617=CARTESIAN_POINT('Ctrl Pts',(64.3374140827711,34.8356923246618,12.));
#169618=CARTESIAN_POINT('Ctrl Pts',(64.3633133635382,34.8384318759248,12.));
#169619=CARTESIAN_POINT('Ctrl Pts',(64.3892529685607,34.8411511979702,12.));
#169620=CARTESIAN_POINT('Ctrl Pts',(64.4152328061515,34.8438502296664,12.));
#169621=CARTESIAN_POINT('Ctrl Pts',(64.4412527848969,34.8465289101622,12.));
#169622=CARTESIAN_POINT('Ctrl Pts',(64.4673128136625,34.8491871788896,12.));
#169623=CARTESIAN_POINT('Ctrl Pts',(64.4934128015985,34.851824975568,12.));
#169624=CARTESIAN_POINT('Ctrl Pts',(64.5195526581407,34.8544422402118,12.));
#169625=CARTESIAN_POINT('Ctrl Pts',(64.5457322930088,34.857038913134,12.));
#169626=CARTESIAN_POINT('Ctrl Pts',(64.5719516161927,34.8596149349257,12.));
#169627=CARTESIAN_POINT('Ctrl Pts',(64.5982105379383,34.8621702464401,12.));
#169628=CARTESIAN_POINT('Ctrl Pts',(64.6245089687277,34.8647047887774,12.));
#169629=CARTESIAN_POINT('Ctrl Pts',(64.6508468192599,34.867218503272,12.));
#169630=CARTESIAN_POINT('Ctrl Pts',(64.6772240004228,34.869711331479,12.));
#169631=CARTESIAN_POINT('Ctrl Pts',(64.7036404233306,34.8721832151975,12.));
#169632=CARTESIAN_POINT('Ctrl Pts',(64.7300959993653,34.8746340964972,12.));
#169633=CARTESIAN_POINT('Ctrl Pts',(64.7565906402151,34.8770639177493,12.));
#169634=CARTESIAN_POINT('Ctrl Pts',(64.7831242579028,34.8794726216513,12.));
#169635=CARTESIAN_POINT('Ctrl Pts',(64.8096967648307,34.881860151273,12.));
#169636=CARTESIAN_POINT('Ctrl Pts',(64.8363080737377,34.8842264500188,12.));
#169637=CARTESIAN_POINT('Ctrl Pts',(64.8629580976063,34.8865714615436,12.));
#169638=CARTESIAN_POINT('Ctrl Pts',(64.8896467495757,34.888895129681,12.));
#169639=CARTESIAN_POINT('Ctrl Pts',(64.9163739428605,34.8911973983785,12.));
#169640=CARTESIAN_POINT('Ctrl Pts',(64.9431395906337,34.8934782116095,12.));
#169641=CARTESIAN_POINT('Ctrl Pts',(64.9699436060169,34.8957375133697,12.));
#169642=CARTESIAN_POINT('Ctrl Pts',(64.9967859023212,34.8979752478616,12.));
#169643=CARTESIAN_POINT('Ctrl Pts',(65.0236663932328,34.9001913596416,12.));
#169644=CARTESIAN_POINT('Ctrl Pts',(65.0505849930171,34.9023857937865,12.));
#169645=CARTESIAN_POINT('Ctrl Pts',(65.0775416167085,34.9045584960509,12.));
#169646=CARTESIAN_POINT('Ctrl Pts',(65.1045361803121,34.9067094130399,12.));
#169647=CARTESIAN_POINT('Ctrl Pts',(65.1315686003516,34.9088384918336,12.));
#169648=CARTESIAN_POINT('Ctrl Pts',(65.1586387934241,34.9109456796213,12.));
#169649=CARTESIAN_POINT('Ctrl Pts',(65.1857466757092,34.9130309233022,12.));
#169650=CARTESIAN_POINT('Ctrl Pts',(65.2128921625823,34.9150941691747,12.));
#169651=CARTESIAN_POINT('Ctrl Pts',(65.2400751679549,34.9171353624113,12.));
#169652=CARTESIAN_POINT('Ctrl Pts',(65.2672956048069,34.9191544474872,12.));
#169653=CARTESIAN_POINT('Ctrl Pts',(65.2945533863761,34.9211513691355,12.));
#169654=CARTESIAN_POINT('Ctrl Pts',(65.321848427191,34.9231260731831,12.));
#169655=CARTESIAN_POINT('Ctrl Pts',(65.3491806440537,34.9250785073477,12.));
#169656=CARTESIAN_POINT('Ctrl Pts',(65.3765499573077,34.9270086222731,12.));
#169657=CARTESIAN_POINT('Ctrl Pts',(65.4039562911352,34.9289163717747,12.));
#169658=CARTESIAN_POINT('Ctrl Pts',(65.4274804996589,34.9305324724445,12.));
#169659=CARTESIAN_POINT('Ctrl Pts',(65.4455359575246,34.931759381316,12.));
#169660=CARTESIAN_POINT('Ctrl Pts',(65.4581063193885,34.9326070346645,12.));
#169661=CARTESIAN_POINT('Ctrl Pts',(65.4651808010812,34.9330820191535,12.));
#169662=CARTESIAN_POINT('Ctrl Pts',(65.4667541478387,34.933187552314,12.));
#169663=CARTESIAN_POINT('',(61.0441813777723,34.2579614092497,0.));
#169664=CARTESIAN_POINT('',(61.0441813777723,34.2579614092497,0.));
#169665=CARTESIAN_POINT('Ctrl Pts',(65.4667541478388,34.933187552314,0.));
#169666=CARTESIAN_POINT('Ctrl Pts',(65.4651808010814,34.9330820191535,0.));
#169667=CARTESIAN_POINT('Ctrl Pts',(65.4581063193886,34.9326070346645,0.));
#169668=CARTESIAN_POINT('Ctrl Pts',(65.4455359575246,34.931759381316,0.));
#169669=CARTESIAN_POINT('Ctrl Pts',(65.427480499659,34.9305324724445,0.));
#169670=CARTESIAN_POINT('Ctrl Pts',(65.4039562911352,34.9289163717747,0.));
#169671=CARTESIAN_POINT('Ctrl Pts',(65.3765499573077,34.9270086222731,0.));
#169672=CARTESIAN_POINT('Ctrl Pts',(65.3491806440537,34.9250785073477,0.));
#169673=CARTESIAN_POINT('Ctrl Pts',(65.321848427191,34.9231260731831,0.));
#169674=CARTESIAN_POINT('Ctrl Pts',(65.2945533863761,34.9211513691355,0.));
#169675=CARTESIAN_POINT('Ctrl Pts',(65.2672956048069,34.9191544474872,0.));
#169676=CARTESIAN_POINT('Ctrl Pts',(65.2400751679549,34.9171353624113,0.));
#169677=CARTESIAN_POINT('Ctrl Pts',(65.2128921625823,34.9150941691747,0.));
#169678=CARTESIAN_POINT('Ctrl Pts',(65.1857466757092,34.9130309233022,0.));
#169679=CARTESIAN_POINT('Ctrl Pts',(65.1586387934241,34.9109456796213,0.));
#169680=CARTESIAN_POINT('Ctrl Pts',(65.1315686003516,34.9088384918336,0.));
#169681=CARTESIAN_POINT('Ctrl Pts',(65.1045361803121,34.9067094130399,0.));
#169682=CARTESIAN_POINT('Ctrl Pts',(65.0775416167085,34.9045584960509,0.));
#169683=CARTESIAN_POINT('Ctrl Pts',(65.0505849930171,34.9023857937865,0.));
#169684=CARTESIAN_POINT('Ctrl Pts',(65.0236663932328,34.9001913596416,0.));
#169685=CARTESIAN_POINT('Ctrl Pts',(64.9967859023212,34.8979752478616,0.));
#169686=CARTESIAN_POINT('Ctrl Pts',(64.9699436060169,34.8957375133697,0.));
#169687=CARTESIAN_POINT('Ctrl Pts',(64.9431395906337,34.8934782116095,0.));
#169688=CARTESIAN_POINT('Ctrl Pts',(64.9163739428605,34.8911973983785,0.));
#169689=CARTESIAN_POINT('Ctrl Pts',(64.8896467495757,34.888895129681,0.));
#169690=CARTESIAN_POINT('Ctrl Pts',(64.8629580976063,34.8865714615436,0.));
#169691=CARTESIAN_POINT('Ctrl Pts',(64.8363080737377,34.8842264500188,0.));
#169692=CARTESIAN_POINT('Ctrl Pts',(64.8096967648307,34.881860151273,0.));
#169693=CARTESIAN_POINT('Ctrl Pts',(64.7831242579028,34.8794726216513,0.));
#169694=CARTESIAN_POINT('Ctrl Pts',(64.7565906402151,34.8770639177493,0.));
#169695=CARTESIAN_POINT('Ctrl Pts',(64.7300959993653,34.8746340964972,0.));
#169696=CARTESIAN_POINT('Ctrl Pts',(64.7036404233306,34.8721832151975,0.));
#169697=CARTESIAN_POINT('Ctrl Pts',(64.6772240004228,34.869711331479,0.));
#169698=CARTESIAN_POINT('Ctrl Pts',(64.6508468192599,34.867218503272,0.));
#169699=CARTESIAN_POINT('Ctrl Pts',(64.6245089687277,34.8647047887774,0.));
#169700=CARTESIAN_POINT('Ctrl Pts',(64.5982105379383,34.8621702464401,0.));
#169701=CARTESIAN_POINT('Ctrl Pts',(64.5719516161927,34.8596149349257,0.));
#169702=CARTESIAN_POINT('Ctrl Pts',(64.5457322930088,34.857038913134,0.));
#169703=CARTESIAN_POINT('Ctrl Pts',(64.5195526581407,34.8544422402118,0.));
#169704=CARTESIAN_POINT('Ctrl Pts',(64.4934128015985,34.851824975568,0.));
#169705=CARTESIAN_POINT('Ctrl Pts',(64.4673128136625,34.8491871788896,0.));
#169706=CARTESIAN_POINT('Ctrl Pts',(64.4412527848969,34.8465289101622,0.));
#169707=CARTESIAN_POINT('Ctrl Pts',(64.4152328061515,34.8438502296664,0.));
#169708=CARTESIAN_POINT('Ctrl Pts',(64.3892529685607,34.8411511979702,0.));
#169709=CARTESIAN_POINT('Ctrl Pts',(64.3633133635382,34.8384318759248,0.));
#169710=CARTESIAN_POINT('Ctrl Pts',(64.3374140827711,34.8356923246618,0.));
#169711=CARTESIAN_POINT('Ctrl Pts',(64.3115552182062,34.8329326055919,0.));
#169712=CARTESIAN_POINT('Ctrl Pts',(64.285736862052,34.8301527804054,0.));
#169713=CARTESIAN_POINT('Ctrl Pts',(64.2599591067916,34.8273529110744,0.));
#169714=CARTESIAN_POINT('Ctrl Pts',(64.234222045188,34.8245330598559,0.));
#169715=CARTESIAN_POINT('Ctrl Pts',(64.2085257702884,34.8216932892969,0.));
#169716=CARTESIAN_POINT('Ctrl Pts',(64.1828703754236,34.8188336622419,0.));
#169717=CARTESIAN_POINT('Ctrl Pts',(64.1572559542086,34.8159542418374,0.));
#169718=CARTESIAN_POINT('Ctrl Pts',(64.1316826005506,34.8130550915287,0.));
#169719=CARTESIAN_POINT('Ctrl Pts',(64.1061504086515,34.8101362750597,0.));
#169720=CARTESIAN_POINT('Ctrl Pts',(64.0806594730085,34.8071978564748,0.));
#169721=CARTESIAN_POINT('Ctrl Pts',(64.0552098884095,34.8042399001211,0.));
#169722=CARTESIAN_POINT('Ctrl Pts',(64.0298017499294,34.8012624706527,0.));
#169723=CARTESIAN_POINT('Ctrl Pts',(64.0044351529402,34.7982656330293,0.));
#169724=CARTESIAN_POINT('Ctrl Pts',(63.9791101931162,34.7952494525178,0.));
#169725=CARTESIAN_POINT('Ctrl Pts',(63.9538269664366,34.7922139946943,0.));
#169726=CARTESIAN_POINT('Ctrl Pts',(63.9285855691845,34.7891593254488,0.));
#169727=CARTESIAN_POINT('Ctrl Pts',(63.9033860979435,34.7860855109911,0.));
#169728=CARTESIAN_POINT('Ctrl Pts',(63.8782286496062,34.7829926178496,0.));
#169729=CARTESIAN_POINT('Ctrl Pts',(63.8531133213793,34.7798807128715,0.));
#169730=CARTESIAN_POINT('Ctrl Pts',(63.8280402107856,34.7767498632243,0.));
#169731=CARTESIAN_POINT('Ctrl Pts',(63.8030094156639,34.7736001363993,0.));
#169732=CARTESIAN_POINT('Ctrl Pts',(63.778021034163,34.7704316002171,0.));
#169733=CARTESIAN_POINT('Ctrl Pts',(63.7530751647494,34.7672443228275,0.));
#169734=CARTESIAN_POINT('Ctrl Pts',(63.7281719062149,34.7640383727101,0.));
#169735=CARTESIAN_POINT('Ctrl Pts',(63.7033113576785,34.7608138186759,0.));
#169736=CARTESIAN_POINT('Ctrl Pts',(63.6784936185885,34.7575707298713,0.));
#169737=CARTESIAN_POINT('Ctrl Pts',(63.6537187887159,34.7543091757833,0.));
#169738=CARTESIAN_POINT('Ctrl Pts',(63.6289869681604,34.7510292262406,0.));
#169739=CARTESIAN_POINT('Ctrl Pts',(63.6042982573588,34.7477309514136,0.));
#169740=CARTESIAN_POINT('Ctrl Pts',(63.5796527570871,34.744414421816,0.));
#169741=CARTESIAN_POINT('Ctrl Pts',(63.5550505684626,34.7410797083081,0.));
#169742=CARTESIAN_POINT('Ctrl Pts',(63.5304917929386,34.7377268821026,0.));
#169743=CARTESIAN_POINT('Ctrl Pts',(63.505976532309,34.7343560147667,0.));
#169744=CARTESIAN_POINT('Ctrl Pts',(63.4815048887165,34.7309671782214,0.));
#169745=CARTESIAN_POINT('Ctrl Pts',(63.4570769646569,34.7275604447439,0.));
#169746=CARTESIAN_POINT('Ctrl Pts',(63.4326928629795,34.7241358869701,0.));
#169747=CARTESIAN_POINT('Ctrl Pts',(63.4083526868836,34.7206935779007,0.));
#169748=CARTESIAN_POINT('Ctrl Pts',(63.3840565399208,34.7172335909038,0.));
#169749=CARTESIAN_POINT('Ctrl Pts',(63.3598045260053,34.7137559997146,0.));
#169750=CARTESIAN_POINT('Ctrl Pts',(63.3355967494171,34.7102608784374,0.));
#169751=CARTESIAN_POINT('Ctrl Pts',(63.3114333148048,34.7067483015491,0.));
#169752=CARTESIAN_POINT('Ctrl Pts',(63.2873143271806,34.7032183439041,0.));
#169753=CARTESIAN_POINT('Ctrl Pts',(63.2632398919225,34.6996710807378,0.));
#169754=CARTESIAN_POINT('Ctrl Pts',(63.2392101147847,34.6961065876666,0.));
#169755=CARTESIAN_POINT('Ctrl Pts',(63.2152251019012,34.6925249406897,0.));
#169756=CARTESIAN_POINT('Ctrl Pts',(63.1912849597887,34.6889262161924,0.));
#169757=CARTESIAN_POINT('Ctrl Pts',(63.1673897953429,34.6853104909518,0.));
#169758=CARTESIAN_POINT('Ctrl Pts',(63.1435397158388,34.6816778421402,0.));
#169759=CARTESIAN_POINT('Ctrl Pts',(63.119734828943,34.6780283473252,0.));
#169760=CARTESIAN_POINT('Ctrl Pts',(63.0959752427168,34.674362084472,0.));
#169761=CARTESIAN_POINT('Ctrl Pts',(63.0722610656194,34.670679131947,0.));
#169762=CARTESIAN_POINT('Ctrl Pts',(63.0485924065045,34.6669795685229,0.));
#169763=CARTESIAN_POINT('Ctrl Pts',(63.0249693746208,34.6632634733824,0.));
#169764=CARTESIAN_POINT('Ctrl Pts',(63.0013920796235,34.6595309261191,0.));
#169765=CARTESIAN_POINT('Ctrl Pts',(62.9778606315783,34.6557820067393,0.));
#169766=CARTESIAN_POINT('Ctrl Pts',(62.9543751409645,34.6520167956655,0.));
#169767=CARTESIAN_POINT('Ctrl Pts',(62.9309357186717,34.6482353737424,0.));
#169768=CARTESIAN_POINT('Ctrl Pts',(62.9075424760015,34.6444378222411,0.));
#169769=CARTESIAN_POINT('Ctrl Pts',(62.8841955246794,34.6406242228592,0.));
#169770=CARTESIAN_POINT('Ctrl Pts',(62.8608949768571,34.6367946577235,0.));
#169771=CARTESIAN_POINT('Ctrl Pts',(62.8376409451175,34.6329492093935,0.));
#169772=CARTESIAN_POINT('Ctrl Pts',(62.8144335424697,34.6290879608673,0.));
#169773=CARTESIAN_POINT('Ctrl Pts',(62.7912728823518,34.6252109955853,0.));
#169774=CARTESIAN_POINT('Ctrl Pts',(62.7681590786429,34.6213183974317,0.));
#169775=CARTESIAN_POINT('Ctrl Pts',(62.7450922456676,34.6174102507375,0.));
#169776=CARTESIAN_POINT('Ctrl Pts',(62.7220724981994,34.6134866402837,0.));
#169777=CARTESIAN_POINT('Ctrl Pts',(62.6990999514563,34.6095476513077,0.));
#169778=CARTESIAN_POINT('Ctrl Pts',(62.6761747211037,34.6055933695069,0.));
#169779=CARTESIAN_POINT('Ctrl Pts',(62.6532969232657,34.6016238810399,0.));
#169780=CARTESIAN_POINT('Ctrl Pts',(62.6304666745306,34.5976392725296,0.));
#169781=CARTESIAN_POINT('Ctrl Pts',(62.6076840919536,34.5936396310679,0.));
#169782=CARTESIAN_POINT('Ctrl Pts',(62.5849492930533,34.5896250442216,0.));
#169783=CARTESIAN_POINT('Ctrl Pts',(62.562262395816,34.5855956000363,0.));
#169784=CARTESIAN_POINT('Ctrl Pts',(62.5396235187079,34.5815513870377,0.));
#169785=CARTESIAN_POINT('Ctrl Pts',(62.5170327806781,34.5774924942355,0.));
#169786=CARTESIAN_POINT('Ctrl Pts',(62.4944903011628,34.5734190111272,0.));
#169787=CARTESIAN_POINT('Ctrl Pts',(62.4719962000808,34.5693310277051,0.));
#169788=CARTESIAN_POINT('Ctrl Pts',(62.4495505978393,34.5652286344593,0.));
#169789=CARTESIAN_POINT('Ctrl Pts',(62.4271536153459,34.5611119223799,0.));
#169790=CARTESIAN_POINT('Ctrl Pts',(62.4048053740127,34.5569809829613,0.));
#169791=CARTESIAN_POINT('Ctrl Pts',(62.3825059957601,34.5528359082075,0.));
#169792=CARTESIAN_POINT('Ctrl Pts',(62.3602556030127,34.5486767906384,0.));
#169793=CARTESIAN_POINT('Ctrl Pts',(62.338054318708,34.5445037232936,0.));
#169794=CARTESIAN_POINT('Ctrl Pts',(62.3159022663058,34.5403167997337,0.));
#169795=CARTESIAN_POINT('Ctrl Pts',(62.2937995697925,34.5361161140449,0.));
#169796=CARTESIAN_POINT('Ctrl Pts',(62.2717463536827,34.5319017608433,0.));
#169797=CARTESIAN_POINT('Ctrl Pts',(62.2497427430135,34.5276738352808,0.));
#169798=CARTESIAN_POINT('Ctrl Pts',(62.2277888633576,34.5234324330491,0.));
#169799=CARTESIAN_POINT('Ctrl Pts',(62.2058848408347,34.5191776503842,0.));
#169800=CARTESIAN_POINT('Ctrl Pts',(62.1840308021171,34.514909584073,0.));
#169801=CARTESIAN_POINT('Ctrl Pts',(62.1622268744336,34.5106283314594,0.));
#169802=CARTESIAN_POINT('Ctrl Pts',(62.1404731855686,34.5063339904533,0.));
#169803=CARTESIAN_POINT('Ctrl Pts',(62.1187698638705,34.5020266595292,0.));
#169804=CARTESIAN_POINT('Ctrl Pts',(62.0971170382565,34.4977064377281,0.));
#169805=CARTESIAN_POINT('Ctrl Pts',(62.0755148382136,34.4933734246593,0.));
#169806=CARTESIAN_POINT('Ctrl Pts',(62.0539633937944,34.4890277205042,0.));
#169807=CARTESIAN_POINT('Ctrl Pts',(62.0324628356152,34.4846694260205,0.));
#169808=CARTESIAN_POINT('Ctrl Pts',(62.0110132948807,34.4802986425535,0.));
#169809=CARTESIAN_POINT('Ctrl Pts',(61.9896149034009,34.4759154720477,0.));
#169810=CARTESIAN_POINT('Ctrl Pts',(61.9682677936048,34.4715200170589,0.));
#169811=CARTESIAN_POINT('Ctrl Pts',(61.9469720985512,34.4671123807706,0.));
#169812=CARTESIAN_POINT('Ctrl Pts',(61.9257279519283,34.462692666996,0.));
#169813=CARTESIAN_POINT('Ctrl Pts',(61.9045354880424,34.4582609801625,0.));
#169814=CARTESIAN_POINT('Ctrl Pts',(61.883394841802,34.4538174253009,0.));
#169815=CARTESIAN_POINT('Ctrl Pts',(61.862306148703,34.4493621080367,0.));
#169816=CARTESIAN_POINT('Ctrl Pts',(61.8412695447951,34.4448951345753,0.));
#169817=CARTESIAN_POINT('Ctrl Pts',(61.8202851667247,34.4404166117313,0.));
#169818=CARTESIAN_POINT('Ctrl Pts',(61.7993531518052,34.4359266469757,0.));
#169819=CARTESIAN_POINT('Ctrl Pts',(61.7784736380727,34.4314253484792,0.));
#169820=CARTESIAN_POINT('Ctrl Pts',(61.7576467643419,34.4269128251569,0.));
#169821=CARTESIAN_POINT('Ctrl Pts',(61.7368726702573,34.4223891867166,0.));
#169822=CARTESIAN_POINT('Ctrl Pts',(61.7161514961892,34.4178545435753,0.));
#169823=CARTESIAN_POINT('Ctrl Pts',(61.6954833831157,34.4133090067696,0.));
#169824=CARTESIAN_POINT('Ctrl Pts',(61.674868472521,34.4087526878815,0.));
#169825=CARTESIAN_POINT('Ctrl Pts',(61.6543069062436,34.4041856989328,0.));
#169826=CARTESIAN_POINT('Ctrl Pts',(61.6337988264586,34.399608152377,0.));
#169827=CARTESIAN_POINT('Ctrl Pts',(61.6133443760168,34.3950201613446,0.));
#169828=CARTESIAN_POINT('Ctrl Pts',(61.5929436987419,34.3904218398642,0.));
#169829=CARTESIAN_POINT('Ctrl Pts',(61.5725969396817,34.3858133030511,0.));
#169830=CARTESIAN_POINT('Ctrl Pts',(61.5523042455127,34.3811946674179,0.));
#169831=CARTESIAN_POINT('Ctrl Pts',(61.5320657642601,34.3765660506659,0.));
#169832=CARTESIAN_POINT('Ctrl Pts',(61.511881644541,34.3719275711179,0.));
#169833=CARTESIAN_POINT('Ctrl Pts',(61.4917520349276,34.3672793472464,0.));
#169834=CARTESIAN_POINT('Ctrl Pts',(61.4716770832924,34.3626214971903,0.));
#169835=CARTESIAN_POINT('Ctrl Pts',(61.4516569360499,34.357954138202,0.));
#169836=CARTESIAN_POINT('Ctrl Pts',(61.4316917395959,34.3532773877112,0.));
#169837=CARTESIAN_POINT('Ctrl Pts',(61.4117816420251,34.3485913645991,0.));
#169838=CARTESIAN_POINT('Ctrl Pts',(61.3919267945293,34.34389619024,0.));
#169839=CARTESIAN_POINT('Ctrl Pts',(61.3721273534222,34.339191990012,0.));
#169840=CARTESIAN_POINT('Ctrl Pts',(61.3523834803144,34.3344788934337,0.));
#169841=CARTESIAN_POINT('Ctrl Pts',(61.3326953378817,34.3297570310126,0.));
#169842=CARTESIAN_POINT('Ctrl Pts',(61.3130630861375,34.3250265314761,0.));
#169843=CARTESIAN_POINT('Ctrl Pts',(61.2934868791875,34.3202875193629,0.));
#169844=CARTESIAN_POINT('Ctrl Pts',(61.2739668600415,34.3155401111777,0.));
#169845=CARTESIAN_POINT('Ctrl Pts',(61.2545031656196,34.3107844191081,0.));
#169846=CARTESIAN_POINT('Ctrl Pts',(61.2350959366987,34.3060205584093,0.));
#169847=CARTESIAN_POINT('Ctrl Pts',(61.2157453259107,34.3012486533474,0.));
#169848=CARTESIAN_POINT('Ctrl Pts',(61.1964515073823,34.296468844362,0.));
#169849=CARTESIAN_POINT('Ctrl Pts',(61.1772146833083,34.2916812929675,0.));
#169850=CARTESIAN_POINT('Ctrl Pts',(61.15803506354,34.2868861666301,0.));
#169851=CARTESIAN_POINT('Ctrl Pts',(61.1389128461815,34.2820836244425,0.));
#169852=CARTESIAN_POINT('Ctrl Pts',(61.119848199783,34.2772738038812,0.));
#169853=CARTESIAN_POINT('Ctrl Pts',(61.100841240023,34.2724568037374,0.));
#169854=CARTESIAN_POINT('Ctrl Pts',(61.0818920286644,34.2676326825846,0.));
#169855=CARTESIAN_POINT('Ctrl Pts',(61.0667788793594,34.2637677132139,0.));
#169856=CARTESIAN_POINT('Ctrl Pts',(61.0554700177206,34.2608658001761,0.));
#169857=CARTESIAN_POINT('Ctrl Pts',(61.0479423318803,34.2589297755482,0.));
#169858=CARTESIAN_POINT('Ctrl Pts',(61.0441813777723,34.2579614092497,0.));
#169859=CARTESIAN_POINT('Ctrl Pts',(68.5875145916629,29.0861280018229,0.));
#169860=CARTESIAN_POINT('Ctrl Pts',(68.5875145916629,29.0861280018229,12.));
#169861=CARTESIAN_POINT('Ctrl Pts',(68.5819214834737,29.0863005247839,0.));
#169862=CARTESIAN_POINT('Ctrl Pts',(68.5819214834737,29.0863005247839,12.));
#169863=CARTESIAN_POINT('Ctrl Pts',(68.5707386600636,29.0866429722093,0.));
#169864=CARTESIAN_POINT('Ctrl Pts',(68.5707386600636,29.0866429722093,12.));
#169865=CARTESIAN_POINT('Ctrl Pts',(68.5539746038542,29.0871488478589,0.));
#169866=CARTESIAN_POINT('Ctrl Pts',(68.5539746038542,29.0871488478589,12.));
#169867=CARTESIAN_POINT('Ctrl Pts',(68.5316428875424,29.0878077571086,0.));
#169868=CARTESIAN_POINT('Ctrl Pts',(68.5316428875424,29.0878077571086,12.));
#169869=CARTESIAN_POINT('Ctrl Pts',(68.5037621824171,29.0886054060563,0.));
#169870=CARTESIAN_POINT('Ctrl Pts',(68.5037621824171,29.0886054060563,12.));
#169871=CARTESIAN_POINT('Ctrl Pts',(68.4759154367939,29.0893770688944,0.));
#169872=CARTESIAN_POINT('Ctrl Pts',(68.4759154367939,29.0893770688944,12.));
#169873=CARTESIAN_POINT('Ctrl Pts',(68.4481026830931,29.0901227535307,0.));
#169874=CARTESIAN_POINT('Ctrl Pts',(68.4481026830931,29.0901227535307,12.));
#169875=CARTESIAN_POINT('Ctrl Pts',(68.4203239694612,29.090842477089,0.));
#169876=CARTESIAN_POINT('Ctrl Pts',(68.4203239694612,29.090842477089,12.));
#169877=CARTESIAN_POINT('Ctrl Pts',(68.3925793637995,29.0915362699455,0.));
#169878=CARTESIAN_POINT('Ctrl Pts',(68.3925793637995,29.0915362699455,12.));
#169879=CARTESIAN_POINT('Ctrl Pts',(68.364868951893,29.0922041749294,0.));
#169880=CARTESIAN_POINT('Ctrl Pts',(68.364868951893,29.0922041749294,12.));
#169881=CARTESIAN_POINT('Ctrl Pts',(68.3371928310161,29.0928462428145,0.));
#169882=CARTESIAN_POINT('Ctrl Pts',(68.3371928310161,29.0928462428145,12.));
#169883=CARTESIAN_POINT('Ctrl Pts',(68.3095511047769,29.0934625288409,0.));
#169884=CARTESIAN_POINT('Ctrl Pts',(68.3095511047769,29.0934625288409,12.));
#169885=CARTESIAN_POINT('Ctrl Pts',(68.2819438775953,29.0940530889149,0.));
#169886=CARTESIAN_POINT('Ctrl Pts',(68.2819438775953,29.0940530889149,12.));
#169887=CARTESIAN_POINT('Ctrl Pts',(68.2543712489906,29.0946179757167,0.));
#169888=CARTESIAN_POINT('Ctrl Pts',(68.2543712489906,29.0946179757167,12.));
#169889=CARTESIAN_POINT('Ctrl Pts',(68.2268333089617,29.0951572355397,0.));
#169890=CARTESIAN_POINT('Ctrl Pts',(68.2268333089617,29.0951572355397,12.));
#169891=CARTESIAN_POINT('Ctrl Pts',(68.1993301412061,29.0956709104627,0.));
#169892=CARTESIAN_POINT('Ctrl Pts',(68.1993301412061,29.0956709104627,12.));
#169893=CARTESIAN_POINT('Ctrl Pts',(68.1718618254281,29.0961590399046,0.));
#169894=CARTESIAN_POINT('Ctrl Pts',(68.1718618254281,29.0961590399046,12.));
#169895=CARTESIAN_POINT('Ctrl Pts',(68.1444284400742,29.0966216624743,0.));
#169896=CARTESIAN_POINT('Ctrl Pts',(68.1444284400742,29.0966216624743,12.));
#169897=CARTESIAN_POINT('Ctrl Pts',(68.1170300646987,29.0970588175728,0.));
#169898=CARTESIAN_POINT('Ctrl Pts',(68.1170300646987,29.0970588175728,12.));
#169899=CARTESIAN_POINT('Ctrl Pts',(68.0896667829567,29.0974705474259,0.));
#169900=CARTESIAN_POINT('Ctrl Pts',(68.0896667829567,29.0974705474259,12.));
#169901=CARTESIAN_POINT('Ctrl Pts',(68.0623386822863,29.0978568968657,0.));
#169902=CARTESIAN_POINT('Ctrl Pts',(68.0623386822863,29.0978568968657,12.));
#169903=CARTESIAN_POINT('Ctrl Pts',(68.0350458525551,29.0982179124097,0.));
#169904=CARTESIAN_POINT('Ctrl Pts',(68.0350458525551,29.0982179124097,12.));
#169905=CARTESIAN_POINT('Ctrl Pts',(68.0077883850121,29.0985536415531,0.));
#169906=CARTESIAN_POINT('Ctrl Pts',(68.0077883850121,29.0985536415531,12.));
#169907=CARTESIAN_POINT('Ctrl Pts',(67.9805663711855,29.0988641320247,0.));
#169908=CARTESIAN_POINT('Ctrl Pts',(67.9805663711855,29.0988641320247,12.));
#169909=CARTESIAN_POINT('Ctrl Pts',(67.9533799016148,29.0991494309404,0.));
#169910=CARTESIAN_POINT('Ctrl Pts',(67.9533799016148,29.0991494309404,12.));
#169911=CARTESIAN_POINT('Ctrl Pts',(67.9262290652829,29.099409584422,0.));
#169912=CARTESIAN_POINT('Ctrl Pts',(67.9262290652829,29.099409584422,12.));
#169913=CARTESIAN_POINT('Ctrl Pts',(67.8991139503193,29.0996446380626,0.));
#169914=CARTESIAN_POINT('Ctrl Pts',(67.8991139503193,29.0996446380626,12.));
#169915=CARTESIAN_POINT('Ctrl Pts',(67.8720346444124,29.0998546372032,0.));
#169916=CARTESIAN_POINT('Ctrl Pts',(67.8720346444124,29.0998546372032,12.));
#169917=CARTESIAN_POINT('Ctrl Pts',(67.8449912353329,29.1000396272867,0.));
#169918=CARTESIAN_POINT('Ctrl Pts',(67.8449912353329,29.1000396272867,12.));
#169919=CARTESIAN_POINT('Ctrl Pts',(67.8179838114099,29.1001996541842,0.));
#169920=CARTESIAN_POINT('Ctrl Pts',(67.8179838114099,29.1001996541842,12.));
#169921=CARTESIAN_POINT('Ctrl Pts',(67.7910124620135,29.1003347645294,0.));
#169922=CARTESIAN_POINT('Ctrl Pts',(67.7910124620135,29.1003347645294,12.));
#169923=CARTESIAN_POINT('Ctrl Pts',(67.7640772773387,29.1004450055643,0.));
#169924=CARTESIAN_POINT('Ctrl Pts',(67.7640772773387,29.1004450055643,12.));
#169925=CARTESIAN_POINT('Ctrl Pts',(67.7371783482035,29.1005304249987,0.));
#169926=CARTESIAN_POINT('Ctrl Pts',(67.7371783482035,29.1005304249987,12.));
#169927=CARTESIAN_POINT('Ctrl Pts',(67.7103157658296,29.1005910708624,0.));
#169928=CARTESIAN_POINT('Ctrl Pts',(67.7103157658296,29.1005910708624,12.));
#169929=CARTESIAN_POINT('Ctrl Pts',(67.6834896216461,29.1006269913747,0.));
#169930=CARTESIAN_POINT('Ctrl Pts',(67.6834896216461,29.1006269913747,12.));
#169931=CARTESIAN_POINT('Ctrl Pts',(67.6567000070326,29.1006382347814,0.));
#169932=CARTESIAN_POINT('Ctrl Pts',(67.6567000070326,29.1006382347814,12.));
#169933=CARTESIAN_POINT('Ctrl Pts',(67.6299470133295,29.100624849358,0.));
#169934=CARTESIAN_POINT('Ctrl Pts',(67.6299470133295,29.100624849358,12.));
#169935=CARTESIAN_POINT('Ctrl Pts',(67.6032307319623,29.1005868834866,0.));
#169936=CARTESIAN_POINT('Ctrl Pts',(67.6032307319623,29.1005868834866,12.));
#169937=CARTESIAN_POINT('Ctrl Pts',(67.5765512545281,29.1005243857139,0.));
#169938=CARTESIAN_POINT('Ctrl Pts',(67.5765512545281,29.1005243857139,12.));
#169939=CARTESIAN_POINT('Ctrl Pts',(67.5499086728888,29.1004374048148,0.));
#169940=CARTESIAN_POINT('Ctrl Pts',(67.5499086728888,29.1004374048148,12.));
#169941=CARTESIAN_POINT('Ctrl Pts',(67.5233030792704,29.1003259898682,0.));
#169942=CARTESIAN_POINT('Ctrl Pts',(67.5233030792704,29.1003259898682,12.));
#169943=CARTESIAN_POINT('Ctrl Pts',(67.4967345663096,29.1001901902909,0.));
#169944=CARTESIAN_POINT('Ctrl Pts',(67.4967345663096,29.1001901902909,12.));
#169945=CARTESIAN_POINT('Ctrl Pts',(67.4702032270048,29.1000300557955,0.));
#169946=CARTESIAN_POINT('Ctrl Pts',(67.4702032270048,29.1000300557955,12.));
#169947=CARTESIAN_POINT('Ctrl Pts',(67.4437091546859,29.0998456363683,0.));
#169948=CARTESIAN_POINT('Ctrl Pts',(67.4437091546859,29.0998456363683,12.));
#169949=CARTESIAN_POINT('Ctrl Pts',(67.4172524429727,29.0996369822418,0.));
#169950=CARTESIAN_POINT('Ctrl Pts',(67.4172524429727,29.0996369822418,12.));
#169951=CARTESIAN_POINT('Ctrl Pts',(67.3908331857323,29.0994041438719,0.));
#169952=CARTESIAN_POINT('Ctrl Pts',(67.3908331857323,29.0994041438719,12.));
#169953=CARTESIAN_POINT('Ctrl Pts',(67.3644514770387,29.0991471719176,0.));
#169954=CARTESIAN_POINT('Ctrl Pts',(67.3644514770387,29.0991471719176,12.));
#169955=CARTESIAN_POINT('Ctrl Pts',(67.3381074112027,29.0988661172531,0.));
#169956=CARTESIAN_POINT('Ctrl Pts',(67.3381074112027,29.0988661172531,12.));
#169957=CARTESIAN_POINT('Ctrl Pts',(67.311801082792,29.0985610309771,0.));
#169958=CARTESIAN_POINT('Ctrl Pts',(67.311801082792,29.0985610309771,12.));
#169959=CARTESIAN_POINT('Ctrl Pts',(67.2855325866517,29.0982319644277,0.));
#169960=CARTESIAN_POINT('Ctrl Pts',(67.2855325866517,29.0982319644277,12.));
#169961=CARTESIAN_POINT('Ctrl Pts',(67.2593020179209,29.0978789691962,0.));
#169962=CARTESIAN_POINT('Ctrl Pts',(67.2593020179209,29.0978789691962,12.));
#169963=CARTESIAN_POINT('Ctrl Pts',(67.2331094720471,29.097502097147,0.));
#169964=CARTESIAN_POINT('Ctrl Pts',(67.2331094720471,29.097502097147,12.));
#169965=CARTESIAN_POINT('Ctrl Pts',(67.2069550447883,29.0971014004131,0.));
#169966=CARTESIAN_POINT('Ctrl Pts',(67.2069550447883,29.0971014004131,12.));
#169967=CARTESIAN_POINT('Ctrl Pts',(67.1808388322109,29.096676931389,0.));
#169968=CARTESIAN_POINT('Ctrl Pts',(67.1808388322109,29.096676931389,12.));
#169969=CARTESIAN_POINT('Ctrl Pts',(67.1547609306843,29.0962287427273,0.));
#169970=CARTESIAN_POINT('Ctrl Pts',(67.1547609306843,29.0962287427273,12.));
#169971=CARTESIAN_POINT('Ctrl Pts',(67.1287214368746,29.0957568873358,0.));
#169972=CARTESIAN_POINT('Ctrl Pts',(67.1287214368746,29.0957568873358,12.));
#169973=CARTESIAN_POINT('Ctrl Pts',(67.1027204477311,29.0952614183779,0.));
#169974=CARTESIAN_POINT('Ctrl Pts',(67.1027204477311,29.0952614183779,12.));
#169975=CARTESIAN_POINT('Ctrl Pts',(67.0767580604879,29.0947423892727,0.));
#169976=CARTESIAN_POINT('Ctrl Pts',(67.0767580604879,29.0947423892727,12.));
#169977=CARTESIAN_POINT('Ctrl Pts',(67.0508343726776,29.0941998536959,0.));
#169978=CARTESIAN_POINT('Ctrl Pts',(67.0508343726776,29.0941998536959,12.));
#169979=CARTESIAN_POINT('Ctrl Pts',(67.0249494821363,29.0936338655828,0.));
#169980=CARTESIAN_POINT('Ctrl Pts',(67.0249494821363,29.0936338655828,12.));
#169981=CARTESIAN_POINT('Ctrl Pts',(66.9991034870083,29.0930444791328,0.));
#169982=CARTESIAN_POINT('Ctrl Pts',(66.9991034870083,29.0930444791328,12.));
#169983=CARTESIAN_POINT('Ctrl Pts',(66.9732964857466,29.092431748817,0.));
#169984=CARTESIAN_POINT('Ctrl Pts',(66.9732964857466,29.092431748817,12.));
#169985=CARTESIAN_POINT('Ctrl Pts',(66.9475285771135,29.0917957293826,0.));
#169986=CARTESIAN_POINT('Ctrl Pts',(66.9475285771135,29.0917957293826,12.));
#169987=CARTESIAN_POINT('Ctrl Pts',(66.9217998601885,29.0911364758487,0.));
#169988=CARTESIAN_POINT('Ctrl Pts',(66.9217998601885,29.0911364758487,12.));
#169989=CARTESIAN_POINT('Ctrl Pts',(66.8961104343707,29.0904540435065,0.));
#169990=CARTESIAN_POINT('Ctrl Pts',(66.8961104343707,29.0904540435065,12.));
#169991=CARTESIAN_POINT('Ctrl Pts',(66.8704603993794,29.0897484879207,0.));
#169992=CARTESIAN_POINT('Ctrl Pts',(66.8704603993794,29.0897484879207,12.));
#169993=CARTESIAN_POINT('Ctrl Pts',(66.8448498552503,29.0890198649323,0.));
#169994=CARTESIAN_POINT('Ctrl Pts',(66.8448498552503,29.0890198649323,12.));
#169995=CARTESIAN_POINT('Ctrl Pts',(66.8192789023312,29.088268230663,0.));
#169996=CARTESIAN_POINT('Ctrl Pts',(66.8192789023312,29.088268230663,12.));
#169997=CARTESIAN_POINT('Ctrl Pts',(66.793747641293,29.0874936415132,0.));
#169998=CARTESIAN_POINT('Ctrl Pts',(66.793747641293,29.0874936415132,12.));
#169999=CARTESIAN_POINT('Ctrl Pts',(66.7682561731341,29.0866961541626,0.));
#170000=CARTESIAN_POINT('Ctrl Pts',(66.7682561731341,29.0866961541626,12.));
#170001=CARTESIAN_POINT('Ctrl Pts',(66.7428045991841,29.0858758255729,0.));
#170002=CARTESIAN_POINT('Ctrl Pts',(66.7428045991841,29.0858758255729,12.));
#170003=CARTESIAN_POINT('Ctrl Pts',(66.7173930211022,29.0850327129916,0.));
#170004=CARTESIAN_POINT('Ctrl Pts',(66.7173930211022,29.0850327129916,12.));
#170005=CARTESIAN_POINT('Ctrl Pts',(66.6920215408751,29.0841668739588,0.));
#170006=CARTESIAN_POINT('Ctrl Pts',(66.6920215408751,29.0841668739588,12.));
#170007=CARTESIAN_POINT('Ctrl Pts',(66.6666902608249,29.083278366305,0.));
#170008=CARTESIAN_POINT('Ctrl Pts',(66.6666902608249,29.083278366305,12.));
#170009=CARTESIAN_POINT('Ctrl Pts',(66.6413992836147,29.0823672481507,0.));
#170010=CARTESIAN_POINT('Ctrl Pts',(66.6413992836147,29.0823672481507,12.));
#170011=CARTESIAN_POINT('Ctrl Pts',(66.6161487122502,29.0814335779084,0.));
#170012=CARTESIAN_POINT('Ctrl Pts',(66.6161487122502,29.0814335779084,12.));
#170013=CARTESIAN_POINT('Ctrl Pts',(66.59093865008,29.0804774142854,0.));
#170014=CARTESIAN_POINT('Ctrl Pts',(66.59093865008,29.0804774142854,12.));
#170015=CARTESIAN_POINT('Ctrl Pts',(66.5657692007906,29.0794988162897,0.));
#170016=CARTESIAN_POINT('Ctrl Pts',(66.5657692007906,29.0794988162897,12.));
#170017=CARTESIAN_POINT('Ctrl Pts',(66.5406404684132,29.0784978432301,0.));
#170018=CARTESIAN_POINT('Ctrl Pts',(66.5406404684132,29.0784978432301,12.));
#170019=CARTESIAN_POINT('Ctrl Pts',(66.5155525573323,29.0774745547152,0.));
#170020=CARTESIAN_POINT('Ctrl Pts',(66.5155525573323,29.0774745547152,12.));
#170021=CARTESIAN_POINT('Ctrl Pts',(66.4905055722868,29.0764290106554,0.));
#170022=CARTESIAN_POINT('Ctrl Pts',(66.4905055722868,29.0764290106554,12.));
#170023=CARTESIAN_POINT('Ctrl Pts',(66.4654996183731,29.0753612712666,0.));
#170024=CARTESIAN_POINT('Ctrl Pts',(66.4654996183731,29.0753612712666,12.));
#170025=CARTESIAN_POINT('Ctrl Pts',(66.4405348010388,29.0742713970755,0.));
#170026=CARTESIAN_POINT('Ctrl Pts',(66.4405348010388,29.0742713970755,12.));
#170027=CARTESIAN_POINT('Ctrl Pts',(66.4156112260887,29.0731594489211,0.));
#170028=CARTESIAN_POINT('Ctrl Pts',(66.4156112260887,29.0731594489211,12.));
#170029=CARTESIAN_POINT('Ctrl Pts',(66.3907289996932,29.072025487953,0.));
#170030=CARTESIAN_POINT('Ctrl Pts',(66.3907289996932,29.072025487953,12.));
#170031=CARTESIAN_POINT('Ctrl Pts',(66.3658882283903,29.0708695756334,0.));
#170032=CARTESIAN_POINT('Ctrl Pts',(66.3658882283903,29.0708695756334,12.));
#170033=CARTESIAN_POINT('Ctrl Pts',(66.3410890190884,29.0696917737399,0.));
#170034=CARTESIAN_POINT('Ctrl Pts',(66.3410890190884,29.0696917737399,12.));
#170035=CARTESIAN_POINT('Ctrl Pts',(66.3163314790615,29.0684921443721,0.));
#170036=CARTESIAN_POINT('Ctrl Pts',(66.3163314790615,29.0684921443721,12.));
#170037=CARTESIAN_POINT('Ctrl Pts',(66.2916157159536,29.067270749953,0.));
#170038=CARTESIAN_POINT('Ctrl Pts',(66.2916157159536,29.067270749953,12.));
#170039=CARTESIAN_POINT('Ctrl Pts',(66.2669418377871,29.0660276532274,0.));
#170040=CARTESIAN_POINT('Ctrl Pts',(66.2669418377871,29.0660276532274,12.));
#170041=CARTESIAN_POINT('Ctrl Pts',(66.2423099529669,29.0647629172645,0.));
#170042=CARTESIAN_POINT('Ctrl Pts',(66.2423099529669,29.0647629172645,12.));
#170043=CARTESIAN_POINT('Ctrl Pts',(66.2177201702818,29.0634766054598,0.));
#170044=CARTESIAN_POINT('Ctrl Pts',(66.2177201702818,29.0634766054598,12.));
#170045=CARTESIAN_POINT('Ctrl Pts',(66.1931725989008,29.062168781542,0.));
#170046=CARTESIAN_POINT('Ctrl Pts',(66.1931725989008,29.062168781542,12.));
#170047=CARTESIAN_POINT('Ctrl Pts',(66.1686673483757,29.0608395095747,0.));
#170048=CARTESIAN_POINT('Ctrl Pts',(66.1686673483757,29.0608395095747,12.));
#170049=CARTESIAN_POINT('Ctrl Pts',(66.144204528652,29.0594888539558,0.));
#170050=CARTESIAN_POINT('Ctrl Pts',(66.144204528652,29.0594888539558,12.));
#170051=CARTESIAN_POINT('Ctrl Pts',(66.1197842500714,29.0581168794191,0.));
#170052=CARTESIAN_POINT('Ctrl Pts',(66.1197842500714,29.0581168794191,12.));
#170053=CARTESIAN_POINT('Ctrl Pts',(66.0954066233752,29.0567236510372,0.));
#170054=CARTESIAN_POINT('Ctrl Pts',(66.0954066233752,29.0567236510372,12.));
#170055=CARTESIAN_POINT('Ctrl Pts',(66.0710717597003,29.0553092342275,0.));
#170056=CARTESIAN_POINT('Ctrl Pts',(66.0710717597003,29.0553092342275,12.));
#170057=CARTESIAN_POINT('Ctrl Pts',(66.0467797705806,29.0538736947547,0.));
#170058=CARTESIAN_POINT('Ctrl Pts',(66.0467797705806,29.0538736947547,12.));
#170059=CARTESIAN_POINT('Ctrl Pts',(66.0225307679584,29.0524170987303,0.));
#170060=CARTESIAN_POINT('Ctrl Pts',(66.0225307679584,29.0524170987303,12.));
#170061=CARTESIAN_POINT('Ctrl Pts',(65.9983248641877,29.0509395126141,0.));
#170062=CARTESIAN_POINT('Ctrl Pts',(65.9983248641877,29.0509395126141,12.));
#170063=CARTESIAN_POINT('Ctrl Pts',(65.9741621720372,29.0494410032173,0.));
#170064=CARTESIAN_POINT('Ctrl Pts',(65.9741621720372,29.0494410032173,12.));
#170065=CARTESIAN_POINT('Ctrl Pts',(65.9500428046873,29.0479216377082,0.));
#170066=CARTESIAN_POINT('Ctrl Pts',(65.9500428046873,29.0479216377082,12.));
#170067=CARTESIAN_POINT('Ctrl Pts',(65.9259668757309,29.0463814836159,0.));
#170068=CARTESIAN_POINT('Ctrl Pts',(65.9259668757309,29.0463814836159,12.));
#170069=CARTESIAN_POINT('Ctrl Pts',(65.9019344991854,29.0448206088288,0.));
#170070=CARTESIAN_POINT('Ctrl Pts',(65.9019344991854,29.0448206088288,12.));
#170071=CARTESIAN_POINT('Ctrl Pts',(65.8779457894959,29.0432390815977,0.));
#170072=CARTESIAN_POINT('Ctrl Pts',(65.8779457894959,29.0432390815977,12.));
#170073=CARTESIAN_POINT('Ctrl Pts',(65.854000861539,29.0416369705375,0.));
#170074=CARTESIAN_POINT('Ctrl Pts',(65.854000861539,29.0416369705375,12.));
#170075=CARTESIAN_POINT('Ctrl Pts',(65.8300998306198,29.0400143446341,0.));
#170076=CARTESIAN_POINT('Ctrl Pts',(65.8300998306198,29.0400143446341,12.));
#170077=CARTESIAN_POINT('Ctrl Pts',(65.8062428124723,29.0383712732473,0.));
#170078=CARTESIAN_POINT('Ctrl Pts',(65.8062428124723,29.0383712732473,12.));
#170079=CARTESIAN_POINT('Ctrl Pts',(65.7824299232715,29.0367078261107,0.));
#170080=CARTESIAN_POINT('Ctrl Pts',(65.7824299232715,29.0367078261107,12.));
#170081=CARTESIAN_POINT('Ctrl Pts',(65.7586612796375,29.0350240733333,0.));
#170082=CARTESIAN_POINT('Ctrl Pts',(65.7586612796375,29.0350240733333,12.));
#170083=CARTESIAN_POINT('Ctrl Pts',(65.7349369986382,29.0333200854026,0.));
#170084=CARTESIAN_POINT('Ctrl Pts',(65.7349369986382,29.0333200854026,12.));
#170085=CARTESIAN_POINT('Ctrl Pts',(65.7112571977874,29.0315959331911,0.));
#170086=CARTESIAN_POINT('Ctrl Pts',(65.7112571977874,29.0315959331911,12.));
#170087=CARTESIAN_POINT('Ctrl Pts',(65.6876219950465,29.0298516879599,0.));
#170088=CARTESIAN_POINT('Ctrl Pts',(65.6876219950465,29.0298516879599,12.));
#170089=CARTESIAN_POINT('Ctrl Pts',(65.664031508836,29.0280874213584,0.));
#170090=CARTESIAN_POINT('Ctrl Pts',(65.664031508836,29.0280874213584,12.));
#170091=CARTESIAN_POINT('Ctrl Pts',(65.6404858580391,29.0263032054261,0.));
#170092=CARTESIAN_POINT('Ctrl Pts',(65.6404858580391,29.0263032054261,12.));
#170093=CARTESIAN_POINT('Ctrl Pts',(65.6169851620054,29.0244991125962,0.));
#170094=CARTESIAN_POINT('Ctrl Pts',(65.6169851620054,29.0244991125962,12.));
#170095=CARTESIAN_POINT('Ctrl Pts',(65.593529540548,29.0226752157013,0.));
#170096=CARTESIAN_POINT('Ctrl Pts',(65.593529540548,29.0226752157013,12.));
#170097=CARTESIAN_POINT('Ctrl Pts',(65.5701191139455,29.0208315879778,0.));
#170098=CARTESIAN_POINT('Ctrl Pts',(65.5701191139455,29.0208315879778,12.));
#170099=CARTESIAN_POINT('Ctrl Pts',(65.5467540029546,29.0189683030654,0.));
#170100=CARTESIAN_POINT('Ctrl Pts',(65.5467540029546,29.0189683030654,12.));
#170101=CARTESIAN_POINT('Ctrl Pts',(65.523434328815,29.01708543501,0.));
#170102=CARTESIAN_POINT('Ctrl Pts',(65.523434328815,29.01708543501,12.));
#170103=CARTESIAN_POINT('Ctrl Pts',(65.5001602132524,29.015183058267,0.));
#170104=CARTESIAN_POINT('Ctrl Pts',(65.5001602132524,29.015183058267,12.));
#170105=CARTESIAN_POINT('Ctrl Pts',(65.4769317784754,29.0132612477075,0.));
#170106=CARTESIAN_POINT('Ctrl Pts',(65.4769317784754,29.0132612477075,12.));
#170107=CARTESIAN_POINT('Ctrl Pts',(65.4537491471782,29.0113200786219,0.));
#170108=CARTESIAN_POINT('Ctrl Pts',(65.4537491471782,29.0113200786219,12.));
#170109=CARTESIAN_POINT('Ctrl Pts',(65.4306124425524,29.0093596267198,0.));
#170110=CARTESIAN_POINT('Ctrl Pts',(65.4306124425524,29.0093596267198,12.));
#170111=CARTESIAN_POINT('Ctrl Pts',(65.4075217882921,29.0073799681336,0.));
#170112=CARTESIAN_POINT('Ctrl Pts',(65.4075217882921,29.0073799681336,12.));
#170113=CARTESIAN_POINT('Ctrl Pts',(65.3844773085976,29.0053811794214,0.));
#170114=CARTESIAN_POINT('Ctrl Pts',(65.3844773085976,29.0053811794214,12.));
#170115=CARTESIAN_POINT('Ctrl Pts',(65.3614791281725,29.0033633375745,0.));
#170116=CARTESIAN_POINT('Ctrl Pts',(65.3614791281725,29.0033633375745,12.));
#170117=CARTESIAN_POINT('Ctrl Pts',(65.3385273722278,29.0013265200201,0.));
#170118=CARTESIAN_POINT('Ctrl Pts',(65.3385273722278,29.0013265200201,12.));
#170119=CARTESIAN_POINT('Ctrl Pts',(65.3156221664942,28.9992708046223,0.));
#170120=CARTESIAN_POINT('Ctrl Pts',(65.3156221664942,28.9992708046223,12.));
#170121=CARTESIAN_POINT('Ctrl Pts',(65.2927636372261,28.9971962696848,0.));
#170122=CARTESIAN_POINT('Ctrl Pts',(65.2927636372261,28.9971962696848,12.));
#170123=CARTESIAN_POINT('Ctrl Pts',(65.2699519112052,28.9951029939551,0.));
#170124=CARTESIAN_POINT('Ctrl Pts',(65.2699519112052,28.9951029939551,12.));
#170125=CARTESIAN_POINT('Ctrl Pts',(65.2471871157375,28.9929910566314,0.));
#170126=CARTESIAN_POINT('Ctrl Pts',(65.2471871157375,28.9929910566314,12.));
#170127=CARTESIAN_POINT('Ctrl Pts',(65.2244693786586,28.9908605373652,0.));
#170128=CARTESIAN_POINT('Ctrl Pts',(65.2244693786586,28.9908605373652,12.));
#170129=CARTESIAN_POINT('Ctrl Pts',(65.2017988283465,28.9887115162626,0.));
#170130=CARTESIAN_POINT('Ctrl Pts',(65.2017988283465,28.9887115162626,12.));
#170131=CARTESIAN_POINT('Ctrl Pts',(65.1791755937254,28.9865440738882,0.));
#170132=CARTESIAN_POINT('Ctrl Pts',(65.1791755937254,28.9865440738882,12.));
#170133=CARTESIAN_POINT('Ctrl Pts',(65.1565998042705,28.9843582912697,0.));
#170134=CARTESIAN_POINT('Ctrl Pts',(65.1565998042705,28.9843582912697,12.));
#170135=CARTESIAN_POINT('Ctrl Pts',(65.1340715900042,28.9821542499049,0.));
#170136=CARTESIAN_POINT('Ctrl Pts',(65.1340715900042,28.9821542499049,12.));
#170137=CARTESIAN_POINT('Ctrl Pts',(65.111591081505,28.9799320317648,0.));
#170138=CARTESIAN_POINT('Ctrl Pts',(65.111591081505,28.9799320317648,12.));
#170139=CARTESIAN_POINT('Ctrl Pts',(65.0891584099174,28.9776917192936,0.));
#170140=CARTESIAN_POINT('Ctrl Pts',(65.0891584099174,28.9776917192936,12.));
#170141=CARTESIAN_POINT('Ctrl Pts',(65.0667737069562,28.9754333954134,0.));
#170142=CARTESIAN_POINT('Ctrl Pts',(65.0667737069562,28.9754333954134,12.));
#170143=CARTESIAN_POINT('Ctrl Pts',(65.0444371049082,28.9731571435281,0.));
#170144=CARTESIAN_POINT('Ctrl Pts',(65.0444371049082,28.9731571435281,12.));
#170145=CARTESIAN_POINT('Ctrl Pts',(65.0221487366279,28.9708630475298,0.));
#170146=CARTESIAN_POINT('Ctrl Pts',(65.0221487366279,28.9708630475298,12.));
#170147=CARTESIAN_POINT('Ctrl Pts',(64.9999087355504,28.9685511918017,0.));
#170148=CARTESIAN_POINT('Ctrl Pts',(64.9999087355504,28.9685511918017,12.));
#170149=CARTESIAN_POINT('Ctrl Pts',(64.9777172357028,28.9662216612216,0.));
#170150=CARTESIAN_POINT('Ctrl Pts',(64.9777172357028,28.9662216612216,12.));
#170151=CARTESIAN_POINT('Ctrl Pts',(64.955574371711,28.9638745411677,0.));
#170152=CARTESIAN_POINT('Ctrl Pts',(64.955574371711,28.9638745411677,12.));
#170153=CARTESIAN_POINT('Ctrl Pts',(64.9334802788037,28.961509917525,0.));
#170154=CARTESIAN_POINT('Ctrl Pts',(64.9334802788037,28.961509917525,12.));
#170155=CARTESIAN_POINT('Ctrl Pts',(64.9114350928124,28.9591278766934,0.));
#170156=CARTESIAN_POINT('Ctrl Pts',(64.9114350928124,28.9591278766934,12.));
#170157=CARTESIAN_POINT('Ctrl Pts',(64.8894389501799,28.9567285055866,0.));
#170158=CARTESIAN_POINT('Ctrl Pts',(64.8894389501799,28.9567285055866,12.));
#170159=CARTESIAN_POINT('Ctrl Pts',(64.8674919879646,28.9543118916327,0.));
#170160=CARTESIAN_POINT('Ctrl Pts',(64.8674919879646,28.9543118916327,12.));
#170161=CARTESIAN_POINT('Ctrl Pts',(64.8455943438423,28.9518781227765,0.));
#170162=CARTESIAN_POINT('Ctrl Pts',(64.8455943438423,28.9518781227765,12.));
#170163=CARTESIAN_POINT('Ctrl Pts',(64.8237461561024,28.9494272874833,0.));
#170164=CARTESIAN_POINT('Ctrl Pts',(64.8237461561024,28.9494272874833,12.));
#170165=CARTESIAN_POINT('Ctrl Pts',(64.8019475636454,28.9469594747436,0.));
#170166=CARTESIAN_POINT('Ctrl Pts',(64.8019475636454,28.9469594747436,12.));
#170167=CARTESIAN_POINT('Ctrl Pts',(64.7801987060097,28.9444747740815,0.));
#170168=CARTESIAN_POINT('Ctrl Pts',(64.7801987060097,28.9444747740815,12.));
#170169=CARTESIAN_POINT('Ctrl Pts',(64.7584997233889,28.9419732755659,0.));
#170170=CARTESIAN_POINT('Ctrl Pts',(64.7584997233889,28.9419732755659,12.));
#170171=CARTESIAN_POINT('Ctrl Pts',(64.7368507566461,28.9394550698201,0.));
#170172=CARTESIAN_POINT('Ctrl Pts',(64.7368507566461,28.9394550698201,12.));
#170173=CARTESIAN_POINT('Ctrl Pts',(64.715251947327,28.9369202480383,0.));
#170174=CARTESIAN_POINT('Ctrl Pts',(64.715251947327,28.9369202480383,12.));
#170175=CARTESIAN_POINT('Ctrl Pts',(64.6937034376591,28.934368901987,0.));
#170176=CARTESIAN_POINT('Ctrl Pts',(64.6937034376591,28.934368901987,12.));
#170177=CARTESIAN_POINT('Ctrl Pts',(64.6722053705389,28.9318011239905,0.));
#170178=CARTESIAN_POINT('Ctrl Pts',(64.6722053705389,28.9318011239905,12.));
#170179=CARTESIAN_POINT('Ctrl Pts',(64.6507578895155,28.9292170069219,0.));
#170180=CARTESIAN_POINT('Ctrl Pts',(64.6507578895155,28.9292170069219,12.));
#170181=CARTESIAN_POINT('Ctrl Pts',(64.6293611387753,28.9266166441956,0.));
#170182=CARTESIAN_POINT('Ctrl Pts',(64.6293611387753,28.9266166441956,12.));
#170183=CARTESIAN_POINT('Ctrl Pts',(64.6080152631065,28.9240001297553,0.));
#170184=CARTESIAN_POINT('Ctrl Pts',(64.6080152631065,28.9240001297553,12.));
#170185=CARTESIAN_POINT('Ctrl Pts',(64.5867204079452,28.9213675580996,0.));
#170186=CARTESIAN_POINT('Ctrl Pts',(64.5867204079452,28.9213675580996,12.));
#170187=CARTESIAN_POINT('Ctrl Pts',(64.5654767194487,28.9187190243231,0.));
#170188=CARTESIAN_POINT('Ctrl Pts',(64.5654767194487,28.9187190243231,12.));
#170189=CARTESIAN_POINT('Ctrl Pts',(64.544284344556,28.9160546241538,0.));
#170190=CARTESIAN_POINT('Ctrl Pts',(64.544284344556,28.9160546241538,12.));
#170191=CARTESIAN_POINT('Ctrl Pts',(64.5231434310457,28.9133744539943,0.));
#170192=CARTESIAN_POINT('Ctrl Pts',(64.5231434310457,28.9133744539943,12.));
#170193=CARTESIAN_POINT('Ctrl Pts',(64.5020541275927,28.9106786109639,0.));
#170194=CARTESIAN_POINT('Ctrl Pts',(64.5020541275927,28.9106786109639,12.));
#170195=CARTESIAN_POINT('Ctrl Pts',(64.4810165836568,28.9079671928253,0.));
#170196=CARTESIAN_POINT('Ctrl Pts',(64.4810165836568,28.9079671928253,12.));
#170197=CARTESIAN_POINT('Ctrl Pts',(64.460030949357,28.9052402979055,0.));
#170198=CARTESIAN_POINT('Ctrl Pts',(64.460030949357,28.9052402979055,12.));
#170199=CARTESIAN_POINT('Ctrl Pts',(64.439097375364,28.9024980250309,0.));
#170200=CARTESIAN_POINT('Ctrl Pts',(64.439097375364,28.9024980250309,12.));
#170201=CARTESIAN_POINT('Ctrl Pts',(64.41821601274,28.899740473435,0.));
#170202=CARTESIAN_POINT('Ctrl Pts',(64.41821601274,28.899740473435,12.));
#170203=CARTESIAN_POINT('Ctrl Pts',(64.3973870129201,28.8969677427519,0.));
#170204=CARTESIAN_POINT('Ctrl Pts',(64.3973870129201,28.8969677427519,12.));
#170205=CARTESIAN_POINT('Ctrl Pts',(64.3766105280715,28.8941799332312,0.));
#170206=CARTESIAN_POINT('Ctrl Pts',(64.3766105280715,28.8941799332312,12.));
#170207=CARTESIAN_POINT('Ctrl Pts',(64.3558867114087,28.8913771459327,0.));
#170208=CARTESIAN_POINT('Ctrl Pts',(64.3558867114087,28.8913771459327,12.));
#170209=CARTESIAN_POINT('Ctrl Pts',(64.3352157174606,28.888559482892,0.));
#170210=CARTESIAN_POINT('Ctrl Pts',(64.3352157174606,28.888559482892,12.));
#170211=CARTESIAN_POINT('Ctrl Pts',(64.3145977025005,28.8857270473944,0.));
#170212=CARTESIAN_POINT('Ctrl Pts',(64.3145977025005,28.8857270473944,12.));
#170213=CARTESIAN_POINT('Ctrl Pts',(64.2940328242482,28.8828799437922,0.));
#170214=CARTESIAN_POINT('Ctrl Pts',(64.2940328242482,28.8828799437922,12.));
#170215=CARTESIAN_POINT('Ctrl Pts',(64.2735212410682,28.8800182770052,0.));
#170216=CARTESIAN_POINT('Ctrl Pts',(64.2735212410682,28.8800182770052,12.));
#170217=CARTESIAN_POINT('Ctrl Pts',(64.2530631112926,28.8771421521058,0.));
#170218=CARTESIAN_POINT('Ctrl Pts',(64.2530631112926,28.8771421521058,12.));
#170219=CARTESIAN_POINT('Ctrl Pts',(64.232658592528,28.8742516738959,0.));
#170220=CARTESIAN_POINT('Ctrl Pts',(64.232658592528,28.8742516738959,12.));
#170221=CARTESIAN_POINT('Ctrl Pts',(64.2123078408507,28.8713469464205,0.));
#170222=CARTESIAN_POINT('Ctrl Pts',(64.2123078408507,28.8713469464205,12.));
#170223=CARTESIAN_POINT('Ctrl Pts',(64.1920110123342,28.8684280739033,0.));
#170224=CARTESIAN_POINT('Ctrl Pts',(64.1920110123342,28.8684280739033,12.));
#170225=CARTESIAN_POINT('Ctrl Pts',(64.1717682648708,28.8654951618659,0.));
#170226=CARTESIAN_POINT('Ctrl Pts',(64.1717682648708,28.8654951618659,12.));
#170227=CARTESIAN_POINT('Ctrl Pts',(64.1515797596555,28.8625483180433,0.));
#170228=CARTESIAN_POINT('Ctrl Pts',(64.1515797596555,28.8625483180433,12.));
#170229=CARTESIAN_POINT('Ctrl Pts',(64.1314456633345,28.8595876537132,0.));
#170230=CARTESIAN_POINT('Ctrl Pts',(64.1314456633345,28.8595876537132,12.));
#170231=CARTESIAN_POINT('Ctrl Pts',(64.1113661481918,28.8566132838157,0.));
#170232=CARTESIAN_POINT('Ctrl Pts',(64.1113661481918,28.8566132838157,12.));
#170233=CARTESIAN_POINT('Ctrl Pts',(64.0913413876586,28.8536253241837,0.));
#170234=CARTESIAN_POINT('Ctrl Pts',(64.0913413876586,28.8536253241837,12.));
#170235=CARTESIAN_POINT('Ctrl Pts',(64.0713715523588,28.8506238891087,0.));
#170236=CARTESIAN_POINT('Ctrl Pts',(64.0713715523588,28.8506238891087,12.));
#170237=CARTESIAN_POINT('Ctrl Pts',(64.0514568066659,28.8476090892242,0.));
#170238=CARTESIAN_POINT('Ctrl Pts',(64.0514568066659,28.8476090892242,12.));
#170239=CARTESIAN_POINT('Ctrl Pts',(64.0315973031994,28.8445810281275,0.));
#170240=CARTESIAN_POINT('Ctrl Pts',(64.0315973031994,28.8445810281275,12.));
#170241=CARTESIAN_POINT('Ctrl Pts',(64.0117931881364,28.841539805646,0.));
#170242=CARTESIAN_POINT('Ctrl Pts',(64.0117931881364,28.841539805646,12.));
#170243=CARTESIAN_POINT('Ctrl Pts',(63.9920446117632,28.8384855243267,0.));
#170244=CARTESIAN_POINT('Ctrl Pts',(63.9920446117632,28.8384855243267,12.));
#170245=CARTESIAN_POINT('Ctrl Pts',(63.9723517369614,28.8354182946601,0.));
#170246=CARTESIAN_POINT('Ctrl Pts',(63.9723517369614,28.8354182946601,12.));
#170247=CARTESIAN_POINT('Ctrl Pts',(63.9527147494351,28.8323382413753,0.));
#170248=CARTESIAN_POINT('Ctrl Pts',(63.9527147494351,28.8323382413753,12.));
#170249=CARTESIAN_POINT('Ctrl Pts',(63.9331338646868,28.8292455077494,0.));
#170250=CARTESIAN_POINT('Ctrl Pts',(63.9331338646868,28.8292455077494,12.));
#170251=CARTESIAN_POINT('Ctrl Pts',(63.9136093063647,28.826140242322,0.));
#170252=CARTESIAN_POINT('Ctrl Pts',(63.9136093063647,28.826140242322,12.));
#170253=CARTESIAN_POINT('Ctrl Pts',(63.894141285685,28.8230225863142,0.));
#170254=CARTESIAN_POINT('Ctrl Pts',(63.894141285685,28.8230225863142,12.));
#170255=CARTESIAN_POINT('Ctrl Pts',(63.8747299825383,28.8198926619893,0.));
#170256=CARTESIAN_POINT('Ctrl Pts',(63.8747299825383,28.8198926619893,12.));
#170257=CARTESIAN_POINT('Ctrl Pts',(63.8553755207732,28.8167505576806,0.));
#170258=CARTESIAN_POINT('Ctrl Pts',(63.8553755207732,28.8167505576806,12.));
#170259=CARTESIAN_POINT('Ctrl Pts',(63.8360779670225,28.8135963263557,0.));
#170260=CARTESIAN_POINT('Ctrl Pts',(63.8360779670225,28.8135963263557,12.));
#170261=CARTESIAN_POINT('Ctrl Pts',(63.8206854735372,28.8110632621133,0.));
#170262=CARTESIAN_POINT('Ctrl Pts',(63.8206854735372,28.8110632621133,12.));
#170263=CARTESIAN_POINT('Ctrl Pts',(63.809166727145,28.8091580239664,0.));
#170264=CARTESIAN_POINT('Ctrl Pts',(63.809166727145,28.8091580239664,12.));
#170265=CARTESIAN_POINT('Ctrl Pts',(63.8014989507575,28.8078854475473,0.));
#170266=CARTESIAN_POINT('Ctrl Pts',(63.8014989507575,28.8078854475473,12.));
#170267=CARTESIAN_POINT('Ctrl Pts',(63.7976679095314,28.8072485549236,0.));
#170268=CARTESIAN_POINT('Ctrl Pts',(63.7976679095314,28.8072485549236,12.));
#170269=CARTESIAN_POINT('',(63.7976679095314,28.8072485549236,12.));
#170270=CARTESIAN_POINT('Ctrl Pts',(63.7976679095314,28.8072485549236,12.));
#170271=CARTESIAN_POINT('Ctrl Pts',(63.8014989507575,28.8078854475473,12.));
#170272=CARTESIAN_POINT('Ctrl Pts',(63.809166727145,28.8091580239664,12.));
#170273=CARTESIAN_POINT('Ctrl Pts',(63.8206854735372,28.8110632621133,12.));
#170274=CARTESIAN_POINT('Ctrl Pts',(63.8360779670225,28.8135963263557,12.));
#170275=CARTESIAN_POINT('Ctrl Pts',(63.8553755207732,28.8167505576806,12.));
#170276=CARTESIAN_POINT('Ctrl Pts',(63.8747299825383,28.8198926619893,12.));
#170277=CARTESIAN_POINT('Ctrl Pts',(63.894141285685,28.8230225863142,12.));
#170278=CARTESIAN_POINT('Ctrl Pts',(63.9136093063647,28.826140242322,12.));
#170279=CARTESIAN_POINT('Ctrl Pts',(63.9331338646868,28.8292455077494,12.));
#170280=CARTESIAN_POINT('Ctrl Pts',(63.9527147494351,28.8323382413753,12.));
#170281=CARTESIAN_POINT('Ctrl Pts',(63.9723517369614,28.8354182946601,12.));
#170282=CARTESIAN_POINT('Ctrl Pts',(63.9920446117632,28.8384855243267,12.));
#170283=CARTESIAN_POINT('Ctrl Pts',(64.0117931881364,28.841539805646,12.));
#170284=CARTESIAN_POINT('Ctrl Pts',(64.0315973031994,28.8445810281275,12.));
#170285=CARTESIAN_POINT('Ctrl Pts',(64.0514568066659,28.8476090892242,12.));
#170286=CARTESIAN_POINT('Ctrl Pts',(64.0713715523588,28.8506238891087,12.));
#170287=CARTESIAN_POINT('Ctrl Pts',(64.0913413876586,28.8536253241837,12.));
#170288=CARTESIAN_POINT('Ctrl Pts',(64.1113661481918,28.8566132838157,12.));
#170289=CARTESIAN_POINT('Ctrl Pts',(64.1314456633345,28.8595876537132,12.));
#170290=CARTESIAN_POINT('Ctrl Pts',(64.1515797596555,28.8625483180433,12.));
#170291=CARTESIAN_POINT('Ctrl Pts',(64.1717682648708,28.8654951618659,12.));
#170292=CARTESIAN_POINT('Ctrl Pts',(64.1920110123342,28.8684280739033,12.));
#170293=CARTESIAN_POINT('Ctrl Pts',(64.2123078408507,28.8713469464205,12.));
#170294=CARTESIAN_POINT('Ctrl Pts',(64.232658592528,28.8742516738959,12.));
#170295=CARTESIAN_POINT('Ctrl Pts',(64.2530631112926,28.8771421521058,12.));
#170296=CARTESIAN_POINT('Ctrl Pts',(64.2735212410682,28.8800182770052,12.));
#170297=CARTESIAN_POINT('Ctrl Pts',(64.2940328242482,28.8828799437922,12.));
#170298=CARTESIAN_POINT('Ctrl Pts',(64.3145977025005,28.8857270473944,12.));
#170299=CARTESIAN_POINT('Ctrl Pts',(64.3352157174606,28.888559482892,12.));
#170300=CARTESIAN_POINT('Ctrl Pts',(64.3558867114087,28.8913771459327,12.));
#170301=CARTESIAN_POINT('Ctrl Pts',(64.3766105280715,28.8941799332312,12.));
#170302=CARTESIAN_POINT('Ctrl Pts',(64.3973870129201,28.8969677427519,12.));
#170303=CARTESIAN_POINT('Ctrl Pts',(64.41821601274,28.899740473435,12.));
#170304=CARTESIAN_POINT('Ctrl Pts',(64.439097375364,28.9024980250309,12.));
#170305=CARTESIAN_POINT('Ctrl Pts',(64.460030949357,28.9052402979055,12.));
#170306=CARTESIAN_POINT('Ctrl Pts',(64.4810165836568,28.9079671928253,12.));
#170307=CARTESIAN_POINT('Ctrl Pts',(64.5020541275927,28.9106786109639,12.));
#170308=CARTESIAN_POINT('Ctrl Pts',(64.5231434310457,28.9133744539943,12.));
#170309=CARTESIAN_POINT('Ctrl Pts',(64.544284344556,28.9160546241538,12.));
#170310=CARTESIAN_POINT('Ctrl Pts',(64.5654767194487,28.9187190243231,12.));
#170311=CARTESIAN_POINT('Ctrl Pts',(64.5867204079452,28.9213675580996,12.));
#170312=CARTESIAN_POINT('Ctrl Pts',(64.6080152631065,28.9240001297553,12.));
#170313=CARTESIAN_POINT('Ctrl Pts',(64.6293611387753,28.9266166441956,12.));
#170314=CARTESIAN_POINT('Ctrl Pts',(64.6507578895155,28.9292170069219,12.));
#170315=CARTESIAN_POINT('Ctrl Pts',(64.6722053705389,28.9318011239905,12.));
#170316=CARTESIAN_POINT('Ctrl Pts',(64.6937034376591,28.934368901987,12.));
#170317=CARTESIAN_POINT('Ctrl Pts',(64.715251947327,28.9369202480383,12.));
#170318=CARTESIAN_POINT('Ctrl Pts',(64.7368507566461,28.9394550698201,12.));
#170319=CARTESIAN_POINT('Ctrl Pts',(64.7584997233889,28.9419732755659,12.));
#170320=CARTESIAN_POINT('Ctrl Pts',(64.7801987060097,28.9444747740815,12.));
#170321=CARTESIAN_POINT('Ctrl Pts',(64.8019475636454,28.9469594747436,12.));
#170322=CARTESIAN_POINT('Ctrl Pts',(64.8237461561024,28.9494272874833,12.));
#170323=CARTESIAN_POINT('Ctrl Pts',(64.8455943438423,28.9518781227765,12.));
#170324=CARTESIAN_POINT('Ctrl Pts',(64.8674919879646,28.9543118916327,12.));
#170325=CARTESIAN_POINT('Ctrl Pts',(64.8894389501799,28.9567285055866,12.));
#170326=CARTESIAN_POINT('Ctrl Pts',(64.9114350928124,28.9591278766934,12.));
#170327=CARTESIAN_POINT('Ctrl Pts',(64.9334802788037,28.961509917525,12.));
#170328=CARTESIAN_POINT('Ctrl Pts',(64.955574371711,28.9638745411677,12.));
#170329=CARTESIAN_POINT('Ctrl Pts',(64.9777172357028,28.9662216612216,12.));
#170330=CARTESIAN_POINT('Ctrl Pts',(64.9999087355504,28.9685511918017,12.));
#170331=CARTESIAN_POINT('Ctrl Pts',(65.0221487366279,28.9708630475298,12.));
#170332=CARTESIAN_POINT('Ctrl Pts',(65.0444371049082,28.9731571435281,12.));
#170333=CARTESIAN_POINT('Ctrl Pts',(65.0667737069562,28.9754333954134,12.));
#170334=CARTESIAN_POINT('Ctrl Pts',(65.0891584099174,28.9776917192936,12.));
#170335=CARTESIAN_POINT('Ctrl Pts',(65.111591081505,28.9799320317648,12.));
#170336=CARTESIAN_POINT('Ctrl Pts',(65.1340715900042,28.9821542499049,12.));
#170337=CARTESIAN_POINT('Ctrl Pts',(65.1565998042705,28.9843582912697,12.));
#170338=CARTESIAN_POINT('Ctrl Pts',(65.1791755937254,28.9865440738882,12.));
#170339=CARTESIAN_POINT('Ctrl Pts',(65.2017988283465,28.9887115162626,12.));
#170340=CARTESIAN_POINT('Ctrl Pts',(65.2244693786586,28.9908605373652,12.));
#170341=CARTESIAN_POINT('Ctrl Pts',(65.2471871157375,28.9929910566314,12.));
#170342=CARTESIAN_POINT('Ctrl Pts',(65.2699519112052,28.9951029939551,12.));
#170343=CARTESIAN_POINT('Ctrl Pts',(65.2927636372261,28.9971962696848,12.));
#170344=CARTESIAN_POINT('Ctrl Pts',(65.3156221664942,28.9992708046223,12.));
#170345=CARTESIAN_POINT('Ctrl Pts',(65.3385273722278,29.0013265200201,12.));
#170346=CARTESIAN_POINT('Ctrl Pts',(65.3614791281725,29.0033633375745,12.));
#170347=CARTESIAN_POINT('Ctrl Pts',(65.3844773085976,29.0053811794214,12.));
#170348=CARTESIAN_POINT('Ctrl Pts',(65.4075217882921,29.0073799681336,12.));
#170349=CARTESIAN_POINT('Ctrl Pts',(65.4306124425524,29.0093596267198,12.));
#170350=CARTESIAN_POINT('Ctrl Pts',(65.4537491471782,29.0113200786219,12.));
#170351=CARTESIAN_POINT('Ctrl Pts',(65.4769317784754,29.0132612477075,12.));
#170352=CARTESIAN_POINT('Ctrl Pts',(65.5001602132524,29.015183058267,12.));
#170353=CARTESIAN_POINT('Ctrl Pts',(65.523434328815,29.01708543501,12.));
#170354=CARTESIAN_POINT('Ctrl Pts',(65.5467540029546,29.0189683030654,12.));
#170355=CARTESIAN_POINT('Ctrl Pts',(65.5701191139455,29.0208315879778,12.));
#170356=CARTESIAN_POINT('Ctrl Pts',(65.593529540548,29.0226752157013,12.));
#170357=CARTESIAN_POINT('Ctrl Pts',(65.6169851620054,29.0244991125962,12.));
#170358=CARTESIAN_POINT('Ctrl Pts',(65.6404858580391,29.0263032054261,12.));
#170359=CARTESIAN_POINT('Ctrl Pts',(65.664031508836,29.0280874213584,12.));
#170360=CARTESIAN_POINT('Ctrl Pts',(65.6876219950465,29.0298516879599,12.));
#170361=CARTESIAN_POINT('Ctrl Pts',(65.7112571977874,29.0315959331911,12.));
#170362=CARTESIAN_POINT('Ctrl Pts',(65.7349369986382,29.0333200854026,12.));
#170363=CARTESIAN_POINT('Ctrl Pts',(65.7586612796375,29.0350240733333,12.));
#170364=CARTESIAN_POINT('Ctrl Pts',(65.7824299232715,29.0367078261107,12.));
#170365=CARTESIAN_POINT('Ctrl Pts',(65.8062428124723,29.0383712732473,12.));
#170366=CARTESIAN_POINT('Ctrl Pts',(65.8300998306198,29.0400143446341,12.));
#170367=CARTESIAN_POINT('Ctrl Pts',(65.854000861539,29.0416369705375,12.));
#170368=CARTESIAN_POINT('Ctrl Pts',(65.8779457894959,29.0432390815977,12.));
#170369=CARTESIAN_POINT('Ctrl Pts',(65.9019344991854,29.0448206088288,12.));
#170370=CARTESIAN_POINT('Ctrl Pts',(65.9259668757309,29.0463814836159,12.));
#170371=CARTESIAN_POINT('Ctrl Pts',(65.9500428046873,29.0479216377082,12.));
#170372=CARTESIAN_POINT('Ctrl Pts',(65.9741621720372,29.0494410032173,12.));
#170373=CARTESIAN_POINT('Ctrl Pts',(65.9983248641877,29.0509395126141,12.));
#170374=CARTESIAN_POINT('Ctrl Pts',(66.0225307679584,29.0524170987303,12.));
#170375=CARTESIAN_POINT('Ctrl Pts',(66.0467797705806,29.0538736947547,12.));
#170376=CARTESIAN_POINT('Ctrl Pts',(66.0710717597003,29.0553092342275,12.));
#170377=CARTESIAN_POINT('Ctrl Pts',(66.0954066233752,29.0567236510372,12.));
#170378=CARTESIAN_POINT('Ctrl Pts',(66.1197842500714,29.0581168794191,12.));
#170379=CARTESIAN_POINT('Ctrl Pts',(66.144204528652,29.0594888539558,12.));
#170380=CARTESIAN_POINT('Ctrl Pts',(66.1686673483757,29.0608395095747,12.));
#170381=CARTESIAN_POINT('Ctrl Pts',(66.1931725989008,29.062168781542,12.));
#170382=CARTESIAN_POINT('Ctrl Pts',(66.2177201702818,29.0634766054598,12.));
#170383=CARTESIAN_POINT('Ctrl Pts',(66.2423099529669,29.0647629172645,12.));
#170384=CARTESIAN_POINT('Ctrl Pts',(66.2669418377871,29.0660276532274,12.));
#170385=CARTESIAN_POINT('Ctrl Pts',(66.2916157159536,29.067270749953,12.));
#170386=CARTESIAN_POINT('Ctrl Pts',(66.3163314790615,29.0684921443721,12.));
#170387=CARTESIAN_POINT('Ctrl Pts',(66.3410890190884,29.0696917737399,12.));
#170388=CARTESIAN_POINT('Ctrl Pts',(66.3658882283903,29.0708695756334,12.));
#170389=CARTESIAN_POINT('Ctrl Pts',(66.3907289996932,29.072025487953,12.));
#170390=CARTESIAN_POINT('Ctrl Pts',(66.4156112260887,29.0731594489211,12.));
#170391=CARTESIAN_POINT('Ctrl Pts',(66.4405348010388,29.0742713970755,12.));
#170392=CARTESIAN_POINT('Ctrl Pts',(66.4654996183731,29.0753612712666,12.));
#170393=CARTESIAN_POINT('Ctrl Pts',(66.4905055722868,29.0764290106554,12.));
#170394=CARTESIAN_POINT('Ctrl Pts',(66.5155525573323,29.0774745547152,12.));
#170395=CARTESIAN_POINT('Ctrl Pts',(66.5406404684132,29.0784978432301,12.));
#170396=CARTESIAN_POINT('Ctrl Pts',(66.5657692007906,29.0794988162897,12.));
#170397=CARTESIAN_POINT('Ctrl Pts',(66.59093865008,29.0804774142854,12.));
#170398=CARTESIAN_POINT('Ctrl Pts',(66.6161487122502,29.0814335779084,12.));
#170399=CARTESIAN_POINT('Ctrl Pts',(66.6413992836147,29.0823672481507,12.));
#170400=CARTESIAN_POINT('Ctrl Pts',(66.6666902608249,29.083278366305,12.));
#170401=CARTESIAN_POINT('Ctrl Pts',(66.6920215408751,29.0841668739588,12.));
#170402=CARTESIAN_POINT('Ctrl Pts',(66.7173930211022,29.0850327129916,12.));
#170403=CARTESIAN_POINT('Ctrl Pts',(66.7428045991841,29.0858758255729,12.));
#170404=CARTESIAN_POINT('Ctrl Pts',(66.7682561731341,29.0866961541626,12.));
#170405=CARTESIAN_POINT('Ctrl Pts',(66.793747641293,29.0874936415132,12.));
#170406=CARTESIAN_POINT('Ctrl Pts',(66.8192789023312,29.088268230663,12.));
#170407=CARTESIAN_POINT('Ctrl Pts',(66.8448498552503,29.0890198649323,12.));
#170408=CARTESIAN_POINT('Ctrl Pts',(66.8704603993794,29.0897484879207,12.));
#170409=CARTESIAN_POINT('Ctrl Pts',(66.8961104343707,29.0904540435065,12.));
#170410=CARTESIAN_POINT('Ctrl Pts',(66.9217998601885,29.0911364758487,12.));
#170411=CARTESIAN_POINT('Ctrl Pts',(66.9475285771135,29.0917957293826,12.));
#170412=CARTESIAN_POINT('Ctrl Pts',(66.9732964857466,29.092431748817,12.));
#170413=CARTESIAN_POINT('Ctrl Pts',(66.9991034870083,29.0930444791328,12.));
#170414=CARTESIAN_POINT('Ctrl Pts',(67.0249494821363,29.0936338655828,12.));
#170415=CARTESIAN_POINT('Ctrl Pts',(67.0508343726776,29.0941998536959,12.));
#170416=CARTESIAN_POINT('Ctrl Pts',(67.0767580604879,29.0947423892727,12.));
#170417=CARTESIAN_POINT('Ctrl Pts',(67.1027204477311,29.0952614183779,12.));
#170418=CARTESIAN_POINT('Ctrl Pts',(67.1287214368746,29.0957568873358,12.));
#170419=CARTESIAN_POINT('Ctrl Pts',(67.1547609306843,29.0962287427273,12.));
#170420=CARTESIAN_POINT('Ctrl Pts',(67.1808388322109,29.096676931389,12.));
#170421=CARTESIAN_POINT('Ctrl Pts',(67.2069550447883,29.0971014004131,12.));
#170422=CARTESIAN_POINT('Ctrl Pts',(67.2331094720471,29.097502097147,12.));
#170423=CARTESIAN_POINT('Ctrl Pts',(67.2593020179209,29.0978789691962,12.));
#170424=CARTESIAN_POINT('Ctrl Pts',(67.2855325866517,29.0982319644277,12.));
#170425=CARTESIAN_POINT('Ctrl Pts',(67.311801082792,29.0985610309771,12.));
#170426=CARTESIAN_POINT('Ctrl Pts',(67.3381074112027,29.0988661172531,12.));
#170427=CARTESIAN_POINT('Ctrl Pts',(67.3644514770387,29.0991471719176,12.));
#170428=CARTESIAN_POINT('Ctrl Pts',(67.3908331857323,29.0994041438719,12.));
#170429=CARTESIAN_POINT('Ctrl Pts',(67.4172524429727,29.0996369822418,12.));
#170430=CARTESIAN_POINT('Ctrl Pts',(67.4437091546859,29.0998456363683,12.));
#170431=CARTESIAN_POINT('Ctrl Pts',(67.4702032270048,29.1000300557955,12.));
#170432=CARTESIAN_POINT('Ctrl Pts',(67.4967345663096,29.1001901902909,12.));
#170433=CARTESIAN_POINT('Ctrl Pts',(67.5233030792704,29.1003259898682,12.));
#170434=CARTESIAN_POINT('Ctrl Pts',(67.5499086728888,29.1004374048148,12.));
#170435=CARTESIAN_POINT('Ctrl Pts',(67.5765512545281,29.1005243857139,12.));
#170436=CARTESIAN_POINT('Ctrl Pts',(67.6032307319623,29.1005868834866,12.));
#170437=CARTESIAN_POINT('Ctrl Pts',(67.6299470133295,29.100624849358,12.));
#170438=CARTESIAN_POINT('Ctrl Pts',(67.6567000070326,29.1006382347814,12.));
#170439=CARTESIAN_POINT('Ctrl Pts',(67.6834896216461,29.1006269913747,12.));
#170440=CARTESIAN_POINT('Ctrl Pts',(67.7103157658296,29.1005910708624,12.));
#170441=CARTESIAN_POINT('Ctrl Pts',(67.7371783482035,29.1005304249987,12.));
#170442=CARTESIAN_POINT('Ctrl Pts',(67.7640772773387,29.1004450055643,12.));
#170443=CARTESIAN_POINT('Ctrl Pts',(67.7910124620135,29.1003347645294,12.));
#170444=CARTESIAN_POINT('Ctrl Pts',(67.8179838114099,29.1001996541842,12.));
#170445=CARTESIAN_POINT('Ctrl Pts',(67.8449912353329,29.1000396272867,12.));
#170446=CARTESIAN_POINT('Ctrl Pts',(67.8720346444124,29.0998546372032,12.));
#170447=CARTESIAN_POINT('Ctrl Pts',(67.8991139503193,29.0996446380626,12.));
#170448=CARTESIAN_POINT('Ctrl Pts',(67.9262290652829,29.099409584422,12.));
#170449=CARTESIAN_POINT('Ctrl Pts',(67.9533799016148,29.0991494309404,12.));
#170450=CARTESIAN_POINT('Ctrl Pts',(67.9805663711855,29.0988641320247,12.));
#170451=CARTESIAN_POINT('Ctrl Pts',(68.0077883850121,29.0985536415531,12.));
#170452=CARTESIAN_POINT('Ctrl Pts',(68.0350458525551,29.0982179124097,12.));
#170453=CARTESIAN_POINT('Ctrl Pts',(68.0623386822863,29.0978568968657,12.));
#170454=CARTESIAN_POINT('Ctrl Pts',(68.0896667829567,29.0974705474259,12.));
#170455=CARTESIAN_POINT('Ctrl Pts',(68.1170300646987,29.0970588175728,12.));
#170456=CARTESIAN_POINT('Ctrl Pts',(68.1444284400742,29.0966216624743,12.));
#170457=CARTESIAN_POINT('Ctrl Pts',(68.1718618254281,29.0961590399046,12.));
#170458=CARTESIAN_POINT('Ctrl Pts',(68.1993301412061,29.0956709104627,12.));
#170459=CARTESIAN_POINT('Ctrl Pts',(68.2229056854683,29.095230591515,12.));
#170460=CARTESIAN_POINT('Ctrl Pts',(68.2409993690197,29.094879194787,12.));
#170461=CARTESIAN_POINT('Ctrl Pts',(68.2535957747187,29.0946280433337,12.));
#170462=CARTESIAN_POINT('Ctrl Pts',(68.2606847334987,29.0944846386568,12.));
#170463=CARTESIAN_POINT('Ctrl Pts',(68.2622612910177,29.0944526440266,12.));
#170464=CARTESIAN_POINT('',(63.7976679095314,28.8072485549236,0.));
#170465=CARTESIAN_POINT('',(63.7976679095314,28.8072485549236,0.));
#170466=CARTESIAN_POINT('Ctrl Pts',(68.2622612910177,29.0944526440266,0.));
#170467=CARTESIAN_POINT('Ctrl Pts',(68.2606847334987,29.0944846386568,0.));
#170468=CARTESIAN_POINT('Ctrl Pts',(68.2535957747187,29.0946280433337,0.));
#170469=CARTESIAN_POINT('Ctrl Pts',(68.2409993690197,29.094879194787,0.));
#170470=CARTESIAN_POINT('Ctrl Pts',(68.2229056854683,29.095230591515,0.));
#170471=CARTESIAN_POINT('Ctrl Pts',(68.1993301412061,29.0956709104627,0.));
#170472=CARTESIAN_POINT('Ctrl Pts',(68.1718618254281,29.0961590399046,0.));
#170473=CARTESIAN_POINT('Ctrl Pts',(68.1444284400742,29.0966216624743,0.));
#170474=CARTESIAN_POINT('Ctrl Pts',(68.1170300646987,29.0970588175728,0.));
#170475=CARTESIAN_POINT('Ctrl Pts',(68.0896667829567,29.0974705474259,0.));
#170476=CARTESIAN_POINT('Ctrl Pts',(68.0623386822863,29.0978568968657,0.));
#170477=CARTESIAN_POINT('Ctrl Pts',(68.0350458525551,29.0982179124097,0.));
#170478=CARTESIAN_POINT('Ctrl Pts',(68.0077883850121,29.0985536415531,0.));
#170479=CARTESIAN_POINT('Ctrl Pts',(67.9805663711855,29.0988641320247,0.));
#170480=CARTESIAN_POINT('Ctrl Pts',(67.9533799016148,29.0991494309404,0.));
#170481=CARTESIAN_POINT('Ctrl Pts',(67.9262290652829,29.099409584422,0.));
#170482=CARTESIAN_POINT('Ctrl Pts',(67.8991139503193,29.0996446380626,0.));
#170483=CARTESIAN_POINT('Ctrl Pts',(67.8720346444124,29.0998546372032,0.));
#170484=CARTESIAN_POINT('Ctrl Pts',(67.8449912353329,29.1000396272867,0.));
#170485=CARTESIAN_POINT('Ctrl Pts',(67.8179838114099,29.1001996541842,0.));
#170486=CARTESIAN_POINT('Ctrl Pts',(67.7910124620135,29.1003347645294,0.));
#170487=CARTESIAN_POINT('Ctrl Pts',(67.7640772773387,29.1004450055643,0.));
#170488=CARTESIAN_POINT('Ctrl Pts',(67.7371783482035,29.1005304249987,0.));
#170489=CARTESIAN_POINT('Ctrl Pts',(67.7103157658296,29.1005910708624,0.));
#170490=CARTESIAN_POINT('Ctrl Pts',(67.6834896216461,29.1006269913747,0.));
#170491=CARTESIAN_POINT('Ctrl Pts',(67.6567000070326,29.1006382347814,0.));
#170492=CARTESIAN_POINT('Ctrl Pts',(67.6299470133295,29.100624849358,0.));
#170493=CARTESIAN_POINT('Ctrl Pts',(67.6032307319623,29.1005868834866,0.));
#170494=CARTESIAN_POINT('Ctrl Pts',(67.5765512545281,29.1005243857139,0.));
#170495=CARTESIAN_POINT('Ctrl Pts',(67.5499086728888,29.1004374048148,0.));
#170496=CARTESIAN_POINT('Ctrl Pts',(67.5233030792704,29.1003259898682,0.));
#170497=CARTESIAN_POINT('Ctrl Pts',(67.4967345663096,29.1001901902909,0.));
#170498=CARTESIAN_POINT('Ctrl Pts',(67.4702032270048,29.1000300557955,0.));
#170499=CARTESIAN_POINT('Ctrl Pts',(67.4437091546859,29.0998456363683,0.));
#170500=CARTESIAN_POINT('Ctrl Pts',(67.4172524429727,29.0996369822418,0.));
#170501=CARTESIAN_POINT('Ctrl Pts',(67.3908331857323,29.0994041438719,0.));
#170502=CARTESIAN_POINT('Ctrl Pts',(67.3644514770387,29.0991471719176,0.));
#170503=CARTESIAN_POINT('Ctrl Pts',(67.3381074112027,29.0988661172531,0.));
#170504=CARTESIAN_POINT('Ctrl Pts',(67.311801082792,29.0985610309771,0.));
#170505=CARTESIAN_POINT('Ctrl Pts',(67.2855325866517,29.0982319644277,0.));
#170506=CARTESIAN_POINT('Ctrl Pts',(67.2593020179209,29.0978789691962,0.));
#170507=CARTESIAN_POINT('Ctrl Pts',(67.2331094720471,29.097502097147,0.));
#170508=CARTESIAN_POINT('Ctrl Pts',(67.2069550447883,29.0971014004131,0.));
#170509=CARTESIAN_POINT('Ctrl Pts',(67.1808388322109,29.096676931389,0.));
#170510=CARTESIAN_POINT('Ctrl Pts',(67.1547609306843,29.0962287427273,0.));
#170511=CARTESIAN_POINT('Ctrl Pts',(67.1287214368746,29.0957568873358,0.));
#170512=CARTESIAN_POINT('Ctrl Pts',(67.1027204477311,29.0952614183779,0.));
#170513=CARTESIAN_POINT('Ctrl Pts',(67.0767580604879,29.0947423892727,0.));
#170514=CARTESIAN_POINT('Ctrl Pts',(67.0508343726776,29.0941998536959,0.));
#170515=CARTESIAN_POINT('Ctrl Pts',(67.0249494821363,29.0936338655828,0.));
#170516=CARTESIAN_POINT('Ctrl Pts',(66.9991034870083,29.0930444791328,0.));
#170517=CARTESIAN_POINT('Ctrl Pts',(66.9732964857466,29.092431748817,0.));
#170518=CARTESIAN_POINT('Ctrl Pts',(66.9475285771135,29.0917957293826,0.));
#170519=CARTESIAN_POINT('Ctrl Pts',(66.9217998601885,29.0911364758487,0.));
#170520=CARTESIAN_POINT('Ctrl Pts',(66.8961104343707,29.0904540435065,0.));
#170521=CARTESIAN_POINT('Ctrl Pts',(66.8704603993794,29.0897484879207,0.));
#170522=CARTESIAN_POINT('Ctrl Pts',(66.8448498552503,29.0890198649323,0.));
#170523=CARTESIAN_POINT('Ctrl Pts',(66.8192789023312,29.088268230663,0.));
#170524=CARTESIAN_POINT('Ctrl Pts',(66.793747641293,29.0874936415132,0.));
#170525=CARTESIAN_POINT('Ctrl Pts',(66.7682561731341,29.0866961541626,0.));
#170526=CARTESIAN_POINT('Ctrl Pts',(66.7428045991841,29.0858758255729,0.));
#170527=CARTESIAN_POINT('Ctrl Pts',(66.7173930211022,29.0850327129916,0.));
#170528=CARTESIAN_POINT('Ctrl Pts',(66.6920215408751,29.0841668739588,0.));
#170529=CARTESIAN_POINT('Ctrl Pts',(66.6666902608249,29.083278366305,0.));
#170530=CARTESIAN_POINT('Ctrl Pts',(66.6413992836147,29.0823672481507,0.));
#170531=CARTESIAN_POINT('Ctrl Pts',(66.6161487122502,29.0814335779084,0.));
#170532=CARTESIAN_POINT('Ctrl Pts',(66.59093865008,29.0804774142854,0.));
#170533=CARTESIAN_POINT('Ctrl Pts',(66.5657692007906,29.0794988162897,0.));
#170534=CARTESIAN_POINT('Ctrl Pts',(66.5406404684132,29.0784978432301,0.));
#170535=CARTESIAN_POINT('Ctrl Pts',(66.5155525573323,29.0774745547152,0.));
#170536=CARTESIAN_POINT('Ctrl Pts',(66.4905055722868,29.0764290106554,0.));
#170537=CARTESIAN_POINT('Ctrl Pts',(66.4654996183731,29.0753612712666,0.));
#170538=CARTESIAN_POINT('Ctrl Pts',(66.4405348010388,29.0742713970755,0.));
#170539=CARTESIAN_POINT('Ctrl Pts',(66.4156112260887,29.0731594489211,0.));
#170540=CARTESIAN_POINT('Ctrl Pts',(66.3907289996932,29.072025487953,0.));
#170541=CARTESIAN_POINT('Ctrl Pts',(66.3658882283903,29.0708695756334,0.));
#170542=CARTESIAN_POINT('Ctrl Pts',(66.3410890190884,29.0696917737399,0.));
#170543=CARTESIAN_POINT('Ctrl Pts',(66.3163314790615,29.0684921443721,0.));
#170544=CARTESIAN_POINT('Ctrl Pts',(66.2916157159536,29.067270749953,0.));
#170545=CARTESIAN_POINT('Ctrl Pts',(66.2669418377871,29.0660276532274,0.));
#170546=CARTESIAN_POINT('Ctrl Pts',(66.2423099529669,29.0647629172645,0.));
#170547=CARTESIAN_POINT('Ctrl Pts',(66.2177201702818,29.0634766054598,0.));
#170548=CARTESIAN_POINT('Ctrl Pts',(66.1931725989008,29.062168781542,0.));
#170549=CARTESIAN_POINT('Ctrl Pts',(66.1686673483757,29.0608395095747,0.));
#170550=CARTESIAN_POINT('Ctrl Pts',(66.144204528652,29.0594888539558,0.));
#170551=CARTESIAN_POINT('Ctrl Pts',(66.1197842500714,29.0581168794191,0.));
#170552=CARTESIAN_POINT('Ctrl Pts',(66.0954066233752,29.0567236510372,0.));
#170553=CARTESIAN_POINT('Ctrl Pts',(66.0710717597003,29.0553092342275,0.));
#170554=CARTESIAN_POINT('Ctrl Pts',(66.0467797705806,29.0538736947547,0.));
#170555=CARTESIAN_POINT('Ctrl Pts',(66.0225307679584,29.0524170987303,0.));
#170556=CARTESIAN_POINT('Ctrl Pts',(65.9983248641877,29.0509395126141,0.));
#170557=CARTESIAN_POINT('Ctrl Pts',(65.9741621720372,29.0494410032173,0.));
#170558=CARTESIAN_POINT('Ctrl Pts',(65.9500428046873,29.0479216377082,0.));
#170559=CARTESIAN_POINT('Ctrl Pts',(65.9259668757309,29.0463814836159,0.));
#170560=CARTESIAN_POINT('Ctrl Pts',(65.9019344991854,29.0448206088288,0.));
#170561=CARTESIAN_POINT('Ctrl Pts',(65.8779457894959,29.0432390815977,0.));
#170562=CARTESIAN_POINT('Ctrl Pts',(65.854000861539,29.0416369705375,0.));
#170563=CARTESIAN_POINT('Ctrl Pts',(65.8300998306198,29.0400143446341,0.));
#170564=CARTESIAN_POINT('Ctrl Pts',(65.8062428124723,29.0383712732473,0.));
#170565=CARTESIAN_POINT('Ctrl Pts',(65.7824299232715,29.0367078261107,0.));
#170566=CARTESIAN_POINT('Ctrl Pts',(65.7586612796375,29.0350240733333,0.));
#170567=CARTESIAN_POINT('Ctrl Pts',(65.7349369986382,29.0333200854026,0.));
#170568=CARTESIAN_POINT('Ctrl Pts',(65.7112571977874,29.0315959331911,0.));
#170569=CARTESIAN_POINT('Ctrl Pts',(65.6876219950465,29.0298516879599,0.));
#170570=CARTESIAN_POINT('Ctrl Pts',(65.664031508836,29.0280874213584,0.));
#170571=CARTESIAN_POINT('Ctrl Pts',(65.6404858580391,29.0263032054261,0.));
#170572=CARTESIAN_POINT('Ctrl Pts',(65.6169851620054,29.0244991125962,0.));
#170573=CARTESIAN_POINT('Ctrl Pts',(65.593529540548,29.0226752157013,0.));
#170574=CARTESIAN_POINT('Ctrl Pts',(65.5701191139455,29.0208315879778,0.));
#170575=CARTESIAN_POINT('Ctrl Pts',(65.5467540029546,29.0189683030654,0.));
#170576=CARTESIAN_POINT('Ctrl Pts',(65.523434328815,29.01708543501,0.));
#170577=CARTESIAN_POINT('Ctrl Pts',(65.5001602132524,29.015183058267,0.));
#170578=CARTESIAN_POINT('Ctrl Pts',(65.4769317784754,29.0132612477075,0.));
#170579=CARTESIAN_POINT('Ctrl Pts',(65.4537491471782,29.0113200786219,0.));
#170580=CARTESIAN_POINT('Ctrl Pts',(65.4306124425524,29.0093596267198,0.));
#170581=CARTESIAN_POINT('Ctrl Pts',(65.4075217882921,29.0073799681336,0.));
#170582=CARTESIAN_POINT('Ctrl Pts',(65.3844773085976,29.0053811794214,0.));
#170583=CARTESIAN_POINT('Ctrl Pts',(65.3614791281725,29.0033633375745,0.));
#170584=CARTESIAN_POINT('Ctrl Pts',(65.3385273722278,29.0013265200201,0.));
#170585=CARTESIAN_POINT('Ctrl Pts',(65.3156221664942,28.9992708046223,0.));
#170586=CARTESIAN_POINT('Ctrl Pts',(65.2927636372261,28.9971962696848,0.));
#170587=CARTESIAN_POINT('Ctrl Pts',(65.2699519112052,28.9951029939551,0.));
#170588=CARTESIAN_POINT('Ctrl Pts',(65.2471871157375,28.9929910566314,0.));
#170589=CARTESIAN_POINT('Ctrl Pts',(65.2244693786586,28.9908605373652,0.));
#170590=CARTESIAN_POINT('Ctrl Pts',(65.2017988283465,28.9887115162626,0.));
#170591=CARTESIAN_POINT('Ctrl Pts',(65.1791755937254,28.9865440738882,0.));
#170592=CARTESIAN_POINT('Ctrl Pts',(65.1565998042705,28.9843582912697,0.));
#170593=CARTESIAN_POINT('Ctrl Pts',(65.1340715900042,28.9821542499049,0.));
#170594=CARTESIAN_POINT('Ctrl Pts',(65.111591081505,28.9799320317648,0.));
#170595=CARTESIAN_POINT('Ctrl Pts',(65.0891584099174,28.9776917192936,0.));
#170596=CARTESIAN_POINT('Ctrl Pts',(65.0667737069562,28.9754333954134,0.));
#170597=CARTESIAN_POINT('Ctrl Pts',(65.0444371049082,28.9731571435281,0.));
#170598=CARTESIAN_POINT('Ctrl Pts',(65.0221487366279,28.9708630475298,0.));
#170599=CARTESIAN_POINT('Ctrl Pts',(64.9999087355504,28.9685511918017,0.));
#170600=CARTESIAN_POINT('Ctrl Pts',(64.9777172357028,28.9662216612216,0.));
#170601=CARTESIAN_POINT('Ctrl Pts',(64.955574371711,28.9638745411677,0.));
#170602=CARTESIAN_POINT('Ctrl Pts',(64.9334802788037,28.961509917525,0.));
#170603=CARTESIAN_POINT('Ctrl Pts',(64.9114350928124,28.9591278766934,0.));
#170604=CARTESIAN_POINT('Ctrl Pts',(64.8894389501799,28.9567285055866,0.));
#170605=CARTESIAN_POINT('Ctrl Pts',(64.8674919879646,28.9543118916327,0.));
#170606=CARTESIAN_POINT('Ctrl Pts',(64.8455943438423,28.9518781227765,0.));
#170607=CARTESIAN_POINT('Ctrl Pts',(64.8237461561024,28.9494272874833,0.));
#170608=CARTESIAN_POINT('Ctrl Pts',(64.8019475636454,28.9469594747436,0.));
#170609=CARTESIAN_POINT('Ctrl Pts',(64.7801987060097,28.9444747740815,0.));
#170610=CARTESIAN_POINT('Ctrl Pts',(64.7584997233889,28.9419732755659,0.));
#170611=CARTESIAN_POINT('Ctrl Pts',(64.7368507566461,28.9394550698201,0.));
#170612=CARTESIAN_POINT('Ctrl Pts',(64.715251947327,28.9369202480383,0.));
#170613=CARTESIAN_POINT('Ctrl Pts',(64.6937034376591,28.934368901987,0.));
#170614=CARTESIAN_POINT('Ctrl Pts',(64.6722053705389,28.9318011239905,0.));
#170615=CARTESIAN_POINT('Ctrl Pts',(64.6507578895155,28.9292170069219,0.));
#170616=CARTESIAN_POINT('Ctrl Pts',(64.6293611387753,28.9266166441956,0.));
#170617=CARTESIAN_POINT('Ctrl Pts',(64.6080152631065,28.9240001297553,0.));
#170618=CARTESIAN_POINT('Ctrl Pts',(64.5867204079452,28.9213675580996,0.));
#170619=CARTESIAN_POINT('Ctrl Pts',(64.5654767194487,28.9187190243231,0.));
#170620=CARTESIAN_POINT('Ctrl Pts',(64.544284344556,28.9160546241538,0.));
#170621=CARTESIAN_POINT('Ctrl Pts',(64.5231434310457,28.9133744539943,0.));
#170622=CARTESIAN_POINT('Ctrl Pts',(64.5020541275927,28.9106786109639,0.));
#170623=CARTESIAN_POINT('Ctrl Pts',(64.4810165836568,28.9079671928253,0.));
#170624=CARTESIAN_POINT('Ctrl Pts',(64.460030949357,28.9052402979055,0.));
#170625=CARTESIAN_POINT('Ctrl Pts',(64.439097375364,28.9024980250309,0.));
#170626=CARTESIAN_POINT('Ctrl Pts',(64.41821601274,28.899740473435,0.));
#170627=CARTESIAN_POINT('Ctrl Pts',(64.3973870129201,28.8969677427519,0.));
#170628=CARTESIAN_POINT('Ctrl Pts',(64.3766105280715,28.8941799332312,0.));
#170629=CARTESIAN_POINT('Ctrl Pts',(64.3558867114087,28.8913771459327,0.));
#170630=CARTESIAN_POINT('Ctrl Pts',(64.3352157174606,28.888559482892,0.));
#170631=CARTESIAN_POINT('Ctrl Pts',(64.3145977025005,28.8857270473944,0.));
#170632=CARTESIAN_POINT('Ctrl Pts',(64.2940328242482,28.8828799437922,0.));
#170633=CARTESIAN_POINT('Ctrl Pts',(64.2735212410682,28.8800182770052,0.));
#170634=CARTESIAN_POINT('Ctrl Pts',(64.2530631112926,28.8771421521058,0.));
#170635=CARTESIAN_POINT('Ctrl Pts',(64.232658592528,28.8742516738959,0.));
#170636=CARTESIAN_POINT('Ctrl Pts',(64.2123078408507,28.8713469464205,0.));
#170637=CARTESIAN_POINT('Ctrl Pts',(64.1920110123342,28.8684280739033,0.));
#170638=CARTESIAN_POINT('Ctrl Pts',(64.1717682648708,28.8654951618659,0.));
#170639=CARTESIAN_POINT('Ctrl Pts',(64.1515797596555,28.8625483180433,0.));
#170640=CARTESIAN_POINT('Ctrl Pts',(64.1314456633345,28.8595876537132,0.));
#170641=CARTESIAN_POINT('Ctrl Pts',(64.1113661481918,28.8566132838157,0.));
#170642=CARTESIAN_POINT('Ctrl Pts',(64.0913413876586,28.8536253241837,0.));
#170643=CARTESIAN_POINT('Ctrl Pts',(64.0713715523588,28.8506238891087,0.));
#170644=CARTESIAN_POINT('Ctrl Pts',(64.0514568066659,28.8476090892242,0.));
#170645=CARTESIAN_POINT('Ctrl Pts',(64.0315973031994,28.8445810281275,0.));
#170646=CARTESIAN_POINT('Ctrl Pts',(64.0117931881364,28.841539805646,0.));
#170647=CARTESIAN_POINT('Ctrl Pts',(63.9920446117632,28.8384855243267,0.));
#170648=CARTESIAN_POINT('Ctrl Pts',(63.9723517369614,28.8354182946601,0.));
#170649=CARTESIAN_POINT('Ctrl Pts',(63.9527147494351,28.8323382413753,0.));
#170650=CARTESIAN_POINT('Ctrl Pts',(63.9331338646868,28.8292455077494,0.));
#170651=CARTESIAN_POINT('Ctrl Pts',(63.9136093063647,28.826140242322,0.));
#170652=CARTESIAN_POINT('Ctrl Pts',(63.894141285685,28.8230225863142,0.));
#170653=CARTESIAN_POINT('Ctrl Pts',(63.8747299825383,28.8198926619893,0.));
#170654=CARTESIAN_POINT('Ctrl Pts',(63.8553755207732,28.8167505576806,0.));
#170655=CARTESIAN_POINT('Ctrl Pts',(63.8360779670225,28.8135963263557,0.));
#170656=CARTESIAN_POINT('Ctrl Pts',(63.8206854735372,28.8110632621133,0.));
#170657=CARTESIAN_POINT('Ctrl Pts',(63.809166727145,28.8091580239664,0.));
#170658=CARTESIAN_POINT('Ctrl Pts',(63.8014989507575,28.8078854475473,0.));
#170659=CARTESIAN_POINT('Ctrl Pts',(63.7976679095314,28.8072485549236,0.));
#170660=CARTESIAN_POINT('Ctrl Pts',(70.8615414811571,22.9976507259816,0.));
#170661=CARTESIAN_POINT('Ctrl Pts',(70.8615414811571,22.9976507259816,12.));
#170662=CARTESIAN_POINT('Ctrl Pts',(70.8559846928,22.9983100639391,0.));
#170663=CARTESIAN_POINT('Ctrl Pts',(70.8559846928,22.9983100639391,12.));
#170664=CARTESIAN_POINT('Ctrl Pts',(70.8448742696689,22.9996258555291,0.));
#170665=CARTESIAN_POINT('Ctrl Pts',(70.8448742696689,22.9996258555291,12.));
#170666=CARTESIAN_POINT('Ctrl Pts',(70.8282180957225,23.0015908899394,0.));
#170667=CARTESIAN_POINT('Ctrl Pts',(70.8282180957225,23.0015908899394,12.));
#170668=CARTESIAN_POINT('Ctrl Pts',(70.8060287860585,23.0041936291626,0.));
#170669=CARTESIAN_POINT('Ctrl Pts',(70.8060287860585,23.0041936291626,12.));
#170670=CARTESIAN_POINT('Ctrl Pts',(70.7783236951202,23.0074182063787,0.));
#170671=CARTESIAN_POINT('Ctrl Pts',(70.7783236951202,23.0074182063787,12.));
#170672=CARTESIAN_POINT('Ctrl Pts',(70.750650169619,23.0106139366046,0.));
#170673=CARTESIAN_POINT('Ctrl Pts',(70.750650169619,23.0106139366046,12.));
#170674=CARTESIAN_POINT('Ctrl Pts',(70.7230082425412,23.0137808248924,0.));
#170675=CARTESIAN_POINT('Ctrl Pts',(70.7230082425412,23.0137808248924,12.));
#170676=CARTESIAN_POINT('Ctrl Pts',(70.6953979633426,23.0169188841045,0.));
#170677=CARTESIAN_POINT('Ctrl Pts',(70.6953979633426,23.0169188841045,12.));
#170678=CARTESIAN_POINT('Ctrl Pts',(70.6678194023135,23.0200281385833,0.));
#170679=CARTESIAN_POINT('Ctrl Pts',(70.6678194023135,23.0200281385833,12.));
#170680=CARTESIAN_POINT('Ctrl Pts',(70.6402726486453,23.0231086235186,0.));
#170681=CARTESIAN_POINT('Ctrl Pts',(70.6402726486453,23.0231086235186,12.));
#170682=CARTESIAN_POINT('Ctrl Pts',(70.6127578036673,23.026160381013,0.));
#170683=CARTESIAN_POINT('Ctrl Pts',(70.6127578036673,23.026160381013,12.));
#170684=CARTESIAN_POINT('Ctrl Pts',(70.5852749754082,23.0291834570663,0.));
#170685=CARTESIAN_POINT('Ctrl Pts',(70.5852749754082,23.0291834570663,12.));
#170686=CARTESIAN_POINT('Ctrl Pts',(70.5578242727627,23.0321778982711,0.));
#170687=CARTESIAN_POINT('Ctrl Pts',(70.5578242727627,23.0321778982711,12.));
#170688=CARTESIAN_POINT('Ctrl Pts',(70.5304057994631,23.0351437484336,0.));
#170689=CARTESIAN_POINT('Ctrl Pts',(70.5304057994631,23.0351437484336,12.));
#170690=CARTESIAN_POINT('Ctrl Pts',(70.5030196492003,23.0380810458271,0.));
#170691=CARTESIAN_POINT('Ctrl Pts',(70.5030196492003,23.0380810458271,12.));
#170692=CARTESIAN_POINT('Ctrl Pts',(70.4756659090209,23.0409898250756,0.));
#170693=CARTESIAN_POINT('Ctrl Pts',(70.4756659090209,23.0409898250756,12.));
#170694=CARTESIAN_POINT('Ctrl Pts',(70.4483446617614,23.0438701185013,0.));
#170695=CARTESIAN_POINT('Ctrl Pts',(70.4483446617614,23.0438701185013,12.));
#170696=CARTESIAN_POINT('Ctrl Pts',(70.4210559889348,23.0467219577291,0.));
#170697=CARTESIAN_POINT('Ctrl Pts',(70.4210559889348,23.0467219577291,12.));
#170698=CARTESIAN_POINT('Ctrl Pts',(70.3937999732267,23.0495453750763,0.));
#170699=CARTESIAN_POINT('Ctrl Pts',(70.3937999732267,23.0495453750763,12.));
#170700=CARTESIAN_POINT('Ctrl Pts',(70.3665767016542,23.0523404053172,0.));
#170701=CARTESIAN_POINT('Ctrl Pts',(70.3665767016542,23.0523404053172,12.));
#170702=CARTESIAN_POINT('Ctrl Pts',(70.3393862652297,23.0551070854926,0.));
#170703=CARTESIAN_POINT('Ctrl Pts',(70.3393862652297,23.0551070854926,12.));
#170704=CARTESIAN_POINT('Ctrl Pts',(70.3122287575335,23.0578454541104,0.));
#170705=CARTESIAN_POINT('Ctrl Pts',(70.3122287575335,23.0578454541104,12.));
#170706=CARTESIAN_POINT('Ctrl Pts',(70.2851042736066,23.0605555505321,0.));
#170707=CARTESIAN_POINT('Ctrl Pts',(70.2851042736066,23.0605555505321,12.));
#170708=CARTESIAN_POINT('Ctrl Pts',(70.2580129087888,23.0632374143279,0.));
#170709=CARTESIAN_POINT('Ctrl Pts',(70.2580129087888,23.0632374143279,12.));
#170710=CARTESIAN_POINT('Ctrl Pts',(70.2309547573815,23.0658910845433,0.));
#170711=CARTESIAN_POINT('Ctrl Pts',(70.2309547573815,23.0658910845433,12.));
#170712=CARTESIAN_POINT('Ctrl Pts',(70.2039299120488,23.0685165993691,0.));
#170713=CARTESIAN_POINT('Ctrl Pts',(70.2039299120488,23.0685165993691,12.));
#170714=CARTESIAN_POINT('Ctrl Pts',(70.1769384645586,23.071113996544,0.));
#170715=CARTESIAN_POINT('Ctrl Pts',(70.1769384645586,23.071113996544,12.));
#170716=CARTESIAN_POINT('Ctrl Pts',(70.1499805062172,23.0736833135938,0.));
#170717=CARTESIAN_POINT('Ctrl Pts',(70.1499805062172,23.0736833135938,12.));
#170718=CARTESIAN_POINT('Ctrl Pts',(70.123056128422,23.0762245881389,0.));
#170719=CARTESIAN_POINT('Ctrl Pts',(70.123056128422,23.0762245881389,12.));
#170720=CARTESIAN_POINT('Ctrl Pts',(70.0961654231639,23.0787378581774,0.));
#170721=CARTESIAN_POINT('Ctrl Pts',(70.0961654231639,23.0787378581774,12.));
#170722=CARTESIAN_POINT('Ctrl Pts',(70.0693084835373,23.0812231623765,0.));
#170723=CARTESIAN_POINT('Ctrl Pts',(70.0693084835373,23.0812231623765,12.));
#170724=CARTESIAN_POINT('Ctrl Pts',(70.0424854035115,23.0836805399374,0.));
#170725=CARTESIAN_POINT('Ctrl Pts',(70.0424854035115,23.0836805399374,12.));
#170726=CARTESIAN_POINT('Ctrl Pts',(70.0156962777169,23.0861100304729,0.));
#170727=CARTESIAN_POINT('Ctrl Pts',(70.0156962777169,23.0861100304729,12.));
#170728=CARTESIAN_POINT('Ctrl Pts',(69.9889412012143,23.0885116738798,0.));
#170729=CARTESIAN_POINT('Ctrl Pts',(69.9889412012143,23.0885116738798,12.));
#170730=CARTESIAN_POINT('Ctrl Pts',(69.9622202692873,23.0908855102251,0.));
#170731=CARTESIAN_POINT('Ctrl Pts',(69.9622202692873,23.0908855102251,12.));
#170732=CARTESIAN_POINT('Ctrl Pts',(69.9355335771729,23.0932315796068,0.));
#170733=CARTESIAN_POINT('Ctrl Pts',(69.9355335771729,23.0932315796068,12.));
#170734=CARTESIAN_POINT('Ctrl Pts',(69.9088812200713,23.0955499221558,0.));
#170735=CARTESIAN_POINT('Ctrl Pts',(69.9088812200713,23.0955499221558,12.));
#170736=CARTESIAN_POINT('Ctrl Pts',(69.8822632932768,23.0978405781021,0.));
#170737=CARTESIAN_POINT('Ctrl Pts',(69.8822632932768,23.0978405781021,12.));
#170738=CARTESIAN_POINT('Ctrl Pts',(69.8556798922693,23.1001035878241,0.));
#170739=CARTESIAN_POINT('Ctrl Pts',(69.8556798922693,23.1001035878241,12.));
#170740=CARTESIAN_POINT('Ctrl Pts',(69.8291311128118,23.1023389919051,0.));
#170741=CARTESIAN_POINT('Ctrl Pts',(69.8291311128118,23.1023389919051,12.));
#170742=CARTESIAN_POINT('Ctrl Pts',(69.8026170510572,23.1045468311991,0.));
#170743=CARTESIAN_POINT('Ctrl Pts',(69.8026170510572,23.1045468311991,12.));
#170744=CARTESIAN_POINT('Ctrl Pts',(69.7761378035964,23.106727146861,0.));
#170745=CARTESIAN_POINT('Ctrl Pts',(69.7761378035964,23.106727146861,12.));
#170746=CARTESIAN_POINT('Ctrl Pts',(69.7496934674069,23.1088799803089,0.));
#170747=CARTESIAN_POINT('Ctrl Pts',(69.7496934674069,23.1088799803089,12.));
#170748=CARTESIAN_POINT('Ctrl Pts',(69.7232841398197,23.1110053732046,0.));
#170749=CARTESIAN_POINT('Ctrl Pts',(69.7232841398197,23.1110053732046,12.));
#170750=CARTESIAN_POINT('Ctrl Pts',(69.6969099184767,23.1131033674301,0.));
#170751=CARTESIAN_POINT('Ctrl Pts',(69.6969099184767,23.1131033674301,12.));
#170752=CARTESIAN_POINT('Ctrl Pts',(69.6705709012852,23.1151740050681,0.));
#170753=CARTESIAN_POINT('Ctrl Pts',(69.6705709012852,23.1151740050681,12.));
#170754=CARTESIAN_POINT('Ctrl Pts',(69.6442671863765,23.1172173283859,0.));
#170755=CARTESIAN_POINT('Ctrl Pts',(69.6442671863765,23.1172173283859,12.));
#170756=CARTESIAN_POINT('Ctrl Pts',(69.6179988721365,23.1192333798441,0.));
#170757=CARTESIAN_POINT('Ctrl Pts',(69.6179988721365,23.1192333798441,12.));
#170758=CARTESIAN_POINT('Ctrl Pts',(69.5917660572265,23.1212222021051,0.));
#170759=CARTESIAN_POINT('Ctrl Pts',(69.5917660572265,23.1212222021051,12.));
#170760=CARTESIAN_POINT('Ctrl Pts',(69.5655688406052,23.1231838380452,0.));
#170761=CARTESIAN_POINT('Ctrl Pts',(69.5655688406052,23.1231838380452,12.));
#170762=CARTESIAN_POINT('Ctrl Pts',(69.539407321546,23.1251183307676,0.));
#170763=CARTESIAN_POINT('Ctrl Pts',(69.539407321546,23.1251183307676,12.));
#170764=CARTESIAN_POINT('Ctrl Pts',(69.5132815996537,23.1270257236204,0.));
#170765=CARTESIAN_POINT('Ctrl Pts',(69.5132815996537,23.1270257236204,12.));
#170766=CARTESIAN_POINT('Ctrl Pts',(69.4871917748654,23.1289060601924,0.));
#170767=CARTESIAN_POINT('Ctrl Pts',(69.4871917748654,23.1289060601924,12.));
#170768=CARTESIAN_POINT('Ctrl Pts',(69.4611379474484,23.1307593843061,0.));
#170769=CARTESIAN_POINT('Ctrl Pts',(69.4611379474484,23.1307593843061,12.));
#170770=CARTESIAN_POINT('Ctrl Pts',(69.4351202179946,23.1325857400144,0.));
#170771=CARTESIAN_POINT('Ctrl Pts',(69.4351202179946,23.1325857400144,12.));
#170772=CARTESIAN_POINT('Ctrl Pts',(69.4091386874132,23.1343851715989,0.));
#170773=CARTESIAN_POINT('Ctrl Pts',(69.4091386874132,23.1343851715989,12.));
#170774=CARTESIAN_POINT('Ctrl Pts',(69.3831934569182,23.1361577235709,0.));
#170775=CARTESIAN_POINT('Ctrl Pts',(69.3831934569182,23.1361577235709,12.));
#170776=CARTESIAN_POINT('Ctrl Pts',(69.3572846280297,23.1379034406718,0.));
#170777=CARTESIAN_POINT('Ctrl Pts',(69.3572846280297,23.1379034406718,12.));
#170778=CARTESIAN_POINT('Ctrl Pts',(69.3314123025869,23.1396223678725,0.));
#170779=CARTESIAN_POINT('Ctrl Pts',(69.3314123025869,23.1396223678725,12.));
#170780=CARTESIAN_POINT('Ctrl Pts',(69.3055765827546,23.1413145503762,0.));
#170781=CARTESIAN_POINT('Ctrl Pts',(69.3055765827546,23.1413145503762,12.));
#170782=CARTESIAN_POINT('Ctrl Pts',(69.2797775710273,23.142980033622,0.));
#170783=CARTESIAN_POINT('Ctrl Pts',(69.2797775710273,23.142980033622,12.));
#170784=CARTESIAN_POINT('Ctrl Pts',(69.254015370231,23.1446188632931,0.));
#170785=CARTESIAN_POINT('Ctrl Pts',(69.254015370231,23.1446188632931,12.));
#170786=CARTESIAN_POINT('Ctrl Pts',(69.2282900835235,23.1462310853206,0.));
#170787=CARTESIAN_POINT('Ctrl Pts',(69.2282900835235,23.1462310853206,12.));
#170788=CARTESIAN_POINT('Ctrl Pts',(69.2026018144028,23.147816745879,0.));
#170789=CARTESIAN_POINT('Ctrl Pts',(69.2026018144028,23.147816745879,12.));
#170790=CARTESIAN_POINT('Ctrl Pts',(69.1769506667084,23.1493758913859,0.));
#170791=CARTESIAN_POINT('Ctrl Pts',(69.1769506667084,23.1493758913859,12.));
#170792=CARTESIAN_POINT('Ctrl Pts',(69.1513367446231,23.1509085685032,0.));
#170793=CARTESIAN_POINT('Ctrl Pts',(69.1513367446231,23.1509085685032,12.));
#170794=CARTESIAN_POINT('Ctrl Pts',(69.1257601526687,23.152414824141,0.));
#170795=CARTESIAN_POINT('Ctrl Pts',(69.1257601526687,23.152414824141,12.));
#170796=CARTESIAN_POINT('Ctrl Pts',(69.1002209957025,23.1538947054615,0.));
#170797=CARTESIAN_POINT('Ctrl Pts',(69.1002209957025,23.1538947054615,12.));
#170798=CARTESIAN_POINT('Ctrl Pts',(69.074719378928,23.1553482598762,0.));
#170799=CARTESIAN_POINT('Ctrl Pts',(69.074719378928,23.1553482598762,12.));
#170800=CARTESIAN_POINT('Ctrl Pts',(69.0492554078992,23.1567755350469,0.));
#170801=CARTESIAN_POINT('Ctrl Pts',(69.0492554078992,23.1567755350469,12.));
#170802=CARTESIAN_POINT('Ctrl Pts',(69.0238291885245,23.1581765788869,0.));
#170803=CARTESIAN_POINT('Ctrl Pts',(69.0238291885245,23.1581765788869,12.));
#170804=CARTESIAN_POINT('Ctrl Pts',(68.9984408270659,23.1595514395656,0.));
#170805=CARTESIAN_POINT('Ctrl Pts',(68.9984408270659,23.1595514395656,12.));
#170806=CARTESIAN_POINT('Ctrl Pts',(68.9730904301369,23.1609001655156,0.));
#170807=CARTESIAN_POINT('Ctrl Pts',(68.9730904301369,23.1609001655156,12.));
#170808=CARTESIAN_POINT('Ctrl Pts',(68.9477781047106,23.1622228054291,0.));
#170809=CARTESIAN_POINT('Ctrl Pts',(68.9477781047106,23.1622228054291,12.));
#170810=CARTESIAN_POINT('Ctrl Pts',(68.9225039581248,23.1635194082581,0.));
#170811=CARTESIAN_POINT('Ctrl Pts',(68.9225039581248,23.1635194082581,12.));
#170812=CARTESIAN_POINT('Ctrl Pts',(68.8972680980842,23.164790023215,0.));
#170813=CARTESIAN_POINT('Ctrl Pts',(68.8972680980842,23.164790023215,12.));
#170814=CARTESIAN_POINT('Ctrl Pts',(68.8720706326609,23.1660346997764,0.));
#170815=CARTESIAN_POINT('Ctrl Pts',(68.8720706326609,23.1660346997764,12.));
#170816=CARTESIAN_POINT('Ctrl Pts',(68.8469116702898,23.1672534876889,0.));
#170817=CARTESIAN_POINT('Ctrl Pts',(68.8469116702898,23.1672534876889,12.));
#170818=CARTESIAN_POINT('Ctrl Pts',(68.8217913197752,23.1684464369686,0.));
#170819=CARTESIAN_POINT('Ctrl Pts',(68.8217913197752,23.1684464369686,12.));
#170820=CARTESIAN_POINT('Ctrl Pts',(68.7967096902996,23.1696135978997,0.));
#170821=CARTESIAN_POINT('Ctrl Pts',(68.7967096902996,23.1696135978997,12.));
#170822=CARTESIAN_POINT('Ctrl Pts',(68.771666891425,23.170755021036,0.));
#170823=CARTESIAN_POINT('Ctrl Pts',(68.771666891425,23.170755021036,12.));
#170824=CARTESIAN_POINT('Ctrl Pts',(68.746663033096,23.1718707572043,0.));
#170825=CARTESIAN_POINT('Ctrl Pts',(68.746663033096,23.1718707572043,12.));
#170826=CARTESIAN_POINT('Ctrl Pts',(68.7216982256341,23.172960857511,0.));
#170827=CARTESIAN_POINT('Ctrl Pts',(68.7216982256341,23.172960857511,12.));
#170828=CARTESIAN_POINT('Ctrl Pts',(68.696772579744,23.1740253733417,0.));
#170829=CARTESIAN_POINT('Ctrl Pts',(68.696772579744,23.1740253733417,12.));
#170830=CARTESIAN_POINT('Ctrl Pts',(68.6718862065216,23.1750643563602,0.));
#170831=CARTESIAN_POINT('Ctrl Pts',(68.6718862065216,23.1750643563602,12.));
#170832=CARTESIAN_POINT('Ctrl Pts',(68.6470392174564,23.1760778585092,0.));
#170833=CARTESIAN_POINT('Ctrl Pts',(68.6470392174564,23.1760778585092,12.));
#170834=CARTESIAN_POINT('Ctrl Pts',(68.6222317244341,23.1770659320138,0.));
#170835=CARTESIAN_POINT('Ctrl Pts',(68.6222317244341,23.1770659320138,12.));
#170836=CARTESIAN_POINT('Ctrl Pts',(68.597463839733,23.1780286293875,0.));
#170837=CARTESIAN_POINT('Ctrl Pts',(68.597463839733,23.1780286293875,12.));
#170838=CARTESIAN_POINT('Ctrl Pts',(68.5727356760278,23.1789660034342,0.));
#170839=CARTESIAN_POINT('Ctrl Pts',(68.5727356760278,23.1789660034342,12.));
#170840=CARTESIAN_POINT('Ctrl Pts',(68.5480473463985,23.179878107245,0.));
#170841=CARTESIAN_POINT('Ctrl Pts',(68.5480473463985,23.179878107245,12.));
#170842=CARTESIAN_POINT('Ctrl Pts',(68.5233989643345,23.180764994201,0.));
#170843=CARTESIAN_POINT('Ctrl Pts',(68.5233989643345,23.180764994201,12.));
#170844=CARTESIAN_POINT('Ctrl Pts',(68.4987906437356,23.1816267179751,0.));
#170845=CARTESIAN_POINT('Ctrl Pts',(68.4987906437356,23.1816267179751,12.));
#170846=CARTESIAN_POINT('Ctrl Pts',(68.4742224989098,23.1824633325385,0.));
#170847=CARTESIAN_POINT('Ctrl Pts',(68.4742224989098,23.1824633325385,12.));
#170848=CARTESIAN_POINT('Ctrl Pts',(68.4496946445758,23.183274892163,0.));
#170849=CARTESIAN_POINT('Ctrl Pts',(68.4496946445758,23.183274892163,12.));
#170850=CARTESIAN_POINT('Ctrl Pts',(68.4252071958729,23.1840614514192,0.));
#170851=CARTESIAN_POINT('Ctrl Pts',(68.4252071958729,23.1840614514192,12.));
#170852=CARTESIAN_POINT('Ctrl Pts',(68.4007602683652,23.1848230651776,0.));
#170853=CARTESIAN_POINT('Ctrl Pts',(68.4007602683652,23.1848230651776,12.));
#170854=CARTESIAN_POINT('Ctrl Pts',(68.376353978044,23.1855597886116,0.));
#170855=CARTESIAN_POINT('Ctrl Pts',(68.376353978044,23.1855597886116,12.));
#170856=CARTESIAN_POINT('Ctrl Pts',(68.3519884413246,23.1862716772031,0.));
#170857=CARTESIAN_POINT('Ctrl Pts',(68.3519884413246,23.1862716772031,12.));
#170858=CARTESIAN_POINT('Ctrl Pts',(68.3276637750485,23.1869587867459,0.));
#170859=CARTESIAN_POINT('Ctrl Pts',(68.3276637750485,23.1869587867459,12.));
#170860=CARTESIAN_POINT('Ctrl Pts',(68.3033800964939,23.1876211733436,0.));
#170861=CARTESIAN_POINT('Ctrl Pts',(68.3033800964939,23.1876211733436,12.));
#170862=CARTESIAN_POINT('Ctrl Pts',(68.2791375233795,23.1882588934107,0.));
#170863=CARTESIAN_POINT('Ctrl Pts',(68.2791375233795,23.1882588934107,12.));
#170864=CARTESIAN_POINT('Ctrl Pts',(68.2549361738681,23.1888720036757,0.));
#170865=CARTESIAN_POINT('Ctrl Pts',(68.2549361738681,23.1888720036757,12.));
#170866=CARTESIAN_POINT('Ctrl Pts',(68.2307761665633,23.1894605611871,0.));
#170867=CARTESIAN_POINT('Ctrl Pts',(68.2307761665633,23.1894605611871,12.));
#170868=CARTESIAN_POINT('Ctrl Pts',(68.2066576205116,23.1900246233165,0.));
#170869=CARTESIAN_POINT('Ctrl Pts',(68.2066576205116,23.1900246233165,12.));
#170870=CARTESIAN_POINT('Ctrl Pts',(68.1825806552129,23.1905642477571,0.));
#170871=CARTESIAN_POINT('Ctrl Pts',(68.1825806552129,23.1905642477571,12.));
#170872=CARTESIAN_POINT('Ctrl Pts',(68.1585453906257,23.1910794925251,0.));
#170873=CARTESIAN_POINT('Ctrl Pts',(68.1585453906257,23.1910794925251,12.));
#170874=CARTESIAN_POINT('Ctrl Pts',(68.1345519471695,23.1915704159623,0.));
#170875=CARTESIAN_POINT('Ctrl Pts',(68.1345519471695,23.1915704159623,12.));
#170876=CARTESIAN_POINT('Ctrl Pts',(68.110600445723,23.1920370767426,0.));
#170877=CARTESIAN_POINT('Ctrl Pts',(68.110600445723,23.1920370767426,12.));
#170878=CARTESIAN_POINT('Ctrl Pts',(68.0866910076251,23.1924795338749,0.));
#170879=CARTESIAN_POINT('Ctrl Pts',(68.0866910076251,23.1924795338749,12.));
#170880=CARTESIAN_POINT('Ctrl Pts',(68.0628237546863,23.1928978467021,0.));
#170881=CARTESIAN_POINT('Ctrl Pts',(68.0628237546863,23.1928978467021,12.));
#170882=CARTESIAN_POINT('Ctrl Pts',(68.0389988091933,23.1932920749023,0.));
#170883=CARTESIAN_POINT('Ctrl Pts',(68.0389988091933,23.1932920749023,12.));
#170884=CARTESIAN_POINT('Ctrl Pts',(68.0152162939121,23.1936622784919,0.));
#170885=CARTESIAN_POINT('Ctrl Pts',(68.0152162939121,23.1936622784919,12.));
#170886=CARTESIAN_POINT('Ctrl Pts',(67.991476332086,23.1940085178313,0.));
#170887=CARTESIAN_POINT('Ctrl Pts',(67.991476332086,23.1940085178313,12.));
#170888=CARTESIAN_POINT('Ctrl Pts',(67.9677790474385,23.1943308536297,0.));
#170889=CARTESIAN_POINT('Ctrl Pts',(67.9677790474385,23.1943308536297,12.));
#170890=CARTESIAN_POINT('Ctrl Pts',(67.9441245641842,23.1946293469427,0.));
#170891=CARTESIAN_POINT('Ctrl Pts',(67.9441245641842,23.1946293469427,12.));
#170892=CARTESIAN_POINT('Ctrl Pts',(67.9205130070324,23.1949040591744,0.));
#170893=CARTESIAN_POINT('Ctrl Pts',(67.9205130070324,23.1949040591744,12.));
#170894=CARTESIAN_POINT('Ctrl Pts',(67.8969445011916,23.1951550520802,0.));
#170895=CARTESIAN_POINT('Ctrl Pts',(67.8969445011916,23.1951550520802,12.));
#170896=CARTESIAN_POINT('Ctrl Pts',(67.8734191723667,23.1953823877734,0.));
#170897=CARTESIAN_POINT('Ctrl Pts',(67.8734191723667,23.1953823877734,12.));
#170898=CARTESIAN_POINT('Ctrl Pts',(67.8499371467616,23.1955861287286,0.));
#170899=CARTESIAN_POINT('Ctrl Pts',(67.8499371467616,23.1955861287286,12.));
#170900=CARTESIAN_POINT('Ctrl Pts',(67.8264985510917,23.1957663377806,0.));
#170901=CARTESIAN_POINT('Ctrl Pts',(67.8264985510917,23.1957663377806,12.));
#170902=CARTESIAN_POINT('Ctrl Pts',(67.8031035125887,23.1959230781269,0.));
#170903=CARTESIAN_POINT('Ctrl Pts',(67.8031035125887,23.1959230781269,12.));
#170904=CARTESIAN_POINT('Ctrl Pts',(67.7797521590045,23.1960564133304,0.));
#170905=CARTESIAN_POINT('Ctrl Pts',(67.7797521590045,23.1960564133304,12.));
#170906=CARTESIAN_POINT('Ctrl Pts',(67.7564446186079,23.1961664073262,0.));
#170907=CARTESIAN_POINT('Ctrl Pts',(67.7564446186079,23.1961664073262,12.));
#170908=CARTESIAN_POINT('Ctrl Pts',(67.7331810201883,23.1962531244245,0.));
#170909=CARTESIAN_POINT('Ctrl Pts',(67.7331810201883,23.1962531244245,12.));
#170910=CARTESIAN_POINT('Ctrl Pts',(67.7099614930671,23.1963166293102,0.));
#170911=CARTESIAN_POINT('Ctrl Pts',(67.7099614930671,23.1963166293102,12.));
#170912=CARTESIAN_POINT('Ctrl Pts',(67.6867861671031,23.1963569870451,0.));
#170913=CARTESIAN_POINT('Ctrl Pts',(67.6867861671031,23.1963569870451,12.));
#170914=CARTESIAN_POINT('Ctrl Pts',(67.6636551726964,23.1963742630715,0.));
#170915=CARTESIAN_POINT('Ctrl Pts',(67.6636551726964,23.1963742630715,12.));
#170916=CARTESIAN_POINT('Ctrl Pts',(67.6405686407863,23.1963685232188,0.));
#170917=CARTESIAN_POINT('Ctrl Pts',(67.6405686407863,23.1963685232188,12.));
#170918=CARTESIAN_POINT('Ctrl Pts',(67.6175267028555,23.1963398337069,0.));
#170919=CARTESIAN_POINT('Ctrl Pts',(67.6175267028555,23.1963398337069,12.));
#170920=CARTESIAN_POINT('Ctrl Pts',(67.5945294909426,23.1962882611453,0.));
#170921=CARTESIAN_POINT('Ctrl Pts',(67.5945294909426,23.1962882611453,12.));
#170922=CARTESIAN_POINT('Ctrl Pts',(67.5715771376461,23.196213872536,0.));
#170923=CARTESIAN_POINT('Ctrl Pts',(67.5715771376461,23.196213872536,12.));
#170924=CARTESIAN_POINT('Ctrl Pts',(67.5486697761288,23.1961167352772,0.));
#170925=CARTESIAN_POINT('Ctrl Pts',(67.5486697761288,23.1961167352772,12.));
#170926=CARTESIAN_POINT('Ctrl Pts',(67.5258075401146,23.1959969171701,0.));
#170927=CARTESIAN_POINT('Ctrl Pts',(67.5258075401146,23.1959969171701,12.));
#170928=CARTESIAN_POINT('Ctrl Pts',(67.5029905638949,23.1958544864215,0.));
#170929=CARTESIAN_POINT('Ctrl Pts',(67.5029905638949,23.1958544864215,12.));
#170930=CARTESIAN_POINT('Ctrl Pts',(67.4802189823408,23.195689511644,0.));
#170931=CARTESIAN_POINT('Ctrl Pts',(67.4802189823408,23.195689511644,12.));
#170932=CARTESIAN_POINT('Ctrl Pts',(67.4574929309076,23.195502061859,0.));
#170933=CARTESIAN_POINT('Ctrl Pts',(67.4574929309076,23.195502061859,12.));
#170934=CARTESIAN_POINT('Ctrl Pts',(67.4348125456398,23.1952922065012,0.));
#170935=CARTESIAN_POINT('Ctrl Pts',(67.4348125456398,23.1952922065012,12.));
#170936=CARTESIAN_POINT('Ctrl Pts',(67.412177963168,23.1950600154265,0.));
#170937=CARTESIAN_POINT('Ctrl Pts',(67.412177963168,23.1950600154265,12.));
#170938=CARTESIAN_POINT('Ctrl Pts',(67.3895893207182,23.1948055589129,0.));
#170939=CARTESIAN_POINT('Ctrl Pts',(67.3895893207182,23.1948055589129,12.));
#170940=CARTESIAN_POINT('Ctrl Pts',(67.3670467561212,23.194528907661,0.));
#170941=CARTESIAN_POINT('Ctrl Pts',(67.3670467561212,23.194528907661,12.));
#170942=CARTESIAN_POINT('Ctrl Pts',(67.3445504078176,23.1942301327978,0.));
#170943=CARTESIAN_POINT('Ctrl Pts',(67.3445504078176,23.1942301327978,12.));
#170944=CARTESIAN_POINT('Ctrl Pts',(67.3221004148603,23.1939093058801,0.));
#170945=CARTESIAN_POINT('Ctrl Pts',(67.3221004148603,23.1939093058801,12.));
#170946=CARTESIAN_POINT('Ctrl Pts',(67.2996969169098,23.1935664989018,0.));
#170947=CARTESIAN_POINT('Ctrl Pts',(67.2996969169098,23.1935664989018,12.));
#170948=CARTESIAN_POINT('Ctrl Pts',(67.2773400542477,23.1932017842953,0.));
#170949=CARTESIAN_POINT('Ctrl Pts',(67.2773400542477,23.1932017842953,12.));
#170950=CARTESIAN_POINT('Ctrl Pts',(67.2550299677888,23.1928152349343,0.));
#170951=CARTESIAN_POINT('Ctrl Pts',(67.2550299677888,23.1928152349343,12.));
#170952=CARTESIAN_POINT('Ctrl Pts',(67.232766799088,23.1924069241385,0.));
#170953=CARTESIAN_POINT('Ctrl Pts',(67.232766799088,23.1924069241385,12.));
#170954=CARTESIAN_POINT('Ctrl Pts',(67.2105506903447,23.1919769256803,0.));
#170955=CARTESIAN_POINT('Ctrl Pts',(67.2105506903447,23.1919769256803,12.));
#170956=CARTESIAN_POINT('Ctrl Pts',(67.1883817844038,23.1915253137924,0.));
#170957=CARTESIAN_POINT('Ctrl Pts',(67.1883817844038,23.1915253137924,12.));
#170958=CARTESIAN_POINT('Ctrl Pts',(67.1662602247639,23.1910521631657,0.));
#170959=CARTESIAN_POINT('Ctrl Pts',(67.1662602247639,23.1910521631657,12.));
#170960=CARTESIAN_POINT('Ctrl Pts',(67.1441861555817,23.1905575489505,0.));
#170961=CARTESIAN_POINT('Ctrl Pts',(67.1441861555817,23.1905575489505,12.));
#170962=CARTESIAN_POINT('Ctrl Pts',(67.1221597216741,23.1900415467574,0.));
#170963=CARTESIAN_POINT('Ctrl Pts',(67.1221597216741,23.1900415467574,12.));
#170964=CARTESIAN_POINT('Ctrl Pts',(67.1001810685143,23.1895042326627,0.));
#170965=CARTESIAN_POINT('Ctrl Pts',(67.1001810685143,23.1895042326627,12.));
#170966=CARTESIAN_POINT('Ctrl Pts',(67.0782503422305,23.1889456832119,0.));
#170967=CARTESIAN_POINT('Ctrl Pts',(67.0782503422305,23.1889456832119,12.));
#170968=CARTESIAN_POINT('Ctrl Pts',(67.0563676896325,23.1883659754271,0.));
#170969=CARTESIAN_POINT('Ctrl Pts',(67.0563676896325,23.1883659754271,12.));
#170970=CARTESIAN_POINT('Ctrl Pts',(67.0345332582306,23.1877651868158,0.));
#170971=CARTESIAN_POINT('Ctrl Pts',(67.0345332582306,23.1877651868158,12.));
#170972=CARTESIAN_POINT('Ctrl Pts',(67.0127471962501,23.1871433953793,0.));
#170973=CARTESIAN_POINT('Ctrl Pts',(67.0127471962501,23.1871433953793,12.));
#170974=CARTESIAN_POINT('Ctrl Pts',(66.9910096526462,23.1865006796283,0.));
#170975=CARTESIAN_POINT('Ctrl Pts',(66.9910096526462,23.1865006796283,12.));
#170976=CARTESIAN_POINT('Ctrl Pts',(66.9693207771031,23.1858371185842,0.));
#170977=CARTESIAN_POINT('Ctrl Pts',(66.9693207771031,23.1858371185842,12.));
#170978=CARTESIAN_POINT('Ctrl Pts',(66.9476807200203,23.1851527917657,0.));
#170979=CARTESIAN_POINT('Ctrl Pts',(66.9476807200203,23.1851527917657,12.));
#170980=CARTESIAN_POINT('Ctrl Pts',(66.9260896324949,23.1844477791814,0.));
#170981=CARTESIAN_POINT('Ctrl Pts',(66.9260896324949,23.1844477791814,12.));
#170982=CARTESIAN_POINT('Ctrl Pts',(66.9045476663063,23.1837221613235,0.));
#170983=CARTESIAN_POINT('Ctrl Pts',(66.9045476663063,23.1837221613235,12.));
#170984=CARTESIAN_POINT('Ctrl Pts',(66.8830549738795,23.1829760191591,0.));
#170985=CARTESIAN_POINT('Ctrl Pts',(66.8830549738795,23.1829760191591,12.));
#170986=CARTESIAN_POINT('Ctrl Pts',(66.8616117083331,23.1822094341517,0.));
#170987=CARTESIAN_POINT('Ctrl Pts',(66.8616117083331,23.1822094341517,12.));
#170988=CARTESIAN_POINT('Ctrl Pts',(66.8402180235566,23.1814224882953,0.));
#170989=CARTESIAN_POINT('Ctrl Pts',(66.8402180235566,23.1814224882953,12.));
#170990=CARTESIAN_POINT('Ctrl Pts',(66.8188740742727,23.1806152641475,0.));
#170991=CARTESIAN_POINT('Ctrl Pts',(66.8188740742727,23.1806152641475,12.));
#170992=CARTESIAN_POINT('Ctrl Pts',(66.7975800161,23.1797878448639,0.));
#170993=CARTESIAN_POINT('Ctrl Pts',(66.7975800161,23.1797878448639,12.));
#170994=CARTESIAN_POINT('Ctrl Pts',(66.776336005612,23.1789403142366,0.));
#170995=CARTESIAN_POINT('Ctrl Pts',(66.776336005612,23.1789403142366,12.));
#170996=CARTESIAN_POINT('Ctrl Pts',(66.7551422002204,23.17807275663,0.));
#170997=CARTESIAN_POINT('Ctrl Pts',(66.7551422002204,23.17807275663,12.));
#170998=CARTESIAN_POINT('Ctrl Pts',(66.7339987580427,23.1771852569131,0.));
#170999=CARTESIAN_POINT('Ctrl Pts',(66.7339987580427,23.1771852569131,12.));
#171000=CARTESIAN_POINT('Ctrl Pts',(66.7129058377896,23.1762779004044,0.));
#171001=CARTESIAN_POINT('Ctrl Pts',(66.7129058377896,23.1762779004044,12.));
#171002=CARTESIAN_POINT('Ctrl Pts',(66.6918635985972,23.1753507727939,0.));
#171003=CARTESIAN_POINT('Ctrl Pts',(66.6918635985972,23.1753507727939,12.));
#171004=CARTESIAN_POINT('Ctrl Pts',(66.6708722000079,23.1744039601382,0.));
#171005=CARTESIAN_POINT('Ctrl Pts',(66.6708722000079,23.1744039601382,12.));
#171006=CARTESIAN_POINT('Ctrl Pts',(66.6499318023473,23.1734375490431,0.));
#171007=CARTESIAN_POINT('Ctrl Pts',(66.6499318023473,23.1734375490431,12.));
#171008=CARTESIAN_POINT('Ctrl Pts',(66.6290425670548,23.1724516268302,0.));
#171009=CARTESIAN_POINT('Ctrl Pts',(66.6290425670548,23.1724516268302,12.));
#171010=CARTESIAN_POINT('Ctrl Pts',(66.6082046569644,23.1714462816789,0.));
#171011=CARTESIAN_POINT('Ctrl Pts',(66.6082046569644,23.1714462816789,12.));
#171012=CARTESIAN_POINT('Ctrl Pts',(66.5874182367563,23.1704216028614,0.));
#171013=CARTESIAN_POINT('Ctrl Pts',(66.5874182367563,23.1704216028614,12.));
#171014=CARTESIAN_POINT('Ctrl Pts',(66.5666834726454,23.1693776805866,0.));
#171015=CARTESIAN_POINT('Ctrl Pts',(66.5666834726454,23.1693776805866,12.));
#171016=CARTESIAN_POINT('Ctrl Pts',(66.5460005315376,23.1683146055726,0.));
#171017=CARTESIAN_POINT('Ctrl Pts',(66.5460005315376,23.1683146055726,12.));
#171018=CARTESIAN_POINT('Ctrl Pts',(66.5253695803205,23.1672324686926,0.));
#171019=CARTESIAN_POINT('Ctrl Pts',(66.5253695803205,23.1672324686926,12.));
#171020=CARTESIAN_POINT('Ctrl Pts',(66.5047907851348,23.1661313606132,0.));
#171021=CARTESIAN_POINT('Ctrl Pts',(66.5047907851348,23.1661313606132,12.));
#171022=CARTESIAN_POINT('Ctrl Pts',(66.4842643105311,23.1650113713808,0.));
#171023=CARTESIAN_POINT('Ctrl Pts',(66.4842643105311,23.1650113713808,12.));
#171024=CARTESIAN_POINT('Ctrl Pts',(66.4637903210727,23.1638725912195,0.));
#171025=CARTESIAN_POINT('Ctrl Pts',(66.4637903210727,23.1638725912195,12.));
#171026=CARTESIAN_POINT('Ctrl Pts',(66.4433689832478,23.1627151114883,0.));
#171027=CARTESIAN_POINT('Ctrl Pts',(66.4433689832478,23.1627151114883,12.));
#171028=CARTESIAN_POINT('Ctrl Pts',(66.4230004670278,23.1615390254632,0.));
#171029=CARTESIAN_POINT('Ctrl Pts',(66.4230004670278,23.1615390254632,12.));
#171030=CARTESIAN_POINT('Ctrl Pts',(66.4026849481232,23.160344429474,0.));
#171031=CARTESIAN_POINT('Ctrl Pts',(66.4026849481232,23.160344429474,12.));
#171032=CARTESIAN_POINT('Ctrl Pts',(66.3824226081801,23.1591314230083,0.));
#171033=CARTESIAN_POINT('Ctrl Pts',(66.3824226081801,23.1591314230083,12.));
#171034=CARTESIAN_POINT('Ctrl Pts',(66.3622136300654,23.1579001063424,0.));
#171035=CARTESIAN_POINT('Ctrl Pts',(66.3622136300654,23.1579001063424,12.));
#171036=CARTESIAN_POINT('Ctrl Pts',(66.3420581937147,23.1566505784621,0.));
#171037=CARTESIAN_POINT('Ctrl Pts',(66.3420581937147,23.1566505784621,12.));
#171038=CARTESIAN_POINT('Ctrl Pts',(66.3219564725184,23.1553829352539,0.));
#171039=CARTESIAN_POINT('Ctrl Pts',(66.3219564725184,23.1553829352539,12.));
#171040=CARTESIAN_POINT('Ctrl Pts',(66.3019086275444,23.1540972666191,0.));
#171041=CARTESIAN_POINT('Ctrl Pts',(66.3019086275444,23.1540972666191,12.));
#171042=CARTESIAN_POINT('Ctrl Pts',(66.281914813114,23.1527936592651,0.));
#171043=CARTESIAN_POINT('Ctrl Pts',(66.281914813114,23.1527936592651,12.));
#171044=CARTESIAN_POINT('Ctrl Pts',(66.2619751878793,23.1514722022503,0.));
#171045=CARTESIAN_POINT('Ctrl Pts',(66.2619751878793,23.1514722022503,12.));
#171046=CARTESIAN_POINT('Ctrl Pts',(66.2420899237318,23.1501329914488,0.));
#171047=CARTESIAN_POINT('Ctrl Pts',(66.2420899237318,23.1501329914488,12.));
#171048=CARTESIAN_POINT('Ctrl Pts',(66.2222592165398,23.1487761349298,0.));
#171049=CARTESIAN_POINT('Ctrl Pts',(66.2222592165398,23.1487761349298,12.));
#171050=CARTESIAN_POINT('Ctrl Pts',(66.2024832934733,23.147401756643,0.));
#171051=CARTESIAN_POINT('Ctrl Pts',(66.2024832934733,23.147401756643,12.));
#171052=CARTESIAN_POINT('Ctrl Pts',(66.1827623902755,23.1460099850704,0.));
#171053=CARTESIAN_POINT('Ctrl Pts',(66.1827623902755,23.1460099850704,12.));
#171054=CARTESIAN_POINT('Ctrl Pts',(66.163096729667,23.1446009424871,0.));
#171055=CARTESIAN_POINT('Ctrl Pts',(66.163096729667,23.1446009424871,12.));
#171056=CARTESIAN_POINT('Ctrl Pts',(66.14348650151,23.1431747350127,0.));
#171057=CARTESIAN_POINT('Ctrl Pts',(66.14348650151,23.1431747350127,12.));
#171058=CARTESIAN_POINT('Ctrl Pts',(66.1239318368803,23.1417314398501,0.));
#171059=CARTESIAN_POINT('Ctrl Pts',(66.1239318368803,23.1417314398501,12.));
#171060=CARTESIAN_POINT('Ctrl Pts',(66.1044328067739,23.140271103958,0.));
#171061=CARTESIAN_POINT('Ctrl Pts',(66.1044328067739,23.140271103958,12.));
#171062=CARTESIAN_POINT('Ctrl Pts',(66.0888781152779,23.1390892229923,0.));
#171063=CARTESIAN_POINT('Ctrl Pts',(66.0888781152779,23.1390892229923,12.));
#171064=CARTESIAN_POINT('Ctrl Pts',(66.0772371487475,23.1381951597491,0.));
#171065=CARTESIAN_POINT('Ctrl Pts',(66.0772371487475,23.1381951597491,12.));
#171066=CARTESIAN_POINT('Ctrl Pts',(66.0694876382212,23.1375957166138,0.));
#171067=CARTESIAN_POINT('Ctrl Pts',(66.0694876382212,23.1375957166138,12.));
#171068=CARTESIAN_POINT('Ctrl Pts',(66.0656156664138,23.1372951448024,0.));
#171069=CARTESIAN_POINT('Ctrl Pts',(66.0656156664138,23.1372951448024,12.));
#171070=CARTESIAN_POINT('',(66.0656156664138,23.1372951448024,12.));
#171071=CARTESIAN_POINT('Ctrl Pts',(66.0656156664138,23.1372951448024,12.));
#171072=CARTESIAN_POINT('Ctrl Pts',(66.0694876382212,23.1375957166138,12.));
#171073=CARTESIAN_POINT('Ctrl Pts',(66.0772371487475,23.1381951597491,12.));
#171074=CARTESIAN_POINT('Ctrl Pts',(66.0888781152779,23.1390892229923,12.));
#171075=CARTESIAN_POINT('Ctrl Pts',(66.1044328067739,23.140271103958,12.));
#171076=CARTESIAN_POINT('Ctrl Pts',(66.1239318368803,23.1417314398501,12.));
#171077=CARTESIAN_POINT('Ctrl Pts',(66.14348650151,23.1431747350127,12.));
#171078=CARTESIAN_POINT('Ctrl Pts',(66.163096729667,23.1446009424871,12.));
#171079=CARTESIAN_POINT('Ctrl Pts',(66.1827623902755,23.1460099850704,12.));
#171080=CARTESIAN_POINT('Ctrl Pts',(66.2024832934733,23.147401756643,12.));
#171081=CARTESIAN_POINT('Ctrl Pts',(66.2222592165398,23.1487761349298,12.));
#171082=CARTESIAN_POINT('Ctrl Pts',(66.2420899237318,23.1501329914488,12.));
#171083=CARTESIAN_POINT('Ctrl Pts',(66.2619751878793,23.1514722022503,12.));
#171084=CARTESIAN_POINT('Ctrl Pts',(66.281914813114,23.1527936592651,12.));
#171085=CARTESIAN_POINT('Ctrl Pts',(66.3019086275444,23.1540972666191,12.));
#171086=CARTESIAN_POINT('Ctrl Pts',(66.3219564725184,23.1553829352539,12.));
#171087=CARTESIAN_POINT('Ctrl Pts',(66.3420581937147,23.1566505784621,12.));
#171088=CARTESIAN_POINT('Ctrl Pts',(66.3622136300654,23.1579001063424,12.));
#171089=CARTESIAN_POINT('Ctrl Pts',(66.3824226081801,23.1591314230083,12.));
#171090=CARTESIAN_POINT('Ctrl Pts',(66.4026849481232,23.160344429474,12.));
#171091=CARTESIAN_POINT('Ctrl Pts',(66.4230004670278,23.1615390254632,12.));
#171092=CARTESIAN_POINT('Ctrl Pts',(66.4433689832478,23.1627151114883,12.));
#171093=CARTESIAN_POINT('Ctrl Pts',(66.4637903210727,23.1638725912195,12.));
#171094=CARTESIAN_POINT('Ctrl Pts',(66.4842643105311,23.1650113713808,12.));
#171095=CARTESIAN_POINT('Ctrl Pts',(66.5047907851348,23.1661313606132,12.));
#171096=CARTESIAN_POINT('Ctrl Pts',(66.5253695803205,23.1672324686926,12.));
#171097=CARTESIAN_POINT('Ctrl Pts',(66.5460005315376,23.1683146055726,12.));
#171098=CARTESIAN_POINT('Ctrl Pts',(66.5666834726454,23.1693776805866,12.));
#171099=CARTESIAN_POINT('Ctrl Pts',(66.5874182367563,23.1704216028614,12.));
#171100=CARTESIAN_POINT('Ctrl Pts',(66.6082046569644,23.1714462816789,12.));
#171101=CARTESIAN_POINT('Ctrl Pts',(66.6290425670548,23.1724516268302,12.));
#171102=CARTESIAN_POINT('Ctrl Pts',(66.6499318023473,23.1734375490431,12.));
#171103=CARTESIAN_POINT('Ctrl Pts',(66.6708722000079,23.1744039601382,12.));
#171104=CARTESIAN_POINT('Ctrl Pts',(66.6918635985972,23.1753507727939,12.));
#171105=CARTESIAN_POINT('Ctrl Pts',(66.7129058377896,23.1762779004044,12.));
#171106=CARTESIAN_POINT('Ctrl Pts',(66.7339987580427,23.1771852569131,12.));
#171107=CARTESIAN_POINT('Ctrl Pts',(66.7551422002204,23.17807275663,12.));
#171108=CARTESIAN_POINT('Ctrl Pts',(66.776336005612,23.1789403142366,12.));
#171109=CARTESIAN_POINT('Ctrl Pts',(66.7975800161,23.1797878448639,12.));
#171110=CARTESIAN_POINT('Ctrl Pts',(66.8188740742727,23.1806152641475,12.));
#171111=CARTESIAN_POINT('Ctrl Pts',(66.8402180235566,23.1814224882953,12.));
#171112=CARTESIAN_POINT('Ctrl Pts',(66.8616117083331,23.1822094341517,12.));
#171113=CARTESIAN_POINT('Ctrl Pts',(66.8830549738795,23.1829760191591,12.));
#171114=CARTESIAN_POINT('Ctrl Pts',(66.9045476663063,23.1837221613235,12.));
#171115=CARTESIAN_POINT('Ctrl Pts',(66.9260896324949,23.1844477791814,12.));
#171116=CARTESIAN_POINT('Ctrl Pts',(66.9476807200203,23.1851527917657,12.));
#171117=CARTESIAN_POINT('Ctrl Pts',(66.9693207771031,23.1858371185842,12.));
#171118=CARTESIAN_POINT('Ctrl Pts',(66.9910096526462,23.1865006796283,12.));
#171119=CARTESIAN_POINT('Ctrl Pts',(67.0127471962501,23.1871433953793,12.));
#171120=CARTESIAN_POINT('Ctrl Pts',(67.0345332582306,23.1877651868158,12.));
#171121=CARTESIAN_POINT('Ctrl Pts',(67.0563676896325,23.1883659754271,12.));
#171122=CARTESIAN_POINT('Ctrl Pts',(67.0782503422305,23.1889456832119,12.));
#171123=CARTESIAN_POINT('Ctrl Pts',(67.1001810685143,23.1895042326627,12.));
#171124=CARTESIAN_POINT('Ctrl Pts',(67.1221597216741,23.1900415467574,12.));
#171125=CARTESIAN_POINT('Ctrl Pts',(67.1441861555817,23.1905575489505,12.));
#171126=CARTESIAN_POINT('Ctrl Pts',(67.1662602247639,23.1910521631657,12.));
#171127=CARTESIAN_POINT('Ctrl Pts',(67.1883817844038,23.1915253137924,12.));
#171128=CARTESIAN_POINT('Ctrl Pts',(67.2105506903447,23.1919769256803,12.));
#171129=CARTESIAN_POINT('Ctrl Pts',(67.232766799088,23.1924069241385,12.));
#171130=CARTESIAN_POINT('Ctrl Pts',(67.2550299677888,23.1928152349343,12.));
#171131=CARTESIAN_POINT('Ctrl Pts',(67.2773400542477,23.1932017842953,12.));
#171132=CARTESIAN_POINT('Ctrl Pts',(67.2996969169098,23.1935664989018,12.));
#171133=CARTESIAN_POINT('Ctrl Pts',(67.3221004148603,23.1939093058801,12.));
#171134=CARTESIAN_POINT('Ctrl Pts',(67.3445504078176,23.1942301327978,12.));
#171135=CARTESIAN_POINT('Ctrl Pts',(67.3670467561212,23.194528907661,12.));
#171136=CARTESIAN_POINT('Ctrl Pts',(67.3895893207182,23.1948055589129,12.));
#171137=CARTESIAN_POINT('Ctrl Pts',(67.412177963168,23.1950600154265,12.));
#171138=CARTESIAN_POINT('Ctrl Pts',(67.4348125456398,23.1952922065012,12.));
#171139=CARTESIAN_POINT('Ctrl Pts',(67.4574929309076,23.195502061859,12.));
#171140=CARTESIAN_POINT('Ctrl Pts',(67.4802189823408,23.195689511644,12.));
#171141=CARTESIAN_POINT('Ctrl Pts',(67.5029905638949,23.1958544864215,12.));
#171142=CARTESIAN_POINT('Ctrl Pts',(67.5258075401146,23.1959969171701,12.));
#171143=CARTESIAN_POINT('Ctrl Pts',(67.5486697761288,23.1961167352772,12.));
#171144=CARTESIAN_POINT('Ctrl Pts',(67.5715771376461,23.196213872536,12.));
#171145=CARTESIAN_POINT('Ctrl Pts',(67.5945294909426,23.1962882611453,12.));
#171146=CARTESIAN_POINT('Ctrl Pts',(67.6175267028555,23.1963398337069,12.));
#171147=CARTESIAN_POINT('Ctrl Pts',(67.6405686407863,23.1963685232188,12.));
#171148=CARTESIAN_POINT('Ctrl Pts',(67.6636551726964,23.1963742630715,12.));
#171149=CARTESIAN_POINT('Ctrl Pts',(67.6867861671031,23.1963569870451,12.));
#171150=CARTESIAN_POINT('Ctrl Pts',(67.7099614930671,23.1963166293102,12.));
#171151=CARTESIAN_POINT('Ctrl Pts',(67.7331810201883,23.1962531244245,12.));
#171152=CARTESIAN_POINT('Ctrl Pts',(67.7564446186079,23.1961664073262,12.));
#171153=CARTESIAN_POINT('Ctrl Pts',(67.7797521590045,23.1960564133304,12.));
#171154=CARTESIAN_POINT('Ctrl Pts',(67.8031035125887,23.1959230781269,12.));
#171155=CARTESIAN_POINT('Ctrl Pts',(67.8264985510917,23.1957663377806,12.));
#171156=CARTESIAN_POINT('Ctrl Pts',(67.8499371467616,23.1955861287286,12.));
#171157=CARTESIAN_POINT('Ctrl Pts',(67.8734191723667,23.1953823877734,12.));
#171158=CARTESIAN_POINT('Ctrl Pts',(67.8969445011916,23.1951550520802,12.));
#171159=CARTESIAN_POINT('Ctrl Pts',(67.9205130070324,23.1949040591744,12.));
#171160=CARTESIAN_POINT('Ctrl Pts',(67.9441245641842,23.1946293469427,12.));
#171161=CARTESIAN_POINT('Ctrl Pts',(67.9677790474385,23.1943308536297,12.));
#171162=CARTESIAN_POINT('Ctrl Pts',(67.991476332086,23.1940085178313,12.));
#171163=CARTESIAN_POINT('Ctrl Pts',(68.0152162939121,23.1936622784919,12.));
#171164=CARTESIAN_POINT('Ctrl Pts',(68.0389988091933,23.1932920749023,12.));
#171165=CARTESIAN_POINT('Ctrl Pts',(68.0628237546863,23.1928978467021,12.));
#171166=CARTESIAN_POINT('Ctrl Pts',(68.0866910076251,23.1924795338749,12.));
#171167=CARTESIAN_POINT('Ctrl Pts',(68.110600445723,23.1920370767426,12.));
#171168=CARTESIAN_POINT('Ctrl Pts',(68.1345519471695,23.1915704159623,12.));
#171169=CARTESIAN_POINT('Ctrl Pts',(68.1585453906257,23.1910794925251,12.));
#171170=CARTESIAN_POINT('Ctrl Pts',(68.1825806552129,23.1905642477571,12.));
#171171=CARTESIAN_POINT('Ctrl Pts',(68.2066576205116,23.1900246233165,12.));
#171172=CARTESIAN_POINT('Ctrl Pts',(68.2307761665633,23.1894605611871,12.));
#171173=CARTESIAN_POINT('Ctrl Pts',(68.2549361738681,23.1888720036757,12.));
#171174=CARTESIAN_POINT('Ctrl Pts',(68.2791375233795,23.1882588934107,12.));
#171175=CARTESIAN_POINT('Ctrl Pts',(68.3033800964939,23.1876211733436,12.));
#171176=CARTESIAN_POINT('Ctrl Pts',(68.3276637750485,23.1869587867459,12.));
#171177=CARTESIAN_POINT('Ctrl Pts',(68.3519884413246,23.1862716772031,12.));
#171178=CARTESIAN_POINT('Ctrl Pts',(68.376353978044,23.1855597886116,12.));
#171179=CARTESIAN_POINT('Ctrl Pts',(68.4007602683652,23.1848230651776,12.));
#171180=CARTESIAN_POINT('Ctrl Pts',(68.4252071958729,23.1840614514192,12.));
#171181=CARTESIAN_POINT('Ctrl Pts',(68.4496946445758,23.183274892163,12.));
#171182=CARTESIAN_POINT('Ctrl Pts',(68.4742224989098,23.1824633325385,12.));
#171183=CARTESIAN_POINT('Ctrl Pts',(68.4987906437356,23.1816267179751,12.));
#171184=CARTESIAN_POINT('Ctrl Pts',(68.5233989643345,23.180764994201,12.));
#171185=CARTESIAN_POINT('Ctrl Pts',(68.5480473463985,23.179878107245,12.));
#171186=CARTESIAN_POINT('Ctrl Pts',(68.5727356760278,23.1789660034342,12.));
#171187=CARTESIAN_POINT('Ctrl Pts',(68.597463839733,23.1780286293875,12.));
#171188=CARTESIAN_POINT('Ctrl Pts',(68.6222317244341,23.1770659320138,12.));
#171189=CARTESIAN_POINT('Ctrl Pts',(68.6470392174564,23.1760778585092,12.));
#171190=CARTESIAN_POINT('Ctrl Pts',(68.6718862065216,23.1750643563602,12.));
#171191=CARTESIAN_POINT('Ctrl Pts',(68.696772579744,23.1740253733417,12.));
#171192=CARTESIAN_POINT('Ctrl Pts',(68.7216982256341,23.172960857511,12.));
#171193=CARTESIAN_POINT('Ctrl Pts',(68.746663033096,23.1718707572043,12.));
#171194=CARTESIAN_POINT('Ctrl Pts',(68.771666891425,23.170755021036,12.));
#171195=CARTESIAN_POINT('Ctrl Pts',(68.7967096902996,23.1696135978997,12.));
#171196=CARTESIAN_POINT('Ctrl Pts',(68.8217913197752,23.1684464369686,12.));
#171197=CARTESIAN_POINT('Ctrl Pts',(68.8469116702898,23.1672534876889,12.));
#171198=CARTESIAN_POINT('Ctrl Pts',(68.8720706326609,23.1660346997764,12.));
#171199=CARTESIAN_POINT('Ctrl Pts',(68.8972680980842,23.164790023215,12.));
#171200=CARTESIAN_POINT('Ctrl Pts',(68.9225039581248,23.1635194082581,12.));
#171201=CARTESIAN_POINT('Ctrl Pts',(68.9477781047106,23.1622228054291,12.));
#171202=CARTESIAN_POINT('Ctrl Pts',(68.9730904301369,23.1609001655156,12.));
#171203=CARTESIAN_POINT('Ctrl Pts',(68.9984408270659,23.1595514395656,12.));
#171204=CARTESIAN_POINT('Ctrl Pts',(69.0238291885245,23.1581765788869,12.));
#171205=CARTESIAN_POINT('Ctrl Pts',(69.0492554078992,23.1567755350469,12.));
#171206=CARTESIAN_POINT('Ctrl Pts',(69.074719378928,23.1553482598762,12.));
#171207=CARTESIAN_POINT('Ctrl Pts',(69.1002209957025,23.1538947054615,12.));
#171208=CARTESIAN_POINT('Ctrl Pts',(69.1257601526687,23.152414824141,12.));
#171209=CARTESIAN_POINT('Ctrl Pts',(69.1513367446231,23.1509085685032,12.));
#171210=CARTESIAN_POINT('Ctrl Pts',(69.1769506667084,23.1493758913859,12.));
#171211=CARTESIAN_POINT('Ctrl Pts',(69.2026018144028,23.147816745879,12.));
#171212=CARTESIAN_POINT('Ctrl Pts',(69.2282900835235,23.1462310853206,12.));
#171213=CARTESIAN_POINT('Ctrl Pts',(69.254015370231,23.1446188632931,12.));
#171214=CARTESIAN_POINT('Ctrl Pts',(69.2797775710273,23.142980033622,12.));
#171215=CARTESIAN_POINT('Ctrl Pts',(69.3055765827546,23.1413145503762,12.));
#171216=CARTESIAN_POINT('Ctrl Pts',(69.3314123025869,23.1396223678725,12.));
#171217=CARTESIAN_POINT('Ctrl Pts',(69.3572846280297,23.1379034406718,12.));
#171218=CARTESIAN_POINT('Ctrl Pts',(69.3831934569182,23.1361577235709,12.));
#171219=CARTESIAN_POINT('Ctrl Pts',(69.4091386874132,23.1343851715989,12.));
#171220=CARTESIAN_POINT('Ctrl Pts',(69.4351202179946,23.1325857400144,12.));
#171221=CARTESIAN_POINT('Ctrl Pts',(69.4611379474484,23.1307593843061,12.));
#171222=CARTESIAN_POINT('Ctrl Pts',(69.4871917748654,23.1289060601924,12.));
#171223=CARTESIAN_POINT('Ctrl Pts',(69.5132815996537,23.1270257236204,12.));
#171224=CARTESIAN_POINT('Ctrl Pts',(69.539407321546,23.1251183307676,12.));
#171225=CARTESIAN_POINT('Ctrl Pts',(69.5655688406052,23.1231838380452,12.));
#171226=CARTESIAN_POINT('Ctrl Pts',(69.5917660572265,23.1212222021051,12.));
#171227=CARTESIAN_POINT('Ctrl Pts',(69.6179988721365,23.1192333798441,12.));
#171228=CARTESIAN_POINT('Ctrl Pts',(69.6442671863765,23.1172173283859,12.));
#171229=CARTESIAN_POINT('Ctrl Pts',(69.6705709012852,23.1151740050681,12.));
#171230=CARTESIAN_POINT('Ctrl Pts',(69.6969099184767,23.1131033674301,12.));
#171231=CARTESIAN_POINT('Ctrl Pts',(69.7232841398197,23.1110053732046,12.));
#171232=CARTESIAN_POINT('Ctrl Pts',(69.7496934674069,23.1088799803089,12.));
#171233=CARTESIAN_POINT('Ctrl Pts',(69.7761378035964,23.106727146861,12.));
#171234=CARTESIAN_POINT('Ctrl Pts',(69.8026170510572,23.1045468311991,12.));
#171235=CARTESIAN_POINT('Ctrl Pts',(69.8291311128118,23.1023389919051,12.));
#171236=CARTESIAN_POINT('Ctrl Pts',(69.8556798922693,23.1001035878241,12.));
#171237=CARTESIAN_POINT('Ctrl Pts',(69.8822632932768,23.0978405781021,12.));
#171238=CARTESIAN_POINT('Ctrl Pts',(69.9088812200713,23.0955499221558,12.));
#171239=CARTESIAN_POINT('Ctrl Pts',(69.9355335771729,23.0932315796068,12.));
#171240=CARTESIAN_POINT('Ctrl Pts',(69.9622202692873,23.0908855102251,12.));
#171241=CARTESIAN_POINT('Ctrl Pts',(69.9889412012143,23.0885116738798,12.));
#171242=CARTESIAN_POINT('Ctrl Pts',(70.0156962777169,23.0861100304729,12.));
#171243=CARTESIAN_POINT('Ctrl Pts',(70.0424854035115,23.0836805399374,12.));
#171244=CARTESIAN_POINT('Ctrl Pts',(70.0693084835373,23.0812231623765,12.));
#171245=CARTESIAN_POINT('Ctrl Pts',(70.0961654231639,23.0787378581774,12.));
#171246=CARTESIAN_POINT('Ctrl Pts',(70.123056128422,23.0762245881389,12.));
#171247=CARTESIAN_POINT('Ctrl Pts',(70.1499805062172,23.0736833135938,12.));
#171248=CARTESIAN_POINT('Ctrl Pts',(70.1769384645586,23.071113996544,12.));
#171249=CARTESIAN_POINT('Ctrl Pts',(70.2039299120488,23.0685165993691,12.));
#171250=CARTESIAN_POINT('Ctrl Pts',(70.2309547573815,23.0658910845433,12.));
#171251=CARTESIAN_POINT('Ctrl Pts',(70.2580129087888,23.0632374143279,12.));
#171252=CARTESIAN_POINT('Ctrl Pts',(70.2851042736066,23.0605555505321,12.));
#171253=CARTESIAN_POINT('Ctrl Pts',(70.3122287575335,23.0578454541104,12.));
#171254=CARTESIAN_POINT('Ctrl Pts',(70.3393862652297,23.0551070854926,12.));
#171255=CARTESIAN_POINT('Ctrl Pts',(70.3665767016542,23.0523404053172,12.));
#171256=CARTESIAN_POINT('Ctrl Pts',(70.3937999732267,23.0495453750763,12.));
#171257=CARTESIAN_POINT('Ctrl Pts',(70.4210559889348,23.0467219577291,12.));
#171258=CARTESIAN_POINT('Ctrl Pts',(70.4483446617614,23.0438701185013,12.));
#171259=CARTESIAN_POINT('Ctrl Pts',(70.4756659090209,23.0409898250756,12.));
#171260=CARTESIAN_POINT('Ctrl Pts',(70.4991133648947,23.0384964376036,12.));
#171261=CARTESIAN_POINT('Ctrl Pts',(70.5171075702746,23.0365694096173,12.));
#171262=CARTESIAN_POINT('Ctrl Pts',(70.5296341535556,23.0352213647764,12.));
#171263=CARTESIAN_POINT('Ctrl Pts',(70.5366836381661,23.0344606623299,12.));
#171264=CARTESIAN_POINT('Ctrl Pts',(70.538251407892,23.0342913834073,12.));
#171265=CARTESIAN_POINT('',(66.0656156664138,23.1372951448024,0.));
#171266=CARTESIAN_POINT('',(66.0656156664138,23.1372951448024,0.));
#171267=CARTESIAN_POINT('Ctrl Pts',(70.538251407892,23.0342913834073,0.));
#171268=CARTESIAN_POINT('Ctrl Pts',(70.5366836381661,23.0344606623299,0.));
#171269=CARTESIAN_POINT('Ctrl Pts',(70.5296341535556,23.0352213647764,0.));
#171270=CARTESIAN_POINT('Ctrl Pts',(70.5171075702746,23.0365694096173,0.));
#171271=CARTESIAN_POINT('Ctrl Pts',(70.4991133648947,23.0384964376036,0.));
#171272=CARTESIAN_POINT('Ctrl Pts',(70.4756659090209,23.0409898250756,0.));
#171273=CARTESIAN_POINT('Ctrl Pts',(70.4483446617614,23.0438701185013,0.));
#171274=CARTESIAN_POINT('Ctrl Pts',(70.4210559889348,23.0467219577291,0.));
#171275=CARTESIAN_POINT('Ctrl Pts',(70.3937999732267,23.0495453750763,0.));
#171276=CARTESIAN_POINT('Ctrl Pts',(70.3665767016542,23.0523404053172,0.));
#171277=CARTESIAN_POINT('Ctrl Pts',(70.3393862652297,23.0551070854926,0.));
#171278=CARTESIAN_POINT('Ctrl Pts',(70.3122287575335,23.0578454541104,0.));
#171279=CARTESIAN_POINT('Ctrl Pts',(70.2851042736066,23.0605555505321,0.));
#171280=CARTESIAN_POINT('Ctrl Pts',(70.2580129087888,23.0632374143279,0.));
#171281=CARTESIAN_POINT('Ctrl Pts',(70.2309547573815,23.0658910845433,0.));
#171282=CARTESIAN_POINT('Ctrl Pts',(70.2039299120488,23.0685165993691,0.));
#171283=CARTESIAN_POINT('Ctrl Pts',(70.1769384645586,23.071113996544,0.));
#171284=CARTESIAN_POINT('Ctrl Pts',(70.1499805062172,23.0736833135938,0.));
#171285=CARTESIAN_POINT('Ctrl Pts',(70.123056128422,23.0762245881389,0.));
#171286=CARTESIAN_POINT('Ctrl Pts',(70.0961654231639,23.0787378581774,0.));
#171287=CARTESIAN_POINT('Ctrl Pts',(70.0693084835373,23.0812231623765,0.));
#171288=CARTESIAN_POINT('Ctrl Pts',(70.0424854035115,23.0836805399374,0.));
#171289=CARTESIAN_POINT('Ctrl Pts',(70.0156962777169,23.0861100304729,0.));
#171290=CARTESIAN_POINT('Ctrl Pts',(69.9889412012143,23.0885116738798,0.));
#171291=CARTESIAN_POINT('Ctrl Pts',(69.9622202692873,23.0908855102251,0.));
#171292=CARTESIAN_POINT('Ctrl Pts',(69.9355335771729,23.0932315796068,0.));
#171293=CARTESIAN_POINT('Ctrl Pts',(69.9088812200713,23.0955499221558,0.));
#171294=CARTESIAN_POINT('Ctrl Pts',(69.8822632932768,23.0978405781021,0.));
#171295=CARTESIAN_POINT('Ctrl Pts',(69.8556798922693,23.1001035878241,0.));
#171296=CARTESIAN_POINT('Ctrl Pts',(69.8291311128118,23.1023389919051,0.));
#171297=CARTESIAN_POINT('Ctrl Pts',(69.8026170510572,23.1045468311991,0.));
#171298=CARTESIAN_POINT('Ctrl Pts',(69.7761378035964,23.106727146861,0.));
#171299=CARTESIAN_POINT('Ctrl Pts',(69.7496934674069,23.1088799803089,0.));
#171300=CARTESIAN_POINT('Ctrl Pts',(69.7232841398197,23.1110053732046,0.));
#171301=CARTESIAN_POINT('Ctrl Pts',(69.6969099184767,23.1131033674301,0.));
#171302=CARTESIAN_POINT('Ctrl Pts',(69.6705709012852,23.1151740050681,0.));
#171303=CARTESIAN_POINT('Ctrl Pts',(69.6442671863765,23.1172173283859,0.));
#171304=CARTESIAN_POINT('Ctrl Pts',(69.6179988721365,23.1192333798441,0.));
#171305=CARTESIAN_POINT('Ctrl Pts',(69.5917660572265,23.1212222021051,0.));
#171306=CARTESIAN_POINT('Ctrl Pts',(69.5655688406052,23.1231838380452,0.));
#171307=CARTESIAN_POINT('Ctrl Pts',(69.539407321546,23.1251183307676,0.));
#171308=CARTESIAN_POINT('Ctrl Pts',(69.5132815996537,23.1270257236204,0.));
#171309=CARTESIAN_POINT('Ctrl Pts',(69.4871917748654,23.1289060601924,0.));
#171310=CARTESIAN_POINT('Ctrl Pts',(69.4611379474484,23.1307593843061,0.));
#171311=CARTESIAN_POINT('Ctrl Pts',(69.4351202179946,23.1325857400144,0.));
#171312=CARTESIAN_POINT('Ctrl Pts',(69.4091386874132,23.1343851715989,0.));
#171313=CARTESIAN_POINT('Ctrl Pts',(69.3831934569182,23.1361577235709,0.));
#171314=CARTESIAN_POINT('Ctrl Pts',(69.3572846280297,23.1379034406718,0.));
#171315=CARTESIAN_POINT('Ctrl Pts',(69.3314123025869,23.1396223678725,0.));
#171316=CARTESIAN_POINT('Ctrl Pts',(69.3055765827546,23.1413145503762,0.));
#171317=CARTESIAN_POINT('Ctrl Pts',(69.2797775710273,23.142980033622,0.));
#171318=CARTESIAN_POINT('Ctrl Pts',(69.254015370231,23.1446188632931,0.));
#171319=CARTESIAN_POINT('Ctrl Pts',(69.2282900835235,23.1462310853206,0.));
#171320=CARTESIAN_POINT('Ctrl Pts',(69.2026018144028,23.147816745879,0.));
#171321=CARTESIAN_POINT('Ctrl Pts',(69.1769506667084,23.1493758913859,0.));
#171322=CARTESIAN_POINT('Ctrl Pts',(69.1513367446231,23.1509085685032,0.));
#171323=CARTESIAN_POINT('Ctrl Pts',(69.1257601526687,23.152414824141,0.));
#171324=CARTESIAN_POINT('Ctrl Pts',(69.1002209957025,23.1538947054615,0.));
#171325=CARTESIAN_POINT('Ctrl Pts',(69.074719378928,23.1553482598762,0.));
#171326=CARTESIAN_POINT('Ctrl Pts',(69.0492554078992,23.1567755350469,0.));
#171327=CARTESIAN_POINT('Ctrl Pts',(69.0238291885245,23.1581765788869,0.));
#171328=CARTESIAN_POINT('Ctrl Pts',(68.9984408270659,23.1595514395656,0.));
#171329=CARTESIAN_POINT('Ctrl Pts',(68.9730904301369,23.1609001655156,0.));
#171330=CARTESIAN_POINT('Ctrl Pts',(68.9477781047106,23.1622228054291,0.));
#171331=CARTESIAN_POINT('Ctrl Pts',(68.9225039581248,23.1635194082581,0.));
#171332=CARTESIAN_POINT('Ctrl Pts',(68.8972680980842,23.164790023215,0.));
#171333=CARTESIAN_POINT('Ctrl Pts',(68.8720706326609,23.1660346997764,0.));
#171334=CARTESIAN_POINT('Ctrl Pts',(68.8469116702898,23.1672534876889,0.));
#171335=CARTESIAN_POINT('Ctrl Pts',(68.8217913197752,23.1684464369686,0.));
#171336=CARTESIAN_POINT('Ctrl Pts',(68.7967096902996,23.1696135978997,0.));
#171337=CARTESIAN_POINT('Ctrl Pts',(68.771666891425,23.170755021036,0.));
#171338=CARTESIAN_POINT('Ctrl Pts',(68.746663033096,23.1718707572043,0.));
#171339=CARTESIAN_POINT('Ctrl Pts',(68.7216982256341,23.172960857511,0.));
#171340=CARTESIAN_POINT('Ctrl Pts',(68.696772579744,23.1740253733417,0.));
#171341=CARTESIAN_POINT('Ctrl Pts',(68.6718862065216,23.1750643563602,0.));
#171342=CARTESIAN_POINT('Ctrl Pts',(68.6470392174564,23.1760778585092,0.));
#171343=CARTESIAN_POINT('Ctrl Pts',(68.6222317244341,23.1770659320138,0.));
#171344=CARTESIAN_POINT('Ctrl Pts',(68.597463839733,23.1780286293875,0.));
#171345=CARTESIAN_POINT('Ctrl Pts',(68.5727356760278,23.1789660034342,0.));
#171346=CARTESIAN_POINT('Ctrl Pts',(68.5480473463985,23.179878107245,0.));
#171347=CARTESIAN_POINT('Ctrl Pts',(68.5233989643345,23.180764994201,0.));
#171348=CARTESIAN_POINT('Ctrl Pts',(68.4987906437356,23.1816267179751,0.));
#171349=CARTESIAN_POINT('Ctrl Pts',(68.4742224989098,23.1824633325385,0.));
#171350=CARTESIAN_POINT('Ctrl Pts',(68.4496946445758,23.183274892163,0.));
#171351=CARTESIAN_POINT('Ctrl Pts',(68.4252071958729,23.1840614514192,0.));
#171352=CARTESIAN_POINT('Ctrl Pts',(68.4007602683652,23.1848230651776,0.));
#171353=CARTESIAN_POINT('Ctrl Pts',(68.376353978044,23.1855597886116,0.));
#171354=CARTESIAN_POINT('Ctrl Pts',(68.3519884413246,23.1862716772031,0.));
#171355=CARTESIAN_POINT('Ctrl Pts',(68.3276637750485,23.1869587867459,0.));
#171356=CARTESIAN_POINT('Ctrl Pts',(68.3033800964939,23.1876211733436,0.));
#171357=CARTESIAN_POINT('Ctrl Pts',(68.2791375233795,23.1882588934107,0.));
#171358=CARTESIAN_POINT('Ctrl Pts',(68.2549361738681,23.1888720036757,0.));
#171359=CARTESIAN_POINT('Ctrl Pts',(68.2307761665633,23.1894605611871,0.));
#171360=CARTESIAN_POINT('Ctrl Pts',(68.2066576205116,23.1900246233165,0.));
#171361=CARTESIAN_POINT('Ctrl Pts',(68.1825806552129,23.1905642477571,0.));
#171362=CARTESIAN_POINT('Ctrl Pts',(68.1585453906257,23.1910794925251,0.));
#171363=CARTESIAN_POINT('Ctrl Pts',(68.1345519471695,23.1915704159623,0.));
#171364=CARTESIAN_POINT('Ctrl Pts',(68.110600445723,23.1920370767426,0.));
#171365=CARTESIAN_POINT('Ctrl Pts',(68.0866910076251,23.1924795338749,0.));
#171366=CARTESIAN_POINT('Ctrl Pts',(68.0628237546863,23.1928978467021,0.));
#171367=CARTESIAN_POINT('Ctrl Pts',(68.0389988091933,23.1932920749023,0.));
#171368=CARTESIAN_POINT('Ctrl Pts',(68.0152162939121,23.1936622784919,0.));
#171369=CARTESIAN_POINT('Ctrl Pts',(67.991476332086,23.1940085178313,0.));
#171370=CARTESIAN_POINT('Ctrl Pts',(67.9677790474385,23.1943308536297,0.));
#171371=CARTESIAN_POINT('Ctrl Pts',(67.9441245641842,23.1946293469427,0.));
#171372=CARTESIAN_POINT('Ctrl Pts',(67.9205130070324,23.1949040591744,0.));
#171373=CARTESIAN_POINT('Ctrl Pts',(67.8969445011916,23.1951550520802,0.));
#171374=CARTESIAN_POINT('Ctrl Pts',(67.8734191723667,23.1953823877734,0.));
#171375=CARTESIAN_POINT('Ctrl Pts',(67.8499371467616,23.1955861287286,0.));
#171376=CARTESIAN_POINT('Ctrl Pts',(67.8264985510917,23.1957663377806,0.));
#171377=CARTESIAN_POINT('Ctrl Pts',(67.8031035125887,23.1959230781269,0.));
#171378=CARTESIAN_POINT('Ctrl Pts',(67.7797521590045,23.1960564133304,0.));
#171379=CARTESIAN_POINT('Ctrl Pts',(67.7564446186079,23.1961664073262,0.));
#171380=CARTESIAN_POINT('Ctrl Pts',(67.7331810201883,23.1962531244245,0.));
#171381=CARTESIAN_POINT('Ctrl Pts',(67.7099614930671,23.1963166293102,0.));
#171382=CARTESIAN_POINT('Ctrl Pts',(67.6867861671031,23.1963569870451,0.));
#171383=CARTESIAN_POINT('Ctrl Pts',(67.6636551726964,23.1963742630715,0.));
#171384=CARTESIAN_POINT('Ctrl Pts',(67.6405686407863,23.1963685232188,0.));
#171385=CARTESIAN_POINT('Ctrl Pts',(67.6175267028555,23.1963398337069,0.));
#171386=CARTESIAN_POINT('Ctrl Pts',(67.5945294909426,23.1962882611453,0.));
#171387=CARTESIAN_POINT('Ctrl Pts',(67.5715771376461,23.196213872536,0.));
#171388=CARTESIAN_POINT('Ctrl Pts',(67.5486697761288,23.1961167352772,0.));
#171389=CARTESIAN_POINT('Ctrl Pts',(67.5258075401146,23.1959969171701,0.));
#171390=CARTESIAN_POINT('Ctrl Pts',(67.5029905638949,23.1958544864215,0.));
#171391=CARTESIAN_POINT('Ctrl Pts',(67.4802189823408,23.195689511644,0.));
#171392=CARTESIAN_POINT('Ctrl Pts',(67.4574929309076,23.195502061859,0.));
#171393=CARTESIAN_POINT('Ctrl Pts',(67.4348125456398,23.1952922065012,0.));
#171394=CARTESIAN_POINT('Ctrl Pts',(67.412177963168,23.1950600154265,0.));
#171395=CARTESIAN_POINT('Ctrl Pts',(67.3895893207182,23.1948055589129,0.));
#171396=CARTESIAN_POINT('Ctrl Pts',(67.3670467561212,23.194528907661,0.));
#171397=CARTESIAN_POINT('Ctrl Pts',(67.3445504078176,23.1942301327978,0.));
#171398=CARTESIAN_POINT('Ctrl Pts',(67.3221004148603,23.1939093058801,0.));
#171399=CARTESIAN_POINT('Ctrl Pts',(67.2996969169098,23.1935664989018,0.));
#171400=CARTESIAN_POINT('Ctrl Pts',(67.2773400542477,23.1932017842953,0.));
#171401=CARTESIAN_POINT('Ctrl Pts',(67.2550299677888,23.1928152349343,0.));
#171402=CARTESIAN_POINT('Ctrl Pts',(67.232766799088,23.1924069241385,0.));
#171403=CARTESIAN_POINT('Ctrl Pts',(67.2105506903447,23.1919769256803,0.));
#171404=CARTESIAN_POINT('Ctrl Pts',(67.1883817844038,23.1915253137924,0.));
#171405=CARTESIAN_POINT('Ctrl Pts',(67.1662602247639,23.1910521631657,0.));
#171406=CARTESIAN_POINT('Ctrl Pts',(67.1441861555817,23.1905575489505,0.));
#171407=CARTESIAN_POINT('Ctrl Pts',(67.1221597216741,23.1900415467574,0.));
#171408=CARTESIAN_POINT('Ctrl Pts',(67.1001810685143,23.1895042326627,0.));
#171409=CARTESIAN_POINT('Ctrl Pts',(67.0782503422305,23.1889456832119,0.));
#171410=CARTESIAN_POINT('Ctrl Pts',(67.0563676896325,23.1883659754271,0.));
#171411=CARTESIAN_POINT('Ctrl Pts',(67.0345332582306,23.1877651868158,0.));
#171412=CARTESIAN_POINT('Ctrl Pts',(67.0127471962501,23.1871433953793,0.));
#171413=CARTESIAN_POINT('Ctrl Pts',(66.9910096526462,23.1865006796283,0.));
#171414=CARTESIAN_POINT('Ctrl Pts',(66.9693207771031,23.1858371185842,0.));
#171415=CARTESIAN_POINT('Ctrl Pts',(66.9476807200203,23.1851527917657,0.));
#171416=CARTESIAN_POINT('Ctrl Pts',(66.9260896324949,23.1844477791814,0.));
#171417=CARTESIAN_POINT('Ctrl Pts',(66.9045476663063,23.1837221613235,0.));
#171418=CARTESIAN_POINT('Ctrl Pts',(66.8830549738795,23.1829760191591,0.));
#171419=CARTESIAN_POINT('Ctrl Pts',(66.8616117083331,23.1822094341517,0.));
#171420=CARTESIAN_POINT('Ctrl Pts',(66.8402180235566,23.1814224882953,0.));
#171421=CARTESIAN_POINT('Ctrl Pts',(66.8188740742727,23.1806152641475,0.));
#171422=CARTESIAN_POINT('Ctrl Pts',(66.7975800161,23.1797878448639,0.));
#171423=CARTESIAN_POINT('Ctrl Pts',(66.776336005612,23.1789403142366,0.));
#171424=CARTESIAN_POINT('Ctrl Pts',(66.7551422002204,23.17807275663,0.));
#171425=CARTESIAN_POINT('Ctrl Pts',(66.7339987580427,23.1771852569131,0.));
#171426=CARTESIAN_POINT('Ctrl Pts',(66.7129058377896,23.1762779004044,0.));
#171427=CARTESIAN_POINT('Ctrl Pts',(66.6918635985972,23.1753507727939,0.));
#171428=CARTESIAN_POINT('Ctrl Pts',(66.6708722000079,23.1744039601382,0.));
#171429=CARTESIAN_POINT('Ctrl Pts',(66.6499318023473,23.1734375490431,0.));
#171430=CARTESIAN_POINT('Ctrl Pts',(66.6290425670548,23.1724516268302,0.));
#171431=CARTESIAN_POINT('Ctrl Pts',(66.6082046569644,23.1714462816789,0.));
#171432=CARTESIAN_POINT('Ctrl Pts',(66.5874182367563,23.1704216028614,0.));
#171433=CARTESIAN_POINT('Ctrl Pts',(66.5666834726454,23.1693776805866,0.));
#171434=CARTESIAN_POINT('Ctrl Pts',(66.5460005315376,23.1683146055726,0.));
#171435=CARTESIAN_POINT('Ctrl Pts',(66.5253695803205,23.1672324686926,0.));
#171436=CARTESIAN_POINT('Ctrl Pts',(66.5047907851348,23.1661313606132,0.));
#171437=CARTESIAN_POINT('Ctrl Pts',(66.4842643105311,23.1650113713808,0.));
#171438=CARTESIAN_POINT('Ctrl Pts',(66.4637903210727,23.1638725912195,0.));
#171439=CARTESIAN_POINT('Ctrl Pts',(66.4433689832478,23.1627151114883,0.));
#171440=CARTESIAN_POINT('Ctrl Pts',(66.4230004670278,23.1615390254632,0.));
#171441=CARTESIAN_POINT('Ctrl Pts',(66.4026849481232,23.160344429474,0.));
#171442=CARTESIAN_POINT('Ctrl Pts',(66.3824226081801,23.1591314230083,0.));
#171443=CARTESIAN_POINT('Ctrl Pts',(66.3622136300654,23.1579001063424,0.));
#171444=CARTESIAN_POINT('Ctrl Pts',(66.3420581937147,23.1566505784621,0.));
#171445=CARTESIAN_POINT('Ctrl Pts',(66.3219564725184,23.1553829352539,0.));
#171446=CARTESIAN_POINT('Ctrl Pts',(66.3019086275444,23.1540972666191,0.));
#171447=CARTESIAN_POINT('Ctrl Pts',(66.281914813114,23.1527936592651,0.));
#171448=CARTESIAN_POINT('Ctrl Pts',(66.2619751878793,23.1514722022503,0.));
#171449=CARTESIAN_POINT('Ctrl Pts',(66.2420899237318,23.1501329914488,0.));
#171450=CARTESIAN_POINT('Ctrl Pts',(66.2222592165398,23.1487761349298,0.));
#171451=CARTESIAN_POINT('Ctrl Pts',(66.2024832934733,23.147401756643,0.));
#171452=CARTESIAN_POINT('Ctrl Pts',(66.1827623902755,23.1460099850704,0.));
#171453=CARTESIAN_POINT('Ctrl Pts',(66.163096729667,23.1446009424871,0.));
#171454=CARTESIAN_POINT('Ctrl Pts',(66.14348650151,23.1431747350127,0.));
#171455=CARTESIAN_POINT('Ctrl Pts',(66.1239318368803,23.1417314398501,0.));
#171456=CARTESIAN_POINT('Ctrl Pts',(66.1044328067739,23.140271103958,0.));
#171457=CARTESIAN_POINT('Ctrl Pts',(66.0888781152779,23.1390892229923,0.));
#171458=CARTESIAN_POINT('Ctrl Pts',(66.0772371487475,23.1381951597491,0.));
#171459=CARTESIAN_POINT('Ctrl Pts',(66.0694876382212,23.1375957166138,0.));
#171460=CARTESIAN_POINT('Ctrl Pts',(66.0656156664138,23.1372951448024,0.));
#171461=CARTESIAN_POINT('Ctrl Pts',(72.5962692526112,16.7341474417544,0.));
#171462=CARTESIAN_POINT('Ctrl Pts',(72.5962692526112,16.7341474417544,12.));
#171463=CARTESIAN_POINT('Ctrl Pts',(72.5907910746008,16.7352885767485,0.));
#171464=CARTESIAN_POINT('Ctrl Pts',(72.5907910746008,16.7352885767485,12.));
#171465=CARTESIAN_POINT('Ctrl Pts',(72.5798376087774,16.7375676985344,0.));
#171466=CARTESIAN_POINT('Ctrl Pts',(72.5798376087774,16.7375676985344,12.));
#171467=CARTESIAN_POINT('Ctrl Pts',(72.5634160806351,16.7409769366072,0.));
#171468=CARTESIAN_POINT('Ctrl Pts',(72.5634160806351,16.7409769366072,12.));
#171469=CARTESIAN_POINT('Ctrl Pts',(72.5415380516637,16.7455036973866,0.));
#171470=CARTESIAN_POINT('Ctrl Pts',(72.5415380516637,16.7455036973866,12.));
#171471=CARTESIAN_POINT('Ctrl Pts',(72.514219427383,16.7511306618915,0.));
#171472=CARTESIAN_POINT('Ctrl Pts',(72.514219427383,16.7511306618915,12.));
#171473=CARTESIAN_POINT('Ctrl Pts',(72.4869297342427,16.7567261380687,0.));
#171474=CARTESIAN_POINT('Ctrl Pts',(72.4869297342427,16.7567261380687,12.));
#171475=CARTESIAN_POINT('Ctrl Pts',(72.4596690055437,16.7622901280758,0.));
#171476=CARTESIAN_POINT('Ctrl Pts',(72.4596690055437,16.7622901280758,12.));
#171477=CARTESIAN_POINT('Ctrl Pts',(72.4324372916746,16.7678226404162,0.));
#171478=CARTESIAN_POINT('Ctrl Pts',(72.4324372916746,16.7678226404162,12.));
#171479=CARTESIAN_POINT('Ctrl Pts',(72.4052346647799,16.7733236932135,0.));
#171480=CARTESIAN_POINT('Ctrl Pts',(72.4052346647799,16.7733236932135,12.));
#171481=CARTESIAN_POINT('Ctrl Pts',(72.3780612167786,16.7787933137498,0.));
#171482=CARTESIAN_POINT('Ctrl Pts',(72.3780612167786,16.7787933137498,12.));
#171483=CARTESIAN_POINT('Ctrl Pts',(72.3509170522838,16.7842315351363,0.));
#171484=CARTESIAN_POINT('Ctrl Pts',(72.3509170522838,16.7842315351363,12.));
#171485=CARTESIAN_POINT('Ctrl Pts',(72.3238022829223,16.7896383937822,0.));
#171486=CARTESIAN_POINT('Ctrl Pts',(72.3238022829223,16.7896383937822,12.));
#171487=CARTESIAN_POINT('Ctrl Pts',(72.2967170212353,16.7950139266122,0.));
#171488=CARTESIAN_POINT('Ctrl Pts',(72.2967170212353,16.7950139266122,12.));
#171489=CARTESIAN_POINT('Ctrl Pts',(72.2696613743782,16.8003581682248,0.));
#171490=CARTESIAN_POINT('Ctrl Pts',(72.2696613743782,16.8003581682248,12.));
#171491=CARTESIAN_POINT('Ctrl Pts',(72.2426354390213,16.8056711485821,0.));
#171492=CARTESIAN_POINT('Ctrl Pts',(72.2426354390213,16.8056711485821,12.));
#171493=CARTESIAN_POINT('Ctrl Pts',(72.2156393048975,16.8109528945896,0.));
#171494=CARTESIAN_POINT('Ctrl Pts',(72.2156393048975,16.8109528945896,12.));
#171495=CARTESIAN_POINT('Ctrl Pts',(72.1886730573452,16.8162034312269,0.));
#171496=CARTESIAN_POINT('Ctrl Pts',(72.1886730573452,16.8162034312269,12.));
#171497=CARTESIAN_POINT('Ctrl Pts',(72.1617367803235,16.8214227828943,0.));
#171498=CARTESIAN_POINT('Ctrl Pts',(72.1617367803235,16.8214227828943,12.));
#171499=CARTESIAN_POINT('Ctrl Pts',(72.13483055902,16.8266109745795,0.));
#171500=CARTESIAN_POINT('Ctrl Pts',(72.13483055902,16.8266109745795,12.));
#171501=CARTESIAN_POINT('Ctrl Pts',(72.1079544831513,16.8317680333404,0.));
#171502=CARTESIAN_POINT('Ctrl Pts',(72.1079544831513,16.8317680333404,12.));
#171503=CARTESIAN_POINT('Ctrl Pts',(72.0811086466121,16.8368939881446,0.));
#171504=CARTESIAN_POINT('Ctrl Pts',(72.0811086466121,16.8368939881446,12.));
#171505=CARTESIAN_POINT('Ctrl Pts',(72.0542931459825,16.8419888691976,0.));
#171506=CARTESIAN_POINT('Ctrl Pts',(72.0542931459825,16.8419888691976,12.));
#171507=CARTESIAN_POINT('Ctrl Pts',(72.0275080793727,16.8470527074275,0.));
#171508=CARTESIAN_POINT('Ctrl Pts',(72.0275080793727,16.8470527074275,12.));
#171509=CARTESIAN_POINT('Ctrl Pts',(72.0007535452081,16.8520855339446,0.));
#171510=CARTESIAN_POINT('Ctrl Pts',(72.0007535452081,16.8520855339446,12.));
#171511=CARTESIAN_POINT('Ctrl Pts',(71.9740296408347,16.8570873794269,0.));
#171512=CARTESIAN_POINT('Ctrl Pts',(71.9740296408347,16.8570873794269,12.));
#171513=CARTESIAN_POINT('Ctrl Pts',(71.9473364618922,16.8620582738437,0.));
#171514=CARTESIAN_POINT('Ctrl Pts',(71.9473364618922,16.8620582738437,12.));
#171515=CARTESIAN_POINT('Ctrl Pts',(71.9206741030887,16.866998246792,0.));
#171516=CARTESIAN_POINT('Ctrl Pts',(71.9206741030887,16.866998246792,12.));
#171517=CARTESIAN_POINT('Ctrl Pts',(71.8940426586534,16.871907327697,0.));
#171518=CARTESIAN_POINT('Ctrl Pts',(71.8940426586534,16.871907327697,12.));
#171519=CARTESIAN_POINT('Ctrl Pts',(71.867442222915,16.87678554607,0.));
#171520=CARTESIAN_POINT('Ctrl Pts',(71.867442222915,16.87678554607,12.));
#171521=CARTESIAN_POINT('Ctrl Pts',(71.8408728908258,16.8816329317471,0.));
#171522=CARTESIAN_POINT('Ctrl Pts',(71.8408728908258,16.8816329317471,12.));
#171523=CARTESIAN_POINT('Ctrl Pts',(71.8143347584962,16.8864495151344,0.));
#171524=CARTESIAN_POINT('Ctrl Pts',(71.8143347584962,16.8864495151344,12.));
#171525=CARTESIAN_POINT('Ctrl Pts',(71.7878279229546,16.8912353270942,0.));
#171526=CARTESIAN_POINT('Ctrl Pts',(71.7878279229546,16.8912353270942,12.));
#171527=CARTESIAN_POINT('Ctrl Pts',(71.7613524819235,16.895990398841,0.));
#171528=CARTESIAN_POINT('Ctrl Pts',(71.7613524819235,16.895990398841,12.));
#171529=CARTESIAN_POINT('Ctrl Pts',(71.7349085335796,16.9007147618344,0.));
#171530=CARTESIAN_POINT('Ctrl Pts',(71.7349085335796,16.9007147618344,12.));
#171531=CARTESIAN_POINT('Ctrl Pts',(71.7084961763357,16.9054084476847,0.));
#171532=CARTESIAN_POINT('Ctrl Pts',(71.7084961763357,16.9054084476847,12.));
#171533=CARTESIAN_POINT('Ctrl Pts',(71.6821155085612,16.9100714880368,0.));
#171534=CARTESIAN_POINT('Ctrl Pts',(71.6821155085612,16.9100714880368,12.));
#171535=CARTESIAN_POINT('Ctrl Pts',(71.6557666285917,16.9147039145717,0.));
#171536=CARTESIAN_POINT('Ctrl Pts',(71.6557666285917,16.9147039145717,12.));
#171537=CARTESIAN_POINT('Ctrl Pts',(71.6294496348653,16.9193057590607,0.));
#171538=CARTESIAN_POINT('Ctrl Pts',(71.6294496348653,16.9193057590607,12.));
#171539=CARTESIAN_POINT('Ctrl Pts',(71.6031646260174,16.9238770534071,0.));
#171540=CARTESIAN_POINT('Ctrl Pts',(71.6031646260174,16.9238770534071,12.));
#171541=CARTESIAN_POINT('Ctrl Pts',(71.5769117009842,16.9284178296933,0.));
#171542=CARTESIAN_POINT('Ctrl Pts',(71.5769117009842,16.9284178296933,12.));
#171543=CARTESIAN_POINT('Ctrl Pts',(71.5506909591129,16.9329281202377,0.));
#171544=CARTESIAN_POINT('Ctrl Pts',(71.5506909591129,16.9329281202377,12.));
#171545=CARTESIAN_POINT('Ctrl Pts',(71.5245025002139,16.9374079576201,0.));
#171546=CARTESIAN_POINT('Ctrl Pts',(71.5245025002139,16.9374079576201,12.));
#171547=CARTESIAN_POINT('Ctrl Pts',(71.4983464245055,16.9418573746489,0.));
#171548=CARTESIAN_POINT('Ctrl Pts',(71.4983464245055,16.9418573746489,12.));
#171549=CARTESIAN_POINT('Ctrl Pts',(71.4722228325794,16.9462764043443,0.));
#171550=CARTESIAN_POINT('Ctrl Pts',(71.4722228325794,16.9462764043443,12.));
#171551=CARTESIAN_POINT('Ctrl Pts',(71.4461318253563,16.9506650799189,0.));
#171552=CARTESIAN_POINT('Ctrl Pts',(71.4461318253563,16.9506650799189,12.));
#171553=CARTESIAN_POINT('Ctrl Pts',(71.4200735040384,16.9550234347621,0.));
#171554=CARTESIAN_POINT('Ctrl Pts',(71.4200735040384,16.9550234347621,12.));
#171555=CARTESIAN_POINT('Ctrl Pts',(71.3940479700677,16.9593515024276,0.));
#171556=CARTESIAN_POINT('Ctrl Pts',(71.3940479700677,16.9593515024276,12.));
#171557=CARTESIAN_POINT('Ctrl Pts',(71.3680553251562,16.9636493166397,0.));
#171558=CARTESIAN_POINT('Ctrl Pts',(71.3680553251562,16.9636493166397,12.));
#171559=CARTESIAN_POINT('Ctrl Pts',(71.3420956713082,16.9679169112994,0.));
#171560=CARTESIAN_POINT('Ctrl Pts',(71.3420956713082,16.9679169112994,12.));
#171561=CARTESIAN_POINT('Ctrl Pts',(71.3161691108427,16.9721543204951,0.));
#171562=CARTESIAN_POINT('Ctrl Pts',(71.3161691108427,16.9721543204951,12.));
#171563=CARTESIAN_POINT('Ctrl Pts',(71.290275746412,16.9763615785137,0.));
#171564=CARTESIAN_POINT('Ctrl Pts',(71.290275746412,16.9763615785137,12.));
#171565=CARTESIAN_POINT('Ctrl Pts',(71.2644156810198,16.9805387198571,0.));
#171566=CARTESIAN_POINT('Ctrl Pts',(71.2644156810198,16.9805387198571,12.));
#171567=CARTESIAN_POINT('Ctrl Pts',(71.2385890180221,16.9846857792384,0.));
#171568=CARTESIAN_POINT('Ctrl Pts',(71.2385890180221,16.9846857792384,12.));
#171569=CARTESIAN_POINT('Ctrl Pts',(71.212795861124,16.9888027915742,0.));
#171570=CARTESIAN_POINT('Ctrl Pts',(71.212795861124,16.9888027915742,12.));
#171571=CARTESIAN_POINT('Ctrl Pts',(71.187036314374,16.9928897919828,0.));
#171572=CARTESIAN_POINT('Ctrl Pts',(71.187036314374,16.9928897919828,12.));
#171573=CARTESIAN_POINT('Ctrl Pts',(71.1613104821568,16.9969468157824,0.));
#171574=CARTESIAN_POINT('Ctrl Pts',(71.1613104821568,16.9969468157824,12.));
#171575=CARTESIAN_POINT('Ctrl Pts',(71.1356184691806,17.0009738984936,0.));
#171576=CARTESIAN_POINT('Ctrl Pts',(71.1356184691806,17.0009738984936,12.));
#171577=CARTESIAN_POINT('Ctrl Pts',(71.1099603804786,17.0049710758394,0.));
#171578=CARTESIAN_POINT('Ctrl Pts',(71.1099603804786,17.0049710758394,12.));
#171579=CARTESIAN_POINT('Ctrl Pts',(71.0843363214221,17.0089383837437,0.));
#171580=CARTESIAN_POINT('Ctrl Pts',(71.0843363214221,17.0089383837437,12.));
#171581=CARTESIAN_POINT('Ctrl Pts',(71.0587463977268,17.0128758583335,0.));
#171582=CARTESIAN_POINT('Ctrl Pts',(71.0587463977268,17.0128758583335,12.));
#171583=CARTESIAN_POINT('Ctrl Pts',(71.0331907154574,17.0167835359419,0.));
#171584=CARTESIAN_POINT('Ctrl Pts',(71.0331907154574,17.0167835359419,12.));
#171585=CARTESIAN_POINT('Ctrl Pts',(71.0076693810301,17.0206614531166,0.));
#171586=CARTESIAN_POINT('Ctrl Pts',(71.0076693810301,17.0206614531166,12.));
#171587=CARTESIAN_POINT('Ctrl Pts',(70.9821825012136,17.0245096466229,0.));
#171588=CARTESIAN_POINT('Ctrl Pts',(70.9821825012136,17.0245096466229,12.));
#171589=CARTESIAN_POINT('Ctrl Pts',(70.956730183136,17.0283281534392,0.));
#171590=CARTESIAN_POINT('Ctrl Pts',(70.956730183136,17.0283281534392,12.));
#171591=CARTESIAN_POINT('Ctrl Pts',(70.9313125342876,17.0321170107564,0.));
#171592=CARTESIAN_POINT('Ctrl Pts',(70.9313125342876,17.0321170107564,12.));
#171593=CARTESIAN_POINT('Ctrl Pts',(70.9059296625214,17.0358762559786,0.));
#171594=CARTESIAN_POINT('Ctrl Pts',(70.9059296625214,17.0358762559786,12.));
#171595=CARTESIAN_POINT('Ctrl Pts',(70.8805816760501,17.0396059267277,0.));
#171596=CARTESIAN_POINT('Ctrl Pts',(70.8805816760501,17.0396059267277,12.));
#171597=CARTESIAN_POINT('Ctrl Pts',(70.8552686834423,17.0433060608475,0.));
#171598=CARTESIAN_POINT('Ctrl Pts',(70.8552686834423,17.0433060608475,12.));
#171599=CARTESIAN_POINT('Ctrl Pts',(70.8299907936334,17.0469766964001,0.));
#171600=CARTESIAN_POINT('Ctrl Pts',(70.8299907936334,17.0469766964001,12.));
#171601=CARTESIAN_POINT('Ctrl Pts',(70.8047481159298,17.0506178716662,0.));
#171602=CARTESIAN_POINT('Ctrl Pts',(70.8047481159298,17.0506178716662,12.));
#171603=CARTESIAN_POINT('Ctrl Pts',(70.7795407600127,17.0542296251462,0.));
#171604=CARTESIAN_POINT('Ctrl Pts',(70.7795407600127,17.0542296251462,12.));
#171605=CARTESIAN_POINT('Ctrl Pts',(70.754368835938,17.0578119955651,0.));
#171606=CARTESIAN_POINT('Ctrl Pts',(70.754368835938,17.0578119955651,12.));
#171607=CARTESIAN_POINT('Ctrl Pts',(70.7292324541348,17.0613650218789,0.));
#171608=CARTESIAN_POINT('Ctrl Pts',(70.7292324541348,17.0613650218789,12.));
#171609=CARTESIAN_POINT('Ctrl Pts',(70.7041317254128,17.0648887432714,0.));
#171610=CARTESIAN_POINT('Ctrl Pts',(70.7041317254128,17.0648887432714,12.));
#171611=CARTESIAN_POINT('Ctrl Pts',(70.6790667609678,17.0683831991532,0.));
#171612=CARTESIAN_POINT('Ctrl Pts',(70.6790667609678,17.0683831991532,12.));
#171613=CARTESIAN_POINT('Ctrl Pts',(70.6540376723839,17.0718484291623,0.));
#171614=CARTESIAN_POINT('Ctrl Pts',(70.6540376723839,17.0718484291623,12.));
#171615=CARTESIAN_POINT('Ctrl Pts',(70.6290445716341,17.0752844731679,0.));
#171616=CARTESIAN_POINT('Ctrl Pts',(70.6290445716341,17.0752844731679,12.));
#171617=CARTESIAN_POINT('Ctrl Pts',(70.6040875710762,17.0786913712767,0.));
#171618=CARTESIAN_POINT('Ctrl Pts',(70.6040875710762,17.0786913712767,12.));
#171619=CARTESIAN_POINT('Ctrl Pts',(70.5791667834599,17.0820691638314,0.));
#171620=CARTESIAN_POINT('Ctrl Pts',(70.5791667834599,17.0820691638314,12.));
#171621=CARTESIAN_POINT('Ctrl Pts',(70.5542823219346,17.085417891409,0.));
#171622=CARTESIAN_POINT('Ctrl Pts',(70.5542823219346,17.085417891409,12.));
#171623=CARTESIAN_POINT('Ctrl Pts',(70.5294343000516,17.0887375948221,0.));
#171624=CARTESIAN_POINT('Ctrl Pts',(70.5294343000516,17.0887375948221,12.));
#171625=CARTESIAN_POINT('Ctrl Pts',(70.5046228317669,17.0920283151217,0.));
#171626=CARTESIAN_POINT('Ctrl Pts',(70.5046228317669,17.0920283151217,12.));
#171627=CARTESIAN_POINT('Ctrl Pts',(70.4798480314364,17.0952900936044,0.));
#171628=CARTESIAN_POINT('Ctrl Pts',(70.4798480314364,17.0952900936044,12.));
#171629=CARTESIAN_POINT('Ctrl Pts',(70.4551100138221,17.098522971812,0.));
#171630=CARTESIAN_POINT('Ctrl Pts',(70.4551100138221,17.098522971812,12.));
#171631=CARTESIAN_POINT('Ctrl Pts',(70.4304088940998,17.1017269915289,0.));
#171632=CARTESIAN_POINT('Ctrl Pts',(70.4304088940998,17.1017269915289,12.));
#171633=CARTESIAN_POINT('Ctrl Pts',(70.4057447878621,17.1049021947833,0.));
#171634=CARTESIAN_POINT('Ctrl Pts',(70.4057447878621,17.1049021947833,12.));
#171635=CARTESIAN_POINT('Ctrl Pts',(70.3811178111206,17.10804862385,0.));
#171636=CARTESIAN_POINT('Ctrl Pts',(70.3811178111206,17.10804862385,12.));
#171637=CARTESIAN_POINT('Ctrl Pts',(70.356528080303,17.111166321257,0.));
#171638=CARTESIAN_POINT('Ctrl Pts',(70.356528080303,17.111166321257,12.));
#171639=CARTESIAN_POINT('Ctrl Pts',(70.3319757122577,17.1142553297869,0.));
#171640=CARTESIAN_POINT('Ctrl Pts',(70.3319757122577,17.1142553297869,12.));
#171641=CARTESIAN_POINT('Ctrl Pts',(70.3074608242613,17.1173156924734,0.));
#171642=CARTESIAN_POINT('Ctrl Pts',(70.3074608242613,17.1173156924734,12.));
#171643=CARTESIAN_POINT('Ctrl Pts',(70.2829835340239,17.1203474526031,0.));
#171644=CARTESIAN_POINT('Ctrl Pts',(70.2829835340239,17.1203474526031,12.));
#171645=CARTESIAN_POINT('Ctrl Pts',(70.2585439596899,17.1233506537176,0.));
#171646=CARTESIAN_POINT('Ctrl Pts',(70.2585439596899,17.1233506537176,12.));
#171647=CARTESIAN_POINT('Ctrl Pts',(70.2341422198363,17.1263253396202,0.));
#171648=CARTESIAN_POINT('Ctrl Pts',(70.2341422198363,17.1263253396202,12.));
#171649=CARTESIAN_POINT('Ctrl Pts',(70.2097784334749,17.1292715543779,0.));
#171650=CARTESIAN_POINT('Ctrl Pts',(70.2097784334749,17.1292715543779,12.));
#171651=CARTESIAN_POINT('Ctrl Pts',(70.1854527200636,17.1321893423183,0.));
#171652=CARTESIAN_POINT('Ctrl Pts',(70.1854527200636,17.1321893423183,12.));
#171653=CARTESIAN_POINT('Ctrl Pts',(70.1611651995085,17.1350787480313,0.));
#171654=CARTESIAN_POINT('Ctrl Pts',(70.1611651995085,17.1350787480313,12.));
#171655=CARTESIAN_POINT('Ctrl Pts',(70.1369159921686,17.1379398163708,0.));
#171656=CARTESIAN_POINT('Ctrl Pts',(70.1369159921686,17.1379398163708,12.));
#171657=CARTESIAN_POINT('Ctrl Pts',(70.1127052188515,17.1407725924615,0.));
#171658=CARTESIAN_POINT('Ctrl Pts',(70.1127052188515,17.1407725924615,12.));
#171659=CARTESIAN_POINT('Ctrl Pts',(70.0885330008169,17.1435771217015,0.));
#171660=CARTESIAN_POINT('Ctrl Pts',(70.0885330008169,17.1435771217015,12.));
#171661=CARTESIAN_POINT('Ctrl Pts',(70.0643994597865,17.1463534497592,0.));
#171662=CARTESIAN_POINT('Ctrl Pts',(70.0643994597865,17.1463534497592,12.));
#171663=CARTESIAN_POINT('Ctrl Pts',(70.0403047179481,17.1491016225748,0.));
#171664=CARTESIAN_POINT('Ctrl Pts',(70.0403047179481,17.1491016225748,12.));
#171665=CARTESIAN_POINT('Ctrl Pts',(70.0162488979587,17.1518216863624,0.));
#171666=CARTESIAN_POINT('Ctrl Pts',(70.0162488979587,17.1518216863624,12.));
#171667=CARTESIAN_POINT('Ctrl Pts',(69.9922321229428,17.1545136876162,0.));
#171668=CARTESIAN_POINT('Ctrl Pts',(69.9922321229428,17.1545136876162,12.));
#171669=CARTESIAN_POINT('Ctrl Pts',(69.9682545164942,17.157177673114,0.));
#171670=CARTESIAN_POINT('Ctrl Pts',(69.9682545164942,17.157177673114,12.));
#171671=CARTESIAN_POINT('Ctrl Pts',(69.9443162026865,17.1598136899144,0.));
#171672=CARTESIAN_POINT('Ctrl Pts',(69.9443162026865,17.1598136899144,12.));
#171673=CARTESIAN_POINT('Ctrl Pts',(69.9204173060779,17.1624217853577,0.));
#171674=CARTESIAN_POINT('Ctrl Pts',(69.9204173060779,17.1624217853577,12.));
#171675=CARTESIAN_POINT('Ctrl Pts',(69.8965579517147,17.1650020070686,0.));
#171676=CARTESIAN_POINT('Ctrl Pts',(69.8965579517147,17.1650020070686,12.));
#171677=CARTESIAN_POINT('Ctrl Pts',(69.8727382651292,17.1675544029622,0.));
#171678=CARTESIAN_POINT('Ctrl Pts',(69.8727382651292,17.1675544029622,12.));
#171679=CARTESIAN_POINT('Ctrl Pts',(69.8489583723417,17.1700790212476,0.));
#171680=CARTESIAN_POINT('Ctrl Pts',(69.8489583723417,17.1700790212476,12.));
#171681=CARTESIAN_POINT('Ctrl Pts',(69.8252183998713,17.1725759104254,0.));
#171682=CARTESIAN_POINT('Ctrl Pts',(69.8252183998713,17.1725759104254,12.));
#171683=CARTESIAN_POINT('Ctrl Pts',(69.8015184747404,17.1750451192887,0.));
#171684=CARTESIAN_POINT('Ctrl Pts',(69.8015184747404,17.1750451192887,12.));
#171685=CARTESIAN_POINT('Ctrl Pts',(69.7778587244788,17.1774866969256,0.));
#171686=CARTESIAN_POINT('Ctrl Pts',(69.7778587244788,17.1774866969256,12.));
#171687=CARTESIAN_POINT('Ctrl Pts',(69.7542392771216,17.1799006927256,0.));
#171688=CARTESIAN_POINT('Ctrl Pts',(69.7542392771216,17.1799006927256,12.));
#171689=CARTESIAN_POINT('Ctrl Pts',(69.7306602612125,17.1822871563835,0.));
#171690=CARTESIAN_POINT('Ctrl Pts',(69.7306602612125,17.1822871563835,12.));
#171691=CARTESIAN_POINT('Ctrl Pts',(69.7071218058149,17.1846461378966,0.));
#171692=CARTESIAN_POINT('Ctrl Pts',(69.7071218058149,17.1846461378966,12.));
#171693=CARTESIAN_POINT('Ctrl Pts',(69.6836240405152,17.1869776875663,0.));
#171694=CARTESIAN_POINT('Ctrl Pts',(69.6836240405152,17.1869776875663,12.));
#171695=CARTESIAN_POINT('Ctrl Pts',(69.6601670954277,17.1892818560004,0.));
#171696=CARTESIAN_POINT('Ctrl Pts',(69.6601670954277,17.1892818560004,12.));
#171697=CARTESIAN_POINT('Ctrl Pts',(69.6367511011927,17.1915586941198,0.));
#171698=CARTESIAN_POINT('Ctrl Pts',(69.6367511011927,17.1915586941198,12.));
#171699=CARTESIAN_POINT('Ctrl Pts',(69.6133761889787,17.193808253162,0.));
#171700=CARTESIAN_POINT('Ctrl Pts',(69.6133761889787,17.193808253162,12.));
#171701=CARTESIAN_POINT('Ctrl Pts',(69.5900424904954,17.1960305846787,0.));
#171702=CARTESIAN_POINT('Ctrl Pts',(69.5900424904954,17.1960305846787,12.));
#171703=CARTESIAN_POINT('Ctrl Pts',(69.5667501379984,17.198225740538,0.));
#171704=CARTESIAN_POINT('Ctrl Pts',(69.5667501379984,17.198225740538,12.));
#171705=CARTESIAN_POINT('Ctrl Pts',(69.5434992642932,17.2003937729266,0.));
#171706=CARTESIAN_POINT('Ctrl Pts',(69.5434992642932,17.2003937729266,12.));
#171707=CARTESIAN_POINT('Ctrl Pts',(69.5202900027329,17.2025347343568,0.));
#171708=CARTESIAN_POINT('Ctrl Pts',(69.5202900027329,17.2025347343568,12.));
#171709=CARTESIAN_POINT('Ctrl Pts',(69.497122487222,17.2046486776697,0.));
#171710=CARTESIAN_POINT('Ctrl Pts',(69.497122487222,17.2046486776697,12.));
#171711=CARTESIAN_POINT('Ctrl Pts',(69.4739968522271,17.2067356560326,0.));
#171712=CARTESIAN_POINT('Ctrl Pts',(69.4739968522271,17.2067356560326,12.));
#171713=CARTESIAN_POINT('Ctrl Pts',(69.4509132327836,17.208795722942,0.));
#171714=CARTESIAN_POINT('Ctrl Pts',(69.4509132327836,17.208795722942,12.));
#171715=CARTESIAN_POINT('Ctrl Pts',(69.4278717644989,17.2108289322258,0.));
#171716=CARTESIAN_POINT('Ctrl Pts',(69.4278717644989,17.2108289322258,12.));
#171717=CARTESIAN_POINT('Ctrl Pts',(69.4048725835516,17.2128353380511,0.));
#171718=CARTESIAN_POINT('Ctrl Pts',(69.4048725835516,17.2128353380511,12.));
#171719=CARTESIAN_POINT('Ctrl Pts',(69.3819158266955,17.2148149949261,0.));
#171720=CARTESIAN_POINT('Ctrl Pts',(69.3819158266955,17.2148149949261,12.));
#171721=CARTESIAN_POINT('Ctrl Pts',(69.359001631272,17.2167679576991,0.));
#171722=CARTESIAN_POINT('Ctrl Pts',(69.359001631272,17.2167679576991,12.));
#171723=CARTESIAN_POINT('Ctrl Pts',(69.3361301352149,17.2186942815604,0.));
#171724=CARTESIAN_POINT('Ctrl Pts',(69.3361301352149,17.2186942815604,12.));
#171725=CARTESIAN_POINT('Ctrl Pts',(69.3133014770541,17.2205940220455,0.));
#171726=CARTESIAN_POINT('Ctrl Pts',(69.3133014770541,17.2205940220455,12.));
#171727=CARTESIAN_POINT('Ctrl Pts',(69.2905157959142,17.2224672350432,0.));
#171728=CARTESIAN_POINT('Ctrl Pts',(69.2905157959142,17.2224672350432,12.));
#171729=CARTESIAN_POINT('Ctrl Pts',(69.26777323152,17.2243139767963,0.));
#171730=CARTESIAN_POINT('Ctrl Pts',(69.26777323152,17.2243139767963,12.));
#171731=CARTESIAN_POINT('Ctrl Pts',(69.2450739242092,17.2261343039015,0.));
#171732=CARTESIAN_POINT('Ctrl Pts',(69.2450739242092,17.2261343039015,12.));
#171733=CARTESIAN_POINT('Ctrl Pts',(69.2224180149377,17.2279282733119,0.));
#171734=CARTESIAN_POINT('Ctrl Pts',(69.2224180149377,17.2279282733119,12.));
#171735=CARTESIAN_POINT('Ctrl Pts',(69.1998056452837,17.229695942341,0.));
#171736=CARTESIAN_POINT('Ctrl Pts',(69.1998056452837,17.229695942341,12.));
#171737=CARTESIAN_POINT('Ctrl Pts',(69.1772369574462,17.2314373686705,0.));
#171738=CARTESIAN_POINT('Ctrl Pts',(69.1772369574462,17.2314373686705,12.));
#171739=CARTESIAN_POINT('Ctrl Pts',(69.1547120942542,17.2331526103511,0.));
#171740=CARTESIAN_POINT('Ctrl Pts',(69.1547120942542,17.2331526103511,12.));
#171741=CARTESIAN_POINT('Ctrl Pts',(69.1322311991759,17.2348417258017,0.));
#171742=CARTESIAN_POINT('Ctrl Pts',(69.1322311991759,17.2348417258017,12.));
#171743=CARTESIAN_POINT('Ctrl Pts',(69.1097944163243,17.2365047738125,0.));
#171744=CARTESIAN_POINT('Ctrl Pts',(69.1097944163243,17.2365047738125,12.));
#171745=CARTESIAN_POINT('Ctrl Pts',(69.0874018904598,17.238141813549,0.));
#171746=CARTESIAN_POINT('Ctrl Pts',(69.0874018904598,17.238141813549,12.));
#171747=CARTESIAN_POINT('Ctrl Pts',(69.0650537669859,17.2397529045587,0.));
#171748=CARTESIAN_POINT('Ctrl Pts',(69.0650537669859,17.2397529045587,12.));
#171749=CARTESIAN_POINT('Ctrl Pts',(69.0427501919636,17.2413381067722,0.));
#171750=CARTESIAN_POINT('Ctrl Pts',(69.0427501919636,17.2413381067722,12.));
#171751=CARTESIAN_POINT('Ctrl Pts',(69.0204913121226,17.2428974805043,0.));
#171752=CARTESIAN_POINT('Ctrl Pts',(69.0204913121226,17.2428974805043,12.));
#171753=CARTESIAN_POINT('Ctrl Pts',(68.9982772748694,17.2444310864585,0.));
#171754=CARTESIAN_POINT('Ctrl Pts',(68.9982772748694,17.2444310864585,12.));
#171755=CARTESIAN_POINT('Ctrl Pts',(68.9761082282922,17.2459389857327,0.));
#171756=CARTESIAN_POINT('Ctrl Pts',(68.9761082282922,17.2459389857327,12.));
#171757=CARTESIAN_POINT('Ctrl Pts',(68.9539843211618,17.2474212398275,0.));
#171758=CARTESIAN_POINT('Ctrl Pts',(68.9539843211618,17.2474212398275,12.));
#171759=CARTESIAN_POINT('Ctrl Pts',(68.9319057029407,17.248877910643,0.));
#171760=CARTESIAN_POINT('Ctrl Pts',(68.9319057029407,17.248877910643,12.));
#171761=CARTESIAN_POINT('Ctrl Pts',(68.9098725237868,17.2503090604792,0.));
#171762=CARTESIAN_POINT('Ctrl Pts',(68.9098725237868,17.2503090604792,12.));
#171763=CARTESIAN_POINT('Ctrl Pts',(68.8878849345557,17.2517147520376,0.));
#171764=CARTESIAN_POINT('Ctrl Pts',(68.8878849345557,17.2517147520376,12.));
#171765=CARTESIAN_POINT('Ctrl Pts',(68.8659430867977,17.2530950484259,0.));
#171766=CARTESIAN_POINT('Ctrl Pts',(68.8659430867977,17.2530950484259,12.));
#171767=CARTESIAN_POINT('Ctrl Pts',(68.8440471327563,17.2544500131627,0.));
#171768=CARTESIAN_POINT('Ctrl Pts',(68.8440471327563,17.2544500131627,12.));
#171769=CARTESIAN_POINT('Ctrl Pts',(68.8221972253954,17.2557797101816,0.));
#171770=CARTESIAN_POINT('Ctrl Pts',(68.8221972253954,17.2557797101816,12.));
#171771=CARTESIAN_POINT('Ctrl Pts',(68.8003935184193,17.2570842038386,0.));
#171772=CARTESIAN_POINT('Ctrl Pts',(68.8003935184193,17.2570842038386,12.));
#171773=CARTESIAN_POINT('Ctrl Pts',(68.7786361662876,17.2583635589197,0.));
#171774=CARTESIAN_POINT('Ctrl Pts',(68.7786361662876,17.2583635589197,12.));
#171775=CARTESIAN_POINT('Ctrl Pts',(68.7569253242312,17.2596178406545,0.));
#171776=CARTESIAN_POINT('Ctrl Pts',(68.7569253242312,17.2596178406545,12.));
#171777=CARTESIAN_POINT('Ctrl Pts',(68.7352611482519,17.2608471147178,0.));
#171778=CARTESIAN_POINT('Ctrl Pts',(68.7352611482519,17.2608471147178,12.));
#171779=CARTESIAN_POINT('Ctrl Pts',(68.7136437951075,17.2620514472176,0.));
#171780=CARTESIAN_POINT('Ctrl Pts',(68.7136437951075,17.2620514472176,12.));
#171781=CARTESIAN_POINT('Ctrl Pts',(68.6920734222932,17.263230904689,0.));
#171782=CARTESIAN_POINT('Ctrl Pts',(68.6920734222932,17.263230904689,12.));
#171783=CARTESIAN_POINT('Ctrl Pts',(68.6705501880263,17.2643855540896,0.));
#171784=CARTESIAN_POINT('Ctrl Pts',(68.6705501880263,17.2643855540896,12.));
#171785=CARTESIAN_POINT('Ctrl Pts',(68.6490742512085,17.2655154627935,0.));
#171786=CARTESIAN_POINT('Ctrl Pts',(68.6490742512085,17.2655154627935,12.));
#171787=CARTESIAN_POINT('Ctrl Pts',(68.6276457714757,17.2666206986091,0.));
#171788=CARTESIAN_POINT('Ctrl Pts',(68.6276457714757,17.2666206986091,12.));
#171789=CARTESIAN_POINT('Ctrl Pts',(68.6062649092781,17.2677013298061,0.));
#171790=CARTESIAN_POINT('Ctrl Pts',(68.6062649092781,17.2677013298061,12.));
#171791=CARTESIAN_POINT('Ctrl Pts',(68.5849318259449,17.2687574251429,0.));
#171792=CARTESIAN_POINT('Ctrl Pts',(68.5849318259449,17.2687574251429,12.));
#171793=CARTESIAN_POINT('Ctrl Pts',(68.5636466837502,17.2697890538956,0.));
#171794=CARTESIAN_POINT('Ctrl Pts',(68.5636466837502,17.2697890538956,12.));
#171795=CARTESIAN_POINT('Ctrl Pts',(68.5424096459746,17.2707962858912,0.));
#171796=CARTESIAN_POINT('Ctrl Pts',(68.5424096459746,17.2707962858912,12.));
#171797=CARTESIAN_POINT('Ctrl Pts',(68.5212208767835,17.2717791914538,0.));
#171798=CARTESIAN_POINT('Ctrl Pts',(68.5212208767835,17.2717791914538,12.));
#171799=CARTESIAN_POINT('Ctrl Pts',(68.5000805410897,17.2727378413485,0.));
#171800=CARTESIAN_POINT('Ctrl Pts',(68.5000805410897,17.2727378413485,12.));
#171801=CARTESIAN_POINT('Ctrl Pts',(68.4789888044357,17.2736723067367,0.));
#171802=CARTESIAN_POINT('Ctrl Pts',(68.4789888044357,17.2736723067367,12.));
#171803=CARTESIAN_POINT('Ctrl Pts',(68.4579458328208,17.2745826591125,0.));
#171804=CARTESIAN_POINT('Ctrl Pts',(68.4579458328208,17.2745826591125,12.));
#171805=CARTESIAN_POINT('Ctrl Pts',(68.4369517926803,17.2754689703001,0.));
#171806=CARTESIAN_POINT('Ctrl Pts',(68.4369517926803,17.2754689703001,12.));
#171807=CARTESIAN_POINT('Ctrl Pts',(68.4160068512781,17.2763313126026,0.));
#171808=CARTESIAN_POINT('Ctrl Pts',(68.4160068512781,17.2763313126026,12.));
#171809=CARTESIAN_POINT('Ctrl Pts',(68.3951111770498,17.2771697589387,0.));
#171810=CARTESIAN_POINT('Ctrl Pts',(68.3951111770498,17.2771697589387,12.));
#171811=CARTESIAN_POINT('Ctrl Pts',(68.374264939895,17.2779843829605,0.));
#171812=CARTESIAN_POINT('Ctrl Pts',(68.374264939895,17.2779843829605,12.));
#171813=CARTESIAN_POINT('Ctrl Pts',(68.353468311648,17.2787752592475,0.));
#171814=CARTESIAN_POINT('Ctrl Pts',(68.353468311648,17.2787752592475,12.));
#171815=CARTESIAN_POINT('Ctrl Pts',(68.3327214657533,17.2795424631789,0.));
#171816=CARTESIAN_POINT('Ctrl Pts',(68.3327214657533,17.2795424631789,12.));
#171817=CARTESIAN_POINT('Ctrl Pts',(68.3120245763884,17.2802860705807,0.));
#171818=CARTESIAN_POINT('Ctrl Pts',(68.3120245763884,17.2802860705807,12.));
#171819=CARTESIAN_POINT('Ctrl Pts',(68.2913778177258,17.2810061574352,0.));
#171820=CARTESIAN_POINT('Ctrl Pts',(68.2913778177258,17.2810061574352,12.));
#171821=CARTESIAN_POINT('Ctrl Pts',(68.2707813631761,17.2817027995838,0.));
#171822=CARTESIAN_POINT('Ctrl Pts',(68.2707813631761,17.2817027995838,12.));
#171823=CARTESIAN_POINT('Ctrl Pts',(68.250235384512,17.2823760723886,0.));
#171824=CARTESIAN_POINT('Ctrl Pts',(68.250235384512,17.2823760723886,12.));
#171825=CARTESIAN_POINT('Ctrl Pts',(68.2297400535339,17.2830260513879,0.));
#171826=CARTESIAN_POINT('Ctrl Pts',(68.2297400535339,17.2830260513879,12.));
#171827=CARTESIAN_POINT('Ctrl Pts',(68.2092955440591,17.2836528130825,0.));
#171828=CARTESIAN_POINT('Ctrl Pts',(68.2092955440591,17.2836528130825,12.));
#171829=CARTESIAN_POINT('Ctrl Pts',(68.1889020335418,17.2842564355796,0.));
#171830=CARTESIAN_POINT('Ctrl Pts',(68.1889020335418,17.2842564355796,12.));
#171831=CARTESIAN_POINT('Ctrl Pts',(68.1685597054193,17.2848369995283,0.));
#171832=CARTESIAN_POINT('Ctrl Pts',(68.1685597054193,17.2848369995283,12.));
#171833=CARTESIAN_POINT('Ctrl Pts',(68.1482687493176,17.2853945882059,0.));
#171834=CARTESIAN_POINT('Ctrl Pts',(68.1482687493176,17.2853945882059,12.));
#171835=CARTESIAN_POINT('Ctrl Pts',(68.1280293561473,17.2859292855694,0.));
#171836=CARTESIAN_POINT('Ctrl Pts',(68.1280293561473,17.2859292855694,12.));
#171837=CARTESIAN_POINT('Ctrl Pts',(68.1078417137865,17.2864411745456,0.));
#171838=CARTESIAN_POINT('Ctrl Pts',(68.1078417137865,17.2864411745456,12.));
#171839=CARTESIAN_POINT('Ctrl Pts',(68.0877060033229,17.2869303355438,0.));
#171840=CARTESIAN_POINT('Ctrl Pts',(68.0877060033229,17.2869303355438,12.));
#171841=CARTESIAN_POINT('Ctrl Pts',(68.0676223930469,17.2873968440855,0.));
#171842=CARTESIAN_POINT('Ctrl Pts',(68.0676223930469,17.2873968440855,12.));
#171843=CARTESIAN_POINT('Ctrl Pts',(68.0475910442494,17.2878407730981,0.));
#171844=CARTESIAN_POINT('Ctrl Pts',(68.0475910442494,17.2878407730981,12.));
#171845=CARTESIAN_POINT('Ctrl Pts',(68.027612122741,17.2882621974737,0.));
#171846=CARTESIAN_POINT('Ctrl Pts',(68.027612122741,17.2882621974737,12.));
#171847=CARTESIAN_POINT('Ctrl Pts',(68.007685808115,17.28866119774,0.));
#171848=CARTESIAN_POINT('Ctrl Pts',(68.007685808115,17.28866119774,12.));
#171849=CARTESIAN_POINT('Ctrl Pts',(67.9878123049133,17.2890378644843,0.));
#171850=CARTESIAN_POINT('Ctrl Pts',(67.9878123049133,17.2890378644843,12.));
#171851=CARTESIAN_POINT('Ctrl Pts',(67.9679918502441,17.2893923013852,0.));
#171852=CARTESIAN_POINT('Ctrl Pts',(67.9679918502441,17.2893923013852,12.));
#171853=CARTESIAN_POINT('Ctrl Pts',(67.9482246901517,17.2897246158895,0.));
#171854=CARTESIAN_POINT('Ctrl Pts',(67.9482246901517,17.2897246158895,12.));
#171855=CARTESIAN_POINT('Ctrl Pts',(67.9285110571662,17.2900349103956,0.));
#171856=CARTESIAN_POINT('Ctrl Pts',(67.9285110571662,17.2900349103956,12.));
#171857=CARTESIAN_POINT('Ctrl Pts',(67.908851149676,17.2903232740717,0.));
#171858=CARTESIAN_POINT('Ctrl Pts',(67.908851149676,17.2903232740717,12.));
#171859=CARTESIAN_POINT('Ctrl Pts',(67.8892451049871,17.2905897724029,0.));
#171860=CARTESIAN_POINT('Ctrl Pts',(67.8892451049871,17.2905897724029,12.));
#171861=CARTESIAN_POINT('Ctrl Pts',(67.8696929979178,17.2908344459816,0.));
#171862=CARTESIAN_POINT('Ctrl Pts',(67.8696929979178,17.2908344459816,12.));
#171863=CARTESIAN_POINT('Ctrl Pts',(67.8540944890057,17.2910127431203,0.));
#171864=CARTESIAN_POINT('Ctrl Pts',(67.8540944890057,17.2910127431203,12.));
#171865=CARTESIAN_POINT('Ctrl Pts',(67.8424198971214,17.2911366591419,0.));
#171866=CARTESIAN_POINT('Ctrl Pts',(67.8424198971214,17.2911366591419,12.));
#171867=CARTESIAN_POINT('Ctrl Pts',(67.8346476309106,17.2912149114145,0.));
#171868=CARTESIAN_POINT('Ctrl Pts',(67.8346476309106,17.2912149114145,12.));
#171869=CARTESIAN_POINT('Ctrl Pts',(67.8307641965655,17.2912529479484,0.));
#171870=CARTESIAN_POINT('Ctrl Pts',(67.8307641965655,17.2912529479484,12.));
#171871=CARTESIAN_POINT('',(67.8307641965655,17.2912529479484,12.));
#171872=CARTESIAN_POINT('Ctrl Pts',(67.8307641965655,17.2912529479484,12.));
#171873=CARTESIAN_POINT('Ctrl Pts',(67.8346476309106,17.2912149114145,12.));
#171874=CARTESIAN_POINT('Ctrl Pts',(67.8424198971214,17.2911366591419,12.));
#171875=CARTESIAN_POINT('Ctrl Pts',(67.8540944890057,17.2910127431203,12.));
#171876=CARTESIAN_POINT('Ctrl Pts',(67.8696929979178,17.2908344459816,12.));
#171877=CARTESIAN_POINT('Ctrl Pts',(67.8892451049871,17.2905897724029,12.));
#171878=CARTESIAN_POINT('Ctrl Pts',(67.908851149676,17.2903232740717,12.));
#171879=CARTESIAN_POINT('Ctrl Pts',(67.9285110571662,17.2900349103956,12.));
#171880=CARTESIAN_POINT('Ctrl Pts',(67.9482246901517,17.2897246158895,12.));
#171881=CARTESIAN_POINT('Ctrl Pts',(67.9679918502441,17.2893923013852,12.));
#171882=CARTESIAN_POINT('Ctrl Pts',(67.9878123049133,17.2890378644843,12.));
#171883=CARTESIAN_POINT('Ctrl Pts',(68.007685808115,17.28866119774,12.));
#171884=CARTESIAN_POINT('Ctrl Pts',(68.027612122741,17.2882621974737,12.));
#171885=CARTESIAN_POINT('Ctrl Pts',(68.0475910442494,17.2878407730981,12.));
#171886=CARTESIAN_POINT('Ctrl Pts',(68.0676223930469,17.2873968440855,12.));
#171887=CARTESIAN_POINT('Ctrl Pts',(68.0877060033229,17.2869303355438,12.));
#171888=CARTESIAN_POINT('Ctrl Pts',(68.1078417137865,17.2864411745456,12.));
#171889=CARTESIAN_POINT('Ctrl Pts',(68.1280293561473,17.2859292855694,12.));
#171890=CARTESIAN_POINT('Ctrl Pts',(68.1482687493176,17.2853945882059,12.));
#171891=CARTESIAN_POINT('Ctrl Pts',(68.1685597054193,17.2848369995283,12.));
#171892=CARTESIAN_POINT('Ctrl Pts',(68.1889020335418,17.2842564355796,12.));
#171893=CARTESIAN_POINT('Ctrl Pts',(68.2092955440591,17.2836528130825,12.));
#171894=CARTESIAN_POINT('Ctrl Pts',(68.2297400535339,17.2830260513879,12.));
#171895=CARTESIAN_POINT('Ctrl Pts',(68.250235384512,17.2823760723886,12.));
#171896=CARTESIAN_POINT('Ctrl Pts',(68.2707813631761,17.2817027995838,12.));
#171897=CARTESIAN_POINT('Ctrl Pts',(68.2913778177258,17.2810061574352,12.));
#171898=CARTESIAN_POINT('Ctrl Pts',(68.3120245763884,17.2802860705807,12.));
#171899=CARTESIAN_POINT('Ctrl Pts',(68.3327214657533,17.2795424631789,12.));
#171900=CARTESIAN_POINT('Ctrl Pts',(68.353468311648,17.2787752592475,12.));
#171901=CARTESIAN_POINT('Ctrl Pts',(68.374264939895,17.2779843829605,12.));
#171902=CARTESIAN_POINT('Ctrl Pts',(68.3951111770498,17.2771697589387,12.));
#171903=CARTESIAN_POINT('Ctrl Pts',(68.4160068512781,17.2763313126026,12.));
#171904=CARTESIAN_POINT('Ctrl Pts',(68.4369517926803,17.2754689703001,12.));
#171905=CARTESIAN_POINT('Ctrl Pts',(68.4579458328208,17.2745826591125,12.));
#171906=CARTESIAN_POINT('Ctrl Pts',(68.4789888044357,17.2736723067367,12.));
#171907=CARTESIAN_POINT('Ctrl Pts',(68.5000805410897,17.2727378413485,12.));
#171908=CARTESIAN_POINT('Ctrl Pts',(68.5212208767835,17.2717791914538,12.));
#171909=CARTESIAN_POINT('Ctrl Pts',(68.5424096459746,17.2707962858912,12.));
#171910=CARTESIAN_POINT('Ctrl Pts',(68.5636466837502,17.2697890538956,12.));
#171911=CARTESIAN_POINT('Ctrl Pts',(68.5849318259449,17.2687574251429,12.));
#171912=CARTESIAN_POINT('Ctrl Pts',(68.6062649092781,17.2677013298061,12.));
#171913=CARTESIAN_POINT('Ctrl Pts',(68.6276457714757,17.2666206986091,12.));
#171914=CARTESIAN_POINT('Ctrl Pts',(68.6490742512085,17.2655154627935,12.));
#171915=CARTESIAN_POINT('Ctrl Pts',(68.6705501880263,17.2643855540896,12.));
#171916=CARTESIAN_POINT('Ctrl Pts',(68.6920734222932,17.263230904689,12.));
#171917=CARTESIAN_POINT('Ctrl Pts',(68.7136437951075,17.2620514472176,12.));
#171918=CARTESIAN_POINT('Ctrl Pts',(68.7352611482519,17.2608471147178,12.));
#171919=CARTESIAN_POINT('Ctrl Pts',(68.7569253242312,17.2596178406545,12.));
#171920=CARTESIAN_POINT('Ctrl Pts',(68.7786361662876,17.2583635589197,12.));
#171921=CARTESIAN_POINT('Ctrl Pts',(68.8003935184193,17.2570842038386,12.));
#171922=CARTESIAN_POINT('Ctrl Pts',(68.8221972253954,17.2557797101816,12.));
#171923=CARTESIAN_POINT('Ctrl Pts',(68.8440471327563,17.2544500131627,12.));
#171924=CARTESIAN_POINT('Ctrl Pts',(68.8659430867977,17.2530950484259,12.));
#171925=CARTESIAN_POINT('Ctrl Pts',(68.8878849345557,17.2517147520376,12.));
#171926=CARTESIAN_POINT('Ctrl Pts',(68.9098725237868,17.2503090604792,12.));
#171927=CARTESIAN_POINT('Ctrl Pts',(68.9319057029407,17.248877910643,12.));
#171928=CARTESIAN_POINT('Ctrl Pts',(68.9539843211618,17.2474212398275,12.));
#171929=CARTESIAN_POINT('Ctrl Pts',(68.9761082282922,17.2459389857327,12.));
#171930=CARTESIAN_POINT('Ctrl Pts',(68.9982772748694,17.2444310864585,12.));
#171931=CARTESIAN_POINT('Ctrl Pts',(69.0204913121226,17.2428974805043,12.));
#171932=CARTESIAN_POINT('Ctrl Pts',(69.0427501919636,17.2413381067722,12.));
#171933=CARTESIAN_POINT('Ctrl Pts',(69.0650537669859,17.2397529045587,12.));
#171934=CARTESIAN_POINT('Ctrl Pts',(69.0874018904598,17.238141813549,12.));
#171935=CARTESIAN_POINT('Ctrl Pts',(69.1097944163243,17.2365047738125,12.));
#171936=CARTESIAN_POINT('Ctrl Pts',(69.1322311991759,17.2348417258017,12.));
#171937=CARTESIAN_POINT('Ctrl Pts',(69.1547120942542,17.2331526103511,12.));
#171938=CARTESIAN_POINT('Ctrl Pts',(69.1772369574462,17.2314373686705,12.));
#171939=CARTESIAN_POINT('Ctrl Pts',(69.1998056452837,17.229695942341,12.));
#171940=CARTESIAN_POINT('Ctrl Pts',(69.2224180149377,17.2279282733119,12.));
#171941=CARTESIAN_POINT('Ctrl Pts',(69.2450739242092,17.2261343039015,12.));
#171942=CARTESIAN_POINT('Ctrl Pts',(69.26777323152,17.2243139767963,12.));
#171943=CARTESIAN_POINT('Ctrl Pts',(69.2905157959142,17.2224672350432,12.));
#171944=CARTESIAN_POINT('Ctrl Pts',(69.3133014770541,17.2205940220455,12.));
#171945=CARTESIAN_POINT('Ctrl Pts',(69.3361301352149,17.2186942815604,12.));
#171946=CARTESIAN_POINT('Ctrl Pts',(69.359001631272,17.2167679576991,12.));
#171947=CARTESIAN_POINT('Ctrl Pts',(69.3819158266955,17.2148149949261,12.));
#171948=CARTESIAN_POINT('Ctrl Pts',(69.4048725835516,17.2128353380511,12.));
#171949=CARTESIAN_POINT('Ctrl Pts',(69.4278717644989,17.2108289322258,12.));
#171950=CARTESIAN_POINT('Ctrl Pts',(69.4509132327836,17.208795722942,12.));
#171951=CARTESIAN_POINT('Ctrl Pts',(69.4739968522271,17.2067356560326,12.));
#171952=CARTESIAN_POINT('Ctrl Pts',(69.497122487222,17.2046486776697,12.));
#171953=CARTESIAN_POINT('Ctrl Pts',(69.5202900027329,17.2025347343568,12.));
#171954=CARTESIAN_POINT('Ctrl Pts',(69.5434992642932,17.2003937729266,12.));
#171955=CARTESIAN_POINT('Ctrl Pts',(69.5667501379984,17.198225740538,12.));
#171956=CARTESIAN_POINT('Ctrl Pts',(69.5900424904954,17.1960305846787,12.));
#171957=CARTESIAN_POINT('Ctrl Pts',(69.6133761889787,17.193808253162,12.));
#171958=CARTESIAN_POINT('Ctrl Pts',(69.6367511011927,17.1915586941198,12.));
#171959=CARTESIAN_POINT('Ctrl Pts',(69.6601670954277,17.1892818560004,12.));
#171960=CARTESIAN_POINT('Ctrl Pts',(69.6836240405152,17.1869776875663,12.));
#171961=CARTESIAN_POINT('Ctrl Pts',(69.7071218058149,17.1846461378966,12.));
#171962=CARTESIAN_POINT('Ctrl Pts',(69.7306602612125,17.1822871563835,12.));
#171963=CARTESIAN_POINT('Ctrl Pts',(69.7542392771216,17.1799006927256,12.));
#171964=CARTESIAN_POINT('Ctrl Pts',(69.7778587244788,17.1774866969256,12.));
#171965=CARTESIAN_POINT('Ctrl Pts',(69.8015184747404,17.1750451192887,12.));
#171966=CARTESIAN_POINT('Ctrl Pts',(69.8252183998713,17.1725759104254,12.));
#171967=CARTESIAN_POINT('Ctrl Pts',(69.8489583723417,17.1700790212476,12.));
#171968=CARTESIAN_POINT('Ctrl Pts',(69.8727382651292,17.1675544029622,12.));
#171969=CARTESIAN_POINT('Ctrl Pts',(69.8965579517147,17.1650020070686,12.));
#171970=CARTESIAN_POINT('Ctrl Pts',(69.9204173060779,17.1624217853577,12.));
#171971=CARTESIAN_POINT('Ctrl Pts',(69.9443162026865,17.1598136899144,12.));
#171972=CARTESIAN_POINT('Ctrl Pts',(69.9682545164942,17.157177673114,12.));
#171973=CARTESIAN_POINT('Ctrl Pts',(69.9922321229428,17.1545136876162,12.));
#171974=CARTESIAN_POINT('Ctrl Pts',(70.0162488979587,17.1518216863624,12.));
#171975=CARTESIAN_POINT('Ctrl Pts',(70.0403047179481,17.1491016225748,12.));
#171976=CARTESIAN_POINT('Ctrl Pts',(70.0643994597865,17.1463534497592,12.));
#171977=CARTESIAN_POINT('Ctrl Pts',(70.0885330008169,17.1435771217015,12.));
#171978=CARTESIAN_POINT('Ctrl Pts',(70.1127052188515,17.1407725924615,12.));
#171979=CARTESIAN_POINT('Ctrl Pts',(70.1369159921686,17.1379398163708,12.));
#171980=CARTESIAN_POINT('Ctrl Pts',(70.1611651995085,17.1350787480313,12.));
#171981=CARTESIAN_POINT('Ctrl Pts',(70.1854527200636,17.1321893423183,12.));
#171982=CARTESIAN_POINT('Ctrl Pts',(70.2097784334749,17.1292715543779,12.));
#171983=CARTESIAN_POINT('Ctrl Pts',(70.2341422198363,17.1263253396202,12.));
#171984=CARTESIAN_POINT('Ctrl Pts',(70.2585439596899,17.1233506537176,12.));
#171985=CARTESIAN_POINT('Ctrl Pts',(70.2829835340239,17.1203474526031,12.));
#171986=CARTESIAN_POINT('Ctrl Pts',(70.3074608242613,17.1173156924734,12.));
#171987=CARTESIAN_POINT('Ctrl Pts',(70.3319757122577,17.1142553297869,12.));
#171988=CARTESIAN_POINT('Ctrl Pts',(70.356528080303,17.111166321257,12.));
#171989=CARTESIAN_POINT('Ctrl Pts',(70.3811178111206,17.10804862385,12.));
#171990=CARTESIAN_POINT('Ctrl Pts',(70.4057447878621,17.1049021947833,12.));
#171991=CARTESIAN_POINT('Ctrl Pts',(70.4304088940998,17.1017269915289,12.));
#171992=CARTESIAN_POINT('Ctrl Pts',(70.4551100138221,17.098522971812,12.));
#171993=CARTESIAN_POINT('Ctrl Pts',(70.4798480314364,17.0952900936044,12.));
#171994=CARTESIAN_POINT('Ctrl Pts',(70.5046228317669,17.0920283151217,12.));
#171995=CARTESIAN_POINT('Ctrl Pts',(70.5294343000516,17.0887375948221,12.));
#171996=CARTESIAN_POINT('Ctrl Pts',(70.5542823219346,17.085417891409,12.));
#171997=CARTESIAN_POINT('Ctrl Pts',(70.5791667834599,17.0820691638314,12.));
#171998=CARTESIAN_POINT('Ctrl Pts',(70.6040875710762,17.0786913712767,12.));
#171999=CARTESIAN_POINT('Ctrl Pts',(70.6290445716341,17.0752844731679,12.));
#172000=CARTESIAN_POINT('Ctrl Pts',(70.6540376723839,17.0718484291623,12.));
#172001=CARTESIAN_POINT('Ctrl Pts',(70.6790667609678,17.0683831991532,12.));
#172002=CARTESIAN_POINT('Ctrl Pts',(70.7041317254128,17.0648887432714,12.));
#172003=CARTESIAN_POINT('Ctrl Pts',(70.7292324541348,17.0613650218789,12.));
#172004=CARTESIAN_POINT('Ctrl Pts',(70.754368835938,17.0578119955651,12.));
#172005=CARTESIAN_POINT('Ctrl Pts',(70.7795407600127,17.0542296251462,12.));
#172006=CARTESIAN_POINT('Ctrl Pts',(70.8047481159298,17.0506178716662,12.));
#172007=CARTESIAN_POINT('Ctrl Pts',(70.8299907936334,17.0469766964001,12.));
#172008=CARTESIAN_POINT('Ctrl Pts',(70.8552686834423,17.0433060608475,12.));
#172009=CARTESIAN_POINT('Ctrl Pts',(70.8805816760501,17.0396059267277,12.));
#172010=CARTESIAN_POINT('Ctrl Pts',(70.9059296625214,17.0358762559786,12.));
#172011=CARTESIAN_POINT('Ctrl Pts',(70.9313125342876,17.0321170107564,12.));
#172012=CARTESIAN_POINT('Ctrl Pts',(70.956730183136,17.0283281534392,12.));
#172013=CARTESIAN_POINT('Ctrl Pts',(70.9821825012136,17.0245096466229,12.));
#172014=CARTESIAN_POINT('Ctrl Pts',(71.0076693810301,17.0206614531166,12.));
#172015=CARTESIAN_POINT('Ctrl Pts',(71.0331907154574,17.0167835359419,12.));
#172016=CARTESIAN_POINT('Ctrl Pts',(71.0587463977268,17.0128758583335,12.));
#172017=CARTESIAN_POINT('Ctrl Pts',(71.0843363214221,17.0089383837437,12.));
#172018=CARTESIAN_POINT('Ctrl Pts',(71.1099603804786,17.0049710758394,12.));
#172019=CARTESIAN_POINT('Ctrl Pts',(71.1356184691806,17.0009738984936,12.));
#172020=CARTESIAN_POINT('Ctrl Pts',(71.1613104821568,16.9969468157824,12.));
#172021=CARTESIAN_POINT('Ctrl Pts',(71.187036314374,16.9928897919828,12.));
#172022=CARTESIAN_POINT('Ctrl Pts',(71.212795861124,16.9888027915742,12.));
#172023=CARTESIAN_POINT('Ctrl Pts',(71.2385890180221,16.9846857792384,12.));
#172024=CARTESIAN_POINT('Ctrl Pts',(71.2644156810198,16.9805387198571,12.));
#172025=CARTESIAN_POINT('Ctrl Pts',(71.290275746412,16.9763615785137,12.));
#172026=CARTESIAN_POINT('Ctrl Pts',(71.3161691108427,16.9721543204951,12.));
#172027=CARTESIAN_POINT('Ctrl Pts',(71.3420956713082,16.9679169112994,12.));
#172028=CARTESIAN_POINT('Ctrl Pts',(71.3680553251562,16.9636493166397,12.));
#172029=CARTESIAN_POINT('Ctrl Pts',(71.3940479700677,16.9593515024276,12.));
#172030=CARTESIAN_POINT('Ctrl Pts',(71.4200735040384,16.9550234347621,12.));
#172031=CARTESIAN_POINT('Ctrl Pts',(71.4461318253563,16.9506650799189,12.));
#172032=CARTESIAN_POINT('Ctrl Pts',(71.4722228325794,16.9462764043443,12.));
#172033=CARTESIAN_POINT('Ctrl Pts',(71.4983464245055,16.9418573746489,12.));
#172034=CARTESIAN_POINT('Ctrl Pts',(71.5245025002139,16.9374079576201,12.));
#172035=CARTESIAN_POINT('Ctrl Pts',(71.5506909591129,16.9329281202377,12.));
#172036=CARTESIAN_POINT('Ctrl Pts',(71.5769117009842,16.9284178296933,12.));
#172037=CARTESIAN_POINT('Ctrl Pts',(71.6031646260174,16.9238770534071,12.));
#172038=CARTESIAN_POINT('Ctrl Pts',(71.6294496348653,16.9193057590607,12.));
#172039=CARTESIAN_POINT('Ctrl Pts',(71.6557666285917,16.9147039145717,12.));
#172040=CARTESIAN_POINT('Ctrl Pts',(71.6821155085612,16.9100714880368,12.));
#172041=CARTESIAN_POINT('Ctrl Pts',(71.7084961763357,16.9054084476847,12.));
#172042=CARTESIAN_POINT('Ctrl Pts',(71.7349085335796,16.9007147618344,12.));
#172043=CARTESIAN_POINT('Ctrl Pts',(71.7613524819235,16.895990398841,12.));
#172044=CARTESIAN_POINT('Ctrl Pts',(71.7878279229546,16.8912353270942,12.));
#172045=CARTESIAN_POINT('Ctrl Pts',(71.8143347584962,16.8864495151344,12.));
#172046=CARTESIAN_POINT('Ctrl Pts',(71.8408728908258,16.8816329317471,12.));
#172047=CARTESIAN_POINT('Ctrl Pts',(71.867442222915,16.87678554607,12.));
#172048=CARTESIAN_POINT('Ctrl Pts',(71.8940426586534,16.871907327697,12.));
#172049=CARTESIAN_POINT('Ctrl Pts',(71.9206741030887,16.866998246792,12.));
#172050=CARTESIAN_POINT('Ctrl Pts',(71.9473364618922,16.8620582738437,12.));
#172051=CARTESIAN_POINT('Ctrl Pts',(71.9740296408347,16.8570873794269,12.));
#172052=CARTESIAN_POINT('Ctrl Pts',(72.0007535452081,16.8520855339446,12.));
#172053=CARTESIAN_POINT('Ctrl Pts',(72.0275080793727,16.8470527074275,12.));
#172054=CARTESIAN_POINT('Ctrl Pts',(72.0542931459825,16.8419888691976,12.));
#172055=CARTESIAN_POINT('Ctrl Pts',(72.0811086466121,16.8368939881446,12.));
#172056=CARTESIAN_POINT('Ctrl Pts',(72.1079544831513,16.8317680333404,12.));
#172057=CARTESIAN_POINT('Ctrl Pts',(72.13483055902,16.8266109745795,12.));
#172058=CARTESIAN_POINT('Ctrl Pts',(72.1617367803235,16.8214227828943,12.));
#172059=CARTESIAN_POINT('Ctrl Pts',(72.1886730573452,16.8162034312269,12.));
#172060=CARTESIAN_POINT('Ctrl Pts',(72.2156393048975,16.8109528945896,12.));
#172061=CARTESIAN_POINT('Ctrl Pts',(72.2387802230856,16.8064254147776,12.));
#172062=CARTESIAN_POINT('Ctrl Pts',(72.256538003526,16.8029374213794,12.));
#172063=CARTESIAN_POINT('Ctrl Pts',(72.2688994295263,16.8005027425863,12.));
#172064=CARTESIAN_POINT('Ctrl Pts',(72.2758557891328,16.799130531775,12.));
#172065=CARTESIAN_POINT('Ctrl Pts',(72.2774028393913,16.7988252568749,12.));
#172066=CARTESIAN_POINT('',(67.8307641965655,17.2912529479484,0.));
#172067=CARTESIAN_POINT('',(67.8307641965655,17.2912529479484,0.));
#172068=CARTESIAN_POINT('Ctrl Pts',(72.2774028393913,16.7988252568749,0.));
#172069=CARTESIAN_POINT('Ctrl Pts',(72.2758557891328,16.7991305317749,0.));
#172070=CARTESIAN_POINT('Ctrl Pts',(72.2688994295263,16.8005027425863,0.));
#172071=CARTESIAN_POINT('Ctrl Pts',(72.256538003526,16.8029374213794,0.));
#172072=CARTESIAN_POINT('Ctrl Pts',(72.2387802230856,16.8064254147776,0.));
#172073=CARTESIAN_POINT('Ctrl Pts',(72.2156393048975,16.8109528945896,0.));
#172074=CARTESIAN_POINT('Ctrl Pts',(72.1886730573452,16.8162034312269,0.));
#172075=CARTESIAN_POINT('Ctrl Pts',(72.1617367803235,16.8214227828943,0.));
#172076=CARTESIAN_POINT('Ctrl Pts',(72.13483055902,16.8266109745795,0.));
#172077=CARTESIAN_POINT('Ctrl Pts',(72.1079544831513,16.8317680333404,0.));
#172078=CARTESIAN_POINT('Ctrl Pts',(72.0811086466121,16.8368939881446,0.));
#172079=CARTESIAN_POINT('Ctrl Pts',(72.0542931459825,16.8419888691976,0.));
#172080=CARTESIAN_POINT('Ctrl Pts',(72.0275080793727,16.8470527074275,0.));
#172081=CARTESIAN_POINT('Ctrl Pts',(72.0007535452081,16.8520855339446,0.));
#172082=CARTESIAN_POINT('Ctrl Pts',(71.9740296408347,16.8570873794269,0.));
#172083=CARTESIAN_POINT('Ctrl Pts',(71.9473364618922,16.8620582738437,0.));
#172084=CARTESIAN_POINT('Ctrl Pts',(71.9206741030887,16.866998246792,0.));
#172085=CARTESIAN_POINT('Ctrl Pts',(71.8940426586534,16.871907327697,0.));
#172086=CARTESIAN_POINT('Ctrl Pts',(71.867442222915,16.87678554607,0.));
#172087=CARTESIAN_POINT('Ctrl Pts',(71.8408728908258,16.8816329317471,0.));
#172088=CARTESIAN_POINT('Ctrl Pts',(71.8143347584962,16.8864495151344,0.));
#172089=CARTESIAN_POINT('Ctrl Pts',(71.7878279229546,16.8912353270942,0.));
#172090=CARTESIAN_POINT('Ctrl Pts',(71.7613524819235,16.895990398841,0.));
#172091=CARTESIAN_POINT('Ctrl Pts',(71.7349085335796,16.9007147618344,0.));
#172092=CARTESIAN_POINT('Ctrl Pts',(71.7084961763357,16.9054084476847,0.));
#172093=CARTESIAN_POINT('Ctrl Pts',(71.6821155085612,16.9100714880368,0.));
#172094=CARTESIAN_POINT('Ctrl Pts',(71.6557666285917,16.9147039145717,0.));
#172095=CARTESIAN_POINT('Ctrl Pts',(71.6294496348653,16.9193057590607,0.));
#172096=CARTESIAN_POINT('Ctrl Pts',(71.6031646260174,16.9238770534071,0.));
#172097=CARTESIAN_POINT('Ctrl Pts',(71.5769117009842,16.9284178296933,0.));
#172098=CARTESIAN_POINT('Ctrl Pts',(71.5506909591129,16.9329281202377,0.));
#172099=CARTESIAN_POINT('Ctrl Pts',(71.5245025002139,16.9374079576201,0.));
#172100=CARTESIAN_POINT('Ctrl Pts',(71.4983464245055,16.9418573746489,0.));
#172101=CARTESIAN_POINT('Ctrl Pts',(71.4722228325794,16.9462764043443,0.));
#172102=CARTESIAN_POINT('Ctrl Pts',(71.4461318253563,16.9506650799189,0.));
#172103=CARTESIAN_POINT('Ctrl Pts',(71.4200735040384,16.9550234347621,0.));
#172104=CARTESIAN_POINT('Ctrl Pts',(71.3940479700677,16.9593515024276,0.));
#172105=CARTESIAN_POINT('Ctrl Pts',(71.3680553251562,16.9636493166397,0.));
#172106=CARTESIAN_POINT('Ctrl Pts',(71.3420956713082,16.9679169112994,0.));
#172107=CARTESIAN_POINT('Ctrl Pts',(71.3161691108427,16.9721543204951,0.));
#172108=CARTESIAN_POINT('Ctrl Pts',(71.290275746412,16.9763615785137,0.));
#172109=CARTESIAN_POINT('Ctrl Pts',(71.2644156810198,16.9805387198571,0.));
#172110=CARTESIAN_POINT('Ctrl Pts',(71.2385890180221,16.9846857792384,0.));
#172111=CARTESIAN_POINT('Ctrl Pts',(71.212795861124,16.9888027915742,0.));
#172112=CARTESIAN_POINT('Ctrl Pts',(71.187036314374,16.9928897919828,0.));
#172113=CARTESIAN_POINT('Ctrl Pts',(71.1613104821568,16.9969468157824,0.));
#172114=CARTESIAN_POINT('Ctrl Pts',(71.1356184691806,17.0009738984936,0.));
#172115=CARTESIAN_POINT('Ctrl Pts',(71.1099603804786,17.0049710758394,0.));
#172116=CARTESIAN_POINT('Ctrl Pts',(71.0843363214221,17.0089383837437,0.));
#172117=CARTESIAN_POINT('Ctrl Pts',(71.0587463977268,17.0128758583335,0.));
#172118=CARTESIAN_POINT('Ctrl Pts',(71.0331907154574,17.0167835359419,0.));
#172119=CARTESIAN_POINT('Ctrl Pts',(71.0076693810301,17.0206614531166,0.));
#172120=CARTESIAN_POINT('Ctrl Pts',(70.9821825012136,17.0245096466229,0.));
#172121=CARTESIAN_POINT('Ctrl Pts',(70.956730183136,17.0283281534392,0.));
#172122=CARTESIAN_POINT('Ctrl Pts',(70.9313125342876,17.0321170107564,0.));
#172123=CARTESIAN_POINT('Ctrl Pts',(70.9059296625214,17.0358762559786,0.));
#172124=CARTESIAN_POINT('Ctrl Pts',(70.8805816760501,17.0396059267277,0.));
#172125=CARTESIAN_POINT('Ctrl Pts',(70.8552686834423,17.0433060608475,0.));
#172126=CARTESIAN_POINT('Ctrl Pts',(70.8299907936334,17.0469766964001,0.));
#172127=CARTESIAN_POINT('Ctrl Pts',(70.8047481159298,17.0506178716662,0.));
#172128=CARTESIAN_POINT('Ctrl Pts',(70.7795407600127,17.0542296251462,0.));
#172129=CARTESIAN_POINT('Ctrl Pts',(70.754368835938,17.0578119955651,0.));
#172130=CARTESIAN_POINT('Ctrl Pts',(70.7292324541348,17.0613650218789,0.));
#172131=CARTESIAN_POINT('Ctrl Pts',(70.7041317254128,17.0648887432714,0.));
#172132=CARTESIAN_POINT('Ctrl Pts',(70.6790667609678,17.0683831991532,0.));
#172133=CARTESIAN_POINT('Ctrl Pts',(70.6540376723839,17.0718484291623,0.));
#172134=CARTESIAN_POINT('Ctrl Pts',(70.6290445716341,17.0752844731679,0.));
#172135=CARTESIAN_POINT('Ctrl Pts',(70.6040875710762,17.0786913712767,0.));
#172136=CARTESIAN_POINT('Ctrl Pts',(70.5791667834599,17.0820691638314,0.));
#172137=CARTESIAN_POINT('Ctrl Pts',(70.5542823219346,17.085417891409,0.));
#172138=CARTESIAN_POINT('Ctrl Pts',(70.5294343000516,17.0887375948221,0.));
#172139=CARTESIAN_POINT('Ctrl Pts',(70.5046228317669,17.0920283151217,0.));
#172140=CARTESIAN_POINT('Ctrl Pts',(70.4798480314364,17.0952900936044,0.));
#172141=CARTESIAN_POINT('Ctrl Pts',(70.4551100138221,17.098522971812,0.));
#172142=CARTESIAN_POINT('Ctrl Pts',(70.4304088940998,17.1017269915289,0.));
#172143=CARTESIAN_POINT('Ctrl Pts',(70.4057447878621,17.1049021947833,0.));
#172144=CARTESIAN_POINT('Ctrl Pts',(70.3811178111206,17.10804862385,0.));
#172145=CARTESIAN_POINT('Ctrl Pts',(70.356528080303,17.111166321257,0.));
#172146=CARTESIAN_POINT('Ctrl Pts',(70.3319757122577,17.1142553297869,0.));
#172147=CARTESIAN_POINT('Ctrl Pts',(70.3074608242613,17.1173156924734,0.));
#172148=CARTESIAN_POINT('Ctrl Pts',(70.2829835340239,17.1203474526031,0.));
#172149=CARTESIAN_POINT('Ctrl Pts',(70.2585439596899,17.1233506537176,0.));
#172150=CARTESIAN_POINT('Ctrl Pts',(70.2341422198363,17.1263253396202,0.));
#172151=CARTESIAN_POINT('Ctrl Pts',(70.2097784334749,17.1292715543779,0.));
#172152=CARTESIAN_POINT('Ctrl Pts',(70.1854527200636,17.1321893423183,0.));
#172153=CARTESIAN_POINT('Ctrl Pts',(70.1611651995085,17.1350787480313,0.));
#172154=CARTESIAN_POINT('Ctrl Pts',(70.1369159921686,17.1379398163708,0.));
#172155=CARTESIAN_POINT('Ctrl Pts',(70.1127052188515,17.1407725924615,0.));
#172156=CARTESIAN_POINT('Ctrl Pts',(70.0885330008169,17.1435771217015,0.));
#172157=CARTESIAN_POINT('Ctrl Pts',(70.0643994597865,17.1463534497592,0.));
#172158=CARTESIAN_POINT('Ctrl Pts',(70.0403047179481,17.1491016225748,0.));
#172159=CARTESIAN_POINT('Ctrl Pts',(70.0162488979587,17.1518216863624,0.));
#172160=CARTESIAN_POINT('Ctrl Pts',(69.9922321229428,17.1545136876162,0.));
#172161=CARTESIAN_POINT('Ctrl Pts',(69.9682545164942,17.157177673114,0.));
#172162=CARTESIAN_POINT('Ctrl Pts',(69.9443162026865,17.1598136899144,0.));
#172163=CARTESIAN_POINT('Ctrl Pts',(69.9204173060779,17.1624217853577,0.));
#172164=CARTESIAN_POINT('Ctrl Pts',(69.8965579517147,17.1650020070686,0.));
#172165=CARTESIAN_POINT('Ctrl Pts',(69.8727382651292,17.1675544029622,0.));
#172166=CARTESIAN_POINT('Ctrl Pts',(69.8489583723417,17.1700790212476,0.));
#172167=CARTESIAN_POINT('Ctrl Pts',(69.8252183998713,17.1725759104254,0.));
#172168=CARTESIAN_POINT('Ctrl Pts',(69.8015184747404,17.1750451192887,0.));
#172169=CARTESIAN_POINT('Ctrl Pts',(69.7778587244788,17.1774866969256,0.));
#172170=CARTESIAN_POINT('Ctrl Pts',(69.7542392771216,17.1799006927256,0.));
#172171=CARTESIAN_POINT('Ctrl Pts',(69.7306602612125,17.1822871563835,0.));
#172172=CARTESIAN_POINT('Ctrl Pts',(69.7071218058149,17.1846461378966,0.));
#172173=CARTESIAN_POINT('Ctrl Pts',(69.6836240405152,17.1869776875663,0.));
#172174=CARTESIAN_POINT('Ctrl Pts',(69.6601670954277,17.1892818560004,0.));
#172175=CARTESIAN_POINT('Ctrl Pts',(69.6367511011927,17.1915586941198,0.));
#172176=CARTESIAN_POINT('Ctrl Pts',(69.6133761889787,17.193808253162,0.));
#172177=CARTESIAN_POINT('Ctrl Pts',(69.5900424904954,17.1960305846787,0.));
#172178=CARTESIAN_POINT('Ctrl Pts',(69.5667501379984,17.198225740538,0.));
#172179=CARTESIAN_POINT('Ctrl Pts',(69.5434992642932,17.2003937729266,0.));
#172180=CARTESIAN_POINT('Ctrl Pts',(69.5202900027329,17.2025347343568,0.));
#172181=CARTESIAN_POINT('Ctrl Pts',(69.497122487222,17.2046486776697,0.));
#172182=CARTESIAN_POINT('Ctrl Pts',(69.4739968522271,17.2067356560326,0.));
#172183=CARTESIAN_POINT('Ctrl Pts',(69.4509132327836,17.208795722942,0.));
#172184=CARTESIAN_POINT('Ctrl Pts',(69.4278717644989,17.2108289322258,0.));
#172185=CARTESIAN_POINT('Ctrl Pts',(69.4048725835516,17.2128353380511,0.));
#172186=CARTESIAN_POINT('Ctrl Pts',(69.3819158266955,17.2148149949261,0.));
#172187=CARTESIAN_POINT('Ctrl Pts',(69.359001631272,17.2167679576991,0.));
#172188=CARTESIAN_POINT('Ctrl Pts',(69.3361301352149,17.2186942815604,0.));
#172189=CARTESIAN_POINT('Ctrl Pts',(69.3133014770541,17.2205940220455,0.));
#172190=CARTESIAN_POINT('Ctrl Pts',(69.2905157959142,17.2224672350432,0.));
#172191=CARTESIAN_POINT('Ctrl Pts',(69.26777323152,17.2243139767963,0.));
#172192=CARTESIAN_POINT('Ctrl Pts',(69.2450739242092,17.2261343039015,0.));
#172193=CARTESIAN_POINT('Ctrl Pts',(69.2224180149377,17.2279282733119,0.));
#172194=CARTESIAN_POINT('Ctrl Pts',(69.1998056452837,17.229695942341,0.));
#172195=CARTESIAN_POINT('Ctrl Pts',(69.1772369574462,17.2314373686705,0.));
#172196=CARTESIAN_POINT('Ctrl Pts',(69.1547120942542,17.2331526103511,0.));
#172197=CARTESIAN_POINT('Ctrl Pts',(69.1322311991759,17.2348417258017,0.));
#172198=CARTESIAN_POINT('Ctrl Pts',(69.1097944163243,17.2365047738125,0.));
#172199=CARTESIAN_POINT('Ctrl Pts',(69.0874018904598,17.238141813549,0.));
#172200=CARTESIAN_POINT('Ctrl Pts',(69.0650537669859,17.2397529045587,0.));
#172201=CARTESIAN_POINT('Ctrl Pts',(69.0427501919636,17.2413381067722,0.));
#172202=CARTESIAN_POINT('Ctrl Pts',(69.0204913121226,17.2428974805043,0.));
#172203=CARTESIAN_POINT('Ctrl Pts',(68.9982772748694,17.2444310864585,0.));
#172204=CARTESIAN_POINT('Ctrl Pts',(68.9761082282922,17.2459389857327,0.));
#172205=CARTESIAN_POINT('Ctrl Pts',(68.9539843211618,17.2474212398275,0.));
#172206=CARTESIAN_POINT('Ctrl Pts',(68.9319057029407,17.248877910643,0.));
#172207=CARTESIAN_POINT('Ctrl Pts',(68.9098725237868,17.2503090604792,0.));
#172208=CARTESIAN_POINT('Ctrl Pts',(68.8878849345557,17.2517147520376,0.));
#172209=CARTESIAN_POINT('Ctrl Pts',(68.8659430867977,17.2530950484259,0.));
#172210=CARTESIAN_POINT('Ctrl Pts',(68.8440471327563,17.2544500131627,0.));
#172211=CARTESIAN_POINT('Ctrl Pts',(68.8221972253954,17.2557797101816,0.));
#172212=CARTESIAN_POINT('Ctrl Pts',(68.8003935184193,17.2570842038386,0.));
#172213=CARTESIAN_POINT('Ctrl Pts',(68.7786361662876,17.2583635589197,0.));
#172214=CARTESIAN_POINT('Ctrl Pts',(68.7569253242312,17.2596178406545,0.));
#172215=CARTESIAN_POINT('Ctrl Pts',(68.7352611482519,17.2608471147178,0.));
#172216=CARTESIAN_POINT('Ctrl Pts',(68.7136437951075,17.2620514472176,0.));
#172217=CARTESIAN_POINT('Ctrl Pts',(68.6920734222932,17.263230904689,0.));
#172218=CARTESIAN_POINT('Ctrl Pts',(68.6705501880263,17.2643855540896,0.));
#172219=CARTESIAN_POINT('Ctrl Pts',(68.6490742512085,17.2655154627935,0.));
#172220=CARTESIAN_POINT('Ctrl Pts',(68.6276457714757,17.2666206986091,0.));
#172221=CARTESIAN_POINT('Ctrl Pts',(68.6062649092781,17.2677013298061,0.));
#172222=CARTESIAN_POINT('Ctrl Pts',(68.5849318259449,17.2687574251429,0.));
#172223=CARTESIAN_POINT('Ctrl Pts',(68.5636466837502,17.2697890538956,0.));
#172224=CARTESIAN_POINT('Ctrl Pts',(68.5424096459746,17.2707962858912,0.));
#172225=CARTESIAN_POINT('Ctrl Pts',(68.5212208767835,17.2717791914538,0.));
#172226=CARTESIAN_POINT('Ctrl Pts',(68.5000805410897,17.2727378413485,0.));
#172227=CARTESIAN_POINT('Ctrl Pts',(68.4789888044357,17.2736723067367,0.));
#172228=CARTESIAN_POINT('Ctrl Pts',(68.4579458328208,17.2745826591125,0.));
#172229=CARTESIAN_POINT('Ctrl Pts',(68.4369517926803,17.2754689703001,0.));
#172230=CARTESIAN_POINT('Ctrl Pts',(68.4160068512781,17.2763313126026,0.));
#172231=CARTESIAN_POINT('Ctrl Pts',(68.3951111770498,17.2771697589387,0.));
#172232=CARTESIAN_POINT('Ctrl Pts',(68.374264939895,17.2779843829605,0.));
#172233=CARTESIAN_POINT('Ctrl Pts',(68.353468311648,17.2787752592475,0.));
#172234=CARTESIAN_POINT('Ctrl Pts',(68.3327214657533,17.2795424631789,0.));
#172235=CARTESIAN_POINT('Ctrl Pts',(68.3120245763884,17.2802860705807,0.));
#172236=CARTESIAN_POINT('Ctrl Pts',(68.2913778177258,17.2810061574352,0.));
#172237=CARTESIAN_POINT('Ctrl Pts',(68.2707813631761,17.2817027995838,0.));
#172238=CARTESIAN_POINT('Ctrl Pts',(68.250235384512,17.2823760723886,0.));
#172239=CARTESIAN_POINT('Ctrl Pts',(68.2297400535339,17.2830260513879,0.));
#172240=CARTESIAN_POINT('Ctrl Pts',(68.2092955440591,17.2836528130825,0.));
#172241=CARTESIAN_POINT('Ctrl Pts',(68.1889020335418,17.2842564355796,0.));
#172242=CARTESIAN_POINT('Ctrl Pts',(68.1685597054193,17.2848369995283,0.));
#172243=CARTESIAN_POINT('Ctrl Pts',(68.1482687493176,17.2853945882059,0.));
#172244=CARTESIAN_POINT('Ctrl Pts',(68.1280293561473,17.2859292855694,0.));
#172245=CARTESIAN_POINT('Ctrl Pts',(68.1078417137865,17.2864411745456,0.));
#172246=CARTESIAN_POINT('Ctrl Pts',(68.0877060033229,17.2869303355438,0.));
#172247=CARTESIAN_POINT('Ctrl Pts',(68.0676223930469,17.2873968440855,0.));
#172248=CARTESIAN_POINT('Ctrl Pts',(68.0475910442494,17.2878407730981,0.));
#172249=CARTESIAN_POINT('Ctrl Pts',(68.027612122741,17.2882621974737,0.));
#172250=CARTESIAN_POINT('Ctrl Pts',(68.007685808115,17.28866119774,0.));
#172251=CARTESIAN_POINT('Ctrl Pts',(67.9878123049133,17.2890378644843,0.));
#172252=CARTESIAN_POINT('Ctrl Pts',(67.9679918502441,17.2893923013852,0.));
#172253=CARTESIAN_POINT('Ctrl Pts',(67.9482246901517,17.2897246158895,0.));
#172254=CARTESIAN_POINT('Ctrl Pts',(67.9285110571662,17.2900349103956,0.));
#172255=CARTESIAN_POINT('Ctrl Pts',(67.908851149676,17.2903232740717,0.));
#172256=CARTESIAN_POINT('Ctrl Pts',(67.8892451049871,17.2905897724029,0.));
#172257=CARTESIAN_POINT('Ctrl Pts',(67.8696929979178,17.2908344459816,0.));
#172258=CARTESIAN_POINT('Ctrl Pts',(67.8540944890057,17.2910127431203,0.));
#172259=CARTESIAN_POINT('Ctrl Pts',(67.8424198971214,17.2911366591419,0.));
#172260=CARTESIAN_POINT('Ctrl Pts',(67.8346476309106,17.2912149114145,0.));
#172261=CARTESIAN_POINT('Ctrl Pts',(67.8307641965655,17.2912529479484,0.));
#172262=CARTESIAN_POINT('Ctrl Pts',(73.778495580227,10.343287191141,0.));
#172263=CARTESIAN_POINT('Ctrl Pts',(73.778495580227,10.343287191141,12.));
#172264=CARTESIAN_POINT('Ctrl Pts',(73.7731377048058,10.3449014384453,0.));
#172265=CARTESIAN_POINT('Ctrl Pts',(73.7731377048058,10.3449014384453,12.));
#172266=CARTESIAN_POINT('Ctrl Pts',(73.7624245587789,10.3481265449342,0.));
#172267=CARTESIAN_POINT('Ctrl Pts',(73.7624245587789,10.3481265449342,12.));
#172268=CARTESIAN_POINT('Ctrl Pts',(73.7463626541854,10.3529540403092,0.));
#172269=CARTESIAN_POINT('Ctrl Pts',(73.7463626541854,10.3529540403092,12.));
#172270=CARTESIAN_POINT('Ctrl Pts',(73.7249624109173,10.359370371262,0.));
#172271=CARTESIAN_POINT('Ctrl Pts',(73.7249624109173,10.359370371262,12.));
#172272=CARTESIAN_POINT('Ctrl Pts',(73.6982381645206,10.3673568984582,0.));
#172273=CARTESIAN_POINT('Ctrl Pts',(73.6982381645206,10.3673568984582,12.));
#172274=CARTESIAN_POINT('Ctrl Pts',(73.6715399947839,10.3753095356342,0.));
#172275=CARTESIAN_POINT('Ctrl Pts',(73.6715399947839,10.3753095356342,12.));
#172276=CARTESIAN_POINT('Ctrl Pts',(73.6448679350696,10.3832282820371,0.));
#172277=CARTESIAN_POINT('Ctrl Pts',(73.6448679350696,10.3832282820371,12.));
#172278=CARTESIAN_POINT('Ctrl Pts',(73.6182220363156,10.3911131417463,0.));
#172279=CARTESIAN_POINT('Ctrl Pts',(73.6182220363156,10.3911131417463,12.));
#172280=CARTESIAN_POINT('Ctrl Pts',(73.5916023719713,10.3989641265286,0.));
#172281=CARTESIAN_POINT('Ctrl Pts',(73.5916023719713,10.3989641265286,12.));
#172282=CARTESIAN_POINT('Ctrl Pts',(73.5650090359839,10.406781255551,0.));
#172283=CARTESIAN_POINT('Ctrl Pts',(73.5650090359839,10.406781255551,12.));
#172284=CARTESIAN_POINT('Ctrl Pts',(73.5384421354543,10.414564552681,0.));
#172285=CARTESIAN_POINT('Ctrl Pts',(73.5384421354543,10.414564552681,12.));
#172286=CARTESIAN_POINT('Ctrl Pts',(73.5119017847575,10.4223140444605,0.));
#172287=CARTESIAN_POINT('Ctrl Pts',(73.5119017847575,10.4223140444605,12.));
#172288=CARTESIAN_POINT('Ctrl Pts',(73.485388099225,10.4300297578651,0.));
#172289=CARTESIAN_POINT('Ctrl Pts',(73.485388099225,10.4300297578651,12.));
#172290=CARTESIAN_POINT('Ctrl Pts',(73.4589011886197,10.4377117180223,0.));
#172291=CARTESIAN_POINT('Ctrl Pts',(73.4589011886197,10.4377117180223,12.));
#172292=CARTESIAN_POINT('Ctrl Pts',(73.4324411518554,10.4453599463547,0.));
#172293=CARTESIAN_POINT('Ctrl Pts',(73.4324411518554,10.4453599463547,12.));
#172294=CARTESIAN_POINT('Ctrl Pts',(73.4060080806686,10.452974461845,0.));
#172295=CARTESIAN_POINT('Ctrl Pts',(73.4060080806686,10.452974461845,12.));
#172296=CARTESIAN_POINT('Ctrl Pts',(73.37960206225,10.4605552819397,0.));
#172297=CARTESIAN_POINT('Ctrl Pts',(73.37960206225,10.4605552819397,12.));
#172298=CARTESIAN_POINT('Ctrl Pts',(73.3532231823659,10.4681024236289,0.));
#172299=CARTESIAN_POINT('Ctrl Pts',(73.3532231823659,10.4681024236289,12.));
#172300=CARTESIAN_POINT('Ctrl Pts',(73.3268715280575,10.4756159043806,0.));
#172301=CARTESIAN_POINT('Ctrl Pts',(73.3268715280575,10.4756159043806,12.));
#172302=CARTESIAN_POINT('Ctrl Pts',(73.3005471910583,10.4830957433305,0.));
#172303=CARTESIAN_POINT('Ctrl Pts',(73.3005471910583,10.4830957433305,12.));
#172304=CARTESIAN_POINT('Ctrl Pts',(73.2742502674304,10.4905419611523,0.));
#172305=CARTESIAN_POINT('Ctrl Pts',(73.2742502674304,10.4905419611523,12.));
#172306=CARTESIAN_POINT('Ctrl Pts',(73.2479808560189,10.4979545795192,0.));
#172307=CARTESIAN_POINT('Ctrl Pts',(73.2479808560189,10.4979545795192,12.));
#172308=CARTESIAN_POINT('Ctrl Pts',(73.2217390572562,10.5053336206908,0.));
#172309=CARTESIAN_POINT('Ctrl Pts',(73.2217390572562,10.5053336206908,12.));
#172310=CARTESIAN_POINT('Ctrl Pts',(73.1955249719048,10.5126791070805,0.));
#172311=CARTESIAN_POINT('Ctrl Pts',(73.1955249719048,10.5126791070805,12.));
#172312=CARTESIAN_POINT('Ctrl Pts',(73.1693386996138,10.5199910607655,0.));
#172313=CARTESIAN_POINT('Ctrl Pts',(73.1693386996138,10.5199910607655,12.));
#172314=CARTESIAN_POINT('Ctrl Pts',(73.1431803382711,10.5272695032653,0.));
#172315=CARTESIAN_POINT('Ctrl Pts',(73.1431803382711,10.5272695032653,12.));
#172316=CARTESIAN_POINT('Ctrl Pts',(73.1170499848039,10.53451445581,0.));
#172317=CARTESIAN_POINT('Ctrl Pts',(73.1170499848039,10.53451445581,12.));
#172318=CARTESIAN_POINT('Ctrl Pts',(73.0909477356474,10.5417259395003,0.));
#172319=CARTESIAN_POINT('Ctrl Pts',(73.0909477356474,10.5417259395003,12.));
#172320=CARTESIAN_POINT('Ctrl Pts',(73.0648736873434,10.5489039755138,0.));
#172321=CARTESIAN_POINT('Ctrl Pts',(73.0648736873434,10.5489039755138,12.));
#172322=CARTESIAN_POINT('Ctrl Pts',(73.0388279370834,10.5560485852974,0.));
#172323=CARTESIAN_POINT('Ctrl Pts',(73.0388279370834,10.5560485852974,12.));
#172324=CARTESIAN_POINT('Ctrl Pts',(73.0128105832621,10.5631597907651,0.));
#172325=CARTESIAN_POINT('Ctrl Pts',(73.0128105832621,10.5631597907651,12.));
#172326=CARTESIAN_POINT('Ctrl Pts',(72.9868217252283,10.570237614205,0.));
#172327=CARTESIAN_POINT('Ctrl Pts',(72.9868217252283,10.570237614205,12.));
#172328=CARTESIAN_POINT('Ctrl Pts',(72.9608614630534,10.5772820781958,0.));
#172329=CARTESIAN_POINT('Ctrl Pts',(72.9608614630534,10.5772820781958,12.));
#172330=CARTESIAN_POINT('Ctrl Pts',(72.9349298972822,10.5842932055209,0.));
#172331=CARTESIAN_POINT('Ctrl Pts',(72.9349298972822,10.5842932055209,12.));
#172332=CARTESIAN_POINT('Ctrl Pts',(72.9090271287083,10.5912710190928,0.));
#172333=CARTESIAN_POINT('Ctrl Pts',(72.9090271287083,10.5912710190928,12.));
#172334=CARTESIAN_POINT('Ctrl Pts',(72.8831532580845,10.5982155418626,0.));
#172335=CARTESIAN_POINT('Ctrl Pts',(72.8831532580845,10.5982155418626,12.));
#172336=CARTESIAN_POINT('Ctrl Pts',(72.8573083861337,10.6051267968203,0.));
#172337=CARTESIAN_POINT('Ctrl Pts',(72.8573083861337,10.6051267968203,12.));
#172338=CARTESIAN_POINT('Ctrl Pts',(72.8314926136881,10.6120048070368,0.));
#172339=CARTESIAN_POINT('Ctrl Pts',(72.8314926136881,10.6120048070368,12.));
#172340=CARTESIAN_POINT('Ctrl Pts',(72.8057060417887,10.6188495956973,0.));
#172341=CARTESIAN_POINT('Ctrl Pts',(72.8057060417887,10.6188495956973,12.));
#172342=CARTESIAN_POINT('Ctrl Pts',(72.7799487717911,10.6256611861394,0.));
#172343=CARTESIAN_POINT('Ctrl Pts',(72.7799487717911,10.6256611861394,12.));
#172344=CARTESIAN_POINT('Ctrl Pts',(72.7542209054812,10.6324396018998,0.));
#172345=CARTESIAN_POINT('Ctrl Pts',(72.7542209054812,10.6324396018998,12.));
#172346=CARTESIAN_POINT('Ctrl Pts',(72.7285225451293,10.6391848667352,0.));
#172347=CARTESIAN_POINT('Ctrl Pts',(72.7285225451293,10.6391848667352,12.));
#172348=CARTESIAN_POINT('Ctrl Pts',(72.7028537934317,10.6458970045946,0.));
#172349=CARTESIAN_POINT('Ctrl Pts',(72.7028537934317,10.6458970045946,12.));
#172350=CARTESIAN_POINT('Ctrl Pts',(72.6772147534752,10.6525760396054,0.));
#172351=CARTESIAN_POINT('Ctrl Pts',(72.6772147534752,10.6525760396054,12.));
#172352=CARTESIAN_POINT('Ctrl Pts',(72.651605528691,10.6592219960581,0.));
#172353=CARTESIAN_POINT('Ctrl Pts',(72.651605528691,10.6592219960581,12.));
#172354=CARTESIAN_POINT('Ctrl Pts',(72.6260262228065,10.6658348983945,0.));
#172355=CARTESIAN_POINT('Ctrl Pts',(72.6260262228065,10.6658348983945,12.));
#172356=CARTESIAN_POINT('Ctrl Pts',(72.6004769398019,10.6724147711995,0.));
#172357=CARTESIAN_POINT('Ctrl Pts',(72.6004769398019,10.6724147711995,12.));
#172358=CARTESIAN_POINT('Ctrl Pts',(72.5749577839415,10.6789616392042,0.));
#172359=CARTESIAN_POINT('Ctrl Pts',(72.5749577839415,10.6789616392042,12.));
#172360=CARTESIAN_POINT('Ctrl Pts',(72.5494688597961,10.6854755272904,0.));
#172361=CARTESIAN_POINT('Ctrl Pts',(72.5494688597961,10.6854755272904,12.));
#172362=CARTESIAN_POINT('Ctrl Pts',(72.5240102722664,10.691956460499,0.));
#172363=CARTESIAN_POINT('Ctrl Pts',(72.5240102722664,10.691956460499,12.));
#172364=CARTESIAN_POINT('Ctrl Pts',(72.4985821266023,10.6984044640398,0.));
#172365=CARTESIAN_POINT('Ctrl Pts',(72.4985821266023,10.6984044640398,12.));
#172366=CARTESIAN_POINT('Ctrl Pts',(72.4731845284227,10.7048195633061,0.));
#172367=CARTESIAN_POINT('Ctrl Pts',(72.4731845284227,10.7048195633061,12.));
#172368=CARTESIAN_POINT('Ctrl Pts',(72.4478175837156,10.7112017838706,0.));
#172369=CARTESIAN_POINT('Ctrl Pts',(72.4478175837156,10.7112017838706,12.));
#172370=CARTESIAN_POINT('Ctrl Pts',(72.4224813988347,10.7175511514789,0.));
#172371=CARTESIAN_POINT('Ctrl Pts',(72.4224813988347,10.7175511514789,12.));
#172372=CARTESIAN_POINT('Ctrl Pts',(72.3971760804933,10.7238676920469,0.));
#172373=CARTESIAN_POINT('Ctrl Pts',(72.3971760804933,10.7238676920469,12.));
#172374=CARTESIAN_POINT('Ctrl Pts',(72.3719017357571,10.7301514316607,0.));
#172375=CARTESIAN_POINT('Ctrl Pts',(72.3719017357571,10.7301514316607,12.));
#172376=CARTESIAN_POINT('Ctrl Pts',(72.3466584720318,10.73640239658,0.));
#172377=CARTESIAN_POINT('Ctrl Pts',(72.3466584720318,10.73640239658,12.));
#172378=CARTESIAN_POINT('Ctrl Pts',(72.3214463970641,10.7426206132375,0.));
#172379=CARTESIAN_POINT('Ctrl Pts',(72.3214463970641,10.7426206132375,12.));
#172380=CARTESIAN_POINT('Ctrl Pts',(72.2962656189556,10.7488061082368,0.));
#172381=CARTESIAN_POINT('Ctrl Pts',(72.2962656189556,10.7488061082368,12.));
#172382=CARTESIAN_POINT('Ctrl Pts',(72.2711162461681,10.7549589083535,0.));
#172383=CARTESIAN_POINT('Ctrl Pts',(72.2711162461681,10.7549589083535,12.));
#172384=CARTESIAN_POINT('Ctrl Pts',(72.2459983875296,10.7610790405385,0.));
#172385=CARTESIAN_POINT('Ctrl Pts',(72.2459983875296,10.7610790405385,12.));
#172386=CARTESIAN_POINT('Ctrl Pts',(72.2209121522366,10.7671665319255,0.));
#172387=CARTESIAN_POINT('Ctrl Pts',(72.2209121522366,10.7671665319255,12.));
#172388=CARTESIAN_POINT('Ctrl Pts',(72.1958576498557,10.7732214098345,0.));
#172389=CARTESIAN_POINT('Ctrl Pts',(72.1958576498557,10.7732214098345,12.));
#172390=CARTESIAN_POINT('Ctrl Pts',(72.1708349903305,10.7792437017662,0.));
#172391=CARTESIAN_POINT('Ctrl Pts',(72.1708349903305,10.7792437017662,12.));
#172392=CARTESIAN_POINT('Ctrl Pts',(72.1458442839834,10.7852334354016,0.));
#172393=CARTESIAN_POINT('Ctrl Pts',(72.1458442839834,10.7852334354016,12.));
#172394=CARTESIAN_POINT('Ctrl Pts',(72.1208856415171,10.7911906386027,0.));
#172395=CARTESIAN_POINT('Ctrl Pts',(72.1208856415171,10.7911906386027,12.));
#172396=CARTESIAN_POINT('Ctrl Pts',(72.0959591740114,10.7971153394166,0.));
#172397=CARTESIAN_POINT('Ctrl Pts',(72.0959591740114,10.7971153394166,12.));
#172398=CARTESIAN_POINT('Ctrl Pts',(72.0710649929202,10.8030075660809,0.));
#172399=CARTESIAN_POINT('Ctrl Pts',(72.0710649929202,10.8030075660809,12.));
#172400=CARTESIAN_POINT('Ctrl Pts',(72.0462032100815,10.8088673470184,0.));
#172401=CARTESIAN_POINT('Ctrl Pts',(72.0462032100815,10.8088673470184,12.));
#172402=CARTESIAN_POINT('Ctrl Pts',(72.0213739377223,10.8146947108375,0.));
#172403=CARTESIAN_POINT('Ctrl Pts',(72.0213739377223,10.8146947108375,12.));
#172404=CARTESIAN_POINT('Ctrl Pts',(71.9965772884619,10.8204896863328,0.));
#172405=CARTESIAN_POINT('Ctrl Pts',(71.9965772884619,10.8204896863328,12.));
#172406=CARTESIAN_POINT('Ctrl Pts',(71.9718133753127,10.8262523024898,0.));
#172407=CARTESIAN_POINT('Ctrl Pts',(71.9718133753127,10.8262523024898,12.));
#172408=CARTESIAN_POINT('Ctrl Pts',(71.9470823116785,10.8319825884918,0.));
#172409=CARTESIAN_POINT('Ctrl Pts',(71.9470823116785,10.8319825884918,12.));
#172410=CARTESIAN_POINT('Ctrl Pts',(71.9223842113625,10.8376805737159,0.));
#172411=CARTESIAN_POINT('Ctrl Pts',(71.9223842113625,10.8376805737159,12.));
#172412=CARTESIAN_POINT('Ctrl Pts',(71.8977191885725,10.8433462877312,0.));
#172413=CARTESIAN_POINT('Ctrl Pts',(71.8977191885725,10.8433462877312,12.));
#172414=CARTESIAN_POINT('Ctrl Pts',(71.8730873579224,10.8489797602998,0.));
#172415=CARTESIAN_POINT('Ctrl Pts',(71.8730873579224,10.8489797602998,12.));
#172416=CARTESIAN_POINT('Ctrl Pts',(71.8484888344339,10.8545810213799,0.));
#172417=CARTESIAN_POINT('Ctrl Pts',(71.8484888344339,10.8545810213799,12.));
#172418=CARTESIAN_POINT('Ctrl Pts',(71.8239237335331,10.8601501011332,0.));
#172419=CARTESIAN_POINT('Ctrl Pts',(71.8239237335331,10.8601501011332,12.));
#172420=CARTESIAN_POINT('Ctrl Pts',(71.7993921710564,10.865687029922,0.));
#172421=CARTESIAN_POINT('Ctrl Pts',(71.7993921710564,10.865687029922,12.));
#172422=CARTESIAN_POINT('Ctrl Pts',(71.7748942632593,10.8711918383073,0.));
#172423=CARTESIAN_POINT('Ctrl Pts',(71.7748942632593,10.8711918383073,12.));
#172424=CARTESIAN_POINT('Ctrl Pts',(71.7504301268181,10.8766645570497,0.));
#172425=CARTESIAN_POINT('Ctrl Pts',(71.7504301268181,10.8766645570497,12.));
#172426=CARTESIAN_POINT('Ctrl Pts',(71.7259998788328,10.8821052171121,0.));
#172427=CARTESIAN_POINT('Ctrl Pts',(71.7259998788328,10.8821052171121,12.));
#172428=CARTESIAN_POINT('Ctrl Pts',(71.7016036368236,10.8875138496671,0.));
#172429=CARTESIAN_POINT('Ctrl Pts',(71.7016036368236,10.8875138496671,12.));
#172430=CARTESIAN_POINT('Ctrl Pts',(71.6772415187364,10.8928904860964,0.));
#172431=CARTESIAN_POINT('Ctrl Pts',(71.6772415187364,10.8928904860964,12.));
#172432=CARTESIAN_POINT('Ctrl Pts',(71.6529136429504,10.8982351579871,0.));
#172433=CARTESIAN_POINT('Ctrl Pts',(71.6529136429504,10.8982351579871,12.));
#172434=CARTESIAN_POINT('Ctrl Pts',(71.6286201282812,10.9035478971328,0.));
#172435=CARTESIAN_POINT('Ctrl Pts',(71.6286201282812,10.9035478971328,12.));
#172436=CARTESIAN_POINT('Ctrl Pts',(71.6043610939835,10.9088287355365,0.));
#172437=CARTESIAN_POINT('Ctrl Pts',(71.6043610939835,10.9088287355365,12.));
#172438=CARTESIAN_POINT('Ctrl Pts',(71.5801366597488,10.914077705417,0.));
#172439=CARTESIAN_POINT('Ctrl Pts',(71.5801366597488,10.914077705417,12.));
#172440=CARTESIAN_POINT('Ctrl Pts',(71.5559469457091,10.91929483921,0.));
#172441=CARTESIAN_POINT('Ctrl Pts',(71.5559469457091,10.91929483921,12.));
#172442=CARTESIAN_POINT('Ctrl Pts',(71.5317920724459,10.9244801695642,0.));
#172443=CARTESIAN_POINT('Ctrl Pts',(71.5317920724459,10.9244801695642,12.));
#172444=CARTESIAN_POINT('Ctrl Pts',(71.5076721609936,10.9296337293425,0.));
#172445=CARTESIAN_POINT('Ctrl Pts',(71.5076721609936,10.9296337293425,12.));
#172446=CARTESIAN_POINT('Ctrl Pts',(71.4835873328423,10.9347555516235,0.));
#172447=CARTESIAN_POINT('Ctrl Pts',(71.4835873328423,10.9347555516235,12.));
#172448=CARTESIAN_POINT('Ctrl Pts',(71.4595377099351,10.9398456697095,0.));
#172449=CARTESIAN_POINT('Ctrl Pts',(71.4595377099351,10.9398456697095,12.));
#172450=CARTESIAN_POINT('Ctrl Pts',(71.435523414672,10.944904117127,0.));
#172451=CARTESIAN_POINT('Ctrl Pts',(71.435523414672,10.944904117127,12.));
#172452=CARTESIAN_POINT('Ctrl Pts',(71.4115445699194,10.9499309276237,0.));
#172453=CARTESIAN_POINT('Ctrl Pts',(71.4115445699194,10.9499309276237,12.));
#172454=CARTESIAN_POINT('Ctrl Pts',(71.3876012990138,10.954926135169,0.));
#172455=CARTESIAN_POINT('Ctrl Pts',(71.3876012990138,10.954926135169,12.));
#172456=CARTESIAN_POINT('Ctrl Pts',(71.3636937257649,10.9598897739565,0.));
#172457=CARTESIAN_POINT('Ctrl Pts',(71.3636937257649,10.9598897739565,12.));
#172458=CARTESIAN_POINT('Ctrl Pts',(71.339821974454,10.9648218784098,0.));
#172459=CARTESIAN_POINT('Ctrl Pts',(71.339821974454,10.9648218784098,12.));
#172460=CARTESIAN_POINT('Ctrl Pts',(71.3159861698358,10.969722483186,0.));
#172461=CARTESIAN_POINT('Ctrl Pts',(71.3159861698358,10.969722483186,12.));
#172462=CARTESIAN_POINT('Ctrl Pts',(71.2921864371491,10.9745916231709,0.));
#172463=CARTESIAN_POINT('Ctrl Pts',(71.2921864371491,10.9745916231709,12.));
#172464=CARTESIAN_POINT('Ctrl Pts',(71.2684229021207,10.9794293334805,0.));
#172465=CARTESIAN_POINT('Ctrl Pts',(71.2684229021207,10.9794293334805,12.));
#172466=CARTESIAN_POINT('Ctrl Pts',(71.2446956909687,10.9842356494627,0.));
#172467=CARTESIAN_POINT('Ctrl Pts',(71.2446956909687,10.9842356494627,12.));
#172468=CARTESIAN_POINT('Ctrl Pts',(71.2210049304014,10.9890106067039,0.));
#172469=CARTESIAN_POINT('Ctrl Pts',(71.2210049304014,10.9890106067039,12.));
#172470=CARTESIAN_POINT('Ctrl Pts',(71.1973507476191,10.993754241032,0.));
#172471=CARTESIAN_POINT('Ctrl Pts',(71.1973507476191,10.993754241032,12.));
#172472=CARTESIAN_POINT('Ctrl Pts',(71.1737332703248,10.9984665885127,0.));
#172473=CARTESIAN_POINT('Ctrl Pts',(71.1737332703248,10.9984665885127,12.));
#172474=CARTESIAN_POINT('Ctrl Pts',(71.1501526267286,11.0031476854502,0.));
#172475=CARTESIAN_POINT('Ctrl Pts',(71.1501526267286,11.0031476854502,12.));
#172476=CARTESIAN_POINT('Ctrl Pts',(71.1266089455517,11.0077975683895,0.));
#172477=CARTESIAN_POINT('Ctrl Pts',(71.1266089455517,11.0077975683895,12.));
#172478=CARTESIAN_POINT('Ctrl Pts',(71.1031023560249,11.0124162741225,0.));
#172479=CARTESIAN_POINT('Ctrl Pts',(71.1031023560249,11.0124162741225,12.));
#172480=CARTESIAN_POINT('Ctrl Pts',(71.0796329878907,11.0170038396915,0.));
#172481=CARTESIAN_POINT('Ctrl Pts',(71.0796329878907,11.0170038396915,12.));
#172482=CARTESIAN_POINT('Ctrl Pts',(71.0562009714136,11.0215603023856,0.));
#172483=CARTESIAN_POINT('Ctrl Pts',(71.0562009714136,11.0215603023856,12.));
#172484=CARTESIAN_POINT('Ctrl Pts',(71.0328064373856,11.0260856997415,0.));
#172485=CARTESIAN_POINT('Ctrl Pts',(71.0328064373856,11.0260856997415,12.));
#172486=CARTESIAN_POINT('Ctrl Pts',(71.0094495171292,11.0305800695456,0.));
#172487=CARTESIAN_POINT('Ctrl Pts',(71.0094495171292,11.0305800695456,12.));
#172488=CARTESIAN_POINT('Ctrl Pts',(70.986130342497,11.0350434498405,0.));
#172489=CARTESIAN_POINT('Ctrl Pts',(70.986130342497,11.0350434498405,12.));
#172490=CARTESIAN_POINT('Ctrl Pts',(70.9628490458748,11.0394758789285,0.));
#172491=CARTESIAN_POINT('Ctrl Pts',(70.9628490458748,11.0394758789285,12.));
#172492=CARTESIAN_POINT('Ctrl Pts',(70.9396057601924,11.0438773953682,0.));
#172493=CARTESIAN_POINT('Ctrl Pts',(70.9396057601924,11.0438773953682,12.));
#172494=CARTESIAN_POINT('Ctrl Pts',(70.916400618927,11.048248037975,0.));
#172495=CARTESIAN_POINT('Ctrl Pts',(70.916400618927,11.048248037975,12.));
#172496=CARTESIAN_POINT('Ctrl Pts',(70.8932337561087,11.0525878458243,0.));
#172497=CARTESIAN_POINT('Ctrl Pts',(70.8932337561087,11.0525878458243,12.));
#172498=CARTESIAN_POINT('Ctrl Pts',(70.8701053063186,11.0568968582569,0.));
#172499=CARTESIAN_POINT('Ctrl Pts',(70.8701053063186,11.0568968582569,12.));
#172500=CARTESIAN_POINT('Ctrl Pts',(70.8470154046919,11.0611751148835,0.));
#172501=CARTESIAN_POINT('Ctrl Pts',(70.8470154046919,11.0611751148835,12.));
#172502=CARTESIAN_POINT('Ctrl Pts',(70.8239641869299,11.0654226555802,0.));
#172503=CARTESIAN_POINT('Ctrl Pts',(70.8239641869299,11.0654226555802,12.));
#172504=CARTESIAN_POINT('Ctrl Pts',(70.8009517893057,11.0696395204909,0.));
#172505=CARTESIAN_POINT('Ctrl Pts',(70.8009517893057,11.0696395204909,12.));
#172506=CARTESIAN_POINT('Ctrl Pts',(70.7779783486677,11.0738257500291,0.));
#172507=CARTESIAN_POINT('Ctrl Pts',(70.7779783486677,11.0738257500291,12.));
#172508=CARTESIAN_POINT('Ctrl Pts',(70.7550440024384,11.0779813848846,0.));
#172509=CARTESIAN_POINT('Ctrl Pts',(70.7550440024384,11.0779813848846,12.));
#172510=CARTESIAN_POINT('Ctrl Pts',(70.732148888618,11.0821064660269,0.));
#172511=CARTESIAN_POINT('Ctrl Pts',(70.732148888618,11.0821064660269,12.));
#172512=CARTESIAN_POINT('Ctrl Pts',(70.7092931457954,11.0862010347016,0.));
#172513=CARTESIAN_POINT('Ctrl Pts',(70.7092931457954,11.0862010347016,12.));
#172514=CARTESIAN_POINT('Ctrl Pts',(70.6864769131546,11.0902651324323,0.));
#172515=CARTESIAN_POINT('Ctrl Pts',(70.6864769131546,11.0902651324323,12.));
#172516=CARTESIAN_POINT('Ctrl Pts',(70.6637003304785,11.0942988010233,0.));
#172517=CARTESIAN_POINT('Ctrl Pts',(70.6637003304785,11.0942988010233,12.));
#172518=CARTESIAN_POINT('Ctrl Pts',(70.6409635381482,11.0983020825667,0.));
#172519=CARTESIAN_POINT('Ctrl Pts',(70.6409635381482,11.0983020825667,12.));
#172520=CARTESIAN_POINT('Ctrl Pts',(70.6182666771481,11.1022750194446,0.));
#172521=CARTESIAN_POINT('Ctrl Pts',(70.6182666771481,11.1022750194446,12.));
#172522=CARTESIAN_POINT('Ctrl Pts',(70.5956098890773,11.1062176543262,0.));
#172523=CARTESIAN_POINT('Ctrl Pts',(70.5956098890773,11.1062176543262,12.));
#172524=CARTESIAN_POINT('Ctrl Pts',(70.5729933161546,11.1101300301702,0.));
#172525=CARTESIAN_POINT('Ctrl Pts',(70.5729933161546,11.1101300301702,12.));
#172526=CARTESIAN_POINT('Ctrl Pts',(70.5504171012233,11.1140121902271,0.));
#172527=CARTESIAN_POINT('Ctrl Pts',(70.5504171012233,11.1140121902271,12.));
#172528=CARTESIAN_POINT('Ctrl Pts',(70.5278813877494,11.1178641780476,0.));
#172529=CARTESIAN_POINT('Ctrl Pts',(70.5278813877494,11.1178641780476,12.));
#172530=CARTESIAN_POINT('Ctrl Pts',(70.505386319828,11.1216860374826,0.));
#172531=CARTESIAN_POINT('Ctrl Pts',(70.505386319828,11.1216860374826,12.));
#172532=CARTESIAN_POINT('Ctrl Pts',(70.4829320421957,11.1254778126821,0.));
#172533=CARTESIAN_POINT('Ctrl Pts',(70.4829320421957,11.1254778126821,12.));
#172534=CARTESIAN_POINT('Ctrl Pts',(70.4605187002354,11.1292395480974,0.));
#172535=CARTESIAN_POINT('Ctrl Pts',(70.4605187002354,11.1292395480974,12.));
#172536=CARTESIAN_POINT('Ctrl Pts',(70.4381464399819,11.1329712884847,0.));
#172537=CARTESIAN_POINT('Ctrl Pts',(70.4381464399819,11.1329712884847,12.));
#172538=CARTESIAN_POINT('Ctrl Pts',(70.4158154081205,11.1366730789126,0.));
#172539=CARTESIAN_POINT('Ctrl Pts',(70.4158154081205,11.1366730789126,12.));
#172540=CARTESIAN_POINT('Ctrl Pts',(70.393525751996,11.1403449647625,0.));
#172541=CARTESIAN_POINT('Ctrl Pts',(70.393525751996,11.1403449647625,12.));
#172542=CARTESIAN_POINT('Ctrl Pts',(70.3712776196223,11.143986991727,0.));
#172543=CARTESIAN_POINT('Ctrl Pts',(70.3712776196223,11.143986991727,12.));
#172544=CARTESIAN_POINT('Ctrl Pts',(70.349071159688,11.1475992058124,0.));
#172545=CARTESIAN_POINT('Ctrl Pts',(70.349071159688,11.1475992058124,12.));
#172546=CARTESIAN_POINT('Ctrl Pts',(70.326906521559,11.1511816533421,0.));
#172547=CARTESIAN_POINT('Ctrl Pts',(70.326906521559,11.1511816533421,12.));
#172548=CARTESIAN_POINT('Ctrl Pts',(70.3047838552756,11.1547343809646,0.));
#172549=CARTESIAN_POINT('Ctrl Pts',(70.3047838552756,11.1547343809646,12.));
#172550=CARTESIAN_POINT('Ctrl Pts',(70.2827033115662,11.1582574356521,0.));
#172551=CARTESIAN_POINT('Ctrl Pts',(70.2827033115662,11.1582574356521,12.));
#172552=CARTESIAN_POINT('Ctrl Pts',(70.2606650418589,11.1617508647016,0.));
#172553=CARTESIAN_POINT('Ctrl Pts',(70.2606650418589,11.1617508647016,12.));
#172554=CARTESIAN_POINT('Ctrl Pts',(70.2386691982902,11.1652147157383,0.));
#172555=CARTESIAN_POINT('Ctrl Pts',(70.2386691982902,11.1652147157383,12.));
#172556=CARTESIAN_POINT('Ctrl Pts',(70.2167159337094,11.168649036721,0.));
#172557=CARTESIAN_POINT('Ctrl Pts',(70.2167159337094,11.168649036721,12.));
#172558=CARTESIAN_POINT('Ctrl Pts',(70.1948054016816,11.1720538759499,0.));
#172559=CARTESIAN_POINT('Ctrl Pts',(70.1948054016816,11.1720538759499,12.));
#172560=CARTESIAN_POINT('Ctrl Pts',(70.1729377564954,11.1754292820631,0.));
#172561=CARTESIAN_POINT('Ctrl Pts',(70.1729377564954,11.1754292820631,12.));
#172562=CARTESIAN_POINT('Ctrl Pts',(70.1511131531672,11.1787753040363,0.));
#172563=CARTESIAN_POINT('Ctrl Pts',(70.1511131531672,11.1787753040363,12.));
#172564=CARTESIAN_POINT('Ctrl Pts',(70.1293317474432,11.1820919911846,0.));
#172565=CARTESIAN_POINT('Ctrl Pts',(70.1293317474432,11.1820919911846,12.));
#172566=CARTESIAN_POINT('Ctrl Pts',(70.1075936957973,11.185379393167,0.));
#172567=CARTESIAN_POINT('Ctrl Pts',(70.1075936957973,11.185379393167,12.));
#172568=CARTESIAN_POINT('Ctrl Pts',(70.0858991554295,11.1886375599916,0.));
#172569=CARTESIAN_POINT('Ctrl Pts',(70.0858991554295,11.1886375599916,12.));
#172570=CARTESIAN_POINT('Ctrl Pts',(70.0642482842942,11.1918665420168,0.));
#172571=CARTESIAN_POINT('Ctrl Pts',(70.0642482842942,11.1918665420168,12.));
#172572=CARTESIAN_POINT('Ctrl Pts',(70.0426412411194,11.1950663899578,0.));
#172573=CARTESIAN_POINT('Ctrl Pts',(70.0426412411194,11.1950663899578,12.));
#172574=CARTESIAN_POINT('Ctrl Pts',(70.0210781854236,11.1982371548918,0.));
#172575=CARTESIAN_POINT('Ctrl Pts',(70.0210781854236,11.1982371548918,12.));
#172576=CARTESIAN_POINT('Ctrl Pts',(69.9995592775322,11.2013788882711,0.));
#172577=CARTESIAN_POINT('Ctrl Pts',(69.9995592775322,11.2013788882711,12.));
#172578=CARTESIAN_POINT('Ctrl Pts',(69.9780846785771,11.2044916419239,0.));
#172579=CARTESIAN_POINT('Ctrl Pts',(69.9780846785771,11.2044916419239,12.));
#172580=CARTESIAN_POINT('Ctrl Pts',(69.9566545504813,11.2075754680445,0.));
#172581=CARTESIAN_POINT('Ctrl Pts',(69.9566545504813,11.2075754680445,12.));
#172582=CARTESIAN_POINT('Ctrl Pts',(69.9352690559399,11.2106304191881,0.));
#172583=CARTESIAN_POINT('Ctrl Pts',(69.9352690559399,11.2106304191881,12.));
#172584=CARTESIAN_POINT('Ctrl Pts',(69.9139283584036,11.213656548268,0.));
#172585=CARTESIAN_POINT('Ctrl Pts',(69.9139283584036,11.213656548268,12.));
#172586=CARTESIAN_POINT('Ctrl Pts',(69.8926326220414,11.2166539085527,0.));
#172587=CARTESIAN_POINT('Ctrl Pts',(69.8926326220414,11.2166539085527,12.));
#172588=CARTESIAN_POINT('Ctrl Pts',(69.8713820117918,11.2196225536794,0.));
#172589=CARTESIAN_POINT('Ctrl Pts',(69.8713820117918,11.2196225536794,12.));
#172590=CARTESIAN_POINT('Ctrl Pts',(69.8501766934445,11.2225625376739,0.));
#172591=CARTESIAN_POINT('Ctrl Pts',(69.8501766934445,11.2225625376739,12.));
#172592=CARTESIAN_POINT('Ctrl Pts',(69.8290168337076,11.225473914972,0.));
#172593=CARTESIAN_POINT('Ctrl Pts',(69.8290168337076,11.225473914972,12.));
#172594=CARTESIAN_POINT('Ctrl Pts',(69.8079026002753,11.2283567404434,0.));
#172595=CARTESIAN_POINT('Ctrl Pts',(69.8079026002753,11.2283567404434,12.));
#172596=CARTESIAN_POINT('Ctrl Pts',(69.7868341618927,11.2312110694183,0.));
#172597=CARTESIAN_POINT('Ctrl Pts',(69.7868341618927,11.2312110694183,12.));
#172598=CARTESIAN_POINT('Ctrl Pts',(69.7658116882298,11.2340369576452,0.));
#172599=CARTESIAN_POINT('Ctrl Pts',(69.7658116882298,11.2340369576452,12.));
#172600=CARTESIAN_POINT('Ctrl Pts',(69.7448353497394,11.236834461247,0.));
#172601=CARTESIAN_POINT('Ctrl Pts',(69.7448353497394,11.236834461247,12.));
#172602=CARTESIAN_POINT('Ctrl Pts',(69.7239053175362,11.2396036366861,0.));
#172603=CARTESIAN_POINT('Ctrl Pts',(69.7239053175362,11.2396036366861,12.));
#172604=CARTESIAN_POINT('Ctrl Pts',(69.7030217632187,11.242344540717,0.));
#172605=CARTESIAN_POINT('Ctrl Pts',(69.7030217632187,11.242344540717,12.));
#172606=CARTESIAN_POINT('Ctrl Pts',(69.6821848588492,11.2450572303847,0.));
#172607=CARTESIAN_POINT('Ctrl Pts',(69.6821848588492,11.2450572303847,12.));
#172608=CARTESIAN_POINT('Ctrl Pts',(69.6613947773563,11.2477417631391,0.));
#172609=CARTESIAN_POINT('Ctrl Pts',(69.6613947773563,11.2477417631391,12.));
#172610=CARTESIAN_POINT('Ctrl Pts',(69.6406516928902,11.2503981969414,0.));
#172611=CARTESIAN_POINT('Ctrl Pts',(69.6406516928902,11.2503981969414,12.));
#172612=CARTESIAN_POINT('Ctrl Pts',(69.6199557811231,11.2530265903555,0.));
#172613=CARTESIAN_POINT('Ctrl Pts',(69.6199557811231,11.2530265903555,12.));
#172614=CARTESIAN_POINT('Ctrl Pts',(69.5993072197355,11.255627002701,0.));
#172615=CARTESIAN_POINT('Ctrl Pts',(69.5993072197355,11.255627002701,12.));
#172616=CARTESIAN_POINT('Ctrl Pts',(69.5787061880815,11.2581994939534,0.));
#172617=CARTESIAN_POINT('Ctrl Pts',(69.5787061880815,11.2581994939534,12.));
#172618=CARTESIAN_POINT('Ctrl Pts',(69.5581528662846,11.2607441244698,0.));
#172619=CARTESIAN_POINT('Ctrl Pts',(69.5581528662846,11.2607441244698,12.));
#172620=CARTESIAN_POINT('Ctrl Pts',(69.5376474344768,11.2632609547629,0.));
#172621=CARTESIAN_POINT('Ctrl Pts',(69.5376474344768,11.2632609547629,12.));
#172622=CARTESIAN_POINT('Ctrl Pts',(69.5171900720188,11.2657500452721,0.));
#172623=CARTESIAN_POINT('Ctrl Pts',(69.5171900720188,11.2657500452721,12.));
#172624=CARTESIAN_POINT('Ctrl Pts',(69.4967809565978,11.2682114561015,0.));
#172625=CARTESIAN_POINT('Ctrl Pts',(69.4967809565978,11.2682114561015,12.));
#172626=CARTESIAN_POINT('Ctrl Pts',(69.4764202659443,11.2706452475287,0.));
#172627=CARTESIAN_POINT('Ctrl Pts',(69.4764202659443,11.2706452475287,12.));
#172628=CARTESIAN_POINT('Ctrl Pts',(69.4561081798815,11.2730514806143,0.));
#172629=CARTESIAN_POINT('Ctrl Pts',(69.4561081798815,11.2730514806143,12.));
#172630=CARTESIAN_POINT('Ctrl Pts',(69.4358448819957,11.2754302177019,0.));
#172631=CARTESIAN_POINT('Ctrl Pts',(69.4358448819957,11.2754302177019,12.));
#172632=CARTESIAN_POINT('Ctrl Pts',(69.4156305620554,11.2777815231462,0.));
#172633=CARTESIAN_POINT('Ctrl Pts',(69.4156305620554,11.2777815231462,12.));
#172634=CARTESIAN_POINT('Ctrl Pts',(69.395465416223,11.2801054633807,0.));
#172635=CARTESIAN_POINT('Ctrl Pts',(69.395465416223,11.2801054633807,12.));
#172636=CARTESIAN_POINT('Ctrl Pts',(69.375349642,11.2824021054038,0.));
#172637=CARTESIAN_POINT('Ctrl Pts',(69.375349642,11.2824021054038,12.));
#172638=CARTESIAN_POINT('Ctrl Pts',(69.3552834337771,11.2846715154521,0.));
#172639=CARTESIAN_POINT('Ctrl Pts',(69.3552834337771,11.2846715154521,12.));
#172640=CARTESIAN_POINT('Ctrl Pts',(69.3352669789611,11.2869137578463,0.));
#172641=CARTESIAN_POINT('Ctrl Pts',(69.3352669789611,11.2869137578463,12.));
#172642=CARTESIAN_POINT('Ctrl Pts',(69.315300451784,11.2891288931528,0.));
#172643=CARTESIAN_POINT('Ctrl Pts',(69.315300451784,11.2891288931528,12.));
#172644=CARTESIAN_POINT('Ctrl Pts',(69.2953840192792,11.2913169799642,0.));
#172645=CARTESIAN_POINT('Ctrl Pts',(69.2953840192792,11.2913169799642,12.));
#172646=CARTESIAN_POINT('Ctrl Pts',(69.2755178531534,11.2934780784362,0.));
#172647=CARTESIAN_POINT('Ctrl Pts',(69.2755178531534,11.2934780784362,12.));
#172648=CARTESIAN_POINT('Ctrl Pts',(69.255702139335,11.2956122531375,0.));
#172649=CARTESIAN_POINT('Ctrl Pts',(69.255702139335,11.2956122531375,12.));
#172650=CARTESIAN_POINT('Ctrl Pts',(69.2359370894828,11.2977195764836,0.));
#172651=CARTESIAN_POINT('Ctrl Pts',(69.2359370894828,11.2977195764836,12.));
#172652=CARTESIAN_POINT('Ctrl Pts',(69.216222948839,11.2998001310934,0.));
#172653=CARTESIAN_POINT('Ctrl Pts',(69.216222948839,11.2998001310934,12.));
#172654=CARTESIAN_POINT('Ctrl Pts',(69.1965599718761,11.3018540025605,0.));
#172655=CARTESIAN_POINT('Ctrl Pts',(69.1965599718761,11.3018540025605,12.));
#172656=CARTESIAN_POINT('Ctrl Pts',(69.1769483991639,11.3038812726275,0.));
#172657=CARTESIAN_POINT('Ctrl Pts',(69.1769483991639,11.3038812726275,12.));
#172658=CARTESIAN_POINT('Ctrl Pts',(69.1573884361076,11.3058820128323,0.));
#172659=CARTESIAN_POINT('Ctrl Pts',(69.1573884361076,11.3058820128323,12.));
#172660=CARTESIAN_POINT('Ctrl Pts',(69.137880225198,11.3078562764442,0.));
#172661=CARTESIAN_POINT('Ctrl Pts',(69.137880225198,11.3078562764442,12.));
#172662=CARTESIAN_POINT('Ctrl Pts',(69.1184238445065,11.3098040973799,0.));
#172663=CARTESIAN_POINT('Ctrl Pts',(69.1184238445065,11.3098040973799,12.));
#172664=CARTESIAN_POINT('Ctrl Pts',(69.1029002322497,11.3113412156742,0.));
#172665=CARTESIAN_POINT('Ctrl Pts',(69.1029002322497,11.3113412156742,12.));
#172666=CARTESIAN_POINT('Ctrl Pts',(69.0912808657051,11.3124821678849,0.));
#172667=CARTESIAN_POINT('Ctrl Pts',(69.0912808657051,11.3124821678849,12.));
#172668=CARTESIAN_POINT('Ctrl Pts',(69.0835449954486,11.3132375200184,0.));
#172669=CARTESIAN_POINT('Ctrl Pts',(69.0835449954486,11.3132375200184,12.));
#172670=CARTESIAN_POINT('Ctrl Pts',(69.079679653846,11.3136138754165,0.));
#172671=CARTESIAN_POINT('Ctrl Pts',(69.079679653846,11.3136138754165,12.));
#172672=CARTESIAN_POINT('',(69.079679653846,11.3136138754165,12.));
#172673=CARTESIAN_POINT('Ctrl Pts',(69.079679653846,11.3136138754165,12.));
#172674=CARTESIAN_POINT('Ctrl Pts',(69.0835449954486,11.3132375200184,12.));
#172675=CARTESIAN_POINT('Ctrl Pts',(69.0912808657051,11.3124821678849,12.));
#172676=CARTESIAN_POINT('Ctrl Pts',(69.1029002322497,11.3113412156742,12.));
#172677=CARTESIAN_POINT('Ctrl Pts',(69.1184238445065,11.3098040973799,12.));
#172678=CARTESIAN_POINT('Ctrl Pts',(69.137880225198,11.3078562764442,12.));
#172679=CARTESIAN_POINT('Ctrl Pts',(69.1573884361076,11.3058820128323,12.));
#172680=CARTESIAN_POINT('Ctrl Pts',(69.1769483991639,11.3038812726275,12.));
#172681=CARTESIAN_POINT('Ctrl Pts',(69.1965599718761,11.3018540025605,12.));
#172682=CARTESIAN_POINT('Ctrl Pts',(69.216222948839,11.2998001310934,12.));
#172683=CARTESIAN_POINT('Ctrl Pts',(69.2359370894828,11.2977195764836,12.));
#172684=CARTESIAN_POINT('Ctrl Pts',(69.255702139335,11.2956122531375,12.));
#172685=CARTESIAN_POINT('Ctrl Pts',(69.2755178531534,11.2934780784362,12.));
#172686=CARTESIAN_POINT('Ctrl Pts',(69.2953840192792,11.2913169799642,12.));
#172687=CARTESIAN_POINT('Ctrl Pts',(69.315300451784,11.2891288931528,12.));
#172688=CARTESIAN_POINT('Ctrl Pts',(69.3352669789611,11.2869137578463,12.));
#172689=CARTESIAN_POINT('Ctrl Pts',(69.3552834337771,11.2846715154521,12.));
#172690=CARTESIAN_POINT('Ctrl Pts',(69.375349642,11.2824021054038,12.));
#172691=CARTESIAN_POINT('Ctrl Pts',(69.395465416223,11.2801054633807,12.));
#172692=CARTESIAN_POINT('Ctrl Pts',(69.4156305620554,11.2777815231462,12.));
#172693=CARTESIAN_POINT('Ctrl Pts',(69.4358448819957,11.2754302177019,12.));
#172694=CARTESIAN_POINT('Ctrl Pts',(69.4561081798815,11.2730514806143,12.));
#172695=CARTESIAN_POINT('Ctrl Pts',(69.4764202659443,11.2706452475287,12.));
#172696=CARTESIAN_POINT('Ctrl Pts',(69.4967809565978,11.2682114561015,12.));
#172697=CARTESIAN_POINT('Ctrl Pts',(69.5171900720188,11.2657500452721,12.));
#172698=CARTESIAN_POINT('Ctrl Pts',(69.5376474344768,11.2632609547629,12.));
#172699=CARTESIAN_POINT('Ctrl Pts',(69.5581528662846,11.2607441244698,12.));
#172700=CARTESIAN_POINT('Ctrl Pts',(69.5787061880815,11.2581994939534,12.));
#172701=CARTESIAN_POINT('Ctrl Pts',(69.5993072197355,11.255627002701,12.));
#172702=CARTESIAN_POINT('Ctrl Pts',(69.6199557811231,11.2530265903555,12.));
#172703=CARTESIAN_POINT('Ctrl Pts',(69.6406516928902,11.2503981969414,12.));
#172704=CARTESIAN_POINT('Ctrl Pts',(69.6613947773563,11.2477417631391,12.));
#172705=CARTESIAN_POINT('Ctrl Pts',(69.6821848588492,11.2450572303847,12.));
#172706=CARTESIAN_POINT('Ctrl Pts',(69.7030217632187,11.242344540717,12.));
#172707=CARTESIAN_POINT('Ctrl Pts',(69.7239053175362,11.2396036366861,12.));
#172708=CARTESIAN_POINT('Ctrl Pts',(69.7448353497394,11.236834461247,12.));
#172709=CARTESIAN_POINT('Ctrl Pts',(69.7658116882298,11.2340369576452,12.));
#172710=CARTESIAN_POINT('Ctrl Pts',(69.7868341618927,11.2312110694183,12.));
#172711=CARTESIAN_POINT('Ctrl Pts',(69.8079026002753,11.2283567404434,12.));
#172712=CARTESIAN_POINT('Ctrl Pts',(69.8290168337076,11.225473914972,12.));
#172713=CARTESIAN_POINT('Ctrl Pts',(69.8501766934445,11.2225625376739,12.));
#172714=CARTESIAN_POINT('Ctrl Pts',(69.8713820117918,11.2196225536794,12.));
#172715=CARTESIAN_POINT('Ctrl Pts',(69.8926326220414,11.2166539085527,12.));
#172716=CARTESIAN_POINT('Ctrl Pts',(69.9139283584036,11.213656548268,12.));
#172717=CARTESIAN_POINT('Ctrl Pts',(69.9352690559399,11.2106304191881,12.));
#172718=CARTESIAN_POINT('Ctrl Pts',(69.9566545504813,11.2075754680445,12.));
#172719=CARTESIAN_POINT('Ctrl Pts',(69.9780846785771,11.2044916419239,12.));
#172720=CARTESIAN_POINT('Ctrl Pts',(69.9995592775322,11.2013788882711,12.));
#172721=CARTESIAN_POINT('Ctrl Pts',(70.0210781854236,11.1982371548918,12.));
#172722=CARTESIAN_POINT('Ctrl Pts',(70.0426412411194,11.1950663899578,12.));
#172723=CARTESIAN_POINT('Ctrl Pts',(70.0642482842942,11.1918665420168,12.));
#172724=CARTESIAN_POINT('Ctrl Pts',(70.0858991554295,11.1886375599916,12.));
#172725=CARTESIAN_POINT('Ctrl Pts',(70.1075936957973,11.185379393167,12.));
#172726=CARTESIAN_POINT('Ctrl Pts',(70.1293317474432,11.1820919911846,12.));
#172727=CARTESIAN_POINT('Ctrl Pts',(70.1511131531672,11.1787753040363,12.));
#172728=CARTESIAN_POINT('Ctrl Pts',(70.1729377564954,11.1754292820631,12.));
#172729=CARTESIAN_POINT('Ctrl Pts',(70.1948054016816,11.1720538759499,12.));
#172730=CARTESIAN_POINT('Ctrl Pts',(70.2167159337094,11.168649036721,12.));
#172731=CARTESIAN_POINT('Ctrl Pts',(70.2386691982902,11.1652147157383,12.));
#172732=CARTESIAN_POINT('Ctrl Pts',(70.2606650418589,11.1617508647016,12.));
#172733=CARTESIAN_POINT('Ctrl Pts',(70.2827033115662,11.1582574356521,12.));
#172734=CARTESIAN_POINT('Ctrl Pts',(70.3047838552756,11.1547343809646,12.));
#172735=CARTESIAN_POINT('Ctrl Pts',(70.326906521559,11.1511816533421,12.));
#172736=CARTESIAN_POINT('Ctrl Pts',(70.349071159688,11.1475992058124,12.));
#172737=CARTESIAN_POINT('Ctrl Pts',(70.3712776196223,11.143986991727,12.));
#172738=CARTESIAN_POINT('Ctrl Pts',(70.393525751996,11.1403449647625,12.));
#172739=CARTESIAN_POINT('Ctrl Pts',(70.4158154081205,11.1366730789126,12.));
#172740=CARTESIAN_POINT('Ctrl Pts',(70.4381464399819,11.1329712884847,12.));
#172741=CARTESIAN_POINT('Ctrl Pts',(70.4605187002354,11.1292395480974,12.));
#172742=CARTESIAN_POINT('Ctrl Pts',(70.4829320421957,11.1254778126821,12.));
#172743=CARTESIAN_POINT('Ctrl Pts',(70.505386319828,11.1216860374826,12.));
#172744=CARTESIAN_POINT('Ctrl Pts',(70.5278813877494,11.1178641780476,12.));
#172745=CARTESIAN_POINT('Ctrl Pts',(70.5504171012233,11.1140121902271,12.));
#172746=CARTESIAN_POINT('Ctrl Pts',(70.5729933161546,11.1101300301702,12.));
#172747=CARTESIAN_POINT('Ctrl Pts',(70.5956098890773,11.1062176543262,12.));
#172748=CARTESIAN_POINT('Ctrl Pts',(70.6182666771481,11.1022750194446,12.));
#172749=CARTESIAN_POINT('Ctrl Pts',(70.6409635381482,11.0983020825667,12.));
#172750=CARTESIAN_POINT('Ctrl Pts',(70.6637003304785,11.0942988010233,12.));
#172751=CARTESIAN_POINT('Ctrl Pts',(70.6864769131546,11.0902651324323,12.));
#172752=CARTESIAN_POINT('Ctrl Pts',(70.7092931457954,11.0862010347016,12.));
#172753=CARTESIAN_POINT('Ctrl Pts',(70.732148888618,11.0821064660269,12.));
#172754=CARTESIAN_POINT('Ctrl Pts',(70.7550440024384,11.0779813848846,12.));
#172755=CARTESIAN_POINT('Ctrl Pts',(70.7779783486677,11.0738257500291,12.));
#172756=CARTESIAN_POINT('Ctrl Pts',(70.8009517893057,11.0696395204909,12.));
#172757=CARTESIAN_POINT('Ctrl Pts',(70.8239641869299,11.0654226555802,12.));
#172758=CARTESIAN_POINT('Ctrl Pts',(70.8470154046919,11.0611751148835,12.));
#172759=CARTESIAN_POINT('Ctrl Pts',(70.8701053063186,11.0568968582569,12.));
#172760=CARTESIAN_POINT('Ctrl Pts',(70.8932337561087,11.0525878458243,12.));
#172761=CARTESIAN_POINT('Ctrl Pts',(70.916400618927,11.048248037975,12.));
#172762=CARTESIAN_POINT('Ctrl Pts',(70.9396057601924,11.0438773953682,12.));
#172763=CARTESIAN_POINT('Ctrl Pts',(70.9628490458748,11.0394758789285,12.));
#172764=CARTESIAN_POINT('Ctrl Pts',(70.986130342497,11.0350434498405,12.));
#172765=CARTESIAN_POINT('Ctrl Pts',(71.0094495171292,11.0305800695456,12.));
#172766=CARTESIAN_POINT('Ctrl Pts',(71.0328064373856,11.0260856997415,12.));
#172767=CARTESIAN_POINT('Ctrl Pts',(71.0562009714136,11.0215603023856,12.));
#172768=CARTESIAN_POINT('Ctrl Pts',(71.0796329878907,11.0170038396915,12.));
#172769=CARTESIAN_POINT('Ctrl Pts',(71.1031023560249,11.0124162741225,12.));
#172770=CARTESIAN_POINT('Ctrl Pts',(71.1266089455517,11.0077975683895,12.));
#172771=CARTESIAN_POINT('Ctrl Pts',(71.1501526267286,11.0031476854502,12.));
#172772=CARTESIAN_POINT('Ctrl Pts',(71.1737332703248,10.9984665885127,12.));
#172773=CARTESIAN_POINT('Ctrl Pts',(71.1973507476191,10.993754241032,12.));
#172774=CARTESIAN_POINT('Ctrl Pts',(71.2210049304014,10.9890106067039,12.));
#172775=CARTESIAN_POINT('Ctrl Pts',(71.2446956909687,10.9842356494627,12.));
#172776=CARTESIAN_POINT('Ctrl Pts',(71.2684229021207,10.9794293334805,12.));
#172777=CARTESIAN_POINT('Ctrl Pts',(71.2921864371491,10.9745916231709,12.));
#172778=CARTESIAN_POINT('Ctrl Pts',(71.3159861698358,10.969722483186,12.));
#172779=CARTESIAN_POINT('Ctrl Pts',(71.339821974454,10.9648218784098,12.));
#172780=CARTESIAN_POINT('Ctrl Pts',(71.3636937257649,10.9598897739565,12.));
#172781=CARTESIAN_POINT('Ctrl Pts',(71.3876012990138,10.954926135169,12.));
#172782=CARTESIAN_POINT('Ctrl Pts',(71.4115445699194,10.9499309276237,12.));
#172783=CARTESIAN_POINT('Ctrl Pts',(71.435523414672,10.944904117127,12.));
#172784=CARTESIAN_POINT('Ctrl Pts',(71.4595377099351,10.9398456697095,12.));
#172785=CARTESIAN_POINT('Ctrl Pts',(71.4835873328423,10.9347555516235,12.));
#172786=CARTESIAN_POINT('Ctrl Pts',(71.5076721609936,10.9296337293425,12.));
#172787=CARTESIAN_POINT('Ctrl Pts',(71.5317920724459,10.9244801695642,12.));
#172788=CARTESIAN_POINT('Ctrl Pts',(71.5559469457091,10.91929483921,12.));
#172789=CARTESIAN_POINT('Ctrl Pts',(71.5801366597488,10.914077705417,12.));
#172790=CARTESIAN_POINT('Ctrl Pts',(71.6043610939835,10.9088287355365,12.));
#172791=CARTESIAN_POINT('Ctrl Pts',(71.6286201282812,10.9035478971328,12.));
#172792=CARTESIAN_POINT('Ctrl Pts',(71.6529136429504,10.8982351579871,12.));
#172793=CARTESIAN_POINT('Ctrl Pts',(71.6772415187364,10.8928904860964,12.));
#172794=CARTESIAN_POINT('Ctrl Pts',(71.7016036368236,10.8875138496671,12.));
#172795=CARTESIAN_POINT('Ctrl Pts',(71.7259998788328,10.8821052171121,12.));
#172796=CARTESIAN_POINT('Ctrl Pts',(71.7504301268181,10.8766645570497,12.));
#172797=CARTESIAN_POINT('Ctrl Pts',(71.7748942632593,10.8711918383073,12.));
#172798=CARTESIAN_POINT('Ctrl Pts',(71.7993921710564,10.865687029922,12.));
#172799=CARTESIAN_POINT('Ctrl Pts',(71.8239237335331,10.8601501011332,12.));
#172800=CARTESIAN_POINT('Ctrl Pts',(71.8484888344339,10.8545810213799,12.));
#172801=CARTESIAN_POINT('Ctrl Pts',(71.8730873579224,10.8489797602998,12.));
#172802=CARTESIAN_POINT('Ctrl Pts',(71.8977191885725,10.8433462877312,12.));
#172803=CARTESIAN_POINT('Ctrl Pts',(71.9223842113625,10.8376805737159,12.));
#172804=CARTESIAN_POINT('Ctrl Pts',(71.9470823116785,10.8319825884918,12.));
#172805=CARTESIAN_POINT('Ctrl Pts',(71.9718133753127,10.8262523024898,12.));
#172806=CARTESIAN_POINT('Ctrl Pts',(71.9965772884619,10.8204896863328,12.));
#172807=CARTESIAN_POINT('Ctrl Pts',(72.0213739377223,10.8146947108375,12.));
#172808=CARTESIAN_POINT('Ctrl Pts',(72.0462032100815,10.8088673470184,12.));
#172809=CARTESIAN_POINT('Ctrl Pts',(72.0710649929202,10.8030075660809,12.));
#172810=CARTESIAN_POINT('Ctrl Pts',(72.0959591740114,10.7971153394166,12.));
#172811=CARTESIAN_POINT('Ctrl Pts',(72.1208856415171,10.7911906386027,12.));
#172812=CARTESIAN_POINT('Ctrl Pts',(72.1458442839834,10.7852334354016,12.));
#172813=CARTESIAN_POINT('Ctrl Pts',(72.1708349903305,10.7792437017662,12.));
#172814=CARTESIAN_POINT('Ctrl Pts',(72.1958576498557,10.7732214098345,12.));
#172815=CARTESIAN_POINT('Ctrl Pts',(72.2209121522366,10.7671665319255,12.));
#172816=CARTESIAN_POINT('Ctrl Pts',(72.2459983875296,10.7610790405385,12.));
#172817=CARTESIAN_POINT('Ctrl Pts',(72.2711162461681,10.7549589083535,12.));
#172818=CARTESIAN_POINT('Ctrl Pts',(72.2962656189556,10.7488061082368,12.));
#172819=CARTESIAN_POINT('Ctrl Pts',(72.3214463970641,10.7426206132375,12.));
#172820=CARTESIAN_POINT('Ctrl Pts',(72.3466584720318,10.73640239658,12.));
#172821=CARTESIAN_POINT('Ctrl Pts',(72.3719017357571,10.7301514316607,12.));
#172822=CARTESIAN_POINT('Ctrl Pts',(72.3971760804933,10.7238676920469,12.));
#172823=CARTESIAN_POINT('Ctrl Pts',(72.4224813988347,10.7175511514789,12.));
#172824=CARTESIAN_POINT('Ctrl Pts',(72.4478175837156,10.7112017838706,12.));
#172825=CARTESIAN_POINT('Ctrl Pts',(72.4731845284227,10.7048195633061,12.));
#172826=CARTESIAN_POINT('Ctrl Pts',(72.4985821266023,10.6984044640398,12.));
#172827=CARTESIAN_POINT('Ctrl Pts',(72.5240102722664,10.691956460499,12.));
#172828=CARTESIAN_POINT('Ctrl Pts',(72.5494688597961,10.6854755272904,12.));
#172829=CARTESIAN_POINT('Ctrl Pts',(72.5749577839415,10.6789616392042,12.));
#172830=CARTESIAN_POINT('Ctrl Pts',(72.6004769398019,10.6724147711995,12.));
#172831=CARTESIAN_POINT('Ctrl Pts',(72.6260262228065,10.6658348983945,12.));
#172832=CARTESIAN_POINT('Ctrl Pts',(72.651605528691,10.6592219960581,12.));
#172833=CARTESIAN_POINT('Ctrl Pts',(72.6772147534752,10.6525760396054,12.));
#172834=CARTESIAN_POINT('Ctrl Pts',(72.7028537934317,10.6458970045946,12.));
#172835=CARTESIAN_POINT('Ctrl Pts',(72.7285225451293,10.6391848667352,12.));
#172836=CARTESIAN_POINT('Ctrl Pts',(72.7542209054812,10.6324396018998,12.));
#172837=CARTESIAN_POINT('Ctrl Pts',(72.7799487717911,10.6256611861394,12.));
#172838=CARTESIAN_POINT('Ctrl Pts',(72.8057060417887,10.6188495956973,12.));
#172839=CARTESIAN_POINT('Ctrl Pts',(72.8314926136881,10.6120048070368,12.));
#172840=CARTESIAN_POINT('Ctrl Pts',(72.8573083861337,10.6051267968203,12.));
#172841=CARTESIAN_POINT('Ctrl Pts',(72.8831532580845,10.5982155418626,12.));
#172842=CARTESIAN_POINT('Ctrl Pts',(72.9090271287083,10.5912710190928,12.));
#172843=CARTESIAN_POINT('Ctrl Pts',(72.9349298972822,10.5842932055209,12.));
#172844=CARTESIAN_POINT('Ctrl Pts',(72.9608614630534,10.5772820781958,12.));
#172845=CARTESIAN_POINT('Ctrl Pts',(72.9868217252283,10.570237614205,12.));
#172846=CARTESIAN_POINT('Ctrl Pts',(73.0128105832621,10.5631597907651,12.));
#172847=CARTESIAN_POINT('Ctrl Pts',(73.0388279370834,10.5560485852974,12.));
#172848=CARTESIAN_POINT('Ctrl Pts',(73.0648736873434,10.5489039755138,12.));
#172849=CARTESIAN_POINT('Ctrl Pts',(73.0909477356474,10.5417259395003,12.));
#172850=CARTESIAN_POINT('Ctrl Pts',(73.1170499848039,10.53451445581,12.));
#172851=CARTESIAN_POINT('Ctrl Pts',(73.1431803382711,10.5272695032653,12.));
#172852=CARTESIAN_POINT('Ctrl Pts',(73.1693386996138,10.5199910607655,12.));
#172853=CARTESIAN_POINT('Ctrl Pts',(73.1955249719048,10.5126791070805,12.));
#172854=CARTESIAN_POINT('Ctrl Pts',(73.2217390572562,10.5053336206908,12.));
#172855=CARTESIAN_POINT('Ctrl Pts',(73.2479808560189,10.4979545795192,12.));
#172856=CARTESIAN_POINT('Ctrl Pts',(73.2742502674304,10.4905419611523,12.));
#172857=CARTESIAN_POINT('Ctrl Pts',(73.3005471910583,10.4830957433305,12.));
#172858=CARTESIAN_POINT('Ctrl Pts',(73.3268715280575,10.4756159043806,12.));
#172859=CARTESIAN_POINT('Ctrl Pts',(73.3532231823659,10.4681024236289,12.));
#172860=CARTESIAN_POINT('Ctrl Pts',(73.37960206225,10.4605552819397,12.));
#172861=CARTESIAN_POINT('Ctrl Pts',(73.4060080806686,10.452974461845,12.));
#172862=CARTESIAN_POINT('Ctrl Pts',(73.4286663448108,10.4464473465479,12.));
#172863=CARTESIAN_POINT('Ctrl Pts',(73.44605255288,10.4414249334739,12.));
#172864=CARTESIAN_POINT('Ctrl Pts',(73.4581547436839,10.4379221501041,12.));
#172865=CARTESIAN_POINT('Ctrl Pts',(73.4649650361894,10.4359488742809,12.));
#172866=CARTESIAN_POINT('Ctrl Pts',(73.466479592994,10.4355099267296,12.));
#172867=CARTESIAN_POINT('',(69.079679653846,11.3136138754165,0.));
#172868=CARTESIAN_POINT('',(69.079679653846,11.3136138754165,0.));
#172869=CARTESIAN_POINT('Ctrl Pts',(73.466479592994,10.4355099267296,0.));
#172870=CARTESIAN_POINT('Ctrl Pts',(73.4649650361895,10.4359488742808,0.));
#172871=CARTESIAN_POINT('Ctrl Pts',(73.4581547436839,10.4379221501041,0.));
#172872=CARTESIAN_POINT('Ctrl Pts',(73.4460525528801,10.4414249334739,0.));
#172873=CARTESIAN_POINT('Ctrl Pts',(73.4286663448108,10.4464473465479,0.));
#172874=CARTESIAN_POINT('Ctrl Pts',(73.4060080806686,10.452974461845,0.));
#172875=CARTESIAN_POINT('Ctrl Pts',(73.37960206225,10.4605552819397,0.));
#172876=CARTESIAN_POINT('Ctrl Pts',(73.3532231823659,10.4681024236289,0.));
#172877=CARTESIAN_POINT('Ctrl Pts',(73.3268715280575,10.4756159043806,0.));
#172878=CARTESIAN_POINT('Ctrl Pts',(73.3005471910583,10.4830957433305,0.));
#172879=CARTESIAN_POINT('Ctrl Pts',(73.2742502674304,10.4905419611523,0.));
#172880=CARTESIAN_POINT('Ctrl Pts',(73.2479808560189,10.4979545795192,0.));
#172881=CARTESIAN_POINT('Ctrl Pts',(73.2217390572562,10.5053336206908,0.));
#172882=CARTESIAN_POINT('Ctrl Pts',(73.1955249719048,10.5126791070805,0.));
#172883=CARTESIAN_POINT('Ctrl Pts',(73.1693386996138,10.5199910607655,0.));
#172884=CARTESIAN_POINT('Ctrl Pts',(73.1431803382711,10.5272695032653,0.));
#172885=CARTESIAN_POINT('Ctrl Pts',(73.1170499848039,10.53451445581,0.));
#172886=CARTESIAN_POINT('Ctrl Pts',(73.0909477356474,10.5417259395003,0.));
#172887=CARTESIAN_POINT('Ctrl Pts',(73.0648736873434,10.5489039755138,0.));
#172888=CARTESIAN_POINT('Ctrl Pts',(73.0388279370834,10.5560485852974,0.));
#172889=CARTESIAN_POINT('Ctrl Pts',(73.0128105832621,10.5631597907651,0.));
#172890=CARTESIAN_POINT('Ctrl Pts',(72.9868217252283,10.570237614205,0.));
#172891=CARTESIAN_POINT('Ctrl Pts',(72.9608614630534,10.5772820781958,0.));
#172892=CARTESIAN_POINT('Ctrl Pts',(72.9349298972822,10.5842932055209,0.));
#172893=CARTESIAN_POINT('Ctrl Pts',(72.9090271287083,10.5912710190928,0.));
#172894=CARTESIAN_POINT('Ctrl Pts',(72.8831532580845,10.5982155418626,0.));
#172895=CARTESIAN_POINT('Ctrl Pts',(72.8573083861337,10.6051267968203,0.));
#172896=CARTESIAN_POINT('Ctrl Pts',(72.8314926136881,10.6120048070368,0.));
#172897=CARTESIAN_POINT('Ctrl Pts',(72.8057060417887,10.6188495956973,0.));
#172898=CARTESIAN_POINT('Ctrl Pts',(72.7799487717911,10.6256611861394,0.));
#172899=CARTESIAN_POINT('Ctrl Pts',(72.7542209054812,10.6324396018998,0.));
#172900=CARTESIAN_POINT('Ctrl Pts',(72.7285225451293,10.6391848667352,0.));
#172901=CARTESIAN_POINT('Ctrl Pts',(72.7028537934317,10.6458970045946,0.));
#172902=CARTESIAN_POINT('Ctrl Pts',(72.6772147534752,10.6525760396054,0.));
#172903=CARTESIAN_POINT('Ctrl Pts',(72.651605528691,10.6592219960581,0.));
#172904=CARTESIAN_POINT('Ctrl Pts',(72.6260262228065,10.6658348983945,0.));
#172905=CARTESIAN_POINT('Ctrl Pts',(72.6004769398019,10.6724147711995,0.));
#172906=CARTESIAN_POINT('Ctrl Pts',(72.5749577839415,10.6789616392042,0.));
#172907=CARTESIAN_POINT('Ctrl Pts',(72.5494688597961,10.6854755272904,0.));
#172908=CARTESIAN_POINT('Ctrl Pts',(72.5240102722664,10.691956460499,0.));
#172909=CARTESIAN_POINT('Ctrl Pts',(72.4985821266023,10.6984044640398,0.));
#172910=CARTESIAN_POINT('Ctrl Pts',(72.4731845284227,10.7048195633061,0.));
#172911=CARTESIAN_POINT('Ctrl Pts',(72.4478175837156,10.7112017838706,0.));
#172912=CARTESIAN_POINT('Ctrl Pts',(72.4224813988347,10.7175511514789,0.));
#172913=CARTESIAN_POINT('Ctrl Pts',(72.3971760804933,10.7238676920469,0.));
#172914=CARTESIAN_POINT('Ctrl Pts',(72.3719017357571,10.7301514316607,0.));
#172915=CARTESIAN_POINT('Ctrl Pts',(72.3466584720318,10.73640239658,0.));
#172916=CARTESIAN_POINT('Ctrl Pts',(72.3214463970641,10.7426206132375,0.));
#172917=CARTESIAN_POINT('Ctrl Pts',(72.2962656189556,10.7488061082368,0.));
#172918=CARTESIAN_POINT('Ctrl Pts',(72.2711162461681,10.7549589083535,0.));
#172919=CARTESIAN_POINT('Ctrl Pts',(72.2459983875296,10.7610790405385,0.));
#172920=CARTESIAN_POINT('Ctrl Pts',(72.2209121522366,10.7671665319255,0.));
#172921=CARTESIAN_POINT('Ctrl Pts',(72.1958576498557,10.7732214098345,0.));
#172922=CARTESIAN_POINT('Ctrl Pts',(72.1708349903305,10.7792437017662,0.));
#172923=CARTESIAN_POINT('Ctrl Pts',(72.1458442839834,10.7852334354016,0.));
#172924=CARTESIAN_POINT('Ctrl Pts',(72.1208856415171,10.7911906386027,0.));
#172925=CARTESIAN_POINT('Ctrl Pts',(72.0959591740114,10.7971153394166,0.));
#172926=CARTESIAN_POINT('Ctrl Pts',(72.0710649929202,10.8030075660809,0.));
#172927=CARTESIAN_POINT('Ctrl Pts',(72.0462032100815,10.8088673470184,0.));
#172928=CARTESIAN_POINT('Ctrl Pts',(72.0213739377223,10.8146947108375,0.));
#172929=CARTESIAN_POINT('Ctrl Pts',(71.9965772884619,10.8204896863328,0.));
#172930=CARTESIAN_POINT('Ctrl Pts',(71.9718133753127,10.8262523024898,0.));
#172931=CARTESIAN_POINT('Ctrl Pts',(71.9470823116785,10.8319825884918,0.));
#172932=CARTESIAN_POINT('Ctrl Pts',(71.9223842113625,10.8376805737159,0.));
#172933=CARTESIAN_POINT('Ctrl Pts',(71.8977191885725,10.8433462877312,0.));
#172934=CARTESIAN_POINT('Ctrl Pts',(71.8730873579224,10.8489797602998,0.));
#172935=CARTESIAN_POINT('Ctrl Pts',(71.8484888344339,10.8545810213799,0.));
#172936=CARTESIAN_POINT('Ctrl Pts',(71.8239237335331,10.8601501011332,0.));
#172937=CARTESIAN_POINT('Ctrl Pts',(71.7993921710564,10.865687029922,0.));
#172938=CARTESIAN_POINT('Ctrl Pts',(71.7748942632593,10.8711918383073,0.));
#172939=CARTESIAN_POINT('Ctrl Pts',(71.7504301268181,10.8766645570497,0.));
#172940=CARTESIAN_POINT('Ctrl Pts',(71.7259998788328,10.8821052171121,0.));
#172941=CARTESIAN_POINT('Ctrl Pts',(71.7016036368236,10.8875138496671,0.));
#172942=CARTESIAN_POINT('Ctrl Pts',(71.6772415187364,10.8928904860964,0.));
#172943=CARTESIAN_POINT('Ctrl Pts',(71.6529136429504,10.8982351579871,0.));
#172944=CARTESIAN_POINT('Ctrl Pts',(71.6286201282812,10.9035478971328,0.));
#172945=CARTESIAN_POINT('Ctrl Pts',(71.6043610939835,10.9088287355365,0.));
#172946=CARTESIAN_POINT('Ctrl Pts',(71.5801366597488,10.914077705417,0.));
#172947=CARTESIAN_POINT('Ctrl Pts',(71.5559469457091,10.91929483921,0.));
#172948=CARTESIAN_POINT('Ctrl Pts',(71.5317920724459,10.9244801695642,0.));
#172949=CARTESIAN_POINT('Ctrl Pts',(71.5076721609936,10.9296337293425,0.));
#172950=CARTESIAN_POINT('Ctrl Pts',(71.4835873328423,10.9347555516235,0.));
#172951=CARTESIAN_POINT('Ctrl Pts',(71.4595377099351,10.9398456697095,0.));
#172952=CARTESIAN_POINT('Ctrl Pts',(71.435523414672,10.944904117127,0.));
#172953=CARTESIAN_POINT('Ctrl Pts',(71.4115445699194,10.9499309276237,0.));
#172954=CARTESIAN_POINT('Ctrl Pts',(71.3876012990138,10.954926135169,0.));
#172955=CARTESIAN_POINT('Ctrl Pts',(71.3636937257649,10.9598897739565,0.));
#172956=CARTESIAN_POINT('Ctrl Pts',(71.339821974454,10.9648218784098,0.));
#172957=CARTESIAN_POINT('Ctrl Pts',(71.3159861698358,10.969722483186,0.));
#172958=CARTESIAN_POINT('Ctrl Pts',(71.2921864371491,10.9745916231709,0.));
#172959=CARTESIAN_POINT('Ctrl Pts',(71.2684229021207,10.9794293334805,0.));
#172960=CARTESIAN_POINT('Ctrl Pts',(71.2446956909687,10.9842356494627,0.));
#172961=CARTESIAN_POINT('Ctrl Pts',(71.2210049304014,10.9890106067039,0.));
#172962=CARTESIAN_POINT('Ctrl Pts',(71.1973507476191,10.993754241032,0.));
#172963=CARTESIAN_POINT('Ctrl Pts',(71.1737332703248,10.9984665885127,0.));
#172964=CARTESIAN_POINT('Ctrl Pts',(71.1501526267286,11.0031476854502,0.));
#172965=CARTESIAN_POINT('Ctrl Pts',(71.1266089455517,11.0077975683895,0.));
#172966=CARTESIAN_POINT('Ctrl Pts',(71.1031023560249,11.0124162741225,0.));
#172967=CARTESIAN_POINT('Ctrl Pts',(71.0796329878907,11.0170038396915,0.));
#172968=CARTESIAN_POINT('Ctrl Pts',(71.0562009714136,11.0215603023856,0.));
#172969=CARTESIAN_POINT('Ctrl Pts',(71.0328064373856,11.0260856997415,0.));
#172970=CARTESIAN_POINT('Ctrl Pts',(71.0094495171292,11.0305800695456,0.));
#172971=CARTESIAN_POINT('Ctrl Pts',(70.986130342497,11.0350434498405,0.));
#172972=CARTESIAN_POINT('Ctrl Pts',(70.9628490458748,11.0394758789285,0.));
#172973=CARTESIAN_POINT('Ctrl Pts',(70.9396057601924,11.0438773953682,0.));
#172974=CARTESIAN_POINT('Ctrl Pts',(70.916400618927,11.048248037975,0.));
#172975=CARTESIAN_POINT('Ctrl Pts',(70.8932337561087,11.0525878458243,0.));
#172976=CARTESIAN_POINT('Ctrl Pts',(70.8701053063186,11.0568968582569,0.));
#172977=CARTESIAN_POINT('Ctrl Pts',(70.8470154046919,11.0611751148835,0.));
#172978=CARTESIAN_POINT('Ctrl Pts',(70.8239641869299,11.0654226555802,0.));
#172979=CARTESIAN_POINT('Ctrl Pts',(70.8009517893057,11.0696395204909,0.));
#172980=CARTESIAN_POINT('Ctrl Pts',(70.7779783486677,11.0738257500291,0.));
#172981=CARTESIAN_POINT('Ctrl Pts',(70.7550440024384,11.0779813848846,0.));
#172982=CARTESIAN_POINT('Ctrl Pts',(70.732148888618,11.0821064660269,0.));
#172983=CARTESIAN_POINT('Ctrl Pts',(70.7092931457954,11.0862010347016,0.));
#172984=CARTESIAN_POINT('Ctrl Pts',(70.6864769131546,11.0902651324323,0.));
#172985=CARTESIAN_POINT('Ctrl Pts',(70.6637003304785,11.0942988010233,0.));
#172986=CARTESIAN_POINT('Ctrl Pts',(70.6409635381482,11.0983020825667,0.));
#172987=CARTESIAN_POINT('Ctrl Pts',(70.6182666771481,11.1022750194446,0.));
#172988=CARTESIAN_POINT('Ctrl Pts',(70.5956098890773,11.1062176543262,0.));
#172989=CARTESIAN_POINT('Ctrl Pts',(70.5729933161546,11.1101300301702,0.));
#172990=CARTESIAN_POINT('Ctrl Pts',(70.5504171012233,11.1140121902271,0.));
#172991=CARTESIAN_POINT('Ctrl Pts',(70.5278813877494,11.1178641780476,0.));
#172992=CARTESIAN_POINT('Ctrl Pts',(70.505386319828,11.1216860374826,0.));
#172993=CARTESIAN_POINT('Ctrl Pts',(70.4829320421957,11.1254778126821,0.));
#172994=CARTESIAN_POINT('Ctrl Pts',(70.4605187002354,11.1292395480974,0.));
#172995=CARTESIAN_POINT('Ctrl Pts',(70.4381464399819,11.1329712884847,0.));
#172996=CARTESIAN_POINT('Ctrl Pts',(70.4158154081205,11.1366730789126,0.));
#172997=CARTESIAN_POINT('Ctrl Pts',(70.393525751996,11.1403449647625,0.));
#172998=CARTESIAN_POINT('Ctrl Pts',(70.3712776196223,11.143986991727,0.));
#172999=CARTESIAN_POINT('Ctrl Pts',(70.349071159688,11.1475992058124,0.));
#173000=CARTESIAN_POINT('Ctrl Pts',(70.326906521559,11.1511816533421,0.));
#173001=CARTESIAN_POINT('Ctrl Pts',(70.3047838552756,11.1547343809646,0.));
#173002=CARTESIAN_POINT('Ctrl Pts',(70.2827033115662,11.1582574356521,0.));
#173003=CARTESIAN_POINT('Ctrl Pts',(70.2606650418589,11.1617508647016,0.));
#173004=CARTESIAN_POINT('Ctrl Pts',(70.2386691982902,11.1652147157383,0.));
#173005=CARTESIAN_POINT('Ctrl Pts',(70.2167159337094,11.168649036721,0.));
#173006=CARTESIAN_POINT('Ctrl Pts',(70.1948054016816,11.1720538759499,0.));
#173007=CARTESIAN_POINT('Ctrl Pts',(70.1729377564954,11.1754292820631,0.));
#173008=CARTESIAN_POINT('Ctrl Pts',(70.1511131531672,11.1787753040363,0.));
#173009=CARTESIAN_POINT('Ctrl Pts',(70.1293317474432,11.1820919911846,0.));
#173010=CARTESIAN_POINT('Ctrl Pts',(70.1075936957973,11.185379393167,0.));
#173011=CARTESIAN_POINT('Ctrl Pts',(70.0858991554295,11.1886375599916,0.));
#173012=CARTESIAN_POINT('Ctrl Pts',(70.0642482842942,11.1918665420168,0.));
#173013=CARTESIAN_POINT('Ctrl Pts',(70.0426412411194,11.1950663899578,0.));
#173014=CARTESIAN_POINT('Ctrl Pts',(70.0210781854236,11.1982371548918,0.));
#173015=CARTESIAN_POINT('Ctrl Pts',(69.9995592775322,11.2013788882711,0.));
#173016=CARTESIAN_POINT('Ctrl Pts',(69.9780846785771,11.2044916419239,0.));
#173017=CARTESIAN_POINT('Ctrl Pts',(69.9566545504813,11.2075754680445,0.));
#173018=CARTESIAN_POINT('Ctrl Pts',(69.9352690559399,11.2106304191881,0.));
#173019=CARTESIAN_POINT('Ctrl Pts',(69.9139283584036,11.213656548268,0.));
#173020=CARTESIAN_POINT('Ctrl Pts',(69.8926326220414,11.2166539085527,0.));
#173021=CARTESIAN_POINT('Ctrl Pts',(69.8713820117918,11.2196225536794,0.));
#173022=CARTESIAN_POINT('Ctrl Pts',(69.8501766934445,11.2225625376739,0.));
#173023=CARTESIAN_POINT('Ctrl Pts',(69.8290168337076,11.225473914972,0.));
#173024=CARTESIAN_POINT('Ctrl Pts',(69.8079026002753,11.2283567404434,0.));
#173025=CARTESIAN_POINT('Ctrl Pts',(69.7868341618927,11.2312110694183,0.));
#173026=CARTESIAN_POINT('Ctrl Pts',(69.7658116882298,11.2340369576452,0.));
#173027=CARTESIAN_POINT('Ctrl Pts',(69.7448353497394,11.236834461247,0.));
#173028=CARTESIAN_POINT('Ctrl Pts',(69.7239053175362,11.2396036366861,0.));
#173029=CARTESIAN_POINT('Ctrl Pts',(69.7030217632187,11.242344540717,0.));
#173030=CARTESIAN_POINT('Ctrl Pts',(69.6821848588492,11.2450572303847,0.));
#173031=CARTESIAN_POINT('Ctrl Pts',(69.6613947773563,11.2477417631391,0.));
#173032=CARTESIAN_POINT('Ctrl Pts',(69.6406516928902,11.2503981969414,0.));
#173033=CARTESIAN_POINT('Ctrl Pts',(69.6199557811231,11.2530265903555,0.));
#173034=CARTESIAN_POINT('Ctrl Pts',(69.5993072197355,11.255627002701,0.));
#173035=CARTESIAN_POINT('Ctrl Pts',(69.5787061880815,11.2581994939534,0.));
#173036=CARTESIAN_POINT('Ctrl Pts',(69.5581528662846,11.2607441244698,0.));
#173037=CARTESIAN_POINT('Ctrl Pts',(69.5376474344768,11.2632609547629,0.));
#173038=CARTESIAN_POINT('Ctrl Pts',(69.5171900720188,11.2657500452721,0.));
#173039=CARTESIAN_POINT('Ctrl Pts',(69.4967809565978,11.2682114561015,0.));
#173040=CARTESIAN_POINT('Ctrl Pts',(69.4764202659443,11.2706452475287,0.));
#173041=CARTESIAN_POINT('Ctrl Pts',(69.4561081798815,11.2730514806143,0.));
#173042=CARTESIAN_POINT('Ctrl Pts',(69.4358448819957,11.2754302177019,0.));
#173043=CARTESIAN_POINT('Ctrl Pts',(69.4156305620554,11.2777815231462,0.));
#173044=CARTESIAN_POINT('Ctrl Pts',(69.395465416223,11.2801054633807,0.));
#173045=CARTESIAN_POINT('Ctrl Pts',(69.375349642,11.2824021054038,0.));
#173046=CARTESIAN_POINT('Ctrl Pts',(69.3552834337771,11.2846715154521,0.));
#173047=CARTESIAN_POINT('Ctrl Pts',(69.3352669789611,11.2869137578463,0.));
#173048=CARTESIAN_POINT('Ctrl Pts',(69.315300451784,11.2891288931528,0.));
#173049=CARTESIAN_POINT('Ctrl Pts',(69.2953840192792,11.2913169799642,0.));
#173050=CARTESIAN_POINT('Ctrl Pts',(69.2755178531534,11.2934780784362,0.));
#173051=CARTESIAN_POINT('Ctrl Pts',(69.255702139335,11.2956122531375,0.));
#173052=CARTESIAN_POINT('Ctrl Pts',(69.2359370894828,11.2977195764836,0.));
#173053=CARTESIAN_POINT('Ctrl Pts',(69.216222948839,11.2998001310934,0.));
#173054=CARTESIAN_POINT('Ctrl Pts',(69.1965599718761,11.3018540025605,0.));
#173055=CARTESIAN_POINT('Ctrl Pts',(69.1769483991639,11.3038812726275,0.));
#173056=CARTESIAN_POINT('Ctrl Pts',(69.1573884361076,11.3058820128323,0.));
#173057=CARTESIAN_POINT('Ctrl Pts',(69.137880225198,11.3078562764442,0.));
#173058=CARTESIAN_POINT('Ctrl Pts',(69.1184238445065,11.3098040973799,0.));
#173059=CARTESIAN_POINT('Ctrl Pts',(69.1029002322497,11.3113412156742,0.));
#173060=CARTESIAN_POINT('Ctrl Pts',(69.0912808657051,11.3124821678849,0.));
#173061=CARTESIAN_POINT('Ctrl Pts',(69.0835449954486,11.3132375200184,0.));
#173062=CARTESIAN_POINT('Ctrl Pts',(69.079679653846,11.3136138754165,0.));
#173063=CARTESIAN_POINT('Origin',(0.,0.,0.));
#173064=CARTESIAN_POINT('',(69.8028570375097,5.24987136994592,0.));
#173065=CARTESIAN_POINT('Origin',(0.,0.,0.));
#173066=CARTESIAN_POINT('',(69.8028570375097,5.24987136994592,12.));
#173067=CARTESIAN_POINT('',(69.8028570375097,5.24987136994592,0.));
#173068=CARTESIAN_POINT('Origin',(0.,0.,12.));
#173069=CARTESIAN_POINT('Origin',(0.,0.,0.));
#173070=CARTESIAN_POINT('Origin',(0.,0.,0.));
#173071=CARTESIAN_POINT('Origin',(0.,0.,12.));
#173072=CARTESIAN_POINT('Origin',(0.,0.,0.));
#173073=CARTESIAN_POINT('Origin',(0.,0.,0.));
#173074=CARTESIAN_POINT('Origin',(0.,0.,12.));
#173075=CARTESIAN_POINT('Origin',(0.,0.,0.));
#173076=CARTESIAN_POINT('Origin',(0.,0.,0.));
#173077=CARTESIAN_POINT('Origin',(0.,0.,12.));
#173078=CARTESIAN_POINT('Origin',(0.,0.,0.));
#173079=CARTESIAN_POINT('Origin',(0.,0.,0.));
#173080=CARTESIAN_POINT('Origin',(0.,0.,12.));
#173081=CARTESIAN_POINT('Origin',(0.,0.,0.));
#173082=CARTESIAN_POINT('Origin',(0.,0.,0.));
#173083=CARTESIAN_POINT('Origin',(0.,0.,12.));
#173084=CARTESIAN_POINT('Origin',(0.,0.,0.));
#173085=CARTESIAN_POINT('Origin',(0.,0.,0.));
#173086=CARTESIAN_POINT('Origin',(0.,0.,12.));
#173087=CARTESIAN_POINT('Origin',(0.,0.,0.));
#173088=CARTESIAN_POINT('Origin',(0.,0.,0.));
#173089=CARTESIAN_POINT('Origin',(0.,0.,12.));
#173090=CARTESIAN_POINT('Origin',(0.,0.,0.));
#173091=CARTESIAN_POINT('Origin',(0.,0.,0.));
#173092=CARTESIAN_POINT('Origin',(0.,0.,12.));
#173093=CARTESIAN_POINT('Origin',(0.,0.,0.));
#173094=CARTESIAN_POINT('Origin',(0.,0.,0.));
#173095=CARTESIAN_POINT('Origin',(0.,0.,12.));
#173096=CARTESIAN_POINT('Origin',(0.,0.,0.));
#173097=CARTESIAN_POINT('Origin',(0.,0.,0.));
#173098=CARTESIAN_POINT('Origin',(0.,0.,12.));
#173099=CARTESIAN_POINT('Origin',(0.,0.,0.));
#173100=CARTESIAN_POINT('Origin',(0.,0.,0.));
#173101=CARTESIAN_POINT('Origin',(0.,0.,12.));
#173102=CARTESIAN_POINT('Origin',(0.,0.,0.));
#173103=CARTESIAN_POINT('Origin',(0.,0.,0.));
#173104=CARTESIAN_POINT('Origin',(0.,0.,12.));
#173105=CARTESIAN_POINT('Origin',(0.,0.,0.));
#173106=CARTESIAN_POINT('Origin',(0.,0.,0.));
#173107=CARTESIAN_POINT('Origin',(0.,0.,12.));
#173108=CARTESIAN_POINT('Origin',(0.,0.,0.));
#173109=CARTESIAN_POINT('Origin',(0.,0.,0.));
#173110=CARTESIAN_POINT('Origin',(0.,0.,12.));
#173111=CARTESIAN_POINT('Origin',(0.,0.,0.));
#173112=CARTESIAN_POINT('Origin',(0.,0.,0.));
#173113=CARTESIAN_POINT('Origin',(0.,0.,12.));
#173114=CARTESIAN_POINT('Origin',(0.,0.,0.));
#173115=CARTESIAN_POINT('Origin',(0.,0.,0.));
#173116=CARTESIAN_POINT('Origin',(0.,0.,12.));
#173117=CARTESIAN_POINT('Origin',(0.,0.,0.));
#173118=CARTESIAN_POINT('Origin',(0.,0.,0.));
#173119=CARTESIAN_POINT('Origin',(0.,0.,12.));
#173120=CARTESIAN_POINT('Origin',(0.,0.,0.));
#173121=CARTESIAN_POINT('Origin',(0.,0.,0.));
#173122=CARTESIAN_POINT('Origin',(0.,0.,12.));
#173123=CARTESIAN_POINT('Origin',(0.,0.,0.));
#173124=CARTESIAN_POINT('Origin',(0.,0.,0.));
#173125=CARTESIAN_POINT('Origin',(0.,0.,12.));
#173126=CARTESIAN_POINT('Origin',(0.,0.,0.));
#173127=CARTESIAN_POINT('Origin',(0.,0.,0.));
#173128=CARTESIAN_POINT('Origin',(0.,0.,12.));
#173129=CARTESIAN_POINT('Origin',(0.,0.,0.));
#173130=CARTESIAN_POINT('Origin',(0.,0.,0.));
#173131=CARTESIAN_POINT('Origin',(0.,0.,12.));
#173132=CARTESIAN_POINT('Origin',(0.,0.,0.));
#173133=CARTESIAN_POINT('Origin',(0.,0.,0.));
#173134=CARTESIAN_POINT('Origin',(0.,0.,12.));
#173135=CARTESIAN_POINT('Origin',(0.,0.,0.));
#173136=CARTESIAN_POINT('Origin',(0.,0.,0.));
#173137=CARTESIAN_POINT('Origin',(0.,0.,12.));
#173138=CARTESIAN_POINT('Origin',(0.,0.,0.));
#173139=CARTESIAN_POINT('Origin',(0.,0.,0.));
#173140=CARTESIAN_POINT('Origin',(0.,0.,12.));
#173141=CARTESIAN_POINT('Origin',(0.,0.,0.));
#173142=CARTESIAN_POINT('Origin',(0.,0.,0.));
#173143=CARTESIAN_POINT('Origin',(0.,0.,12.));
#173144=CARTESIAN_POINT('Origin',(0.,0.,0.));
#173145=CARTESIAN_POINT('Origin',(0.,0.,0.));
#173146=CARTESIAN_POINT('Origin',(0.,0.,12.));
#173147=CARTESIAN_POINT('Origin',(0.,0.,0.));
#173148=CARTESIAN_POINT('Origin',(0.,0.,0.));
#173149=CARTESIAN_POINT('Origin',(0.,0.,12.));
#173150=CARTESIAN_POINT('Origin',(0.,0.,0.));
#173151=CARTESIAN_POINT('Origin',(0.,0.,0.));
#173152=CARTESIAN_POINT('Origin',(0.,0.,12.));
#173153=CARTESIAN_POINT('Origin',(0.,0.,0.));
#173154=CARTESIAN_POINT('Origin',(0.,0.,0.));
#173155=CARTESIAN_POINT('Origin',(0.,0.,12.));
#173156=CARTESIAN_POINT('Origin',(0.,0.,0.));
#173157=CARTESIAN_POINT('Origin',(0.,0.,0.));
#173158=CARTESIAN_POINT('Origin',(0.,0.,12.));
#173159=CARTESIAN_POINT('Origin',(0.,0.,0.));
#173160=CARTESIAN_POINT('Origin',(0.,0.,0.));
#173161=CARTESIAN_POINT('Origin',(0.,0.,12.));
#173162=CARTESIAN_POINT('Origin',(0.,0.,0.));
#173163=CARTESIAN_POINT('Origin',(0.,0.,0.));
#173164=CARTESIAN_POINT('Origin',(0.,0.,12.));
#173165=CARTESIAN_POINT('Origin',(0.,0.,0.));
#173166=CARTESIAN_POINT('Origin',(0.,0.,0.));
#173167=CARTESIAN_POINT('Origin',(0.,0.,12.));
#173168=CARTESIAN_POINT('Origin',(0.,0.,0.));
#173169=CARTESIAN_POINT('Origin',(0.,0.,0.));
#173170=CARTESIAN_POINT('Origin',(0.,0.,12.));
#173171=CARTESIAN_POINT('Origin',(0.,0.,0.));
#173172=CARTESIAN_POINT('Origin',(0.,0.,0.));
#173173=CARTESIAN_POINT('Origin',(0.,0.,12.));
#173174=CARTESIAN_POINT('Origin',(0.,0.,0.));
#173175=CARTESIAN_POINT('Origin',(0.,0.,0.));
#173176=CARTESIAN_POINT('Origin',(0.,0.,12.));
#173177=CARTESIAN_POINT('Origin',(0.,0.,0.));
#173178=CARTESIAN_POINT('Origin',(0.,0.,0.));
#173179=CARTESIAN_POINT('Origin',(0.,0.,12.));
#173180=CARTESIAN_POINT('Origin',(0.,0.,0.));
#173181=CARTESIAN_POINT('Origin',(0.,0.,0.));
#173182=CARTESIAN_POINT('Origin',(0.,0.,12.));
#173183=CARTESIAN_POINT('Origin',(0.,0.,0.));
#173184=CARTESIAN_POINT('Origin',(0.,0.,0.));
#173185=CARTESIAN_POINT('Origin',(0.,0.,12.));
#173186=CARTESIAN_POINT('Origin',(0.,0.,0.));
#173187=CARTESIAN_POINT('Origin',(0.,0.,0.));
#173188=CARTESIAN_POINT('Origin',(0.,0.,12.));
#173189=CARTESIAN_POINT('Origin',(0.,0.,0.));
#173190=CARTESIAN_POINT('Origin',(0.,0.,0.));
#173191=CARTESIAN_POINT('Origin',(0.,0.,12.));
#173192=CARTESIAN_POINT('Origin',(0.,0.,0.));
#173193=CARTESIAN_POINT('Origin',(0.,0.,0.));
#173194=CARTESIAN_POINT('Origin',(0.,0.,12.));
#173195=CARTESIAN_POINT('Origin',(0.,0.,0.));
#173196=CARTESIAN_POINT('Origin',(0.,0.,0.));
#173197=CARTESIAN_POINT('Origin',(0.,0.,12.));
#173198=CARTESIAN_POINT('Origin',(0.,0.,0.));
#173199=CARTESIAN_POINT('Origin',(0.,0.,0.));
#173200=CARTESIAN_POINT('Origin',(0.,0.,12.));
#173201=CARTESIAN_POINT('Origin',(0.,0.,0.));
#173202=CARTESIAN_POINT('Origin',(0.,0.,0.));
#173203=CARTESIAN_POINT('Origin',(0.,0.,12.));
#173204=CARTESIAN_POINT('Origin',(0.,0.,0.));
#173205=CARTESIAN_POINT('Origin',(0.,0.,0.));
#173206=CARTESIAN_POINT('Origin',(0.,0.,12.));
#173207=CARTESIAN_POINT('Origin',(0.,0.,0.));
#173208=CARTESIAN_POINT('Origin',(0.,0.,0.));
#173209=CARTESIAN_POINT('Origin',(0.,0.,12.));
#173210=CARTESIAN_POINT('Origin',(0.,0.,0.));
#173211=CARTESIAN_POINT('Origin',(0.,0.,0.));
#173212=CARTESIAN_POINT('Origin',(0.,0.,12.));
#173213=CARTESIAN_POINT('Origin',(0.,0.,0.));
#173214=CARTESIAN_POINT('Origin',(0.,0.,0.));
#173215=CARTESIAN_POINT('Origin',(0.,0.,12.));
#173216=CARTESIAN_POINT('Origin',(0.,0.,0.));
#173217=CARTESIAN_POINT('Origin',(0.,0.,0.));
#173218=CARTESIAN_POINT('Origin',(0.,0.,12.));
#173219=CARTESIAN_POINT('Origin',(0.,0.,0.));
#173220=CARTESIAN_POINT('Origin',(0.,0.,0.));
#173221=CARTESIAN_POINT('Origin',(0.,0.,12.));
#173222=CARTESIAN_POINT('Origin',(0.,0.,0.));
#173223=CARTESIAN_POINT('Origin',(0.,0.,0.));
#173224=CARTESIAN_POINT('Origin',(0.,0.,12.));
#173225=CARTESIAN_POINT('Origin',(0.,0.,0.));
#173226=CARTESIAN_POINT('Origin',(0.,0.,0.));
#173227=CARTESIAN_POINT('Origin',(0.,0.,12.));
#173228=CARTESIAN_POINT('Origin',(0.,0.,0.));
#173229=CARTESIAN_POINT('Origin',(0.,0.,0.));
#173230=CARTESIAN_POINT('Origin',(0.,0.,12.));
#173231=CARTESIAN_POINT('Origin',(0.,0.,0.));
#173232=CARTESIAN_POINT('Origin',(0.,0.,0.));
#173233=CARTESIAN_POINT('Origin',(0.,0.,12.));
#173234=CARTESIAN_POINT('Origin',(0.,0.,0.));
#173235=CARTESIAN_POINT('Origin',(0.,0.,0.));
#173236=CARTESIAN_POINT('Origin',(0.,0.,12.));
#173237=CARTESIAN_POINT('Origin',(0.,0.,0.));
#173238=CARTESIAN_POINT('Origin',(0.,0.,0.));
#173239=CARTESIAN_POINT('Origin',(0.,0.,12.));
#173240=CARTESIAN_POINT('Origin',(0.,0.,0.));
#173241=CARTESIAN_POINT('Origin',(0.,0.,0.));
#173242=CARTESIAN_POINT('Origin',(0.,0.,12.));
#173243=CARTESIAN_POINT('Origin',(0.,0.,0.));
#173244=CARTESIAN_POINT('Origin',(0.,0.,0.));
#173245=CARTESIAN_POINT('Origin',(0.,0.,12.));
#173246=CARTESIAN_POINT('Origin',(0.,0.,0.));
#173247=CARTESIAN_POINT('Origin',(0.,0.,0.));
#173248=CARTESIAN_POINT('Origin',(0.,0.,12.));
#173249=CARTESIAN_POINT('Origin',(0.,0.,0.));
#173250=CARTESIAN_POINT('Origin',(0.,0.,0.));
#173251=CARTESIAN_POINT('Origin',(0.,0.,12.));
#173252=CARTESIAN_POINT('Origin',(0.,0.,0.));
#173253=CARTESIAN_POINT('Origin',(0.,0.,0.));
#173254=CARTESIAN_POINT('Origin',(0.,0.,12.));
#173255=CARTESIAN_POINT('Origin',(0.,0.,0.));
#173256=CARTESIAN_POINT('Origin',(0.,0.,0.));
#173257=CARTESIAN_POINT('Origin',(0.,0.,12.));
#173258=CARTESIAN_POINT('Origin',(0.,0.,0.));
#173259=CARTESIAN_POINT('Origin',(0.,0.,0.));
#173260=CARTESIAN_POINT('Origin',(0.,0.,12.));
#173261=CARTESIAN_POINT('Origin',(0.,0.,0.));
#173262=CARTESIAN_POINT('Origin',(0.,0.,0.));
#173263=CARTESIAN_POINT('Origin',(0.,0.,12.));
#173264=CARTESIAN_POINT('Origin',(0.,0.,0.));
#173265=CARTESIAN_POINT('Origin',(0.,0.,0.));
#173266=CARTESIAN_POINT('Origin',(0.,0.,12.));
#173267=CARTESIAN_POINT('Origin',(0.,0.,0.));
#173268=CARTESIAN_POINT('Origin',(0.,0.,0.));
#173269=CARTESIAN_POINT('Origin',(0.,0.,12.));
#173270=CARTESIAN_POINT('Origin',(0.,0.,0.));
#173271=CARTESIAN_POINT('Origin',(0.,0.,0.));
#173272=CARTESIAN_POINT('Origin',(0.,0.,12.));
#173273=CARTESIAN_POINT('Origin',(0.,0.,0.));
#173274=CARTESIAN_POINT('Origin',(0.,0.,0.));
#173275=CARTESIAN_POINT('Origin',(0.,0.,12.));
#173276=CARTESIAN_POINT('Origin',(0.,0.,0.));
#173277=CARTESIAN_POINT('',(69.9947925310006,0.853825826608988,12.));
#173278=CARTESIAN_POINT('Origin',(0.,0.,12.));
#173279=CARTESIAN_POINT('',(69.9947925310006,0.853825826608988,0.));
#173280=CARTESIAN_POINT('',(69.9947925310006,0.853825826608988,0.));
#173281=CARTESIAN_POINT('Origin',(0.,0.,0.));
#173282=CARTESIAN_POINT('Ctrl Pts',(74.4416140848738,2.94891377268297,0.));
#173283=CARTESIAN_POINT('Ctrl Pts',(74.4416140848738,2.94891377268297,4.));
#173284=CARTESIAN_POINT('Ctrl Pts',(74.4416140848738,2.94891377268294,8.));
#173285=CARTESIAN_POINT('Ctrl Pts',(74.4416140848738,2.94891377268294,12.));
#173286=CARTESIAN_POINT('Ctrl Pts',(74.4459635334396,2.83911742169665,0.));
#173287=CARTESIAN_POINT('Ctrl Pts',(74.4459635334396,2.83911742169665,4.));
#173288=CARTESIAN_POINT('Ctrl Pts',(74.4459635334396,2.8391174216966,8.));
#173289=CARTESIAN_POINT('Ctrl Pts',(74.4459635334396,2.8391174216966,12.));
#173290=CARTESIAN_POINT('Ctrl Pts',(74.3877786926472,2.64498412359347,-7.30788408216183E-17));
#173291=CARTESIAN_POINT('Ctrl Pts',(74.3877786926472,2.64498412359347,4.00000000000001));
#173292=CARTESIAN_POINT('Ctrl Pts',(74.3877786926472,2.64498412359339,8.00000000000001));
#173293=CARTESIAN_POINT('Ctrl Pts',(74.3877786926472,2.64498412359339,12.));
#173294=CARTESIAN_POINT('Ctrl Pts',(74.2364344282701,2.51668625693798,-2.46611180232484E-16));
#173295=CARTESIAN_POINT('Ctrl Pts',(74.2364344282701,2.51668625693798,3.99999999999999));
#173296=CARTESIAN_POINT('Ctrl Pts',(74.2364344282701,2.51668625693788,8.));
#173297=CARTESIAN_POINT('Ctrl Pts',(74.2364344282701,2.51668625693788,12.));
#173298=CARTESIAN_POINT('Ctrl Pts',(74.1624659714555,2.48034921843216,-3.30265160469911E-16));
#173299=CARTESIAN_POINT('Ctrl Pts',(74.1624659714555,2.48034921843216,4.));
#173300=CARTESIAN_POINT('Ctrl Pts',(74.1624659714554,2.48034921843206,8.));
#173301=CARTESIAN_POINT('Ctrl Pts',(74.1624659714554,2.48034921843206,12.));
#173302=CARTESIAN_POINT('',(74.4416140848738,2.94891377268297,0.));
#173303=CARTESIAN_POINT('',(74.1624659714554,2.48034921843225,0.));
#173304=CARTESIAN_POINT('Ctrl Pts',(74.4416140848738,2.94891377268297,6.36152171223239E-17));
#173305=CARTESIAN_POINT('Ctrl Pts',(74.4459635334396,2.83911742169665,6.36152171223239E-17));
#173306=CARTESIAN_POINT('Ctrl Pts',(74.4127150529868,2.72818410849483,2.18558795099707E-17));
#173307=CARTESIAN_POINT('Ctrl Pts',(74.3490471689145,2.63874807903103,-5.27046004988717E-17));
#173308=CARTESIAN_POINT('Ctrl Pts',(74.3012962558603,2.57167105693319,-1.08624960505504E-16));
#173309=CARTESIAN_POINT('Ctrl Pts',(74.2364344282701,2.51668625693798,-1.82995963110161E-16));
#173310=CARTESIAN_POINT('Ctrl Pts',(74.1624659714555,2.48034921843216,-2.66649943347587E-16));
#173311=CARTESIAN_POINT('',(74.1624659714554,2.48034921843222,12.));
#173312=CARTESIAN_POINT('Ctrl Pts',(74.1624659714555,2.48034921843216,-3.30265160469911E-16));
#173313=CARTESIAN_POINT('Ctrl Pts',(74.1624659714555,2.48034921843216,4.));
#173314=CARTESIAN_POINT('Ctrl Pts',(74.1624659714554,2.48034921843206,8.));
#173315=CARTESIAN_POINT('Ctrl Pts',(74.1624659714554,2.48034921843206,12.));
#173316=CARTESIAN_POINT('',(74.4416140848738,2.94891377268294,12.));
#173317=CARTESIAN_POINT('Ctrl Pts',(74.1624659714554,2.48034921843206,12.));
#173318=CARTESIAN_POINT('Ctrl Pts',(74.2364344282701,2.51668625693788,12.));
#173319=CARTESIAN_POINT('Ctrl Pts',(74.3012962558603,2.5716710569331,12.));
#173320=CARTESIAN_POINT('Ctrl Pts',(74.3490471689145,2.63874807903096,12.));
#173321=CARTESIAN_POINT('Ctrl Pts',(74.4127150529868,2.72818410849477,12.));
#173322=CARTESIAN_POINT('Ctrl Pts',(74.4459635334396,2.8391174216966,12.));
#173323=CARTESIAN_POINT('Ctrl Pts',(74.4416140848738,2.94891377268294,12.));
#173324=CARTESIAN_POINT('Ctrl Pts',(74.4416140848738,2.94891377268294,12.));
#173325=CARTESIAN_POINT('Ctrl Pts',(74.4416140848738,2.94891377268294,8.));
#173326=CARTESIAN_POINT('Ctrl Pts',(74.4416140848738,2.94891377268297,4.));
#173327=CARTESIAN_POINT('Ctrl Pts',(74.4416140848738,2.94891377268297,0.));
#173328=CARTESIAN_POINT('Ctrl Pts',(69.9947925310006,0.853825826608988,
0.));
#173329=CARTESIAN_POINT('Ctrl Pts',(69.9947925310006,0.853825826608988,
12.));
#173330=CARTESIAN_POINT('Ctrl Pts',(69.9985337959407,0.854867673848601,
0.));
#173331=CARTESIAN_POINT('Ctrl Pts',(69.9985337959407,0.854867673848601,
12.));
#173332=CARTESIAN_POINT('Ctrl Pts',(70.0060209754087,0.85695487025921,0.));
#173333=CARTESIAN_POINT('Ctrl Pts',(70.0060209754087,0.85695487025921,12.));
#173334=CARTESIAN_POINT('Ctrl Pts',(70.0172656933806,0.86009617066874,0.));
#173335=CARTESIAN_POINT('Ctrl Pts',(70.0172656933806,0.86009617066874,12.));
#173336=CARTESIAN_POINT('Ctrl Pts',(70.0322865492925,0.86430558366155,0.));
#173337=CARTESIAN_POINT('Ctrl Pts',(70.0322865492925,0.86430558366155,12.));
#173338=CARTESIAN_POINT('Ctrl Pts',(70.051109108301,0.869602377871129,0.));
#173339=CARTESIAN_POINT('Ctrl Pts',(70.051109108301,0.869602377871129,12.));
#173340=CARTESIAN_POINT('Ctrl Pts',(70.0699781183935,0.874934213255844,
0.));
#173341=CARTESIAN_POINT('Ctrl Pts',(70.0699781183935,0.874934213255844,
12.));
#173342=CARTESIAN_POINT('Ctrl Pts',(70.0888934967855,0.880301109660733,
0.));
#173343=CARTESIAN_POINT('Ctrl Pts',(70.0888934967855,0.880301109660733,
12.));
#173344=CARTESIAN_POINT('Ctrl Pts',(70.1078550938958,0.88570309480254,0.));
#173345=CARTESIAN_POINT('Ctrl Pts',(70.1078550938958,0.88570309480254,12.));
#173346=CARTESIAN_POINT('Ctrl Pts',(70.1268626950175,0.891140203464248,
0.));
#173347=CARTESIAN_POINT('Ctrl Pts',(70.1268626950175,0.891140203464248,
12.));
#173348=CARTESIAN_POINT('Ctrl Pts',(70.1459160490446,0.896612474371848,
0.));
#173349=CARTESIAN_POINT('Ctrl Pts',(70.1459160490446,0.896612474371848,
12.));
#173350=CARTESIAN_POINT('Ctrl Pts',(70.1650148905109,0.902119947629775,
0.));
#173351=CARTESIAN_POINT('Ctrl Pts',(70.1650148905109,0.902119947629775,
12.));
#173352=CARTESIAN_POINT('Ctrl Pts',(70.1841589635574,0.907662662015791,
0.));
#173353=CARTESIAN_POINT('Ctrl Pts',(70.1841589635574,0.907662662015791,
12.));
#173354=CARTESIAN_POINT('Ctrl Pts',(70.2033480471676,0.913240652090985,
0.));
#173355=CARTESIAN_POINT('Ctrl Pts',(70.2033480471676,0.913240652090985,
12.));
#173356=CARTESIAN_POINT('Ctrl Pts',(70.2225819470248,0.918853949157122,
0.));
#173357=CARTESIAN_POINT('Ctrl Pts',(70.2225819470248,0.918853949157122,
12.));
#173358=CARTESIAN_POINT('Ctrl Pts',(70.2418604835836,0.924502582639461,
0.));
#173359=CARTESIAN_POINT('Ctrl Pts',(70.2418604835836,0.924502582639461,
12.));
#173360=CARTESIAN_POINT('Ctrl Pts',(70.2611834821723,0.930186581235552,
0.));
#173361=CARTESIAN_POINT('Ctrl Pts',(70.2611834821723,0.930186581235552,
12.));
#173362=CARTESIAN_POINT('Ctrl Pts',(70.2805507606872,0.935905974336485,
0.));
#173363=CARTESIAN_POINT('Ctrl Pts',(70.2805507606872,0.935905974336485,
12.));
#173364=CARTESIAN_POINT('Ctrl Pts',(70.299962123399,0.941660792742984,0.));
#173365=CARTESIAN_POINT('Ctrl Pts',(70.299962123399,0.941660792742984,12.));
#173366=CARTESIAN_POINT('Ctrl Pts',(70.3194173673674,0.947451067929609,
0.));
#173367=CARTESIAN_POINT('Ctrl Pts',(70.3194173673674,0.947451067929609,
12.));
#173368=CARTESIAN_POINT('Ctrl Pts',(70.338916286458,0.953276831581247,0.));
#173369=CARTESIAN_POINT('Ctrl Pts',(70.338916286458,0.953276831581247,12.));
#173370=CARTESIAN_POINT('Ctrl Pts',(70.3584586759536,0.959138115058838,
0.));
#173371=CARTESIAN_POINT('Ctrl Pts',(70.3584586759536,0.959138115058838,
12.));
#173372=CARTESIAN_POINT('Ctrl Pts',(70.3780443377956,0.965034948786454,
0.));
#173373=CARTESIAN_POINT('Ctrl Pts',(70.3780443377956,0.965034948786454,
12.));
#173374=CARTESIAN_POINT('Ctrl Pts',(70.3976730803613,0.970967362281179,
0.));
#173375=CARTESIAN_POINT('Ctrl Pts',(70.3976730803613,0.970967362281179,
12.));
#173376=CARTESIAN_POINT('Ctrl Pts',(70.417344715957,0.976935384450047,0.));
#173377=CARTESIAN_POINT('Ctrl Pts',(70.417344715957,0.976935384450047,12.));
#173378=CARTESIAN_POINT('Ctrl Pts',(70.4370590590842,0.982939043792161,
0.));
#173379=CARTESIAN_POINT('Ctrl Pts',(70.4370590590842,0.982939043792161,
12.));
#173380=CARTESIAN_POINT('Ctrl Pts',(70.4568159243163,0.988978368643654,
0.));
#173381=CARTESIAN_POINT('Ctrl Pts',(70.4568159243163,0.988978368643654,
12.));
#173382=CARTESIAN_POINT('Ctrl Pts',(70.4766151245212,0.99505338737976,0.));
#173383=CARTESIAN_POINT('Ctrl Pts',(70.4766151245212,0.99505338737976,12.));
#173384=CARTESIAN_POINT('Ctrl Pts',(70.4964564717953,1.00116412831443,0.));
#173385=CARTESIAN_POINT('Ctrl Pts',(70.4964564717953,1.00116412831443,12.));
#173386=CARTESIAN_POINT('Ctrl Pts',(70.5163397782713,1.00731061960969,0.));
#173387=CARTESIAN_POINT('Ctrl Pts',(70.5163397782713,1.00731061960969,12.));
#173388=CARTESIAN_POINT('Ctrl Pts',(70.5362648569061,1.01349288918538,0.));
#173389=CARTESIAN_POINT('Ctrl Pts',(70.5362648569061,1.01349288918538,12.));
#173390=CARTESIAN_POINT('Ctrl Pts',(70.556231522419,1.01971096460597,0.));
#173391=CARTESIAN_POINT('Ctrl Pts',(70.556231522419,1.01971096460597,12.));
#173392=CARTESIAN_POINT('Ctrl Pts',(70.5762395916377,1.02596487304049,0.));
#173393=CARTESIAN_POINT('Ctrl Pts',(70.5762395916377,1.02596487304049,12.));
#173394=CARTESIAN_POINT('Ctrl Pts',(70.5962888829934,1.03225464132871,0.));
#173395=CARTESIAN_POINT('Ctrl Pts',(70.5962888829934,1.03225464132871,12.));
#173396=CARTESIAN_POINT('Ctrl Pts',(70.6163792162073,1.03858029601904,0.));
#173397=CARTESIAN_POINT('Ctrl Pts',(70.6163792162073,1.03858029601904,12.));
#173398=CARTESIAN_POINT('Ctrl Pts',(70.6365104119252,1.04494186341157,0.));
#173399=CARTESIAN_POINT('Ctrl Pts',(70.6365104119252,1.04494186341157,12.));
#173400=CARTESIAN_POINT('Ctrl Pts',(70.6566822912991,1.05133936960072,0.));
#173401=CARTESIAN_POINT('Ctrl Pts',(70.6566822912991,1.05133936960072,12.));
#173402=CARTESIAN_POINT('Ctrl Pts',(70.676894676009,1.05777284047731,0.));
#173403=CARTESIAN_POINT('Ctrl Pts',(70.676894676009,1.05777284047731,12.));
#173404=CARTESIAN_POINT('Ctrl Pts',(70.6971473884459,1.06424230171281,0.));
#173405=CARTESIAN_POINT('Ctrl Pts',(70.6971473884459,1.06424230171281,12.));
#173406=CARTESIAN_POINT('Ctrl Pts',(70.7174402518378,1.07074777874596,0.));
#173407=CARTESIAN_POINT('Ctrl Pts',(70.7174402518378,1.07074777874596,12.));
#173408=CARTESIAN_POINT('Ctrl Pts',(70.7377730903953,1.07728929676409,0.));
#173409=CARTESIAN_POINT('Ctrl Pts',(70.7377730903953,1.07728929676409,12.));
#173410=CARTESIAN_POINT('Ctrl Pts',(70.7581457294447,1.08386688068343,0.));
#173411=CARTESIAN_POINT('Ctrl Pts',(70.7581457294447,1.08386688068343,12.));
#173412=CARTESIAN_POINT('Ctrl Pts',(70.7785579953583,1.09048055516427,0.));
#173413=CARTESIAN_POINT('Ctrl Pts',(70.7785579953583,1.09048055516427,12.));
#173414=CARTESIAN_POINT('Ctrl Pts',(70.799009715484,1.09713034462266,0.));
#173415=CARTESIAN_POINT('Ctrl Pts',(70.799009715484,1.09713034462266,12.));
#173416=CARTESIAN_POINT('Ctrl Pts',(70.8195007180745,1.10381627323947,0.));
#173417=CARTESIAN_POINT('Ctrl Pts',(70.8195007180745,1.10381627323947,12.));
#173418=CARTESIAN_POINT('Ctrl Pts',(70.8400308322037,1.1105383649664,0.));
#173419=CARTESIAN_POINT('Ctrl Pts',(70.8400308322037,1.1105383649664,12.));
#173420=CARTESIAN_POINT('Ctrl Pts',(70.8605998877149,1.11729664352993,0.));
#173421=CARTESIAN_POINT('Ctrl Pts',(70.8605998877149,1.11729664352993,12.));
#173422=CARTESIAN_POINT('Ctrl Pts',(70.8812077152586,1.12409113243514,0.));
#173423=CARTESIAN_POINT('Ctrl Pts',(70.8812077152586,1.12409113243514,12.));
#173424=CARTESIAN_POINT('Ctrl Pts',(70.9018541463089,1.13092185496565,0.));
#173425=CARTESIAN_POINT('Ctrl Pts',(70.9018541463089,1.13092185496565,12.));
#173426=CARTESIAN_POINT('Ctrl Pts',(70.9225390131826,1.13778883418214,0.));
#173427=CARTESIAN_POINT('Ctrl Pts',(70.9225390131826,1.13778883418214,12.));
#173428=CARTESIAN_POINT('Ctrl Pts',(70.9432621490566,1.14469209291489,0.));
#173429=CARTESIAN_POINT('Ctrl Pts',(70.9432621490566,1.14469209291489,12.));
#173430=CARTESIAN_POINT('Ctrl Pts',(70.9640233879659,1.15163165376525,0.));
#173431=CARTESIAN_POINT('Ctrl Pts',(70.9640233879659,1.15163165376525,12.));
#173432=CARTESIAN_POINT('Ctrl Pts',(70.9848225647871,1.15860753911486,0.));
#173433=CARTESIAN_POINT('Ctrl Pts',(70.9848225647871,1.15860753911486,12.));
#173434=CARTESIAN_POINT('Ctrl Pts',(71.0056595152204,1.16561977112881,0.));
#173435=CARTESIAN_POINT('Ctrl Pts',(71.0056595152204,1.16561977112881,12.));
#173436=CARTESIAN_POINT('Ctrl Pts',(71.0265340757699,1.17266837175778,0.));
#173437=CARTESIAN_POINT('Ctrl Pts',(71.0265340757699,1.17266837175778,12.));
#173438=CARTESIAN_POINT('Ctrl Pts',(71.0474460837159,1.17975336273505,0.));
#173439=CARTESIAN_POINT('Ctrl Pts',(71.0474460837159,1.17975336273505,12.));
#173440=CARTESIAN_POINT('Ctrl Pts',(71.0683953771149,1.18687476558133,0.));
#173441=CARTESIAN_POINT('Ctrl Pts',(71.0683953771149,1.18687476558133,12.));
#173442=CARTESIAN_POINT('Ctrl Pts',(71.089381794801,1.19403260161003,0.));
#173443=CARTESIAN_POINT('Ctrl Pts',(71.089381794801,1.19403260161003,12.));
#173444=CARTESIAN_POINT('Ctrl Pts',(71.1104051763839,1.20122689192837,0.));
#173445=CARTESIAN_POINT('Ctrl Pts',(71.1104051763839,1.20122689192837,12.));
#173446=CARTESIAN_POINT('Ctrl Pts',(71.1314653622442,1.20845765743648,0.));
#173447=CARTESIAN_POINT('Ctrl Pts',(71.1314653622442,1.20845765743648,12.));
#173448=CARTESIAN_POINT('Ctrl Pts',(71.1525621935267,1.21572491882263,0.));
#173449=CARTESIAN_POINT('Ctrl Pts',(71.1525621935267,1.21572491882263,12.));
#173450=CARTESIAN_POINT('Ctrl Pts',(71.1736955121362,1.22302869657018,0.));
#173451=CARTESIAN_POINT('Ctrl Pts',(71.1736955121362,1.22302869657018,12.));
#173452=CARTESIAN_POINT('Ctrl Pts',(71.194865160732,1.2303690109624,0.));
#173453=CARTESIAN_POINT('Ctrl Pts',(71.194865160732,1.2303690109624,12.));
#173454=CARTESIAN_POINT('Ctrl Pts',(71.2160709827191,1.23774588208428,0.));
#173455=CARTESIAN_POINT('Ctrl Pts',(71.2160709827191,1.23774588208428,12.));
#173456=CARTESIAN_POINT('Ctrl Pts',(71.2373128222352,1.24515932982113,0.));
#173457=CARTESIAN_POINT('Ctrl Pts',(71.2373128222352,1.24515932982113,12.));
#173458=CARTESIAN_POINT('Ctrl Pts',(71.2585905241406,1.25260937385569,0.));
#173459=CARTESIAN_POINT('Ctrl Pts',(71.2585905241406,1.25260937385569,12.));
#173460=CARTESIAN_POINT('Ctrl Pts',(71.2799039340175,1.26009603367571,0.));
#173461=CARTESIAN_POINT('Ctrl Pts',(71.2799039340175,1.26009603367571,12.));
#173462=CARTESIAN_POINT('Ctrl Pts',(71.3012528981661,1.26761932857725,0.));
#173463=CARTESIAN_POINT('Ctrl Pts',(71.3012528981661,1.26761932857725,12.));
#173464=CARTESIAN_POINT('Ctrl Pts',(71.3226372635996,1.27517927766609,0.));
#173465=CARTESIAN_POINT('Ctrl Pts',(71.3226372635996,1.27517927766609,12.));
#173466=CARTESIAN_POINT('Ctrl Pts',(71.3440568780347,1.28277589985472,0.));
#173467=CARTESIAN_POINT('Ctrl Pts',(71.3440568780347,1.28277589985472,12.));
#173468=CARTESIAN_POINT('Ctrl Pts',(71.3655115898827,1.2904092138606,0.));
#173469=CARTESIAN_POINT('Ctrl Pts',(71.3655115898827,1.2904092138606,12.));
#173470=CARTESIAN_POINT('Ctrl Pts',(71.3870012482499,1.29807923821414,0.));
#173471=CARTESIAN_POINT('Ctrl Pts',(71.3870012482499,1.29807923821414,12.));
#173472=CARTESIAN_POINT('Ctrl Pts',(71.4085257029322,1.3057859912614,0.));
#173473=CARTESIAN_POINT('Ctrl Pts',(71.4085257029322,1.3057859912614,12.));
#173474=CARTESIAN_POINT('Ctrl Pts',(71.4300848044087,1.31352949116538,0.));
#173475=CARTESIAN_POINT('Ctrl Pts',(71.4300848044087,1.31352949116538,12.));
#173476=CARTESIAN_POINT('Ctrl Pts',(71.4516784038317,1.32130975590226,0.));
#173477=CARTESIAN_POINT('Ctrl Pts',(71.4516784038317,1.32130975590226,12.));
#173478=CARTESIAN_POINT('Ctrl Pts',(71.4733063530187,1.32912680326124,0.));
#173479=CARTESIAN_POINT('Ctrl Pts',(71.4733063530187,1.32912680326124,12.));
#173480=CARTESIAN_POINT('Ctrl Pts',(71.4949685044522,1.3369806508522,0.));
#173481=CARTESIAN_POINT('Ctrl Pts',(71.4949685044522,1.3369806508522,12.));
#173482=CARTESIAN_POINT('Ctrl Pts',(71.516664711275,1.34487131610781,0.));
#173483=CARTESIAN_POINT('Ctrl Pts',(71.516664711275,1.34487131610781,12.));
#173484=CARTESIAN_POINT('Ctrl Pts',(71.5383948272845,1.35279881628455,0.));
#173485=CARTESIAN_POINT('Ctrl Pts',(71.5383948272845,1.35279881628455,12.));
#173486=CARTESIAN_POINT('Ctrl Pts',(71.5601587069217,1.36076316845817,0.));
#173487=CARTESIAN_POINT('Ctrl Pts',(71.5601587069217,1.36076316845817,12.));
#173488=CARTESIAN_POINT('Ctrl Pts',(71.5819562052663,1.36876438952466,0.));
#173489=CARTESIAN_POINT('Ctrl Pts',(71.5819562052663,1.36876438952466,12.));
#173490=CARTESIAN_POINT('Ctrl Pts',(71.6037871780385,1.3768024962078,0.));
#173491=CARTESIAN_POINT('Ctrl Pts',(71.6037871780385,1.3768024962078,12.));
#173492=CARTESIAN_POINT('Ctrl Pts',(71.625651481593,1.38487750506083,0.));
#173493=CARTESIAN_POINT('Ctrl Pts',(71.625651481593,1.38487750506083,12.));
#173494=CARTESIAN_POINT('Ctrl Pts',(71.6475489729134,1.39298943246723,0.));
#173495=CARTESIAN_POINT('Ctrl Pts',(71.6475489729134,1.39298943246723,12.));
#173496=CARTESIAN_POINT('Ctrl Pts',(71.6694795096001,1.40113829463577,0.));
#173497=CARTESIAN_POINT('Ctrl Pts',(71.6694795096001,1.40113829463577,12.));
#173498=CARTESIAN_POINT('Ctrl Pts',(71.6914429498663,1.40932410760249,0.));
#173499=CARTESIAN_POINT('Ctrl Pts',(71.6914429498663,1.40932410760249,12.));
#173500=CARTESIAN_POINT('Ctrl Pts',(71.7134391525389,1.41754688723773,0.));
#173501=CARTESIAN_POINT('Ctrl Pts',(71.7134391525389,1.41754688723773,12.));
#173502=CARTESIAN_POINT('Ctrl Pts',(71.7354679770528,1.4258066492477,0.));
#173503=CARTESIAN_POINT('Ctrl Pts',(71.7354679770528,1.4258066492477,12.));
#173504=CARTESIAN_POINT('Ctrl Pts',(71.7575292834469,1.43410340917496,0.));
#173505=CARTESIAN_POINT('Ctrl Pts',(71.7575292834469,1.43410340917496,12.));
#173506=CARTESIAN_POINT('Ctrl Pts',(71.7796229323526,1.44243718239316,0.));
#173507=CARTESIAN_POINT('Ctrl Pts',(71.7796229323526,1.44243718239316,12.));
#173508=CARTESIAN_POINT('Ctrl Pts',(71.8017487849895,1.45080798410966,0.));
#173509=CARTESIAN_POINT('Ctrl Pts',(71.8017487849895,1.45080798410966,12.));
#173510=CARTESIAN_POINT('Ctrl Pts',(71.8239067031683,1.45921582937232,0.));
#173511=CARTESIAN_POINT('Ctrl Pts',(71.8239067031683,1.45921582937232,12.));
#173512=CARTESIAN_POINT('Ctrl Pts',(71.8460965492838,1.46766073307089,0.));
#173513=CARTESIAN_POINT('Ctrl Pts',(71.8460965492838,1.46766073307089,12.));
#173514=CARTESIAN_POINT('Ctrl Pts',(71.8683181863116,1.47614270993729,0.));
#173515=CARTESIAN_POINT('Ctrl Pts',(71.8683181863116,1.47614270993729,12.));
#173516=CARTESIAN_POINT('Ctrl Pts',(71.8905714777961,1.4846617745402,0.));
#173517=CARTESIAN_POINT('Ctrl Pts',(71.8905714777961,1.4846617745402,12.));
#173518=CARTESIAN_POINT('Ctrl Pts',(71.912856287848,1.49321794128799,0.));
#173519=CARTESIAN_POINT('Ctrl Pts',(71.912856287848,1.49321794128799,12.));
#173520=CARTESIAN_POINT('Ctrl Pts',(71.9351724811443,1.50181122443535,0.));
#173521=CARTESIAN_POINT('Ctrl Pts',(71.9351724811443,1.50181122443535,12.));
#173522=CARTESIAN_POINT('Ctrl Pts',(71.9575199229241,1.51044163808454,0.));
#173523=CARTESIAN_POINT('Ctrl Pts',(71.9575199229241,1.51044163808454,12.));
#173524=CARTESIAN_POINT('Ctrl Pts',(71.979898478983,1.51910919618566,0.));
#173525=CARTESIAN_POINT('Ctrl Pts',(71.979898478983,1.51910919618566,12.));
#173526=CARTESIAN_POINT('Ctrl Pts',(72.0023080156647,1.52781391253102,0.));
#173527=CARTESIAN_POINT('Ctrl Pts',(72.0023080156647,1.52781391253102,12.));
#173528=CARTESIAN_POINT('Ctrl Pts',(72.0247483998578,1.53655580075813,0.));
#173529=CARTESIAN_POINT('Ctrl Pts',(72.0247483998578,1.53655580075813,12.));
#173530=CARTESIAN_POINT('Ctrl Pts',(72.0472194989963,1.54533487435627,0.));
#173531=CARTESIAN_POINT('Ctrl Pts',(72.0472194989963,1.54533487435627,12.));
#173532=CARTESIAN_POINT('Ctrl Pts',(72.0697211810545,1.55415114666774,0.));
#173533=CARTESIAN_POINT('Ctrl Pts',(72.0697211810545,1.55415114666774,12.));
#173534=CARTESIAN_POINT('Ctrl Pts',(72.0922533145433,1.56300463088809,0.));
#173535=CARTESIAN_POINT('Ctrl Pts',(72.0922533145433,1.56300463088809,12.));
#173536=CARTESIAN_POINT('Ctrl Pts',(72.1148157684995,1.57189534006041,0.));
#173537=CARTESIAN_POINT('Ctrl Pts',(72.1148157684995,1.57189534006041,12.));
#173538=CARTESIAN_POINT('Ctrl Pts',(72.1374084124839,1.58082328707804,0.));
#173539=CARTESIAN_POINT('Ctrl Pts',(72.1374084124839,1.58082328707804,12.));
#173540=CARTESIAN_POINT('Ctrl Pts',(72.1600311165821,1.58978848469124,0.));
#173541=CARTESIAN_POINT('Ctrl Pts',(72.1600311165821,1.58978848469124,12.));
#173542=CARTESIAN_POINT('Ctrl Pts',(72.1826837514001,1.59879094550848,0.));
#173543=CARTESIAN_POINT('Ctrl Pts',(72.1826837514001,1.59879094550848,12.));
#173544=CARTESIAN_POINT('Ctrl Pts',(72.2053661880608,1.60783068199664,0.));
#173545=CARTESIAN_POINT('Ctrl Pts',(72.2053661880608,1.60783068199664,12.));
#173546=CARTESIAN_POINT('Ctrl Pts',(72.2280782981937,1.61690770647541,0.));
#173547=CARTESIAN_POINT('Ctrl Pts',(72.2280782981937,1.61690770647541,12.));
#173548=CARTESIAN_POINT('Ctrl Pts',(72.2508199539323,1.62602203111931,0.));
#173549=CARTESIAN_POINT('Ctrl Pts',(72.2508199539323,1.62602203111931,12.));
#173550=CARTESIAN_POINT('Ctrl Pts',(72.2735910279149,1.63517366796464,0.));
#173551=CARTESIAN_POINT('Ctrl Pts',(72.2735910279149,1.63517366796464,12.));
#173552=CARTESIAN_POINT('Ctrl Pts',(72.2963913932813,1.64436262891079,0.));
#173553=CARTESIAN_POINT('Ctrl Pts',(72.2963913932813,1.64436262891079,12.));
#173554=CARTESIAN_POINT('Ctrl Pts',(72.319220923669,1.65358892572063,0.));
#173555=CARTESIAN_POINT('Ctrl Pts',(72.319220923669,1.65358892572063,12.));
#173556=CARTESIAN_POINT('Ctrl Pts',(72.3420794932047,1.66285257001497,0.));
#173557=CARTESIAN_POINT('Ctrl Pts',(72.3420794932047,1.66285257001497,12.));
#173558=CARTESIAN_POINT('Ctrl Pts',(72.3649669765004,1.67215357327366,0.));
#173559=CARTESIAN_POINT('Ctrl Pts',(72.3649669765004,1.67215357327366,12.));
#173560=CARTESIAN_POINT('Ctrl Pts',(72.387883248654,1.68149194684282,0.));
#173561=CARTESIAN_POINT('Ctrl Pts',(72.387883248654,1.68149194684282,12.));
#173562=CARTESIAN_POINT('Ctrl Pts',(72.4108281852467,1.69086770193638,0.));
#173563=CARTESIAN_POINT('Ctrl Pts',(72.4108281852467,1.69086770193638,12.));
#173564=CARTESIAN_POINT('Ctrl Pts',(72.4338016623391,1.70028084963648,0.));
#173565=CARTESIAN_POINT('Ctrl Pts',(72.4338016623391,1.70028084963648,12.));
#173566=CARTESIAN_POINT('Ctrl Pts',(72.456803556463,1.70973140088842,0.));
#173567=CARTESIAN_POINT('Ctrl Pts',(72.456803556463,1.70973140088842,12.));
#173568=CARTESIAN_POINT('Ctrl Pts',(72.479833744618,1.71921936650039,0.));
#173569=CARTESIAN_POINT('Ctrl Pts',(72.479833744618,1.71921936650039,12.));
#173570=CARTESIAN_POINT('Ctrl Pts',(72.5028921042721,1.72874475715104,0.));
#173571=CARTESIAN_POINT('Ctrl Pts',(72.5028921042721,1.72874475715104,12.));
#173572=CARTESIAN_POINT('Ctrl Pts',(72.5259785133595,1.73830758339125,0.));
#173573=CARTESIAN_POINT('Ctrl Pts',(72.5259785133595,1.73830758339125,12.));
#173574=CARTESIAN_POINT('Ctrl Pts',(72.5490928502769,1.74790785564474,0.));
#173575=CARTESIAN_POINT('Ctrl Pts',(72.5490928502769,1.74790785564474,12.));
#173576=CARTESIAN_POINT('Ctrl Pts',(72.5722349938774,1.75754558420345,0.));
#173577=CARTESIAN_POINT('Ctrl Pts',(72.5722349938774,1.75754558420345,12.));
#173578=CARTESIAN_POINT('Ctrl Pts',(72.5954048234638,1.76722077922575,0.));
#173579=CARTESIAN_POINT('Ctrl Pts',(72.5954048234638,1.76722077922575,12.));
#173580=CARTESIAN_POINT('Ctrl Pts',(72.6186022187907,1.77693345074427,0.));
#173581=CARTESIAN_POINT('Ctrl Pts',(72.6186022187907,1.77693345074427,12.));
#173582=CARTESIAN_POINT('Ctrl Pts',(72.6418270600619,1.78668360866812,0.));
#173583=CARTESIAN_POINT('Ctrl Pts',(72.6418270600619,1.78668360866812,12.));
#173584=CARTESIAN_POINT('Ctrl Pts',(72.6650792279274,1.79647126278359,0.));
#173585=CARTESIAN_POINT('Ctrl Pts',(72.6650792279274,1.79647126278359,12.));
#173586=CARTESIAN_POINT('Ctrl Pts',(72.6883586034769,1.80629642275051,0.));
#173587=CARTESIAN_POINT('Ctrl Pts',(72.6883586034769,1.80629642275051,12.));
#173588=CARTESIAN_POINT('Ctrl Pts',(72.7116650682344,1.81615909809871,0.));
#173589=CARTESIAN_POINT('Ctrl Pts',(72.7116650682344,1.81615909809871,12.));
#173590=CARTESIAN_POINT('Ctrl Pts',(72.7349985041592,1.82605929823565,0.));
#173591=CARTESIAN_POINT('Ctrl Pts',(72.7349985041592,1.82605929823565,12.));
#173592=CARTESIAN_POINT('Ctrl Pts',(72.7583587936447,1.83599703244925,0.));
#173593=CARTESIAN_POINT('Ctrl Pts',(72.7583587936447,1.83599703244925,12.));
#173594=CARTESIAN_POINT('Ctrl Pts',(72.7817458195155,1.84597230990858,0.));
#173595=CARTESIAN_POINT('Ctrl Pts',(72.7817458195155,1.84597230990858,12.));
#173596=CARTESIAN_POINT('Ctrl Pts',(72.8051594650222,1.85598513966114,0.));
#173597=CARTESIAN_POINT('Ctrl Pts',(72.8051594650222,1.85598513966114,12.));
#173598=CARTESIAN_POINT('Ctrl Pts',(72.8285996138359,1.86603553062772,0.));
#173599=CARTESIAN_POINT('Ctrl Pts',(72.8285996138359,1.86603553062772,12.));
#173600=CARTESIAN_POINT('Ctrl Pts',(72.8520661500477,1.87612349160945,0.));
#173601=CARTESIAN_POINT('Ctrl Pts',(72.8520661500477,1.87612349160945,12.));
#173602=CARTESIAN_POINT('Ctrl Pts',(72.875558958168,1.88624903129189,0.));
#173603=CARTESIAN_POINT('Ctrl Pts',(72.875558958168,1.88624903129189,12.));
#173604=CARTESIAN_POINT('Ctrl Pts',(72.8990779231226,1.89641215824583,0.));
#173605=CARTESIAN_POINT('Ctrl Pts',(72.8990779231226,1.89641215824583,12.));
#173606=CARTESIAN_POINT('Ctrl Pts',(72.9226229302478,1.90661288092587,0.));
#173607=CARTESIAN_POINT('Ctrl Pts',(72.9226229302478,1.90661288092587,12.));
#173608=CARTESIAN_POINT('Ctrl Pts',(72.9461938652811,1.91685120766437,0.));
#173609=CARTESIAN_POINT('Ctrl Pts',(72.9461938652811,1.91685120766437,12.));
#173610=CARTESIAN_POINT('Ctrl Pts',(72.9697906143636,1.92712714667661,0.));
#173611=CARTESIAN_POINT('Ctrl Pts',(72.9697906143636,1.92712714667661,12.));
#173612=CARTESIAN_POINT('Ctrl Pts',(72.9934130640415,1.93744070606566,0.));
#173613=CARTESIAN_POINT('Ctrl Pts',(72.9934130640415,1.93744070606566,12.));
#173614=CARTESIAN_POINT('Ctrl Pts',(73.0170611012661,1.94779189382303,0.));
#173615=CARTESIAN_POINT('Ctrl Pts',(73.0170611012661,1.94779189382303,12.));
#173616=CARTESIAN_POINT('Ctrl Pts',(73.040734613391,1.95818071782768,0.));
#173617=CARTESIAN_POINT('Ctrl Pts',(73.040734613391,1.95818071782768,12.));
#173618=CARTESIAN_POINT('Ctrl Pts',(73.0644334881673,1.96860718583933,0.));
#173619=CARTESIAN_POINT('Ctrl Pts',(73.0644334881673,1.96860718583933,12.));
#173620=CARTESIAN_POINT('Ctrl Pts',(73.0881576137407,1.97907130550158,0.));
#173621=CARTESIAN_POINT('Ctrl Pts',(73.0881576137407,1.97907130550158,12.));
#173622=CARTESIAN_POINT('Ctrl Pts',(73.1119068786475,1.98957308434919,0.));
#173623=CARTESIAN_POINT('Ctrl Pts',(73.1119068786475,1.98957308434919,12.));
#173624=CARTESIAN_POINT('Ctrl Pts',(73.1356811718091,2.00011252980982,0.));
#173625=CARTESIAN_POINT('Ctrl Pts',(73.1356811718091,2.00011252980982,12.));
#173626=CARTESIAN_POINT('Ctrl Pts',(73.1594803825252,2.01068964920468,0.));
#173627=CARTESIAN_POINT('Ctrl Pts',(73.1594803825252,2.01068964920468,12.));
#173628=CARTESIAN_POINT('Ctrl Pts',(73.183304400462,2.02130444974362,0.));
#173629=CARTESIAN_POINT('Ctrl Pts',(73.183304400462,2.02130444974362,12.));
#173630=CARTESIAN_POINT('Ctrl Pts',(73.2071531156504,2.03195693852455,0.));
#173631=CARTESIAN_POINT('Ctrl Pts',(73.2071531156504,2.03195693852455,12.));
#173632=CARTESIAN_POINT('Ctrl Pts',(73.2310264184976,2.04264712253929,0.));
#173633=CARTESIAN_POINT('Ctrl Pts',(73.2310264184976,2.04264712253929,12.));
#173634=CARTESIAN_POINT('Ctrl Pts',(73.2549241997953,2.05337500867403,0.));
#173635=CARTESIAN_POINT('Ctrl Pts',(73.2549241997953,2.05337500867403,12.));
#173636=CARTESIAN_POINT('Ctrl Pts',(73.2788463507246,2.06414060370835,0.));
#173637=CARTESIAN_POINT('Ctrl Pts',(73.2788463507246,2.06414060370835,12.));
#173638=CARTESIAN_POINT('Ctrl Pts',(73.3027927628626,2.07494391430941,0.));
#173639=CARTESIAN_POINT('Ctrl Pts',(73.3027927628626,2.07494391430941,12.));
#173640=CARTESIAN_POINT('Ctrl Pts',(73.3267633281807,2.08578494702744,0.));
#173641=CARTESIAN_POINT('Ctrl Pts',(73.3267633281807,2.08578494702744,12.));
#173642=CARTESIAN_POINT('Ctrl Pts',(73.3507579390239,2.09666370830717,0.));
#173643=CARTESIAN_POINT('Ctrl Pts',(73.3507579390239,2.09666370830717,12.));
#173644=CARTESIAN_POINT('Ctrl Pts',(73.3747764880893,2.1075802044939,0.));
#173645=CARTESIAN_POINT('Ctrl Pts',(73.3747764880893,2.1075802044939,12.));
#173646=CARTESIAN_POINT('Ctrl Pts',(73.3988188684021,2.11853444183762,0.));
#173647=CARTESIAN_POINT('Ctrl Pts',(73.3988188684021,2.11853444183762,12.));
#173648=CARTESIAN_POINT('Ctrl Pts',(73.4228849732925,2.12952642649368,0.));
#173649=CARTESIAN_POINT('Ctrl Pts',(73.4228849732925,2.12952642649368,12.));
#173650=CARTESIAN_POINT('Ctrl Pts',(73.4469746963637,2.14055616452058,0.));
#173651=CARTESIAN_POINT('Ctrl Pts',(73.4469746963637,2.14055616452058,12.));
#173652=CARTESIAN_POINT('Ctrl Pts',(73.4710879315382,2.15162366187907,0.));
#173653=CARTESIAN_POINT('Ctrl Pts',(73.4710879315382,2.15162366187907,12.));
#173654=CARTESIAN_POINT('Ctrl Pts',(73.4952245731054,2.1627289244292,0.));
#173655=CARTESIAN_POINT('Ctrl Pts',(73.4952245731054,2.1627289244292,12.));
#173656=CARTESIAN_POINT('Ctrl Pts',(73.5193845157708,2.17387195792306,0.));
#173657=CARTESIAN_POINT('Ctrl Pts',(73.5193845157708,2.17387195792306,12.));
#173658=CARTESIAN_POINT('Ctrl Pts',(73.5435676546929,2.18505276799754,0.));
#173659=CARTESIAN_POINT('Ctrl Pts',(73.5435676546929,2.18505276799754,12.));
#173660=CARTESIAN_POINT('Ctrl Pts',(73.5677738855452,2.19627136015679,0.));
#173661=CARTESIAN_POINT('Ctrl Pts',(73.5677738855452,2.19627136015679,12.));
#173662=CARTESIAN_POINT('Ctrl Pts',(73.5920031044595,2.20752773978349,0.));
#173663=CARTESIAN_POINT('Ctrl Pts',(73.5920031044595,2.20752773978349,12.));
#173664=CARTESIAN_POINT('Ctrl Pts',(73.6162552079038,2.21882191216519,0.));
#173665=CARTESIAN_POINT('Ctrl Pts',(73.6162552079038,2.21882191216519,12.));
#173666=CARTESIAN_POINT('Ctrl Pts',(73.6405300925712,2.23015388251288,0.));
#173667=CARTESIAN_POINT('Ctrl Pts',(73.6405300925712,2.23015388251288,12.));
#173668=CARTESIAN_POINT('Ctrl Pts',(73.6648276552767,2.24152365597698,0.));
#173669=CARTESIAN_POINT('Ctrl Pts',(73.6648276552767,2.24152365597698,12.));
#173670=CARTESIAN_POINT('Ctrl Pts',(73.6891477928129,2.25293123766425,0.));
#173671=CARTESIAN_POINT('Ctrl Pts',(73.6891477928129,2.25293123766425,12.));
#173672=CARTESIAN_POINT('Ctrl Pts',(73.7134904019389,2.26437663263667,0.));
#173673=CARTESIAN_POINT('Ctrl Pts',(73.7134904019389,2.26437663263667,12.));
#173674=CARTESIAN_POINT('Ctrl Pts',(73.7378553796807,2.27585984587199,0.));
#173675=CARTESIAN_POINT('Ctrl Pts',(73.7378553796807,2.27585984587199,12.));
#173676=CARTESIAN_POINT('Ctrl Pts',(73.762242623566,2.28738088222864,0.));
#173677=CARTESIAN_POINT('Ctrl Pts',(73.762242623566,2.28738088222864,12.));
#173678=CARTESIAN_POINT('Ctrl Pts',(73.786652031885,2.29893974640435,0.));
#173679=CARTESIAN_POINT('Ctrl Pts',(73.786652031885,2.29893974640435,12.));
#173680=CARTESIAN_POINT('Ctrl Pts',(73.8110835039327,2.31053644289417,0.));
#173681=CARTESIAN_POINT('Ctrl Pts',(73.8110835039327,2.31053644289417,12.));
#173682=CARTESIAN_POINT('Ctrl Pts',(73.8355369402706,2.32217097594198,0.));
#173683=CARTESIAN_POINT('Ctrl Pts',(73.8355369402706,2.32217097594198,12.));
#173684=CARTESIAN_POINT('Ctrl Pts',(73.8600122421468,2.33384334963958,0.));
#173685=CARTESIAN_POINT('Ctrl Pts',(73.8600122421468,2.33384334963958,12.));
#173686=CARTESIAN_POINT('Ctrl Pts',(73.8845093109274,2.34555356802121,0.));
#173687=CARTESIAN_POINT('Ctrl Pts',(73.8845093109274,2.34555356802121,12.));
#173688=CARTESIAN_POINT('Ctrl Pts',(73.9090280474712,2.35730163516316,0.));
#173689=CARTESIAN_POINT('Ctrl Pts',(73.9090280474712,2.35730163516316,12.));
#173690=CARTESIAN_POINT('Ctrl Pts',(73.9335683516404,2.36908755526004,0.));
#173691=CARTESIAN_POINT('Ctrl Pts',(73.9335683516404,2.36908755526004,12.));
#173692=CARTESIAN_POINT('Ctrl Pts',(73.958130121465,2.38091133274961,0.));
#173693=CARTESIAN_POINT('Ctrl Pts',(73.958130121465,2.38091133274961,12.));
#173694=CARTESIAN_POINT('Ctrl Pts',(73.9827132538206,2.39277297220757,0.));
#173695=CARTESIAN_POINT('Ctrl Pts',(73.9827132538206,2.39277297220757,12.));
#173696=CARTESIAN_POINT('Ctrl Pts',(74.0073176459344,2.40467247811537,0.));
#173697=CARTESIAN_POINT('Ctrl Pts',(74.0073176459344,2.40467247811537,12.));
#173698=CARTESIAN_POINT('Ctrl Pts',(74.0319431966989,2.41660985465252,0.));
#173699=CARTESIAN_POINT('Ctrl Pts',(74.0319431966989,2.41660985465252,12.));
#173700=CARTESIAN_POINT('Ctrl Pts',(74.0565898079218,2.42858510549779,0.));
#173701=CARTESIAN_POINT('Ctrl Pts',(74.0565898079218,2.42858510549779,12.));
#173702=CARTESIAN_POINT('Ctrl Pts',(74.0812573859411,2.44059823356676,0.));
#173703=CARTESIAN_POINT('Ctrl Pts',(74.0812573859411,2.44059823356676,12.));
#173704=CARTESIAN_POINT('Ctrl Pts',(74.1059458420067,2.45264924094776,0.));
#173705=CARTESIAN_POINT('Ctrl Pts',(74.1059458420067,2.45264924094776,12.));
#173706=CARTESIAN_POINT('Ctrl Pts',(74.1306550887071,2.4647381294796,0.));
#173707=CARTESIAN_POINT('Ctrl Pts',(74.1306550887071,2.4647381294796,12.));
#173708=CARTESIAN_POINT('Ctrl Pts',(74.155385037148,2.47686490120355,0.));
#173709=CARTESIAN_POINT('Ctrl Pts',(74.155385037148,2.47686490120355,12.));
#173710=CARTESIAN_POINT('Ctrl Pts',(74.1801355936907,2.48902955888385,0.));
#173711=CARTESIAN_POINT('Ctrl Pts',(74.1801355936907,2.48902955888385,12.));
#173712=CARTESIAN_POINT('Ctrl Pts',(74.2049066572031,2.50123210644136,0.));
#173713=CARTESIAN_POINT('Ctrl Pts',(74.2049066572031,2.50123210644136,12.));
#173714=CARTESIAN_POINT('Ctrl Pts',(74.229698115223,2.51347254956168,0.));
#173715=CARTESIAN_POINT('Ctrl Pts',(74.229698115223,2.51347254956168,12.));
#173716=CARTESIAN_POINT('Ctrl Pts',(74.2545098494824,2.52575089478304,0.));
#173717=CARTESIAN_POINT('Ctrl Pts',(74.2545098494824,2.52575089478304,12.));
#173718=CARTESIAN_POINT('Ctrl Pts',(74.2793417427308,2.53806714838287,0.));
#173719=CARTESIAN_POINT('Ctrl Pts',(74.2793417427308,2.53806714838287,12.));
#173720=CARTESIAN_POINT('Ctrl Pts',(74.3041936853468,2.55042131526781,0.));
#173721=CARTESIAN_POINT('Ctrl Pts',(74.3041936853468,2.55042131526781,12.));
#173722=CARTESIAN_POINT('Ctrl Pts',(74.329065581483,2.56281339800018,0.));
#173723=CARTESIAN_POINT('Ctrl Pts',(74.329065581483,2.56281339800018,12.));
#173724=CARTESIAN_POINT('Ctrl Pts',(74.3539573567672,2.5752433954139,0.));
#173725=CARTESIAN_POINT('Ctrl Pts',(74.3539573567672,2.5752433954139,12.));
#173726=CARTESIAN_POINT('Ctrl Pts',(74.3788689603363,2.58771130268176,0.));
#173727=CARTESIAN_POINT('Ctrl Pts',(74.3788689603363,2.58771130268176,12.));
#173728=CARTESIAN_POINT('Ctrl Pts',(74.4038003594771,2.60021711326978,0.));
#173729=CARTESIAN_POINT('Ctrl Pts',(74.4038003594771,2.60021711326978,12.));
#173730=CARTESIAN_POINT('Ctrl Pts',(74.4237613007988,2.61025207898403,0.));
#173731=CARTESIAN_POINT('Ctrl Pts',(74.4237613007988,2.61025207898403,12.));
#173732=CARTESIAN_POINT('Ctrl Pts',(74.4387409032207,2.61779535432113,0.));
#173733=CARTESIAN_POINT('Ctrl Pts',(74.4387409032207,2.61779535432113,12.));
#173734=CARTESIAN_POINT('Ctrl Pts',(74.4487312586464,2.62283178248203,0.));
#173735=CARTESIAN_POINT('Ctrl Pts',(74.4487312586464,2.62283178248203,12.));
#173736=CARTESIAN_POINT('Ctrl Pts',(74.4537274248118,2.62535189104656,0.));
#173737=CARTESIAN_POINT('Ctrl Pts',(74.4537274248118,2.62535189104656,12.));
#173738=CARTESIAN_POINT('Ctrl Pts',(69.9947925310006,0.853825826608988,
0.));
#173739=CARTESIAN_POINT('Ctrl Pts',(69.9985337959407,0.854867673848601,
0.));
#173740=CARTESIAN_POINT('Ctrl Pts',(70.0060209754087,0.85695487025921,0.));
#173741=CARTESIAN_POINT('Ctrl Pts',(70.0172656933806,0.86009617066874,0.));
#173742=CARTESIAN_POINT('Ctrl Pts',(70.0322865492925,0.86430558366155,0.));
#173743=CARTESIAN_POINT('Ctrl Pts',(70.051109108301,0.869602377871129,0.));
#173744=CARTESIAN_POINT('Ctrl Pts',(70.0699781183935,0.874934213255844,
0.));
#173745=CARTESIAN_POINT('Ctrl Pts',(70.0888934967855,0.880301109660733,
0.));
#173746=CARTESIAN_POINT('Ctrl Pts',(70.1078550938958,0.88570309480254,0.));
#173747=CARTESIAN_POINT('Ctrl Pts',(70.1268626950175,0.891140203464248,
0.));
#173748=CARTESIAN_POINT('Ctrl Pts',(70.1459160490446,0.896612474371848,
0.));
#173749=CARTESIAN_POINT('Ctrl Pts',(70.1650148905109,0.902119947629775,
0.));
#173750=CARTESIAN_POINT('Ctrl Pts',(70.1841589635574,0.907662662015791,
0.));
#173751=CARTESIAN_POINT('Ctrl Pts',(70.2033480471676,0.913240652090985,
0.));
#173752=CARTESIAN_POINT('Ctrl Pts',(70.2225819470248,0.918853949157122,
0.));
#173753=CARTESIAN_POINT('Ctrl Pts',(70.2418604835836,0.924502582639461,
0.));
#173754=CARTESIAN_POINT('Ctrl Pts',(70.2611834821723,0.930186581235552,
0.));
#173755=CARTESIAN_POINT('Ctrl Pts',(70.2805507606872,0.935905974336485,
0.));
#173756=CARTESIAN_POINT('Ctrl Pts',(70.299962123399,0.941660792742984,0.));
#173757=CARTESIAN_POINT('Ctrl Pts',(70.3194173673674,0.947451067929609,
0.));
#173758=CARTESIAN_POINT('Ctrl Pts',(70.338916286458,0.953276831581247,0.));
#173759=CARTESIAN_POINT('Ctrl Pts',(70.3584586759536,0.959138115058838,
0.));
#173760=CARTESIAN_POINT('Ctrl Pts',(70.3780443377956,0.965034948786454,
0.));
#173761=CARTESIAN_POINT('Ctrl Pts',(70.3976730803613,0.970967362281179,
0.));
#173762=CARTESIAN_POINT('Ctrl Pts',(70.417344715957,0.976935384450047,0.));
#173763=CARTESIAN_POINT('Ctrl Pts',(70.4370590590842,0.982939043792161,
0.));
#173764=CARTESIAN_POINT('Ctrl Pts',(70.4568159243163,0.988978368643654,
0.));
#173765=CARTESIAN_POINT('Ctrl Pts',(70.4766151245212,0.99505338737976,0.));
#173766=CARTESIAN_POINT('Ctrl Pts',(70.4964564717953,1.00116412831443,0.));
#173767=CARTESIAN_POINT('Ctrl Pts',(70.5163397782713,1.00731061960969,0.));
#173768=CARTESIAN_POINT('Ctrl Pts',(70.5362648569061,1.01349288918538,0.));
#173769=CARTESIAN_POINT('Ctrl Pts',(70.556231522419,1.01971096460597,0.));
#173770=CARTESIAN_POINT('Ctrl Pts',(70.5762395916377,1.02596487304049,0.));
#173771=CARTESIAN_POINT('Ctrl Pts',(70.5962888829934,1.03225464132871,0.));
#173772=CARTESIAN_POINT('Ctrl Pts',(70.6163792162073,1.03858029601904,0.));
#173773=CARTESIAN_POINT('Ctrl Pts',(70.6365104119252,1.04494186341157,0.));
#173774=CARTESIAN_POINT('Ctrl Pts',(70.6566822912991,1.05133936960072,0.));
#173775=CARTESIAN_POINT('Ctrl Pts',(70.676894676009,1.05777284047731,0.));
#173776=CARTESIAN_POINT('Ctrl Pts',(70.6971473884459,1.06424230171281,0.));
#173777=CARTESIAN_POINT('Ctrl Pts',(70.7174402518378,1.07074777874596,0.));
#173778=CARTESIAN_POINT('Ctrl Pts',(70.7377730903953,1.07728929676409,0.));
#173779=CARTESIAN_POINT('Ctrl Pts',(70.7581457294447,1.08386688068343,0.));
#173780=CARTESIAN_POINT('Ctrl Pts',(70.7785579953583,1.09048055516427,0.));
#173781=CARTESIAN_POINT('Ctrl Pts',(70.799009715484,1.09713034462266,0.));
#173782=CARTESIAN_POINT('Ctrl Pts',(70.8195007180745,1.10381627323947,0.));
#173783=CARTESIAN_POINT('Ctrl Pts',(70.8400308322037,1.1105383649664,0.));
#173784=CARTESIAN_POINT('Ctrl Pts',(70.8605998877149,1.11729664352993,0.));
#173785=CARTESIAN_POINT('Ctrl Pts',(70.8812077152586,1.12409113243514,0.));
#173786=CARTESIAN_POINT('Ctrl Pts',(70.9018541463089,1.13092185496565,0.));
#173787=CARTESIAN_POINT('Ctrl Pts',(70.9225390131826,1.13778883418214,0.));
#173788=CARTESIAN_POINT('Ctrl Pts',(70.9432621490566,1.14469209291489,0.));
#173789=CARTESIAN_POINT('Ctrl Pts',(70.9640233879659,1.15163165376525,0.));
#173790=CARTESIAN_POINT('Ctrl Pts',(70.9848225647871,1.15860753911486,0.));
#173791=CARTESIAN_POINT('Ctrl Pts',(71.0056595152204,1.16561977112881,0.));
#173792=CARTESIAN_POINT('Ctrl Pts',(71.0265340757699,1.17266837175778,0.));
#173793=CARTESIAN_POINT('Ctrl Pts',(71.0474460837159,1.17975336273505,0.));
#173794=CARTESIAN_POINT('Ctrl Pts',(71.0683953771149,1.18687476558133,0.));
#173795=CARTESIAN_POINT('Ctrl Pts',(71.089381794801,1.19403260161003,0.));
#173796=CARTESIAN_POINT('Ctrl Pts',(71.1104051763839,1.20122689192837,0.));
#173797=CARTESIAN_POINT('Ctrl Pts',(71.1314653622442,1.20845765743648,0.));
#173798=CARTESIAN_POINT('Ctrl Pts',(71.1525621935267,1.21572491882263,0.));
#173799=CARTESIAN_POINT('Ctrl Pts',(71.1736955121362,1.22302869657018,0.));
#173800=CARTESIAN_POINT('Ctrl Pts',(71.194865160732,1.2303690109624,0.));
#173801=CARTESIAN_POINT('Ctrl Pts',(71.2160709827191,1.23774588208428,0.));
#173802=CARTESIAN_POINT('Ctrl Pts',(71.2373128222352,1.24515932982113,0.));
#173803=CARTESIAN_POINT('Ctrl Pts',(71.2585905241406,1.25260937385569,0.));
#173804=CARTESIAN_POINT('Ctrl Pts',(71.2799039340175,1.26009603367571,0.));
#173805=CARTESIAN_POINT('Ctrl Pts',(71.3012528981661,1.26761932857725,0.));
#173806=CARTESIAN_POINT('Ctrl Pts',(71.3226372635996,1.27517927766609,0.));
#173807=CARTESIAN_POINT('Ctrl Pts',(71.3440568780347,1.28277589985472,0.));
#173808=CARTESIAN_POINT('Ctrl Pts',(71.3655115898827,1.2904092138606,0.));
#173809=CARTESIAN_POINT('Ctrl Pts',(71.3870012482499,1.29807923821414,0.));
#173810=CARTESIAN_POINT('Ctrl Pts',(71.4085257029322,1.3057859912614,0.));
#173811=CARTESIAN_POINT('Ctrl Pts',(71.4300848044087,1.31352949116538,0.));
#173812=CARTESIAN_POINT('Ctrl Pts',(71.4516784038317,1.32130975590226,0.));
#173813=CARTESIAN_POINT('Ctrl Pts',(71.4733063530187,1.32912680326124,0.));
#173814=CARTESIAN_POINT('Ctrl Pts',(71.4949685044522,1.3369806508522,0.));
#173815=CARTESIAN_POINT('Ctrl Pts',(71.516664711275,1.34487131610781,0.));
#173816=CARTESIAN_POINT('Ctrl Pts',(71.5383948272845,1.35279881628455,0.));
#173817=CARTESIAN_POINT('Ctrl Pts',(71.5601587069217,1.36076316845817,0.));
#173818=CARTESIAN_POINT('Ctrl Pts',(71.5819562052663,1.36876438952466,0.));
#173819=CARTESIAN_POINT('Ctrl Pts',(71.6037871780385,1.3768024962078,0.));
#173820=CARTESIAN_POINT('Ctrl Pts',(71.625651481593,1.38487750506083,0.));
#173821=CARTESIAN_POINT('Ctrl Pts',(71.6475489729134,1.39298943246723,0.));
#173822=CARTESIAN_POINT('Ctrl Pts',(71.6694795096001,1.40113829463577,0.));
#173823=CARTESIAN_POINT('Ctrl Pts',(71.6914429498663,1.40932410760249,0.));
#173824=CARTESIAN_POINT('Ctrl Pts',(71.7134391525389,1.41754688723773,0.));
#173825=CARTESIAN_POINT('Ctrl Pts',(71.7354679770528,1.4258066492477,0.));
#173826=CARTESIAN_POINT('Ctrl Pts',(71.7575292834469,1.43410340917496,0.));
#173827=CARTESIAN_POINT('Ctrl Pts',(71.7796229323526,1.44243718239316,0.));
#173828=CARTESIAN_POINT('Ctrl Pts',(71.8017487849895,1.45080798410966,0.));
#173829=CARTESIAN_POINT('Ctrl Pts',(71.8239067031683,1.45921582937232,0.));
#173830=CARTESIAN_POINT('Ctrl Pts',(71.8460965492838,1.46766073307089,0.));
#173831=CARTESIAN_POINT('Ctrl Pts',(71.8683181863116,1.47614270993729,0.));
#173832=CARTESIAN_POINT('Ctrl Pts',(71.8905714777961,1.4846617745402,0.));
#173833=CARTESIAN_POINT('Ctrl Pts',(71.912856287848,1.49321794128799,0.));
#173834=CARTESIAN_POINT('Ctrl Pts',(71.9351724811443,1.50181122443535,0.));
#173835=CARTESIAN_POINT('Ctrl Pts',(71.9575199229241,1.51044163808454,0.));
#173836=CARTESIAN_POINT('Ctrl Pts',(71.979898478983,1.51910919618566,0.));
#173837=CARTESIAN_POINT('Ctrl Pts',(72.0023080156647,1.52781391253102,0.));
#173838=CARTESIAN_POINT('Ctrl Pts',(72.0247483998578,1.53655580075813,0.));
#173839=CARTESIAN_POINT('Ctrl Pts',(72.0472194989963,1.54533487435627,0.));
#173840=CARTESIAN_POINT('Ctrl Pts',(72.0697211810545,1.55415114666774,0.));
#173841=CARTESIAN_POINT('Ctrl Pts',(72.0922533145433,1.56300463088809,0.));
#173842=CARTESIAN_POINT('Ctrl Pts',(72.1148157684995,1.57189534006041,0.));
#173843=CARTESIAN_POINT('Ctrl Pts',(72.1374084124839,1.58082328707804,0.));
#173844=CARTESIAN_POINT('Ctrl Pts',(72.1600311165821,1.58978848469124,0.));
#173845=CARTESIAN_POINT('Ctrl Pts',(72.1826837514001,1.59879094550848,0.));
#173846=CARTESIAN_POINT('Ctrl Pts',(72.2053661880608,1.60783068199664,0.));
#173847=CARTESIAN_POINT('Ctrl Pts',(72.2280782981937,1.61690770647541,0.));
#173848=CARTESIAN_POINT('Ctrl Pts',(72.2508199539323,1.62602203111931,0.));
#173849=CARTESIAN_POINT('Ctrl Pts',(72.2735910279149,1.63517366796464,0.));
#173850=CARTESIAN_POINT('Ctrl Pts',(72.2963913932813,1.64436262891079,0.));
#173851=CARTESIAN_POINT('Ctrl Pts',(72.319220923669,1.65358892572063,0.));
#173852=CARTESIAN_POINT('Ctrl Pts',(72.3420794932047,1.66285257001497,0.));
#173853=CARTESIAN_POINT('Ctrl Pts',(72.3649669765004,1.67215357327366,0.));
#173854=CARTESIAN_POINT('Ctrl Pts',(72.387883248654,1.68149194684282,0.));
#173855=CARTESIAN_POINT('Ctrl Pts',(72.4108281852467,1.69086770193638,0.));
#173856=CARTESIAN_POINT('Ctrl Pts',(72.4338016623391,1.70028084963648,0.));
#173857=CARTESIAN_POINT('Ctrl Pts',(72.456803556463,1.70973140088842,0.));
#173858=CARTESIAN_POINT('Ctrl Pts',(72.479833744618,1.71921936650039,0.));
#173859=CARTESIAN_POINT('Ctrl Pts',(72.5028921042721,1.72874475715104,0.));
#173860=CARTESIAN_POINT('Ctrl Pts',(72.5259785133595,1.73830758339125,0.));
#173861=CARTESIAN_POINT('Ctrl Pts',(72.5490928502769,1.74790785564474,0.));
#173862=CARTESIAN_POINT('Ctrl Pts',(72.5722349938774,1.75754558420345,0.));
#173863=CARTESIAN_POINT('Ctrl Pts',(72.5954048234638,1.76722077922575,0.));
#173864=CARTESIAN_POINT('Ctrl Pts',(72.6186022187907,1.77693345074427,0.));
#173865=CARTESIAN_POINT('Ctrl Pts',(72.6418270600619,1.78668360866812,0.));
#173866=CARTESIAN_POINT('Ctrl Pts',(72.6650792279274,1.79647126278359,0.));
#173867=CARTESIAN_POINT('Ctrl Pts',(72.6883586034769,1.80629642275051,0.));
#173868=CARTESIAN_POINT('Ctrl Pts',(72.7116650682344,1.81615909809871,0.));
#173869=CARTESIAN_POINT('Ctrl Pts',(72.7349985041592,1.82605929823565,0.));
#173870=CARTESIAN_POINT('Ctrl Pts',(72.7583587936447,1.83599703244925,0.));
#173871=CARTESIAN_POINT('Ctrl Pts',(72.7817458195155,1.84597230990858,0.));
#173872=CARTESIAN_POINT('Ctrl Pts',(72.8051594650222,1.85598513966114,0.));
#173873=CARTESIAN_POINT('Ctrl Pts',(72.8285996138359,1.86603553062772,0.));
#173874=CARTESIAN_POINT('Ctrl Pts',(72.8520661500477,1.87612349160945,0.));
#173875=CARTESIAN_POINT('Ctrl Pts',(72.875558958168,1.88624903129189,0.));
#173876=CARTESIAN_POINT('Ctrl Pts',(72.8990779231226,1.89641215824583,0.));
#173877=CARTESIAN_POINT('Ctrl Pts',(72.9226229302478,1.90661288092587,0.));
#173878=CARTESIAN_POINT('Ctrl Pts',(72.9461938652811,1.91685120766437,0.));
#173879=CARTESIAN_POINT('Ctrl Pts',(72.9697906143636,1.92712714667661,0.));
#173880=CARTESIAN_POINT('Ctrl Pts',(72.9934130640415,1.93744070606566,0.));
#173881=CARTESIAN_POINT('Ctrl Pts',(73.0170611012661,1.94779189382303,0.));
#173882=CARTESIAN_POINT('Ctrl Pts',(73.040734613391,1.95818071782768,0.));
#173883=CARTESIAN_POINT('Ctrl Pts',(73.0644334881673,1.96860718583933,0.));
#173884=CARTESIAN_POINT('Ctrl Pts',(73.0881576137407,1.97907130550158,0.));
#173885=CARTESIAN_POINT('Ctrl Pts',(73.1119068786475,1.98957308434919,0.));
#173886=CARTESIAN_POINT('Ctrl Pts',(73.1356811718091,2.00011252980982,0.));
#173887=CARTESIAN_POINT('Ctrl Pts',(73.1594803825252,2.01068964920468,0.));
#173888=CARTESIAN_POINT('Ctrl Pts',(73.183304400462,2.02130444974362,0.));
#173889=CARTESIAN_POINT('Ctrl Pts',(73.2071531156504,2.03195693852455,0.));
#173890=CARTESIAN_POINT('Ctrl Pts',(73.2310264184976,2.04264712253929,0.));
#173891=CARTESIAN_POINT('Ctrl Pts',(73.2549241997953,2.05337500867403,0.));
#173892=CARTESIAN_POINT('Ctrl Pts',(73.2788463507246,2.06414060370835,0.));
#173893=CARTESIAN_POINT('Ctrl Pts',(73.3027927628626,2.07494391430941,0.));
#173894=CARTESIAN_POINT('Ctrl Pts',(73.3267633281807,2.08578494702744,0.));
#173895=CARTESIAN_POINT('Ctrl Pts',(73.3507579390239,2.09666370830717,0.));
#173896=CARTESIAN_POINT('Ctrl Pts',(73.3747764880893,2.1075802044939,0.));
#173897=CARTESIAN_POINT('Ctrl Pts',(73.3988188684021,2.11853444183762,0.));
#173898=CARTESIAN_POINT('Ctrl Pts',(73.4228849732925,2.12952642649368,0.));
#173899=CARTESIAN_POINT('Ctrl Pts',(73.4469746963637,2.14055616452058,0.));
#173900=CARTESIAN_POINT('Ctrl Pts',(73.4710879315382,2.15162366187907,0.));
#173901=CARTESIAN_POINT('Ctrl Pts',(73.4952245731054,2.1627289244292,0.));
#173902=CARTESIAN_POINT('Ctrl Pts',(73.5193845157708,2.17387195792306,0.));
#173903=CARTESIAN_POINT('Ctrl Pts',(73.5435676546929,2.18505276799754,0.));
#173904=CARTESIAN_POINT('Ctrl Pts',(73.5677738855452,2.19627136015679,0.));
#173905=CARTESIAN_POINT('Ctrl Pts',(73.5920031044595,2.20752773978349,0.));
#173906=CARTESIAN_POINT('Ctrl Pts',(73.6162552079038,2.21882191216519,0.));
#173907=CARTESIAN_POINT('Ctrl Pts',(73.6405300925712,2.23015388251288,0.));
#173908=CARTESIAN_POINT('Ctrl Pts',(73.6648276552767,2.24152365597698,0.));
#173909=CARTESIAN_POINT('Ctrl Pts',(73.6891477928129,2.25293123766425,0.));
#173910=CARTESIAN_POINT('Ctrl Pts',(73.7134904019389,2.26437663263667,0.));
#173911=CARTESIAN_POINT('Ctrl Pts',(73.7378553796807,2.27585984587199,0.));
#173912=CARTESIAN_POINT('Ctrl Pts',(73.762242623566,2.28738088222864,0.));
#173913=CARTESIAN_POINT('Ctrl Pts',(73.786652031885,2.29893974640435,0.));
#173914=CARTESIAN_POINT('Ctrl Pts',(73.8110835039327,2.31053644289417,0.));
#173915=CARTESIAN_POINT('Ctrl Pts',(73.8355369402706,2.32217097594198,0.));
#173916=CARTESIAN_POINT('Ctrl Pts',(73.8600122421468,2.33384334963958,0.));
#173917=CARTESIAN_POINT('Ctrl Pts',(73.8845093109274,2.34555356802121,0.));
#173918=CARTESIAN_POINT('Ctrl Pts',(73.9090280474712,2.35730163516316,0.));
#173919=CARTESIAN_POINT('Ctrl Pts',(73.9335683516404,2.36908755526004,0.));
#173920=CARTESIAN_POINT('Ctrl Pts',(73.958130121465,2.38091133274961,0.));
#173921=CARTESIAN_POINT('Ctrl Pts',(73.9827132538206,2.39277297220757,0.));
#173922=CARTESIAN_POINT('Ctrl Pts',(74.0073176459344,2.40467247811537,0.));
#173923=CARTESIAN_POINT('Ctrl Pts',(74.0319431966989,2.41660985465252,0.));
#173924=CARTESIAN_POINT('Ctrl Pts',(74.0565898079218,2.42858510549779,0.));
#173925=CARTESIAN_POINT('Ctrl Pts',(74.0812573859411,2.44059823356676,0.));
#173926=CARTESIAN_POINT('Ctrl Pts',(74.1059458420067,2.45264924094776,0.));
#173927=CARTESIAN_POINT('Ctrl Pts',(74.1271264545189,2.46301176097118,0.));
#173928=CARTESIAN_POINT('Ctrl Pts',(74.143376394138,2.47097695564992,0.));
#173929=CARTESIAN_POINT('Ctrl Pts',(74.1546864735166,2.47652804724536,0.));
#173930=CARTESIAN_POINT('Ctrl Pts',(74.1610506466205,2.47965393945472,0.));
#173931=CARTESIAN_POINT('Ctrl Pts',(74.1624659714554,2.48034921843225,0.));
#173932=CARTESIAN_POINT('Ctrl Pts',(74.1624659714553,2.48034921843222,12.));
#173933=CARTESIAN_POINT('Ctrl Pts',(74.1610506466205,2.4796539394547,12.));
#173934=CARTESIAN_POINT('Ctrl Pts',(74.1546864735166,2.47652804724534,12.));
#173935=CARTESIAN_POINT('Ctrl Pts',(74.1433763941379,2.47097695564991,12.));
#173936=CARTESIAN_POINT('Ctrl Pts',(74.1271264545189,2.46301176097117,12.));
#173937=CARTESIAN_POINT('Ctrl Pts',(74.1059458420067,2.45264924094776,12.));
#173938=CARTESIAN_POINT('Ctrl Pts',(74.0812573859411,2.44059823356676,12.));
#173939=CARTESIAN_POINT('Ctrl Pts',(74.0565898079218,2.42858510549779,12.));
#173940=CARTESIAN_POINT('Ctrl Pts',(74.0319431966989,2.41660985465252,12.));
#173941=CARTESIAN_POINT('Ctrl Pts',(74.0073176459344,2.40467247811537,12.));
#173942=CARTESIAN_POINT('Ctrl Pts',(73.9827132538206,2.39277297220757,12.));
#173943=CARTESIAN_POINT('Ctrl Pts',(73.958130121465,2.38091133274961,12.));
#173944=CARTESIAN_POINT('Ctrl Pts',(73.9335683516404,2.36908755526004,12.));
#173945=CARTESIAN_POINT('Ctrl Pts',(73.9090280474712,2.35730163516316,12.));
#173946=CARTESIAN_POINT('Ctrl Pts',(73.8845093109274,2.34555356802121,12.));
#173947=CARTESIAN_POINT('Ctrl Pts',(73.8600122421468,2.33384334963958,12.));
#173948=CARTESIAN_POINT('Ctrl Pts',(73.8355369402706,2.32217097594198,12.));
#173949=CARTESIAN_POINT('Ctrl Pts',(73.8110835039327,2.31053644289417,12.));
#173950=CARTESIAN_POINT('Ctrl Pts',(73.786652031885,2.29893974640435,12.));
#173951=CARTESIAN_POINT('Ctrl Pts',(73.762242623566,2.28738088222864,12.));
#173952=CARTESIAN_POINT('Ctrl Pts',(73.7378553796807,2.27585984587199,12.));
#173953=CARTESIAN_POINT('Ctrl Pts',(73.7134904019389,2.26437663263667,12.));
#173954=CARTESIAN_POINT('Ctrl Pts',(73.6891477928129,2.25293123766425,12.));
#173955=CARTESIAN_POINT('Ctrl Pts',(73.6648276552767,2.24152365597698,12.));
#173956=CARTESIAN_POINT('Ctrl Pts',(73.6405300925712,2.23015388251288,12.));
#173957=CARTESIAN_POINT('Ctrl Pts',(73.6162552079038,2.21882191216519,12.));
#173958=CARTESIAN_POINT('Ctrl Pts',(73.5920031044595,2.20752773978349,12.));
#173959=CARTESIAN_POINT('Ctrl Pts',(73.5677738855452,2.19627136015679,12.));
#173960=CARTESIAN_POINT('Ctrl Pts',(73.5435676546929,2.18505276799754,12.));
#173961=CARTESIAN_POINT('Ctrl Pts',(73.5193845157708,2.17387195792306,12.));
#173962=CARTESIAN_POINT('Ctrl Pts',(73.4952245731054,2.1627289244292,12.));
#173963=CARTESIAN_POINT('Ctrl Pts',(73.4710879315382,2.15162366187907,12.));
#173964=CARTESIAN_POINT('Ctrl Pts',(73.4469746963637,2.14055616452058,12.));
#173965=CARTESIAN_POINT('Ctrl Pts',(73.4228849732925,2.12952642649368,12.));
#173966=CARTESIAN_POINT('Ctrl Pts',(73.3988188684021,2.11853444183762,12.));
#173967=CARTESIAN_POINT('Ctrl Pts',(73.3747764880893,2.1075802044939,12.));
#173968=CARTESIAN_POINT('Ctrl Pts',(73.3507579390239,2.09666370830717,12.));
#173969=CARTESIAN_POINT('Ctrl Pts',(73.3267633281807,2.08578494702744,12.));
#173970=CARTESIAN_POINT('Ctrl Pts',(73.3027927628626,2.07494391430941,12.));
#173971=CARTESIAN_POINT('Ctrl Pts',(73.2788463507246,2.06414060370835,12.));
#173972=CARTESIAN_POINT('Ctrl Pts',(73.2549241997953,2.05337500867403,12.));
#173973=CARTESIAN_POINT('Ctrl Pts',(73.2310264184976,2.04264712253929,12.));
#173974=CARTESIAN_POINT('Ctrl Pts',(73.2071531156504,2.03195693852455,12.));
#173975=CARTESIAN_POINT('Ctrl Pts',(73.183304400462,2.02130444974362,12.));
#173976=CARTESIAN_POINT('Ctrl Pts',(73.1594803825252,2.01068964920468,12.));
#173977=CARTESIAN_POINT('Ctrl Pts',(73.1356811718091,2.00011252980982,12.));
#173978=CARTESIAN_POINT('Ctrl Pts',(73.1119068786475,1.98957308434919,12.));
#173979=CARTESIAN_POINT('Ctrl Pts',(73.0881576137407,1.97907130550158,12.));
#173980=CARTESIAN_POINT('Ctrl Pts',(73.0644334881673,1.96860718583933,12.));
#173981=CARTESIAN_POINT('Ctrl Pts',(73.040734613391,1.95818071782768,12.));
#173982=CARTESIAN_POINT('Ctrl Pts',(73.0170611012661,1.94779189382303,12.));
#173983=CARTESIAN_POINT('Ctrl Pts',(72.9934130640415,1.93744070606566,12.));
#173984=CARTESIAN_POINT('Ctrl Pts',(72.9697906143636,1.92712714667661,12.));
#173985=CARTESIAN_POINT('Ctrl Pts',(72.9461938652811,1.91685120766437,12.));
#173986=CARTESIAN_POINT('Ctrl Pts',(72.9226229302478,1.90661288092587,12.));
#173987=CARTESIAN_POINT('Ctrl Pts',(72.8990779231226,1.89641215824583,12.));
#173988=CARTESIAN_POINT('Ctrl Pts',(72.875558958168,1.88624903129189,12.));
#173989=CARTESIAN_POINT('Ctrl Pts',(72.8520661500477,1.87612349160945,12.));
#173990=CARTESIAN_POINT('Ctrl Pts',(72.8285996138359,1.86603553062772,12.));
#173991=CARTESIAN_POINT('Ctrl Pts',(72.8051594650222,1.85598513966114,12.));
#173992=CARTESIAN_POINT('Ctrl Pts',(72.7817458195155,1.84597230990858,12.));
#173993=CARTESIAN_POINT('Ctrl Pts',(72.7583587936447,1.83599703244925,12.));
#173994=CARTESIAN_POINT('Ctrl Pts',(72.7349985041592,1.82605929823565,12.));
#173995=CARTESIAN_POINT('Ctrl Pts',(72.7116650682344,1.81615909809871,12.));
#173996=CARTESIAN_POINT('Ctrl Pts',(72.6883586034769,1.80629642275051,12.));
#173997=CARTESIAN_POINT('Ctrl Pts',(72.6650792279274,1.79647126278359,12.));
#173998=CARTESIAN_POINT('Ctrl Pts',(72.6418270600619,1.78668360866812,12.));
#173999=CARTESIAN_POINT('Ctrl Pts',(72.6186022187907,1.77693345074427,12.));
#174000=CARTESIAN_POINT('Ctrl Pts',(72.5954048234638,1.76722077922575,12.));
#174001=CARTESIAN_POINT('Ctrl Pts',(72.5722349938774,1.75754558420345,12.));
#174002=CARTESIAN_POINT('Ctrl Pts',(72.5490928502769,1.74790785564474,12.));
#174003=CARTESIAN_POINT('Ctrl Pts',(72.5259785133595,1.73830758339125,12.));
#174004=CARTESIAN_POINT('Ctrl Pts',(72.5028921042721,1.72874475715104,12.));
#174005=CARTESIAN_POINT('Ctrl Pts',(72.479833744618,1.71921936650039,12.));
#174006=CARTESIAN_POINT('Ctrl Pts',(72.456803556463,1.70973140088842,12.));
#174007=CARTESIAN_POINT('Ctrl Pts',(72.4338016623391,1.70028084963648,12.));
#174008=CARTESIAN_POINT('Ctrl Pts',(72.4108281852467,1.69086770193638,12.));
#174009=CARTESIAN_POINT('Ctrl Pts',(72.387883248654,1.68149194684282,12.));
#174010=CARTESIAN_POINT('Ctrl Pts',(72.3649669765004,1.67215357327366,12.));
#174011=CARTESIAN_POINT('Ctrl Pts',(72.3420794932047,1.66285257001497,12.));
#174012=CARTESIAN_POINT('Ctrl Pts',(72.319220923669,1.65358892572063,12.));
#174013=CARTESIAN_POINT('Ctrl Pts',(72.2963913932813,1.64436262891079,12.));
#174014=CARTESIAN_POINT('Ctrl Pts',(72.2735910279149,1.63517366796464,12.));
#174015=CARTESIAN_POINT('Ctrl Pts',(72.2508199539323,1.62602203111931,12.));
#174016=CARTESIAN_POINT('Ctrl Pts',(72.2280782981937,1.61690770647541,12.));
#174017=CARTESIAN_POINT('Ctrl Pts',(72.2053661880608,1.60783068199664,12.));
#174018=CARTESIAN_POINT('Ctrl Pts',(72.1826837514001,1.59879094550848,12.));
#174019=CARTESIAN_POINT('Ctrl Pts',(72.1600311165821,1.58978848469124,12.));
#174020=CARTESIAN_POINT('Ctrl Pts',(72.1374084124839,1.58082328707804,12.));
#174021=CARTESIAN_POINT('Ctrl Pts',(72.1148157684995,1.57189534006041,12.));
#174022=CARTESIAN_POINT('Ctrl Pts',(72.0922533145433,1.56300463088809,12.));
#174023=CARTESIAN_POINT('Ctrl Pts',(72.0697211810545,1.55415114666774,12.));
#174024=CARTESIAN_POINT('Ctrl Pts',(72.0472194989963,1.54533487435627,12.));
#174025=CARTESIAN_POINT('Ctrl Pts',(72.0247483998578,1.53655580075813,12.));
#174026=CARTESIAN_POINT('Ctrl Pts',(72.0023080156647,1.52781391253102,12.));
#174027=CARTESIAN_POINT('Ctrl Pts',(71.979898478983,1.51910919618566,12.));
#174028=CARTESIAN_POINT('Ctrl Pts',(71.9575199229241,1.51044163808454,12.));
#174029=CARTESIAN_POINT('Ctrl Pts',(71.9351724811443,1.50181122443535,12.));
#174030=CARTESIAN_POINT('Ctrl Pts',(71.912856287848,1.49321794128799,12.));
#174031=CARTESIAN_POINT('Ctrl Pts',(71.8905714777961,1.4846617745402,12.));
#174032=CARTESIAN_POINT('Ctrl Pts',(71.8683181863116,1.47614270993729,12.));
#174033=CARTESIAN_POINT('Ctrl Pts',(71.8460965492838,1.46766073307089,12.));
#174034=CARTESIAN_POINT('Ctrl Pts',(71.8239067031683,1.45921582937232,12.));
#174035=CARTESIAN_POINT('Ctrl Pts',(71.8017487849895,1.45080798410966,12.));
#174036=CARTESIAN_POINT('Ctrl Pts',(71.7796229323526,1.44243718239316,12.));
#174037=CARTESIAN_POINT('Ctrl Pts',(71.7575292834469,1.43410340917496,12.));
#174038=CARTESIAN_POINT('Ctrl Pts',(71.7354679770528,1.4258066492477,12.));
#174039=CARTESIAN_POINT('Ctrl Pts',(71.7134391525389,1.41754688723773,12.));
#174040=CARTESIAN_POINT('Ctrl Pts',(71.6914429498663,1.40932410760249,12.));
#174041=CARTESIAN_POINT('Ctrl Pts',(71.6694795096001,1.40113829463577,12.));
#174042=CARTESIAN_POINT('Ctrl Pts',(71.6475489729134,1.39298943246723,12.));
#174043=CARTESIAN_POINT('Ctrl Pts',(71.625651481593,1.38487750506083,12.));
#174044=CARTESIAN_POINT('Ctrl Pts',(71.6037871780385,1.3768024962078,12.));
#174045=CARTESIAN_POINT('Ctrl Pts',(71.5819562052663,1.36876438952466,12.));
#174046=CARTESIAN_POINT('Ctrl Pts',(71.5601587069217,1.36076316845817,12.));
#174047=CARTESIAN_POINT('Ctrl Pts',(71.5383948272845,1.35279881628455,12.));
#174048=CARTESIAN_POINT('Ctrl Pts',(71.516664711275,1.34487131610781,12.));
#174049=CARTESIAN_POINT('Ctrl Pts',(71.4949685044522,1.3369806508522,12.));
#174050=CARTESIAN_POINT('Ctrl Pts',(71.4733063530187,1.32912680326124,12.));
#174051=CARTESIAN_POINT('Ctrl Pts',(71.4516784038317,1.32130975590226,12.));
#174052=CARTESIAN_POINT('Ctrl Pts',(71.4300848044087,1.31352949116538,12.));
#174053=CARTESIAN_POINT('Ctrl Pts',(71.4085257029322,1.3057859912614,12.));
#174054=CARTESIAN_POINT('Ctrl Pts',(71.3870012482499,1.29807923821414,12.));
#174055=CARTESIAN_POINT('Ctrl Pts',(71.3655115898827,1.2904092138606,12.));
#174056=CARTESIAN_POINT('Ctrl Pts',(71.3440568780347,1.28277589985472,12.));
#174057=CARTESIAN_POINT('Ctrl Pts',(71.3226372635996,1.27517927766609,12.));
#174058=CARTESIAN_POINT('Ctrl Pts',(71.3012528981661,1.26761932857725,12.));
#174059=CARTESIAN_POINT('Ctrl Pts',(71.2799039340175,1.26009603367571,12.));
#174060=CARTESIAN_POINT('Ctrl Pts',(71.2585905241406,1.25260937385569,12.));
#174061=CARTESIAN_POINT('Ctrl Pts',(71.2373128222352,1.24515932982113,12.));
#174062=CARTESIAN_POINT('Ctrl Pts',(71.2160709827191,1.23774588208428,12.));
#174063=CARTESIAN_POINT('Ctrl Pts',(71.194865160732,1.2303690109624,12.));
#174064=CARTESIAN_POINT('Ctrl Pts',(71.1736955121362,1.22302869657018,12.));
#174065=CARTESIAN_POINT('Ctrl Pts',(71.1525621935267,1.21572491882263,12.));
#174066=CARTESIAN_POINT('Ctrl Pts',(71.1314653622442,1.20845765743648,12.));
#174067=CARTESIAN_POINT('Ctrl Pts',(71.1104051763839,1.20122689192837,12.));
#174068=CARTESIAN_POINT('Ctrl Pts',(71.089381794801,1.19403260161003,12.));
#174069=CARTESIAN_POINT('Ctrl Pts',(71.0683953771149,1.18687476558133,12.));
#174070=CARTESIAN_POINT('Ctrl Pts',(71.0474460837159,1.17975336273505,12.));
#174071=CARTESIAN_POINT('Ctrl Pts',(71.0265340757699,1.17266837175778,12.));
#174072=CARTESIAN_POINT('Ctrl Pts',(71.0056595152204,1.16561977112881,12.));
#174073=CARTESIAN_POINT('Ctrl Pts',(70.9848225647871,1.15860753911486,12.));
#174074=CARTESIAN_POINT('Ctrl Pts',(70.9640233879659,1.15163165376525,12.));
#174075=CARTESIAN_POINT('Ctrl Pts',(70.9432621490566,1.14469209291489,12.));
#174076=CARTESIAN_POINT('Ctrl Pts',(70.9225390131826,1.13778883418214,12.));
#174077=CARTESIAN_POINT('Ctrl Pts',(70.9018541463089,1.13092185496565,12.));
#174078=CARTESIAN_POINT('Ctrl Pts',(70.8812077152586,1.12409113243514,12.));
#174079=CARTESIAN_POINT('Ctrl Pts',(70.8605998877149,1.11729664352993,12.));
#174080=CARTESIAN_POINT('Ctrl Pts',(70.8400308322037,1.1105383649664,12.));
#174081=CARTESIAN_POINT('Ctrl Pts',(70.8195007180745,1.10381627323947,12.));
#174082=CARTESIAN_POINT('Ctrl Pts',(70.799009715484,1.09713034462266,12.));
#174083=CARTESIAN_POINT('Ctrl Pts',(70.7785579953583,1.09048055516427,12.));
#174084=CARTESIAN_POINT('Ctrl Pts',(70.7581457294447,1.08386688068343,12.));
#174085=CARTESIAN_POINT('Ctrl Pts',(70.7377730903953,1.07728929676409,12.));
#174086=CARTESIAN_POINT('Ctrl Pts',(70.7174402518378,1.07074777874596,12.));
#174087=CARTESIAN_POINT('Ctrl Pts',(70.6971473884459,1.06424230171281,12.));
#174088=CARTESIAN_POINT('Ctrl Pts',(70.676894676009,1.05777284047731,12.));
#174089=CARTESIAN_POINT('Ctrl Pts',(70.6566822912991,1.05133936960072,12.));
#174090=CARTESIAN_POINT('Ctrl Pts',(70.6365104119252,1.04494186341157,12.));
#174091=CARTESIAN_POINT('Ctrl Pts',(70.6163792162073,1.03858029601904,12.));
#174092=CARTESIAN_POINT('Ctrl Pts',(70.5962888829934,1.03225464132871,12.));
#174093=CARTESIAN_POINT('Ctrl Pts',(70.5762395916377,1.02596487304049,12.));
#174094=CARTESIAN_POINT('Ctrl Pts',(70.556231522419,1.01971096460597,12.));
#174095=CARTESIAN_POINT('Ctrl Pts',(70.5362648569061,1.01349288918538,12.));
#174096=CARTESIAN_POINT('Ctrl Pts',(70.5163397782713,1.00731061960969,12.));
#174097=CARTESIAN_POINT('Ctrl Pts',(70.4964564717953,1.00116412831443,12.));
#174098=CARTESIAN_POINT('Ctrl Pts',(70.4766151245212,0.99505338737976,12.));
#174099=CARTESIAN_POINT('Ctrl Pts',(70.4568159243163,0.988978368643654,
12.));
#174100=CARTESIAN_POINT('Ctrl Pts',(70.4370590590842,0.982939043792161,
12.));
#174101=CARTESIAN_POINT('Ctrl Pts',(70.417344715957,0.976935384450047,12.));
#174102=CARTESIAN_POINT('Ctrl Pts',(70.3976730803613,0.970967362281179,
12.));
#174103=CARTESIAN_POINT('Ctrl Pts',(70.3780443377956,0.965034948786454,
12.));
#174104=CARTESIAN_POINT('Ctrl Pts',(70.3584586759536,0.959138115058838,
12.));
#174105=CARTESIAN_POINT('Ctrl Pts',(70.338916286458,0.953276831581247,12.));
#174106=CARTESIAN_POINT('Ctrl Pts',(70.3194173673674,0.947451067929609,
12.));
#174107=CARTESIAN_POINT('Ctrl Pts',(70.299962123399,0.941660792742984,12.));
#174108=CARTESIAN_POINT('Ctrl Pts',(70.2805507606872,0.935905974336485,
12.));
#174109=CARTESIAN_POINT('Ctrl Pts',(70.2611834821723,0.930186581235552,
12.));
#174110=CARTESIAN_POINT('Ctrl Pts',(70.2418604835836,0.924502582639461,
12.));
#174111=CARTESIAN_POINT('Ctrl Pts',(70.2225819470248,0.918853949157122,
12.));
#174112=CARTESIAN_POINT('Ctrl Pts',(70.2033480471676,0.913240652090985,
12.));
#174113=CARTESIAN_POINT('Ctrl Pts',(70.1841589635574,0.907662662015791,
12.));
#174114=CARTESIAN_POINT('Ctrl Pts',(70.1650148905109,0.902119947629775,
12.));
#174115=CARTESIAN_POINT('Ctrl Pts',(70.1459160490446,0.896612474371848,
12.));
#174116=CARTESIAN_POINT('Ctrl Pts',(70.1268626950175,0.891140203464248,
12.));
#174117=CARTESIAN_POINT('Ctrl Pts',(70.1078550938958,0.88570309480254,12.));
#174118=CARTESIAN_POINT('Ctrl Pts',(70.0888934967855,0.880301109660733,
12.));
#174119=CARTESIAN_POINT('Ctrl Pts',(70.0699781183935,0.874934213255844,
12.));
#174120=CARTESIAN_POINT('Ctrl Pts',(70.051109108301,0.869602377871129,12.));
#174121=CARTESIAN_POINT('Ctrl Pts',(70.0322865492925,0.86430558366155,12.));
#174122=CARTESIAN_POINT('Ctrl Pts',(70.0172656933806,0.86009617066874,12.));
#174123=CARTESIAN_POINT('Ctrl Pts',(70.0060209754087,0.85695487025921,12.));
#174124=CARTESIAN_POINT('Ctrl Pts',(69.9985337959407,0.854867673848601,
12.));
#174125=CARTESIAN_POINT('Ctrl Pts',(69.9947925310006,0.853825826608988,
12.));
#174126=CARTESIAN_POINT('Ctrl Pts',(74.0964320766207,3.99277406490871,0.));
#174127=CARTESIAN_POINT('Ctrl Pts',(74.0964320766207,3.99277406490871,4.));
#174128=CARTESIAN_POINT('Ctrl Pts',(74.0964320766208,3.9927740649087,8.));
#174129=CARTESIAN_POINT('Ctrl Pts',(74.0964320766208,3.9927740649087,12.));
#174130=CARTESIAN_POINT('Ctrl Pts',(74.1989040313893,3.9531047458223,0.));
#174131=CARTESIAN_POINT('Ctrl Pts',(74.1989040313893,3.9531047458223,4.));
#174132=CARTESIAN_POINT('Ctrl Pts',(74.1989040313893,3.95310474582228,8.));
#174133=CARTESIAN_POINT('Ctrl Pts',(74.1989040313893,3.95310474582228,12.));
#174134=CARTESIAN_POINT('Ctrl Pts',(74.3538917248566,3.82252142018533,0.));
#174135=CARTESIAN_POINT('Ctrl Pts',(74.3538917248566,3.82252142018533,4.));
#174136=CARTESIAN_POINT('Ctrl Pts',(74.3538917248566,3.82252142018531,7.99999999999999));
#174137=CARTESIAN_POINT('Ctrl Pts',(74.3538917248566,3.82252142018531,12.));
#174138=CARTESIAN_POINT('Ctrl Pts',(74.4114286752098,3.63264011802873,0.));
#174139=CARTESIAN_POINT('Ctrl Pts',(74.4114286752098,3.63264011802873,4.));
#174140=CARTESIAN_POINT('Ctrl Pts',(74.4114286752098,3.63264011802872,8.00000000000001));
#174141=CARTESIAN_POINT('Ctrl Pts',(74.4114286752098,3.63264011802872,12.));
#174142=CARTESIAN_POINT('Ctrl Pts',(74.4153560388998,3.55032190142809,0.));
#174143=CARTESIAN_POINT('Ctrl Pts',(74.4153560388998,3.55032190142809,4.));
#174144=CARTESIAN_POINT('Ctrl Pts',(74.4153560388998,3.55032190142808,8.));
#174145=CARTESIAN_POINT('Ctrl Pts',(74.4153560388998,3.55032190142808,12.));
#174146=CARTESIAN_POINT('',(74.0964320766207,3.99277406490871,0.));
#174147=CARTESIAN_POINT('',(74.4153560388999,3.5503219014281,0.));
#174148=CARTESIAN_POINT('Ctrl Pts',(74.0964320766207,3.99277406490871,0.));
#174149=CARTESIAN_POINT('Ctrl Pts',(74.1989040313893,3.9531047458223,0.));
#174150=CARTESIAN_POINT('Ctrl Pts',(74.2874684276563,3.87848570260117,0.));
#174151=CARTESIAN_POINT('Ctrl Pts',(74.3442121731106,3.78450405480221,0.));
#174152=CARTESIAN_POINT('Ctrl Pts',(74.3867699822013,3.71401781895299,0.));
#174153=CARTESIAN_POINT('Ctrl Pts',(74.4114286752098,3.63264011802873,0.));
#174154=CARTESIAN_POINT('Ctrl Pts',(74.4153560388998,3.55032190142809,0.));
#174155=CARTESIAN_POINT('',(74.4153560388999,3.55032190142809,12.));
#174156=CARTESIAN_POINT('Ctrl Pts',(74.4153560388998,3.55032190142809,0.));
#174157=CARTESIAN_POINT('Ctrl Pts',(74.4153560388998,3.55032190142809,4.));
#174158=CARTESIAN_POINT('Ctrl Pts',(74.4153560388998,3.55032190142808,8.));
#174159=CARTESIAN_POINT('Ctrl Pts',(74.4153560388998,3.55032190142808,12.));
#174160=CARTESIAN_POINT('',(74.0964320766208,3.99277406490869,12.));
#174161=CARTESIAN_POINT('Ctrl Pts',(74.4153560388998,3.55032190142808,12.));
#174162=CARTESIAN_POINT('Ctrl Pts',(74.4114286752098,3.63264011802872,12.));
#174163=CARTESIAN_POINT('Ctrl Pts',(74.3867699822013,3.71401781895297,12.));
#174164=CARTESIAN_POINT('Ctrl Pts',(74.3442121731106,3.78450405480219,12.));
#174165=CARTESIAN_POINT('Ctrl Pts',(74.2874684276563,3.87848570260115,12.));
#174166=CARTESIAN_POINT('Ctrl Pts',(74.1989040313893,3.95310474582228,12.));
#174167=CARTESIAN_POINT('Ctrl Pts',(74.0964320766208,3.9927740649087,12.));
#174168=CARTESIAN_POINT('Ctrl Pts',(74.0964320766208,3.9927740649087,12.));
#174169=CARTESIAN_POINT('Ctrl Pts',(74.0964320766208,3.9927740649087,8.));
#174170=CARTESIAN_POINT('Ctrl Pts',(74.0964320766207,3.99277406490871,4.));
#174171=CARTESIAN_POINT('Ctrl Pts',(74.0964320766207,3.99277406490871,0.));
#174172=CARTESIAN_POINT('Origin',(3.74482667098164E-10,1.64496194443586E-11,
0.));
#174173=CARTESIAN_POINT('Origin',(3.74482667098164E-10,1.64496194443586E-11,
12.));
#174174=CARTESIAN_POINT('Origin',(3.74482667098164E-10,1.64496194443586E-11,
0.));
#174175=CARTESIAN_POINT('Ctrl Pts',(74.3992230078037,3.87370827955544,0.));
#174176=CARTESIAN_POINT('Ctrl Pts',(74.3992230078037,3.87370827955544,12.));
#174177=CARTESIAN_POINT('Ctrl Pts',(74.3940262116388,3.87578335377326,0.));
#174178=CARTESIAN_POINT('Ctrl Pts',(74.3940262116388,3.87578335377326,12.));
#174179=CARTESIAN_POINT('Ctrl Pts',(74.3836349189184,3.87992989995748,0.));
#174180=CARTESIAN_POINT('Ctrl Pts',(74.3836349189184,3.87992989995748,12.));
#174181=CARTESIAN_POINT('Ctrl Pts',(74.3680548786661,3.88613891247984,0.));
#174182=CARTESIAN_POINT('Ctrl Pts',(74.3680548786661,3.88613891247984,12.));
#174183=CARTESIAN_POINT('Ctrl Pts',(74.3472952898745,3.89439598145329,0.));
#174184=CARTESIAN_POINT('Ctrl Pts',(74.3472952898745,3.89439598145329,12.));
#174185=CARTESIAN_POINT('Ctrl Pts',(74.3213688090133,3.90468128904635,0.));
#174186=CARTESIAN_POINT('Ctrl Pts',(74.3213688090133,3.90468128904635,12.));
#174187=CARTESIAN_POINT('Ctrl Pts',(74.2954653518728,3.91493056285031,0.));
#174188=CARTESIAN_POINT('Ctrl Pts',(74.2954653518728,3.91493056285031,12.));
#174189=CARTESIAN_POINT('Ctrl Pts',(74.2695849516226,3.92514379920744,0.));
#174190=CARTESIAN_POINT('Ctrl Pts',(74.2695849516226,3.92514379920744,12.));
#174191=CARTESIAN_POINT('Ctrl Pts',(74.2437276593623,3.93532099774204,0.));
#174192=CARTESIAN_POINT('Ctrl Pts',(74.2437276593623,3.93532099774204,12.));
#174193=CARTESIAN_POINT('Ctrl Pts',(74.2178935492876,3.94546216377452,0.));
#174194=CARTESIAN_POINT('Ctrl Pts',(74.2178935492876,3.94546216377452,12.));
#174195=CARTESIAN_POINT('Ctrl Pts',(74.1920827166585,3.95556730821111,0.));
#174196=CARTESIAN_POINT('Ctrl Pts',(74.1920827166585,3.95556730821111,12.));
#174197=CARTESIAN_POINT('Ctrl Pts',(74.1662952702485,3.96563644549386,0.));
#174198=CARTESIAN_POINT('Ctrl Pts',(74.1662952702485,3.96563644549386,12.));
#174199=CARTESIAN_POINT('Ctrl Pts',(74.1405313263109,3.97566959209529,0.));
#174200=CARTESIAN_POINT('Ctrl Pts',(74.1405313263109,3.97566959209529,12.));
#174201=CARTESIAN_POINT('Ctrl Pts',(74.1147910020891,3.98566676483642,0.));
#174202=CARTESIAN_POINT('Ctrl Pts',(74.1147910020891,3.98566676483642,12.));
#174203=CARTESIAN_POINT('Ctrl Pts',(74.0890744091186,3.99562797918288,0.));
#174204=CARTESIAN_POINT('Ctrl Pts',(74.0890744091186,3.99562797918288,12.));
#174205=CARTESIAN_POINT('Ctrl Pts',(74.0633816478037,4.00555324785481,0.));
#174206=CARTESIAN_POINT('Ctrl Pts',(74.0633816478037,4.00555324785481,12.));
#174207=CARTESIAN_POINT('Ctrl Pts',(74.0377128111863,4.01544258176711,0.));
#174208=CARTESIAN_POINT('Ctrl Pts',(74.0377128111863,4.01544258176711,12.));
#174209=CARTESIAN_POINT('Ctrl Pts',(74.012067987646,4.02529599070095,0.));
#174210=CARTESIAN_POINT('Ctrl Pts',(74.012067987646,4.02529599070095,12.));
#174211=CARTESIAN_POINT('Ctrl Pts',(73.9864472641033,4.0351134841066,0.));
#174212=CARTESIAN_POINT('Ctrl Pts',(73.9864472641033,4.0351134841066,12.));
#174213=CARTESIAN_POINT('Ctrl Pts',(73.9608507287909,4.04489507179958,0.));
#174214=CARTESIAN_POINT('Ctrl Pts',(73.9608507287909,4.04489507179958,12.));
#174215=CARTESIAN_POINT('Ctrl Pts',(73.9352784747608,4.05464076484752,0.));
#174216=CARTESIAN_POINT('Ctrl Pts',(73.9352784747608,4.05464076484752,12.));
#174217=CARTESIAN_POINT('Ctrl Pts',(73.9097305995115,4.06435057547325,0.));
#174218=CARTESIAN_POINT('Ctrl Pts',(73.9097305995115,4.06435057547325,12.));
#174219=CARTESIAN_POINT('Ctrl Pts',(73.8842072034008,4.07402451665245,0.));
#174220=CARTESIAN_POINT('Ctrl Pts',(73.8842072034008,4.07402451665245,12.));
#174221=CARTESIAN_POINT('Ctrl Pts',(73.8587083884191,4.08366260180675,0.));
#174222=CARTESIAN_POINT('Ctrl Pts',(73.8587083884191,4.08366260180675,12.));
#174223=CARTESIAN_POINT('Ctrl Pts',(73.8332342568989,4.09326484448233,0.));
#174224=CARTESIAN_POINT('Ctrl Pts',(73.8332342568989,4.09326484448233,12.));
#174225=CARTESIAN_POINT('Ctrl Pts',(73.8077849100342,4.1028312579873,0.));
#174226=CARTESIAN_POINT('Ctrl Pts',(73.8077849100342,4.1028312579873,12.));
#174227=CARTESIAN_POINT('Ctrl Pts',(73.7823604472159,4.11236185522788,0.));
#174228=CARTESIAN_POINT('Ctrl Pts',(73.7823604472159,4.11236185522788,12.));
#174229=CARTESIAN_POINT('Ctrl Pts',(73.7569609668528,4.12185664890557,0.));
#174230=CARTESIAN_POINT('Ctrl Pts',(73.7569609668528,4.12185664890557,12.));
#174231=CARTESIAN_POINT('Ctrl Pts',(73.7315865668522,4.13131565163579,0.));
#174232=CARTESIAN_POINT('Ctrl Pts',(73.7315865668522,4.13131565163579,12.));
#174233=CARTESIAN_POINT('Ctrl Pts',(73.7062373452342,4.14073887610154,0.));
#174234=CARTESIAN_POINT('Ctrl Pts',(73.7062373452342,4.14073887610154,12.));
#174235=CARTESIAN_POINT('Ctrl Pts',(73.6809134006897,4.15012633519724,0.));
#174236=CARTESIAN_POINT('Ctrl Pts',(73.6809134006897,4.15012633519724,12.));
#174237=CARTESIAN_POINT('Ctrl Pts',(73.6556148331489,4.15947804217784,0.));
#174238=CARTESIAN_POINT('Ctrl Pts',(73.6556148331489,4.15947804217784,12.));
#174239=CARTESIAN_POINT('Ctrl Pts',(73.6303417435251,4.16879401058781,0.));
#174240=CARTESIAN_POINT('Ctrl Pts',(73.6303417435251,4.16879401058781,12.));
#174241=CARTESIAN_POINT('Ctrl Pts',(73.6050942334768,4.17807425419813,0.));
#174242=CARTESIAN_POINT('Ctrl Pts',(73.6050942334768,4.17807425419813,12.));
#174243=CARTESIAN_POINT('Ctrl Pts',(73.5798724051519,4.18731878694237,0.));
#174244=CARTESIAN_POINT('Ctrl Pts',(73.5798724051519,4.18731878694237,12.));
#174245=CARTESIAN_POINT('Ctrl Pts',(73.5546763609572,4.19652762286128,0.));
#174246=CARTESIAN_POINT('Ctrl Pts',(73.5546763609572,4.19652762286128,12.));
#174247=CARTESIAN_POINT('Ctrl Pts',(73.5295062032628,4.2057007760373,0.));
#174248=CARTESIAN_POINT('Ctrl Pts',(73.5295062032628,4.2057007760373,12.));
#174249=CARTESIAN_POINT('Ctrl Pts',(73.5043620344116,4.21483826059441,0.));
#174250=CARTESIAN_POINT('Ctrl Pts',(73.5043620344116,4.21483826059441,12.));
#174251=CARTESIAN_POINT('Ctrl Pts',(73.4792439568633,4.22394009072757,0.));
#174252=CARTESIAN_POINT('Ctrl Pts',(73.4792439568633,4.22394009072757,12.));
#174253=CARTESIAN_POINT('Ctrl Pts',(73.4541520732948,4.23300628072759,0.));
#174254=CARTESIAN_POINT('Ctrl Pts',(73.4541520732948,4.23300628072759,12.));
#174255=CARTESIAN_POINT('Ctrl Pts',(73.4290864867101,4.24203684500939,0.));
#174256=CARTESIAN_POINT('Ctrl Pts',(73.4290864867101,4.24203684500939,12.));
#174257=CARTESIAN_POINT('Ctrl Pts',(73.4040473005592,4.25103179814887,0.));
#174258=CARTESIAN_POINT('Ctrl Pts',(73.4040473005592,4.25103179814887,12.));
#174259=CARTESIAN_POINT('Ctrl Pts',(73.3790346187938,4.259991154899,0.));
#174260=CARTESIAN_POINT('Ctrl Pts',(73.3790346187938,4.259991154899,12.));
#174261=CARTESIAN_POINT('Ctrl Pts',(73.3540485458065,4.268914930167,0.));
#174262=CARTESIAN_POINT('Ctrl Pts',(73.3540485458065,4.268914930167,12.));
#174263=CARTESIAN_POINT('Ctrl Pts',(73.3290891863949,4.2778031390039,0.));
#174264=CARTESIAN_POINT('Ctrl Pts',(73.3290891863949,4.2778031390039,12.));
#174265=CARTESIAN_POINT('Ctrl Pts',(73.3041566457135,4.28665579659302,0.));
#174266=CARTESIAN_POINT('Ctrl Pts',(73.3041566457135,4.28665579659302,12.));
#174267=CARTESIAN_POINT('Ctrl Pts',(73.2792510292253,4.29547291824287,0.));
#174268=CARTESIAN_POINT('Ctrl Pts',(73.2792510292253,4.29547291824287,12.));
#174269=CARTESIAN_POINT('Ctrl Pts',(73.2543724426577,4.30425451938231,0.));
#174270=CARTESIAN_POINT('Ctrl Pts',(73.2543724426577,4.30425451938231,12.));
#174271=CARTESIAN_POINT('Ctrl Pts',(73.2295209920334,4.31300061556098,0.));
#174272=CARTESIAN_POINT('Ctrl Pts',(73.2295209920334,4.31300061556098,12.));
#174273=CARTESIAN_POINT('Ctrl Pts',(73.204696783694,4.32171122245214,0.));
#174274=CARTESIAN_POINT('Ctrl Pts',(73.204696783694,4.32171122245214,12.));
#174275=CARTESIAN_POINT('Ctrl Pts',(73.1798999243235,4.33038635585877,0.));
#174276=CARTESIAN_POINT('Ctrl Pts',(73.1798999243235,4.33038635585877,12.));
#174277=CARTESIAN_POINT('Ctrl Pts',(73.1551305209685,4.33902603172141,0.));
#174278=CARTESIAN_POINT('Ctrl Pts',(73.1551305209685,4.33902603172141,12.));
#174279=CARTESIAN_POINT('Ctrl Pts',(73.130388681059,4.34763026613158,0.));
#174280=CARTESIAN_POINT('Ctrl Pts',(73.130388681059,4.34763026613158,12.));
#174281=CARTESIAN_POINT('Ctrl Pts',(73.1056745124087,4.3561990753272,0.));
#174282=CARTESIAN_POINT('Ctrl Pts',(73.1056745124087,4.3561990753272,12.));
#174283=CARTESIAN_POINT('Ctrl Pts',(73.0809881232103,4.36473247568642,0.));
#174284=CARTESIAN_POINT('Ctrl Pts',(73.0809881232103,4.36473247568642,12.));
#174285=CARTESIAN_POINT('Ctrl Pts',(73.0563296220299,4.37323048372608,0.));
#174286=CARTESIAN_POINT('Ctrl Pts',(73.0563296220299,4.37323048372608,12.));
#174287=CARTESIAN_POINT('Ctrl Pts',(73.0316991177993,4.38169311610151,0.));
#174288=CARTESIAN_POINT('Ctrl Pts',(73.0316991177993,4.38169311610151,12.));
#174289=CARTESIAN_POINT('Ctrl Pts',(73.007096719804,4.3901203896114,0.));
#174290=CARTESIAN_POINT('Ctrl Pts',(73.007096719804,4.3901203896114,12.));
#174291=CARTESIAN_POINT('Ctrl Pts',(72.9825225376846,4.39851232119723,0.));
#174292=CARTESIAN_POINT('Ctrl Pts',(72.9825225376846,4.39851232119723,12.));
#174293=CARTESIAN_POINT('Ctrl Pts',(72.95797668145,4.40686892793958,0.));
#174294=CARTESIAN_POINT('Ctrl Pts',(72.95797668145,4.40686892793958,12.));
#174295=CARTESIAN_POINT('Ctrl Pts',(72.9334592614829,4.41519022705922,0.));
#174296=CARTESIAN_POINT('Ctrl Pts',(72.9334592614829,4.41519022705922,12.));
#174297=CARTESIAN_POINT('Ctrl Pts',(72.9089703885462,4.42347623591942,0.));
#174298=CARTESIAN_POINT('Ctrl Pts',(72.9089703885462,4.42347623591942,12.));
#174299=CARTESIAN_POINT('Ctrl Pts',(72.8845101737855,4.4317269720335,0.));
#174300=CARTESIAN_POINT('Ctrl Pts',(72.8845101737855,4.4317269720335,12.));
#174301=CARTESIAN_POINT('Ctrl Pts',(72.8600787287318,4.43994245306819,0.));
#174302=CARTESIAN_POINT('Ctrl Pts',(72.8600787287318,4.43994245306819,12.));
#174303=CARTESIAN_POINT('Ctrl Pts',(72.8356761653069,4.44812269683738,0.));
#174304=CARTESIAN_POINT('Ctrl Pts',(72.8356761653069,4.44812269683738,12.));
#174305=CARTESIAN_POINT('Ctrl Pts',(72.8113025958262,4.45626772130147,0.));
#174306=CARTESIAN_POINT('Ctrl Pts',(72.8113025958262,4.45626772130147,12.));
#174307=CARTESIAN_POINT('Ctrl Pts',(72.7869581329994,4.46437754456793,0.));
#174308=CARTESIAN_POINT('Ctrl Pts',(72.7869581329994,4.46437754456793,12.));
#174309=CARTESIAN_POINT('Ctrl Pts',(72.7626428899281,4.4724521848961,0.));
#174310=CARTESIAN_POINT('Ctrl Pts',(72.7626428899281,4.4724521848961,12.));
#174311=CARTESIAN_POINT('Ctrl Pts',(72.738356980103,4.48049166070206,0.));
#174312=CARTESIAN_POINT('Ctrl Pts',(72.738356980103,4.48049166070206,12.));
#174313=CARTESIAN_POINT('Ctrl Pts',(72.714100517414,4.48849599055338,0.));
#174314=CARTESIAN_POINT('Ctrl Pts',(72.714100517414,4.48849599055338,12.));
#174315=CARTESIAN_POINT('Ctrl Pts',(72.6898736161542,4.49646519316813,0.));
#174316=CARTESIAN_POINT('Ctrl Pts',(72.6898736161542,4.49646519316813,12.));
#174317=CARTESIAN_POINT('Ctrl Pts',(72.6656763910241,4.50439928741604,0.));
#174318=CARTESIAN_POINT('Ctrl Pts',(72.6656763910241,4.50439928741604,12.));
#174319=CARTESIAN_POINT('Ctrl Pts',(72.6415089571321,4.51229829232264,0.));
#174320=CARTESIAN_POINT('Ctrl Pts',(72.6415089571321,4.51229829232264,12.));
#174321=CARTESIAN_POINT('Ctrl Pts',(72.6173714299942,4.52016222707638,0.));
#174322=CARTESIAN_POINT('Ctrl Pts',(72.6173714299942,4.52016222707638,12.));
#174323=CARTESIAN_POINT('Ctrl Pts',(72.5932639255409,4.52799111102392,0.));
#174324=CARTESIAN_POINT('Ctrl Pts',(72.5932639255409,4.52799111102392,12.));
#174325=CARTESIAN_POINT('Ctrl Pts',(72.5691865601223,4.535784963668,0.));
#174326=CARTESIAN_POINT('Ctrl Pts',(72.5691865601223,4.535784963668,12.));
#174327=CARTESIAN_POINT('Ctrl Pts',(72.5451394505103,4.54354380466823,0.));
#174328=CARTESIAN_POINT('Ctrl Pts',(72.5451394505103,4.54354380466823,12.));
#174329=CARTESIAN_POINT('Ctrl Pts',(72.5211227139001,4.55126765384405,0.));
#174330=CARTESIAN_POINT('Ctrl Pts',(72.5211227139001,4.55126765384405,12.));
#174331=CARTESIAN_POINT('Ctrl Pts',(72.4971364679068,4.55895653118221,0.));
#174332=CARTESIAN_POINT('Ctrl Pts',(72.4971364679068,4.55895653118221,12.));
#174333=CARTESIAN_POINT('Ctrl Pts',(72.4731808305728,4.56661045683376,0.));
#174334=CARTESIAN_POINT('Ctrl Pts',(72.4731808305728,4.56661045683376,12.));
#174335=CARTESIAN_POINT('Ctrl Pts',(72.4492559203745,4.57422945111103,0.));
#174336=CARTESIAN_POINT('Ctrl Pts',(72.4492559203745,4.57422945111103,12.));
#174337=CARTESIAN_POINT('Ctrl Pts',(72.4253618562252,4.58181353448852,0.));
#174338=CARTESIAN_POINT('Ctrl Pts',(72.4253618562252,4.58181353448852,12.));
#174339=CARTESIAN_POINT('Ctrl Pts',(72.401498757478,4.58936272760545,0.));
#174340=CARTESIAN_POINT('Ctrl Pts',(72.401498757478,4.58936272760545,12.));
#174341=CARTESIAN_POINT('Ctrl Pts',(72.3776667439227,4.5968770512733,0.));
#174342=CARTESIAN_POINT('Ctrl Pts',(72.3776667439227,4.5968770512733,12.));
#174343=CARTESIAN_POINT('Ctrl Pts',(72.3538659357913,4.60435652647454,0.));
#174344=CARTESIAN_POINT('Ctrl Pts',(72.3538659357913,4.60435652647454,12.));
#174345=CARTESIAN_POINT('Ctrl Pts',(72.3300964537658,4.61180117435863,0.));
#174346=CARTESIAN_POINT('Ctrl Pts',(72.3300964537658,4.61180117435863,12.));
#174347=CARTESIAN_POINT('Ctrl Pts',(72.3063584189807,4.61921101624292,0.));
#174348=CARTESIAN_POINT('Ctrl Pts',(72.3063584189807,4.61921101624292,12.));
#174349=CARTESIAN_POINT('Ctrl Pts',(72.2826519530259,4.62658607361466,0.));
#174350=CARTESIAN_POINT('Ctrl Pts',(72.2826519530259,4.62658607361466,12.));
#174351=CARTESIAN_POINT('Ctrl Pts',(72.2589771779456,4.63392636813844,0.));
#174352=CARTESIAN_POINT('Ctrl Pts',(72.2589771779456,4.63392636813844,12.));
#174353=CARTESIAN_POINT('Ctrl Pts',(72.2353342162417,4.64123192165628,0.));
#174354=CARTESIAN_POINT('Ctrl Pts',(72.2353342162417,4.64123192165628,12.));
#174355=CARTESIAN_POINT('Ctrl Pts',(72.2117231908822,4.64850275618324,0.));
#174356=CARTESIAN_POINT('Ctrl Pts',(72.2117231908822,4.64850275618324,12.));
#174357=CARTESIAN_POINT('Ctrl Pts',(72.1881442253053,4.65573889390823,0.));
#174358=CARTESIAN_POINT('Ctrl Pts',(72.1881442253053,4.65573889390823,12.));
#174359=CARTESIAN_POINT('Ctrl Pts',(72.1645974434216,4.6629403571957,0.));
#174360=CARTESIAN_POINT('Ctrl Pts',(72.1645974434216,4.6629403571957,12.));
#174361=CARTESIAN_POINT('Ctrl Pts',(72.1410829696128,4.67010716859286,0.));
#174362=CARTESIAN_POINT('Ctrl Pts',(72.1410829696128,4.67010716859286,12.));
#174363=CARTESIAN_POINT('Ctrl Pts',(72.1176009287351,4.67723935083095,0.));
#174364=CARTESIAN_POINT('Ctrl Pts',(72.1176009287351,4.67723935083095,12.));
#174365=CARTESIAN_POINT('Ctrl Pts',(72.0941514461287,4.68433692682069,0.));
#174366=CARTESIAN_POINT('Ctrl Pts',(72.0941514461287,4.68433692682069,12.));
#174367=CARTESIAN_POINT('Ctrl Pts',(72.0707346476213,4.69139991965284,0.));
#174368=CARTESIAN_POINT('Ctrl Pts',(72.0707346476213,4.69139991965284,12.));
#174369=CARTESIAN_POINT('Ctrl Pts',(72.0473506595318,4.69842835259993,0.));
#174370=CARTESIAN_POINT('Ctrl Pts',(72.0473506595318,4.69842835259993,12.));
#174371=CARTESIAN_POINT('Ctrl Pts',(72.0239996086686,4.70542224912301,0.));
#174372=CARTESIAN_POINT('Ctrl Pts',(72.0239996086686,4.70542224912301,12.));
#174373=CARTESIAN_POINT('Ctrl Pts',(72.0006816223325,4.71238163287397,0.));
#174374=CARTESIAN_POINT('Ctrl Pts',(72.0006816223325,4.71238163287397,12.));
#174375=CARTESIAN_POINT('Ctrl Pts',(71.9773968283259,4.71930652769071,0.));
#174376=CARTESIAN_POINT('Ctrl Pts',(71.9773968283259,4.71930652769071,12.));
#174377=CARTESIAN_POINT('Ctrl Pts',(71.9541453549579,4.72619695759774,0.));
#174378=CARTESIAN_POINT('Ctrl Pts',(71.9541453549579,4.72619695759774,12.));
#174379=CARTESIAN_POINT('Ctrl Pts',(71.9309273310471,4.73305294680786,0.));
#174380=CARTESIAN_POINT('Ctrl Pts',(71.9309273310471,4.73305294680786,12.));
#174381=CARTESIAN_POINT('Ctrl Pts',(71.9077428859212,4.73987451972864,0.));
#174382=CARTESIAN_POINT('Ctrl Pts',(71.9077428859212,4.73987451972864,12.));
#174383=CARTESIAN_POINT('Ctrl Pts',(71.8845921494189,4.74666170096548,0.));
#174384=CARTESIAN_POINT('Ctrl Pts',(71.8845921494189,4.74666170096548,12.));
#174385=CARTESIAN_POINT('Ctrl Pts',(71.8614752519008,4.7534145153167,0.));
#174386=CARTESIAN_POINT('Ctrl Pts',(71.8614752519008,4.7534145153167,12.));
#174387=CARTESIAN_POINT('Ctrl Pts',(71.8383923242531,4.7601329877742,0.));
#174388=CARTESIAN_POINT('Ctrl Pts',(71.8383923242531,4.7601329877742,12.));
#174389=CARTESIAN_POINT('Ctrl Pts',(71.8153434978923,4.76681714352503,0.));
#174390=CARTESIAN_POINT('Ctrl Pts',(71.8153434978923,4.76681714352503,12.));
#174391=CARTESIAN_POINT('Ctrl Pts',(71.7923289047643,4.77346700795792,0.));
#174392=CARTESIAN_POINT('Ctrl Pts',(71.7923289047643,4.77346700795792,12.));
#174393=CARTESIAN_POINT('Ctrl Pts',(71.769348677346,4.78008260666651,0.));
#174394=CARTESIAN_POINT('Ctrl Pts',(71.769348677346,4.78008260666651,12.));
#174395=CARTESIAN_POINT('Ctrl Pts',(71.7464029486563,4.78666396544459,0.));
#174396=CARTESIAN_POINT('Ctrl Pts',(71.7464029486563,4.78666396544459,12.));
#174397=CARTESIAN_POINT('Ctrl Pts',(71.723491852261,4.79321111028676,0.));
#174398=CARTESIAN_POINT('Ctrl Pts',(71.723491852261,4.79321111028676,12.));
#174399=CARTESIAN_POINT('Ctrl Pts',(71.7006155222764,4.79972406739011,0.));
#174400=CARTESIAN_POINT('Ctrl Pts',(71.7006155222764,4.79972406739011,12.));
#174401=CARTESIAN_POINT('Ctrl Pts',(71.6777740933687,4.80620286316076,0.));
#174402=CARTESIAN_POINT('Ctrl Pts',(71.6777740933687,4.80620286316076,12.));
#174403=CARTESIAN_POINT('Ctrl Pts',(71.6549677007582,4.81264752421714,0.));
#174404=CARTESIAN_POINT('Ctrl Pts',(71.6549677007582,4.81264752421714,12.));
#174405=CARTESIAN_POINT('Ctrl Pts',(71.6321964802297,4.81905807738542,0.));
#174406=CARTESIAN_POINT('Ctrl Pts',(71.6321964802297,4.81905807738542,12.));
#174407=CARTESIAN_POINT('Ctrl Pts',(71.6094605681353,4.82543454970021,0.));
#174408=CARTESIAN_POINT('Ctrl Pts',(71.6094605681353,4.82543454970021,12.));
#174409=CARTESIAN_POINT('Ctrl Pts',(71.5867601014008,4.83177696840641,0.));
#174410=CARTESIAN_POINT('Ctrl Pts',(71.5867601014008,4.83177696840641,12.));
#174411=CARTESIAN_POINT('Ctrl Pts',(71.5640952175239,4.8380853609659,0.));
#174412=CARTESIAN_POINT('Ctrl Pts',(71.5640952175239,4.8380853609659,12.));
#174413=CARTESIAN_POINT('Ctrl Pts',(71.5414660545778,4.84435975506057,0.));
#174414=CARTESIAN_POINT('Ctrl Pts',(71.5414660545778,4.84435975506057,12.));
#174415=CARTESIAN_POINT('Ctrl Pts',(71.5188727512231,4.85060017858787,0.));
#174416=CARTESIAN_POINT('Ctrl Pts',(71.5188727512231,4.85060017858787,12.));
#174417=CARTESIAN_POINT('Ctrl Pts',(71.4963154467128,4.85680665966185,0.));
#174418=CARTESIAN_POINT('Ctrl Pts',(71.4963154467128,4.85680665966185,12.));
#174419=CARTESIAN_POINT('Ctrl Pts',(71.4737942808971,4.86297922661499,0.));
#174420=CARTESIAN_POINT('Ctrl Pts',(71.4737942808971,4.86297922661499,12.));
#174421=CARTESIAN_POINT('Ctrl Pts',(71.4513093942216,4.86911790800534,0.));
#174422=CARTESIAN_POINT('Ctrl Pts',(71.4513093942216,4.86911790800534,12.));
#174423=CARTESIAN_POINT('Ctrl Pts',(71.4288609277324,4.87522273261881,0.));
#174424=CARTESIAN_POINT('Ctrl Pts',(71.4288609277324,4.87522273261881,12.));
#174425=CARTESIAN_POINT('Ctrl Pts',(71.4064490230857,4.88129372946525,0.));
#174426=CARTESIAN_POINT('Ctrl Pts',(71.4064490230857,4.88129372946525,12.));
#174427=CARTESIAN_POINT('Ctrl Pts',(71.3840738225547,4.88733092777965,0.));
#174428=CARTESIAN_POINT('Ctrl Pts',(71.3840738225547,4.88733092777965,12.));
#174429=CARTESIAN_POINT('Ctrl Pts',(71.3617354690342,4.89333435702424,0.));
#174430=CARTESIAN_POINT('Ctrl Pts',(71.3617354690342,4.89333435702424,12.));
#174431=CARTESIAN_POINT('Ctrl Pts',(71.3394341060396,4.899304046896,0.));
#174432=CARTESIAN_POINT('Ctrl Pts',(71.3394341060396,4.899304046896,12.));
#174433=CARTESIAN_POINT('Ctrl Pts',(71.3171698777124,4.90524002732806,0.));
#174434=CARTESIAN_POINT('Ctrl Pts',(71.3171698777124,4.90524002732806,12.));
#174435=CARTESIAN_POINT('Ctrl Pts',(71.2949429288319,4.91114232848623,0.));
#174436=CARTESIAN_POINT('Ctrl Pts',(71.2949429288319,4.91114232848623,12.));
#174437=CARTESIAN_POINT('Ctrl Pts',(71.27275340482,4.91701098077042,0.));
#174438=CARTESIAN_POINT('Ctrl Pts',(71.27275340482,4.91701098077042,12.));
#174439=CARTESIAN_POINT('Ctrl Pts',(71.2506014517457,4.92284601481711,0.));
#174440=CARTESIAN_POINT('Ctrl Pts',(71.2506014517457,4.92284601481711,12.));
#174441=CARTESIAN_POINT('Ctrl Pts',(71.2284872163248,4.92864746150711,0.));
#174442=CARTESIAN_POINT('Ctrl Pts',(71.2284872163248,4.92864746150711,12.));
#174443=CARTESIAN_POINT('Ctrl Pts',(71.206410845926,4.93441535196594,0.));
#174444=CARTESIAN_POINT('Ctrl Pts',(71.206410845926,4.93441535196594,12.));
#174445=CARTESIAN_POINT('Ctrl Pts',(71.184372488583,4.94014971756097,0.));
#174446=CARTESIAN_POINT('Ctrl Pts',(71.184372488583,4.94014971756097,12.));
#174447=CARTESIAN_POINT('Ctrl Pts',(71.1623722929998,4.94585058990337,0.));
#174448=CARTESIAN_POINT('Ctrl Pts',(71.1623722929998,4.94585058990337,12.));
#174449=CARTESIAN_POINT('Ctrl Pts',(71.1404104085561,4.95151800085111,0.));
#174450=CARTESIAN_POINT('Ctrl Pts',(71.1404104085561,4.95151800085111,12.));
#174451=CARTESIAN_POINT('Ctrl Pts',(71.1184869853071,4.95715198251704,0.));
#174452=CARTESIAN_POINT('Ctrl Pts',(71.1184869853071,4.95715198251704,12.));
#174453=CARTESIAN_POINT('Ctrl Pts',(71.0966021739922,4.96275256726787,0.));
#174454=CARTESIAN_POINT('Ctrl Pts',(71.0966021739922,4.96275256726787,12.));
#174455=CARTESIAN_POINT('Ctrl Pts',(71.0747561260443,4.96831978772202,0.));
#174456=CARTESIAN_POINT('Ctrl Pts',(71.0747561260443,4.96831978772202,12.));
#174457=CARTESIAN_POINT('Ctrl Pts',(71.0529489935959,4.97385367675158,0.));
#174458=CARTESIAN_POINT('Ctrl Pts',(71.0529489935959,4.97385367675158,12.));
#174459=CARTESIAN_POINT('Ctrl Pts',(71.031180929482,4.97935426748578,0.));
#174460=CARTESIAN_POINT('Ctrl Pts',(71.031180929482,4.97935426748578,12.));
#174461=CARTESIAN_POINT('Ctrl Pts',(71.0094520872375,4.98482159331852,0.));
#174462=CARTESIAN_POINT('Ctrl Pts',(71.0094520872375,4.98482159331852,12.));
#174463=CARTESIAN_POINT('Ctrl Pts',(70.9877626211112,4.99025568790653,0.));
#174464=CARTESIAN_POINT('Ctrl Pts',(70.9877626211112,4.99025568790653,12.));
#174465=CARTESIAN_POINT('Ctrl Pts',(70.9661126860773,4.99565658516906,0.));
#174466=CARTESIAN_POINT('Ctrl Pts',(70.9661126860773,4.99565658516906,12.));
#174467=CARTESIAN_POINT('Ctrl Pts',(70.9445024378439,5.0010243192904,0.));
#174468=CARTESIAN_POINT('Ctrl Pts',(70.9445024378439,5.0010243192904,12.));
#174469=CARTESIAN_POINT('Ctrl Pts',(70.9229320328588,5.00635892472518,0.));
#174470=CARTESIAN_POINT('Ctrl Pts',(70.9229320328588,5.00635892472518,12.));
#174471=CARTESIAN_POINT('Ctrl Pts',(70.9014016283123,5.01166043620574,0.));
#174472=CARTESIAN_POINT('Ctrl Pts',(70.9014016283123,5.01166043620574,12.));
#174473=CARTESIAN_POINT('Ctrl Pts',(70.8799113821449,5.01692888873793,0.));
#174474=CARTESIAN_POINT('Ctrl Pts',(70.8799113821449,5.01692888873793,12.));
#174475=CARTESIAN_POINT('Ctrl Pts',(70.8584614530517,5.02216431760061,0.));
#174476=CARTESIAN_POINT('Ctrl Pts',(70.8584614530517,5.02216431760061,12.));
#174477=CARTESIAN_POINT('Ctrl Pts',(70.8370520004844,5.02736675834692,0.));
#174478=CARTESIAN_POINT('Ctrl Pts',(70.8370520004844,5.02736675834692,12.));
#174479=CARTESIAN_POINT('Ctrl Pts',(70.8156831846493,5.03253624680941,0.));
#174480=CARTESIAN_POINT('Ctrl Pts',(70.8156831846493,5.03253624680941,12.));
#174481=CARTESIAN_POINT('Ctrl Pts',(70.7943551665071,5.03767281910484,0.));
#174482=CARTESIAN_POINT('Ctrl Pts',(70.7943551665071,5.03767281910484,12.));
#174483=CARTESIAN_POINT('Ctrl Pts',(70.7730681077997,5.04277651163357,0.));
#174484=CARTESIAN_POINT('Ctrl Pts',(70.7730681077997,5.04277651163357,12.));
#174485=CARTESIAN_POINT('Ctrl Pts',(70.7518221710715,5.04784736108351,0.));
#174486=CARTESIAN_POINT('Ctrl Pts',(70.7518221710715,5.04784736108351,12.));
#174487=CARTESIAN_POINT('Ctrl Pts',(70.7306175196856,5.05288540443478,0.));
#174488=CARTESIAN_POINT('Ctrl Pts',(70.7306175196856,5.05288540443478,12.));
#174489=CARTESIAN_POINT('Ctrl Pts',(70.7094543178416,5.05789067897041,0.));
#174490=CARTESIAN_POINT('Ctrl Pts',(70.7094543178416,5.05789067897041,12.));
#174491=CARTESIAN_POINT('Ctrl Pts',(70.6883327305755,5.06286322227797,0.));
#174492=CARTESIAN_POINT('Ctrl Pts',(70.6883327305755,5.06286322227797,12.));
#174493=CARTESIAN_POINT('Ctrl Pts',(70.6672529237431,5.06780307224053,0.));
#174494=CARTESIAN_POINT('Ctrl Pts',(70.6672529237431,5.06780307224053,12.));
#174495=CARTESIAN_POINT('Ctrl Pts',(70.6462150640009,5.07271026703351,0.));
#174496=CARTESIAN_POINT('Ctrl Pts',(70.6462150640009,5.07271026703351,12.));
#174497=CARTESIAN_POINT('Ctrl Pts',(70.6252193187892,5.07758484512311,0.));
#174498=CARTESIAN_POINT('Ctrl Pts',(70.6252193187892,5.07758484512311,12.));
#174499=CARTESIAN_POINT('Ctrl Pts',(70.6042658562951,5.08242684526704,0.));
#174500=CARTESIAN_POINT('Ctrl Pts',(70.6042658562951,5.08242684526704,12.));
#174501=CARTESIAN_POINT('Ctrl Pts',(70.5833548455043,5.08723630652291,0.));
#174502=CARTESIAN_POINT('Ctrl Pts',(70.5833548455043,5.08723630652291,12.));
#174503=CARTESIAN_POINT('Ctrl Pts',(70.5624864562841,5.09201326826146,0.));
#174504=CARTESIAN_POINT('Ctrl Pts',(70.5624864562841,5.09201326826146,12.));
#174505=CARTESIAN_POINT('Ctrl Pts',(70.5416608594526,5.09675777018183,0.));
#174506=CARTESIAN_POINT('Ctrl Pts',(70.5416608594526,5.09675777018183,12.));
#174507=CARTESIAN_POINT('Ctrl Pts',(70.5208782268482,5.10146985232929,0.));
#174508=CARTESIAN_POINT('Ctrl Pts',(70.5208782268482,5.10146985232929,12.));
#174509=CARTESIAN_POINT('Ctrl Pts',(70.5001387313963,5.10614955511643,0.));
#174510=CARTESIAN_POINT('Ctrl Pts',(70.5001387313963,5.10614955511643,12.));
#174511=CARTESIAN_POINT('Ctrl Pts',(70.4794425469799,5.11079691929193,0.));
#174512=CARTESIAN_POINT('Ctrl Pts',(70.4794425469799,5.11079691929193,12.));
#174513=CARTESIAN_POINT('Ctrl Pts',(70.4587898482946,5.1154119859092,0.));
#174514=CARTESIAN_POINT('Ctrl Pts',(70.4587898482946,5.1154119859092,12.));
#174515=CARTESIAN_POINT('Ctrl Pts',(70.438180810725,5.11999479630215,0.));
#174516=CARTESIAN_POINT('Ctrl Pts',(70.438180810725,5.11999479630215,12.));
#174517=CARTESIAN_POINT('Ctrl Pts',(70.4176156101633,5.12454539205347,0.));
#174518=CARTESIAN_POINT('Ctrl Pts',(70.4176156101633,5.12454539205347,12.));
#174519=CARTESIAN_POINT('Ctrl Pts',(70.3970944229885,5.12906381499486,0.));
#174520=CARTESIAN_POINT('Ctrl Pts',(70.3970944229885,5.12906381499486,12.));
#174521=CARTESIAN_POINT('Ctrl Pts',(70.3766174264786,5.13355010728591,0.));
#174522=CARTESIAN_POINT('Ctrl Pts',(70.3766174264786,5.13355010728591,12.));
#174523=CARTESIAN_POINT('Ctrl Pts',(70.3561847991725,5.13800431148911,0.));
#174524=CARTESIAN_POINT('Ctrl Pts',(70.3561847991725,5.13800431148911,12.));
#174525=CARTESIAN_POINT('Ctrl Pts',(70.3357967211782,5.14242647063468,0.));
#174526=CARTESIAN_POINT('Ctrl Pts',(70.3357967211782,5.14242647063468,12.));
#174527=CARTESIAN_POINT('Ctrl Pts',(70.31545337467,5.14681662833054,0.));
#174528=CARTESIAN_POINT('Ctrl Pts',(70.31545337467,5.14681662833054,12.));
#174529=CARTESIAN_POINT('Ctrl Pts',(70.2951549435469,5.15117482869225,0.));
#174530=CARTESIAN_POINT('Ctrl Pts',(70.2951549435469,5.15117482869225,12.));
#174531=CARTESIAN_POINT('Ctrl Pts',(70.2749016125073,5.15550111614838,0.));
#174532=CARTESIAN_POINT('Ctrl Pts',(70.2749016125073,5.15550111614838,12.));
#174533=CARTESIAN_POINT('Ctrl Pts',(70.2546935662719,5.15979553528201,0.));
#174534=CARTESIAN_POINT('Ctrl Pts',(70.2546935662719,5.15979553528201,12.));
#174535=CARTESIAN_POINT('Ctrl Pts',(70.2345309887864,5.16405813066995,0.));
#174536=CARTESIAN_POINT('Ctrl Pts',(70.2345309887864,5.16405813066995,12.));
#174537=CARTESIAN_POINT('Ctrl Pts',(70.2144140623004,5.1682889467014,0.));
#174538=CARTESIAN_POINT('Ctrl Pts',(70.2144140623004,5.1682889467014,12.));
#174539=CARTESIAN_POINT('Ctrl Pts',(70.1943429691214,5.1724880279342,0.));
#174540=CARTESIAN_POINT('Ctrl Pts',(70.1943429691214,5.1724880279342,12.));
#174541=CARTESIAN_POINT('Ctrl Pts',(70.1743178937102,5.176655419524,0.));
#174542=CARTESIAN_POINT('Ctrl Pts',(70.1743178937102,5.176655419524,12.));
#174543=CARTESIAN_POINT('Ctrl Pts',(70.1543390243882,5.18079116757659,0.));
#174544=CARTESIAN_POINT('Ctrl Pts',(70.1543390243882,5.18079116757659,12.));
#174545=CARTESIAN_POINT('Ctrl Pts',(70.1344065558106,5.18489531966235,0.));
#174546=CARTESIAN_POINT('Ctrl Pts',(70.1344065558106,5.18489531966235,12.));
#174547=CARTESIAN_POINT('Ctrl Pts',(70.1145206891833,5.18896792486523,0.));
#174548=CARTESIAN_POINT('Ctrl Pts',(70.1145206891833,5.18896792486523,12.));
#174549=CARTESIAN_POINT('Ctrl Pts',(70.0946816270957,5.19300903271544,0.));
#174550=CARTESIAN_POINT('Ctrl Pts',(70.0946816270957,5.19300903271544,12.));
#174551=CARTESIAN_POINT('Ctrl Pts',(70.0748895689716,5.19701869225515,0.));
#174552=CARTESIAN_POINT('Ctrl Pts',(70.0748895689716,5.19701869225515,12.));
#174553=CARTESIAN_POINT('Ctrl Pts',(70.0551447071106,5.20099695122678,0.));
#174554=CARTESIAN_POINT('Ctrl Pts',(70.0551447071106,5.20099695122678,12.));
#174555=CARTESIAN_POINT('Ctrl Pts',(70.0354472203604,5.20494385478084,0.));
#174556=CARTESIAN_POINT('Ctrl Pts',(70.0354472203604,5.20494385478084,12.));
#174557=CARTESIAN_POINT('Ctrl Pts',(70.0157972802255,5.20885944672915,0.));
#174558=CARTESIAN_POINT('Ctrl Pts',(70.0157972802255,5.20885944672915,12.));
#174559=CARTESIAN_POINT('Ctrl Pts',(69.996195063002,5.21274377203322,0.));
#174560=CARTESIAN_POINT('Ctrl Pts',(69.996195063002,5.21274377203322,12.));
#174561=CARTESIAN_POINT('Ctrl Pts',(69.9766407595385,5.21659687881139,0.));
#174562=CARTESIAN_POINT('Ctrl Pts',(69.9766407595385,5.21659687881139,12.));
#174563=CARTESIAN_POINT('Ctrl Pts',(69.9571345869996,5.22041882075627,0.));
#174564=CARTESIAN_POINT('Ctrl Pts',(69.9571345869996,5.22041882075627,12.));
#174565=CARTESIAN_POINT('Ctrl Pts',(69.9376767968951,5.22420965879808,0.));
#174566=CARTESIAN_POINT('Ctrl Pts',(69.9376767968951,5.22420965879808,12.));
#174567=CARTESIAN_POINT('Ctrl Pts',(69.9182676501892,5.22796945602603,0.));
#174568=CARTESIAN_POINT('Ctrl Pts',(69.9182676501892,5.22796945602603,12.));
#174569=CARTESIAN_POINT('Ctrl Pts',(69.8989073936606,5.23169827290452,0.));
#174570=CARTESIAN_POINT('Ctrl Pts',(69.8989073936606,5.23169827290452,12.));
#174571=CARTESIAN_POINT('Ctrl Pts',(69.8795962381676,5.23539616279715,0.));
#174572=CARTESIAN_POINT('Ctrl Pts',(69.8795962381676,5.23539616279715,12.));
#174573=CARTESIAN_POINT('Ctrl Pts',(69.8603343303016,5.23906316635141,0.));
#174574=CARTESIAN_POINT('Ctrl Pts',(69.8603343303016,5.23906316635141,12.));
#174575=CARTESIAN_POINT('Ctrl Pts',(69.8411217507931,5.24269931055076,0.));
#174576=CARTESIAN_POINT('Ctrl Pts',(69.8411217507931,5.24269931055076,12.));
#174577=CARTESIAN_POINT('Ctrl Pts',(69.8257911792542,5.24558355160221,0.));
#174578=CARTESIAN_POINT('Ctrl Pts',(69.8257911792542,5.24558355160221,12.));
#174579=CARTESIAN_POINT('Ctrl Pts',(69.8143154684447,5.24773285666674,0.));
#174580=CARTESIAN_POINT('Ctrl Pts',(69.8143154684447,5.24773285666674,12.));
#174581=CARTESIAN_POINT('Ctrl Pts',(69.8066748687863,5.24915955997537,0.));
#174582=CARTESIAN_POINT('Ctrl Pts',(69.8066748687863,5.24915955997537,12.));
#174583=CARTESIAN_POINT('Ctrl Pts',(69.8028570375097,5.24987136994592,0.));
#174584=CARTESIAN_POINT('Ctrl Pts',(69.8028570375097,5.24987136994592,12.));
#174585=CARTESIAN_POINT('Ctrl Pts',(69.8028570375097,5.24987136994592,12.));
#174586=CARTESIAN_POINT('Ctrl Pts',(69.8066748687863,5.24915955997537,12.));
#174587=CARTESIAN_POINT('Ctrl Pts',(69.8143154684447,5.24773285666674,12.));
#174588=CARTESIAN_POINT('Ctrl Pts',(69.8257911792542,5.24558355160221,12.));
#174589=CARTESIAN_POINT('Ctrl Pts',(69.8411217507931,5.24269931055076,12.));
#174590=CARTESIAN_POINT('Ctrl Pts',(69.8603343303016,5.23906316635141,12.));
#174591=CARTESIAN_POINT('Ctrl Pts',(69.8795962381676,5.23539616279715,12.));
#174592=CARTESIAN_POINT('Ctrl Pts',(69.8989073936606,5.23169827290452,12.));
#174593=CARTESIAN_POINT('Ctrl Pts',(69.9182676501892,5.22796945602603,12.));
#174594=CARTESIAN_POINT('Ctrl Pts',(69.9376767968951,5.22420965879808,12.));
#174595=CARTESIAN_POINT('Ctrl Pts',(69.9571345869996,5.22041882075627,12.));
#174596=CARTESIAN_POINT('Ctrl Pts',(69.9766407595385,5.21659687881139,12.));
#174597=CARTESIAN_POINT('Ctrl Pts',(69.996195063002,5.21274377203322,12.));
#174598=CARTESIAN_POINT('Ctrl Pts',(70.0157972802255,5.20885944672915,12.));
#174599=CARTESIAN_POINT('Ctrl Pts',(70.0354472203604,5.20494385478084,12.));
#174600=CARTESIAN_POINT('Ctrl Pts',(70.0551447071106,5.20099695122678,12.));
#174601=CARTESIAN_POINT('Ctrl Pts',(70.0748895689716,5.19701869225515,12.));
#174602=CARTESIAN_POINT('Ctrl Pts',(70.0946816270957,5.19300903271544,12.));
#174603=CARTESIAN_POINT('Ctrl Pts',(70.1145206891833,5.18896792486523,12.));
#174604=CARTESIAN_POINT('Ctrl Pts',(70.1344065558106,5.18489531966235,12.));
#174605=CARTESIAN_POINT('Ctrl Pts',(70.1543390243882,5.18079116757659,12.));
#174606=CARTESIAN_POINT('Ctrl Pts',(70.1743178937102,5.176655419524,12.));
#174607=CARTESIAN_POINT('Ctrl Pts',(70.1943429691214,5.1724880279342,12.));
#174608=CARTESIAN_POINT('Ctrl Pts',(70.2144140623004,5.1682889467014,12.));
#174609=CARTESIAN_POINT('Ctrl Pts',(70.2345309887864,5.16405813066995,12.));
#174610=CARTESIAN_POINT('Ctrl Pts',(70.2546935662719,5.15979553528201,12.));
#174611=CARTESIAN_POINT('Ctrl Pts',(70.2749016125073,5.15550111614838,12.));
#174612=CARTESIAN_POINT('Ctrl Pts',(70.2951549435469,5.15117482869225,12.));
#174613=CARTESIAN_POINT('Ctrl Pts',(70.31545337467,5.14681662833054,12.));
#174614=CARTESIAN_POINT('Ctrl Pts',(70.3357967211782,5.14242647063468,12.));
#174615=CARTESIAN_POINT('Ctrl Pts',(70.3561847991725,5.13800431148911,12.));
#174616=CARTESIAN_POINT('Ctrl Pts',(70.3766174264786,5.13355010728591,12.));
#174617=CARTESIAN_POINT('Ctrl Pts',(70.3970944229885,5.12906381499486,12.));
#174618=CARTESIAN_POINT('Ctrl Pts',(70.4176156101633,5.12454539205347,12.));
#174619=CARTESIAN_POINT('Ctrl Pts',(70.438180810725,5.11999479630215,12.));
#174620=CARTESIAN_POINT('Ctrl Pts',(70.4587898482946,5.1154119859092,12.));
#174621=CARTESIAN_POINT('Ctrl Pts',(70.4794425469799,5.11079691929193,12.));
#174622=CARTESIAN_POINT('Ctrl Pts',(70.5001387313963,5.10614955511643,12.));
#174623=CARTESIAN_POINT('Ctrl Pts',(70.5208782268482,5.10146985232929,12.));
#174624=CARTESIAN_POINT('Ctrl Pts',(70.5416608594526,5.09675777018183,12.));
#174625=CARTESIAN_POINT('Ctrl Pts',(70.5624864562841,5.09201326826146,12.));
#174626=CARTESIAN_POINT('Ctrl Pts',(70.5833548455043,5.08723630652291,12.));
#174627=CARTESIAN_POINT('Ctrl Pts',(70.6042658562951,5.08242684526704,12.));
#174628=CARTESIAN_POINT('Ctrl Pts',(70.6252193187892,5.07758484512311,12.));
#174629=CARTESIAN_POINT('Ctrl Pts',(70.6462150640009,5.07271026703351,12.));
#174630=CARTESIAN_POINT('Ctrl Pts',(70.6672529237431,5.06780307224053,12.));
#174631=CARTESIAN_POINT('Ctrl Pts',(70.6883327305755,5.06286322227797,12.));
#174632=CARTESIAN_POINT('Ctrl Pts',(70.7094543178416,5.05789067897041,12.));
#174633=CARTESIAN_POINT('Ctrl Pts',(70.7306175196856,5.05288540443478,12.));
#174634=CARTESIAN_POINT('Ctrl Pts',(70.7518221710715,5.04784736108351,12.));
#174635=CARTESIAN_POINT('Ctrl Pts',(70.7730681077997,5.04277651163357,12.));
#174636=CARTESIAN_POINT('Ctrl Pts',(70.7943551665071,5.03767281910484,12.));
#174637=CARTESIAN_POINT('Ctrl Pts',(70.8156831846493,5.03253624680941,12.));
#174638=CARTESIAN_POINT('Ctrl Pts',(70.8370520004844,5.02736675834692,12.));
#174639=CARTESIAN_POINT('Ctrl Pts',(70.8584614530517,5.02216431760061,12.));
#174640=CARTESIAN_POINT('Ctrl Pts',(70.8799113821449,5.01692888873793,12.));
#174641=CARTESIAN_POINT('Ctrl Pts',(70.9014016283123,5.01166043620574,12.));
#174642=CARTESIAN_POINT('Ctrl Pts',(70.9229320328588,5.00635892472518,12.));
#174643=CARTESIAN_POINT('Ctrl Pts',(70.9445024378439,5.0010243192904,12.));
#174644=CARTESIAN_POINT('Ctrl Pts',(70.9661126860773,4.99565658516906,12.));
#174645=CARTESIAN_POINT('Ctrl Pts',(70.9877626211112,4.99025568790653,12.));
#174646=CARTESIAN_POINT('Ctrl Pts',(71.0094520872375,4.98482159331852,12.));
#174647=CARTESIAN_POINT('Ctrl Pts',(71.031180929482,4.97935426748578,12.));
#174648=CARTESIAN_POINT('Ctrl Pts',(71.0529489935959,4.97385367675158,12.));
#174649=CARTESIAN_POINT('Ctrl Pts',(71.0747561260443,4.96831978772202,12.));
#174650=CARTESIAN_POINT('Ctrl Pts',(71.0966021739922,4.96275256726787,12.));
#174651=CARTESIAN_POINT('Ctrl Pts',(71.1184869853071,4.95715198251704,12.));
#174652=CARTESIAN_POINT('Ctrl Pts',(71.1404104085561,4.95151800085111,12.));
#174653=CARTESIAN_POINT('Ctrl Pts',(71.1623722929998,4.94585058990337,12.));
#174654=CARTESIAN_POINT('Ctrl Pts',(71.184372488583,4.94014971756097,12.));
#174655=CARTESIAN_POINT('Ctrl Pts',(71.206410845926,4.93441535196594,12.));
#174656=CARTESIAN_POINT('Ctrl Pts',(71.2284872163248,4.92864746150711,12.));
#174657=CARTESIAN_POINT('Ctrl Pts',(71.2506014517457,4.92284601481711,12.));
#174658=CARTESIAN_POINT('Ctrl Pts',(71.27275340482,4.91701098077042,12.));
#174659=CARTESIAN_POINT('Ctrl Pts',(71.2949429288319,4.91114232848623,12.));
#174660=CARTESIAN_POINT('Ctrl Pts',(71.3171698777124,4.90524002732806,12.));
#174661=CARTESIAN_POINT('Ctrl Pts',(71.3394341060396,4.899304046896,12.));
#174662=CARTESIAN_POINT('Ctrl Pts',(71.3617354690342,4.89333435702424,12.));
#174663=CARTESIAN_POINT('Ctrl Pts',(71.3840738225547,4.88733092777965,12.));
#174664=CARTESIAN_POINT('Ctrl Pts',(71.4064490230857,4.88129372946525,12.));
#174665=CARTESIAN_POINT('Ctrl Pts',(71.4288609277324,4.87522273261881,12.));
#174666=CARTESIAN_POINT('Ctrl Pts',(71.4513093942216,4.86911790800534,12.));
#174667=CARTESIAN_POINT('Ctrl Pts',(71.4737942808971,4.86297922661499,12.));
#174668=CARTESIAN_POINT('Ctrl Pts',(71.4963154467128,4.85680665966185,12.));
#174669=CARTESIAN_POINT('Ctrl Pts',(71.5188727512231,4.85060017858787,12.));
#174670=CARTESIAN_POINT('Ctrl Pts',(71.5414660545778,4.84435975506057,12.));
#174671=CARTESIAN_POINT('Ctrl Pts',(71.5640952175239,4.8380853609659,12.));
#174672=CARTESIAN_POINT('Ctrl Pts',(71.5867601014008,4.83177696840641,12.));
#174673=CARTESIAN_POINT('Ctrl Pts',(71.6094605681353,4.82543454970021,12.));
#174674=CARTESIAN_POINT('Ctrl Pts',(71.6321964802297,4.81905807738542,12.));
#174675=CARTESIAN_POINT('Ctrl Pts',(71.6549677007582,4.81264752421714,12.));
#174676=CARTESIAN_POINT('Ctrl Pts',(71.6777740933687,4.80620286316076,12.));
#174677=CARTESIAN_POINT('Ctrl Pts',(71.7006155222764,4.79972406739011,12.));
#174678=CARTESIAN_POINT('Ctrl Pts',(71.723491852261,4.79321111028676,12.));
#174679=CARTESIAN_POINT('Ctrl Pts',(71.7464029486563,4.78666396544459,12.));
#174680=CARTESIAN_POINT('Ctrl Pts',(71.769348677346,4.78008260666651,12.));
#174681=CARTESIAN_POINT('Ctrl Pts',(71.7923289047643,4.77346700795792,12.));
#174682=CARTESIAN_POINT('Ctrl Pts',(71.8153434978923,4.76681714352503,12.));
#174683=CARTESIAN_POINT('Ctrl Pts',(71.8383923242531,4.7601329877742,12.));
#174684=CARTESIAN_POINT('Ctrl Pts',(71.8614752519008,4.7534145153167,12.));
#174685=CARTESIAN_POINT('Ctrl Pts',(71.8845921494189,4.74666170096548,12.));
#174686=CARTESIAN_POINT('Ctrl Pts',(71.9077428859212,4.73987451972864,12.));
#174687=CARTESIAN_POINT('Ctrl Pts',(71.9309273310471,4.73305294680786,12.));
#174688=CARTESIAN_POINT('Ctrl Pts',(71.9541453549579,4.72619695759774,12.));
#174689=CARTESIAN_POINT('Ctrl Pts',(71.9773968283259,4.71930652769071,12.));
#174690=CARTESIAN_POINT('Ctrl Pts',(72.0006816223325,4.71238163287397,12.));
#174691=CARTESIAN_POINT('Ctrl Pts',(72.0239996086686,4.70542224912301,12.));
#174692=CARTESIAN_POINT('Ctrl Pts',(72.0473506595318,4.69842835259993,12.));
#174693=CARTESIAN_POINT('Ctrl Pts',(72.0707346476213,4.69139991965284,12.));
#174694=CARTESIAN_POINT('Ctrl Pts',(72.0941514461287,4.68433692682069,12.));
#174695=CARTESIAN_POINT('Ctrl Pts',(72.1176009287351,4.67723935083095,12.));
#174696=CARTESIAN_POINT('Ctrl Pts',(72.1410829696128,4.67010716859286,12.));
#174697=CARTESIAN_POINT('Ctrl Pts',(72.1645974434216,4.6629403571957,12.));
#174698=CARTESIAN_POINT('Ctrl Pts',(72.1881442253053,4.65573889390823,12.));
#174699=CARTESIAN_POINT('Ctrl Pts',(72.2117231908822,4.64850275618324,12.));
#174700=CARTESIAN_POINT('Ctrl Pts',(72.2353342162417,4.64123192165628,12.));
#174701=CARTESIAN_POINT('Ctrl Pts',(72.2589771779456,4.63392636813844,12.));
#174702=CARTESIAN_POINT('Ctrl Pts',(72.2826519530259,4.62658607361466,12.));
#174703=CARTESIAN_POINT('Ctrl Pts',(72.3063584189807,4.61921101624292,12.));
#174704=CARTESIAN_POINT('Ctrl Pts',(72.3300964537658,4.61180117435863,12.));
#174705=CARTESIAN_POINT('Ctrl Pts',(72.3538659357913,4.60435652647454,12.));
#174706=CARTESIAN_POINT('Ctrl Pts',(72.3776667439227,4.5968770512733,12.));
#174707=CARTESIAN_POINT('Ctrl Pts',(72.401498757478,4.58936272760545,12.));
#174708=CARTESIAN_POINT('Ctrl Pts',(72.4253618562252,4.58181353448852,12.));
#174709=CARTESIAN_POINT('Ctrl Pts',(72.4492559203745,4.57422945111103,12.));
#174710=CARTESIAN_POINT('Ctrl Pts',(72.4731808305728,4.56661045683376,12.));
#174711=CARTESIAN_POINT('Ctrl Pts',(72.4971364679068,4.55895653118221,12.));
#174712=CARTESIAN_POINT('Ctrl Pts',(72.5211227139001,4.55126765384405,12.));
#174713=CARTESIAN_POINT('Ctrl Pts',(72.5451394505103,4.54354380466823,12.));
#174714=CARTESIAN_POINT('Ctrl Pts',(72.5691865601223,4.535784963668,12.));
#174715=CARTESIAN_POINT('Ctrl Pts',(72.5932639255409,4.52799111102392,12.));
#174716=CARTESIAN_POINT('Ctrl Pts',(72.6173714299942,4.52016222707638,12.));
#174717=CARTESIAN_POINT('Ctrl Pts',(72.6415089571321,4.51229829232264,12.));
#174718=CARTESIAN_POINT('Ctrl Pts',(72.6656763910241,4.50439928741604,12.));
#174719=CARTESIAN_POINT('Ctrl Pts',(72.6898736161542,4.49646519316813,12.));
#174720=CARTESIAN_POINT('Ctrl Pts',(72.714100517414,4.48849599055338,12.));
#174721=CARTESIAN_POINT('Ctrl Pts',(72.738356980103,4.48049166070206,12.));
#174722=CARTESIAN_POINT('Ctrl Pts',(72.7626428899281,4.4724521848961,12.));
#174723=CARTESIAN_POINT('Ctrl Pts',(72.7869581329994,4.46437754456793,12.));
#174724=CARTESIAN_POINT('Ctrl Pts',(72.8113025958262,4.45626772130147,12.));
#174725=CARTESIAN_POINT('Ctrl Pts',(72.8356761653069,4.44812269683738,12.));
#174726=CARTESIAN_POINT('Ctrl Pts',(72.8600787287318,4.43994245306819,12.));
#174727=CARTESIAN_POINT('Ctrl Pts',(72.8845101737855,4.4317269720335,12.));
#174728=CARTESIAN_POINT('Ctrl Pts',(72.9089703885462,4.42347623591942,12.));
#174729=CARTESIAN_POINT('Ctrl Pts',(72.9334592614829,4.41519022705922,12.));
#174730=CARTESIAN_POINT('Ctrl Pts',(72.95797668145,4.40686892793958,12.));
#174731=CARTESIAN_POINT('Ctrl Pts',(72.9825225376846,4.39851232119723,12.));
#174732=CARTESIAN_POINT('Ctrl Pts',(73.007096719804,4.3901203896114,12.));
#174733=CARTESIAN_POINT('Ctrl Pts',(73.0316991177993,4.38169311610151,12.));
#174734=CARTESIAN_POINT('Ctrl Pts',(73.0563296220299,4.37323048372608,12.));
#174735=CARTESIAN_POINT('Ctrl Pts',(73.0809881232103,4.36473247568642,12.));
#174736=CARTESIAN_POINT('Ctrl Pts',(73.1056745124087,4.3561990753272,12.));
#174737=CARTESIAN_POINT('Ctrl Pts',(73.130388681059,4.34763026613158,12.));
#174738=CARTESIAN_POINT('Ctrl Pts',(73.1551305209685,4.33902603172141,12.));
#174739=CARTESIAN_POINT('Ctrl Pts',(73.1798999243235,4.33038635585877,12.));
#174740=CARTESIAN_POINT('Ctrl Pts',(73.204696783694,4.32171122245214,12.));
#174741=CARTESIAN_POINT('Ctrl Pts',(73.2295209920334,4.31300061556098,12.));
#174742=CARTESIAN_POINT('Ctrl Pts',(73.2543724426577,4.30425451938231,12.));
#174743=CARTESIAN_POINT('Ctrl Pts',(73.2792510292253,4.29547291824287,12.));
#174744=CARTESIAN_POINT('Ctrl Pts',(73.3041566457135,4.28665579659302,12.));
#174745=CARTESIAN_POINT('Ctrl Pts',(73.3290891863949,4.2778031390039,12.));
#174746=CARTESIAN_POINT('Ctrl Pts',(73.3540485458065,4.268914930167,12.));
#174747=CARTESIAN_POINT('Ctrl Pts',(73.3790346187938,4.259991154899,12.));
#174748=CARTESIAN_POINT('Ctrl Pts',(73.4040473005592,4.25103179814887,12.));
#174749=CARTESIAN_POINT('Ctrl Pts',(73.4290864867101,4.24203684500939,12.));
#174750=CARTESIAN_POINT('Ctrl Pts',(73.4541520732948,4.23300628072759,12.));
#174751=CARTESIAN_POINT('Ctrl Pts',(73.4792439568633,4.22394009072757,12.));
#174752=CARTESIAN_POINT('Ctrl Pts',(73.5043620344116,4.21483826059441,12.));
#174753=CARTESIAN_POINT('Ctrl Pts',(73.5295062032628,4.2057007760373,12.));
#174754=CARTESIAN_POINT('Ctrl Pts',(73.5546763609572,4.19652762286128,12.));
#174755=CARTESIAN_POINT('Ctrl Pts',(73.5798724051519,4.18731878694237,12.));
#174756=CARTESIAN_POINT('Ctrl Pts',(73.6050942334768,4.17807425419813,12.));
#174757=CARTESIAN_POINT('Ctrl Pts',(73.6303417435251,4.16879401058781,12.));
#174758=CARTESIAN_POINT('Ctrl Pts',(73.6556148331489,4.15947804217784,12.));
#174759=CARTESIAN_POINT('Ctrl Pts',(73.6809134006897,4.15012633519724,12.));
#174760=CARTESIAN_POINT('Ctrl Pts',(73.7062373452342,4.14073887610154,12.));
#174761=CARTESIAN_POINT('Ctrl Pts',(73.7315865668522,4.13131565163579,12.));
#174762=CARTESIAN_POINT('Ctrl Pts',(73.7569609668528,4.12185664890557,12.));
#174763=CARTESIAN_POINT('Ctrl Pts',(73.7823604472159,4.11236185522788,12.));
#174764=CARTESIAN_POINT('Ctrl Pts',(73.8077849100342,4.1028312579873,12.));
#174765=CARTESIAN_POINT('Ctrl Pts',(73.8332342568989,4.09326484448233,12.));
#174766=CARTESIAN_POINT('Ctrl Pts',(73.8587083884191,4.08366260180675,12.));
#174767=CARTESIAN_POINT('Ctrl Pts',(73.8842072034008,4.07402451665245,12.));
#174768=CARTESIAN_POINT('Ctrl Pts',(73.9097305995115,4.06435057547325,12.));
#174769=CARTESIAN_POINT('Ctrl Pts',(73.9352784747608,4.05464076484752,12.));
#174770=CARTESIAN_POINT('Ctrl Pts',(73.9608507287909,4.04489507179958,12.));
#174771=CARTESIAN_POINT('Ctrl Pts',(73.9864472641033,4.0351134841066,12.));
#174772=CARTESIAN_POINT('Ctrl Pts',(74.012067987646,4.02529599070095,12.));
#174773=CARTESIAN_POINT('Ctrl Pts',(74.0377128111863,4.01544258176711,12.));
#174774=CARTESIAN_POINT('Ctrl Pts',(74.059715978211,4.00696550627364,12.));
#174775=CARTESIAN_POINT('Ctrl Pts',(74.0765982943677,4.00044689711983,12.));
#174776=CARTESIAN_POINT('Ctrl Pts',(74.0883491449955,3.9959026674699,12.));
#174777=CARTESIAN_POINT('Ctrl Pts',(74.094961539962,3.99334334445527,12.));
#174778=CARTESIAN_POINT('Ctrl Pts',(74.0964320766208,3.9927740649087,12.));
#174779=CARTESIAN_POINT('Ctrl Pts',(74.0964320766207,3.99277406490872,0.));
#174780=CARTESIAN_POINT('Ctrl Pts',(74.0949615399619,3.99334334445528,0.));
#174781=CARTESIAN_POINT('Ctrl Pts',(74.0883491449955,3.99590266746991,0.));
#174782=CARTESIAN_POINT('Ctrl Pts',(74.0765982943677,4.00044689711983,0.));
#174783=CARTESIAN_POINT('Ctrl Pts',(74.0597159782109,4.00696550627365,0.));
#174784=CARTESIAN_POINT('Ctrl Pts',(74.0377128111863,4.01544258176711,0.));
#174785=CARTESIAN_POINT('Ctrl Pts',(74.012067987646,4.02529599070095,0.));
#174786=CARTESIAN_POINT('Ctrl Pts',(73.9864472641033,4.0351134841066,0.));
#174787=CARTESIAN_POINT('Ctrl Pts',(73.9608507287909,4.04489507179958,0.));
#174788=CARTESIAN_POINT('Ctrl Pts',(73.9352784747608,4.05464076484752,0.));
#174789=CARTESIAN_POINT('Ctrl Pts',(73.9097305995115,4.06435057547325,0.));
#174790=CARTESIAN_POINT('Ctrl Pts',(73.8842072034008,4.07402451665245,0.));
#174791=CARTESIAN_POINT('Ctrl Pts',(73.8587083884191,4.08366260180675,0.));
#174792=CARTESIAN_POINT('Ctrl Pts',(73.8332342568989,4.09326484448233,0.));
#174793=CARTESIAN_POINT('Ctrl Pts',(73.8077849100342,4.1028312579873,0.));
#174794=CARTESIAN_POINT('Ctrl Pts',(73.7823604472159,4.11236185522788,0.));
#174795=CARTESIAN_POINT('Ctrl Pts',(73.7569609668528,4.12185664890557,0.));
#174796=CARTESIAN_POINT('Ctrl Pts',(73.7315865668522,4.13131565163579,0.));
#174797=CARTESIAN_POINT('Ctrl Pts',(73.7062373452342,4.14073887610154,0.));
#174798=CARTESIAN_POINT('Ctrl Pts',(73.6809134006897,4.15012633519724,0.));
#174799=CARTESIAN_POINT('Ctrl Pts',(73.6556148331489,4.15947804217784,0.));
#174800=CARTESIAN_POINT('Ctrl Pts',(73.6303417435251,4.16879401058781,0.));
#174801=CARTESIAN_POINT('Ctrl Pts',(73.6050942334768,4.17807425419813,0.));
#174802=CARTESIAN_POINT('Ctrl Pts',(73.5798724051519,4.18731878694237,0.));
#174803=CARTESIAN_POINT('Ctrl Pts',(73.5546763609572,4.19652762286128,0.));
#174804=CARTESIAN_POINT('Ctrl Pts',(73.5295062032628,4.2057007760373,0.));
#174805=CARTESIAN_POINT('Ctrl Pts',(73.5043620344116,4.21483826059441,0.));
#174806=CARTESIAN_POINT('Ctrl Pts',(73.4792439568633,4.22394009072757,0.));
#174807=CARTESIAN_POINT('Ctrl Pts',(73.4541520732948,4.23300628072759,0.));
#174808=CARTESIAN_POINT('Ctrl Pts',(73.4290864867101,4.24203684500939,0.));
#174809=CARTESIAN_POINT('Ctrl Pts',(73.4040473005592,4.25103179814887,0.));
#174810=CARTESIAN_POINT('Ctrl Pts',(73.3790346187938,4.259991154899,0.));
#174811=CARTESIAN_POINT('Ctrl Pts',(73.3540485458065,4.268914930167,0.));
#174812=CARTESIAN_POINT('Ctrl Pts',(73.3290891863949,4.2778031390039,0.));
#174813=CARTESIAN_POINT('Ctrl Pts',(73.3041566457135,4.28665579659302,0.));
#174814=CARTESIAN_POINT('Ctrl Pts',(73.2792510292253,4.29547291824287,0.));
#174815=CARTESIAN_POINT('Ctrl Pts',(73.2543724426577,4.30425451938231,0.));
#174816=CARTESIAN_POINT('Ctrl Pts',(73.2295209920334,4.31300061556098,0.));
#174817=CARTESIAN_POINT('Ctrl Pts',(73.204696783694,4.32171122245214,0.));
#174818=CARTESIAN_POINT('Ctrl Pts',(73.1798999243235,4.33038635585877,0.));
#174819=CARTESIAN_POINT('Ctrl Pts',(73.1551305209685,4.33902603172141,0.));
#174820=CARTESIAN_POINT('Ctrl Pts',(73.130388681059,4.34763026613158,0.));
#174821=CARTESIAN_POINT('Ctrl Pts',(73.1056745124087,4.3561990753272,0.));
#174822=CARTESIAN_POINT('Ctrl Pts',(73.0809881232103,4.36473247568642,0.));
#174823=CARTESIAN_POINT('Ctrl Pts',(73.0563296220299,4.37323048372608,0.));
#174824=CARTESIAN_POINT('Ctrl Pts',(73.0316991177993,4.38169311610151,0.));
#174825=CARTESIAN_POINT('Ctrl Pts',(73.007096719804,4.3901203896114,0.));
#174826=CARTESIAN_POINT('Ctrl Pts',(72.9825225376846,4.39851232119723,0.));
#174827=CARTESIAN_POINT('Ctrl Pts',(72.95797668145,4.40686892793958,0.));
#174828=CARTESIAN_POINT('Ctrl Pts',(72.9334592614829,4.41519022705922,0.));
#174829=CARTESIAN_POINT('Ctrl Pts',(72.9089703885462,4.42347623591942,0.));
#174830=CARTESIAN_POINT('Ctrl Pts',(72.8845101737855,4.4317269720335,0.));
#174831=CARTESIAN_POINT('Ctrl Pts',(72.8600787287318,4.43994245306819,0.));
#174832=CARTESIAN_POINT('Ctrl Pts',(72.8356761653069,4.44812269683738,0.));
#174833=CARTESIAN_POINT('Ctrl Pts',(72.8113025958262,4.45626772130147,0.));
#174834=CARTESIAN_POINT('Ctrl Pts',(72.7869581329994,4.46437754456793,0.));
#174835=CARTESIAN_POINT('Ctrl Pts',(72.7626428899281,4.4724521848961,0.));
#174836=CARTESIAN_POINT('Ctrl Pts',(72.738356980103,4.48049166070206,0.));
#174837=CARTESIAN_POINT('Ctrl Pts',(72.714100517414,4.48849599055338,0.));
#174838=CARTESIAN_POINT('Ctrl Pts',(72.6898736161542,4.49646519316813,0.));
#174839=CARTESIAN_POINT('Ctrl Pts',(72.6656763910241,4.50439928741604,0.));
#174840=CARTESIAN_POINT('Ctrl Pts',(72.6415089571321,4.51229829232264,0.));
#174841=CARTESIAN_POINT('Ctrl Pts',(72.6173714299942,4.52016222707638,0.));
#174842=CARTESIAN_POINT('Ctrl Pts',(72.5932639255409,4.52799111102392,0.));
#174843=CARTESIAN_POINT('Ctrl Pts',(72.5691865601223,4.535784963668,0.));
#174844=CARTESIAN_POINT('Ctrl Pts',(72.5451394505103,4.54354380466823,0.));
#174845=CARTESIAN_POINT('Ctrl Pts',(72.5211227139001,4.55126765384405,0.));
#174846=CARTESIAN_POINT('Ctrl Pts',(72.4971364679068,4.55895653118221,0.));
#174847=CARTESIAN_POINT('Ctrl Pts',(72.4731808305728,4.56661045683376,0.));
#174848=CARTESIAN_POINT('Ctrl Pts',(72.4492559203745,4.57422945111103,0.));
#174849=CARTESIAN_POINT('Ctrl Pts',(72.4253618562252,4.58181353448852,0.));
#174850=CARTESIAN_POINT('Ctrl Pts',(72.401498757478,4.58936272760545,0.));
#174851=CARTESIAN_POINT('Ctrl Pts',(72.3776667439227,4.5968770512733,0.));
#174852=CARTESIAN_POINT('Ctrl Pts',(72.3538659357913,4.60435652647454,0.));
#174853=CARTESIAN_POINT('Ctrl Pts',(72.3300964537658,4.61180117435863,0.));
#174854=CARTESIAN_POINT('Ctrl Pts',(72.3063584189807,4.61921101624292,0.));
#174855=CARTESIAN_POINT('Ctrl Pts',(72.2826519530259,4.62658607361466,0.));
#174856=CARTESIAN_POINT('Ctrl Pts',(72.2589771779456,4.63392636813844,0.));
#174857=CARTESIAN_POINT('Ctrl Pts',(72.2353342162417,4.64123192165628,0.));
#174858=CARTESIAN_POINT('Ctrl Pts',(72.2117231908822,4.64850275618324,0.));
#174859=CARTESIAN_POINT('Ctrl Pts',(72.1881442253053,4.65573889390823,0.));
#174860=CARTESIAN_POINT('Ctrl Pts',(72.1645974434216,4.6629403571957,0.));
#174861=CARTESIAN_POINT('Ctrl Pts',(72.1410829696128,4.67010716859286,0.));
#174862=CARTESIAN_POINT('Ctrl Pts',(72.1176009287351,4.67723935083095,0.));
#174863=CARTESIAN_POINT('Ctrl Pts',(72.0941514461287,4.68433692682069,0.));
#174864=CARTESIAN_POINT('Ctrl Pts',(72.0707346476213,4.69139991965284,0.));
#174865=CARTESIAN_POINT('Ctrl Pts',(72.0473506595318,4.69842835259993,0.));
#174866=CARTESIAN_POINT('Ctrl Pts',(72.0239996086686,4.70542224912301,0.));
#174867=CARTESIAN_POINT('Ctrl Pts',(72.0006816223325,4.71238163287397,0.));
#174868=CARTESIAN_POINT('Ctrl Pts',(71.9773968283259,4.71930652769071,0.));
#174869=CARTESIAN_POINT('Ctrl Pts',(71.9541453549579,4.72619695759774,0.));
#174870=CARTESIAN_POINT('Ctrl Pts',(71.9309273310471,4.73305294680786,0.));
#174871=CARTESIAN_POINT('Ctrl Pts',(71.9077428859212,4.73987451972864,0.));
#174872=CARTESIAN_POINT('Ctrl Pts',(71.8845921494189,4.74666170096548,0.));
#174873=CARTESIAN_POINT('Ctrl Pts',(71.8614752519008,4.7534145153167,0.));
#174874=CARTESIAN_POINT('Ctrl Pts',(71.8383923242531,4.7601329877742,0.));
#174875=CARTESIAN_POINT('Ctrl Pts',(71.8153434978923,4.76681714352503,0.));
#174876=CARTESIAN_POINT('Ctrl Pts',(71.7923289047643,4.77346700795792,0.));
#174877=CARTESIAN_POINT('Ctrl Pts',(71.769348677346,4.78008260666651,0.));
#174878=CARTESIAN_POINT('Ctrl Pts',(71.7464029486563,4.78666396544459,0.));
#174879=CARTESIAN_POINT('Ctrl Pts',(71.723491852261,4.79321111028676,0.));
#174880=CARTESIAN_POINT('Ctrl Pts',(71.7006155222764,4.79972406739011,0.));
#174881=CARTESIAN_POINT('Ctrl Pts',(71.6777740933687,4.80620286316076,0.));
#174882=CARTESIAN_POINT('Ctrl Pts',(71.6549677007582,4.81264752421714,0.));
#174883=CARTESIAN_POINT('Ctrl Pts',(71.6321964802297,4.81905807738542,0.));
#174884=CARTESIAN_POINT('Ctrl Pts',(71.6094605681353,4.82543454970021,0.));
#174885=CARTESIAN_POINT('Ctrl Pts',(71.5867601014008,4.83177696840641,0.));
#174886=CARTESIAN_POINT('Ctrl Pts',(71.5640952175239,4.8380853609659,0.));
#174887=CARTESIAN_POINT('Ctrl Pts',(71.5414660545778,4.84435975506057,0.));
#174888=CARTESIAN_POINT('Ctrl Pts',(71.5188727512231,4.85060017858787,0.));
#174889=CARTESIAN_POINT('Ctrl Pts',(71.4963154467128,4.85680665966185,0.));
#174890=CARTESIAN_POINT('Ctrl Pts',(71.4737942808971,4.86297922661499,0.));
#174891=CARTESIAN_POINT('Ctrl Pts',(71.4513093942216,4.86911790800534,0.));
#174892=CARTESIAN_POINT('Ctrl Pts',(71.4288609277324,4.87522273261881,0.));
#174893=CARTESIAN_POINT('Ctrl Pts',(71.4064490230857,4.88129372946525,0.));
#174894=CARTESIAN_POINT('Ctrl Pts',(71.3840738225547,4.88733092777965,0.));
#174895=CARTESIAN_POINT('Ctrl Pts',(71.3617354690342,4.89333435702424,0.));
#174896=CARTESIAN_POINT('Ctrl Pts',(71.3394341060396,4.899304046896,0.));
#174897=CARTESIAN_POINT('Ctrl Pts',(71.3171698777124,4.90524002732806,0.));
#174898=CARTESIAN_POINT('Ctrl Pts',(71.2949429288319,4.91114232848623,0.));
#174899=CARTESIAN_POINT('Ctrl Pts',(71.27275340482,4.91701098077042,0.));
#174900=CARTESIAN_POINT('Ctrl Pts',(71.2506014517457,4.92284601481711,0.));
#174901=CARTESIAN_POINT('Ctrl Pts',(71.2284872163248,4.92864746150711,0.));
#174902=CARTESIAN_POINT('Ctrl Pts',(71.206410845926,4.93441535196594,0.));
#174903=CARTESIAN_POINT('Ctrl Pts',(71.184372488583,4.94014971756097,0.));
#174904=CARTESIAN_POINT('Ctrl Pts',(71.1623722929998,4.94585058990337,0.));
#174905=CARTESIAN_POINT('Ctrl Pts',(71.1404104085561,4.95151800085111,0.));
#174906=CARTESIAN_POINT('Ctrl Pts',(71.1184869853071,4.95715198251704,0.));
#174907=CARTESIAN_POINT('Ctrl Pts',(71.0966021739922,4.96275256726787,0.));
#174908=CARTESIAN_POINT('Ctrl Pts',(71.0747561260443,4.96831978772202,0.));
#174909=CARTESIAN_POINT('Ctrl Pts',(71.0529489935959,4.97385367675158,0.));
#174910=CARTESIAN_POINT('Ctrl Pts',(71.031180929482,4.97935426748578,0.));
#174911=CARTESIAN_POINT('Ctrl Pts',(71.0094520872375,4.98482159331852,0.));
#174912=CARTESIAN_POINT('Ctrl Pts',(70.9877626211112,4.99025568790653,0.));
#174913=CARTESIAN_POINT('Ctrl Pts',(70.9661126860773,4.99565658516906,0.));
#174914=CARTESIAN_POINT('Ctrl Pts',(70.9445024378439,5.0010243192904,0.));
#174915=CARTESIAN_POINT('Ctrl Pts',(70.9229320328588,5.00635892472518,0.));
#174916=CARTESIAN_POINT('Ctrl Pts',(70.9014016283123,5.01166043620574,0.));
#174917=CARTESIAN_POINT('Ctrl Pts',(70.8799113821449,5.01692888873793,0.));
#174918=CARTESIAN_POINT('Ctrl Pts',(70.8584614530517,5.02216431760061,0.));
#174919=CARTESIAN_POINT('Ctrl Pts',(70.8370520004844,5.02736675834692,0.));
#174920=CARTESIAN_POINT('Ctrl Pts',(70.8156831846493,5.03253624680941,0.));
#174921=CARTESIAN_POINT('Ctrl Pts',(70.7943551665071,5.03767281910484,0.));
#174922=CARTESIAN_POINT('Ctrl Pts',(70.7730681077997,5.04277651163357,0.));
#174923=CARTESIAN_POINT('Ctrl Pts',(70.7518221710715,5.04784736108351,0.));
#174924=CARTESIAN_POINT('Ctrl Pts',(70.7306175196856,5.05288540443478,0.));
#174925=CARTESIAN_POINT('Ctrl Pts',(70.7094543178416,5.05789067897041,0.));
#174926=CARTESIAN_POINT('Ctrl Pts',(70.6883327305755,5.06286322227797,0.));
#174927=CARTESIAN_POINT('Ctrl Pts',(70.6672529237431,5.06780307224053,0.));
#174928=CARTESIAN_POINT('Ctrl Pts',(70.6462150640009,5.07271026703351,0.));
#174929=CARTESIAN_POINT('Ctrl Pts',(70.6252193187892,5.07758484512311,0.));
#174930=CARTESIAN_POINT('Ctrl Pts',(70.6042658562951,5.08242684526704,0.));
#174931=CARTESIAN_POINT('Ctrl Pts',(70.5833548455043,5.08723630652291,0.));
#174932=CARTESIAN_POINT('Ctrl Pts',(70.5624864562841,5.09201326826146,0.));
#174933=CARTESIAN_POINT('Ctrl Pts',(70.5416608594526,5.09675777018183,0.));
#174934=CARTESIAN_POINT('Ctrl Pts',(70.5208782268482,5.10146985232929,0.));
#174935=CARTESIAN_POINT('Ctrl Pts',(70.5001387313963,5.10614955511643,0.));
#174936=CARTESIAN_POINT('Ctrl Pts',(70.4794425469799,5.11079691929193,0.));
#174937=CARTESIAN_POINT('Ctrl Pts',(70.4587898482946,5.1154119859092,0.));
#174938=CARTESIAN_POINT('Ctrl Pts',(70.438180810725,5.11999479630215,0.));
#174939=CARTESIAN_POINT('Ctrl Pts',(70.4176156101633,5.12454539205347,0.));
#174940=CARTESIAN_POINT('Ctrl Pts',(70.3970944229885,5.12906381499486,0.));
#174941=CARTESIAN_POINT('Ctrl Pts',(70.3766174264786,5.13355010728591,0.));
#174942=CARTESIAN_POINT('Ctrl Pts',(70.3561847991725,5.13800431148911,0.));
#174943=CARTESIAN_POINT('Ctrl Pts',(70.3357967211782,5.14242647063468,0.));
#174944=CARTESIAN_POINT('Ctrl Pts',(70.31545337467,5.14681662833054,0.));
#174945=CARTESIAN_POINT('Ctrl Pts',(70.2951549435469,5.15117482869225,0.));
#174946=CARTESIAN_POINT('Ctrl Pts',(70.2749016125073,5.15550111614838,0.));
#174947=CARTESIAN_POINT('Ctrl Pts',(70.2546935662719,5.15979553528201,0.));
#174948=CARTESIAN_POINT('Ctrl Pts',(70.2345309887864,5.16405813066995,0.));
#174949=CARTESIAN_POINT('Ctrl Pts',(70.2144140623004,5.1682889467014,0.));
#174950=CARTESIAN_POINT('Ctrl Pts',(70.1943429691214,5.1724880279342,0.));
#174951=CARTESIAN_POINT('Ctrl Pts',(70.1743178937102,5.176655419524,0.));
#174952=CARTESIAN_POINT('Ctrl Pts',(70.1543390243882,5.18079116757659,0.));
#174953=CARTESIAN_POINT('Ctrl Pts',(70.1344065558106,5.18489531966235,0.));
#174954=CARTESIAN_POINT('Ctrl Pts',(70.1145206891833,5.18896792486523,0.));
#174955=CARTESIAN_POINT('Ctrl Pts',(70.0946816270957,5.19300903271544,0.));
#174956=CARTESIAN_POINT('Ctrl Pts',(70.0748895689716,5.19701869225515,0.));
#174957=CARTESIAN_POINT('Ctrl Pts',(70.0551447071106,5.20099695122678,0.));
#174958=CARTESIAN_POINT('Ctrl Pts',(70.0354472203604,5.20494385478084,0.));
#174959=CARTESIAN_POINT('Ctrl Pts',(70.0157972802255,5.20885944672915,0.));
#174960=CARTESIAN_POINT('Ctrl Pts',(69.996195063002,5.21274377203322,0.));
#174961=CARTESIAN_POINT('Ctrl Pts',(69.9766407595385,5.21659687881139,0.));
#174962=CARTESIAN_POINT('Ctrl Pts',(69.9571345869996,5.22041882075627,0.));
#174963=CARTESIAN_POINT('Ctrl Pts',(69.9376767968951,5.22420965879808,0.));
#174964=CARTESIAN_POINT('Ctrl Pts',(69.9182676501892,5.22796945602603,0.));
#174965=CARTESIAN_POINT('Ctrl Pts',(69.8989073936606,5.23169827290452,0.));
#174966=CARTESIAN_POINT('Ctrl Pts',(69.8795962381676,5.23539616279715,0.));
#174967=CARTESIAN_POINT('Ctrl Pts',(69.8603343303016,5.23906316635141,0.));
#174968=CARTESIAN_POINT('Ctrl Pts',(69.8411217507931,5.24269931055076,0.));
#174969=CARTESIAN_POINT('Ctrl Pts',(69.8257911792542,5.24558355160221,0.));
#174970=CARTESIAN_POINT('Ctrl Pts',(69.8143154684447,5.24773285666674,0.));
#174971=CARTESIAN_POINT('Ctrl Pts',(69.8066748687863,5.24915955997537,0.));
#174972=CARTESIAN_POINT('Ctrl Pts',(69.8028570375097,5.24987136994592,0.));
#174973=CARTESIAN_POINT('Origin',(0.,0.,12.));
#174974=CARTESIAN_POINT('',(-90.,-1.10218211923262E-14,12.));
#174975=CARTESIAN_POINT('Origin',(0.,0.,12.));
#174976=CARTESIAN_POINT('Origin',(0.,0.,12.));
#174977=CARTESIAN_POINT('Origin',(0.,0.,0.));
#174978=CARTESIAN_POINT('Origin',(0.,0.,0.));
#174979=CARTESIAN_POINT('Origin',(0.,0.,0.));
#174980=CARTESIAN_POINT('',(-90.,-1.10218211923262E-14,0.));
#174981=CARTESIAN_POINT('',(-90.,-1.10218211923262E-14,0.));
#174982=CARTESIAN_POINT('',(-90.,-1.10218211923262E-14,0.));
#174983=CARTESIAN_POINT('Origin',(0.,0.,0.));
#174984=CARTESIAN_POINT('Origin',(0.,0.,0.));
#259186=UNCERTAINTY_MEASURE_WITH_UNIT(LENGTH_MEASURE(0.01),#259225,
'DISTANCE_ACCURACY_VALUE',
'Maximum model space distance between geometric entities at asserted c
onnectivities');
#259202=UNCERTAINTY_MEASURE_WITH_UNIT(LENGTH_MEASURE(0.01),#259225,
'DISTANCE_ACCURACY_VALUE',
'Maximum model space distance between geometric entities at asserted c
onnectivities');
#259208=(
GEOMETRIC_REPRESENTATION_CONTEXT(3)
GLOBAL_UNCERTAINTY_ASSIGNED_CONTEXT((#259186))
GLOBAL_UNIT_ASSIGNED_CONTEXT((#259225,#259227,#259228))
REPRESENTATION_CONTEXT('','3D')
);
#259224=(
GEOMETRIC_REPRESENTATION_CONTEXT(3)
GLOBAL_UNCERTAINTY_ASSIGNED_CONTEXT((#259202))
GLOBAL_UNIT_ASSIGNED_CONTEXT((#259225,#259227,#259228))
REPRESENTATION_CONTEXT('','3D')
);
#259225=(
LENGTH_UNIT()
NAMED_UNIT(*)
SI_UNIT(.MILLI.,.METRE.)
);
#259227=(
NAMED_UNIT(*)
PLANE_ANGLE_UNIT()
SI_UNIT($,.RADIAN.)
);
#259228=(
NAMED_UNIT(*)
SI_UNIT($,.STERADIAN.)
SOLID_ANGLE_UNIT()
);
#259234=SHAPE_DEFINITION_REPRESENTATION(#259255,#259374);
#259255=PRODUCT_DEFINITION_SHAPE('',$,#259396);
#259374=SHAPE_REPRESENTATION('',(#25864),#259208);
#259390=PRODUCT_DEFINITION_CONTEXT('part definition',#259455,'design');
#259396=PRODUCT_DEFINITION('Ring gear','Ring gear',#259417,#259390);
#259417=PRODUCT_DEFINITION_FORMATION('',$,#259462);
#259455=APPLICATION_CONTEXT(
'Core Data for Automotive Mechanical Design Process');
#259456=PRODUCT_CONTEXT('part definition',#259455,'mechanical');
#259462=PRODUCT('Ring gear','Ring gear',
'{"standard_geometry": "Unshifted20degree involute", "teeth": 72, "mod
ule_mm": 2, "pitch_diameter_mm": 144.0, "root_diameter_mm": 149.0, "ti
p_diameter_mm": 140.0, "face_mm": 12, "per_gear_circular_tooth_thinnin
g_mm": 0.1, "derived_root_fillet_mm": 0.5, "involute_fit_points_per_fl
ank": 41, "internal": true, "source_stock": "Native reusable Gear blan
k; assembly-specific machining", "manufacturing_scope": "Standard prof
ile reference; grade, cutter/root transition validation, tolerances, b
acklash and load rating require production selection."}',(#259456));
#259483=PRESENTATION_STYLE_ASSIGNMENT((#259498));
#259498=SURFACE_STYLE_USAGE(.BOTH.,#259513);
#259513=SURFACE_SIDE_STYLE('',(#259528));
#259528=SURFACE_STYLE_FILL_AREA(#259543);
#259543=FILL_AREA_STYLE('Ring dark blue',(#259558));
#259558=FILL_AREA_STYLE_COLOUR('Ring dark blue',#259573);
#259573=COLOUR_RGB('Ring dark blue',0.0901960784313725,0.270588235294118,
0.513725490196078);
ENDSEC;
END-ISO-10303-21;
